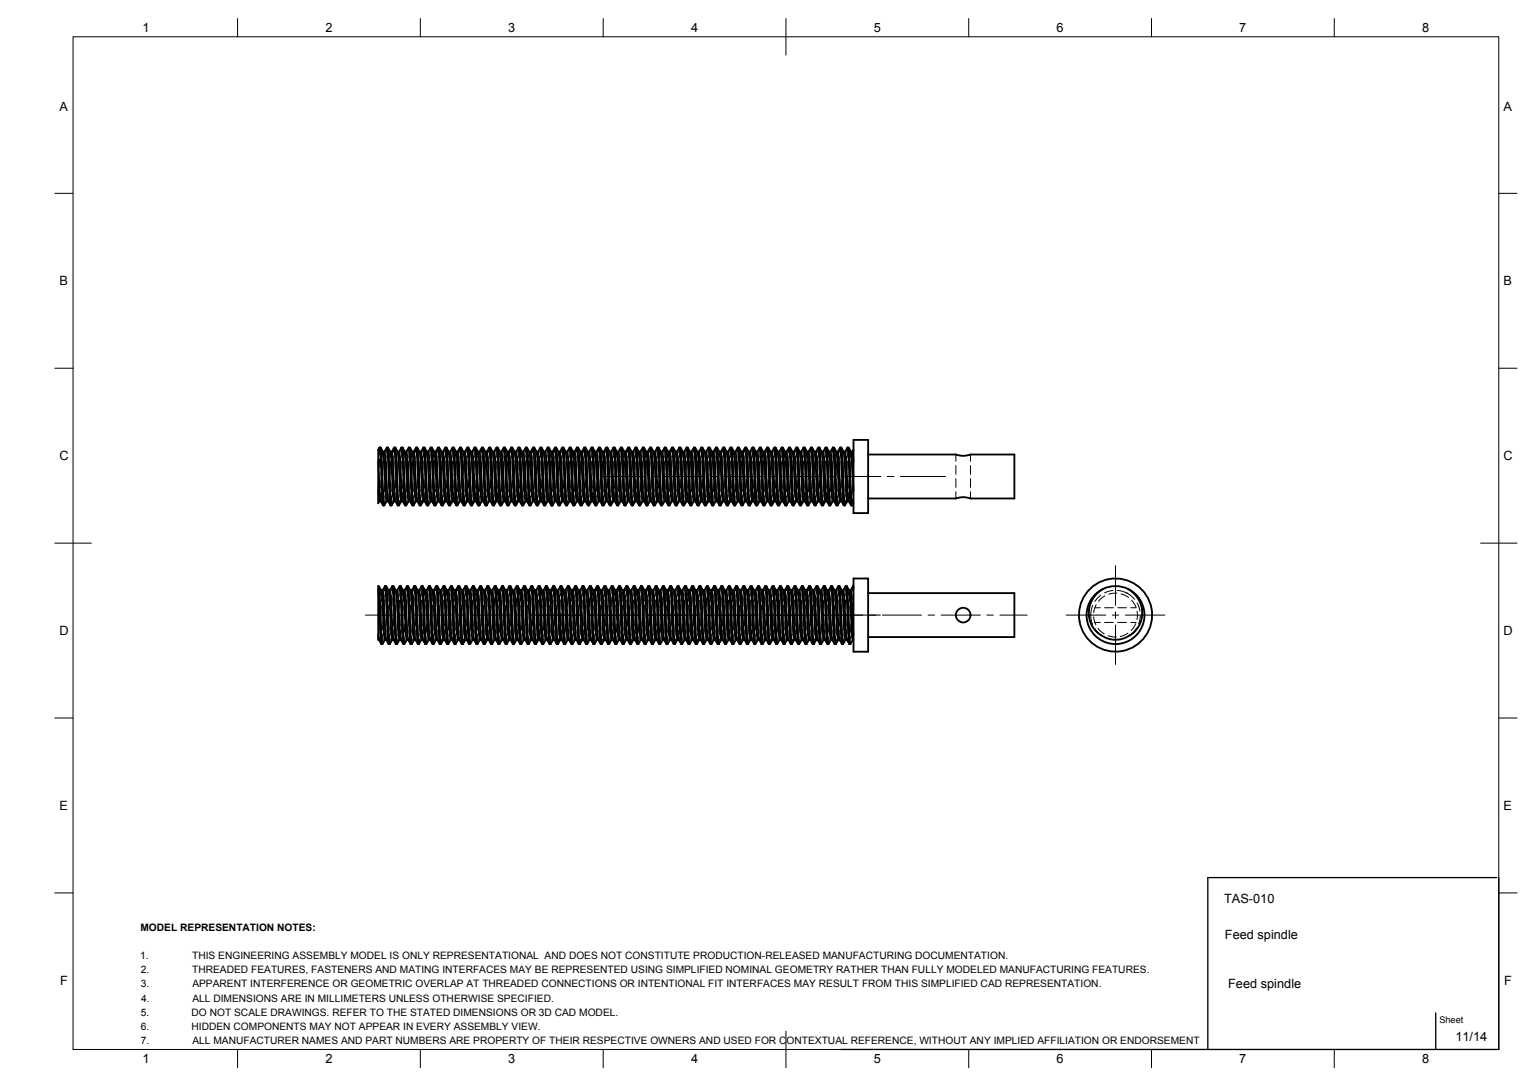
ISO-10303-21;
HEADER;
/* Generated by software containing ST-Developer
 * from STEP Tools, Inc. (www.steptools.com) 
 */

FILE_DESCRIPTION(
/* description */ (
'Independent keyed-quill tailstock, native coupled50mm slider andM16x2
 feed screw, conical dead center, bronze sleeves/thrust washers, cross
-pinned handwheel and bolted guide key. Custom center taper; no standa
rd taper compatibility, machine-bed compatibility or load rating assig
ned.'),
/* implementation_level */ '2;1');

FILE_NAME(
/* name */ 'Feed spindle.step',
/* time_stamp */ '2026-11-14T07:17:36-08:00',
/* author */ (''),
/* organization */ (''),
/* preprocessor_version */ 'ST-DEVELOPER v20.2',
/* originating_system */ 'Autodesk Translation Framework v15.17.0.0',
/* authorisation */ '');

FILE_SCHEMA (('AUTOMOTIVE_DESIGN { 1 0 10303 214 3 1 1 }'));
ENDSEC;

DATA;
#10=MECHANICAL_DESIGN_GEOMETRIC_PRESENTATION_REPRESENTATION('',(#161),#289387);
#127=SHAPE_REPRESENTATION_RELATIONSHIP('SRR','None',#289462,#144);
#144=ADVANCED_BREP_SHAPE_REPRESENTATION('',(#178),#289378);
#161=STYLED_ITEM('',(#289548),#178);
#178=MANIFOLD_SOLID_BREP('Body1',#16849);
#240=FACE_BOUND('',#1641,.T.);
#241=FACE_BOUND('',#1644,.T.);
#242=FACE_BOUND('',#1646,.T.);
#295=B_SPLINE_SURFACE_WITH_KNOTS('',3,3,((#241865,#241866,#241867,#241868,
#241869,#241870,#241871,#241872,#241873,#241874,#241875,#241876,#241877,
#241878,#241879,#241880,#241881,#241882,#241883,#241884,#241885,#241886,
#241887,#241888,#241889,#241890,#241891,#241892,#241893,#241894,#241895,
#241896,#241897,#241898,#241899,#241900,#241901,#241902,#241903,#241904,
#241905,#241906,#241907,#241908,#241909,#241910,#241911,#241912,#241913,
#241914,#241915,#241916,#241917,#241918,#241919,#241920,#241921,#241922,
#241923,#241924,#241925,#241926,#241927,#241928,#241929,#241930,#241931,
#241932,#241933,#241934,#241935,#241936,#241937,#241938,#241939,#241940,
#241941,#241942,#241943,#241944,#241945,#241946,#241947,#241948,#241949,
#241950,#241951,#241952,#241953,#241954,#241955,#241956,#241957,#241958,
#241959,#241960,#241961,#241962,#241963,#241964,#241965,#241966,#241967,
#241968,#241969,#241970,#241971,#241972,#241973,#241974,#241975,#241976,
#241977,#241978,#241979,#241980,#241981,#241982,#241983,#241984,#241985,
#241986,#241987,#241988,#241989,#241990,#241991,#241992,#241993,#241994,
#241995,#241996,#241997,#241998,#241999,#242000,#242001,#242002,#242003,
#242004,#242005,#242006,#242007,#242008,#242009,#242010,#242011,#242012,
#242013,#242014,#242015,#242016,#242017,#242018,#242019,#242020,#242021,
#242022,#242023,#242024,#242025,#242026,#242027,#242028,#242029,#242030,
#242031,#242032,#242033,#242034,#242035,#242036,#242037,#242038,#242039,
#242040,#242041,#242042,#242043,#242044,#242045,#242046,#242047,#242048,
#242049,#242050,#242051,#242052,#242053,#242054,#242055,#242056,#242057,
#242058,#242059,#242060,#242061,#242062,#242063,#242064,#242065,#242066,
#242067,#242068,#242069,#242070,#242071,#242072,#242073,#242074,#242075,
#242076,#242077,#242078,#242079,#242080,#242081,#242082,#242083,#242084,
#242085,#242086,#242087,#242088,#242089,#242090,#242091,#242092,#242093,
#242094,#242095,#242096,#242097,#242098,#242099,#242100,#242101,#242102,
#242103,#242104,#242105,#242106,#242107,#242108,#242109,#242110,#242111,
#242112,#242113,#242114,#242115,#242116,#242117,#242118,#242119,#242120,
#242121,#242122,#242123,#242124,#242125,#242126,#242127,#242128,#242129,
#242130,#242131,#242132,#242133,#242134,#242135,#242136,#242137,#242138,
#242139,#242140,#242141,#242142,#242143,#242144,#242145,#242146,#242147,
#242148,#242149,#242150,#242151,#242152,#242153,#242154,#242155,#242156,
#242157,#242158,#242159,#242160,#242161,#242162,#242163,#242164,#242165,
#242166,#242167,#242168,#242169,#242170,#242171,#242172,#242173,#242174,
#242175,#242176,#242177,#242178,#242179,#242180,#242181,#242182,#242183,
#242184,#242185,#242186,#242187,#242188,#242189,#242190,#242191,#242192,
#242193,#242194,#242195,#242196,#242197,#242198,#242199,#242200,#242201,
#242202,#242203,#242204,#242205,#242206,#242207,#242208,#242209,#242210,
#242211,#242212,#242213,#242214,#242215,#242216,#242217,#242218,#242219,
#242220,#242221,#242222,#242223,#242224,#242225,#242226,#242227,#242228,
#242229,#242230,#242231,#242232,#242233,#242234,#242235,#242236,#242237,
#242238,#242239,#242240,#242241,#242242,#242243,#242244,#242245,#242246,
#242247,#242248,#242249,#242250,#242251,#242252,#242253,#242254,#242255,
#242256,#242257,#242258,#242259,#242260,#242261,#242262,#242263,#242264,
#242265,#242266,#242267,#242268,#242269,#242270,#242271,#242272,#242273,
#242274,#242275,#242276,#242277,#242278,#242279,#242280,#242281,#242282,
#242283,#242284,#242285,#242286,#242287,#242288,#242289,#242290,#242291,
#242292,#242293,#242294,#242295,#242296,#242297,#242298,#242299,#242300,
#242301,#242302,#242303,#242304,#242305,#242306,#242307,#242308,#242309,
#242310,#242311,#242312,#242313,#242314,#242315,#242316,#242317,#242318,
#242319,#242320,#242321,#242322,#242323,#242324,#242325,#242326,#242327,
#242328,#242329,#242330,#242331,#242332,#242333,#242334,#242335,#242336,
#242337,#242338,#242339,#242340,#242341,#242342,#242343,#242344,#242345,
#242346,#242347,#242348,#242349,#242350,#242351,#242352,#242353,#242354,
#242355,#242356,#242357,#242358,#242359,#242360,#242361,#242362,#242363,
#242364,#242365,#242366,#242367,#242368,#242369,#242370,#242371,#242372,
#242373,#242374,#242375,#242376,#242377,#242378,#242379,#242380,#242381,
#242382,#242383,#242384,#242385,#242386,#242387,#242388,#242389,#242390,
#242391,#242392,#242393,#242394,#242395,#242396,#242397,#242398,#242399,
#242400,#242401,#242402,#242403,#242404,#242405,#242406,#242407,#242408,
#242409,#242410,#242411,#242412,#242413,#242414,#242415,#242416,#242417,
#242418,#242419,#242420,#242421,#242422,#242423,#242424,#242425,#242426,
#242427,#242428,#242429,#242430,#242431,#242432,#242433,#242434,#242435,
#242436,#242437,#242438,#242439,#242440,#242441,#242442,#242443,#242444,
#242445,#242446,#242447,#242448,#242449,#242450,#242451,#242452,#242453),
(#242454,#242455,#242456,#242457,#242458,#242459,#242460,#242461,#242462,
#242463,#242464,#242465,#242466,#242467,#242468,#242469,#242470,#242471,
#242472,#242473,#242474,#242475,#242476,#242477,#242478,#242479,#242480,
#242481,#242482,#242483,#242484,#242485,#242486,#242487,#242488,#242489,
#242490,#242491,#242492,#242493,#242494,#242495,#242496,#242497,#242498,
#242499,#242500,#242501,#242502,#242503,#242504,#242505,#242506,#242507,
#242508,#242509,#242510,#242511,#242512,#242513,#242514,#242515,#242516,
#242517,#242518,#242519,#242520,#242521,#242522,#242523,#242524,#242525,
#242526,#242527,#242528,#242529,#242530,#242531,#242532,#242533,#242534,
#242535,#242536,#242537,#242538,#242539,#242540,#242541,#242542,#242543,
#242544,#242545,#242546,#242547,#242548,#242549,#242550,#242551,#242552,
#242553,#242554,#242555,#242556,#242557,#242558,#242559,#242560,#242561,
#242562,#242563,#242564,#242565,#242566,#242567,#242568,#242569,#242570,
#242571,#242572,#242573,#242574,#242575,#242576,#242577,#242578,#242579,
#242580,#242581,#242582,#242583,#242584,#242585,#242586,#242587,#242588,
#242589,#242590,#242591,#242592,#242593,#242594,#242595,#242596,#242597,
#242598,#242599,#242600,#242601,#242602,#242603,#242604,#242605,#242606,
#242607,#242608,#242609,#242610,#242611,#242612,#242613,#242614,#242615,
#242616,#242617,#242618,#242619,#242620,#242621,#242622,#242623,#242624,
#242625,#242626,#242627,#242628,#242629,#242630,#242631,#242632,#242633,
#242634,#242635,#242636,#242637,#242638,#242639,#242640,#242641,#242642,
#242643,#242644,#242645,#242646,#242647,#242648,#242649,#242650,#242651,
#242652,#242653,#242654,#242655,#242656,#242657,#242658,#242659,#242660,
#242661,#242662,#242663,#242664,#242665,#242666,#242667,#242668,#242669,
#242670,#242671,#242672,#242673,#242674,#242675,#242676,#242677,#242678,
#242679,#242680,#242681,#242682,#242683,#242684,#242685,#242686,#242687,
#242688,#242689,#242690,#242691,#242692,#242693,#242694,#242695,#242696,
#242697,#242698,#242699,#242700,#242701,#242702,#242703,#242704,#242705,
#242706,#242707,#242708,#242709,#242710,#242711,#242712,#242713,#242714,
#242715,#242716,#242717,#242718,#242719,#242720,#242721,#242722,#242723,
#242724,#242725,#242726,#242727,#242728,#242729,#242730,#242731,#242732,
#242733,#242734,#242735,#242736,#242737,#242738,#242739,#242740,#242741,
#242742,#242743,#242744,#242745,#242746,#242747,#242748,#242749,#242750,
#242751,#242752,#242753,#242754,#242755,#242756,#242757,#242758,#242759,
#242760,#242761,#242762,#242763,#242764,#242765,#242766,#242767,#242768,
#242769,#242770,#242771,#242772,#242773,#242774,#242775,#242776,#242777,
#242778,#242779,#242780,#242781,#242782,#242783,#242784,#242785,#242786,
#242787,#242788,#242789,#242790,#242791,#242792,#242793,#242794,#242795,
#242796,#242797,#242798,#242799,#242800,#242801,#242802,#242803,#242804,
#242805,#242806,#242807,#242808,#242809,#242810,#242811,#242812,#242813,
#242814,#242815,#242816,#242817,#242818,#242819,#242820,#242821,#242822,
#242823,#242824,#242825,#242826,#242827,#242828,#242829,#242830,#242831,
#242832,#242833,#242834,#242835,#242836,#242837,#242838,#242839,#242840,
#242841,#242842,#242843,#242844,#242845,#242846,#242847,#242848,#242849,
#242850,#242851,#242852,#242853,#242854,#242855,#242856,#242857,#242858,
#242859,#242860,#242861,#242862,#242863,#242864,#242865,#242866,#242867,
#242868,#242869,#242870,#242871,#242872,#242873,#242874,#242875,#242876,
#242877,#242878,#242879,#242880,#242881,#242882,#242883,#242884,#242885,
#242886,#242887,#242888,#242889,#242890,#242891,#242892,#242893,#242894,
#242895,#242896,#242897,#242898,#242899,#242900,#242901,#242902,#242903,
#242904,#242905,#242906,#242907,#242908,#242909,#242910,#242911,#242912,
#242913,#242914,#242915,#242916,#242917,#242918,#242919,#242920,#242921,
#242922,#242923,#242924,#242925,#242926,#242927,#242928,#242929,#242930,
#242931,#242932,#242933,#242934,#242935,#242936,#242937,#242938,#242939,
#242940,#242941,#242942,#242943,#242944,#242945,#242946,#242947,#242948,
#242949,#242950,#242951,#242952,#242953,#242954,#242955,#242956,#242957,
#242958,#242959,#242960,#242961,#242962,#242963,#242964,#242965,#242966,
#242967,#242968,#242969,#242970,#242971,#242972,#242973,#242974,#242975,
#242976,#242977,#242978,#242979,#242980,#242981,#242982,#242983,#242984,
#242985,#242986,#242987,#242988,#242989,#242990,#242991,#242992,#242993,
#242994,#242995,#242996,#242997,#242998,#242999,#243000,#243001,#243002,
#243003,#243004,#243005,#243006,#243007,#243008,#243009,#243010,#243011,
#243012,#243013,#243014,#243015,#243016,#243017,#243018,#243019,#243020,
#243021,#243022,#243023,#243024,#243025,#243026,#243027,#243028,#243029,
#243030,#243031,#243032,#243033,#243034,#243035,#243036,#243037,#243038,
#243039,#243040,#243041,#243042),(#243043,#243044,#243045,#243046,#243047,
#243048,#243049,#243050,#243051,#243052,#243053,#243054,#243055,#243056,
#243057,#243058,#243059,#243060,#243061,#243062,#243063,#243064,#243065,
#243066,#243067,#243068,#243069,#243070,#243071,#243072,#243073,#243074,
#243075,#243076,#243077,#243078,#243079,#243080,#243081,#243082,#243083,
#243084,#243085,#243086,#243087,#243088,#243089,#243090,#243091,#243092,
#243093,#243094,#243095,#243096,#243097,#243098,#243099,#243100,#243101,
#243102,#243103,#243104,#243105,#243106,#243107,#243108,#243109,#243110,
#243111,#243112,#243113,#243114,#243115,#243116,#243117,#243118,#243119,
#243120,#243121,#243122,#243123,#243124,#243125,#243126,#243127,#243128,
#243129,#243130,#243131,#243132,#243133,#243134,#243135,#243136,#243137,
#243138,#243139,#243140,#243141,#243142,#243143,#243144,#243145,#243146,
#243147,#243148,#243149,#243150,#243151,#243152,#243153,#243154,#243155,
#243156,#243157,#243158,#243159,#243160,#243161,#243162,#243163,#243164,
#243165,#243166,#243167,#243168,#243169,#243170,#243171,#243172,#243173,
#243174,#243175,#243176,#243177,#243178,#243179,#243180,#243181,#243182,
#243183,#243184,#243185,#243186,#243187,#243188,#243189,#243190,#243191,
#243192,#243193,#243194,#243195,#243196,#243197,#243198,#243199,#243200,
#243201,#243202,#243203,#243204,#243205,#243206,#243207,#243208,#243209,
#243210,#243211,#243212,#243213,#243214,#243215,#243216,#243217,#243218,
#243219,#243220,#243221,#243222,#243223,#243224,#243225,#243226,#243227,
#243228,#243229,#243230,#243231,#243232,#243233,#243234,#243235,#243236,
#243237,#243238,#243239,#243240,#243241,#243242,#243243,#243244,#243245,
#243246,#243247,#243248,#243249,#243250,#243251,#243252,#243253,#243254,
#243255,#243256,#243257,#243258,#243259,#243260,#243261,#243262,#243263,
#243264,#243265,#243266,#243267,#243268,#243269,#243270,#243271,#243272,
#243273,#243274,#243275,#243276,#243277,#243278,#243279,#243280,#243281,
#243282,#243283,#243284,#243285,#243286,#243287,#243288,#243289,#243290,
#243291,#243292,#243293,#243294,#243295,#243296,#243297,#243298,#243299,
#243300,#243301,#243302,#243303,#243304,#243305,#243306,#243307,#243308,
#243309,#243310,#243311,#243312,#243313,#243314,#243315,#243316,#243317,
#243318,#243319,#243320,#243321,#243322,#243323,#243324,#243325,#243326,
#243327,#243328,#243329,#243330,#243331,#243332,#243333,#243334,#243335,
#243336,#243337,#243338,#243339,#243340,#243341,#243342,#243343,#243344,
#243345,#243346,#243347,#243348,#243349,#243350,#243351,#243352,#243353,
#243354,#243355,#243356,#243357,#243358,#243359,#243360,#243361,#243362,
#243363,#243364,#243365,#243366,#243367,#243368,#243369,#243370,#243371,
#243372,#243373,#243374,#243375,#243376,#243377,#243378,#243379,#243380,
#243381,#243382,#243383,#243384,#243385,#243386,#243387,#243388,#243389,
#243390,#243391,#243392,#243393,#243394,#243395,#243396,#243397,#243398,
#243399,#243400,#243401,#243402,#243403,#243404,#243405,#243406,#243407,
#243408,#243409,#243410,#243411,#243412,#243413,#243414,#243415,#243416,
#243417,#243418,#243419,#243420,#243421,#243422,#243423,#243424,#243425,
#243426,#243427,#243428,#243429,#243430,#243431,#243432,#243433,#243434,
#243435,#243436,#243437,#243438,#243439,#243440,#243441,#243442,#243443,
#243444,#243445,#243446,#243447,#243448,#243449,#243450,#243451,#243452,
#243453,#243454,#243455,#243456,#243457,#243458,#243459,#243460,#243461,
#243462,#243463,#243464,#243465,#243466,#243467,#243468,#243469,#243470,
#243471,#243472,#243473,#243474,#243475,#243476,#243477,#243478,#243479,
#243480,#243481,#243482,#243483,#243484,#243485,#243486,#243487,#243488,
#243489,#243490,#243491,#243492,#243493,#243494,#243495,#243496,#243497,
#243498,#243499,#243500,#243501,#243502,#243503,#243504,#243505,#243506,
#243507,#243508,#243509,#243510,#243511,#243512,#243513,#243514,#243515,
#243516,#243517,#243518,#243519,#243520,#243521,#243522,#243523,#243524,
#243525,#243526,#243527,#243528,#243529,#243530,#243531,#243532,#243533,
#243534,#243535,#243536,#243537,#243538,#243539,#243540,#243541,#243542,
#243543,#243544,#243545,#243546,#243547,#243548,#243549,#243550,#243551,
#243552,#243553,#243554,#243555,#243556,#243557,#243558,#243559,#243560,
#243561,#243562,#243563,#243564,#243565,#243566,#243567,#243568,#243569,
#243570,#243571,#243572,#243573,#243574,#243575,#243576,#243577,#243578,
#243579,#243580,#243581,#243582,#243583,#243584,#243585,#243586,#243587,
#243588,#243589,#243590,#243591,#243592,#243593,#243594,#243595,#243596,
#243597,#243598,#243599,#243600,#243601,#243602,#243603,#243604,#243605,
#243606,#243607,#243608,#243609,#243610,#243611,#243612,#243613,#243614,
#243615,#243616,#243617,#243618,#243619,#243620,#243621,#243622,#243623,
#243624,#243625,#243626,#243627,#243628,#243629,#243630,#243631),(#243632,
#243633,#243634,#243635,#243636,#243637,#243638,#243639,#243640,#243641,
#243642,#243643,#243644,#243645,#243646,#243647,#243648,#243649,#243650,
#243651,#243652,#243653,#243654,#243655,#243656,#243657,#243658,#243659,
#243660,#243661,#243662,#243663,#243664,#243665,#243666,#243667,#243668,
#243669,#243670,#243671,#243672,#243673,#243674,#243675,#243676,#243677,
#243678,#243679,#243680,#243681,#243682,#243683,#243684,#243685,#243686,
#243687,#243688,#243689,#243690,#243691,#243692,#243693,#243694,#243695,
#243696,#243697,#243698,#243699,#243700,#243701,#243702,#243703,#243704,
#243705,#243706,#243707,#243708,#243709,#243710,#243711,#243712,#243713,
#243714,#243715,#243716,#243717,#243718,#243719,#243720,#243721,#243722,
#243723,#243724,#243725,#243726,#243727,#243728,#243729,#243730,#243731,
#243732,#243733,#243734,#243735,#243736,#243737,#243738,#243739,#243740,
#243741,#243742,#243743,#243744,#243745,#243746,#243747,#243748,#243749,
#243750,#243751,#243752,#243753,#243754,#243755,#243756,#243757,#243758,
#243759,#243760,#243761,#243762,#243763,#243764,#243765,#243766,#243767,
#243768,#243769,#243770,#243771,#243772,#243773,#243774,#243775,#243776,
#243777,#243778,#243779,#243780,#243781,#243782,#243783,#243784,#243785,
#243786,#243787,#243788,#243789,#243790,#243791,#243792,#243793,#243794,
#243795,#243796,#243797,#243798,#243799,#243800,#243801,#243802,#243803,
#243804,#243805,#243806,#243807,#243808,#243809,#243810,#243811,#243812,
#243813,#243814,#243815,#243816,#243817,#243818,#243819,#243820,#243821,
#243822,#243823,#243824,#243825,#243826,#243827,#243828,#243829,#243830,
#243831,#243832,#243833,#243834,#243835,#243836,#243837,#243838,#243839,
#243840,#243841,#243842,#243843,#243844,#243845,#243846,#243847,#243848,
#243849,#243850,#243851,#243852,#243853,#243854,#243855,#243856,#243857,
#243858,#243859,#243860,#243861,#243862,#243863,#243864,#243865,#243866,
#243867,#243868,#243869,#243870,#243871,#243872,#243873,#243874,#243875,
#243876,#243877,#243878,#243879,#243880,#243881,#243882,#243883,#243884,
#243885,#243886,#243887,#243888,#243889,#243890,#243891,#243892,#243893,
#243894,#243895,#243896,#243897,#243898,#243899,#243900,#243901,#243902,
#243903,#243904,#243905,#243906,#243907,#243908,#243909,#243910,#243911,
#243912,#243913,#243914,#243915,#243916,#243917,#243918,#243919,#243920,
#243921,#243922,#243923,#243924,#243925,#243926,#243927,#243928,#243929,
#243930,#243931,#243932,#243933,#243934,#243935,#243936,#243937,#243938,
#243939,#243940,#243941,#243942,#243943,#243944,#243945,#243946,#243947,
#243948,#243949,#243950,#243951,#243952,#243953,#243954,#243955,#243956,
#243957,#243958,#243959,#243960,#243961,#243962,#243963,#243964,#243965,
#243966,#243967,#243968,#243969,#243970,#243971,#243972,#243973,#243974,
#243975,#243976,#243977,#243978,#243979,#243980,#243981,#243982,#243983,
#243984,#243985,#243986,#243987,#243988,#243989,#243990,#243991,#243992,
#243993,#243994,#243995,#243996,#243997,#243998,#243999,#244000,#244001,
#244002,#244003,#244004,#244005,#244006,#244007,#244008,#244009,#244010,
#244011,#244012,#244013,#244014,#244015,#244016,#244017,#244018,#244019,
#244020,#244021,#244022,#244023,#244024,#244025,#244026,#244027,#244028,
#244029,#244030,#244031,#244032,#244033,#244034,#244035,#244036,#244037,
#244038,#244039,#244040,#244041,#244042,#244043,#244044,#244045,#244046,
#244047,#244048,#244049,#244050,#244051,#244052,#244053,#244054,#244055,
#244056,#244057,#244058,#244059,#244060,#244061,#244062,#244063,#244064,
#244065,#244066,#244067,#244068,#244069,#244070,#244071,#244072,#244073,
#244074,#244075,#244076,#244077,#244078,#244079,#244080,#244081,#244082,
#244083,#244084,#244085,#244086,#244087,#244088,#244089,#244090,#244091,
#244092,#244093,#244094,#244095,#244096,#244097,#244098,#244099,#244100,
#244101,#244102,#244103,#244104,#244105,#244106,#244107,#244108,#244109,
#244110,#244111,#244112,#244113,#244114,#244115,#244116,#244117,#244118,
#244119,#244120,#244121,#244122,#244123,#244124,#244125,#244126,#244127,
#244128,#244129,#244130,#244131,#244132,#244133,#244134,#244135,#244136,
#244137,#244138,#244139,#244140,#244141,#244142,#244143,#244144,#244145,
#244146,#244147,#244148,#244149,#244150,#244151,#244152,#244153,#244154,
#244155,#244156,#244157,#244158,#244159,#244160,#244161,#244162,#244163,
#244164,#244165,#244166,#244167,#244168,#244169,#244170,#244171,#244172,
#244173,#244174,#244175,#244176,#244177,#244178,#244179,#244180,#244181,
#244182,#244183,#244184,#244185,#244186,#244187,#244188,#244189,#244190,
#244191,#244192,#244193,#244194,#244195,#244196,#244197,#244198,#244199,
#244200,#244201,#244202,#244203,#244204,#244205,#244206,#244207,#244208,
#244209,#244210,#244211,#244212,#244213,#244214,#244215,#244216,#244217,
#244218,#244219,#244220)),.UNSPECIFIED.,.F.,.F.,.F.,(4,4),(4,1,1,1,1,1,
1,1,1,1,1,1,1,1,1,1,1,1,1,1,1,1,1,1,1,1,1,1,1,1,1,1,1,1,1,1,1,1,1,1,1,1,
1,1,1,1,1,1,1,1,1,1,1,1,1,1,1,1,1,1,1,1,1,1,1,1,1,1,1,1,1,1,1,1,1,1,1,1,
1,1,1,1,1,1,1,1,1,1,1,1,1,1,1,1,1,1,1,1,1,1,1,1,1,1,1,1,1,1,1,1,1,1,1,1,
1,1,1,1,1,1,1,1,1,1,1,1,1,1,1,1,1,1,1,1,1,1,1,1,1,1,1,1,1,1,1,1,1,1,1,1,
1,1,1,1,1,1,1,1,1,1,1,1,1,1,1,1,1,1,1,1,1,1,1,1,1,1,1,1,1,1,1,1,1,1,1,1,
1,1,1,1,1,1,1,1,1,1,1,1,1,1,1,1,1,1,1,1,1,1,1,1,1,1,1,1,1,1,1,1,1,1,1,1,
1,1,1,1,1,1,1,1,1,1,1,1,1,1,1,1,1,1,1,1,1,1,1,1,1,1,1,1,1,1,1,1,1,1,1,1,
1,1,1,1,1,1,1,1,1,1,1,1,1,1,1,1,1,1,1,1,1,1,1,1,1,1,1,1,1,1,1,1,1,1,1,1,
1,1,1,1,1,1,1,1,1,1,1,1,1,1,1,1,1,1,1,1,1,1,1,1,1,1,1,1,1,1,1,1,1,1,1,1,
1,1,1,1,1,1,1,1,1,1,1,1,1,1,1,1,1,1,1,1,1,1,1,1,1,1,1,1,1,1,1,1,1,1,1,1,
1,1,1,1,1,1,1,1,1,1,1,1,1,1,1,1,1,1,1,1,1,1,1,1,1,1,1,1,1,1,1,1,1,1,1,1,
1,1,1,1,1,1,1,1,1,1,1,1,1,1,1,1,1,1,1,1,1,1,1,1,1,1,1,1,1,1,1,1,1,1,1,1,
1,1,1,1,1,1,1,1,1,1,1,1,1,1,1,1,1,1,1,1,1,1,1,1,1,1,1,1,1,1,1,1,1,1,1,1,
1,1,1,1,1,1,1,1,1,1,1,1,1,1,1,1,1,1,1,1,1,1,1,1,1,1,1,1,1,1,1,1,1,1,1,1,
1,1,1,1,1,1,1,1,1,1,1,1,1,1,1,1,1,1,1,1,1,1,1,1,1,1,1,1,1,1,1,1,1,1,1,1,
1,1,1,1,1,1,1,1,1,1,1,1,1,1,1,1,1,1,1,1,1,1,1,1,1,1,1,1,1,1,1,1,1,1,1,1,
1,1,1,1,4),(-0.000839536803422264,0.135425581403526),(8.30104296596843,
8.80049912255811,9.2998689904892,9.79923885842029,10.2986087263514,11.2973484622136,
12.2960881980758,13.2948279339379,13.794197801869,14.2935676698001,14.7929375377312,
15.2923074056623,16.2910471415245,16.7904170094556,17.2897868773867,18.2885266132489,
19.287266349111,20.2860060849732,20.7853759529043,21.2847458208354,21.7841156887665,
22.2834855566976,23.2822252925598,23.7815951604909,24.280965028422,25.2797047642841,
26.2784445001463,27.2771842360085,27.7765541039396,28.2759239718707,28.7752938398018,
29.2746637077329,30.2734034435951,30.7727733115261,31.2721431794572,32.2708829153194,
33.2696226511816,34.2683623870438,34.7677322549749,35.267102122906,35.7664719908371,
36.2658418587681,37.2645815946303,37.7639514625614,38.2633213304925,39.2620610663547,
40.2608008022169,41.2595405380791,41.7589104060102,42.2582802739413,42.7576501418723,
43.2570200098034,44.2557597456656,44.7551296135967,45.2544994815278,46.25323921739,
47.2519789532522,48.2507186891144,48.7500885570454,49.2494584249765,49.7488282929076,
50.2481981608387,51.2469378967009,51.746307764632,52.2456776325631,53.2444173684253,
54.2431571042874,55.2418968401496,55.7412667080807,56.2406365760118,56.7400064439429,
57.239376311874,58.2381160477362,58.7374859156673,59.2368557835984,60.2355955194606,
61.2343352553227,62.2330749911849,62.732444859116,63.2318147270471,63.7311845949782,
64.2305544629093,65.2292941987715,65.7286640667025,66.2280339346336,67.2267736704958,
68.225513406358,69.2242531422202,69.7236230101513,70.2229928780824,70.7223627460135,
71.2217326139446,72.2204723498067,72.7198422177378,73.2192120856689,74.2179518215311,
75.2166915573933,76.2154312932555,76.7148011611866,77.2141710291177,77.7135408970487,
78.2129107649798,79.211650500842,79.7110203687731,80.2103902367042,81.2091299725664,
82.2078697084286,83.2066094442908,83.7059793122218,84.2053491801529,84.704719048084,
85.2040889160151,86.2028286518773,86.7021985198084,87.2015683877395,88.2003081236017,
89.1990478594639,90.197787595326,90.6971574632571,91.1965273311882,91.6958971991193,
92.1952670670504,93.1940068029126,93.6933766708437,94.1927465387748,95.191486274637,
96.1902260104991,97.1889657463613,97.6883356142924,98.1877054822235,98.6870753501546,
99.1864452180857,100.185184953948,100.684554821879,101.18392468981,102.182664425672,
103.181404161534,104.180143897397,104.679513765328,105.178883633259,105.67825350119,
106.177623369121,107.176363104983,107.675732972914,108.175102840845,109.173842576708,
110.17258231257,111.171322048432,111.670691916363,112.170061784294,112.669431652225,
113.168801520156,114.167541256018,114.66691112395,115.166280991881,116.165020727743,
117.163760463605,118.162500199467,118.661870067398,119.161239935329,119.66060980326,
120.159979671192,121.158719407054,121.658089274985,122.157459142916,123.156198878778,
124.15493861464,125.153678350502,125.653048218434,126.152418086365,126.651787954296,
127.151157822227,128.149897558089,128.64926742602,129.148637293951,130.147377029813,
131.146116765676,132.144856501538,132.644226369469,133.1435962374,133.642966105331,
134.142335973262,135.141075709124,135.640445577055,136.139815444986,137.138555180849,
138.137294916711,139.136034652573,139.635404520504,140.134774388435,140.634144256366,
141.133514124297,142.13225386016,142.631623728091,143.130993596022,144.129733331884,
145.128473067746,146.127212803608,146.626582671539,147.12595253947,147.625322407402,
148.124692275333,149.123432011195,149.622801879126,150.122171747057,151.120911482919,
152.119651218781,153.118390954644,153.617760822575,154.117130690506,154.616500558437,
155.115870426368,156.11461016223,156.613980030161,157.113349898092,158.112089633955,
159.110829369817,160.109569105679,160.60893897361,161.108308841541,161.607678709472,
162.107048577403,163.105788313265,163.605158181197,164.104528049128,165.10326778499,
166.102007520852,167.100747256714,167.600117124645,168.099486992576,168.598856860507,
169.098226728439,170.096966464301,170.596336332232,171.095706200163,172.094445936025,
173.093185671887,174.091925407749,174.591295275681,175.090665143612,175.590035011543,
176.089404879474,177.088144615336,177.587514483267,178.086884351198,179.08562408706,
180.084363822923,181.083103558785,181.582473426716,182.081843294647,182.581213162578,
183.080583030509,184.079322766371,184.578692634302,185.078062502233,186.076802238096,
187.075541973958,188.07428170982,188.573651577751,189.073021445682,189.572391313613,
190.071761181544,191.070500917407,191.569870785338,192.069240653269,193.067980389131,
194.066720124993,195.065459860855,195.564829728786,196.064199596717,196.563569464649,
197.06293933258,198.061679068442,198.561048936373,199.060418804304,200.059158540166,
201.057898276028,202.056638011891,202.556007879822,203.055377747753,203.554747615684,
204.054117483615,205.052857219477,205.552227087408,206.051596955339,207.050336691201,
208.049076427064,209.047816162926,209.547186030857,210.046555898788,210.545925766719,
211.04529563465,212.044035370512,212.543405238443,213.042775106375,214.041514842237,
215.040254578099,216.038994313961,217.037734049823,218.036473785686,219.035213521548,
220.03395325741,221.032692993272,221.532062861203,222.031432729134,223.030172464996,
223.529542332928,224.028912200859,224.52828206879,225.027651936721,226.026391672583,
227.025131408445,228.023871144307,228.523241012238,229.02261088017,230.021350616032,
230.520720483963,231.020090351894,231.519460219825,232.018830087756,233.017569823618,
234.01630955948,235.015049295343,235.514419163274,236.013789031205,237.012528767067,
237.511898634998,238.011268502929,238.51063837086,239.010008238791,240.008747974654,
241.007487710516,242.006227446378,242.505597314309,243.00496718224,244.003706918102,
244.503076786033,245.002446653964,245.501816521896,246.001186389827,246.999926125689,
247.998665861551,248.997405597413,249.496775465344,249.996145333275,250.994885069138,
251.494254937069,251.993624805,252.492994672931,252.992364540862,253.991104276724,
254.989844012586,255.988583748448,256.48795361638,256.987323484311,257.986063220173,
258.485433088104,258.984802956035,259.484172823966,259.983542691897,260.982282427759,
261.981022163622,262.979761899484,263.479131767415,263.978501635346,264.977241371208,
265.476611239139,265.97598110707,266.475350975001,266.974720842932,267.973460578795,
268.972200314657,269.970940050519,270.47030991845,270.969679786381,271.968419522243,
272.467789390175,272.967159258106,273.466529126037,273.965898993968,274.96463872983,
275.963378465692,276.962118201554,277.461488069485,277.960857937417,278.959597673279,
279.45896754121,279.958337409141,280.457707277072,280.957077145003,281.955816880865,
282.954556616727,283.95329635259,284.452666220521,284.952036088452,285.950775824314,
286.450145692245,286.949515560176,287.448885428107,287.948255296038,288.946995031901,
289.945734767763,290.944474503625,291.443844371556,291.943214239487,292.941953975349,
293.44132384328,293.940693711211,294.440063579143,294.939433447074,295.938173182936,
296.936912918798,297.93565265466,298.435022522591,298.934392390522,299.933132126385,
300.432501994316,300.931871862247,301.431241730178,301.930611598109,302.929351333971,
303.928091069833,304.926830805695,305.426200673627,305.925570541558,306.92431027742,
307.423680145351,307.923050013282,308.422419881213,308.921789749144,309.920529485006,
310.919269220869,311.918008956731,312.417378824662,312.916748692593,313.915488428455,
314.414858296386,314.914228164317,315.413598032248,315.912967900179,316.911707636042,
317.910447371904,318.909187107766,319.408556975697,319.907926843628,320.90666657949,
321.406036447421,321.905406315353,322.404776183284,322.904146051215,323.902885787077,
324.901625522939,325.900365258801,326.399735126732,326.899104994664,327.897844730526,
328.397214598457,328.896584466388,329.395954334319,329.89532420225,330.894063938112,
331.892803673974,332.891543409837,333.390913277768,333.890283145699,334.889022881561,
335.388392749492,335.887762617423,336.387132485354,336.886502353285,337.885242089147,
338.88398182501,339.882721560872,340.382091428803,340.881461296734,341.880201032596,
342.379570900527,342.878940768458,343.37831063639,343.877680504321,344.876420240183,
345.875159976045,346.873899711907,347.373269579838,347.872639447769,348.871379183632,
349.370749051563,349.870118919494,350.369488787425,350.868858655356,351.867598391218,
352.86633812708,353.865077862942,354.364447730874,354.863817598805,355.862557334667,
356.361927202598,356.861297070529,357.36066693846,357.860036806391,358.858776542253,
359.857516278115,360.856256013978,361.355625881909,361.85499574984,362.853735485702,
363.353105353633,363.852475221564,364.351845089495,364.851214957426,365.849954693289,
366.848694429151,367.847434165013,368.346804032944,368.846173900875,369.844913636737,
370.344283504668,370.8436533726,371.343023240531,371.842393108462,372.841132844324,
373.839872580186,374.838612316048,375.337982183979,375.83735205191,376.836091787773,
377.335461655704,377.834831523635,378.334201391566,378.833571259497,379.832310995359,
380.831050731221,381.829790467084,382.329160335015,382.828530202946,383.827269938808,
384.326639806739,384.82600967467,385.325379542601,385.824749410532,386.823489146394,
387.822228882257,388.820968618119,389.32033848605,389.819708353981,390.818448089843,
391.317817957774,391.817187825705,392.316557693636,392.815927561568,393.81466729743,
394.813407033292,395.812146769154,396.311516637085,396.810886505016,397.809626240879,
398.30899610881,398.808365976741,399.307735844672,399.807105712603,400.805845448465,
401.804585184327,402.803324920189,403.302694788121,403.802064656052,404.800804391914,
405.300174259845,405.799544127776,406.298913995707,406.798283863638,407.7970235995,
408.795763335362,409.794503071225,410.293872939156,410.793242807087,411.791982542949,
412.29135241088,412.790722278811,413.290092146742,413.789462014673,414.788201750536,
415.786941486398,416.78568122226,417.285051090191,417.784420958122,418.283790826053,
418.783223976954),.UNSPECIFIED.);
#296=B_SPLINE_SURFACE_WITH_KNOTS('',3,3,((#244442,#244443,#244444,#244445,
#244446,#244447,#244448,#244449,#244450,#244451,#244452,#244453,#244454,
#244455,#244456,#244457,#244458,#244459,#244460,#244461,#244462,#244463,
#244464,#244465,#244466,#244467,#244468,#244469,#244470,#244471,#244472,
#244473,#244474,#244475,#244476,#244477,#244478,#244479,#244480,#244481,
#244482,#244483,#244484,#244485,#244486,#244487,#244488,#244489,#244490,
#244491,#244492,#244493,#244494,#244495,#244496,#244497,#244498,#244499,
#244500,#244501,#244502,#244503,#244504,#244505,#244506,#244507,#244508,
#244509,#244510,#244511,#244512,#244513,#244514,#244515,#244516,#244517,
#244518,#244519,#244520,#244521,#244522,#244523,#244524,#244525,#244526,
#244527,#244528,#244529,#244530,#244531,#244532,#244533,#244534,#244535,
#244536,#244537,#244538,#244539,#244540,#244541,#244542,#244543,#244544,
#244545,#244546,#244547,#244548,#244549,#244550,#244551,#244552,#244553,
#244554,#244555,#244556,#244557,#244558,#244559,#244560,#244561,#244562,
#244563,#244564,#244565,#244566,#244567,#244568,#244569,#244570,#244571,
#244572,#244573,#244574,#244575,#244576,#244577,#244578,#244579,#244580,
#244581,#244582,#244583,#244584,#244585,#244586,#244587,#244588,#244589,
#244590,#244591,#244592,#244593,#244594,#244595,#244596,#244597,#244598,
#244599,#244600,#244601,#244602,#244603,#244604,#244605,#244606,#244607,
#244608,#244609,#244610,#244611,#244612,#244613,#244614,#244615,#244616,
#244617,#244618,#244619,#244620,#244621,#244622,#244623,#244624,#244625,
#244626,#244627,#244628,#244629,#244630,#244631,#244632,#244633,#244634,
#244635,#244636,#244637,#244638,#244639,#244640,#244641,#244642,#244643,
#244644,#244645,#244646,#244647,#244648,#244649,#244650,#244651,#244652,
#244653,#244654,#244655,#244656,#244657,#244658,#244659,#244660,#244661,
#244662,#244663,#244664,#244665,#244666,#244667,#244668,#244669,#244670,
#244671,#244672,#244673,#244674,#244675,#244676,#244677,#244678,#244679,
#244680,#244681,#244682,#244683,#244684,#244685,#244686,#244687,#244688,
#244689,#244690,#244691,#244692,#244693,#244694,#244695,#244696,#244697,
#244698,#244699,#244700,#244701,#244702,#244703,#244704,#244705,#244706,
#244707,#244708,#244709,#244710,#244711,#244712,#244713,#244714,#244715,
#244716,#244717,#244718,#244719,#244720,#244721,#244722,#244723,#244724,
#244725,#244726,#244727,#244728,#244729,#244730,#244731,#244732,#244733,
#244734,#244735,#244736,#244737,#244738,#244739,#244740,#244741,#244742,
#244743,#244744,#244745,#244746,#244747,#244748,#244749,#244750,#244751,
#244752,#244753,#244754,#244755,#244756,#244757,#244758,#244759,#244760,
#244761,#244762,#244763,#244764,#244765,#244766,#244767,#244768,#244769,
#244770,#244771,#244772,#244773,#244774,#244775,#244776,#244777,#244778,
#244779,#244780,#244781,#244782,#244783,#244784,#244785,#244786,#244787,
#244788,#244789,#244790,#244791,#244792,#244793,#244794,#244795,#244796,
#244797,#244798,#244799,#244800,#244801,#244802,#244803,#244804,#244805,
#244806,#244807,#244808,#244809,#244810,#244811,#244812,#244813,#244814,
#244815,#244816,#244817,#244818,#244819,#244820,#244821,#244822,#244823,
#244824,#244825,#244826,#244827,#244828,#244829,#244830,#244831,#244832,
#244833,#244834,#244835,#244836,#244837,#244838,#244839,#244840,#244841,
#244842,#244843,#244844,#244845,#244846,#244847,#244848,#244849,#244850,
#244851,#244852,#244853,#244854,#244855,#244856,#244857,#244858,#244859,
#244860,#244861,#244862,#244863,#244864,#244865,#244866,#244867,#244868,
#244869,#244870,#244871,#244872,#244873,#244874,#244875,#244876,#244877,
#244878,#244879,#244880,#244881,#244882,#244883,#244884,#244885,#244886,
#244887,#244888,#244889,#244890,#244891,#244892,#244893,#244894,#244895,
#244896,#244897,#244898,#244899,#244900,#244901,#244902,#244903,#244904,
#244905,#244906,#244907,#244908,#244909,#244910,#244911,#244912,#244913,
#244914,#244915,#244916,#244917,#244918,#244919,#244920,#244921,#244922,
#244923,#244924,#244925,#244926,#244927,#244928,#244929,#244930,#244931,
#244932,#244933,#244934,#244935,#244936,#244937,#244938,#244939,#244940,
#244941,#244942,#244943,#244944,#244945,#244946,#244947,#244948,#244949,
#244950,#244951,#244952,#244953,#244954,#244955,#244956,#244957,#244958,
#244959,#244960,#244961,#244962,#244963,#244964,#244965,#244966,#244967,
#244968,#244969,#244970,#244971,#244972,#244973,#244974,#244975,#244976,
#244977,#244978,#244979,#244980,#244981,#244982,#244983,#244984,#244985,
#244986,#244987,#244988,#244989,#244990,#244991,#244992,#244993,#244994,
#244995,#244996,#244997,#244998,#244999,#245000,#245001,#245002,#245003,
#245004,#245005,#245006,#245007,#245008,#245009,#245010,#245011,#245012,
#245013,#245014,#245015,#245016,#245017,#245018,#245019,#245020,#245021,
#245022,#245023,#245024,#245025,#245026,#245027,#245028,#245029,#245030),
(#245031,#245032,#245033,#245034,#245035,#245036,#245037,#245038,#245039,
#245040,#245041,#245042,#245043,#245044,#245045,#245046,#245047,#245048,
#245049,#245050,#245051,#245052,#245053,#245054,#245055,#245056,#245057,
#245058,#245059,#245060,#245061,#245062,#245063,#245064,#245065,#245066,
#245067,#245068,#245069,#245070,#245071,#245072,#245073,#245074,#245075,
#245076,#245077,#245078,#245079,#245080,#245081,#245082,#245083,#245084,
#245085,#245086,#245087,#245088,#245089,#245090,#245091,#245092,#245093,
#245094,#245095,#245096,#245097,#245098,#245099,#245100,#245101,#245102,
#245103,#245104,#245105,#245106,#245107,#245108,#245109,#245110,#245111,
#245112,#245113,#245114,#245115,#245116,#245117,#245118,#245119,#245120,
#245121,#245122,#245123,#245124,#245125,#245126,#245127,#245128,#245129,
#245130,#245131,#245132,#245133,#245134,#245135,#245136,#245137,#245138,
#245139,#245140,#245141,#245142,#245143,#245144,#245145,#245146,#245147,
#245148,#245149,#245150,#245151,#245152,#245153,#245154,#245155,#245156,
#245157,#245158,#245159,#245160,#245161,#245162,#245163,#245164,#245165,
#245166,#245167,#245168,#245169,#245170,#245171,#245172,#245173,#245174,
#245175,#245176,#245177,#245178,#245179,#245180,#245181,#245182,#245183,
#245184,#245185,#245186,#245187,#245188,#245189,#245190,#245191,#245192,
#245193,#245194,#245195,#245196,#245197,#245198,#245199,#245200,#245201,
#245202,#245203,#245204,#245205,#245206,#245207,#245208,#245209,#245210,
#245211,#245212,#245213,#245214,#245215,#245216,#245217,#245218,#245219,
#245220,#245221,#245222,#245223,#245224,#245225,#245226,#245227,#245228,
#245229,#245230,#245231,#245232,#245233,#245234,#245235,#245236,#245237,
#245238,#245239,#245240,#245241,#245242,#245243,#245244,#245245,#245246,
#245247,#245248,#245249,#245250,#245251,#245252,#245253,#245254,#245255,
#245256,#245257,#245258,#245259,#245260,#245261,#245262,#245263,#245264,
#245265,#245266,#245267,#245268,#245269,#245270,#245271,#245272,#245273,
#245274,#245275,#245276,#245277,#245278,#245279,#245280,#245281,#245282,
#245283,#245284,#245285,#245286,#245287,#245288,#245289,#245290,#245291,
#245292,#245293,#245294,#245295,#245296,#245297,#245298,#245299,#245300,
#245301,#245302,#245303,#245304,#245305,#245306,#245307,#245308,#245309,
#245310,#245311,#245312,#245313,#245314,#245315,#245316,#245317,#245318,
#245319,#245320,#245321,#245322,#245323,#245324,#245325,#245326,#245327,
#245328,#245329,#245330,#245331,#245332,#245333,#245334,#245335,#245336,
#245337,#245338,#245339,#245340,#245341,#245342,#245343,#245344,#245345,
#245346,#245347,#245348,#245349,#245350,#245351,#245352,#245353,#245354,
#245355,#245356,#245357,#245358,#245359,#245360,#245361,#245362,#245363,
#245364,#245365,#245366,#245367,#245368,#245369,#245370,#245371,#245372,
#245373,#245374,#245375,#245376,#245377,#245378,#245379,#245380,#245381,
#245382,#245383,#245384,#245385,#245386,#245387,#245388,#245389,#245390,
#245391,#245392,#245393,#245394,#245395,#245396,#245397,#245398,#245399,
#245400,#245401,#245402,#245403,#245404,#245405,#245406,#245407,#245408,
#245409,#245410,#245411,#245412,#245413,#245414,#245415,#245416,#245417,
#245418,#245419,#245420,#245421,#245422,#245423,#245424,#245425,#245426,
#245427,#245428,#245429,#245430,#245431,#245432,#245433,#245434,#245435,
#245436,#245437,#245438,#245439,#245440,#245441,#245442,#245443,#245444,
#245445,#245446,#245447,#245448,#245449,#245450,#245451,#245452,#245453,
#245454,#245455,#245456,#245457,#245458,#245459,#245460,#245461,#245462,
#245463,#245464,#245465,#245466,#245467,#245468,#245469,#245470,#245471,
#245472,#245473,#245474,#245475,#245476,#245477,#245478,#245479,#245480,
#245481,#245482,#245483,#245484,#245485,#245486,#245487,#245488,#245489,
#245490,#245491,#245492,#245493,#245494,#245495,#245496,#245497,#245498,
#245499,#245500,#245501,#245502,#245503,#245504,#245505,#245506,#245507,
#245508,#245509,#245510,#245511,#245512,#245513,#245514,#245515,#245516,
#245517,#245518,#245519,#245520,#245521,#245522,#245523,#245524,#245525,
#245526,#245527,#245528,#245529,#245530,#245531,#245532,#245533,#245534,
#245535,#245536,#245537,#245538,#245539,#245540,#245541,#245542,#245543,
#245544,#245545,#245546,#245547,#245548,#245549,#245550,#245551,#245552,
#245553,#245554,#245555,#245556,#245557,#245558,#245559,#245560,#245561,
#245562,#245563,#245564,#245565,#245566,#245567,#245568,#245569,#245570,
#245571,#245572,#245573,#245574,#245575,#245576,#245577,#245578,#245579,
#245580,#245581,#245582,#245583,#245584,#245585,#245586,#245587,#245588,
#245589,#245590,#245591,#245592,#245593,#245594,#245595,#245596,#245597,
#245598,#245599,#245600,#245601,#245602,#245603,#245604,#245605,#245606,
#245607,#245608,#245609,#245610,#245611,#245612,#245613,#245614,#245615,
#245616,#245617,#245618,#245619),(#245620,#245621,#245622,#245623,#245624,
#245625,#245626,#245627,#245628,#245629,#245630,#245631,#245632,#245633,
#245634,#245635,#245636,#245637,#245638,#245639,#245640,#245641,#245642,
#245643,#245644,#245645,#245646,#245647,#245648,#245649,#245650,#245651,
#245652,#245653,#245654,#245655,#245656,#245657,#245658,#245659,#245660,
#245661,#245662,#245663,#245664,#245665,#245666,#245667,#245668,#245669,
#245670,#245671,#245672,#245673,#245674,#245675,#245676,#245677,#245678,
#245679,#245680,#245681,#245682,#245683,#245684,#245685,#245686,#245687,
#245688,#245689,#245690,#245691,#245692,#245693,#245694,#245695,#245696,
#245697,#245698,#245699,#245700,#245701,#245702,#245703,#245704,#245705,
#245706,#245707,#245708,#245709,#245710,#245711,#245712,#245713,#245714,
#245715,#245716,#245717,#245718,#245719,#245720,#245721,#245722,#245723,
#245724,#245725,#245726,#245727,#245728,#245729,#245730,#245731,#245732,
#245733,#245734,#245735,#245736,#245737,#245738,#245739,#245740,#245741,
#245742,#245743,#245744,#245745,#245746,#245747,#245748,#245749,#245750,
#245751,#245752,#245753,#245754,#245755,#245756,#245757,#245758,#245759,
#245760,#245761,#245762,#245763,#245764,#245765,#245766,#245767,#245768,
#245769,#245770,#245771,#245772,#245773,#245774,#245775,#245776,#245777,
#245778,#245779,#245780,#245781,#245782,#245783,#245784,#245785,#245786,
#245787,#245788,#245789,#245790,#245791,#245792,#245793,#245794,#245795,
#245796,#245797,#245798,#245799,#245800,#245801,#245802,#245803,#245804,
#245805,#245806,#245807,#245808,#245809,#245810,#245811,#245812,#245813,
#245814,#245815,#245816,#245817,#245818,#245819,#245820,#245821,#245822,
#245823,#245824,#245825,#245826,#245827,#245828,#245829,#245830,#245831,
#245832,#245833,#245834,#245835,#245836,#245837,#245838,#245839,#245840,
#245841,#245842,#245843,#245844,#245845,#245846,#245847,#245848,#245849,
#245850,#245851,#245852,#245853,#245854,#245855,#245856,#245857,#245858,
#245859,#245860,#245861,#245862,#245863,#245864,#245865,#245866,#245867,
#245868,#245869,#245870,#245871,#245872,#245873,#245874,#245875,#245876,
#245877,#245878,#245879,#245880,#245881,#245882,#245883,#245884,#245885,
#245886,#245887,#245888,#245889,#245890,#245891,#245892,#245893,#245894,
#245895,#245896,#245897,#245898,#245899,#245900,#245901,#245902,#245903,
#245904,#245905,#245906,#245907,#245908,#245909,#245910,#245911,#245912,
#245913,#245914,#245915,#245916,#245917,#245918,#245919,#245920,#245921,
#245922,#245923,#245924,#245925,#245926,#245927,#245928,#245929,#245930,
#245931,#245932,#245933,#245934,#245935,#245936,#245937,#245938,#245939,
#245940,#245941,#245942,#245943,#245944,#245945,#245946,#245947,#245948,
#245949,#245950,#245951,#245952,#245953,#245954,#245955,#245956,#245957,
#245958,#245959,#245960,#245961,#245962,#245963,#245964,#245965,#245966,
#245967,#245968,#245969,#245970,#245971,#245972,#245973,#245974,#245975,
#245976,#245977,#245978,#245979,#245980,#245981,#245982,#245983,#245984,
#245985,#245986,#245987,#245988,#245989,#245990,#245991,#245992,#245993,
#245994,#245995,#245996,#245997,#245998,#245999,#246000,#246001,#246002,
#246003,#246004,#246005,#246006,#246007,#246008,#246009,#246010,#246011,
#246012,#246013,#246014,#246015,#246016,#246017,#246018,#246019,#246020,
#246021,#246022,#246023,#246024,#246025,#246026,#246027,#246028,#246029,
#246030,#246031,#246032,#246033,#246034,#246035,#246036,#246037,#246038,
#246039,#246040,#246041,#246042,#246043,#246044,#246045,#246046,#246047,
#246048,#246049,#246050,#246051,#246052,#246053,#246054,#246055,#246056,
#246057,#246058,#246059,#246060,#246061,#246062,#246063,#246064,#246065,
#246066,#246067,#246068,#246069,#246070,#246071,#246072,#246073,#246074,
#246075,#246076,#246077,#246078,#246079,#246080,#246081,#246082,#246083,
#246084,#246085,#246086,#246087,#246088,#246089,#246090,#246091,#246092,
#246093,#246094,#246095,#246096,#246097,#246098,#246099,#246100,#246101,
#246102,#246103,#246104,#246105,#246106,#246107,#246108,#246109,#246110,
#246111,#246112,#246113,#246114,#246115,#246116,#246117,#246118,#246119,
#246120,#246121,#246122,#246123,#246124,#246125,#246126,#246127,#246128,
#246129,#246130,#246131,#246132,#246133,#246134,#246135,#246136,#246137,
#246138,#246139,#246140,#246141,#246142,#246143,#246144,#246145,#246146,
#246147,#246148,#246149,#246150,#246151,#246152,#246153,#246154,#246155,
#246156,#246157,#246158,#246159,#246160,#246161,#246162,#246163,#246164,
#246165,#246166,#246167,#246168,#246169,#246170,#246171,#246172,#246173,
#246174,#246175,#246176,#246177,#246178,#246179,#246180,#246181,#246182,
#246183,#246184,#246185,#246186,#246187,#246188,#246189,#246190,#246191,
#246192,#246193,#246194,#246195,#246196,#246197,#246198,#246199,#246200,
#246201,#246202,#246203,#246204,#246205,#246206,#246207,#246208),(#246209,
#246210,#246211,#246212,#246213,#246214,#246215,#246216,#246217,#246218,
#246219,#246220,#246221,#246222,#246223,#246224,#246225,#246226,#246227,
#246228,#246229,#246230,#246231,#246232,#246233,#246234,#246235,#246236,
#246237,#246238,#246239,#246240,#246241,#246242,#246243,#246244,#246245,
#246246,#246247,#246248,#246249,#246250,#246251,#246252,#246253,#246254,
#246255,#246256,#246257,#246258,#246259,#246260,#246261,#246262,#246263,
#246264,#246265,#246266,#246267,#246268,#246269,#246270,#246271,#246272,
#246273,#246274,#246275,#246276,#246277,#246278,#246279,#246280,#246281,
#246282,#246283,#246284,#246285,#246286,#246287,#246288,#246289,#246290,
#246291,#246292,#246293,#246294,#246295,#246296,#246297,#246298,#246299,
#246300,#246301,#246302,#246303,#246304,#246305,#246306,#246307,#246308,
#246309,#246310,#246311,#246312,#246313,#246314,#246315,#246316,#246317,
#246318,#246319,#246320,#246321,#246322,#246323,#246324,#246325,#246326,
#246327,#246328,#246329,#246330,#246331,#246332,#246333,#246334,#246335,
#246336,#246337,#246338,#246339,#246340,#246341,#246342,#246343,#246344,
#246345,#246346,#246347,#246348,#246349,#246350,#246351,#246352,#246353,
#246354,#246355,#246356,#246357,#246358,#246359,#246360,#246361,#246362,
#246363,#246364,#246365,#246366,#246367,#246368,#246369,#246370,#246371,
#246372,#246373,#246374,#246375,#246376,#246377,#246378,#246379,#246380,
#246381,#246382,#246383,#246384,#246385,#246386,#246387,#246388,#246389,
#246390,#246391,#246392,#246393,#246394,#246395,#246396,#246397,#246398,
#246399,#246400,#246401,#246402,#246403,#246404,#246405,#246406,#246407,
#246408,#246409,#246410,#246411,#246412,#246413,#246414,#246415,#246416,
#246417,#246418,#246419,#246420,#246421,#246422,#246423,#246424,#246425,
#246426,#246427,#246428,#246429,#246430,#246431,#246432,#246433,#246434,
#246435,#246436,#246437,#246438,#246439,#246440,#246441,#246442,#246443,
#246444,#246445,#246446,#246447,#246448,#246449,#246450,#246451,#246452,
#246453,#246454,#246455,#246456,#246457,#246458,#246459,#246460,#246461,
#246462,#246463,#246464,#246465,#246466,#246467,#246468,#246469,#246470,
#246471,#246472,#246473,#246474,#246475,#246476,#246477,#246478,#246479,
#246480,#246481,#246482,#246483,#246484,#246485,#246486,#246487,#246488,
#246489,#246490,#246491,#246492,#246493,#246494,#246495,#246496,#246497,
#246498,#246499,#246500,#246501,#246502,#246503,#246504,#246505,#246506,
#246507,#246508,#246509,#246510,#246511,#246512,#246513,#246514,#246515,
#246516,#246517,#246518,#246519,#246520,#246521,#246522,#246523,#246524,
#246525,#246526,#246527,#246528,#246529,#246530,#246531,#246532,#246533,
#246534,#246535,#246536,#246537,#246538,#246539,#246540,#246541,#246542,
#246543,#246544,#246545,#246546,#246547,#246548,#246549,#246550,#246551,
#246552,#246553,#246554,#246555,#246556,#246557,#246558,#246559,#246560,
#246561,#246562,#246563,#246564,#246565,#246566,#246567,#246568,#246569,
#246570,#246571,#246572,#246573,#246574,#246575,#246576,#246577,#246578,
#246579,#246580,#246581,#246582,#246583,#246584,#246585,#246586,#246587,
#246588,#246589,#246590,#246591,#246592,#246593,#246594,#246595,#246596,
#246597,#246598,#246599,#246600,#246601,#246602,#246603,#246604,#246605,
#246606,#246607,#246608,#246609,#246610,#246611,#246612,#246613,#246614,
#246615,#246616,#246617,#246618,#246619,#246620,#246621,#246622,#246623,
#246624,#246625,#246626,#246627,#246628,#246629,#246630,#246631,#246632,
#246633,#246634,#246635,#246636,#246637,#246638,#246639,#246640,#246641,
#246642,#246643,#246644,#246645,#246646,#246647,#246648,#246649,#246650,
#246651,#246652,#246653,#246654,#246655,#246656,#246657,#246658,#246659,
#246660,#246661,#246662,#246663,#246664,#246665,#246666,#246667,#246668,
#246669,#246670,#246671,#246672,#246673,#246674,#246675,#246676,#246677,
#246678,#246679,#246680,#246681,#246682,#246683,#246684,#246685,#246686,
#246687,#246688,#246689,#246690,#246691,#246692,#246693,#246694,#246695,
#246696,#246697,#246698,#246699,#246700,#246701,#246702,#246703,#246704,
#246705,#246706,#246707,#246708,#246709,#246710,#246711,#246712,#246713,
#246714,#246715,#246716,#246717,#246718,#246719,#246720,#246721,#246722,
#246723,#246724,#246725,#246726,#246727,#246728,#246729,#246730,#246731,
#246732,#246733,#246734,#246735,#246736,#246737,#246738,#246739,#246740,
#246741,#246742,#246743,#246744,#246745,#246746,#246747,#246748,#246749,
#246750,#246751,#246752,#246753,#246754,#246755,#246756,#246757,#246758,
#246759,#246760,#246761,#246762,#246763,#246764,#246765,#246766,#246767,
#246768,#246769,#246770,#246771,#246772,#246773,#246774,#246775,#246776,
#246777,#246778,#246779,#246780,#246781,#246782,#246783,#246784,#246785,
#246786,#246787,#246788,#246789,#246790,#246791,#246792,#246793,#246794,
#246795,#246796,#246797)),.UNSPECIFIED.,.F.,.F.,.F.,(4,4),(4,1,1,1,1,1,
1,1,1,1,1,1,1,1,1,1,1,1,1,1,1,1,1,1,1,1,1,1,1,1,1,1,1,1,1,1,1,1,1,1,1,1,
1,1,1,1,1,1,1,1,1,1,1,1,1,1,1,1,1,1,1,1,1,1,1,1,1,1,1,1,1,1,1,1,1,1,1,1,
1,1,1,1,1,1,1,1,1,1,1,1,1,1,1,1,1,1,1,1,1,1,1,1,1,1,1,1,1,1,1,1,1,1,1,1,
1,1,1,1,1,1,1,1,1,1,1,1,1,1,1,1,1,1,1,1,1,1,1,1,1,1,1,1,1,1,1,1,1,1,1,1,
1,1,1,1,1,1,1,1,1,1,1,1,1,1,1,1,1,1,1,1,1,1,1,1,1,1,1,1,1,1,1,1,1,1,1,1,
1,1,1,1,1,1,1,1,1,1,1,1,1,1,1,1,1,1,1,1,1,1,1,1,1,1,1,1,1,1,1,1,1,1,1,1,
1,1,1,1,1,1,1,1,1,1,1,1,1,1,1,1,1,1,1,1,1,1,1,1,1,1,1,1,1,1,1,1,1,1,1,1,
1,1,1,1,1,1,1,1,1,1,1,1,1,1,1,1,1,1,1,1,1,1,1,1,1,1,1,1,1,1,1,1,1,1,1,1,
1,1,1,1,1,1,1,1,1,1,1,1,1,1,1,1,1,1,1,1,1,1,1,1,1,1,1,1,1,1,1,1,1,1,1,1,
1,1,1,1,1,1,1,1,1,1,1,1,1,1,1,1,1,1,1,1,1,1,1,1,1,1,1,1,1,1,1,1,1,1,1,1,
1,1,1,1,1,1,1,1,1,1,1,1,1,1,1,1,1,1,1,1,1,1,1,1,1,1,1,1,1,1,1,1,1,1,1,1,
1,1,1,1,1,1,1,1,1,1,1,1,1,1,1,1,1,1,1,1,1,1,1,1,1,1,1,1,1,1,1,1,1,1,1,1,
1,1,1,1,1,1,1,1,1,1,1,1,1,1,1,1,1,1,1,1,1,1,1,1,1,1,1,1,1,1,1,1,1,1,1,1,
1,1,1,1,1,1,1,1,1,1,1,1,1,1,1,1,1,1,1,1,1,1,1,1,1,1,1,1,1,1,1,1,1,1,1,1,
1,1,1,1,1,1,1,1,1,1,1,1,1,1,1,1,1,1,1,1,1,1,1,1,1,1,1,1,1,1,1,1,1,1,1,1,
1,1,1,1,1,1,1,1,1,1,1,1,1,1,1,1,1,1,1,1,1,1,1,1,1,1,1,1,1,1,1,1,1,1,1,1,
1,1,1,1,4),(-0.00304463950594017,0.132890720296283),(11.6147257896704,12.1144027157503,
12.6137725836814,13.1131424516125,13.6125123195436,14.6112520554058,15.6099917912679,
16.6087315271301,17.1081013950612,17.6074712629923,18.1068411309234,18.6062109988545,
19.6049507347167,20.1043206026478,20.6036904705788,21.602430206441,22.6011699423032,
23.5999096781654,24.0992795460965,24.5986494140276,25.0980192819587,25.5973891498898,
26.5961288857519,27.095498753683,27.5948686216141,28.5936083574763,29.5923480933385,
30.5910878292007,31.0904576971318,31.5898275650629,32.0891974329939,32.588567300925,
33.5873070367872,34.0866769047183,34.5860467726494,35.5847865085116,36.5835262443738,
37.582265980236,38.081635848167,38.5810057160981,39.0803755840292,39.5797454519603,
40.5784851878225,41.0778550557536,41.5772249236847,42.5759646595469,43.5747043954091,
44.5734441312712,45.0728139992023,45.5721838671334,46.0715537350645,46.5709236029956,
47.5696633388578,48.0690332067889,48.56840307472,49.5671428105821,50.5658825464443,
51.5646222823065,52.0639921502376,52.5633620181687,53.0627318860998,53.5621017540309,
54.5608414898931,55.0602113578242,55.5595812257552,56.5583209616174,57.5570606974796,
58.5558004333418,59.0551703012729,59.554540169204,60.0539100371351,60.5532799050662,
61.5520196409283,62.0513895088594,62.5507593767905,63.5494991126527,64.5482388485149,
65.5469785843771,66.0463484523082,66.5457183202393,67.0450881881704,67.5444580561014,
68.5431977919636,69.0425676598947,69.5419375278258,70.540677263688,71.5394169995502,
72.5381567354124,73.0375266033435,73.5368964712745,74.0362663392056,74.5356362071367,
75.5343759429989,76.03374581093,76.5331156788611,77.5318554147233,78.5305951505855,
79.5293348864476,80.0287047543787,80.5280746223098,81.0274444902409,81.526814358172,
82.5255540940342,83.0249239619653,83.5242938298964,84.5230335657586,85.5217733016207,
86.5205130374829,87.019882905414,87.5192527733451,88.0186226412762,88.5179925092073,
89.5167322450695,90.0161021130006,90.5154719809317,91.5142117167938,92.512951452656,
93.5116911885182,94.0110610564493,94.5104309243804,95.0098007923115,95.5091706602426,
96.5079103961047,97.0072802640358,97.5066501319669,98.5053898678291,99.5041296036913,
100.502869339553,101.002239207485,101.501609075416,102.000978943347,102.500348811278,
103.49908854714,103.998458415071,104.497828283002,105.496568018864,106.495307754727,
107.494047490589,107.99341735852,108.492787226451,108.992157094382,109.491526962313,
110.490266698175,110.989636566106,111.489006434037,112.4877461699,113.486485905762,
114.485225641624,114.984595509555,115.483965377486,115.983335245417,116.482705113348,
117.481444849211,117.980814717142,118.480184585073,119.478924320935,120.477664056797,
121.476403792659,121.97577366059,122.475143528521,122.974513396453,123.473883264384,
124.472623000246,124.971992868177,125.471362736108,126.47010247197,127.468842207832,
128.467581943695,128.966951811626,129.466321679557,129.965691547488,130.465061415419,
131.463801151281,131.963171019212,132.462540887143,133.461280623006,134.460020358868,
135.45876009473,135.958129962661,136.457499830592,136.956869698523,137.456239566454,
138.454979302316,138.954349170247,139.453719038179,140.452458774041,141.451198509903,
142.449938245765,142.949308113696,143.448677981627,143.948047849558,144.44741771749,
145.446157453352,145.945527321283,146.444897189214,147.443636925076,148.442376660938,
149.4411163968,149.940486264732,150.439856132663,150.939226000594,151.438595868525,
152.437335604387,152.936705472318,153.436075340249,154.434815076111,155.433554811974,
156.432294547836,156.931664415767,157.431034283698,157.930404151629,158.42977401956,
159.428513755422,159.927883623353,160.427253491284,161.425993227147,162.424732963009,
163.423472698871,163.922842566802,164.422212434733,164.921582302664,165.420952170595,
166.419691906458,166.919061774389,167.41843164232,168.417171378182,169.415911114044,
170.414650849906,170.914020717837,171.413390585768,171.9127604537,172.412130321631,
173.410870057493,173.910239925424,174.409609793355,175.408349529217,176.407089265079,
177.405829000942,177.905198868873,178.404568736804,178.903938604735,179.403308472666,
180.402048208528,180.901418076459,181.40078794439,182.399527680252,183.398267416115,
184.397007151977,184.896377019908,185.395746887839,185.89511675577,186.394486623701,
187.393226359563,187.892596227494,188.391966095426,189.390705831288,190.38944556715,
191.388185303012,191.887555170943,192.386925038874,192.886294906805,193.385664774736,
194.384404510599,194.88377437853,195.383144246461,196.381883982323,197.380623718185,
198.379363454047,198.878733321978,199.37810318991,199.877473057841,200.376842925772,
201.375582661634,201.874952529565,202.374322397496,203.373062133358,204.37180186922,
205.370541605083,205.869911473014,206.369281340945,206.868651208876,207.368021076807,
208.366760812669,208.8661306806,209.365500548531,210.364240284394,211.362980020256,
212.361719756118,212.861089624049,213.36045949198,213.859829359911,214.359199227842,
215.357938963704,215.857308831636,216.356678699567,217.355418435429,218.354158171291,
219.352897907153,220.351637643015,221.350377378878,222.34911711474,223.347856850602,
224.346596586464,224.845966454395,225.345336322326,226.344076058189,226.84344592612,
227.342815794051,227.842185661982,228.341555529913,229.340295265775,230.339035001637,
231.337774737499,231.837144605431,232.336514473362,233.335254209224,233.834624077155,
234.333993945086,234.833363813017,235.332733680948,236.33147341681,237.330213152673,
238.328952888535,238.828322756466,239.327692624397,240.326432360259,240.82580222819,
241.325172096121,241.824541964052,242.323911831983,243.322651567846,244.321391303708,
245.32013103957,245.819500907501,246.318870775432,247.317610511294,247.816980379225,
248.316350247157,248.815720115088,249.315089983019,250.313829718881,251.312569454743,
252.311309190605,252.810679058536,253.310048926467,254.30878866233,254.808158530261,
255.307528398192,255.806898266123,256.306268134054,257.305007869916,258.303747605778,
259.302487341641,259.801857209572,260.301227077503,261.299966813365,261.799336681296,
262.298706549227,262.798076417158,263.297446285089,264.296186020951,265.294925756814,
266.293665492676,266.793035360607,267.292405228538,268.2911449644,268.790514832331,
269.289884700262,269.789254568193,270.288624436125,271.287364171987,272.286103907849,
273.284843643711,273.784213511642,274.283583379573,275.282323115435,275.781692983366,
276.281062851298,276.780432719229,277.27980258716,278.278542323022,279.277282058884,
280.276021794746,280.775391662677,281.274761530609,282.273501266471,282.772871134402,
283.272241002333,283.771610870264,284.270980738195,285.269720474057,286.268460209919,
287.267199945782,287.766569813713,288.265939681644,289.264679417506,289.764049285437,
290.263419153368,290.762789021299,291.26215888923,292.260898625093,293.259638360955,
294.258378096817,294.757747964748,295.257117832679,296.255857568541,296.755227436472,
297.254597304403,297.753967172335,298.253337040266,299.252076776128,300.25081651199,
301.249556247852,301.748926115783,302.248295983714,303.247035719577,303.746405587508,
304.245775455439,304.74514532337,305.244515191301,306.243254927163,307.241994663025,
308.240734398887,308.740104266819,309.23947413475,310.238213870612,310.737583738543,
311.236953606474,311.736323474405,312.235693342336,313.234433078198,314.233172814061,
315.231912549923,315.731282417854,316.230652285785,317.229392021647,317.728761889578,
318.228131757509,318.72750162544,319.226871493372,320.225611229234,321.224350965096,
322.223090700958,322.722460568889,323.22183043682,324.220570172682,324.719940040613,
325.219309908545,325.718679776476,326.218049644407,327.216789380269,328.215529116131,
329.214268851993,329.713638719924,330.213008587855,331.211748323718,331.711118191649,
332.21048805958,332.709857927511,333.209227795442,334.207967531304,335.206707267166,
336.205447003029,336.70481687096,337.204186738891,338.202926474753,338.702296342684,
339.201666210615,339.701036078546,340.200405946477,341.19914568234,342.197885418202,
343.196625154064,343.695995021995,344.195364889926,345.194104625788,345.693474493719,
346.19284436165,346.692214229582,347.191584097513,348.190323833375,349.189063569237,
350.187803305099,350.68717317303,351.186543040961,352.185282776823,352.684652644755,
353.184022512686,353.683392380617,354.182762248548,355.18150198441,356.180241720272,
357.178981456134,357.678351324065,358.177721191997,359.176460927859,359.67583079579,
360.175200663721,360.674570531652,361.173940399583,362.172680135445,363.171419871308,
364.17015960717,364.669529475101,365.168899343032,366.167639078894,366.667008946825,
367.166378814756,367.665748682687,368.165118550618,369.163858286481,370.162598022343,
371.161337758205,371.660707626136,372.160077494067,373.158817229929,373.65818709786,
374.157556965792,374.656926833723,375.156296701654,376.155036437516,377.153776173378,
378.15251590924,378.651885777171,379.151255645102,380.149995380965,380.649365248896,
381.148735116827,381.648104984758,382.147474852689,383.146214588551,384.144954324413,
385.143694060276,385.643063928207,386.142433796138,387.141173532,387.640543399931,
388.139913267862,388.639283135793,389.138653003724,390.137392739586,391.136132475449,
392.134872211311,392.634242079242,393.133611947173,394.132351683035,394.631721550966,
395.131091418897,395.630461286828,396.12983115476,397.128570890622,398.127310626484,
399.126050362346,399.625420230277,400.124790098208,401.12352983407,401.622899702002,
402.122269569933,402.621639437864,403.121009305795,404.119749041657,405.118488777519,
406.117228513381,406.616598381312,407.115968249244,408.114707985106,408.614077853037,
409.113447720968,409.612817588899,410.11218745683,411.110927192692,412.109666928554,
413.108406664417,413.607776532348,414.107146400279,415.105886136141,415.605256004072,
416.104625872003,416.603995739934,417.103365607865,418.102105343728,419.10084507959,
420.099584815452,420.598954683383,421.098324551314,421.597694419245,422.097674725987),
 .UNSPECIFIED.);
#373=PLANE('',#17657);
#374=PLANE('',#17658);
#375=PLANE('',#17665);
#376=PLANE('',#17666);
#866=FACE_OUTER_BOUND('',#1569,.T.);
#867=FACE_OUTER_BOUND('',#1570,.T.);
#868=FACE_OUTER_BOUND('',#1571,.T.);
#869=FACE_OUTER_BOUND('',#1572,.T.);
#870=FACE_OUTER_BOUND('',#1573,.T.);
#871=FACE_OUTER_BOUND('',#1574,.T.);
#872=FACE_OUTER_BOUND('',#1575,.T.);
#873=FACE_OUTER_BOUND('',#1576,.T.);
#874=FACE_OUTER_BOUND('',#1577,.T.);
#875=FACE_OUTER_BOUND('',#1578,.T.);
#876=FACE_OUTER_BOUND('',#1579,.T.);
#877=FACE_OUTER_BOUND('',#1580,.T.);
#878=FACE_OUTER_BOUND('',#1581,.T.);
#879=FACE_OUTER_BOUND('',#1582,.T.);
#880=FACE_OUTER_BOUND('',#1583,.T.);
#881=FACE_OUTER_BOUND('',#1584,.T.);
#882=FACE_OUTER_BOUND('',#1585,.T.);
#883=FACE_OUTER_BOUND('',#1586,.T.);
#884=FACE_OUTER_BOUND('',#1587,.T.);
#885=FACE_OUTER_BOUND('',#1588,.T.);
#886=FACE_OUTER_BOUND('',#1589,.T.);
#887=FACE_OUTER_BOUND('',#1590,.T.);
#888=FACE_OUTER_BOUND('',#1591,.T.);
#889=FACE_OUTER_BOUND('',#1592,.T.);
#890=FACE_OUTER_BOUND('',#1593,.T.);
#891=FACE_OUTER_BOUND('',#1594,.T.);
#892=FACE_OUTER_BOUND('',#1595,.T.);
#893=FACE_OUTER_BOUND('',#1596,.T.);
#894=FACE_OUTER_BOUND('',#1597,.T.);
#895=FACE_OUTER_BOUND('',#1598,.T.);
#896=FACE_OUTER_BOUND('',#1599,.T.);
#897=FACE_OUTER_BOUND('',#1600,.T.);
#898=FACE_OUTER_BOUND('',#1601,.T.);
#899=FACE_OUTER_BOUND('',#1602,.T.);
#900=FACE_OUTER_BOUND('',#1603,.T.);
#901=FACE_OUTER_BOUND('',#1604,.T.);
#902=FACE_OUTER_BOUND('',#1605,.T.);
#903=FACE_OUTER_BOUND('',#1606,.T.);
#904=FACE_OUTER_BOUND('',#1607,.T.);
#905=FACE_OUTER_BOUND('',#1608,.T.);
#906=FACE_OUTER_BOUND('',#1609,.T.);
#907=FACE_OUTER_BOUND('',#1610,.T.);
#908=FACE_OUTER_BOUND('',#1611,.T.);
#909=FACE_OUTER_BOUND('',#1612,.T.);
#910=FACE_OUTER_BOUND('',#1613,.T.);
#911=FACE_OUTER_BOUND('',#1614,.T.);
#912=FACE_OUTER_BOUND('',#1615,.T.);
#913=FACE_OUTER_BOUND('',#1616,.T.);
#914=FACE_OUTER_BOUND('',#1617,.T.);
#915=FACE_OUTER_BOUND('',#1618,.T.);
#916=FACE_OUTER_BOUND('',#1619,.T.);
#917=FACE_OUTER_BOUND('',#1620,.T.);
#918=FACE_OUTER_BOUND('',#1621,.T.);
#919=FACE_OUTER_BOUND('',#1622,.T.);
#920=FACE_OUTER_BOUND('',#1623,.T.);
#921=FACE_OUTER_BOUND('',#1624,.T.);
#922=FACE_OUTER_BOUND('',#1625,.T.);
#923=FACE_OUTER_BOUND('',#1626,.T.);
#924=FACE_OUTER_BOUND('',#1627,.T.);
#925=FACE_OUTER_BOUND('',#1628,.T.);
#926=FACE_OUTER_BOUND('',#1629,.T.);
#927=FACE_OUTER_BOUND('',#1630,.T.);
#928=FACE_OUTER_BOUND('',#1631,.T.);
#929=FACE_OUTER_BOUND('',#1632,.T.);
#930=FACE_OUTER_BOUND('',#1633,.T.);
#931=FACE_OUTER_BOUND('',#1634,.T.);
#932=FACE_OUTER_BOUND('',#1635,.T.);
#933=FACE_OUTER_BOUND('',#1636,.T.);
#934=FACE_OUTER_BOUND('',#1637,.T.);
#935=FACE_OUTER_BOUND('',#1638,.T.);
#936=FACE_OUTER_BOUND('',#1639,.T.);
#937=FACE_OUTER_BOUND('',#1640,.T.);
#938=FACE_OUTER_BOUND('',#1642,.T.);
#939=FACE_OUTER_BOUND('',#1643,.T.);
#940=FACE_OUTER_BOUND('',#1645,.T.);
#941=FACE_OUTER_BOUND('',#1647,.T.);
#1569=EDGE_LOOP('',(#13799,#13800,#13801,#13802));
#1570=EDGE_LOOP('',(#13803,#13804,#13805,#13806,#13807,#13808));
#1571=EDGE_LOOP('',(#13809,#13810,#13811,#13812,#13813,#13814));
#1572=EDGE_LOOP('',(#13815,#13816,#13817,#13818,#13819,#13820));
#1573=EDGE_LOOP('',(#13821,#13822,#13823,#13824,#13825,#13826));
#1574=EDGE_LOOP('',(#13827,#13828,#13829,#13830,#13831,#13832));
#1575=EDGE_LOOP('',(#13833,#13834,#13835,#13836,#13837,#13838));
#1576=EDGE_LOOP('',(#13839,#13840,#13841,#13842,#13843,#13844));
#1577=EDGE_LOOP('',(#13845,#13846,#13847,#13848,#13849,#13850));
#1578=EDGE_LOOP('',(#13851,#13852,#13853,#13854,#13855,#13856));
#1579=EDGE_LOOP('',(#13857,#13858,#13859,#13860,#13861,#13862));
#1580=EDGE_LOOP('',(#13863,#13864,#13865,#13866,#13867,#13868));
#1581=EDGE_LOOP('',(#13869,#13870,#13871,#13872,#13873,#13874));
#1582=EDGE_LOOP('',(#13875,#13876,#13877,#13878,#13879,#13880));
#1583=EDGE_LOOP('',(#13881,#13882,#13883,#13884,#13885,#13886));
#1584=EDGE_LOOP('',(#13887,#13888,#13889,#13890,#13891,#13892));
#1585=EDGE_LOOP('',(#13893,#13894,#13895,#13896,#13897,#13898));
#1586=EDGE_LOOP('',(#13899,#13900,#13901,#13902,#13903,#13904));
#1587=EDGE_LOOP('',(#13905,#13906,#13907,#13908,#13909,#13910));
#1588=EDGE_LOOP('',(#13911,#13912,#13913,#13914,#13915,#13916));
#1589=EDGE_LOOP('',(#13917,#13918,#13919,#13920,#13921,#13922));
#1590=EDGE_LOOP('',(#13923,#13924,#13925,#13926,#13927,#13928));
#1591=EDGE_LOOP('',(#13929,#13930,#13931,#13932,#13933,#13934));
#1592=EDGE_LOOP('',(#13935,#13936,#13937,#13938,#13939,#13940));
#1593=EDGE_LOOP('',(#13941,#13942,#13943,#13944,#13945,#13946));
#1594=EDGE_LOOP('',(#13947,#13948,#13949,#13950,#13951,#13952));
#1595=EDGE_LOOP('',(#13953,#13954,#13955,#13956,#13957,#13958));
#1596=EDGE_LOOP('',(#13959,#13960,#13961,#13962,#13963,#13964));
#1597=EDGE_LOOP('',(#13965,#13966,#13967,#13968,#13969,#13970));
#1598=EDGE_LOOP('',(#13971,#13972,#13973,#13974,#13975,#13976));
#1599=EDGE_LOOP('',(#13977,#13978,#13979,#13980,#13981,#13982));
#1600=EDGE_LOOP('',(#13983,#13984,#13985,#13986,#13987,#13988));
#1601=EDGE_LOOP('',(#13989,#13990,#13991,#13992,#13993,#13994));
#1602=EDGE_LOOP('',(#13995,#13996,#13997,#13998,#13999,#14000));
#1603=EDGE_LOOP('',(#14001,#14002,#14003,#14004,#14005,#14006));
#1604=EDGE_LOOP('',(#14007,#14008,#14009,#14010,#14011,#14012));
#1605=EDGE_LOOP('',(#14013,#14014,#14015,#14016,#14017,#14018));
#1606=EDGE_LOOP('',(#14019,#14020,#14021,#14022,#14023,#14024));
#1607=EDGE_LOOP('',(#14025,#14026,#14027,#14028,#14029,#14030));
#1608=EDGE_LOOP('',(#14031,#14032,#14033,#14034,#14035,#14036));
#1609=EDGE_LOOP('',(#14037,#14038,#14039,#14040,#14041,#14042));
#1610=EDGE_LOOP('',(#14043,#14044,#14045,#14046,#14047,#14048));
#1611=EDGE_LOOP('',(#14049,#14050,#14051,#14052,#14053,#14054));
#1612=EDGE_LOOP('',(#14055,#14056,#14057,#14058,#14059,#14060));
#1613=EDGE_LOOP('',(#14061,#14062,#14063,#14064,#14065,#14066));
#1614=EDGE_LOOP('',(#14067,#14068,#14069,#14070,#14071,#14072));
#1615=EDGE_LOOP('',(#14073,#14074,#14075,#14076,#14077,#14078));
#1616=EDGE_LOOP('',(#14079,#14080,#14081,#14082,#14083,#14084));
#1617=EDGE_LOOP('',(#14085,#14086,#14087,#14088,#14089,#14090));
#1618=EDGE_LOOP('',(#14091,#14092,#14093,#14094,#14095,#14096));
#1619=EDGE_LOOP('',(#14097,#14098,#14099,#14100,#14101,#14102));
#1620=EDGE_LOOP('',(#14103,#14104,#14105,#14106,#14107,#14108));
#1621=EDGE_LOOP('',(#14109,#14110,#14111,#14112,#14113,#14114));
#1622=EDGE_LOOP('',(#14115,#14116,#14117,#14118,#14119,#14120));
#1623=EDGE_LOOP('',(#14121,#14122,#14123,#14124,#14125,#14126));
#1624=EDGE_LOOP('',(#14127,#14128,#14129,#14130,#14131,#14132));
#1625=EDGE_LOOP('',(#14133,#14134,#14135,#14136,#14137,#14138));
#1626=EDGE_LOOP('',(#14139,#14140,#14141,#14142,#14143,#14144));
#1627=EDGE_LOOP('',(#14145,#14146,#14147,#14148,#14149,#14150));
#1628=EDGE_LOOP('',(#14151,#14152,#14153,#14154,#14155,#14156));
#1629=EDGE_LOOP('',(#14157,#14158,#14159,#14160,#14161,#14162));
#1630=EDGE_LOOP('',(#14163,#14164,#14165,#14166,#14167,#14168));
#1631=EDGE_LOOP('',(#14169,#14170,#14171,#14172,#14173,#14174));
#1632=EDGE_LOOP('',(#14175,#14176,#14177,#14178,#14179,#14180));
#1633=EDGE_LOOP('',(#14181,#14182,#14183,#14184,#14185,#14186));
#1634=EDGE_LOOP('',(#14187,#14188,#14189,#14190,#14191,#14192,#14193,#14194,
#14195,#14196,#14197,#14198,#14199,#14200,#14201,#14202,#14203,#14204,#14205,
#14206,#14207,#14208,#14209,#14210,#14211,#14212,#14213,#14214,#14215,#14216,
#14217,#14218,#14219,#14220,#14221,#14222,#14223,#14224,#14225,#14226,#14227,
#14228,#14229,#14230,#14231,#14232,#14233,#14234,#14235,#14236,#14237,#14238,
#14239,#14240,#14241,#14242,#14243,#14244,#14245,#14246,#14247,#14248,#14249,
#14250,#14251,#14252,#14253,#14254,#14255,#14256,#14257,#14258,#14259,#14260,
#14261,#14262,#14263,#14264,#14265,#14266,#14267,#14268,#14269,#14270,#14271,
#14272,#14273,#14274,#14275,#14276,#14277,#14278,#14279,#14280,#14281,#14282,
#14283,#14284,#14285));
#1635=EDGE_LOOP('',(#14286,#14287,#14288,#14289,#14290,#14291));
#1636=EDGE_LOOP('',(#14292,#14293,#14294,#14295,#14296,#14297,#14298,#14299));
#1637=EDGE_LOOP('',(#14300,#14301,#14302,#14303,#14304,#14305,#14306,#14307,
#14308,#14309,#14310,#14311,#14312,#14313,#14314,#14315,#14316,#14317,#14318,
#14319,#14320,#14321,#14322,#14323,#14324,#14325,#14326,#14327,#14328,#14329,
#14330,#14331,#14332,#14333,#14334,#14335,#14336,#14337,#14338,#14339,#14340,
#14341,#14342,#14343,#14344,#14345,#14346,#14347,#14348,#14349,#14350,#14351,
#14352,#14353,#14354,#14355,#14356,#14357,#14358,#14359,#14360,#14361,#14362,
#14363,#14364,#14365,#14366,#14367,#14368,#14369,#14370,#14371,#14372,#14373,
#14374,#14375,#14376,#14377,#14378,#14379,#14380,#14381,#14382,#14383,#14384,
#14385,#14386,#14387,#14388,#14389,#14390,#14391,#14392,#14393,#14394,#14395,
#14396,#14397,#14398,#14399,#14400,#14401,#14402,#14403,#14404,#14405,#14406,
#14407,#14408,#14409,#14410,#14411,#14412,#14413,#14414,#14415,#14416,#14417,
#14418,#14419,#14420,#14421,#14422,#14423,#14424,#14425,#14426,#14427,#14428,
#14429,#14430,#14431,#14432,#14433,#14434,#14435,#14436,#14437,#14438,#14439,
#14440,#14441,#14442,#14443,#14444,#14445,#14446,#14447,#14448,#14449,#14450,
#14451,#14452,#14453,#14454,#14455,#14456,#14457,#14458,#14459,#14460,#14461,
#14462,#14463,#14464,#14465,#14466,#14467,#14468,#14469,#14470,#14471,#14472,
#14473,#14474,#14475,#14476,#14477,#14478,#14479,#14480,#14481));
#1638=EDGE_LOOP('',(#14482,#14483,#14484,#14485,#14486,#14487,#14488,#14489,
#14490,#14491,#14492,#14493,#14494,#14495,#14496,#14497,#14498,#14499,#14500,
#14501,#14502,#14503,#14504,#14505,#14506,#14507,#14508,#14509,#14510,#14511,
#14512,#14513,#14514,#14515,#14516,#14517,#14518,#14519,#14520,#14521,#14522,
#14523,#14524,#14525,#14526,#14527,#14528,#14529,#14530,#14531,#14532,#14533,
#14534,#14535,#14536,#14537,#14538,#14539,#14540,#14541,#14542,#14543,#14544,
#14545,#14546,#14547,#14548,#14549,#14550,#14551,#14552,#14553,#14554,#14555,
#14556,#14557,#14558,#14559,#14560,#14561,#14562,#14563,#14564,#14565,#14566,
#14567,#14568,#14569,#14570,#14571,#14572,#14573,#14574,#14575,#14576,#14577,
#14578,#14579,#14580,#14581,#14582,#14583,#14584,#14585,#14586,#14587,#14588,
#14589,#14590,#14591,#14592,#14593,#14594,#14595,#14596,#14597,#14598,#14599,
#14600,#14601,#14602,#14603,#14604,#14605,#14606,#14607,#14608,#14609,#14610,
#14611,#14612,#14613,#14614,#14615,#14616,#14617,#14618,#14619,#14620,#14621,
#14622,#14623,#14624,#14625,#14626,#14627,#14628,#14629,#14630,#14631,#14632,
#14633,#14634,#14635,#14636,#14637,#14638,#14639,#14640,#14641,#14642,#14643,
#14644,#14645,#14646,#14647,#14648,#14649,#14650,#14651,#14652,#14653,#14654,
#14655,#14656,#14657,#14658,#14659,#14660,#14661,#14662));
#1639=EDGE_LOOP('',(#14663,#14664,#14665,#14666));
#1640=EDGE_LOOP('',(#14667));
#1641=EDGE_LOOP('',(#14668));
#1642=EDGE_LOOP('',(#14669,#14670,#14671,#14672));
#1643=EDGE_LOOP('',(#14673,#14674,#14675,#14676,#14677,#14678,#14679,#14680,
#14681));
#1644=EDGE_LOOP('',(#14682,#14683,#14684));
#1645=EDGE_LOOP('',(#14685));
#1646=EDGE_LOOP('',(#14686,#14687,#14688,#14689));
#1647=EDGE_LOOP('',(#14690));
#1917=CIRCLE('',#17586,6.767);
#1918=CIRCLE('',#17652,7.911);
#1919=CIRCLE('',#17653,7.911);
#1920=CIRCLE('',#17655,6.767);
#1921=CIRCLE('',#17659,10.);
#1922=CIRCLE('',#17660,6.);
#1923=CIRCLE('',#17662,10.);
#1924=CIRCLE('',#17664,6.);
#3267=B_SPLINE_CURVE_WITH_KNOTS('',3,(#185306,#185307,#185308,#185309,#185310,
#185311,#185312,#185313,#185314,#185315,#185316,#185317,#185318,#185319,
#185320,#185321,#185322,#185323,#185324,#185325,#185326,#185327,#185328,
#185329,#185330,#185331,#185332,#185333,#185334,#185335,#185336,#185337,
#185338,#185339,#185340,#185341,#185342,#185343,#185344,#185345,#185346,
#185347,#185348,#185349,#185350,#185351,#185352,#185353,#185354,#185355,
#185356,#185357,#185358,#185359,#185360,#185361,#185362,#185363,#185364,
#185365,#185366,#185367,#185368,#185369,#185370,#185371,#185372,#185373,
#185374,#185375,#185376,#185377,#185378,#185379,#185380,#185381,#185382,
#185383,#185384,#185385,#185386,#185387,#185388,#185389,#185390,#185391,
#185392,#185393,#185394,#185395,#185396,#185397,#185398,#185399,#185400,
#185401,#185402,#185403,#185404,#185405,#185406,#185407,#185408,#185409,
#185410,#185411,#185412,#185413,#185414,#185415,#185416,#185417,#185418,
#185419,#185420,#185421,#185422,#185423,#185424,#185425,#185426,#185427,
#185428,#185429,#185430,#185431,#185432,#185433,#185434,#185435,#185436,
#185437,#185438),.UNSPECIFIED.,.F.,.F.,(4,3,3,3,3,3,3,3,3,3,3,3,3,3,3,3,
3,3,3,3,3,3,3,3,3,3,3,3,3,3,3,3,3,3,3,3,3,3,3,3,3,3,3,3,4),(10.3763777524407,
10.4542232522646,10.53200845239,10.6097484354634,10.6874582514084,10.7651674175212,
10.8428794104451,10.9206078434063,10.9983663362618,11.0762147773958,11.1541105300842,
11.2321249227821,11.2973484622136,11.3732369885882,11.4490299366276,11.5247441915214,
11.6003965522182,11.6760037517047,11.7535143075011,11.8290965955637,11.904686794747,
11.9802999913294,12.059247043016,12.134995161763,12.2108009921308,12.2867151833181,
12.2960881980758,12.374419020755,12.4526550318628,12.5308110341746,12.6089017742511,
12.6869419524188,12.764949288339,12.842939589717,12.9209261159944,12.9989221219091,
13.076974473593,13.1550558360197,13.233223596569,13.2948279339379,13.3750325299376,
13.4551442153435,13.5352002283623,13.6151987913663,13.6615588095422),
 .UNSPECIFIED.);
#3268=B_SPLINE_CURVE_WITH_KNOTS('',3,(#185441,#185442,#185443,#185444,#185445,
#185446,#185447,#185448,#185449,#185450,#185451,#185452,#185453,#185454,
#185455,#185456,#185457,#185458,#185459,#185460,#185461,#185462,#185463,
#185464,#185465,#185466,#185467,#185468,#185469,#185470,#185471,#185472,
#185473,#185474,#185475,#185476,#185477,#185478,#185479,#185480,#185481,
#185482,#185483,#185484,#185485,#185486,#185487,#185488,#185489,#185490,
#185491,#185492,#185493,#185494,#185495,#185496,#185497,#185498,#185499,
#185500,#185501,#185502,#185503,#185504,#185505,#185506,#185507,#185508,
#185509,#185510,#185511,#185512,#185513,#185514,#185515,#185516,#185517,
#185518,#185519,#185520,#185521,#185522),.UNSPECIFIED.,.F.,.F.,(4,3,3,3,
3,3,3,3,3,3,3,3,3,3,3,3,3,3,3,3,3,3,3,3,3,3,3,4),(11.6150328478192,11.6997947966607,
11.7845824496215,11.8693850422671,11.9541730765905,12.0389208866034,12.1144027157503,
12.1914322579443,12.2684369525882,12.3454311630728,12.4224505903829,12.4994839724856,
12.5765733135033,12.6137725836814,12.7012857649444,12.7888168916037,12.8762822893983,
12.9636620303614,13.0508381795771,13.1131424516125,13.1910545333156,13.2689596642437,
13.3468712530953,13.4248300535109,13.5028157561103,13.5808723881572,13.6125123195436,
13.6615967360777),.UNSPECIFIED.);
#3269=B_SPLINE_CURVE_WITH_KNOTS('',3,(#185528,#185529,#185530,#185531,#185532,
#185533,#185534,#185535,#185536,#185537,#185538,#185539,#185540,#185541,
#185542,#185543,#185544,#185545,#185546,#185547,#185548,#185549,#185550,
#185551,#185552,#185553,#185554,#185555,#185556,#185557,#185558,#185559,
#185560,#185561,#185562,#185563,#185564,#185565,#185566,#185567,#185568,
#185569,#185570,#185571,#185572,#185573,#185574,#185575,#185576,#185577,
#185578,#185579,#185580,#185581,#185582,#185583,#185584,#185585,#185586,
#185587,#185588,#185589,#185590,#185591,#185592,#185593,#185594,#185595,
#185596,#185597,#185598,#185599,#185600,#185601,#185602,#185603,#185604,
#185605,#185606,#185607,#185608,#185609,#185610,#185611,#185612,#185613,
#185614,#185615,#185616,#185617,#185618,#185619,#185620,#185621,#185622,
#185623,#185624,#185625,#185626,#185627,#185628,#185629,#185630,#185631,
#185632,#185633,#185634,#185635,#185636,#185637,#185638,#185639,#185640,
#185641,#185642,#185643,#185644,#185645,#185646,#185647,#185648,#185649,
#185650,#185651,#185652,#185653,#185654,#185655,#185656,#185657,#185658,
#185659,#185660,#185661,#185662,#185663,#185664,#185665,#185666,#185667,
#185668,#185669,#185670,#185671,#185672,#185673,#185674,#185675,#185676,
#185677,#185678,#185679,#185680,#185681,#185682,#185683,#185684),
 .UNSPECIFIED.,.F.,.F.,(4,3,3,3,3,3,3,3,3,3,3,3,3,3,3,3,3,3,3,3,3,3,3,3,
3,3,3,3,3,3,3,3,3,3,3,3,3,3,3,3,3,3,3,3,3,3,3,3,3,3,3,3,4),(15.7079632679498,
15.7904254740354,15.8728873318234,15.9553488481645,16.0378100299085,16.1202708839052,
16.202731417004,16.2851916360542,16.3676515479046,16.4501111594039,16.5325704774007,
16.6150295087427,16.697488260278,16.7799467388542,16.8624049513188,16.944862904519,
17.0273206053015,17.1097780605135,17.1922352770009,17.2782478647903,17.3615725592112,
17.4440391647695,17.5265049261203,17.6089698706785,17.6914340258564,17.7738974190637,
17.8563600777072,17.9388220291911,18.0212833009174,18.1037439202856,18.1862039146928,
18.268663311534,18.3511221382023,18.4335804220887,18.5160381905821,18.5984954710698,
18.6826293845192,18.7650953828176,18.8475597593663,18.9300226238083,19.0124840857651,
19.094944254839,19.1774032406137,19.2598611526566,19.3454582693571,19.4279230063008,
19.5103847785989,19.5928440246899,19.6753011828687,19.7577637017675,19.8402213730509,
19.9226801639591,19.9446380862602),.UNSPECIFIED.);
#3270=B_SPLINE_CURVE_WITH_KNOTS('',3,(#185685,#185686,#185687,#185688,#185689,
#185690,#185691,#185692,#185693,#185694,#185695,#185696,#185697,#185698,
#185699,#185700,#185701,#185702,#185703,#185704,#185705,#185706,#185707,
#185708,#185709,#185710,#185711,#185712,#185713,#185714,#185715,#185716,
#185717,#185718,#185719,#185720,#185721,#185722,#185723,#185724,#185725,
#185726,#185727,#185728,#185729,#185730,#185731,#185732,#185733,#185734,
#185735,#185736,#185737,#185738,#185739,#185740,#185741,#185742,#185743,
#185744,#185745,#185746,#185747,#185748,#185749,#185750,#185751,#185752,
#185753,#185754,#185755,#185756,#185757,#185758,#185759,#185760,#185761,
#185762,#185763,#185764,#185765,#185766),.UNSPECIFIED.,.F.,.F.,(4,3,3,3,
3,3,3,3,3,3,3,3,3,3,3,3,3,3,3,3,3,3,3,3,3,3,3,4),(13.6615588095422,13.7414980263516,
13.794197801869,13.8750436869468,13.955930516902,14.0403398051265,14.1213664543982,
14.2024435631694,14.2836058572761,14.2935676698001,14.3790087171045,14.4643727588897,
14.5495839125019,14.6346852202888,14.719586329486,14.7929375377312,14.8694577764537,
14.9459724650645,15.0224962268134,15.0990757955442,15.1756865300405,15.252380955568,
15.2923074056623,15.379635702775,15.4667829706427,15.5537849884522,15.6404952190153,
15.7079632679498),.UNSPECIFIED.);
#3271=B_SPLINE_CURVE_WITH_KNOTS('',3,(#185768,#185769,#185770,#185771,#185772,
#185773,#185774,#185775,#185776,#185777,#185778,#185779,#185780,#185781,
#185782,#185783,#185784,#185785,#185786,#185787,#185788,#185789,#185790,
#185791,#185792,#185793,#185794,#185795,#185796,#185797,#185798,#185799,
#185800,#185801,#185802,#185803,#185804,#185805,#185806,#185807,#185808,
#185809,#185810,#185811,#185812,#185813,#185814,#185815,#185816,#185817,
#185818,#185819,#185820,#185821,#185822,#185823,#185824,#185825,#185826,
#185827,#185828,#185829,#185830,#185831,#185832,#185833,#185834,#185835,
#185836,#185837,#185838,#185839,#185840,#185841,#185842,#185843,#185844,
#185845,#185846,#185847,#185848,#185849),.UNSPECIFIED.,.F.,.F.,(4,3,3,3,
3,3,3,3,3,3,3,3,3,3,3,3,3,3,3,3,3,3,3,3,3,3,3,4),(13.6615967360777,13.7400356036608,
13.8184202198503,13.8967647778476,13.9750834408796,14.0546045176954,14.1329331115179,
14.2112797336207,14.2896572211474,14.370055929712,14.4485745617826,14.5299133085942,
14.6112520554058,14.6871405817804,14.7629335298198,14.8386477847136,14.9143001454103,
14.9899073448968,15.0674179006932,15.1430001887558,15.2185903879391,15.2942035845215,
15.3731506362081,15.4488987549552,15.5247045853228,15.6006187765102,15.6099917912679,
15.7079632679497),.UNSPECIFIED.);
#3272=B_SPLINE_CURVE_WITH_KNOTS('',3,(#185850,#185851,#185852,#185853,#185854,
#185855,#185856,#185857,#185858,#185859,#185860,#185861,#185862,#185863,
#185864,#185865,#185866,#185867,#185868,#185869,#185870,#185871,#185872,
#185873,#185874,#185875,#185876,#185877,#185878,#185879,#185880,#185881,
#185882,#185883,#185884,#185885,#185886,#185887,#185888,#185889,#185890,
#185891,#185892,#185893,#185894,#185895,#185896,#185897,#185898,#185899,
#185900,#185901,#185902,#185903,#185904,#185905,#185906,#185907,#185908,
#185909,#185910,#185911,#185912,#185913,#185914,#185915,#185916,#185917,
#185918,#185919,#185920,#185921,#185922,#185923,#185924,#185925,#185926,
#185927,#185928,#185929,#185930,#185931,#185932,#185933,#185934,#185935,
#185936,#185937,#185938,#185939,#185940,#185941,#185942,#185943,#185944,
#185945,#185946,#185947,#185948,#185949,#185950,#185951,#185952,#185953,
#185954,#185955,#185956,#185957,#185958,#185959,#185960,#185961,#185962,
#185963,#185964,#185965,#185966,#185967,#185968,#185969,#185970,#185971,
#185972,#185973,#185974,#185975,#185976,#185977,#185978,#185979,#185980,
#185981,#185982,#185983,#185984,#185985,#185986,#185987,#185988,#185989,
#185990,#185991,#185992,#185993,#185994,#185995,#185996,#185997,#185998,
#185999,#186000,#186001,#186002,#186003,#186004,#186005,#186006,#186007,
#186008,#186009,#186010,#186011,#186012,#186013,#186014,#186015,#186016,
#186017,#186018,#186019,#186020,#186021),.UNSPECIFIED.,.F.,.F.,(4,3,3,3,
3,3,3,3,3,3,3,3,3,3,3,3,3,3,3,3,3,3,3,3,3,3,3,3,3,3,3,3,3,3,3,3,3,3,3,3,
3,3,3,3,3,3,3,3,3,3,3,3,3,3,3,3,3,4),(15.7079632680314,15.7849793680378,
15.8619042262796,15.9387539940356,16.0155447640273,16.092293415879,16.1690200754061,
16.2457392290518,16.322465356366,16.3992465261494,16.4760567060718,16.5529541571788,
16.6087315271301,16.6889240591598,16.7690457679708,16.8491062886745,16.9291045159356,
17.0090647219482,17.0889926797773,17.1081013950612,17.1889472801389,17.2698341100947,
17.3542433983191,17.4352700475907,17.5163471563621,17.5975094504688,17.6074712629923,
17.6929123102967,17.7782763520816,17.8634875056938,17.948588813481,18.033489922678,
18.1068411309234,18.1833613696459,18.2598760582566,18.336399820006,18.4129793887368,
18.4895901232335,18.5662845487608,18.6062109988545,18.6857500135597,18.7652285718676,
18.8446589586676,18.9240534212649,19.0034241783015,19.0827960418154,19.1621705106544,
19.2415586849842,19.3209716725316,19.4004560674958,19.4799788538006,19.5595906113493,
19.6049507347167,19.6826484633713,19.760232488877,19.8377508195051,19.9152048727785,
19.9450452040236),.UNSPECIFIED.);
#3273=B_SPLINE_CURVE_WITH_KNOTS('',3,(#186027,#186028,#186029,#186030,#186031,
#186032,#186033,#186034,#186035,#186036,#186037,#186038,#186039,#186040,
#186041,#186042,#186043,#186044,#186045,#186046,#186047,#186048,#186049,
#186050,#186051,#186052,#186053,#186054,#186055,#186056,#186057,#186058,
#186059,#186060,#186061,#186062,#186063,#186064,#186065,#186066,#186067,
#186068,#186069,#186070,#186071,#186072,#186073,#186074,#186075,#186076,
#186077,#186078,#186079,#186080,#186081,#186082,#186083,#186084,#186085,
#186086,#186087,#186088,#186089,#186090,#186091,#186092,#186093,#186094,
#186095,#186096,#186097,#186098,#186099,#186100,#186101,#186102,#186103,
#186104,#186105,#186106,#186107,#186108,#186109,#186110,#186111,#186112,
#186113,#186114,#186115,#186116,#186117,#186118,#186119,#186120,#186121,
#186122,#186123,#186124,#186125,#186126,#186127,#186128,#186129,#186130,
#186131,#186132,#186133,#186134,#186135,#186136,#186137,#186138,#186139,
#186140,#186141,#186142,#186143,#186144,#186145,#186146,#186147,#186148,
#186149,#186150,#186151,#186152,#186153,#186154,#186155,#186156,#186157,
#186158,#186159,#186160,#186161,#186162,#186163,#186164,#186165,#186166,
#186167,#186168,#186169,#186170,#186171,#186172,#186173,#186174,#186175,
#186176,#186177,#186178,#186179,#186180,#186181,#186182,#186183,#186184,
#186185,#186186,#186187,#186188,#186189,#186190,#186191,#186192,#186193,
#186194,#186195),.UNSPECIFIED.,.F.,.F.,(4,3,3,3,3,3,3,3,3,3,3,3,3,3,3,3,
3,3,3,3,3,3,3,3,3,3,3,3,3,3,3,3,3,3,3,3,3,3,3,3,3,3,3,3,3,3,3,3,3,3,3,3,
3,3,3,3,4),(21.9911485751294,22.0726737883961,22.154293407887,22.2360745796861,
22.2834855566976,22.3630326170872,22.4425194078618,22.5219581940468,22.6013612031951,
22.6807406342982,22.7601213131529,22.839504673154,22.918901797279,22.99832377612,
23.0778171653712,23.1573489506337,23.236969634884,23.2822252925598,23.3598810959616,
23.4374507067199,23.5149480581544,23.5923767409349,23.6697656311381,23.7471285688627,
23.7815951604909,23.8650899412174,23.9487415907991,24.0326319574194,24.1166363736405,
24.2008273023064,24.280965028422,24.3584623761376,24.4358776955364,24.5132266162488,
24.5905247202617,24.6677875526241,24.7450435667727,24.8222987213559,24.8995670637133,
24.9768626459753,25.0542462549469,25.1316754641953,25.2092248062607,25.2797047642841,
25.3557591657399,25.4317180853077,25.5075983137797,25.5834165609126,25.6591894742179,
25.7349418055907,25.8106859395986,25.8864368811234,25.9622096389604,26.0380580195377,
26.113949162002,26.1899412660023,26.2270156338182),.UNSPECIFIED.);
#3274=B_SPLINE_CURVE_WITH_KNOTS('',3,(#186196,#186197,#186198,#186199,#186200,
#186201,#186202,#186203,#186204,#186205,#186206,#186207,#186208,#186209,
#186210,#186211,#186212,#186213,#186214,#186215,#186216,#186217,#186218,
#186219,#186220,#186221,#186222,#186223,#186224,#186225,#186226,#186227,
#186228,#186229,#186230,#186231,#186232,#186233,#186234,#186235,#186236,
#186237,#186238,#186239,#186240,#186241,#186242,#186243,#186244,#186245,
#186246,#186247,#186248,#186249,#186250,#186251,#186252,#186253,#186254,
#186255,#186256,#186257,#186258,#186259,#186260,#186261,#186262,#186263,
#186264,#186265,#186266,#186267,#186268,#186269,#186270,#186271),
 .UNSPECIFIED.,.F.,.F.,(4,3,3,3,3,3,3,3,3,3,3,3,3,3,3,3,3,3,3,3,3,3,3,3,
3,4),(19.9446380862602,20.0270996900187,20.1095606278978,20.1920209272959,
20.274480615609,20.3569397202312,20.4393982685543,20.5218562879684,20.6043138058615,
20.6909909789407,20.7734577645493,20.8559228776805,20.9383864279875,21.0208485251015,
21.1033092786334,21.1857687981754,21.2682271933024,21.3506845735733,21.4331509593925,
21.5156141610166,21.5980746169651,21.6805327656015,21.7629983696133,21.8454582481907,
21.9279223599272,21.9911485751294),.UNSPECIFIED.);
#3275=B_SPLINE_CURVE_WITH_KNOTS('',3,(#186273,#186274,#186275,#186276,#186277,
#186278,#186279,#186280,#186281,#186282,#186283,#186284,#186285,#186286,
#186287,#186288,#186289,#186290,#186291,#186292,#186293,#186294,#186295,
#186296,#186297,#186298,#186299,#186300,#186301,#186302,#186303,#186304,
#186305,#186306,#186307,#186308,#186309,#186310,#186311,#186312,#186313,
#186314,#186315,#186316,#186317,#186318,#186319,#186320,#186321,#186322,
#186323,#186324,#186325,#186326,#186327,#186328,#186329,#186330,#186331,
#186332,#186333,#186334,#186335,#186336,#186337,#186338,#186339,#186340,
#186341,#186342,#186343,#186344,#186345,#186346,#186347,#186348,#186349,
#186350,#186351),.UNSPECIFIED.,.F.,.F.,(4,3,3,3,3,3,3,3,3,3,3,3,3,3,3,3,
3,3,3,3,3,3,3,3,3,3,4),(19.9450452040236,20.0246829033357,20.1043206026478,
20.1877984857314,20.271432448796,20.3553042128251,20.4392896029479,20.5234611307425,
20.6036904705788,20.6811895841971,20.758606693462,20.8359574260042,20.9132573618335,
20.9905220440399,21.0677799289761,21.1450369669192,21.2223072034865,21.2996046890923,
21.3769902053478,21.4544213269495,21.5319725714035,21.602430206441,21.6880000236565,
21.7731542207063,21.8580499988725,21.9425343151533,21.9911485750218),
 .UNSPECIFIED.);
#3276=B_SPLINE_CURVE_WITH_KNOTS('',3,(#186352,#186353,#186354,#186355,#186356,
#186357,#186358,#186359,#186360,#186361,#186362,#186363,#186364,#186365,
#186366,#186367,#186368,#186369,#186370,#186371,#186372,#186373,#186374,
#186375,#186376,#186377,#186378,#186379,#186380,#186381,#186382,#186383,
#186384,#186385,#186386,#186387,#186388,#186389,#186390,#186391,#186392,
#186393,#186394,#186395,#186396,#186397,#186398,#186399,#186400,#186401,
#186402,#186403,#186404,#186405,#186406,#186407,#186408,#186409,#186410,
#186411,#186412,#186413,#186414,#186415,#186416,#186417,#186418,#186419,
#186420,#186421,#186422,#186423,#186424,#186425,#186426,#186427,#186428,
#186429,#186430,#186431,#186432,#186433,#186434,#186435,#186436,#186437,
#186438,#186439,#186440,#186441,#186442,#186443,#186444,#186445,#186446,
#186447,#186448,#186449,#186450,#186451,#186452,#186453,#186454,#186455,
#186456,#186457,#186458,#186459,#186460,#186461,#186462,#186463,#186464,
#186465,#186466,#186467,#186468,#186469,#186470,#186471,#186472,#186473,
#186474,#186475,#186476,#186477,#186478,#186479,#186480,#186481,#186482,
#186483,#186484,#186485,#186486,#186487,#186488,#186489,#186490,#186491,
#186492,#186493,#186494,#186495,#186496,#186497,#186498,#186499,#186500,
#186501,#186502,#186503,#186504,#186505,#186506,#186507,#186508,#186509,
#186510,#186511,#186512,#186513,#186514,#186515,#186516,#186517),
 .UNSPECIFIED.,.F.,.F.,(4,3,3,3,3,3,3,3,3,3,3,3,3,3,3,3,3,3,3,3,3,3,3,3,
3,3,3,3,3,3,3,3,3,3,3,3,3,3,3,3,3,3,3,3,3,3,3,3,3,3,3,3,3,3,3,4),(21.9911485751293,
22.0674915472375,22.1438420973543,22.2202147938274,22.2966242166123,22.3731393315767,
22.4497090626853,22.5264184263459,22.6011699423032,22.6797052338162,22.758147708736,
22.8365118763931,22.9148121906576,22.9930630597149,23.0712819476143,23.1494841985966,
23.2276828124449,23.3058907843889,23.3841537662605,23.462445209092,23.5408203684972,
23.5999096781654,23.6795524499783,23.7591249324589,23.8386380197198,23.9180942011272,
23.9975162177901,24.0769137064076,24.0992795460965,24.180509249891,24.2617877412199,
24.3460031594218,24.4274336038537,24.5130415089407,24.5986494140276,24.6838926817792,
24.7690577231954,24.8540720556098,24.9389793277104,25.0236937917839,25.0980192819587,
25.1745623672306,25.2510999951783,25.3276467728086,25.4042493995774,25.4808832323577,
25.5576007087503,25.5973891498898,25.6769295574756,25.7564129775381,25.8358505730622,
25.9152534756883,25.9946399097677,26.0740134122289,26.1534040307968,26.2275350298928),
 .UNSPECIFIED.);
#3277=B_SPLINE_CURVE_WITH_KNOTS('',3,(#186523,#186524,#186525,#186526,#186527,
#186528,#186529,#186530,#186531,#186532,#186533,#186534,#186535,#186536,
#186537,#186538,#186539,#186540,#186541,#186542,#186543,#186544,#186545,
#186546,#186547,#186548,#186549,#186550,#186551,#186552,#186553,#186554,
#186555,#186556,#186557,#186558,#186559,#186560,#186561,#186562,#186563,
#186564,#186565,#186566,#186567,#186568,#186569,#186570,#186571,#186572,
#186573,#186574,#186575,#186576,#186577,#186578,#186579,#186580,#186581,
#186582,#186583,#186584,#186585,#186586,#186587,#186588,#186589,#186590,
#186591,#186592,#186593,#186594,#186595,#186596,#186597,#186598,#186599,
#186600,#186601,#186602,#186603,#186604,#186605,#186606,#186607,#186608,
#186609,#186610,#186611,#186612,#186613,#186614,#186615,#186616,#186617,
#186618,#186619,#186620,#186621,#186622,#186623,#186624,#186625,#186626,
#186627,#186628,#186629,#186630,#186631,#186632,#186633,#186634,#186635,
#186636,#186637,#186638,#186639,#186640,#186641,#186642,#186643,#186644,
#186645,#186646,#186647,#186648,#186649,#186650,#186651,#186652,#186653,
#186654,#186655,#186656,#186657,#186658,#186659,#186660,#186661,#186662,
#186663,#186664,#186665,#186666,#186667,#186668,#186669,#186670,#186671,
#186672,#186673,#186674,#186675,#186676,#186677,#186678,#186679,#186680,
#186681,#186682,#186683,#186684,#186685,#186686,#186687,#186688,#186689,
#186690,#186691,#186692,#186693,#186694),.UNSPECIFIED.,.F.,.F.,(4,3,3,3,
3,3,3,3,3,3,3,3,3,3,3,3,3,3,3,3,3,3,3,3,3,3,3,3,3,3,3,3,3,3,3,3,3,3,3,3,
3,3,3,3,3,3,3,3,3,3,3,3,3,3,3,3,3,4),(28.274333882309,28.2759239718707,
28.3611672689883,28.4463323419476,28.5313467086318,28.6162540162447,28.7009685173684,
28.7752938398018,28.8518368432037,28.9283743879683,29.0049210811626,29.0815236218832,
29.1581573676352,29.2348747559209,29.2746637077329,29.3542108077167,29.4336976389849,
29.5131364664643,29.5925395176092,29.6719189913133,29.7512997134264,29.8306831170345,
29.9100802850296,29.9895023079184,30.0689957411893,30.1485275704695,30.2281482983423,
30.2734034435951,30.3510592018246,30.4286287675895,30.506126074255,30.5835547127227,
30.6609435588824,30.7383064530928,30.7727733115261,30.8562681185707,30.9399197955601,
31.0238101908009,31.1078146361851,31.1920055944091,31.2721431794572,31.3496405261199,
31.4270558444663,31.5044047641279,31.5817028670928,31.6589656984109,31.7362217115251,
31.8134768650799,31.8907452064159,31.9680407876647,32.0454243956414,32.1228536039036,
32.2004029450071,32.2708829153194,32.3469363365831,32.4229060797825,32.4987893170115,
32.5119151775653),.UNSPECIFIED.);
#3278=B_SPLINE_CURVE_WITH_KNOTS('',3,(#186695,#186696,#186697,#186698,#186699,
#186700,#186701,#186702,#186703,#186704,#186705,#186706,#186707,#186708,
#186709,#186710,#186711,#186712,#186713,#186714,#186715,#186716,#186717,
#186718,#186719,#186720,#186721,#186722,#186723,#186724,#186725,#186726,
#186727,#186728,#186729,#186730,#186731,#186732,#186733,#186734,#186735,
#186736,#186737,#186738,#186739,#186740,#186741,#186742,#186743,#186744,
#186745,#186746,#186747,#186748,#186749,#186750,#186751,#186752,#186753,
#186754,#186755,#186756,#186757,#186758,#186759,#186760,#186761,#186762,
#186763,#186764,#186765,#186766,#186767,#186768,#186769,#186770,#186771,
#186772,#186773,#186774,#186775,#186776),.UNSPECIFIED.,.F.,.F.,(4,3,3,3,
3,3,3,3,3,3,3,3,3,3,3,3,3,3,3,3,3,3,3,3,3,3,3,4),(26.2270156338182,26.2784445001463,
26.3569804390247,26.4354235674566,26.5137883938099,26.5920893709949,26.6703409062375,
26.7485604625677,26.8267633829094,26.9049626661928,26.9831713067947,27.0614349524559,
27.1397270569375,27.2181028689108,27.2771842360085,27.356826142552,27.4363977624051,
27.5159099914782,27.5953653252633,27.6747865014101,27.7541831630675,27.7765541039396,
27.8577521425003,27.938998564499,28.0228323939217,28.1042298637321,28.189281872961,
28.2743338821898),.UNSPECIFIED.);
#3279=B_SPLINE_CURVE_WITH_KNOTS('',3,(#186778,#186779,#186780,#186781,#186782,
#186783,#186784,#186785,#186786,#186787,#186788,#186789,#186790,#186791,
#186792,#186793,#186794,#186795,#186796,#186797,#186798,#186799,#186800,
#186801,#186802,#186803,#186804,#186805,#186806,#186807,#186808,#186809,
#186810,#186811,#186812,#186813,#186814,#186815,#186816,#186817,#186818,
#186819,#186820,#186821,#186822,#186823,#186824,#186825,#186826,#186827,
#186828,#186829,#186830,#186831,#186832,#186833,#186834,#186835,#186836,
#186837,#186838,#186839,#186840,#186841,#186842,#186843,#186844,#186845,
#186846,#186847,#186848,#186849,#186850,#186851,#186852,#186853,#186854,
#186855,#186856,#186857,#186858,#186859),.UNSPECIFIED.,.F.,.F.,(4,3,3,3,
3,3,3,3,3,3,3,3,3,3,3,3,3,3,3,3,3,3,3,3,3,3,3,4),(26.2275350298928,26.3069550152091,
26.3864462180847,26.4659751401512,26.5455941531207,26.5961288857519,26.6737846891537,
26.7513542999119,26.8288516513463,26.9062803341267,26.9836692243299,27.0610321620547,
27.095498753683,27.1789935344097,27.2626451839921,27.3465355506126,27.4305399668345,
27.5147308955004,27.5948686216141,27.6711802459415,27.7473856470892,27.8235298949968,
27.8996279536925,27.9756947522701,28.0517610378082,28.1278240927466,28.2039301637871,
28.2743338823088),.UNSPECIFIED.);
#3280=B_SPLINE_CURVE_WITH_KNOTS('',3,(#186860,#186861,#186862,#186863,#186864,
#186865,#186866,#186867,#186868,#186869,#186870,#186871,#186872,#186873,
#186874,#186875,#186876,#186877,#186878,#186879,#186880,#186881,#186882,
#186883,#186884,#186885,#186886,#186887,#186888,#186889,#186890,#186891,
#186892,#186893,#186894,#186895,#186896,#186897,#186898,#186899,#186900,
#186901,#186902,#186903,#186904,#186905,#186906,#186907,#186908,#186909,
#186910,#186911,#186912,#186913,#186914,#186915,#186916,#186917,#186918,
#186919,#186920,#186921,#186922,#186923,#186924,#186925,#186926,#186927,
#186928,#186929,#186930,#186931,#186932,#186933,#186934,#186935,#186936,
#186937,#186938,#186939,#186940,#186941,#186942,#186943,#186944,#186945,
#186946,#186947,#186948,#186949,#186950,#186951,#186952,#186953,#186954,
#186955,#186956,#186957,#186958,#186959,#186960,#186961,#186962,#186963,
#186964,#186965,#186966,#186967,#186968,#186969,#186970,#186971,#186972,
#186973,#186974,#186975,#186976,#186977,#186978,#186979,#186980,#186981,
#186982,#186983,#186984,#186985,#186986,#186987,#186988,#186989,#186990,
#186991,#186992,#186993,#186994,#186995,#186996,#186997,#186998,#186999,
#187000,#187001,#187002,#187003,#187004,#187005,#187006,#187007,#187008,
#187009,#187010,#187011,#187012,#187013,#187014,#187015,#187016,#187017,
#187018,#187019,#187020,#187021,#187022,#187023,#187024,#187025,#187026,
#187027,#187028),.UNSPECIFIED.,.F.,.F.,(4,3,3,3,3,3,3,3,3,3,3,3,3,3,3,3,
3,3,3,3,3,3,3,3,3,3,3,3,3,3,3,3,3,3,3,3,3,3,3,3,3,3,3,3,3,3,3,3,3,3,3,3,
3,3,3,3,4),(28.2743338824115,28.3702372203524,28.4672653007767,28.5654433825602,
28.5936083574763,28.669659806962,28.7456163996417,28.8214949223753,28.8973120818936,
28.9730845234877,29.050492469719,29.1262405199265,29.2019965838076,29.2777756722776,
29.3564187775428,29.4323316922924,29.5083020741959,29.584379569782,29.5923480933385,
29.6708840322169,29.7493271606488,29.8276919870021,29.9059929641869,29.9842444994295,
30.0624640557597,30.1406669761014,30.2188662593847,30.2970748999866,30.3753385456478,
30.4536306501294,30.5320064621028,30.5910878292007,30.6707297357442,30.7503013555972,
30.8298135846705,30.9092689184556,30.9886900946024,31.0680867562597,31.0904576971318,
31.1716877944818,31.2529666862774,31.3371819059738,31.4186127601752,31.504220162619,
31.5898275650629,31.6750708621805,31.7602359351399,31.8452503018241,31.9301576094371,
32.0148721105607,32.0891974329939,32.165737337151,32.2422704943354,32.3188353761641,
32.3954178255919,32.4720627947504,32.5104908631869),.UNSPECIFIED.);
#3281=B_SPLINE_CURVE_WITH_KNOTS('',3,(#187034,#187035,#187036,#187037,#187038,
#187039,#187040,#187041,#187042,#187043,#187044,#187045,#187046,#187047,
#187048,#187049,#187050,#187051,#187052,#187053,#187054,#187055,#187056,
#187057,#187058,#187059,#187060,#187061,#187062,#187063,#187064,#187065,
#187066,#187067,#187068,#187069,#187070,#187071,#187072,#187073,#187074,
#187075,#187076,#187077,#187078,#187079,#187080,#187081,#187082,#187083,
#187084,#187085,#187086,#187087,#187088,#187089,#187090,#187091,#187092,
#187093,#187094,#187095,#187096,#187097,#187098,#187099,#187100,#187101,
#187102,#187103,#187104,#187105,#187106,#187107,#187108,#187109,#187110,
#187111,#187112,#187113,#187114,#187115,#187116,#187117,#187118,#187119,
#187120,#187121,#187122,#187123,#187124,#187125,#187126,#187127,#187128,
#187129,#187130,#187131,#187132,#187133,#187134,#187135,#187136,#187137,
#187138,#187139,#187140,#187141,#187142,#187143,#187144,#187145,#187146,
#187147,#187148,#187149,#187150,#187151,#187152,#187153,#187154,#187155,
#187156,#187157,#187158,#187159,#187160,#187161,#187162,#187163,#187164,
#187165,#187166,#187167,#187168,#187169,#187170,#187171,#187172,#187173,
#187174,#187175,#187176,#187177,#187178,#187179,#187180,#187181,#187182,
#187183,#187184,#187185,#187186,#187187,#187188,#187189,#187190,#187191,
#187192,#187193,#187194,#187195,#187196,#187197,#187198,#187199),
 .UNSPECIFIED.,.F.,.F.,(4,3,3,3,3,3,3,3,3,3,3,3,3,3,3,3,3,3,3,3,3,3,3,3,
3,3,3,3,3,3,3,3,3,3,3,3,3,3,3,3,3,3,3,3,3,3,3,3,3,3,3,3,3,3,3,4),(34.5575191896334,
34.6328940346518,34.7082620826187,34.7677322549749,34.8489623516055,34.9302412426614,
35.0144564627225,35.0958873161479,35.181494719527,35.267102122906,35.3523454212009,
35.4375104953517,35.5225248632253,35.6074321720173,35.6921466742857,35.7664719908371,
35.8430149938238,35.9195525381677,35.9960992309372,36.0727017712263,36.1493355165433,
36.2260529043906,36.2658418587681,36.3453889588483,36.4248757902154,36.5043146177953,
36.583717669043,36.6630971428506,36.7424778650691,36.8218612687835,36.9012584368857,
36.980680459882,37.0601738932601,37.1397057226475,37.2193264506264,37.2645815946303,
37.3422373528249,37.4198069185552,37.4973042251867,37.5747328636208,37.6521217097477,
37.7294846039253,37.7639514625614,37.8474462696074,37.9310979465984,38.0149883418392,
38.0989927872228,38.1831837454459,38.2633213304925,38.3408158465093,38.4182316833689,
38.4955830039888,38.5728791596455,38.650142327992,38.7273960430041,38.7941774417346),
 .UNSPECIFIED.);
#3282=B_SPLINE_CURVE_WITH_KNOTS('',3,(#187200,#187201,#187202,#187203,#187204,
#187205,#187206,#187207,#187208,#187209,#187210,#187211,#187212,#187213,
#187214,#187215,#187216,#187217,#187218,#187219,#187220,#187221,#187222,
#187223,#187224,#187225,#187226,#187227,#187228,#187229,#187230,#187231,
#187232,#187233,#187234,#187235,#187236,#187237,#187238,#187239,#187240,
#187241,#187242,#187243,#187244,#187245,#187246,#187247,#187248,#187249,
#187250,#187251,#187252,#187253,#187254,#187255,#187256,#187257,#187258,
#187259,#187260,#187261,#187262,#187263,#187264,#187265,#187266,#187267,
#187268,#187269,#187270,#187271,#187272,#187273,#187274,#187275,#187276,
#187277,#187278,#187279,#187280,#187281),.UNSPECIFIED.,.F.,.F.,(4,3,3,3,
3,3,3,3,3,3,3,3,3,3,3,3,3,3,3,3,3,3,3,3,3,3,3,4),(32.5119151775653,32.5877233929837,
32.6634897706898,32.7392563807513,32.8150046791788,32.8907632674804,32.9665471583332,
33.0424205102964,33.118339341866,33.1943848037333,33.2696226511816,33.3481585912356,
33.4266017208537,33.5049665484019,33.5832675267887,33.6615190632388,33.7397386207794,
33.8179415423325,33.8961408268268,33.9743494686376,34.0526131154981,34.1309052211746,
34.2092810343257,34.2683623870438,34.3540517742216,34.4396129126855,34.5249606887323,
34.5575191894886),.UNSPECIFIED.);
#3283=B_SPLINE_CURVE_WITH_KNOTS('',3,(#187283,#187284,#187285,#187286,#187287,
#187288,#187289,#187290,#187291,#187292,#187293,#187294,#187295,#187296,
#187297,#187298,#187299,#187300,#187301,#187302,#187303,#187304,#187305,
#187306,#187307,#187308,#187309,#187310,#187311,#187312,#187313,#187314,
#187315,#187316,#187317,#187318,#187319,#187320,#187321,#187322,#187323,
#187324,#187325,#187326,#187327,#187328,#187329,#187330,#187331,#187332,
#187333,#187334,#187335,#187336,#187337,#187338,#187339,#187340,#187341,
#187342,#187343,#187344,#187345,#187346,#187347,#187348,#187349,#187350,
#187351,#187352,#187353,#187354,#187355,#187356,#187357,#187358,#187359,
#187360,#187361,#187362,#187363,#187364),.UNSPECIFIED.,.F.,.F.,(4,3,3,3,
3,3,3,3,3,3,3,3,3,3,3,3,3,3,3,3,3,3,3,3,3,3,3,4),(32.5104908631869,32.588567300925,
32.6681144009088,32.7476012321771,32.8270400596564,32.9064431108012,32.9858225845053,
33.0652033066184,33.1445867102266,33.2239838782218,33.3034059011105,33.3828993343814,
33.4624311636617,33.5420518915345,33.5873070367872,33.6649627950167,33.7425323607817,
33.8200296674471,33.8974583059148,33.9748471520747,34.0522100462851,34.0866769047183,
34.1690285568191,34.2515062577281,34.3341851486432,34.4169666610317,34.4999193372927,
34.5575191894884),.UNSPECIFIED.);
#3284=B_SPLINE_CURVE_WITH_KNOTS('',3,(#187365,#187366,#187367,#187368,#187369,
#187370,#187371,#187372,#187373,#187374,#187375,#187376,#187377,#187378,
#187379,#187380,#187381,#187382,#187383,#187384,#187385,#187386,#187387,
#187388,#187389,#187390,#187391,#187392,#187393,#187394,#187395,#187396,
#187397,#187398,#187399,#187400,#187401,#187402,#187403,#187404,#187405,
#187406,#187407,#187408,#187409,#187410,#187411,#187412,#187413,#187414,
#187415,#187416,#187417,#187418,#187419,#187420,#187421,#187422,#187423,
#187424,#187425,#187426,#187427,#187428,#187429,#187430,#187431,#187432,
#187433,#187434,#187435,#187436,#187437,#187438,#187439,#187440,#187441,
#187442,#187443,#187444,#187445,#187446,#187447,#187448,#187449,#187450,
#187451,#187452,#187453,#187454,#187455,#187456,#187457,#187458,#187459,
#187460,#187461,#187462,#187463,#187464,#187465,#187466,#187467,#187468,
#187469,#187470,#187471,#187472,#187473,#187474,#187475,#187476,#187477,
#187478,#187479,#187480,#187481,#187482,#187483,#187484,#187485,#187486,
#187487,#187488,#187489,#187490,#187491,#187492,#187493,#187494,#187495,
#187496,#187497,#187498,#187499,#187500,#187501,#187502,#187503,#187504,
#187505,#187506,#187507,#187508,#187509,#187510,#187511,#187512,#187513,
#187514,#187515,#187516,#187517,#187518,#187519,#187520,#187521,#187522,
#187523,#187524,#187525,#187526,#187527,#187528,#187529,#187530,#187531,
#187532,#187533,#187534,#187535,#187536),.UNSPECIFIED.,.F.,.F.,(4,3,3,3,
3,3,3,3,3,3,3,3,3,3,3,3,3,3,3,3,3,3,3,3,3,3,3,3,3,3,3,3,3,3,3,3,3,3,3,3,
3,3,3,3,3,3,3,3,3,3,3,3,3,3,3,3,3,4),(34.5575191895731,34.5860467726494,
34.6635441193121,34.7409594376583,34.8183083573198,34.8956064602846,34.9728692916032,
35.0501253047173,35.1273804582721,35.2046487996079,35.2819443808566,35.3593279888334,
35.4367571970956,35.5143065381991,35.5847865085116,35.6608379562356,35.7367945471342,
35.8126730680686,35.8884902257706,35.9642626655325,36.0416706128877,36.117418661229,
36.1931747232324,36.2689538098139,36.3475969184539,36.4235098313013,36.499480211296,
36.5755577049752,36.5835262443738,36.6620621844278,36.7405053140459,36.8188701415938,
36.8971711199808,36.9754226564305,37.0536422139711,37.1318451355242,37.2100444200183,
37.288253061829,37.3665167086894,37.4448088143658,37.5231846275169,37.582265980236,
37.6619078866581,37.7414795063955,37.8209917353596,37.9004470690454,37.9798682450988,
38.0592649066717,38.081635848167,38.1628659447976,38.244144835853,38.3283600559143,
38.4097909093397,38.4953983127189,38.5810057160981,38.6662559661317,38.7514079237039,
38.7947201030774),.UNSPECIFIED.);
#3285=B_SPLINE_CURVE_WITH_KNOTS('',3,(#187542,#187543,#187544,#187545,#187546,
#187547,#187548,#187549,#187550,#187551,#187552,#187553,#187554,#187555,
#187556,#187557,#187558,#187559,#187560,#187561,#187562,#187563,#187564,
#187565,#187566,#187567,#187568,#187569,#187570,#187571,#187572,#187573,
#187574,#187575,#187576,#187577,#187578,#187579,#187580,#187581,#187582,
#187583,#187584,#187585,#187586,#187587,#187588,#187589,#187590,#187591,
#187592,#187593,#187594,#187595,#187596,#187597,#187598,#187599,#187600,
#187601,#187602,#187603,#187604,#187605,#187606,#187607,#187608,#187609,
#187610,#187611,#187612,#187613,#187614,#187615,#187616,#187617,#187618,
#187619,#187620,#187621,#187622,#187623,#187624,#187625,#187626,#187627,
#187628,#187629,#187630,#187631,#187632,#187633,#187634,#187635,#187636,
#187637,#187638,#187639,#187640,#187641,#187642,#187643,#187644,#187645,
#187646,#187647,#187648,#187649,#187650,#187651,#187652,#187653,#187654,
#187655,#187656,#187657,#187658,#187659,#187660,#187661,#187662,#187663,
#187664,#187665,#187666,#187667,#187668,#187669,#187670,#187671,#187672,
#187673,#187674,#187675,#187676,#187677,#187678,#187679,#187680,#187681,
#187682,#187683,#187684,#187685,#187686,#187687,#187688,#187689,#187690,
#187691,#187692,#187693,#187694,#187695,#187696,#187697,#187698,#187699,
#187700,#187701,#187702,#187703,#187704,#187705,#187706,#187707),
 .UNSPECIFIED.,.F.,.F.,(4,3,3,3,3,3,3,3,3,3,3,3,3,3,3,3,3,3,3,3,3,3,3,3,
3,3,3,3,3,3,3,3,3,3,3,3,3,3,3,3,3,3,3,3,3,3,3,3,3,3,3,3,3,3,3,4),(40.840704496776,
40.9237050242495,41.0076639027069,41.0909770223219,41.1752587802005,41.2595405380791,
41.3391824445055,41.4187540642474,41.4982662932161,41.5777216269065,41.657142802964,
41.736539464541,41.7589104060102,41.840140502636,41.9214193936874,42.0056346137509,
42.0870654671712,42.1726728705562,42.2582802739413,42.3435235722402,42.4286886463948,
42.5137030142724,42.5986103230683,42.6833248253405,42.7576501418723,42.8341931448579,
42.910730689201,42.9872773819693,43.0638799222574,43.1405136675733,43.2172310554195,
43.2570200098034,43.3365671098839,43.4160539412511,43.4954927688313,43.5748958200785,
43.654275293886,43.7336560161045,43.8130394198191,43.892436587921,43.9718586109174,
44.0513520442956,44.1308838736832,44.2105046016622,44.2557597456656,44.3334155038604,
44.4109850695909,44.488482376222,44.5659110146563,44.643299860783,44.7206627549609,
44.7551296135967,44.8386682155131,44.9223372298337,45.0062151375915,45.0768851922591),
 .UNSPECIFIED.);
#3286=B_SPLINE_CURVE_WITH_KNOTS('',3,(#187708,#187709,#187710,#187711,#187712,
#187713,#187714,#187715,#187716,#187717,#187718,#187719,#187720,#187721,
#187722,#187723,#187724,#187725,#187726,#187727,#187728,#187729,#187730,
#187731,#187732,#187733,#187734,#187735,#187736,#187737,#187738,#187739,
#187740,#187741,#187742,#187743,#187744,#187745,#187746,#187747,#187748,
#187749,#187750,#187751,#187752,#187753,#187754,#187755,#187756,#187757,
#187758,#187759,#187760,#187761,#187762,#187763,#187764,#187765,#187766,
#187767,#187768,#187769,#187770,#187771,#187772,#187773,#187774,#187775,
#187776,#187777,#187778,#187779,#187780,#187781,#187782,#187783,#187784,
#187785,#187786,#187787,#187788,#187789),.UNSPECIFIED.,.F.,.F.,(4,3,3,3,
3,3,3,3,3,3,3,3,3,3,3,3,3,3,3,3,3,3,3,3,3,3,3,4),(38.7941774417346,38.8714431711455,
38.9487342341965,39.027065942236,39.1044888483819,39.1832749573683,39.2620610663547,
39.3381125140738,39.4140691049675,39.4899476258966,39.5657647835933,39.6415372233501,
39.7189451707085,39.7946932190448,39.8704492810428,39.9462283676192,40.0248714762686,
40.1007843891105,40.1767547690997,40.2528322627735,40.2608008022169,40.3424778464143,
40.4240390918976,40.5054902891725,40.5892938410464,40.6705052510868,40.7556048738775,
40.8407044966682),.UNSPECIFIED.);
#3287=B_SPLINE_CURVE_WITH_KNOTS('',3,(#187791,#187792,#187793,#187794,#187795,
#187796,#187797,#187798,#187799,#187800,#187801,#187802,#187803,#187804,
#187805,#187806,#187807,#187808,#187809,#187810,#187811,#187812,#187813,
#187814,#187815,#187816,#187817,#187818,#187819,#187820,#187821,#187822,
#187823,#187824,#187825,#187826,#187827,#187828,#187829,#187830,#187831,
#187832,#187833,#187834,#187835,#187836,#187837,#187838,#187839,#187840,
#187841,#187842,#187843,#187844,#187845,#187846,#187847,#187848,#187849,
#187850,#187851,#187852,#187853,#187854,#187855,#187856,#187857,#187858,
#187859,#187860,#187861,#187862,#187863,#187864,#187865,#187866,#187867,
#187868,#187869,#187870,#187871,#187872),.UNSPECIFIED.,.F.,.F.,(4,3,3,3,
3,3,3,3,3,3,3,3,3,3,3,3,3,3,3,3,3,3,3,3,3,3,3,4),(38.7947201030774,38.8796814331916,
38.9645296960449,39.0491959488369,39.0803755840292,39.1569185870159,39.2334561313597,
39.3100028241287,39.3866053644178,39.4632391097346,39.5399564975818,39.5797454519603,
39.6592925520407,39.7387793834081,39.8182182109875,39.897621262235,39.9770007360423,
40.0563814582608,40.1357648619751,40.2151620300772,40.2945840530733,40.3740774864513,
40.4536093158385,40.5332300438175,40.5784851878225,40.6649478372961,40.752826166982,
40.840704496668),.UNSPECIFIED.);
#3288=B_SPLINE_CURVE_WITH_KNOTS('',3,(#187873,#187874,#187875,#187876,#187877,
#187878,#187879,#187880,#187881,#187882,#187883,#187884,#187885,#187886,
#187887,#187888,#187889,#187890,#187891,#187892,#187893,#187894,#187895,
#187896,#187897,#187898,#187899,#187900,#187901,#187902,#187903,#187904,
#187905,#187906,#187907,#187908,#187909,#187910,#187911,#187912,#187913,
#187914,#187915,#187916,#187917,#187918,#187919,#187920,#187921,#187922,
#187923,#187924,#187925,#187926,#187927,#187928,#187929,#187930,#187931,
#187932,#187933,#187934,#187935,#187936,#187937,#187938,#187939,#187940,
#187941,#187942,#187943,#187944,#187945,#187946,#187947,#187948,#187949,
#187950,#187951,#187952,#187953,#187954,#187955,#187956,#187957,#187958,
#187959,#187960,#187961,#187962,#187963,#187964,#187965,#187966,#187967,
#187968,#187969,#187970,#187971,#187972,#187973,#187974,#187975,#187976,
#187977,#187978,#187979,#187980,#187981,#187982,#187983,#187984,#187985,
#187986,#187987,#187988,#187989,#187990,#187991,#187992,#187993,#187994,
#187995,#187996,#187997,#187998,#187999,#188000,#188001,#188002,#188003,
#188004,#188005,#188006,#188007,#188008,#188009,#188010,#188011,#188012,
#188013,#188014,#188015,#188016,#188017,#188018,#188019,#188020,#188021,
#188022,#188023,#188024,#188025,#188026,#188027,#188028,#188029),
 .UNSPECIFIED.,.F.,.F.,(4,3,3,3,3,3,3,3,3,3,3,3,3,3,3,3,3,3,3,3,3,3,3,3,
3,3,3,3,3,3,3,3,3,3,3,3,3,3,3,3,3,3,3,3,3,3,3,3,3,3,3,3,4),(40.840704496668,
40.9231667027535,41.0056285605417,41.0880900768827,41.1705512586267,41.2530121126234,
41.3354726457222,41.4179328647724,41.5003927766228,41.5828523881221,41.6653117061188,
41.7477707374609,41.8302294889962,41.9126879675725,41.9951461800371,42.0776041332372,
42.1600618340199,42.2425192892318,42.3249765057192,42.4109890935085,42.4943137879295,
42.5767803934878,42.6592461548385,42.7417110993968,42.8241752545748,42.906638647782,
42.9891013064255,43.0715632579094,43.1540245296357,43.2364851490039,43.3189451434111,
43.4014045402525,43.4838633669209,43.5663216508072,43.6487794193006,43.7312366997883,
43.8153706132377,43.8978366115361,43.9803009880848,44.0627638525268,44.1452253144836,
44.2276854835575,44.3101444693322,44.3926023813751,44.4781994980755,44.5606642350192,
44.6431260073173,44.7255852534083,44.808042411587,44.8905049304858,44.9729626017693,
45.0554213926776,45.0773793149784),.UNSPECIFIED.);
#3289=B_SPLINE_CURVE_WITH_KNOTS('',3,(#188035,#188036,#188037,#188038,#188039,
#188040,#188041,#188042,#188043,#188044,#188045,#188046,#188047,#188048,
#188049,#188050,#188051,#188052,#188053,#188054,#188055,#188056,#188057,
#188058,#188059,#188060,#188061,#188062,#188063,#188064,#188065,#188066,
#188067,#188068,#188069,#188070,#188071,#188072,#188073,#188074,#188075,
#188076,#188077,#188078,#188079,#188080,#188081,#188082,#188083,#188084,
#188085,#188086,#188087,#188088,#188089,#188090,#188091,#188092,#188093,
#188094,#188095,#188096,#188097,#188098,#188099,#188100,#188101,#188102,
#188103,#188104,#188105,#188106,#188107,#188108,#188109,#188110,#188111,
#188112,#188113,#188114,#188115,#188116,#188117,#188118,#188119,#188120,
#188121,#188122,#188123,#188124,#188125,#188126,#188127,#188128,#188129,
#188130,#188131,#188132,#188133,#188134,#188135,#188136,#188137,#188138,
#188139,#188140,#188141,#188142,#188143,#188144,#188145,#188146,#188147,
#188148,#188149,#188150,#188151,#188152,#188153,#188154,#188155,#188156,
#188157,#188158,#188159,#188160,#188161,#188162,#188163,#188164,#188165,
#188166,#188167,#188168,#188169,#188170,#188171,#188172,#188173,#188174,
#188175,#188176,#188177,#188178,#188179,#188180,#188181,#188182,#188183,
#188184,#188185,#188186,#188187,#188188,#188189,#188190,#188191,#188192,
#188193,#188194,#188195,#188196,#188197,#188198,#188199,#188200),
 .UNSPECIFIED.,.F.,.F.,(4,3,3,3,3,3,3,3,3,3,3,3,3,3,3,3,3,3,3,3,3,3,3,3,
3,3,3,3,3,3,3,3,3,3,3,3,3,3,3,3,3,3,3,3,3,3,3,3,3,3,3,3,3,3,3,4),(47.1238898038478,
47.2519789532522,47.3305148933068,47.4089580229256,47.4873228504744,47.5656238288619,
47.6438753653124,47.7220949228536,47.8002978444074,47.8784971289024,47.9567057707139,
48.0349694175751,48.1132615232523,48.191637336404,48.2507186891144,48.3303605955408,
48.4099322152827,48.4894444442513,48.5688997779416,48.6483209539991,48.7277176155761,
48.7500885570454,48.8313186536713,48.9125975447225,48.996812764786,49.0782436182063,
49.1638510215914,49.2494584249765,49.3347017232755,49.4198667974303,49.5048811653079,
49.5897884741038,49.674502976376,49.7488282929076,49.8253712958932,49.9019088402362,
49.9784555330044,50.0550580732925,50.1316918186085,50.2084092064547,50.2481981608387,
50.3277452609192,50.4072320922864,50.4866709198666,50.566073971114,50.6454534449221,
50.7248341671407,50.8042175708552,50.8836147389574,50.9630367619537,51.0425301953319,
51.1220620247194,51.2016827526985,51.2469378967009,51.3245982517907,51.3612654433028),
 .UNSPECIFIED.);
#3290=B_SPLINE_CURVE_WITH_KNOTS('',3,(#188201,#188202,#188203,#188204,#188205,
#188206,#188207,#188208,#188209,#188210,#188211,#188212,#188213,#188214,
#188215,#188216,#188217,#188218,#188219,#188220,#188221,#188222,#188223,
#188224,#188225,#188226,#188227,#188228,#188229,#188230,#188231,#188232,
#188233,#188234,#188235,#188236,#188237,#188238,#188239,#188240,#188241,
#188242,#188243,#188244,#188245,#188246,#188247,#188248,#188249,#188250,
#188251,#188252,#188253,#188254,#188255,#188256,#188257,#188258,#188259,
#188260,#188261,#188262,#188263,#188264,#188265,#188266,#188267,#188268,
#188269,#188270,#188271,#188272,#188273,#188274,#188275,#188276,#188277,
#188278,#188279,#188280,#188281,#188282,#188283,#188284,#188285),
 .UNSPECIFIED.,.F.,.F.,(4,3,3,3,3,3,3,3,3,3,3,3,3,3,3,3,3,3,3,3,3,3,3,3,
3,3,3,3,4),(45.0768851922591,45.1609818802953,45.2452240064905,45.2544994815278,
45.3319968281964,45.409412146549,45.4867610662168,45.5640591691881,45.6413220005125,
45.7185780136331,45.7958331671945,45.8731015085371,45.9503970897929,46.0277806977766,
46.1052099060459,46.1827592471565,46.25323921739,46.328304170038,46.4032756128253,
46.4781708251655,46.553006967628,46.6278037590125,46.7025804818811,46.7773525137875,
46.8521352282683,46.9269801359669,47.0018586874943,47.0768308934441,47.1238898037031),
 .UNSPECIFIED.);
#3291=B_SPLINE_CURVE_WITH_KNOTS('',3,(#188287,#188288,#188289,#188290,#188291,
#188292,#188293,#188294,#188295,#188296,#188297,#188298,#188299,#188300,
#188301,#188302,#188303,#188304,#188305,#188306,#188307,#188308,#188309,
#188310,#188311,#188312,#188313,#188314,#188315,#188316,#188317,#188318,
#188319,#188320,#188321,#188322,#188323,#188324,#188325,#188326,#188327,
#188328,#188329,#188330,#188331,#188332,#188333,#188334,#188335,#188336,
#188337,#188338,#188339,#188340,#188341,#188342,#188343,#188344,#188345,
#188346,#188347,#188348,#188349,#188350,#188351,#188352,#188353,#188354,
#188355,#188356,#188357,#188358,#188359,#188360,#188361,#188362),
 .UNSPECIFIED.,.F.,.F.,(4,3,3,3,3,3,3,3,3,3,3,3,3,3,3,3,3,3,3,3,3,3,3,3,
3,4),(45.0773793149784,45.1598409187369,45.242301856616,45.3247621560141,
45.4072218443272,45.4896809489494,45.5721394972725,45.6545975166866,45.7370550345797,
45.8237322076589,45.9061989932676,45.9886641063988,46.0711276567057,46.1535897538197,
46.2360505073517,46.3185100268937,46.4009684220207,46.4834258022916,46.5658921881108,
46.648355389735,46.7308158456834,46.8132739943198,46.8957395983315,46.9781994769089,
47.0606635886454,47.1238898038476),.UNSPECIFIED.);
#3292=B_SPLINE_CURVE_WITH_KNOTS('',3,(#188363,#188364,#188365,#188366,#188367,
#188368,#188369,#188370,#188371,#188372,#188373,#188374,#188375,#188376,
#188377,#188378,#188379,#188380,#188381,#188382,#188383,#188384,#188385,
#188386,#188387,#188388,#188389,#188390,#188391,#188392,#188393,#188394,
#188395,#188396,#188397,#188398,#188399,#188400,#188401,#188402,#188403,
#188404,#188405,#188406,#188407,#188408,#188409,#188410,#188411,#188412,
#188413,#188414,#188415,#188416,#188417,#188418,#188419,#188420,#188421,
#188422,#188423,#188424,#188425,#188426,#188427,#188428,#188429,#188430,
#188431,#188432,#188433,#188434,#188435,#188436,#188437,#188438,#188439,
#188440,#188441,#188442,#188443,#188444,#188445,#188446,#188447,#188448,
#188449,#188450,#188451,#188452,#188453,#188454,#188455,#188456,#188457,
#188458,#188459,#188460,#188461,#188462,#188463,#188464,#188465,#188466,
#188467,#188468,#188469,#188470,#188471,#188472,#188473,#188474,#188475,
#188476,#188477,#188478,#188479,#188480,#188481,#188482,#188483,#188484,
#188485,#188486,#188487,#188488,#188489,#188490,#188491,#188492,#188493,
#188494,#188495,#188496,#188497,#188498,#188499,#188500,#188501,#188502,
#188503,#188504,#188505,#188506,#188507,#188508,#188509,#188510,#188511,
#188512,#188513,#188514,#188515,#188516,#188517,#188518,#188519,#188520,
#188521,#188522,#188523,#188524,#188525,#188526,#188527,#188528,#188529,
#188530,#188531),.UNSPECIFIED.,.F.,.F.,(4,3,3,3,3,3,3,3,3,3,3,3,3,3,3,3,
3,3,3,3,3,3,3,3,3,3,3,3,3,3,3,3,3,3,3,3,3,3,3,3,3,3,3,3,3,3,3,3,3,3,3,3,
3,3,3,3,4),(47.1238898038476,47.2096860330639,47.2996803595124,47.3859918106304,
47.4724364228933,47.5590287646913,47.5696633388578,47.6473190970526,47.724888662783,
47.8023859694146,47.8798146078488,47.9572034539753,48.0345663481531,48.0690332067889,
48.1525280138346,48.2361796908249,48.3200700860656,48.4040745314492,48.4882654896721,
48.56840307472,48.6459004213886,48.7233157397411,48.8006646594089,48.8779627623801,
48.9552255937045,49.0324816068252,49.1097367603867,49.1870051017294,49.264300682985,
49.3416842909687,49.4191134992377,49.4966628403483,49.5671428105821,49.6431942583012,
49.7191508491948,49.7950293701242,49.8708465278211,49.9466189675774,50.0240269149358,
50.0997749632719,50.17553102527,50.2513101118463,50.3299532204958,50.4058661333378,
50.4818365133272,50.5579140070008,50.5658825464443,50.644430733797,50.7228840545284,
50.8025633954618,50.8808565526102,50.9591043756868,51.0373198985842,51.118069619437,
51.1962715095341,51.2782951457648,51.3603187819955),.UNSPECIFIED.);
#3293=B_SPLINE_CURVE_WITH_KNOTS('',3,(#188537,#188538,#188539,#188540,#188541,
#188542,#188543,#188544,#188545,#188546,#188547,#188548,#188549,#188550,
#188551,#188552,#188553,#188554,#188555,#188556,#188557,#188558,#188559,
#188560,#188561,#188562,#188563,#188564,#188565,#188566,#188567,#188568,
#188569,#188570,#188571,#188572,#188573,#188574,#188575,#188576,#188577,
#188578,#188579,#188580,#188581,#188582,#188583,#188584,#188585,#188586,
#188587,#188588,#188589,#188590,#188591,#188592,#188593,#188594,#188595,
#188596,#188597,#188598,#188599,#188600,#188601,#188602,#188603,#188604,
#188605,#188606,#188607,#188608,#188609,#188610,#188611,#188612,#188613,
#188614,#188615,#188616,#188617,#188618,#188619,#188620,#188621,#188622,
#188623,#188624,#188625,#188626,#188627,#188628,#188629,#188630,#188631,
#188632,#188633,#188634,#188635,#188636,#188637,#188638,#188639,#188640,
#188641,#188642,#188643,#188644,#188645,#188646,#188647,#188648,#188649,
#188650,#188651,#188652,#188653,#188654,#188655,#188656,#188657,#188658,
#188659,#188660,#188661,#188662,#188663,#188664,#188665,#188666,#188667,
#188668,#188669,#188670,#188671,#188672,#188673,#188674,#188675,#188676,
#188677,#188678,#188679,#188680,#188681,#188682,#188683,#188684,#188685,
#188686,#188687,#188688,#188689,#188690,#188691,#188692,#188693,#188694,
#188695,#188696,#188697,#188698,#188699,#188700,#188701,#188702,#188703,
#188704,#188705),.UNSPECIFIED.,.F.,.F.,(4,3,3,3,3,3,3,3,3,3,3,3,3,3,3,3,
3,3,3,3,3,3,3,3,3,3,3,3,3,3,3,3,3,3,3,3,3,3,3,3,3,3,3,3,3,3,3,3,3,3,3,3,
3,3,3,3,4),(53.407075111169,53.4818186122275,53.5564918818662,53.6311121197668,
53.7076177428319,53.7821957165587,53.856775421336,53.9313722927244,54.0093184956152,
54.0840378541353,54.1588108193862,54.2336875061842,54.2431571042874,54.3216930443421,
54.4001361739608,54.4785010015096,54.5568019798971,54.6350535163474,54.7132730738886,
54.7914759954425,54.8696752799374,54.947883921749,55.0261475686102,55.1044396742875,
55.1828154874391,55.2418968401496,55.321538746576,55.401110366318,55.4806225952867,
55.5600779289768,55.6394991050345,55.7188957666113,55.7412667080807,55.8224968047066,
55.9037756957573,55.9879909158209,56.0694217692412,56.1550291726265,56.2406365760118,
56.3258798743107,56.4110449484651,56.4960593163427,56.5809666251388,56.665681127411,
56.7400064439429,56.8165494469285,56.8930869912719,56.9696336840399,57.0462362243281,
57.1228699696442,57.1995873574904,57.239376311874,57.3189296601009,57.4001097541118,
57.4795461996596,57.5615981179021,57.6436500361446),.UNSPECIFIED.);
#3294=B_SPLINE_CURVE_WITH_KNOTS('',3,(#188706,#188707,#188708,#188709,#188710,
#188711,#188712,#188713,#188714,#188715,#188716,#188717,#188718,#188719,
#188720,#188721,#188722,#188723,#188724,#188725,#188726,#188727,#188728,
#188729,#188730,#188731,#188732,#188733,#188734,#188735,#188736,#188737,
#188738,#188739,#188740,#188741,#188742,#188743,#188744,#188745,#188746,
#188747,#188748,#188749,#188750,#188751,#188752,#188753,#188754,#188755,
#188756,#188757,#188758,#188759,#188760,#188761,#188762,#188763,#188764,
#188765,#188766,#188767,#188768,#188769,#188770,#188771,#188772,#188773,
#188774,#188775,#188776,#188777,#188778,#188779,#188780,#188781,#188782,
#188783,#188784),.UNSPECIFIED.,.F.,.F.,(4,3,3,3,3,3,3,3,3,3,3,3,3,3,3,3,
3,3,3,3,3,3,3,3,3,3,4),(51.3612654433028,51.4387991235156,51.5162537536312,
51.5936620423316,51.6710398777053,51.746307764632,51.8298025716777,51.9134542486678,
51.9973446439085,52.0813490892922,52.1655400475151,52.2456776325631,52.3231749792317,
52.4005902975842,52.477939217252,52.555237320223,52.6325001515477,52.7097561646683,
52.7870113182299,52.8642796595726,52.9415752408281,53.0189588488118,53.0963880570809,
53.1739373981914,53.2444173684253,53.3640063522608,53.4070751110274),
 .UNSPECIFIED.);
#3295=B_SPLINE_CURVE_WITH_KNOTS('',3,(#188786,#188787,#188788,#188789,#188790,
#188791,#188792,#188793,#188794,#188795,#188796,#188797,#188798,#188799,
#188800,#188801,#188802,#188803,#188804,#188805,#188806,#188807,#188808,
#188809,#188810,#188811,#188812,#188813,#188814,#188815,#188816,#188817,
#188818,#188819,#188820,#188821,#188822,#188823,#188824,#188825,#188826,
#188827,#188828,#188829,#188830,#188831,#188832,#188833,#188834,#188835,
#188836,#188837,#188838,#188839,#188840,#188841,#188842,#188843,#188844,
#188845,#188846,#188847,#188848,#188849,#188850,#188851,#188852,#188853,
#188854,#188855,#188856,#188857,#188858,#188859,#188860,#188861,#188862,
#188863,#188864,#188865,#188866,#188867),.UNSPECIFIED.,.F.,.F.,(4,3,3,3,
3,3,3,3,3,3,3,3,3,3,3,3,3,3,3,3,3,3,3,3,3,3,3,4),(51.3603187819955,51.4386160327591,
51.5169947417649,51.5646222823065,51.6442641887329,51.723835808475,51.8033480374435,
51.8828033711338,51.9622245471915,52.0416212087684,52.0639921502376,52.1452222468635,
52.2265011379145,52.310716357978,52.3921472113984,52.4777546147836,52.5633620181687,
52.6486053164676,52.7337703906224,52.8187847585,52.9036920672959,52.9884065695682,
53.0627318860998,53.1365034122465,53.2102786527495,53.2840539656421,53.3578729667789,
53.4064687028836),.UNSPECIFIED.);
#3296=B_SPLINE_CURVE_WITH_KNOTS('',3,(#188868,#188869,#188870,#188871,#188872,
#188873,#188874,#188875,#188876,#188877,#188878,#188879,#188880,#188881,
#188882,#188883,#188884,#188885,#188886,#188887,#188888,#188889,#188890,
#188891,#188892,#188893,#188894,#188895,#188896,#188897,#188898,#188899,
#188900,#188901,#188902,#188903,#188904,#188905,#188906,#188907,#188908,
#188909,#188910,#188911,#188912,#188913,#188914,#188915,#188916,#188917,
#188918,#188919,#188920,#188921,#188922,#188923,#188924,#188925,#188926,
#188927,#188928,#188929,#188930,#188931,#188932,#188933,#188934,#188935,
#188936,#188937,#188938,#188939,#188940,#188941,#188942,#188943,#188944,
#188945,#188946,#188947,#188948,#188949,#188950,#188951,#188952,#188953,
#188954,#188955,#188956,#188957,#188958,#188959,#188960,#188961,#188962,
#188963,#188964,#188965,#188966,#188967,#188968,#188969,#188970,#188971,
#188972,#188973,#188974,#188975,#188976,#188977,#188978,#188979,#188980,
#188981,#188982,#188983,#188984,#188985,#188986,#188987,#188988,#188989,
#188990,#188991,#188992,#188993,#188994,#188995,#188996,#188997,#188998,
#188999,#189000,#189001,#189002,#189003,#189004,#189005,#189006,#189007,
#189008,#189009,#189010,#189011,#189012,#189013,#189014,#189015,#189016,
#189017,#189018,#189019,#189020,#189021,#189022,#189023,#189024),
 .UNSPECIFIED.,.F.,.F.,(4,3,3,3,3,3,3,3,3,3,3,3,3,3,3,3,3,3,3,3,3,3,3,3,
3,3,3,3,3,3,3,3,3,3,3,3,3,3,3,3,3,3,3,3,3,3,3,3,3,3,3,3,4),(53.4070751110272,
53.4895373171128,53.5719991749009,53.6544606912419,53.7369218729858,53.8193827269824,
53.9018432600811,53.9843034791314,54.0667633909818,54.1492230024812,54.2316823204779,
54.3141413518198,54.3966001033552,54.4790585819315,54.5615167943962,54.6439747475963,
54.7264324483789,54.8088899035909,54.8913471200785,54.9773597078678,55.0606844022887,
55.1431510078471,55.2256167691978,55.308081713756,55.3905458689339,55.4730092621412,
55.5554719207847,55.6379338722686,55.7203951439949,55.8028557633631,55.8853157577703,
55.9677751546117,56.0502339812801,56.1326922651665,56.2151500336598,56.2976073141475,
56.3817412275969,56.4642072258953,56.546671602444,56.629134466886,56.7115959288428,
56.7940560979166,56.8765150836914,56.9589729957343,57.0445701124347,57.1270348493784,
57.2094966216766,57.2919558677675,57.3744130259463,57.4568755448451,57.5393332161285,
57.6217920070367,57.6437499293376),.UNSPECIFIED.);
#3297=B_SPLINE_CURVE_WITH_KNOTS('',3,(#189030,#189031,#189032,#189033,#189034,
#189035,#189036,#189037,#189038,#189039,#189040,#189041,#189042,#189043,
#189044,#189045,#189046,#189047,#189048,#189049,#189050,#189051,#189052,
#189053,#189054,#189055,#189056,#189057,#189058,#189059,#189060,#189061,
#189062,#189063,#189064,#189065,#189066,#189067,#189068,#189069,#189070,
#189071,#189072,#189073,#189074,#189075,#189076,#189077,#189078,#189079,
#189080,#189081,#189082,#189083,#189084,#189085,#189086,#189087,#189088,
#189089,#189090,#189091,#189092,#189093,#189094,#189095,#189096,#189097,
#189098,#189099,#189100,#189101,#189102,#189103,#189104,#189105,#189106,
#189107,#189108,#189109,#189110,#189111,#189112,#189113,#189114,#189115,
#189116,#189117,#189118,#189119,#189120,#189121,#189122,#189123,#189124,
#189125,#189126,#189127,#189128,#189129,#189130,#189131,#189132,#189133,
#189134,#189135,#189136,#189137,#189138,#189139,#189140,#189141,#189142,
#189143,#189144,#189145,#189146,#189147,#189148,#189149,#189150,#189151,
#189152,#189153,#189154,#189155,#189156,#189157,#189158,#189159,#189160,
#189161,#189162,#189163,#189164,#189165,#189166,#189167,#189168,#189169,
#189170,#189171,#189172,#189173,#189174,#189175,#189176,#189177,#189178,
#189179,#189180,#189181,#189182,#189183,#189184,#189185,#189186,#189187,
#189188,#189189,#189190,#189191,#189192,#189193,#189194,#189195,#189196,
#189197,#189198),.UNSPECIFIED.,.F.,.F.,(4,3,3,3,3,3,3,3,3,3,3,3,3,3,3,3,
3,3,3,3,3,3,3,3,3,3,3,3,3,3,3,3,3,3,3,3,3,3,3,3,3,3,3,3,3,3,3,3,3,3,3,3,
3,3,3,3,4),(59.690260418207,59.7714338090463,59.8527099136974,59.9340935351152,
60.015661963685,60.0973276863695,60.1791662424323,60.2355955194606,60.3116469671796,
60.3876035580731,60.4634820790026,60.5392992366994,60.6150716764559,60.6924796238143,
60.7682276721505,60.8439837341485,60.9197628207247,60.9984059293742,61.0743188422161,
61.1502892222055,61.2263667158793,61.2343352553227,61.3128711953773,61.391314324996,
61.4696791525447,61.5479801309325,61.6262316673828,61.704451224924,61.7826541464778,
61.8608534309728,61.9390620727846,62.0173257196457,62.0956178253228,62.1739936384745,
62.2330749911849,62.3127168976113,62.3922885173533,62.4718007463221,62.5512560800124,
62.63067725607,62.7100739176467,62.732444859116,62.8136749557419,62.8949538467934,
62.9791690668568,63.0605999202773,63.1462073236622,63.2318147270471,63.3170580253461,
63.4022230995004,63.4872374673781,63.5721447761732,63.6568592784457,63.7311845949782,
63.8077235797901,63.8842647097723,63.926723068348),.UNSPECIFIED.);
#3298=B_SPLINE_CURVE_WITH_KNOTS('',3,(#189199,#189200,#189201,#189202,#189203,
#189204,#189205,#189206,#189207,#189208,#189209,#189210,#189211,#189212,
#189213,#189214,#189215,#189216,#189217,#189218,#189219,#189220,#189221,
#189222,#189223,#189224,#189225,#189226,#189227,#189228,#189229,#189230,
#189231,#189232,#189233,#189234,#189235,#189236,#189237,#189238,#189239,
#189240,#189241,#189242,#189243,#189244,#189245,#189246,#189247,#189248,
#189249,#189250,#189251,#189252,#189253,#189254,#189255,#189256,#189257,
#189258,#189259,#189260,#189261,#189262,#189263,#189264,#189265,#189266,
#189267,#189268,#189269,#189270,#189271,#189272,#189273,#189274,#189275,
#189276,#189277,#189278,#189279,#189280),.UNSPECIFIED.,.F.,.F.,(4,3,3,3,
3,3,3,3,3,3,3,3,3,3,3,3,3,3,3,3,3,3,3,3,3,3,3,4),(57.6436500361446,57.7230305488865,
57.8024147228682,57.8818136413679,57.9612383959083,58.040734811436,58.120270524691,
58.199893569992,58.2381160477362,58.3157718059308,58.3933413716611,58.4708386782927,
58.5482673167271,58.6256561628535,58.7030190570312,58.7374859156673,58.8209807227125,
58.9046323997037,58.9885227949444,59.0725272403283,59.1567181985513,59.2368557835984,
59.3178587346514,59.3987378950705,59.4794550555494,59.5600762076632,59.6405734332376,
59.6902604181083),.UNSPECIFIED.);
#3299=B_SPLINE_CURVE_WITH_KNOTS('',3,(#189282,#189283,#189284,#189285,#189286,
#189287,#189288,#189289,#189290,#189291,#189292,#189293,#189294,#189295,
#189296,#189297,#189298,#189299,#189300,#189301,#189302,#189303,#189304,
#189305,#189306,#189307,#189308,#189309,#189310,#189311,#189312,#189313,
#189314,#189315,#189316,#189317,#189318,#189319,#189320,#189321,#189322,
#189323,#189324,#189325,#189326,#189327,#189328,#189329,#189330,#189331,
#189332,#189333,#189334,#189335,#189336,#189337,#189338,#189339,#189340,
#189341,#189342,#189343,#189344,#189345,#189346,#189347,#189348,#189349,
#189350,#189351,#189352,#189353,#189354,#189355,#189356,#189357),
 .UNSPECIFIED.,.F.,.F.,(4,3,3,3,3,3,3,3,3,3,3,3,3,3,3,3,3,3,3,3,3,3,3,3,
3,4),(57.6437499293376,57.7262115330961,57.8086724709752,57.8911327703733,
57.9735924586864,58.0560515633085,58.1385101116317,58.2209681310457,58.3034256489388,
58.3901028220181,58.4725696076267,58.5550347207579,58.6374982710648,58.7199603681788,
58.8024211217109,58.8848806412531,58.96733903638,59.0497964166511,59.1322628024703,
59.2147260040945,59.2971864600429,59.3796446086792,59.4621102126909,59.5445700912683,
59.6270342030048,59.6902604182068),.UNSPECIFIED.);
#3300=B_SPLINE_CURVE_WITH_KNOTS('',3,(#189358,#189359,#189360,#189361,#189362,
#189363,#189364,#189365,#189366,#189367,#189368,#189369,#189370,#189371,
#189372,#189373,#189374,#189375,#189376,#189377,#189378,#189379,#189380,
#189381,#189382,#189383,#189384,#189385,#189386,#189387,#189388,#189389,
#189390,#189391,#189392,#189393,#189394,#189395,#189396,#189397,#189398,
#189399,#189400,#189401,#189402,#189403,#189404,#189405,#189406,#189407,
#189408,#189409,#189410,#189411,#189412,#189413,#189414,#189415,#189416,
#189417,#189418,#189419,#189420,#189421,#189422,#189423,#189424,#189425,
#189426,#189427,#189428,#189429,#189430,#189431,#189432,#189433,#189434,
#189435,#189436,#189437,#189438,#189439,#189440,#189441,#189442,#189443,
#189444,#189445,#189446,#189447,#189448,#189449,#189450,#189451,#189452,
#189453,#189454,#189455,#189456,#189457,#189458,#189459,#189460,#189461,
#189462,#189463,#189464,#189465,#189466,#189467,#189468,#189469,#189470,
#189471,#189472,#189473,#189474,#189475,#189476,#189477,#189478,#189479,
#189480,#189481,#189482,#189483,#189484,#189485,#189486,#189487,#189488,
#189489,#189490,#189491,#189492,#189493,#189494,#189495,#189496,#189497,
#189498,#189499,#189500,#189501,#189502,#189503,#189504,#189505,#189506,
#189507,#189508,#189509,#189510,#189511,#189512,#189513,#189514,#189515,
#189516,#189517,#189518,#189519,#189520,#189521,#189522,#189523,#189524,
#189525,#189526),.UNSPECIFIED.,.F.,.F.,(4,3,3,3,3,3,3,3,3,3,3,3,3,3,3,3,
3,3,3,3,3,3,3,3,3,3,3,3,3,3,3,3,3,3,3,3,3,3,3,3,3,3,3,3,3,3,3,3,3,3,3,3,
3,3,3,3,4),(59.6906622995972,59.7735023348937,59.8562048725928,59.9388187775212,
60.0213101921048,60.0539100371351,60.1304530401207,60.2069905844637,60.2835372772316,
60.3601398175197,60.4367735628356,60.5134909506818,60.5532799050662,60.6328270051466,
60.7123138365137,60.7917526640939,60.8711557153416,60.9505351891497,61.0299159113684,
61.1092993150829,61.1886964831849,61.2681185061813,61.3476119395595,61.427143768947,
61.5067644969261,61.5520196409283,61.6296753991229,61.7072449648534,61.7847422714853,
61.8621709099195,61.9395597560468,62.0169226502247,62.0513895088594,62.1348843159051,
62.2185359928955,62.3024263881361,62.3864308335196,62.4706217917426,62.5507593767905,
62.628256723459,62.7056720418116,62.7830209614793,62.8603190644503,62.9375818957749,
63.0148379088958,63.0920930624573,63.1693614037999,63.246656985055,63.3240405930387,
63.401469801308,63.4790191424186,63.5494991126527,63.625565547796,63.7015113736145,
63.7773881367892,63.8532008171584,63.9274178287548),.UNSPECIFIED.);
#3301=B_SPLINE_CURVE_WITH_KNOTS('',3,(#189532,#189533,#189534,#189535,#189536,
#189537,#189538,#189539,#189540,#189541,#189542,#189543,#189544,#189545,
#189546,#189547,#189548,#189549,#189550,#189551,#189552,#189553,#189554,
#189555,#189556,#189557,#189558,#189559,#189560,#189561,#189562,#189563,
#189564,#189565,#189566,#189567,#189568,#189569,#189570,#189571,#189572,
#189573,#189574,#189575,#189576,#189577,#189578,#189579,#189580,#189581,
#189582,#189583,#189584,#189585,#189586,#189587,#189588,#189589,#189590,
#189591,#189592,#189593,#189594,#189595,#189596,#189597,#189598,#189599,
#189600,#189601,#189602,#189603,#189604,#189605,#189606,#189607,#189608,
#189609,#189610,#189611,#189612,#189613,#189614,#189615,#189616,#189617,
#189618,#189619,#189620,#189621,#189622,#189623,#189624,#189625,#189626,
#189627,#189628,#189629,#189630,#189631,#189632,#189633,#189634,#189635,
#189636,#189637,#189638,#189639,#189640,#189641,#189642,#189643,#189644,
#189645,#189646,#189647,#189648,#189649,#189650,#189651,#189652,#189653,
#189654,#189655,#189656,#189657,#189658,#189659,#189660,#189661,#189662,
#189663,#189664,#189665,#189666,#189667,#189668,#189669,#189670,#189671,
#189672,#189673,#189674,#189675,#189676,#189677,#189678,#189679,#189680,
#189681,#189682,#189683,#189684,#189685,#189686,#189687,#189688,#189689,
#189690,#189691,#189692,#189693,#189694,#189695,#189696,#189697,#189698,
#189699,#189700),.UNSPECIFIED.,.F.,.F.,(4,3,3,3,3,3,3,3,3,3,3,3,3,3,3,3,
3,3,3,3,3,3,3,3,3,3,3,3,3,3,3,3,3,3,3,3,3,3,3,3,3,3,3,3,3,3,3,3,3,3,3,3,
3,3,3,3,4),(65.9734457253866,66.0711042468504,66.1699732343143,66.2280339346336,
66.3055312813023,66.3829465996547,66.4602955193225,66.5375936222937,66.6148564536183,
66.692112466739,66.7693676203005,66.8466359616432,66.9239315428988,67.0013151508825,
67.0787443591515,67.1562937002621,67.2267736704958,67.3028251182149,67.3787817091085,
67.4546602300379,67.5304773877348,67.6062498274911,67.6836577748495,67.7594058231856,
67.8351618851837,67.91094097176,67.9895840804095,68.0654969932515,68.141467373241,
68.2175448669146,68.225513406358,68.3040493464127,68.3824924760314,68.4608573035802,
68.5391582819678,68.6174098184182,68.6956293759595,68.7738322975133,68.8520315820083,
68.9302402238199,69.008503870681,69.0867959763583,69.1651717895099,69.2242531422202,
69.3038950486466,69.3834666683886,69.4629788973572,69.5424342310475,69.6218554071051,
69.701252068682,69.7236230101513,69.8048514931,69.8861287412328,69.9675063542346,
70.0489314636608,70.1304618817983,70.2100096701984),.UNSPECIFIED.);
#3302=B_SPLINE_CURVE_WITH_KNOTS('',3,(#189701,#189702,#189703,#189704,#189705,
#189706,#189707,#189708,#189709,#189710,#189711,#189712,#189713,#189714,
#189715,#189716,#189717,#189718,#189719,#189720,#189721,#189722,#189723,
#189724,#189725,#189726,#189727,#189728,#189729,#189730,#189731,#189732,
#189733,#189734,#189735,#189736,#189737,#189738,#189739,#189740,#189741,
#189742,#189743,#189744,#189745,#189746,#189747,#189748,#189749,#189750,
#189751,#189752,#189753,#189754,#189755,#189756,#189757,#189758,#189759,
#189760,#189761,#189762,#189763,#189764,#189765,#189766,#189767,#189768,
#189769,#189770,#189771,#189772,#189773,#189774,#189775,#189776,#189777,
#189778,#189779,#189780,#189781,#189782,#189783,#189784,#189785),
 .UNSPECIFIED.,.F.,.F.,(4,3,3,3,3,3,3,3,3,3,3,3,3,3,3,3,3,3,3,3,3,3,3,3,
3,3,3,3,4),(63.926723068348,64.0033159369046,64.0799341730901,64.1566430225131,
64.2305544629093,64.3101015629897,64.3895883943566,64.4690272219369,64.5484302731841,
64.6278097469924,64.7071904692108,64.7865738729253,64.8659710410277,64.9453930640241,
65.0248864974022,65.1044183267901,65.1840390547689,65.2292941987715,65.3069499569662,
65.3845195226964,65.4620168293273,65.5394454677618,65.6168343138883,65.6941972080664,
65.7286640667025,65.8058153750841,65.8830026586947,65.9602676708148,65.9734457253088),
 .UNSPECIFIED.);
#3303=B_SPLINE_CURVE_WITH_KNOTS('',3,(#189787,#189788,#189789,#189790,#189791,
#189792,#189793,#189794,#189795,#189796,#189797,#189798,#189799,#189800,
#189801,#189802,#189803,#189804,#189805,#189806,#189807,#189808,#189809,
#189810,#189811,#189812,#189813,#189814,#189815,#189816,#189817,#189818,
#189819,#189820,#189821,#189822,#189823,#189824,#189825,#189826,#189827,
#189828,#189829,#189830,#189831,#189832,#189833,#189834,#189835,#189836,
#189837,#189838,#189839,#189840,#189841,#189842,#189843,#189844,#189845,
#189846,#189847,#189848,#189849,#189850,#189851,#189852,#189853,#189854,
#189855,#189856,#189857,#189858,#189859,#189860,#189861,#189862,#189863,
#189864,#189865,#189866,#189867,#189868,#189869,#189870,#189871),
 .UNSPECIFIED.,.F.,.F.,(4,3,3,3,3,3,3,3,3,3,3,3,3,3,3,3,3,3,3,3,3,3,3,3,
3,3,3,3,4),(63.9274178287548,64.0050204562248,64.0807684977985,64.1565242830619,
64.2323028227389,64.3112868291829,64.3871990601391,64.4631685755102,64.5392454837294,
64.5482388485149,64.6267747885695,64.7052179181885,64.7835827457373,64.861883724125,
64.9401352605756,65.018354818117,65.0965577396707,65.1747570241658,65.252965665978,
65.3312293128392,65.4095214185164,65.4878972316681,65.5469785843771,65.6279655672961,
65.7088722640397,65.789683790522,65.8704366165766,65.9511241904645,65.9734457252612),
 .UNSPECIFIED.);
#3304=B_SPLINE_CURVE_WITH_KNOTS('',3,(#189872,#189873,#189874,#189875,#189876,
#189877,#189878,#189879,#189880,#189881,#189882,#189883,#189884,#189885,
#189886,#189887,#189888,#189889,#189890,#189891,#189892,#189893,#189894,
#189895,#189896,#189897,#189898,#189899,#189900,#189901,#189902,#189903,
#189904,#189905,#189906,#189907,#189908,#189909,#189910,#189911,#189912,
#189913,#189914,#189915,#189916,#189917,#189918,#189919,#189920,#189921,
#189922,#189923,#189924,#189925,#189926,#189927,#189928,#189929,#189930,
#189931,#189932,#189933,#189934,#189935,#189936,#189937,#189938,#189939,
#189940,#189941,#189942,#189943,#189944,#189945,#189946,#189947,#189948,
#189949,#189950,#189951,#189952,#189953,#189954,#189955,#189956,#189957,
#189958,#189959,#189960,#189961,#189962,#189963,#189964,#189965,#189966,
#189967,#189968,#189969,#189970,#189971,#189972,#189973,#189974,#189975,
#189976,#189977,#189978,#189979,#189980,#189981,#189982,#189983,#189984,
#189985,#189986,#189987,#189988,#189989,#189990,#189991,#189992,#189993,
#189994,#189995,#189996,#189997,#189998,#189999,#190000,#190001,#190002,
#190003,#190004,#190005,#190006,#190007,#190008,#190009,#190010,#190011,
#190012,#190013,#190014,#190015,#190016,#190017,#190018,#190019,#190020,
#190021,#190022,#190023,#190024,#190025,#190026,#190027,#190028,#190029,
#190030,#190031,#190032,#190033,#190034,#190035,#190036,#190037),
 .UNSPECIFIED.,.F.,.F.,(4,3,3,3,3,3,3,3,3,3,3,3,3,3,3,3,3,3,3,3,3,3,3,3,
3,3,3,3,3,3,3,3,3,3,3,3,3,3,3,3,3,3,3,3,3,3,3,3,3,3,3,3,3,3,3,4),(65.9734457253864,
66.0463484523082,66.1275785489341,66.2088574399853,66.2930726600488,66.3745035134692,
66.4601109168542,66.5457183202393,66.6309616185382,66.7161266926928,66.8011410605704,
66.8860483693661,66.9707628716383,67.0450881881704,67.121631191156,67.1981687354991,
67.2747154282674,67.3513179685556,67.4279517138715,67.5046691017177,67.5444580561014,
67.6240051561819,67.7034919875491,67.7829308151293,67.8623338663768,67.9417133401849,
68.0210940624036,68.100477466118,68.1798746342201,68.2592966572163,68.3387900905945,
68.4183219199819,68.497942647961,68.5431977919636,68.6208535501583,68.6984231158888,
68.7759204225202,68.8533490609544,68.930737907081,69.0081008012588,69.0425676598947,
69.1260624669404,69.2097141439304,69.2936045391711,69.3776089845548,69.4617999427777,
69.5419375278258,69.6194523907518,69.696859920406,69.7742050948759,69.8515020304642,
69.9287648132369,70.0060176813371,70.083263625084,70.1605369550174,70.2098018511721),
 .UNSPECIFIED.);
#3305=B_SPLINE_CURVE_WITH_KNOTS('',3,(#190043,#190044,#190045,#190046,#190047,
#190048,#190049,#190050,#190051,#190052,#190053,#190054,#190055,#190056,
#190057,#190058,#190059,#190060,#190061,#190062,#190063,#190064,#190065,
#190066,#190067,#190068,#190069,#190070,#190071,#190072,#190073,#190074,
#190075,#190076,#190077,#190078,#190079,#190080,#190081,#190082,#190083,
#190084,#190085,#190086,#190087,#190088,#190089,#190090,#190091,#190092,
#190093,#190094,#190095,#190096,#190097,#190098,#190099,#190100,#190101,
#190102,#190103,#190104,#190105,#190106,#190107,#190108,#190109,#190110,
#190111,#190112,#190113,#190114,#190115,#190116,#190117,#190118,#190119,
#190120,#190121,#190122,#190123,#190124,#190125,#190126,#190127,#190128,
#190129,#190130,#190131,#190132,#190133,#190134,#190135,#190136,#190137,
#190138,#190139,#190140,#190141,#190142,#190143,#190144,#190145,#190146,
#190147,#190148,#190149,#190150,#190151,#190152,#190153,#190154,#190155,
#190156,#190157,#190158,#190159,#190160,#190161,#190162,#190163,#190164,
#190165,#190166,#190167,#190168,#190169,#190170,#190171,#190172,#190173,
#190174,#190175,#190176,#190177,#190178,#190179,#190180,#190181,#190182,
#190183,#190184,#190185,#190186,#190187,#190188,#190189,#190190,#190191,
#190192,#190193,#190194,#190195,#190196,#190197,#190198,#190199,#190200,
#190201,#190202,#190203,#190204,#190205,#190206,#190207,#190208,#190209,
#190210,#190211),.UNSPECIFIED.,.F.,.F.,(4,3,3,3,3,3,3,3,3,3,3,3,3,3,3,3,
3,3,3,3,3,3,3,3,3,3,3,3,3,3,3,3,3,3,3,3,3,3,3,3,3,3,3,3,3,3,3,3,3,3,3,3,
3,3,3,3,4),(72.256631032664,72.3331585331301,72.4096077409919,72.4871663601784,
72.5634973406898,72.6416697792138,72.7198422177378,72.8033370247836,72.8869887017734,
72.9708790970142,73.0548835423979,73.1390745006208,73.2192120856689,73.2967094323376,
73.3741247506899,73.4514736703576,73.5287717733287,73.6060346046528,73.6832906177735,
73.7605457713351,73.8378141126778,73.915109693933,73.9924933019167,74.0699225101859,
74.1474718512964,74.2179518215311,74.2940032692501,74.3699598601438,74.4458383810733,
74.52165553877,74.5974279785262,74.6748359258846,74.7505839742207,74.8263400362187,
74.902119122795,74.9807622314445,75.0566751442866,75.1326455242761,75.2087230179496,
75.2166915573933,75.295227497448,75.3736706270668,75.4520354546155,75.530336433003,
75.6085879694537,75.686807526995,75.7650104485489,75.8432097330439,75.9214183748554,
75.9996820217166,76.0779741273936,76.1563499405453,76.2154312932555,76.2950688021106,
76.3746420616796,76.4541474077323,76.4935350358379),.UNSPECIFIED.);
#3306=B_SPLINE_CURVE_WITH_KNOTS('',3,(#190212,#190213,#190214,#190215,#190216,
#190217,#190218,#190219,#190220,#190221,#190222,#190223,#190224,#190225,
#190226,#190227,#190228,#190229,#190230,#190231,#190232,#190233,#190234,
#190235,#190236,#190237,#190238,#190239,#190240,#190241,#190242,#190243,
#190244,#190245,#190246,#190247,#190248,#190249,#190250,#190251,#190252,
#190253,#190254,#190255,#190256,#190257,#190258,#190259,#190260,#190261,
#190262,#190263,#190264,#190265,#190266,#190267,#190268,#190269,#190270,
#190271,#190272,#190273,#190274,#190275,#190276,#190277,#190278,#190279,
#190280,#190281,#190282,#190283,#190284,#190285,#190286,#190287,#190288,
#190289,#190290,#190291,#190292,#190293,#190294,#190295,#190296),
 .UNSPECIFIED.,.F.,.F.,(4,3,3,3,3,3,3,3,3,3,3,3,3,3,3,3,3,3,3,3,3,3,3,3,
3,3,3,3,4),(70.2100096701984,70.2229928780824,70.3082361763814,70.3934012505361,
70.4784156184137,70.5633229272095,70.6480374294818,70.7223627460135,70.7989057489991,
70.8754432933422,70.9519899861104,71.0285925263986,71.1052262717146,71.1819436595607,
71.2217326139446,71.3012797140251,71.3807665453923,71.4602053729725,71.53960842422,
71.6189878980283,71.6983686202469,71.7777520239615,71.8571491920635,71.9365712150598,
72.0160646484379,72.0955964778254,72.1752172058044,72.2204723498067,72.2566310325662),
 .UNSPECIFIED.);
#3307=B_SPLINE_CURVE_WITH_KNOTS('',3,(#190298,#190299,#190300,#190301,#190302,
#190303,#190304,#190305,#190306,#190307,#190308,#190309,#190310,#190311,
#190312,#190313,#190314,#190315,#190316,#190317,#190318,#190319,#190320,
#190321,#190322,#190323,#190324,#190325,#190326,#190327,#190328,#190329,
#190330,#190331,#190332,#190333,#190334,#190335,#190336,#190337,#190338,
#190339,#190340,#190341,#190342,#190343,#190344,#190345,#190346,#190347,
#190348,#190349,#190350,#190351,#190352,#190353,#190354,#190355,#190356,
#190357,#190358,#190359,#190360,#190361,#190362,#190363,#190364,#190365,
#190366,#190367,#190368,#190369,#190370,#190371,#190372,#190373,#190374,
#190375,#190376,#190377,#190378,#190379,#190380,#190381,#190382),
 .UNSPECIFIED.,.F.,.F.,(4,3,3,3,3,3,3,3,3,3,3,3,3,3,3,3,3,3,3,3,3,3,3,3,
3,3,3,3,4),(70.2098018511721,70.2871221325254,70.3645333234971,70.4419981804235,
70.5195694389141,70.540677263688,70.6167287114071,70.6926853023007,70.7685638232301,
70.844380980927,70.9201534206834,70.9975613680417,71.0733094163779,71.1490654783759,
71.2248445649522,71.3034876736017,71.3794005864437,71.4553709664332,71.5314484601067,
71.5394169995502,71.6181874416752,71.6979928905366,71.7765557243939,71.8550549720682,
71.9335033793759,72.0142852926734,72.0926727142568,72.1746518734114,72.256631032566),
 .UNSPECIFIED.);
#3308=B_SPLINE_CURVE_WITH_KNOTS('',3,(#190383,#190384,#190385,#190386,#190387,
#190388,#190389,#190390,#190391,#190392,#190393,#190394,#190395,#190396,
#190397,#190398,#190399,#190400,#190401,#190402,#190403,#190404,#190405,
#190406,#190407,#190408,#190409,#190410,#190411,#190412,#190413,#190414,
#190415,#190416,#190417,#190418,#190419,#190420,#190421,#190422,#190423,
#190424,#190425,#190426,#190427,#190428,#190429,#190430,#190431,#190432,
#190433,#190434,#190435,#190436,#190437,#190438,#190439,#190440,#190441,
#190442,#190443,#190444,#190445,#190446,#190447,#190448,#190449,#190450,
#190451,#190452,#190453,#190454,#190455,#190456,#190457,#190458,#190459,
#190460,#190461,#190462,#190463,#190464,#190465,#190466,#190467,#190468,
#190469,#190470,#190471,#190472,#190473,#190474,#190475,#190476,#190477,
#190478,#190479,#190480,#190481,#190482,#190483,#190484,#190485,#190486,
#190487,#190488,#190489,#190490,#190491,#190492,#190493,#190494,#190495,
#190496,#190497,#190498,#190499,#190500,#190501,#190502,#190503,#190504,
#190505,#190506,#190507,#190508,#190509,#190510,#190511,#190512,#190513,
#190514,#190515,#190516,#190517,#190518,#190519,#190520,#190521,#190522,
#190523,#190524,#190525,#190526,#190527,#190528,#190529,#190530,#190531,
#190532,#190533,#190534,#190535,#190536,#190537,#190538,#190539,#190540,
#190541,#190542,#190543,#190544,#190545,#190546,#190547,#190548),
 .UNSPECIFIED.,.F.,.F.,(4,3,3,3,3,3,3,3,3,3,3,3,3,3,3,3,3,3,3,3,3,3,3,3,
3,3,3,3,3,3,3,3,3,3,3,3,3,3,3,3,3,3,3,3,3,3,3,3,3,3,3,3,3,3,3,4),(72.2566310326855,
72.3483969715894,72.4432768535009,72.5381567354124,72.6177986418387,72.6973702615807,
72.7768824905492,72.8563378242394,72.9357590002969,73.0151556618737,73.0375266033435,
73.1187566999694,73.2000355910207,73.2842508110841,73.3656816645046,73.4512890678896,
73.5368964712745,73.6221397695734,73.7073048437281,73.7923192116057,73.8772265204015,
73.9619410226737,74.0362663392056,74.1128093421912,74.1893468865343,74.2658935793025,
74.3424961195907,74.4191298649066,74.4958472527529,74.5356362071367,74.6151833072172,
74.6946701385845,74.7741089661647,74.8535120174121,74.9328914912201,75.0122722134388,
75.0916556171533,75.1710527852555,75.2504748082516,75.3299682416298,75.4095000710173,
75.4891207989964,75.5343759429989,75.6120317011936,75.6896012669241,75.7670985735555,
75.8445272119897,75.9219160581163,75.9992789522941,76.03374581093,76.1172286053278,
76.2008689671098,76.2847376552225,76.3687219964419,76.4528751460584,76.4932994035531),
 .UNSPECIFIED.);
#3309=B_SPLINE_CURVE_WITH_KNOTS('',3,(#190554,#190555,#190556,#190557,#190558,
#190559,#190560,#190561,#190562,#190563,#190564,#190565,#190566,#190567,
#190568,#190569,#190570,#190571,#190572,#190573,#190574,#190575,#190576,
#190577,#190578,#190579,#190580,#190581,#190582,#190583,#190584,#190585,
#190586,#190587,#190588,#190589,#190590,#190591,#190592,#190593,#190594,
#190595,#190596,#190597,#190598,#190599,#190600,#190601,#190602,#190603,
#190604,#190605,#190606,#190607,#190608,#190609,#190610,#190611,#190612,
#190613,#190614,#190615,#190616,#190617,#190618,#190619,#190620,#190621,
#190622,#190623,#190624,#190625,#190626,#190627,#190628,#190629,#190630,
#190631,#190632,#190633,#190634,#190635,#190636,#190637,#190638,#190639,
#190640,#190641,#190642,#190643,#190644,#190645,#190646,#190647,#190648,
#190649,#190650,#190651,#190652,#190653,#190654,#190655,#190656,#190657,
#190658,#190659,#190660,#190661,#190662,#190663,#190664,#190665,#190666,
#190667,#190668,#190669,#190670,#190671,#190672,#190673,#190674,#190675,
#190676,#190677,#190678,#190679,#190680,#190681,#190682,#190683,#190684,
#190685,#190686,#190687,#190688,#190689,#190690,#190691,#190692,#190693,
#190694,#190695,#190696,#190697,#190698,#190699,#190700,#190701,#190702,
#190703,#190704,#190705,#190706,#190707,#190708,#190709,#190710),
 .UNSPECIFIED.,.F.,.F.,(4,3,3,3,3,3,3,3,3,3,3,3,3,3,3,3,3,3,3,3,3,3,3,3,
3,3,3,3,3,3,3,3,3,3,3,3,3,3,3,3,3,3,3,3,3,3,3,3,3,3,3,3,4),(78.5398163397457,
78.6222785458313,78.7047404036194,78.7872019199604,78.8696631017043,78.952123955701,
79.0345844887998,79.11704470785,79.1995046197004,79.2819642311997,79.3644235491964,
79.4468825805385,79.529341332074,79.6117998106502,79.694258023115,79.7767159763152,
79.8591736770979,79.9416311323097,80.0240883487972,80.1101009365866,80.1934256310075,
80.2758922365658,80.3583579979165,80.4408229424747,80.5232870976527,80.60575049086,
80.6882131495035,80.7706751009875,80.8531363727139,80.9355969920821,81.0180569864893,
81.1005163833306,81.1829752099989,81.2654334938853,81.3478912623787,81.4303485428664,
81.5144824563158,81.5969484546142,81.6794128311629,81.7618756956048,81.8443371575617,
81.9267973266356,82.0092563124103,82.0917142244532,82.1773113411536,82.2597760780973,
82.3422378503955,82.4246970964865,82.5071542546652,82.589616773564,82.6720744448474,
82.7545332357556,82.7764911580561),.UNSPECIFIED.);
#3310=B_SPLINE_CURVE_WITH_KNOTS('',3,(#190711,#190712,#190713,#190714,#190715,
#190716,#190717,#190718,#190719,#190720,#190721,#190722,#190723,#190724,
#190725,#190726,#190727,#190728,#190729,#190730,#190731,#190732,#190733,
#190734,#190735,#190736,#190737,#190738,#190739,#190740,#190741,#190742,
#190743,#190744,#190745,#190746,#190747,#190748,#190749,#190750,#190751,
#190752,#190753,#190754,#190755,#190756,#190757,#190758,#190759,#190760,
#190761,#190762,#190763,#190764,#190765,#190766,#190767,#190768,#190769,
#190770,#190771,#190772,#190773,#190774,#190775,#190776,#190777,#190778,
#190779,#190780,#190781,#190782,#190783,#190784,#190785,#190786,#190787,
#190788,#190789),.UNSPECIFIED.,.F.,.F.,(4,3,3,3,3,3,3,3,3,3,3,3,3,3,3,3,
3,3,3,3,3,3,3,3,3,3,4),(76.4935350358379,76.5729722034727,76.6523811635924,
76.7148011611866,76.7960312578123,76.8773101488636,76.9615253689272,77.0429562223475,
77.1285636257326,77.2141710291177,77.2994143274164,77.3845794015709,77.4695937694484,
77.5545010782443,77.6392155805164,77.7135408970487,77.7900839000344,77.8666214443776,
77.9431681371463,78.0197706774343,78.09640442275,78.1731218105964,78.2129107649798,
78.3067930419023,78.4004431333198,78.4934298877469,78.5398163397457),
 .UNSPECIFIED.);
#3311=B_SPLINE_CURVE_WITH_KNOTS('',3,(#190791,#190792,#190793,#190794,#190795,
#190796,#190797,#190798,#190799,#190800,#190801,#190802,#190803,#190804,
#190805,#190806,#190807,#190808,#190809,#190810,#190811,#190812,#190813,
#190814,#190815,#190816,#190817,#190818,#190819,#190820,#190821,#190822,
#190823,#190824,#190825,#190826,#190827,#190828,#190829,#190830,#190831,
#190832,#190833,#190834,#190835,#190836,#190837,#190838,#190839,#190840,
#190841,#190842,#190843,#190844,#190845,#190846,#190847,#190848,#190849,
#190850,#190851,#190852,#190853,#190854,#190855,#190856,#190857,#190858,
#190859,#190860,#190861,#190862,#190863,#190864,#190865,#190866,#190867,
#190868,#190869,#190870,#190871,#190872,#190873,#190874,#190875,#190876,
#190877,#190878),.UNSPECIFIED.,.F.,.F.,(4,3,3,3,3,3,3,3,3,3,3,3,3,3,3,3,
3,3,3,3,3,3,3,3,3,3,3,3,3,4),(76.4932994035531,76.5331156788611,76.6106130255297,
76.6880283438822,76.76537726355,76.8426753665212,76.9199381978456,76.9971942109663,
77.0744493645278,77.1517177058706,77.2290132871261,77.3063968951098,77.3838261033788,
77.4613754444894,77.5318554147233,77.6079068624424,77.683863453336,77.7597419742654,
77.8355591319623,77.9113315717187,77.9887395190771,78.0644875674132,78.1402436294113,
78.2160227159876,78.2946658246371,78.370578737479,78.4465491174684,78.5226266111422,
78.5305951505855,78.5398163397456),.UNSPECIFIED.);
#3312=B_SPLINE_CURVE_WITH_KNOTS('',3,(#190879,#190880,#190881,#190882,#190883,
#190884,#190885,#190886,#190887,#190888,#190889,#190890,#190891,#190892,
#190893,#190894,#190895,#190896,#190897,#190898,#190899,#190900,#190901,
#190902,#190903,#190904,#190905,#190906,#190907,#190908,#190909,#190910,
#190911,#190912,#190913,#190914,#190915,#190916,#190917,#190918,#190919,
#190920,#190921,#190922,#190923,#190924,#190925,#190926,#190927,#190928,
#190929,#190930,#190931,#190932,#190933,#190934,#190935,#190936,#190937,
#190938,#190939,#190940,#190941,#190942,#190943,#190944,#190945,#190946,
#190947,#190948,#190949,#190950,#190951,#190952,#190953,#190954,#190955,
#190956,#190957,#190958,#190959,#190960,#190961,#190962,#190963,#190964,
#190965,#190966,#190967,#190968,#190969,#190970,#190971,#190972,#190973,
#190974,#190975,#190976,#190977,#190978,#190979,#190980,#190981,#190982,
#190983,#190984,#190985,#190986,#190987,#190988,#190989,#190990,#190991,
#190992,#190993,#190994,#190995,#190996,#190997,#190998,#190999,#191000,
#191001,#191002,#191003,#191004,#191005,#191006,#191007,#191008,#191009,
#191010,#191011,#191012,#191013,#191014,#191015,#191016,#191017,#191018,
#191019,#191020,#191021,#191022,#191023,#191024,#191025,#191026,#191027,
#191028,#191029,#191030,#191031,#191032,#191033,#191034,#191035,#191036,
#191037,#191038,#191039,#191040,#191041,#191042,#191043,#191044,#191045,
#191046,#191047),.UNSPECIFIED.,.F.,.F.,(4,3,3,3,3,3,3,3,3,3,3,3,3,3,3,3,
3,3,3,3,3,3,3,3,3,3,3,3,3,3,3,3,3,3,3,3,3,3,3,3,3,3,3,3,3,3,3,3,3,3,3,3,
3,3,3,3,4),(78.539816339824,78.6181976215257,78.6964854105407,78.7746944375514,
78.8528393777969,78.9309348609844,79.0089986587314,79.087046253989,79.1650908450107,
79.2431456257895,79.3212559760837,79.3993959103608,79.4776186213982,79.5293348864476,
79.608976792874,79.688548412616,79.7680606415843,79.8475159752746,79.9269371513323,
80.0063338129092,80.0287047543787,80.1099348510046,80.1912137420557,80.2754289621192,
80.3568598155396,80.4424672189247,80.5280746223098,80.6133179206088,80.6984829947637,
80.7834973626413,80.8684046714371,80.9531191737094,81.0274444902409,81.1039874932265,
81.1805250375696,81.2570717303378,81.3336742706259,81.4103080159419,81.4870254037881,
81.526814358172,81.6063614582525,81.6858482896197,81.7652871172,81.8446901684473,
81.9240696422554,82.0034503644741,82.0828337681886,82.1622309362907,82.2416529592869,
82.3211463926651,82.4006782220526,82.4802989500318,82.5255540940342,82.6032094524399,
82.680786144195,82.7582804784433,82.7771312059986),.UNSPECIFIED.);
#3313=B_SPLINE_CURVE_WITH_KNOTS('',3,(#191053,#191054,#191055,#191056,#191057,
#191058,#191059,#191060,#191061,#191062,#191063,#191064,#191065,#191066,
#191067,#191068,#191069,#191070,#191071,#191072,#191073,#191074,#191075,
#191076,#191077,#191078,#191079,#191080,#191081,#191082,#191083,#191084,
#191085,#191086,#191087,#191088,#191089,#191090,#191091,#191092,#191093,
#191094,#191095,#191096,#191097,#191098,#191099,#191100,#191101,#191102,
#191103,#191104,#191105,#191106,#191107,#191108,#191109,#191110,#191111,
#191112,#191113,#191114,#191115,#191116,#191117,#191118,#191119,#191120,
#191121,#191122,#191123,#191124,#191125,#191126,#191127,#191128,#191129,
#191130,#191131,#191132,#191133,#191134,#191135,#191136,#191137,#191138,
#191139,#191140,#191141,#191142,#191143,#191144,#191145,#191146,#191147,
#191148,#191149,#191150,#191151,#191152,#191153,#191154,#191155,#191156,
#191157,#191158,#191159,#191160,#191161,#191162,#191163,#191164,#191165,
#191166,#191167,#191168,#191169,#191170,#191171,#191172,#191173,#191174,
#191175,#191176,#191177,#191178,#191179,#191180,#191181,#191182,#191183,
#191184,#191185,#191186,#191187,#191188,#191189,#191190,#191191,#191192,
#191193,#191194,#191195,#191196,#191197,#191198,#191199,#191200,#191201,
#191202,#191203,#191204,#191205,#191206,#191207,#191208,#191209,#191210,
#191211,#191212,#191213,#191214,#191215,#191216,#191217,#191218,#191219,
#191220,#191221),.UNSPECIFIED.,.F.,.F.,(4,3,3,3,3,3,3,3,3,3,3,3,3,3,3,3,
3,3,3,3,3,3,3,3,3,3,3,3,3,3,3,3,3,3,3,3,3,3,3,3,3,3,3,3,3,3,3,3,3,3,3,3,
3,3,3,3,4),(84.8230016469253,84.9016360502303,84.9803592002422,85.0591284898765,
85.1380107058712,85.2040889160151,85.2836360160956,85.3631228474628,85.4425616750429,
85.5219647262902,85.601344200098,85.6807249223166,85.7601083260311,85.8395054941333,
85.9189275171295,85.9984209505077,86.0779527798951,86.1575735078742,86.2028286518773,
86.280484410072,86.3580539758025,86.4355512824339,86.5129799208681,86.5903687669946,
86.6677316611725,86.7021985198084,86.7856933268541,86.8693450038441,86.9532353990847,
87.0372398444685,87.1214308026914,87.2015683877395,87.2790657344081,87.3564810527606,
87.4338299724283,87.5111280753995,87.5883909067241,87.6656469198448,87.7429020734063,
87.820170414749,87.8974659960045,87.9748496039882,88.0522788122573,88.1298281533679,
88.2003081236017,88.2763679139956,88.3523311401638,88.4282145998417,88.5070125135111,
88.5827841972536,88.658531741077,88.73427015711,88.8100144490699,88.8858076076066,
88.9616299313289,89.0375258059729,89.058597909197),.UNSPECIFIED.);
#3314=B_SPLINE_CURVE_WITH_KNOTS('',3,(#191222,#191223,#191224,#191225,#191226,
#191227,#191228,#191229,#191230,#191231,#191232,#191233,#191234,#191235,
#191236,#191237,#191238,#191239,#191240,#191241,#191242,#191243,#191244,
#191245,#191246,#191247,#191248,#191249,#191250,#191251,#191252,#191253,
#191254,#191255,#191256,#191257,#191258,#191259,#191260,#191261,#191262,
#191263,#191264,#191265,#191266,#191267,#191268,#191269,#191270,#191271,
#191272,#191273,#191274,#191275,#191276,#191277,#191278,#191279,#191280,
#191281,#191282,#191283,#191284,#191285,#191286,#191287,#191288,#191289,
#191290,#191291,#191292,#191293,#191294,#191295,#191296,#191297),
 .UNSPECIFIED.,.F.,.F.,(4,3,3,3,3,3,3,3,3,3,3,3,3,3,3,3,3,3,3,3,3,3,3,3,
3,4),(82.7764911580561,82.8589527618145,82.9414136996937,83.0238739990917,
83.1063336874048,83.188792792027,83.2712513403501,83.3537093597642,83.4361668776573,
83.5228440507365,83.6053108363451,83.6877759494763,83.7702394997832,83.8527015968972,
83.9351623504291,84.0176218699713,84.1000802650985,84.1825376453695,84.2650040311887,
84.3474672328128,84.4299276887613,84.5123858373977,84.5948514414094,84.6773113199869,
84.7597754317234,84.8230016469253),.UNSPECIFIED.);
#3315=B_SPLINE_CURVE_WITH_KNOTS('',3,(#191299,#191300,#191301,#191302,#191303,
#191304,#191305,#191306,#191307,#191308,#191309,#191310,#191311,#191312,
#191313,#191314,#191315,#191316,#191317,#191318,#191319,#191320,#191321,
#191322,#191323,#191324,#191325,#191326,#191327,#191328,#191329,#191330,
#191331,#191332,#191333,#191334,#191335,#191336,#191337,#191338,#191339,
#191340,#191341,#191342,#191343,#191344,#191345,#191346,#191347,#191348,
#191349,#191350,#191351,#191352,#191353,#191354,#191355,#191356,#191357,
#191358,#191359,#191360,#191361,#191362,#191363,#191364,#191365,#191366,
#191367,#191368,#191369,#191370,#191371,#191372,#191373,#191374,#191375,
#191376,#191377,#191378,#191379,#191380),.UNSPECIFIED.,.F.,.F.,(4,3,3,3,
3,3,3,3,3,3,3,3,3,3,3,3,3,3,3,3,3,3,3,3,3,3,3,4),(82.7771312059986,82.8545490138819,
82.9319300501453,83.0092874835167,83.0249239619653,83.1084187690111,83.1920704460012,
83.2759608412419,83.3599652866256,83.4441562448485,83.5242938298964,83.601791176565,
83.6792064949175,83.7565554145853,83.8338535175563,83.9111163488808,83.9883723620015,
84.0656275155629,84.1428958569057,84.2201914381612,84.2975750461449,84.375004254414,
84.4525535955245,84.5230335657586,84.6158752198683,84.7080796541723,84.7992061973053,
84.8230016467793),.UNSPECIFIED.);
#3316=B_SPLINE_CURVE_WITH_KNOTS('',3,(#191381,#191382,#191383,#191384,#191385,
#191386,#191387,#191388,#191389,#191390,#191391,#191392,#191393,#191394,
#191395,#191396,#191397,#191398,#191399,#191400,#191401,#191402,#191403,
#191404,#191405,#191406,#191407,#191408,#191409,#191410,#191411,#191412,
#191413,#191414,#191415,#191416,#191417,#191418,#191419,#191420,#191421,
#191422,#191423,#191424,#191425,#191426,#191427,#191428,#191429,#191430,
#191431,#191432,#191433,#191434,#191435,#191436,#191437,#191438,#191439,
#191440,#191441,#191442,#191443,#191444,#191445,#191446,#191447,#191448,
#191449,#191450,#191451,#191452,#191453,#191454,#191455,#191456,#191457,
#191458,#191459,#191460,#191461,#191462,#191463,#191464,#191465,#191466,
#191467,#191468,#191469,#191470,#191471,#191472,#191473,#191474,#191475,
#191476,#191477,#191478,#191479,#191480,#191481,#191482,#191483,#191484,
#191485,#191486,#191487,#191488,#191489,#191490,#191491,#191492,#191493,
#191494,#191495,#191496,#191497,#191498,#191499,#191500,#191501,#191502,
#191503,#191504,#191505,#191506,#191507,#191508,#191509,#191510,#191511,
#191512,#191513,#191514,#191515,#191516,#191517,#191518,#191519,#191520,
#191521,#191522,#191523,#191524,#191525,#191526,#191527,#191528,#191529,
#191530,#191531,#191532,#191533,#191534,#191535,#191536,#191537,#191538,
#191539,#191540,#191541,#191542,#191543,#191544,#191545,#191546,#191547,
#191548,#191549),.UNSPECIFIED.,.F.,.F.,(4,3,3,3,3,3,3,3,3,3,3,3,3,3,3,3,
3,3,3,3,3,3,3,3,3,3,3,3,3,3,3,3,3,3,3,3,3,3,3,3,3,3,3,3,3,3,3,3,3,3,3,3,
3,3,3,3,4),(84.8230016469252,84.8981957460114,84.9761429404625,85.0513035388916,
85.126469067077,85.2016547669266,85.2768759001131,85.3521896409006,85.4275584136209,
85.5030372070134,85.5217733016207,85.6003092416753,85.6787523712939,85.7571171988428,
85.83541817723,85.9136697136805,85.9918892712217,86.0700921927756,86.1482914772705,
86.2265001190823,86.3047637659434,86.3830558716207,86.4614316847723,86.5205130374829,
86.6001549439093,86.6797265636513,86.7592387926201,86.8386941263103,86.9181153023685,
86.997511963945,87.019882905414,87.1011130020399,87.1823918930907,87.2666071131543,
87.3480379665746,87.4336453699599,87.5192527733451,87.6044960716438,87.689661145799,
87.7746755136765,87.8595828224724,87.9442973247445,88.0186226412762,88.0951656442619,
88.1717031886047,88.2482498813727,88.3248524216608,88.4014861669768,88.4782035548231,
88.5179925092073,88.59753722332,88.677023957123,88.756463877152,88.8358679414933,
88.9152488021237,88.9946280383445,89.0594462566544),.UNSPECIFIED.);
#3317=B_SPLINE_CURVE_WITH_KNOTS('',3,(#191555,#191556,#191557,#191558,#191559,
#191560,#191561,#191562,#191563,#191564,#191565,#191566,#191567,#191568,
#191569,#191570,#191571,#191572,#191573,#191574,#191575,#191576,#191577,
#191578,#191579,#191580,#191581,#191582,#191583,#191584,#191585,#191586,
#191587,#191588,#191589,#191590,#191591,#191592,#191593,#191594,#191595,
#191596,#191597,#191598,#191599,#191600,#191601,#191602,#191603,#191604,
#191605,#191606,#191607,#191608,#191609,#191610,#191611,#191612,#191613,
#191614,#191615,#191616,#191617,#191618,#191619,#191620,#191621,#191622,
#191623,#191624,#191625,#191626,#191627,#191628,#191629,#191630,#191631,
#191632,#191633,#191634,#191635,#191636,#191637,#191638,#191639,#191640,
#191641,#191642,#191643,#191644,#191645,#191646,#191647,#191648,#191649,
#191650,#191651,#191652,#191653,#191654,#191655,#191656,#191657,#191658,
#191659,#191660,#191661,#191662,#191663,#191664,#191665,#191666,#191667,
#191668,#191669,#191670,#191671,#191672,#191673,#191674,#191675,#191676,
#191677,#191678,#191679,#191680,#191681,#191682,#191683,#191684,#191685,
#191686,#191687,#191688,#191689,#191690,#191691,#191692,#191693,#191694,
#191695,#191696,#191697,#191698,#191699,#191700,#191701,#191702,#191703,
#191704,#191705,#191706,#191707,#191708,#191709,#191710,#191711,#191712,
#191713,#191714,#191715,#191716,#191717,#191718,#191719,#191720),
 .UNSPECIFIED.,.F.,.F.,(4,3,3,3,3,3,3,3,3,3,3,3,3,3,3,3,3,3,3,3,3,3,3,3,
3,3,3,3,3,3,3,3,3,3,3,3,3,3,3,3,3,3,3,3,3,3,3,3,3,3,3,3,3,3,3,4),(91.1061869541049,
91.1965273311882,91.2817706294871,91.3669357036419,91.4519500715196,91.5368573803156,
91.6215718825877,91.6958971991193,91.7724402021049,91.8489777464479,91.9255244392161,
92.0021269795043,92.0787607248203,92.1554781126665,92.1952670670504,92.2748141671309,
92.3543009984982,92.4337398260784,92.5131428773258,92.5925223511339,92.6719030733525,
92.751286477067,92.8306836451692,92.9101056681653,92.9895991015435,93.0691309309309,
93.14875165891,93.1940068029126,93.2716625611073,93.3492321268378,93.4267294334692,
93.5041580719034,93.58154691803,93.6589098122078,93.6933766708437,93.7768714778894,
93.8605231548795,93.9444135501201,94.0284179955038,94.1126089537267,94.1927465387748,
94.2702438854434,94.3476592037959,94.4250081234637,94.5023062264348,94.5795690577594,
94.65682507088,94.7340802244415,94.8113485657843,94.8886441470398,94.9660277550235,
95.0434569632925,95.1210063044031,95.191486274637,95.2676491241019,95.3438119735668),
 .UNSPECIFIED.);
#3318=B_SPLINE_CURVE_WITH_KNOTS('',3,(#191721,#191722,#191723,#191724,#191725,
#191726,#191727,#191728,#191729,#191730,#191731,#191732,#191733,#191734,
#191735,#191736,#191737,#191738,#191739,#191740,#191741,#191742,#191743,
#191744,#191745,#191746,#191747,#191748,#191749,#191750,#191751,#191752,
#191753,#191754,#191755,#191756,#191757,#191758,#191759,#191760,#191761,
#191762,#191763,#191764,#191765,#191766,#191767,#191768,#191769,#191770,
#191771,#191772,#191773,#191774,#191775,#191776,#191777,#191778,#191779,
#191780,#191781,#191782,#191783,#191784,#191785,#191786,#191787,#191788,
#191789,#191790,#191791,#191792,#191793,#191794,#191795,#191796,#191797,
#191798,#191799,#191800,#191801,#191802),.UNSPECIFIED.,.F.,.F.,(4,3,3,3,
3,3,3,3,3,3,3,3,3,3,3,3,3,3,3,3,3,3,3,3,3,3,3,4),(89.058597909197,89.1346476530498,
89.1990478594639,89.2775837995186,89.3560269291372,89.4343917566861,89.5126927350737,
89.590944271524,89.6691638290653,89.7473667506191,89.8255660351141,89.9037746769256,
89.9820383237868,90.0603304294641,90.1387062426157,90.197787595326,90.2774295017524,
90.3570011214944,90.4365133504632,90.5159686841535,90.5953898602109,90.6747865217878,
90.6971574632571,90.7769810610411,90.8592825342846,90.9392150863258,91.0227010201705,
91.1061869540151),.UNSPECIFIED.);
#3319=B_SPLINE_CURVE_WITH_KNOTS('',3,(#191804,#191805,#191806,#191807,#191808,
#191809,#191810,#191811,#191812,#191813,#191814,#191815,#191816,#191817,
#191818,#191819,#191820,#191821,#191822,#191823,#191824,#191825,#191826,
#191827,#191828,#191829,#191830,#191831,#191832,#191833,#191834,#191835,
#191836,#191837,#191838,#191839,#191840,#191841,#191842,#191843,#191844,
#191845,#191846,#191847,#191848,#191849,#191850,#191851,#191852,#191853,
#191854,#191855,#191856,#191857,#191858,#191859,#191860,#191861,#191862,
#191863,#191864,#191865,#191866,#191867,#191868,#191869,#191870,#191871,
#191872,#191873,#191874,#191875,#191876,#191877,#191878,#191879,#191880,
#191881,#191882,#191883,#191884,#191885),.UNSPECIFIED.,.F.,.F.,(4,3,3,3,
3,3,3,3,3,3,3,3,3,3,3,3,3,3,3,3,3,3,3,3,3,3,3,4),(89.0594462566544,89.1388400688914,
89.2182567002861,89.2977441991114,89.3772682231841,89.4568844740184,89.5167322450695,
89.5943880032642,89.6719575689949,89.7494548756267,89.8268835140609,89.9042723601875,
89.9816352543653,90.0161021130006,90.0995969200461,90.1832485970364,90.2671389922769,
90.35114343766,90.4353343958829,90.5154719809317,90.5929183426514,90.6702799673374,
90.7475710092086,90.8248055785584,90.9019963422042,90.9791610576861,91.0563236669859,
91.1061869541047),.UNSPECIFIED.);
#3320=B_SPLINE_CURVE_WITH_KNOTS('',3,(#191886,#191887,#191888,#191889,#191890,
#191891,#191892,#191893,#191894,#191895,#191896,#191897,#191898,#191899,
#191900,#191901,#191902,#191903,#191904,#191905,#191906,#191907,#191908,
#191909,#191910,#191911,#191912,#191913,#191914,#191915,#191916,#191917,
#191918,#191919,#191920,#191921,#191922,#191923,#191924,#191925,#191926,
#191927,#191928,#191929,#191930,#191931,#191932,#191933,#191934,#191935,
#191936,#191937,#191938,#191939,#191940,#191941,#191942,#191943,#191944,
#191945,#191946,#191947,#191948,#191949,#191950,#191951,#191952,#191953,
#191954,#191955,#191956,#191957,#191958,#191959,#191960,#191961,#191962,
#191963,#191964,#191965,#191966,#191967,#191968,#191969,#191970,#191971,
#191972,#191973,#191974,#191975,#191976,#191977,#191978,#191979,#191980,
#191981,#191982,#191983,#191984,#191985,#191986,#191987,#191988,#191989,
#191990,#191991,#191992,#191993,#191994,#191995,#191996,#191997,#191998,
#191999,#192000,#192001,#192002,#192003,#192004,#192005,#192006,#192007,
#192008,#192009,#192010,#192011,#192012,#192013,#192014,#192015,#192016,
#192017,#192018,#192019,#192020,#192021,#192022,#192023,#192024,#192025,
#192026,#192027,#192028,#192029,#192030,#192031,#192032,#192033,#192034,
#192035,#192036,#192037,#192038,#192039,#192040,#192041,#192042,#192043,
#192044,#192045,#192046,#192047,#192048,#192049,#192050,#192051,#192052,
#192053,#192054),.UNSPECIFIED.,.F.,.F.,(4,3,3,3,3,3,3,3,3,3,3,3,3,3,3,3,
3,3,3,3,3,3,3,3,3,3,3,3,3,3,3,3,3,3,3,3,3,3,3,3,3,3,3,3,3,3,3,3,3,3,3,3,
3,3,3,3,4),(91.1061869542419,91.1938025881983,91.2820948836687,91.3707154500607,
91.4597496548414,91.5142117167938,91.5902631645129,91.6662197554065,91.7420982763358,
91.8179154340327,91.893687873789,91.9710958211474,92.0468438694835,92.1225999314816,
92.1983790180579,92.2770221267074,92.3529350395494,92.4289054195389,92.5049829132124,
92.512951452656,92.5914873927107,92.6699305223293,92.7482953498781,92.8265963282656,
92.904847864716,92.9830674222573,93.0612703438111,93.139469628306,93.2176782701176,
93.2959419169788,93.3742340226561,93.4526098358077,93.5116911885182,93.5913330949446,
93.6709047146866,93.7504169436552,93.8298722773454,93.9092934534031,93.98869011498,
94.0110610564493,94.0922911530752,94.1735700441262,94.2577852641898,94.3392161176101,
94.4248235209953,94.5104309243804,94.5956742226793,94.6808392968341,94.7658536647118,
94.8507609735076,94.9354754757799,95.0098007923115,95.0863384425137,95.1628822781568,
95.2394299895684,95.3160157765372,95.3423550910411),.UNSPECIFIED.);
#3321=B_SPLINE_CURVE_WITH_KNOTS('',3,(#192060,#192061,#192062,#192063,#192064,
#192065,#192066,#192067,#192068,#192069,#192070,#192071,#192072,#192073,
#192074,#192075,#192076,#192077,#192078,#192079,#192080,#192081,#192082,
#192083,#192084,#192085,#192086,#192087,#192088,#192089,#192090,#192091,
#192092,#192093,#192094,#192095,#192096,#192097,#192098,#192099,#192100,
#192101,#192102,#192103,#192104,#192105,#192106,#192107,#192108,#192109,
#192110,#192111,#192112,#192113,#192114,#192115,#192116,#192117,#192118,
#192119,#192120,#192121,#192122,#192123,#192124,#192125,#192126,#192127,
#192128,#192129,#192130,#192131,#192132,#192133,#192134,#192135,#192136,
#192137,#192138,#192139,#192140,#192141,#192142,#192143,#192144,#192145,
#192146,#192147,#192148,#192149,#192150,#192151,#192152,#192153,#192154,
#192155,#192156,#192157,#192158,#192159,#192160,#192161,#192162,#192163,
#192164,#192165,#192166,#192167,#192168,#192169,#192170,#192171,#192172,
#192173,#192174,#192175,#192176,#192177,#192178,#192179,#192180,#192181,
#192182,#192183,#192184,#192185,#192186,#192187,#192188,#192189,#192190,
#192191,#192192,#192193,#192194,#192195,#192196,#192197,#192198,#192199,
#192200,#192201,#192202,#192203,#192204,#192205,#192206,#192207,#192208,
#192209,#192210,#192211,#192212,#192213,#192214,#192215,#192216,#192217,
#192218,#192219,#192220,#192221,#192222,#192223,#192224,#192225),
 .UNSPECIFIED.,.F.,.F.,(4,3,3,3,3,3,3,3,3,3,3,3,3,3,3,3,3,3,3,3,3,3,3,3,
3,3,3,3,3,3,3,3,3,3,3,3,3,3,3,3,3,3,3,3,3,3,3,3,3,3,3,3,3,3,3,4),(97.3893722613826,
97.4652312909182,97.5410553653612,97.6168713919726,97.6883356142924,97.7695657109184,
97.8508446019692,97.9350598220328,98.0164906754531,98.1020980788383,98.1877054822235,
98.2729487805224,98.3581138546769,98.4431282225546,98.5280355313507,98.612750033623,
98.6870753501546,98.7636183531402,98.8401558974831,98.916702590252,98.9933051305401,
99.069938875856,99.1466562637022,99.1864452180857,99.2659923181663,99.3454791495333,
99.4249179771133,99.5043210283606,99.5837005021682,99.6630812243868,99.7424646281013,
99.8218617962035,99.9012838191999,99.9807772525781,100.060309081966,100.139929809945,
100.185184953948,100.262840712143,100.340410277873,100.417907584505,100.495336222939,
100.572725069066,100.650087963244,100.684554821879,100.768049628925,100.851701305914,
100.935591701155,101.019596146539,101.103787104761,101.18392468981,101.261427571921,
101.338850375907,101.416193775241,101.49349100672,101.570755819008,101.626277039953),
 .UNSPECIFIED.);
#3322=B_SPLINE_CURVE_WITH_KNOTS('',3,(#192226,#192227,#192228,#192229,#192230,
#192231,#192232,#192233,#192234,#192235,#192236,#192237,#192238,#192239,
#192240,#192241,#192242,#192243,#192244,#192245,#192246,#192247,#192248,
#192249,#192250,#192251,#192252,#192253,#192254,#192255,#192256,#192257,
#192258,#192259,#192260,#192261,#192262,#192263,#192264,#192265,#192266,
#192267,#192268,#192269,#192270,#192271,#192272,#192273,#192274,#192275,
#192276,#192277,#192278,#192279,#192280,#192281,#192282,#192283,#192284,
#192285,#192286,#192287,#192288,#192289,#192290,#192291,#192292,#192293,
#192294,#192295,#192296,#192297,#192298,#192299,#192300,#192301,#192302,
#192303,#192304,#192305,#192306,#192307),.UNSPECIFIED.,.F.,.F.,(4,3,3,3,
3,3,3,3,3,3,3,3,3,3,3,3,3,3,3,3,3,3,3,3,3,3,3,4),(95.3438119735668,95.4196902029664,
95.4955071389005,95.5712794264404,95.6486477494477,95.7243957997551,95.8001519186736,
95.8759311171591,95.9545048404941,96.0304178924257,96.1103219514624,96.1902260104991,
96.2687619505538,96.3472050801724,96.4255699077212,96.5038708861088,96.5821224225593,
96.6603419801005,96.7385449016544,96.8167441861493,96.8949528279609,96.973216474822,
97.0515085804993,97.129884393651,97.1889657463613,97.280334839224,97.371304386611,
97.3893722612845),.UNSPECIFIED.);
#3323=B_SPLINE_CURVE_WITH_KNOTS('',3,(#192309,#192310,#192311,#192312,#192313,
#192314,#192315,#192316,#192317,#192318,#192319,#192320,#192321,#192322,
#192323,#192324,#192325,#192326,#192327,#192328,#192329,#192330,#192331,
#192332,#192333,#192334,#192335,#192336,#192337,#192338,#192339,#192340,
#192341,#192342,#192343,#192344,#192345,#192346,#192347,#192348,#192349,
#192350,#192351,#192352,#192353,#192354,#192355,#192356,#192357,#192358,
#192359,#192360,#192361,#192362,#192363,#192364,#192365,#192366,#192367,
#192368,#192369,#192370,#192371,#192372,#192373,#192374,#192375,#192376,
#192377,#192378,#192379,#192380,#192381,#192382,#192383,#192384,#192385,
#192386,#192387,#192388,#192389,#192390,#192391,#192392,#192393),
 .UNSPECIFIED.,.F.,.F.,(4,3,3,3,3,3,3,3,3,3,3,3,3,3,3,3,3,3,3,3,3,3,3,3,
3,3,3,3,4),(95.3423550910411,95.419002585791,95.4957287477094,95.5091706602426,
95.5887177603231,95.6682045916903,95.7476434192705,95.8270464705179,95.9064259443261,
95.9858066665447,96.0651900702593,96.1445872383614,96.2240092613575,96.3035026947357,
96.3830345241231,96.4626552521022,96.5079103961047,96.5855661542994,96.6631357200298,
96.7406330266612,96.8180616650954,96.895450511222,96.9728134053998,97.0072802640358,
97.0868812783776,97.1666126545292,97.2464127750382,97.3263553451898,97.3893722611653),
 .UNSPECIFIED.);
#3324=B_SPLINE_CURVE_WITH_KNOTS('',3,(#192394,#192395,#192396,#192397,#192398,
#192399,#192400,#192401,#192402,#192403,#192404,#192405,#192406,#192407,
#192408,#192409,#192410,#192411,#192412,#192413,#192414,#192415,#192416,
#192417,#192418,#192419,#192420,#192421,#192422,#192423,#192424,#192425,
#192426,#192427,#192428,#192429,#192430,#192431,#192432,#192433,#192434,
#192435,#192436,#192437,#192438,#192439,#192440,#192441,#192442,#192443,
#192444,#192445,#192446,#192447,#192448,#192449,#192450,#192451,#192452,
#192453,#192454,#192455,#192456,#192457,#192458,#192459,#192460,#192461,
#192462,#192463,#192464,#192465,#192466,#192467,#192468,#192469,#192470,
#192471,#192472,#192473,#192474,#192475,#192476,#192477,#192478,#192479,
#192480,#192481,#192482,#192483,#192484,#192485,#192486,#192487,#192488,
#192489,#192490,#192491,#192492,#192493,#192494,#192495,#192496,#192497,
#192498,#192499,#192500,#192501,#192502,#192503,#192504,#192505,#192506,
#192507,#192508,#192509,#192510,#192511,#192512,#192513,#192514,#192515,
#192516,#192517,#192518,#192519,#192520,#192521,#192522,#192523,#192524,
#192525,#192526,#192527,#192528,#192529,#192530,#192531,#192532,#192533,
#192534,#192535,#192536,#192537,#192538,#192539,#192540,#192541,#192542,
#192543,#192544,#192545,#192546,#192547,#192548,#192549,#192550,#192551,
#192552,#192553,#192554,#192555,#192556,#192557,#192558,#192559,#192560,
#192561,#192562),.UNSPECIFIED.,.F.,.F.,(4,3,3,3,3,3,3,3,3,3,3,3,3,3,3,3,
3,3,3,3,3,3,3,3,3,3,3,3,3,3,3,3,3,3,3,3,3,3,3,3,3,3,3,3,3,3,3,3,3,3,3,3,
3,3,3,3,4),(97.3893722612844,97.5066501319669,97.5841474786355,97.661562796988,
97.738911716656,97.8162098196274,97.8934726509519,97.9707286640726,98.0479838176341,
98.1252521589769,98.2025477402324,98.2799313482162,98.3573605564852,98.4349098975958,
98.5053898678291,98.5814413155481,98.6573979064417,98.733276427371,98.8090935850679,
98.8848660248241,98.9622739721825,99.0380220205186,99.1137780825166,99.1895571690929,
99.2682002777425,99.3441131905844,99.4200835705738,99.4961610642474,99.5041296036913,
99.582665543746,99.6611086733647,99.7394735009136,99.8177744793012,99.8960260157516,
99.9742455732929,100.052448494847,100.130647779342,100.208856421153,100.287120068014,
100.365412173692,100.443787986843,100.502869339553,100.582511245979,100.662082865721,
100.74159509469,100.82105042838,100.900471604438,100.979868266015,101.002239207485,
101.083469304111,101.164748195163,101.248963415226,101.330394268647,101.416001672031,
101.501609075416,101.586852402349,101.626377961936),.UNSPECIFIED.);
#3325=B_SPLINE_CURVE_WITH_KNOTS('',3,(#192568,#192569,#192570,#192571,#192572,
#192573,#192574,#192575,#192576,#192577,#192578,#192579,#192580,#192581,
#192582,#192583,#192584,#192585,#192586,#192587,#192588,#192589,#192590,
#192591,#192592,#192593,#192594,#192595,#192596,#192597,#192598,#192599,
#192600,#192601,#192602,#192603,#192604,#192605,#192606,#192607,#192608,
#192609,#192610,#192611,#192612,#192613,#192614,#192615,#192616,#192617,
#192618,#192619,#192620,#192621,#192622,#192623,#192624,#192625,#192626,
#192627,#192628,#192629,#192630,#192631,#192632,#192633,#192634,#192635,
#192636,#192637,#192638,#192639,#192640,#192641,#192642,#192643,#192644,
#192645,#192646,#192647,#192648,#192649,#192650,#192651,#192652,#192653,
#192654,#192655,#192656,#192657,#192658,#192659,#192660,#192661,#192662,
#192663,#192664,#192665,#192666,#192667,#192668,#192669,#192670,#192671,
#192672,#192673,#192674,#192675,#192676,#192677,#192678,#192679,#192680,
#192681,#192682,#192683,#192684,#192685,#192686,#192687,#192688,#192689,
#192690,#192691,#192692,#192693,#192694,#192695,#192696,#192697,#192698,
#192699,#192700,#192701,#192702,#192703,#192704,#192705,#192706,#192707,
#192708,#192709,#192710,#192711,#192712,#192713,#192714,#192715,#192716,
#192717,#192718,#192719,#192720,#192721,#192722,#192723,#192724),
 .UNSPECIFIED.,.F.,.F.,(4,3,3,3,3,3,3,3,3,3,3,3,3,3,3,3,3,3,3,3,3,3,3,3,
3,3,3,3,3,3,3,3,3,3,3,3,3,3,3,3,3,3,3,3,3,3,3,3,3,3,3,3,4),(103.672557568464,
103.75501977455,103.837481632338,103.919943148679,104.002404330423,104.084865184419,
104.167325717518,104.249785936568,104.332245848419,104.414705459918,104.497164777915,
104.579623809257,104.662082560792,104.744541039368,104.826999251833,104.909457205033,
104.991914905816,105.074372361028,105.156829577515,105.242842165305,105.326166859726,
105.408633465284,105.491099226635,105.573564171193,105.656028326371,105.738491719578,
105.820954378222,105.903416329706,105.985877601432,106.0683382208,106.150798215207,
106.233257612049,106.315716438717,106.398174722603,106.480632491097,106.563089771585,
106.647223685034,106.729689683332,106.812154059881,106.894616924323,106.97707838628,
107.059538555354,107.141997541128,107.224455453171,107.310052569872,107.392517306815,
107.474979079114,107.557438325205,107.639895483383,107.722358002282,107.804815673566,
107.887274464474,107.909232386775),.UNSPECIFIED.);
#3326=B_SPLINE_CURVE_WITH_KNOTS('',3,(#192725,#192726,#192727,#192728,#192729,
#192730,#192731,#192732,#192733,#192734,#192735,#192736,#192737,#192738,
#192739,#192740,#192741,#192742,#192743,#192744,#192745,#192746,#192747,
#192748,#192749,#192750,#192751,#192752,#192753,#192754,#192755,#192756,
#192757,#192758,#192759,#192760,#192761,#192762,#192763,#192764,#192765,
#192766,#192767,#192768,#192769,#192770,#192771,#192772,#192773,#192774,
#192775,#192776,#192777,#192778,#192779,#192780,#192781,#192782,#192783,
#192784,#192785,#192786,#192787,#192788,#192789,#192790,#192791,#192792,
#192793,#192794,#192795,#192796,#192797,#192798,#192799,#192800,#192801,
#192802,#192803,#192804,#192805,#192806,#192807,#192808,#192809),
 .UNSPECIFIED.,.F.,.F.,(4,3,3,3,3,3,3,3,3,3,3,3,3,3,3,3,3,3,3,3,3,3,3,3,
3,3,3,3,4),(101.626277039953,101.703531015496,101.780794228109,101.858080727786,
101.939226652258,102.016644139276,102.094116948687,102.171693488692,102.182664425672,
102.258715873391,102.334672464285,102.410550985214,102.486368142911,102.562140582667,
102.639548530025,102.715296578361,102.79105264036,102.866831726936,102.945474835586,
103.021387748428,103.097358128417,103.173435622091,103.181404161534,103.266548277653,
103.351528959913,103.436236242929,103.520771012648,103.605017726543,103.672557568464),
 .UNSPECIFIED.);
#3327=B_SPLINE_CURVE_WITH_KNOTS('',3,(#192811,#192812,#192813,#192814,#192815,
#192816,#192817,#192818,#192819,#192820,#192821,#192822,#192823,#192824,
#192825,#192826,#192827,#192828,#192829,#192830,#192831,#192832,#192833,
#192834,#192835,#192836,#192837,#192838,#192839,#192840,#192841,#192842,
#192843,#192844,#192845,#192846,#192847,#192848,#192849,#192850,#192851,
#192852,#192853,#192854,#192855,#192856,#192857,#192858,#192859,#192860,
#192861,#192862,#192863,#192864,#192865,#192866,#192867,#192868,#192869,
#192870,#192871,#192872,#192873,#192874,#192875,#192876,#192877,#192878,
#192879,#192880,#192881,#192882,#192883,#192884,#192885,#192886,#192887,
#192888,#192889,#192890,#192891,#192892),.UNSPECIFIED.,.F.,.F.,(4,3,3,3,
3,3,3,3,3,3,3,3,3,3,3,3,3,3,3,3,3,3,3,3,3,3,3,4),(101.626377961936,101.71150068053,
101.796466817973,101.881320416128,101.965990945276,102.000978943347,102.077521946333,
102.154059490676,102.230606183444,102.307208723732,102.383842469048,102.460559856894,
102.500348811278,102.579895911359,102.659382742726,102.738821570306,102.818224621553,
102.897604095361,102.97698481758,103.056368221294,103.135765389396,103.215187412392,
103.29468084577,103.374212675158,103.453833403137,103.49908854714,103.592986426315,
103.672557568464),.UNSPECIFIED.);
#3328=B_SPLINE_CURVE_WITH_KNOTS('',3,(#192893,#192894,#192895,#192896,#192897,
#192898,#192899,#192900,#192901,#192902,#192903,#192904,#192905,#192906,
#192907,#192908,#192909,#192910,#192911,#192912,#192913,#192914,#192915,
#192916,#192917,#192918,#192919,#192920,#192921,#192922,#192923,#192924,
#192925,#192926,#192927,#192928,#192929,#192930,#192931,#192932,#192933,
#192934,#192935,#192936,#192937,#192938,#192939,#192940,#192941,#192942,
#192943,#192944,#192945,#192946,#192947,#192948,#192949,#192950,#192951,
#192952,#192953,#192954,#192955,#192956,#192957,#192958,#192959,#192960,
#192961,#192962,#192963,#192964,#192965,#192966,#192967,#192968,#192969,
#192970,#192971,#192972,#192973,#192974,#192975,#192976,#192977,#192978,
#192979,#192980,#192981,#192982,#192983,#192984,#192985,#192986,#192987,
#192988,#192989,#192990,#192991,#192992,#192993,#192994,#192995,#192996,
#192997,#192998,#192999,#193000,#193001,#193002,#193003,#193004,#193005,
#193006,#193007,#193008,#193009,#193010,#193011,#193012,#193013,#193014,
#193015,#193016,#193017,#193018,#193019,#193020,#193021,#193022,#193023,
#193024,#193025,#193026,#193027,#193028,#193029,#193030,#193031,#193032,
#193033,#193034,#193035,#193036,#193037,#193038,#193039,#193040,#193041,
#193042,#193043,#193044,#193045,#193046,#193047,#193048,#193049,#193050,
#193051,#193052,#193053,#193054,#193055,#193056,#193057,#193058,#193059,
#193060,#193061,#193062,#193063,#193064),.UNSPECIFIED.,.F.,.F.,(4,3,3,3,
3,3,3,3,3,3,3,3,3,3,3,3,3,3,3,3,3,3,3,3,3,3,3,3,3,3,3,3,3,3,3,3,3,3,3,3,
3,3,3,3,3,3,3,3,3,3,3,3,3,3,3,3,3,4),(103.67255756858,103.746175586763,
103.819744102075,103.893283544664,103.966817544084,103.998458415071,104.081953222117,
104.165604899106,104.249495294347,104.33349973973,104.417690697953,104.497828283002,
104.575325629671,104.652740948023,104.730089867691,104.807387970662,104.884650801987,
104.961906815107,105.039161968669,105.116430310012,105.193725891267,105.271109499251,
105.34853870752,105.426088048631,105.496568018864,105.572619466583,105.648576057477,
105.724454578406,105.800271736103,105.876044175859,105.953452123218,106.029200171554,
106.104956233552,106.180735320128,106.259378428778,106.33529134162,106.41126172161,
106.487339215283,106.495307754727,106.573843694782,106.652286824401,106.73065165195,
106.808952630337,106.887204166788,106.96542372433,107.043626645884,107.121825930379,
107.20003457219,107.278298219051,107.356590324728,107.43496613788,107.494047490589,
107.573696677105,107.653274666236,107.732778556315,107.812238285843,107.891659120703,
107.909226129751),.UNSPECIFIED.);
#3329=B_SPLINE_CURVE_WITH_KNOTS('',3,(#193070,#193071,#193072,#193073,#193074,
#193075,#193076,#193077,#193078,#193079,#193080,#193081,#193082,#193083,
#193084,#193085,#193086,#193087,#193088,#193089,#193090,#193091,#193092,
#193093,#193094,#193095,#193096,#193097,#193098,#193099,#193100,#193101,
#193102,#193103,#193104,#193105,#193106,#193107,#193108,#193109,#193110,
#193111,#193112,#193113,#193114,#193115,#193116,#193117,#193118,#193119,
#193120,#193121,#193122,#193123,#193124,#193125,#193126,#193127,#193128,
#193129,#193130,#193131,#193132,#193133,#193134,#193135,#193136,#193137,
#193138,#193139,#193140,#193141,#193142,#193143,#193144,#193145,#193146,
#193147,#193148,#193149,#193150,#193151,#193152,#193153,#193154,#193155,
#193156,#193157,#193158,#193159,#193160,#193161,#193162,#193163,#193164,
#193165,#193166,#193167,#193168,#193169,#193170,#193171,#193172,#193173,
#193174,#193175,#193176,#193177,#193178,#193179,#193180,#193181,#193182,
#193183,#193184,#193185,#193186,#193187,#193188,#193189,#193190,#193191,
#193192,#193193,#193194,#193195,#193196,#193197,#193198,#193199,#193200,
#193201,#193202,#193203,#193204,#193205,#193206,#193207,#193208,#193209,
#193210,#193211,#193212,#193213,#193214,#193215,#193216,#193217,#193218,
#193219,#193220,#193221,#193222,#193223,#193224,#193225,#193226,#193227,
#193228,#193229,#193230,#193231,#193232,#193233,#193234,#193235,#193236,
#193237,#193238),.UNSPECIFIED.,.F.,.F.,(4,3,3,3,3,3,3,3,3,3,3,3,3,3,3,3,
3,3,3,3,3,3,3,3,3,3,3,3,3,3,3,3,3,3,3,3,3,3,3,3,3,3,3,3,3,3,3,3,3,3,3,3,
3,3,3,3,4),(109.955742875644,110.055365128407,110.157813204224,110.17258231257,
110.251118252625,110.329561382243,110.407926209792,110.48622718818,110.56447872463,
110.642698282171,110.720901203725,110.79910048822,110.877309130032,110.955572776893,
111.03386488257,111.112240695722,111.171322048432,111.250963954858,111.3305355746,
111.410047803569,111.489503137259,111.568924313317,111.648320974894,111.670691916363,
111.751922012989,111.83320090404,111.917416124103,111.998846977524,112.084454380909,
112.170061784294,112.255305082593,112.340470156748,112.425484524625,112.510391833421,
112.595106335693,112.669431652225,112.745974655211,112.822512199553,112.899058892321,
112.975661432609,113.052295177925,113.129012565771,113.168801520156,113.248348620237,
113.327835451604,113.407274279184,113.486677330432,113.56605680424,113.645437526458,
113.724820930173,113.804218098275,113.883640121271,113.96313355465,114.042665384037,
114.122286112016,114.167541256018,114.192890879176),.UNSPECIFIED.);
#3330=B_SPLINE_CURVE_WITH_KNOTS('',3,(#193239,#193240,#193241,#193242,#193243,
#193244,#193245,#193246,#193247,#193248,#193249,#193250,#193251,#193252,
#193253,#193254,#193255,#193256,#193257,#193258,#193259,#193260,#193261,
#193262,#193263,#193264,#193265,#193266,#193267,#193268,#193269,#193270,
#193271,#193272,#193273,#193274,#193275,#193276,#193277,#193278,#193279,
#193280,#193281,#193282,#193283,#193284,#193285,#193286,#193287,#193288,
#193289,#193290,#193291,#193292,#193293,#193294,#193295,#193296,#193297,
#193298,#193299,#193300,#193301,#193302,#193303,#193304,#193305,#193306,
#193307,#193308,#193309,#193310,#193311,#193312,#193313,#193314),
 .UNSPECIFIED.,.F.,.F.,(4,3,3,3,3,3,3,3,3,3,3,3,3,3,3,3,3,3,3,3,3,3,3,3,
3,4),(107.909232386775,107.991693990533,108.074154928412,108.15661522781,
108.239074916123,108.321534020746,108.403992569069,108.486450588483,108.568908106376,
108.655585279455,108.738052065064,108.820517178195,108.902980728502,108.985442825616,
109.067903579148,109.15036309869,109.232821493817,109.315278874088,109.397745259907,
109.480208461531,109.56266891748,109.645127066116,109.727592670128,109.810052548705,
109.892516660442,109.955742875644),.UNSPECIFIED.);
#3331=B_SPLINE_CURVE_WITH_KNOTS('',3,(#193316,#193317,#193318,#193319,#193320,
#193321,#193322,#193323,#193324,#193325,#193326,#193327,#193328,#193329,
#193330,#193331,#193332,#193333,#193334,#193335,#193336,#193337,#193338,
#193339,#193340,#193341,#193342,#193343,#193344,#193345,#193346,#193347,
#193348,#193349,#193350,#193351,#193352,#193353,#193354,#193355,#193356,
#193357,#193358,#193359,#193360,#193361,#193362,#193363,#193364,#193365,
#193366,#193367,#193368,#193369,#193370,#193371,#193372,#193373,#193374,
#193375,#193376,#193377,#193378,#193379,#193380,#193381,#193382,#193383,
#193384,#193385,#193386,#193387,#193388,#193389,#193390,#193391,#193392,
#193393,#193394,#193395,#193396,#193397),.UNSPECIFIED.,.F.,.F.,(4,3,3,3,
3,3,3,3,3,3,3,3,3,3,3,3,3,3,3,3,3,3,3,3,3,3,3,4),(107.909226129751,107.988618440932,
107.99341735852,108.074647455146,108.155926346196,108.24014156626,108.32157241968,
108.407179823066,108.492787226451,108.57803052475,108.663195598904,108.748209966782,
108.833117275578,108.91783177785,108.992157094382,109.068700097368,109.145237641711,
109.221784334479,109.298386874767,109.375020620084,109.45173800793,109.491526962313,
109.576384599114,109.661154257058,109.745770463507,109.830278775386,109.9146126653,
109.955655827855),.UNSPECIFIED.);
#3332=B_SPLINE_CURVE_WITH_KNOTS('',3,(#193398,#193399,#193400,#193401,#193402,
#193403,#193404,#193405,#193406,#193407,#193408,#193409,#193410,#193411,
#193412,#193413,#193414,#193415,#193416,#193417,#193418,#193419,#193420,
#193421,#193422,#193423,#193424,#193425,#193426,#193427,#193428,#193429,
#193430,#193431,#193432,#193433,#193434,#193435,#193436,#193437,#193438,
#193439,#193440,#193441,#193442,#193443,#193444,#193445,#193446,#193447,
#193448,#193449,#193450,#193451,#193452,#193453,#193454,#193455,#193456,
#193457,#193458,#193459,#193460,#193461,#193462,#193463,#193464,#193465,
#193466,#193467,#193468,#193469,#193470,#193471,#193472,#193473,#193474,
#193475,#193476,#193477,#193478,#193479,#193480,#193481,#193482,#193483,
#193484,#193485,#193486,#193487,#193488,#193489,#193490,#193491,#193492,
#193493,#193494,#193495,#193496,#193497,#193498,#193499,#193500,#193501,
#193502,#193503,#193504,#193505,#193506,#193507,#193508,#193509,#193510,
#193511,#193512,#193513,#193514,#193515,#193516,#193517,#193518,#193519,
#193520,#193521,#193522,#193523,#193524,#193525,#193526,#193527,#193528,
#193529,#193530,#193531,#193532,#193533,#193534,#193535,#193536,#193537,
#193538,#193539,#193540,#193541,#193542,#193543,#193544,#193545,#193546,
#193547,#193548,#193549,#193550,#193551,#193552,#193553,#193554),
 .UNSPECIFIED.,.F.,.F.,(4,3,3,3,3,3,3,3,3,3,3,3,3,3,3,3,3,3,3,3,3,3,3,3,
3,3,3,3,3,3,3,3,3,3,3,3,3,3,3,3,3,3,3,3,3,3,3,3,3,3,3,3,4),(109.95577038367,
110.038232589638,110.120694447311,110.203155963539,110.285617145173,110.368077999061,
110.450538532054,110.532998751001,110.61545866275,110.69791827415,110.78037759205,
110.862836623298,110.945295374741,111.027753853227,111.110212065604,111.192670018719,
111.275127719419,111.35758517455,111.440042390959,111.526054119178,111.609377980889,
111.691844586179,111.77431034727,111.856775291577,111.939239446512,112.021702839485,
112.104165497903,112.18662744917,112.269088720687,112.351549339856,112.434009334072,
112.51646873073,112.598927557224,112.681385840945,112.763843609281,112.846300889621,
112.930433189891,113.012899187698,113.095363563787,113.177826427801,113.260287889363,
113.342748058073,113.425207043517,113.507664955261,113.593259047597,113.675723783724,
113.758185555317,113.840644800816,113.923101958515,114.005564475944,114.088022146208,
114.170480934839,114.192417693954),.UNSPECIFIED.);
#3333=B_SPLINE_CURVE_WITH_KNOTS('',3,(#193560,#193561,#193562,#193563,#193564,
#193565,#193566,#193567,#193568,#193569,#193570,#193571,#193572,#193573,
#193574,#193575,#193576,#193577,#193578,#193579,#193580,#193581,#193582,
#193583,#193584,#193585,#193586,#193587,#193588,#193589,#193590,#193591,
#193592,#193593,#193594,#193595,#193596,#193597,#193598,#193599,#193600,
#193601,#193602,#193603,#193604,#193605,#193606,#193607,#193608,#193609,
#193610,#193611,#193612,#193613,#193614,#193615,#193616,#193617,#193618,
#193619,#193620,#193621,#193622,#193623,#193624,#193625,#193626,#193627,
#193628,#193629,#193630,#193631,#193632,#193633,#193634,#193635,#193636,
#193637,#193638,#193639,#193640,#193641,#193642,#193643,#193644,#193645,
#193646,#193647,#193648,#193649,#193650,#193651,#193652,#193653,#193654,
#193655,#193656,#193657,#193658,#193659,#193660,#193661,#193662,#193663,
#193664,#193665,#193666,#193667,#193668,#193669,#193670,#193671,#193672,
#193673,#193674,#193675,#193676,#193677,#193678,#193679,#193680,#193681,
#193682,#193683,#193684,#193685,#193686,#193687,#193688,#193689,#193690,
#193691,#193692,#193693,#193694,#193695,#193696,#193697,#193698,#193699,
#193700,#193701,#193702,#193703,#193704,#193705,#193706,#193707,#193708,
#193709,#193710,#193711,#193712,#193713,#193714,#193715,#193716,#193717,
#193718,#193719,#193720,#193721,#193722,#193723,#193724,#193725,#193726,
#193727,#193728),.UNSPECIFIED.,.F.,.F.,(4,3,3,3,3,3,3,3,3,3,3,3,3,3,3,3,
3,3,3,3,3,3,3,3,3,3,3,3,3,3,3,3,3,3,3,3,3,3,3,3,3,3,3,3,3,3,3,3,3,3,3,3,
3,3,3,3,4),(116.238928182907,116.314137825691,116.389260630726,116.464313746745,
116.539314224263,116.617370004181,116.692328870866,116.767289769362,116.842268021846,
116.917278970001,116.992379284292,117.067532383174,117.142793754632,117.163760463605,
117.24229640366,117.320739533279,117.399104360828,117.477405339215,117.555656875666,
117.633876433207,117.712079354761,117.790278639256,117.868487281067,117.946750927929,
118.025043033606,118.103418846758,118.162500199467,118.242142105893,118.321713725635,
118.401225954604,118.480681288294,118.560102464352,118.639499125928,118.661870067398,
118.743100164024,118.824379055075,118.908594275139,118.990025128559,119.075632531944,
119.161239935329,119.246483233628,119.331648307784,119.416662675662,119.501569984457,
119.58628448673,119.66060980326,119.737152806246,119.813690350589,119.890237043357,
119.966839583645,120.043473328961,120.120190716807,120.159979671192,120.239520074869,
120.319006382661,120.398442502006,120.475571182131),.UNSPECIFIED.);
#3334=B_SPLINE_CURVE_WITH_KNOTS('',3,(#193729,#193730,#193731,#193732,#193733,
#193734,#193735,#193736,#193737,#193738,#193739,#193740,#193741,#193742,
#193743,#193744,#193745,#193746,#193747,#193748,#193749,#193750,#193751,
#193752,#193753,#193754,#193755,#193756,#193757,#193758,#193759,#193760,
#193761,#193762,#193763,#193764,#193765,#193766,#193767,#193768,#193769,
#193770,#193771,#193772,#193773,#193774,#193775,#193776,#193777,#193778,
#193779,#193780,#193781,#193782,#193783,#193784,#193785,#193786,#193787,
#193788,#193789,#193790,#193791,#193792,#193793,#193794,#193795,#193796,
#193797,#193798,#193799,#193800,#193801,#193802,#193803,#193804,#193805,
#193806,#193807),.UNSPECIFIED.,.F.,.F.,(4,3,3,3,3,3,3,3,3,3,3,3,3,3,3,3,
3,3,3,3,3,3,3,3,3,3,4),(114.192890879176,114.270516977951,114.3480614362,
114.427773858137,114.505186939995,114.586049031973,114.66691112395,114.750405930996,
114.834057607986,114.917948003227,115.001952448611,115.086143406834,115.166280991881,
115.24377833855,115.321193656902,115.39854257657,115.475840679541,115.553103510865,
115.630359523986,115.707614677547,115.78488301889,115.862178600146,115.939562208129,
116.016991416398,116.094540757509,116.165020727743,116.238928182823),
 .UNSPECIFIED.);
#3335=B_SPLINE_CURVE_WITH_KNOTS('',3,(#193809,#193810,#193811,#193812,#193813,
#193814,#193815,#193816,#193817,#193818,#193819,#193820,#193821,#193822,
#193823,#193824,#193825,#193826,#193827,#193828,#193829,#193830,#193831,
#193832,#193833,#193834,#193835,#193836,#193837,#193838,#193839,#193840,
#193841,#193842,#193843,#193844,#193845,#193846,#193847,#193848,#193849,
#193850,#193851,#193852,#193853,#193854,#193855,#193856,#193857,#193858,
#193859,#193860,#193861,#193862,#193863,#193864,#193865,#193866,#193867,
#193868,#193869,#193870,#193871,#193872,#193873,#193874,#193875,#193876,
#193877,#193878,#193879,#193880,#193881,#193882,#193883,#193884),
 .UNSPECIFIED.,.F.,.F.,(4,3,3,3,3,3,3,3,3,3,3,3,3,3,3,3,3,3,3,3,3,3,3,3,
3,4),(114.192417693954,114.274879297712,114.357340235592,114.43980053499,
114.522260223303,114.604719327925,114.687177876248,114.769635895662,114.852093413555,
114.938770586626,115.021237372234,115.103702485365,115.186166035672,115.268628132786,
115.351088886318,115.43354840586,115.516006800987,115.598464181258,115.680930567077,
115.763393768702,115.84585422465,115.928312373286,116.010777977298,116.093237855875,
116.175701967612,116.238928182684),.UNSPECIFIED.);
#3336=B_SPLINE_CURVE_WITH_KNOTS('',3,(#193885,#193886,#193887,#193888,#193889,
#193890,#193891,#193892,#193893,#193894,#193895,#193896,#193897,#193898,
#193899,#193900,#193901,#193902,#193903,#193904,#193905,#193906,#193907,
#193908,#193909,#193910,#193911,#193912,#193913,#193914,#193915,#193916,
#193917,#193918,#193919,#193920,#193921,#193922,#193923,#193924,#193925,
#193926,#193927,#193928,#193929,#193930,#193931,#193932,#193933,#193934,
#193935,#193936,#193937,#193938,#193939,#193940,#193941,#193942,#193943,
#193944,#193945,#193946,#193947,#193948,#193949,#193950,#193951,#193952,
#193953,#193954,#193955,#193956,#193957,#193958,#193959,#193960,#193961,
#193962,#193963,#193964,#193965,#193966,#193967,#193968,#193969,#193970,
#193971,#193972,#193973,#193974,#193975,#193976,#193977,#193978,#193979,
#193980,#193981,#193982,#193983,#193984,#193985,#193986,#193987,#193988,
#193989,#193990,#193991,#193992,#193993,#193994,#193995,#193996,#193997,
#193998,#193999,#194000,#194001,#194002,#194003,#194004,#194005,#194006,
#194007,#194008,#194009,#194010,#194011,#194012,#194013,#194014,#194015,
#194016,#194017,#194018,#194019,#194020,#194021,#194022,#194023,#194024,
#194025,#194026,#194027,#194028,#194029,#194030,#194031,#194032,#194033,
#194034,#194035,#194036,#194037,#194038,#194039,#194040,#194041),
 .UNSPECIFIED.,.F.,.F.,(4,3,3,3,3,3,3,3,3,3,3,3,3,3,3,3,3,3,3,3,3,3,3,3,
3,3,3,3,3,3,3,3,3,3,3,3,3,3,3,3,3,3,3,3,3,3,3,3,3,3,3,3,4),(116.238928182823,
116.321390388909,116.403852246697,116.486313763038,116.568774944782,116.651235798778,
116.733696331877,116.816156550927,116.898616462778,116.981076074277,117.063535392274,
117.145994423616,117.228453175152,117.310911653728,117.393369866193,117.475827819393,
117.558285520175,117.640742975387,117.723200191875,117.809212779664,117.892537474085,
117.975004079643,118.057469840994,118.139934785552,118.22239894073,118.304862333937,
118.387324992581,118.469786944065,118.552248215791,118.634708835159,118.717168829567,
118.799628226408,118.882087053076,118.964545336963,119.047003105456,119.129460385944,
119.213594299393,119.296060297691,119.37852467424,119.460987538682,119.543449000639,
119.625909169713,119.708368155488,119.790826067531,119.876423184231,119.958887921175,
120.041349693473,120.123808939564,120.206266097742,120.288728616641,120.371186287925,
120.453645078833,120.475603001134),.UNSPECIFIED.);
#3337=B_SPLINE_CURVE_WITH_KNOTS('',3,(#194047,#194048,#194049,#194050,#194051,
#194052,#194053,#194054,#194055,#194056,#194057,#194058,#194059,#194060,
#194061,#194062,#194063,#194064,#194065,#194066,#194067,#194068,#194069,
#194070,#194071,#194072,#194073,#194074,#194075,#194076,#194077,#194078,
#194079,#194080,#194081,#194082,#194083,#194084,#194085,#194086,#194087,
#194088,#194089,#194090,#194091,#194092,#194093,#194094,#194095,#194096,
#194097,#194098,#194099,#194100,#194101,#194102,#194103,#194104,#194105,
#194106,#194107,#194108,#194109,#194110,#194111,#194112,#194113,#194114,
#194115,#194116,#194117,#194118,#194119,#194120,#194121,#194122,#194123,
#194124,#194125,#194126,#194127,#194128,#194129,#194130,#194131,#194132,
#194133,#194134,#194135,#194136,#194137,#194138,#194139,#194140,#194141,
#194142,#194143,#194144,#194145,#194146,#194147,#194148,#194149,#194150,
#194151,#194152,#194153,#194154,#194155,#194156,#194157,#194158,#194159,
#194160,#194161,#194162,#194163,#194164,#194165,#194166,#194167,#194168,
#194169,#194170,#194171,#194172,#194173,#194174,#194175,#194176,#194177,
#194178,#194179,#194180,#194181,#194182,#194183,#194184,#194185,#194186,
#194187,#194188,#194189,#194190,#194191,#194192,#194193,#194194,#194195,
#194196,#194197,#194198,#194199,#194200,#194201,#194202,#194203,#194204,
#194205,#194206,#194207,#194208,#194209,#194210,#194211,#194212,#194213,
#194214,#194215),.UNSPECIFIED.,.F.,.F.,(4,3,3,3,3,3,3,3,3,3,3,3,3,3,3,3,
3,3,3,3,3,3,3,3,3,3,3,3,3,3,3,3,3,3,3,3,3,3,3,3,3,3,3,3,3,3,3,3,3,3,3,3,
3,3,3,3,4),(122.522113490003,122.6013741636,122.680240720641,122.75914499531,
122.838098684334,122.917623732945,122.996756414602,123.07647764669,123.156198878778,
123.232250326497,123.308206917391,123.38408543832,123.459902596017,123.535675035773,
123.613082983131,123.688831031467,123.764587093465,123.840366180041,123.919009288691,
123.994922201533,124.070892581522,124.146970075196,124.15493861464,124.233474554695,
124.311917684314,124.390282511863,124.46858349025,124.5468350267,124.625054584241,
124.703257505795,124.78145679029,124.859665432102,124.937929078963,125.01622118464,
125.094596997792,125.153678350502,125.233320256929,125.312891876671,125.392404105639,
125.47185943933,125.551280615387,125.630677276964,125.653048218434,125.73427831506,
125.815557206111,125.899772426174,125.981203279595,126.06681068298,126.152418086365,
126.237661384664,126.322826458819,126.407840826696,126.492748135492,126.577462637764,
126.651787954296,126.728328092807,126.758858075524),.UNSPECIFIED.);
#3338=B_SPLINE_CURVE_WITH_KNOTS('',3,(#194216,#194217,#194218,#194219,#194220,
#194221,#194222,#194223,#194224,#194225,#194226,#194227,#194228,#194229,
#194230,#194231,#194232,#194233,#194234,#194235,#194236,#194237,#194238,
#194239,#194240,#194241,#194242,#194243,#194244,#194245,#194246,#194247,
#194248,#194249,#194250,#194251,#194252,#194253,#194254,#194255,#194256,
#194257,#194258,#194259,#194260,#194261,#194262,#194263,#194264,#194265,
#194266,#194267,#194268,#194269,#194270,#194271,#194272,#194273,#194274,
#194275,#194276,#194277,#194278,#194279,#194280,#194281,#194282,#194283,
#194284,#194285,#194286,#194287,#194288,#194289,#194290,#194291,#194292,
#194293,#194294,#194295,#194296,#194297),.UNSPECIFIED.,.F.,.F.,(4,3,3,3,
3,3,3,3,3,3,3,3,3,3,3,3,3,3,3,3,3,3,3,3,3,3,3,4),(120.475571182131,120.55495116409,
120.634331973151,120.713715144904,120.793111762126,120.872532915006,120.952025395174,
121.031555977971,121.111175974327,121.158719407054,121.236375165248,121.313944730979,
121.39144203761,121.468870676044,121.54625952217,121.623622416347,121.658089274985,
121.741584082031,121.825235759021,121.909126154262,121.993130599645,122.077321557868,
122.157459142916,122.242489520718,122.327223768168,122.411766191998,122.496020247112,
122.522113489888),.UNSPECIFIED.);
#3339=B_SPLINE_CURVE_WITH_KNOTS('',3,(#194299,#194300,#194301,#194302,#194303,
#194304,#194305,#194306,#194307,#194308,#194309,#194310,#194311,#194312,
#194313,#194314,#194315,#194316,#194317,#194318,#194319,#194320,#194321,
#194322,#194323,#194324,#194325,#194326,#194327,#194328,#194329,#194330,
#194331,#194332,#194333,#194334,#194335,#194336,#194337,#194338,#194339,
#194340,#194341,#194342,#194343,#194344,#194345,#194346,#194347,#194348,
#194349,#194350,#194351,#194352,#194353,#194354,#194355,#194356,#194357,
#194358,#194359,#194360,#194361,#194362,#194363,#194364,#194365,#194366,
#194367,#194368,#194369,#194370,#194371,#194372,#194373,#194374),
 .UNSPECIFIED.,.F.,.F.,(4,3,3,3,3,3,3,3,3,3,3,3,3,3,3,3,3,3,3,3,3,3,3,3,
3,4),(120.475603001134,120.558064604892,120.640525542771,120.722985842169,
120.805445530482,120.887904635105,120.970363183428,121.052821202842,121.135278720735,
121.221955893814,121.304422679423,121.386887792554,121.469351342861,121.551813439975,
121.634274193507,121.716733713049,121.799192108176,121.881649488447,121.964115874266,
122.04657907589,122.129039531839,122.211497680475,122.293963284487,122.376423163064,
122.458887274801,122.522113490003),.UNSPECIFIED.);
#3340=B_SPLINE_CURVE_WITH_KNOTS('',3,(#194375,#194376,#194377,#194378,#194379,
#194380,#194381,#194382,#194383,#194384,#194385,#194386,#194387,#194388,
#194389,#194390,#194391,#194392,#194393,#194394,#194395,#194396,#194397,
#194398,#194399,#194400,#194401,#194402,#194403,#194404,#194405,#194406,
#194407,#194408,#194409,#194410,#194411,#194412,#194413,#194414,#194415,
#194416,#194417,#194418,#194419,#194420,#194421,#194422,#194423,#194424,
#194425,#194426,#194427,#194428,#194429,#194430,#194431,#194432,#194433,
#194434,#194435,#194436,#194437,#194438,#194439,#194440,#194441,#194442,
#194443,#194444,#194445,#194446,#194447,#194448,#194449,#194450,#194451,
#194452,#194453,#194454,#194455,#194456,#194457,#194458,#194459,#194460,
#194461,#194462,#194463,#194464,#194465,#194466,#194467,#194468,#194469,
#194470,#194471,#194472,#194473,#194474,#194475,#194476,#194477,#194478,
#194479,#194480,#194481,#194482,#194483,#194484,#194485,#194486,#194487,
#194488,#194489,#194490,#194491,#194492,#194493,#194494,#194495,#194496,
#194497,#194498,#194499,#194500,#194501,#194502,#194503,#194504,#194505,
#194506,#194507,#194508,#194509,#194510,#194511,#194512,#194513,#194514,
#194515,#194516,#194517,#194518,#194519,#194520,#194521,#194522,#194523,
#194524,#194525,#194526,#194527,#194528,#194529,#194530,#194531,#194532,
#194533,#194534,#194535,#194536,#194537,#194538,#194539,#194540,#194541,
#194542,#194543),.UNSPECIFIED.,.F.,.F.,(4,3,3,3,3,3,3,3,3,3,3,3,3,3,3,3,
3,3,3,3,3,3,3,3,3,3,3,3,3,3,3,3,3,3,3,3,3,3,3,3,3,3,3,3,3,3,3,3,3,3,3,3,
3,3,3,3,4),(122.522220451277,122.606401533941,122.690490111526,122.774431321878,
122.858272049895,122.941960963335,122.974513396453,123.051056399439,123.127593943782,
123.204140636549,123.280743176838,123.357376922153,123.434094309999,123.473883264384,
123.553430364464,123.632917195832,123.712356023412,123.791759074659,123.871138548467,
123.950519270686,124.0299026744,124.109299842502,124.188721865498,124.268215298876,
124.347747128264,124.427367856243,124.472623000246,124.550278758441,124.627848324171,
124.705345630803,124.782774269237,124.860163115363,124.937526009541,124.971992868177,
125.055487675223,125.139139352212,125.223029747452,125.307034192836,125.391225151059,
125.471362736108,125.548860082777,125.626275401129,125.703624320797,125.780922423768,
125.858185255093,125.935441268213,126.012696421775,126.089964763117,126.167260344372,
126.244643952356,126.322073160625,126.399622501736,126.47010247197,126.546145536087,
126.622105287442,126.697977128334,126.759584805783),.UNSPECIFIED.);
#3341=B_SPLINE_CURVE_WITH_KNOTS('',3,(#194549,#194550,#194551,#194552,#194553,
#194554,#194555,#194556,#194557,#194558,#194559,#194560,#194561,#194562,
#194563,#194564,#194565,#194566,#194567,#194568,#194569,#194570,#194571,
#194572,#194573,#194574,#194575,#194576,#194577,#194578,#194579,#194580,
#194581,#194582,#194583,#194584,#194585,#194586,#194587,#194588,#194589,
#194590,#194591,#194592,#194593,#194594,#194595,#194596,#194597,#194598,
#194599,#194600,#194601,#194602,#194603,#194604,#194605,#194606,#194607,
#194608,#194609,#194610,#194611,#194612,#194613,#194614,#194615,#194616,
#194617,#194618,#194619,#194620,#194621,#194622,#194623,#194624,#194625,
#194626,#194627,#194628,#194629,#194630,#194631,#194632,#194633,#194634,
#194635,#194636,#194637,#194638,#194639,#194640,#194641,#194642,#194643,
#194644,#194645,#194646,#194647,#194648,#194649,#194650,#194651,#194652,
#194653,#194654,#194655,#194656,#194657,#194658,#194659,#194660,#194661,
#194662,#194663,#194664,#194665,#194666,#194667,#194668,#194669,#194670,
#194671,#194672,#194673,#194674,#194675,#194676,#194677,#194678,#194679,
#194680,#194681,#194682,#194683,#194684,#194685,#194686,#194687,#194688,
#194689,#194690,#194691,#194692,#194693,#194694,#194695,#194696,#194697,
#194698,#194699,#194700,#194701,#194702,#194703,#194704,#194705,#194706,
#194707,#194708,#194709,#194710,#194711,#194712,#194713,#194714,#194715,
#194716,#194717),.UNSPECIFIED.,.F.,.F.,(4,3,3,3,3,3,3,3,3,3,3,3,3,3,3,3,
3,3,3,3,3,3,3,3,3,3,3,3,3,3,3,3,3,3,3,3,3,3,3,3,3,3,3,3,3,3,3,3,3,3,3,3,
3,3,3,3,4),(128.805298797316,128.895499662665,128.986091025251,129.077130579346,
129.148637293951,129.22613464062,129.303549958972,129.38089887864,129.458196981611,
129.535459812936,129.612715826056,129.689970979618,129.767239320961,129.844534902216,
129.9219185102,129.999347718469,130.07689705958,130.147377029813,130.223428477532,
130.299385068426,130.375263589355,130.451080747052,130.526853186808,130.604261134167,
130.680009182503,130.755765244501,130.831544331078,130.910187439727,130.986100352569,
131.062070732559,131.138148226232,131.146116765676,131.224652705731,131.303095835349,
131.381460662898,131.459761641286,131.538013177737,131.616232735278,131.694435656832,
131.772634941327,131.850843583138,131.92910723,132.007399335677,132.085775148829,
132.144856501538,132.224498407964,132.304070027706,132.383582256675,132.463037590365,
132.542458766422,132.621855427999,132.644226369469,132.725444205775,132.806752399596,
132.888103408676,132.969548948727,133.041617861985),.UNSPECIFIED.);
#3342=B_SPLINE_CURVE_WITH_KNOTS('',3,(#194718,#194719,#194720,#194721,#194722,
#194723,#194724,#194725,#194726,#194727,#194728,#194729,#194730,#194731,
#194732,#194733,#194734,#194735,#194736,#194737,#194738,#194739,#194740,
#194741,#194742,#194743,#194744,#194745,#194746,#194747,#194748,#194749,
#194750,#194751,#194752,#194753,#194754,#194755,#194756,#194757,#194758,
#194759,#194760,#194761,#194762,#194763,#194764,#194765,#194766,#194767,
#194768,#194769,#194770,#194771,#194772,#194773,#194774,#194775,#194776,
#194777,#194778,#194779,#194780,#194781,#194782,#194783,#194784,#194785,
#194786,#194787,#194788,#194789,#194790,#194791,#194792,#194793,#194794,
#194795,#194796,#194797,#194798,#194799),.UNSPECIFIED.,.F.,.F.,(4,3,3,3,
3,3,3,3,3,3,3,3,3,3,3,3,3,3,3,3,3,3,3,3,3,3,3,4),(126.758858075524,126.835397517614,
126.914337593767,126.990951939283,127.071054880755,127.151157822227,127.230704922307,
127.310191753675,127.389630581255,127.469033632501,127.54841310631,127.627793828529,
127.707177232243,127.786574400345,127.865996423342,127.94548985672,128.025021686108,
128.104642414087,128.149897558089,128.227553316283,128.305122882014,128.382620188644,
128.460048827078,128.537437673205,128.614800567382,128.64926742602,128.727283111602,
128.805298797183),.UNSPECIFIED.);
#3343=B_SPLINE_CURVE_WITH_KNOTS('',3,(#194801,#194802,#194803,#194804,#194805,
#194806,#194807,#194808,#194809,#194810,#194811,#194812,#194813,#194814,
#194815,#194816,#194817,#194818,#194819,#194820,#194821,#194822,#194823,
#194824,#194825,#194826,#194827,#194828,#194829,#194830,#194831,#194832,
#194833,#194834,#194835,#194836,#194837,#194838,#194839,#194840,#194841,
#194842,#194843,#194844,#194845,#194846,#194847,#194848,#194849,#194850,
#194851,#194852,#194853,#194854,#194855,#194856,#194857,#194858,#194859,
#194860,#194861,#194862,#194863,#194864,#194865,#194866,#194867,#194868,
#194869,#194870,#194871,#194872,#194873,#194874,#194875,#194876,#194877,
#194878,#194879,#194880,#194881,#194882),.UNSPECIFIED.,.F.,.F.,(4,3,3,3,
3,3,3,3,3,3,3,3,3,3,3,3,3,3,3,3,3,3,3,3,3,3,3,4),(126.759584805783,126.835364369514,
126.914549099304,126.990297266019,127.066050982518,127.141825258102,127.217635116655,
127.293538098483,127.369495818183,127.445564880084,127.468842207832,127.547378147886,
127.625821277505,127.704186105054,127.782487083442,127.860738619892,127.938958177434,
128.017161098987,128.095360383483,128.173569025294,128.251832672155,128.330124777833,
128.408500590984,128.467581943695,128.552011157067,128.635508513281,128.720403655231,
128.805298797182),.UNSPECIFIED.);
#3344=B_SPLINE_CURVE_WITH_KNOTS('',3,(#194883,#194884,#194885,#194886,#194887,
#194888,#194889,#194890,#194891,#194892,#194893,#194894,#194895,#194896,
#194897,#194898,#194899,#194900,#194901,#194902,#194903,#194904,#194905,
#194906,#194907,#194908,#194909,#194910,#194911,#194912,#194913,#194914,
#194915,#194916,#194917,#194918,#194919,#194920,#194921,#194922,#194923,
#194924,#194925,#194926,#194927,#194928,#194929,#194930,#194931,#194932,
#194933,#194934,#194935,#194936,#194937,#194938,#194939,#194940,#194941,
#194942,#194943,#194944,#194945,#194946,#194947,#194948,#194949,#194950,
#194951,#194952,#194953,#194954,#194955,#194956,#194957,#194958,#194959,
#194960,#194961,#194962,#194963,#194964,#194965,#194966,#194967,#194968,
#194969,#194970,#194971,#194972,#194973,#194974,#194975,#194976,#194977,
#194978,#194979,#194980,#194981,#194982,#194983,#194984,#194985,#194986,
#194987,#194988,#194989,#194990,#194991,#194992,#194993,#194994,#194995,
#194996,#194997,#194998,#194999,#195000,#195001,#195002,#195003,#195004,
#195005,#195006,#195007,#195008,#195009,#195010,#195011,#195012,#195013,
#195014,#195015,#195016,#195017,#195018,#195019,#195020,#195021,#195022,
#195023,#195024,#195025,#195026,#195027,#195028,#195029,#195030,#195031,
#195032,#195033,#195034,#195035,#195036,#195037,#195038,#195039,#195040,
#195041,#195042,#195043,#195044,#195045,#195046,#195047,#195048,#195049,
#195050,#195051),.UNSPECIFIED.,.F.,.F.,(4,3,3,3,3,3,3,3,3,3,3,3,3,3,3,3,
3,3,3,3,3,3,3,3,3,3,3,3,3,3,3,3,3,3,3,3,3,3,3,3,3,3,3,3,3,3,3,3,3,3,3,3,
3,3,3,3,4),(128.805298797286,128.880674391654,128.95604640739,128.966951811626,
129.048181908252,129.129460799303,129.213676019366,129.295106872787,129.380714276172,
129.466321679557,129.551564977856,129.63673005201,129.721744419888,129.806651728683,
129.891366230955,129.965691547488,130.042234550474,130.118772094817,130.195318787584,
130.271921327873,130.348555073189,130.425272461035,130.465061415419,130.544608515499,
130.624095346867,130.703534174447,130.782937225694,130.862316699502,130.941697421721,
131.021080825435,131.100477993537,131.179900016534,131.259393449912,131.338925279299,
131.418546007278,131.463801151281,131.541456909475,131.619026475206,131.696523781837,
131.773952420271,131.851341266397,131.928704160575,131.963171019212,132.046665826258,
132.130317503248,132.214207898489,132.298212343873,132.382403302096,132.462540887143,
132.540031362984,132.617443924814,132.694792732576,132.772091906516,132.849356943872,
132.926601905208,133.003851393021,133.041832180143),.UNSPECIFIED.);
#3345=B_SPLINE_CURVE_WITH_KNOTS('',3,(#195057,#195058,#195059,#195060,#195061,
#195062,#195063,#195064,#195065,#195066,#195067,#195068,#195069,#195070,
#195071,#195072,#195073,#195074,#195075,#195076,#195077,#195078,#195079,
#195080,#195081,#195082,#195083,#195084,#195085,#195086,#195087,#195088,
#195089,#195090,#195091,#195092,#195093,#195094,#195095,#195096,#195097,
#195098,#195099,#195100,#195101,#195102,#195103,#195104,#195105,#195106,
#195107,#195108,#195109,#195110,#195111,#195112,#195113,#195114,#195115,
#195116,#195117,#195118,#195119,#195120,#195121,#195122,#195123,#195124,
#195125,#195126,#195127,#195128,#195129,#195130,#195131,#195132,#195133,
#195134,#195135,#195136,#195137,#195138,#195139,#195140,#195141,#195142,
#195143,#195144,#195145,#195146,#195147,#195148,#195149,#195150,#195151,
#195152,#195153,#195154,#195155,#195156,#195157,#195158,#195159,#195160,
#195161,#195162,#195163,#195164,#195165,#195166,#195167,#195168,#195169,
#195170,#195171,#195172,#195173,#195174,#195175,#195176,#195177,#195178,
#195179,#195180,#195181,#195182,#195183,#195184,#195185,#195186,#195187,
#195188,#195189,#195190,#195191,#195192,#195193,#195194,#195195,#195196,
#195197,#195198,#195199,#195200,#195201,#195202,#195203,#195204,#195205,
#195206,#195207,#195208,#195209,#195210,#195211,#195212,#195213,#195214,
#195215,#195216,#195217,#195218,#195219,#195220,#195221,#195222,#195223,
#195224,#195225,#195226,#195227,#195228),.UNSPECIFIED.,.F.,.F.,(4,3,3,3,
3,3,3,3,3,3,3,3,3,3,3,3,3,3,3,3,3,3,3,3,3,3,3,3,3,3,3,3,3,3,3,3,3,3,3,3,
3,3,3,3,3,3,3,3,3,3,3,3,3,3,3,3,3,4),(135.088484104362,135.141075709124,
135.218731467319,135.296301033049,135.37379833968,135.451226978114,135.528615824241,
135.605978718418,135.640445577055,135.723940384101,135.807592061091,135.891482456332,
135.975486901716,136.059677859939,136.139815444986,136.217312791655,136.294728110007,
136.372077029675,136.449375132646,136.526637963971,136.603893977092,136.681149130653,
136.758417471996,136.835713053252,136.913096661236,136.990525869505,137.068075210615,
137.138555180849,137.214606628568,137.290563219462,137.366441740391,137.442258898088,
137.518031337845,137.595439285203,137.67118733354,137.746943395538,137.822722482114,
137.901365590763,137.977278503605,138.053248883594,138.129326377268,138.137294916711,
138.215830856766,138.294273986384,138.372638813933,138.450939792321,138.529191328772,
138.607410886313,138.685613807867,138.763813092361,138.842021734173,138.920285381034,
138.998577486712,139.076953299863,139.136034652573,139.215687266484,139.295257544978,
139.325441263557),.UNSPECIFIED.);
#3346=B_SPLINE_CURVE_WITH_KNOTS('',3,(#195229,#195230,#195231,#195232,#195233,
#195234,#195235,#195236,#195237,#195238,#195239,#195240,#195241,#195242,
#195243,#195244,#195245,#195246,#195247,#195248,#195249,#195250,#195251,
#195252,#195253,#195254,#195255,#195256,#195257,#195258,#195259,#195260,
#195261,#195262,#195263,#195264,#195265,#195266,#195267,#195268,#195269,
#195270,#195271,#195272,#195273,#195274,#195275,#195276,#195277,#195278,
#195279,#195280,#195281,#195282,#195283,#195284,#195285,#195286,#195287,
#195288,#195289,#195290,#195291,#195292,#195293,#195294,#195295,#195296,
#195297,#195298,#195299,#195300,#195301,#195302,#195303,#195304,#195305,
#195306,#195307,#195308,#195309,#195310),.UNSPECIFIED.,.F.,.F.,(4,3,3,3,
3,3,3,3,3,3,3,3,3,3,3,3,3,3,3,3,3,3,3,3,3,3,3,4),(133.041617861985,133.123183016486,
133.1435962374,133.228839535699,133.314004609853,133.399018977731,133.483926286527,
133.568640788799,133.642966105331,133.719509108317,133.79604665266,133.872593345428,
133.949195885716,134.025829631032,134.102547018878,134.142335973262,134.221219674072,
134.300040126623,134.378810938376,134.457545679513,134.536412982609,134.615128988621,
134.693851432986,134.772592595606,134.851565472774,134.930412978058,135.009448541169,
135.088484104279),.UNSPECIFIED.);
#3347=B_SPLINE_CURVE_WITH_KNOTS('',3,(#195312,#195313,#195314,#195315,#195316,
#195317,#195318,#195319,#195320,#195321,#195322,#195323,#195324,#195325,
#195326,#195327,#195328,#195329,#195330,#195331,#195332,#195333,#195334,
#195335,#195336,#195337,#195338,#195339,#195340,#195341,#195342,#195343,
#195344,#195345,#195346,#195347,#195348,#195349,#195350,#195351,#195352,
#195353,#195354,#195355,#195356,#195357,#195358,#195359,#195360,#195361,
#195362,#195363,#195364,#195365,#195366,#195367,#195368,#195369,#195370,
#195371,#195372,#195373,#195374,#195375,#195376,#195377,#195378,#195379,
#195380,#195381,#195382,#195383,#195384,#195385,#195386,#195387,#195388,
#195389,#195390,#195391,#195392,#195393,#195394,#195395,#195396),
 .UNSPECIFIED.,.F.,.F.,(4,3,3,3,3,3,3,3,3,3,3,3,3,3,3,3,3,3,3,3,3,3,3,3,
3,3,3,3,4),(133.041832180143,133.119112147236,133.196426261864,133.27383067654,
133.351286907555,133.42885258256,133.461280623006,133.537332070725,133.613288661619,
133.689167182548,133.764984340245,133.840756780002,133.91816472736,133.993912775696,
134.069668837694,134.14544792427,134.22409103292,134.300003945762,134.375974325751,
134.452051819425,134.460020358868,134.54038040468,134.620637838083,134.700802381432,
134.780883694742,134.860868989518,134.940796938601,135.020664980668,135.088484104362),
 .UNSPECIFIED.);
#3348=B_SPLINE_CURVE_WITH_KNOTS('',3,(#195397,#195398,#195399,#195400,#195401,
#195402,#195403,#195404,#195405,#195406,#195407,#195408,#195409,#195410,
#195411,#195412,#195413,#195414,#195415,#195416,#195417,#195418,#195419,
#195420,#195421,#195422,#195423,#195424,#195425,#195426,#195427,#195428,
#195429,#195430,#195431,#195432,#195433,#195434,#195435,#195436,#195437,
#195438,#195439,#195440,#195441,#195442,#195443,#195444,#195445,#195446,
#195447,#195448,#195449,#195450,#195451,#195452,#195453,#195454,#195455,
#195456,#195457,#195458,#195459,#195460,#195461,#195462,#195463,#195464,
#195465,#195466,#195467,#195468,#195469,#195470,#195471,#195472,#195473,
#195474,#195475,#195476,#195477,#195478,#195479,#195480,#195481,#195482,
#195483,#195484,#195485,#195486,#195487,#195488,#195489,#195490,#195491,
#195492,#195493,#195494,#195495,#195496,#195497,#195498,#195499,#195500,
#195501,#195502,#195503,#195504,#195505,#195506,#195507,#195508,#195509,
#195510,#195511,#195512,#195513,#195514,#195515,#195516,#195517,#195518,
#195519,#195520,#195521,#195522,#195523,#195524,#195525,#195526,#195527,
#195528,#195529,#195530,#195531,#195532,#195533,#195534,#195535,#195536,
#195537,#195538,#195539,#195540,#195541,#195542,#195543,#195544,#195545,
#195546,#195547,#195548,#195549,#195550,#195551,#195552,#195553,#195554,
#195555,#195556,#195557,#195558,#195559,#195560,#195561,#195562,#195563,
#195564,#195565),.UNSPECIFIED.,.F.,.F.,(4,3,3,3,3,3,3,3,3,3,3,3,3,3,3,3,
3,3,3,3,3,3,3,3,3,3,3,3,3,3,3,3,3,3,3,3,3,3,3,3,3,3,3,3,3,3,3,3,3,3,3,3,
3,3,3,3,4),(135.088484104466,135.173794025916,135.259420181161,135.345202545235,
135.431180372423,135.45876009473,135.538402001156,135.617973620898,135.697485849867,
135.776941183557,135.856362359615,135.935759021192,135.958129962661,136.039360059287,
136.120638950338,136.204854170401,136.286285023822,136.371892427207,136.457499830592,
136.542743128891,136.627908203046,136.712922570923,136.797829879719,136.882544381991,
136.956869698523,137.033412701509,137.109950245852,137.18649693862,137.263099478908,
137.339733224224,137.41645061207,137.456239566454,137.535786666534,137.615273497902,
137.694712325482,137.774115376729,137.853494850537,137.932875572756,138.01225897647,
138.091656144572,138.171078167568,138.250571600946,138.330103430334,138.409724158313,
138.454979302316,138.532635060511,138.610204626241,138.687701932873,138.765130571307,
138.842519417434,138.919882311612,138.954349170247,139.037805216196,139.121502012315,
139.205322739821,139.289322335834,139.324800290729),.UNSPECIFIED.);
#3349=B_SPLINE_CURVE_WITH_KNOTS('',3,(#195571,#195572,#195573,#195574,#195575,
#195576,#195577,#195578,#195579,#195580,#195581,#195582,#195583,#195584,
#195585,#195586,#195587,#195588,#195589,#195590,#195591,#195592,#195593,
#195594,#195595,#195596,#195597,#195598,#195599,#195600,#195601,#195602,
#195603,#195604,#195605,#195606,#195607,#195608,#195609,#195610,#195611,
#195612,#195613,#195614,#195615,#195616,#195617,#195618,#195619,#195620,
#195621,#195622,#195623,#195624,#195625,#195626,#195627,#195628,#195629,
#195630,#195631,#195632,#195633,#195634,#195635,#195636,#195637,#195638,
#195639,#195640,#195641,#195642,#195643,#195644,#195645,#195646,#195647,
#195648,#195649,#195650,#195651,#195652,#195653,#195654,#195655,#195656,
#195657,#195658,#195659,#195660,#195661,#195662,#195663,#195664,#195665,
#195666,#195667,#195668,#195669,#195670,#195671,#195672,#195673,#195674,
#195675,#195676,#195677,#195678,#195679,#195680,#195681,#195682,#195683,
#195684,#195685,#195686,#195687,#195688,#195689,#195690,#195691,#195692,
#195693,#195694,#195695,#195696,#195697,#195698,#195699,#195700,#195701,
#195702,#195703,#195704,#195705,#195706,#195707,#195708,#195709,#195710,
#195711,#195712,#195713,#195714,#195715,#195716,#195717,#195718,#195719,
#195720,#195721,#195722,#195723,#195724,#195725,#195726,#195727),
 .UNSPECIFIED.,.F.,.F.,(4,3,3,3,3,3,3,3,3,3,3,3,3,3,3,3,3,3,3,3,3,3,3,3,
3,3,3,3,3,3,3,3,3,3,3,3,3,3,3,3,3,3,3,3,3,3,3,3,3,3,3,3,4),(141.371669411542,
141.454131617628,141.536593475416,141.619054991757,141.701516173501,141.783977027497,
141.866437560596,141.948897779646,142.031357691497,142.113817302996,142.196276620993,
142.278735652335,142.36119440387,142.443652882447,142.526111094911,142.608569048111,
142.691026748894,142.773484204106,142.855941420593,142.941954008383,143.025278702804,
143.107745308362,143.190211069713,143.272676014271,143.355140169449,143.437603562656,
143.5200662213,143.602528172784,143.68498944451,143.767450063878,143.849910058285,
143.932369455127,144.014828281795,144.097286565681,144.179744334175,144.262201614663,
144.346335528112,144.42880152641,144.511265902959,144.593728767401,144.676190229358,
144.758650398432,144.841109384206,144.923567296249,145.00916441295,145.091629149893,
145.174090922191,145.256550168282,145.339007326461,145.42146984536,145.503927516643,
145.586386307552,145.608344229852),.UNSPECIFIED.);
#3350=B_SPLINE_CURVE_WITH_KNOTS('',3,(#195728,#195729,#195730,#195731,#195732,
#195733,#195734,#195735,#195736,#195737,#195738,#195739,#195740,#195741,
#195742,#195743,#195744,#195745,#195746,#195747,#195748,#195749,#195750,
#195751,#195752,#195753,#195754,#195755,#195756,#195757,#195758,#195759,
#195760,#195761,#195762,#195763,#195764,#195765,#195766,#195767,#195768,
#195769,#195770,#195771,#195772,#195773,#195774,#195775,#195776,#195777,
#195778,#195779,#195780,#195781,#195782,#195783,#195784,#195785,#195786,
#195787,#195788,#195789,#195790,#195791,#195792,#195793,#195794,#195795,
#195796,#195797,#195798,#195799,#195800,#195801,#195802,#195803,#195804,
#195805,#195806),.UNSPECIFIED.,.F.,.F.,(4,3,3,3,3,3,3,3,3,3,3,3,3,3,3,3,
3,3,3,3,3,3,3,3,3,3,4),(139.325441263557,139.404922780061,139.484363981108,
139.563776237547,139.635404520504,139.71663461713,139.797913508182,139.882128728245,
139.963559581665,140.04916698505,140.134774388435,140.220017686734,140.305182760888,
140.390197128765,140.475104437561,140.559818939832,140.634144256366,140.710687259352,
140.787224803695,140.863771496464,140.940374036752,141.017007782067,141.093725169914,
141.133514124297,141.240036454045,141.344973964139,141.371669411542),
 .UNSPECIFIED.);
#3351=B_SPLINE_CURVE_WITH_KNOTS('',3,(#195808,#195809,#195810,#195811,#195812,
#195813,#195814,#195815,#195816,#195817,#195818,#195819,#195820,#195821,
#195822,#195823,#195824,#195825,#195826,#195827,#195828,#195829,#195830,
#195831,#195832,#195833,#195834,#195835,#195836,#195837,#195838,#195839,
#195840,#195841,#195842,#195843,#195844,#195845,#195846,#195847,#195848,
#195849,#195850,#195851,#195852,#195853,#195854,#195855,#195856,#195857,
#195858,#195859,#195860,#195861,#195862,#195863,#195864,#195865,#195866,
#195867,#195868,#195869,#195870,#195871,#195872,#195873,#195874,#195875,
#195876,#195877,#195878,#195879,#195880,#195881,#195882,#195883,#195884,
#195885,#195886,#195887,#195888,#195889,#195890,#195891,#195892),
 .UNSPECIFIED.,.F.,.F.,(4,3,3,3,3,3,3,3,3,3,3,3,3,3,3,3,3,3,3,3,3,3,3,3,
3,3,3,3,4),(139.324800290729,139.409016625214,139.453719038179,139.531216384848,
139.6086317032,139.685980622868,139.763278725839,139.840541557164,139.917797570284,
139.995052723846,140.072321065189,140.149616646444,140.227000254428,140.304429462697,
140.381978803807,140.452458774041,140.527741820882,140.60293120538,140.678044107417,
140.753097598991,140.83041907555,140.905413675403,140.980403801278,141.055404759923,
141.130431870016,141.205537522519,141.280690322145,141.355940608412,141.371669411466),
 .UNSPECIFIED.);
#3352=B_SPLINE_CURVE_WITH_KNOTS('',3,(#195893,#195894,#195895,#195896,#195897,
#195898,#195899,#195900,#195901,#195902,#195903,#195904,#195905,#195906,
#195907,#195908,#195909,#195910,#195911,#195912,#195913,#195914,#195915,
#195916,#195917,#195918,#195919,#195920,#195921,#195922,#195923,#195924,
#195925,#195926,#195927,#195928,#195929,#195930,#195931,#195932,#195933,
#195934,#195935,#195936,#195937,#195938,#195939,#195940,#195941,#195942,
#195943,#195944,#195945,#195946,#195947,#195948,#195949,#195950,#195951,
#195952,#195953,#195954,#195955,#195956,#195957,#195958,#195959,#195960,
#195961,#195962,#195963,#195964,#195965,#195966,#195967,#195968,#195969,
#195970,#195971,#195972,#195973,#195974,#195975,#195976,#195977,#195978,
#195979,#195980,#195981,#195982,#195983,#195984,#195985,#195986,#195987,
#195988,#195989,#195990,#195991,#195992,#195993,#195994,#195995,#195996,
#195997,#195998,#195999,#196000,#196001,#196002,#196003,#196004,#196005,
#196006,#196007,#196008,#196009,#196010,#196011,#196012,#196013,#196014,
#196015,#196016,#196017,#196018,#196019,#196020,#196021,#196022,#196023,
#196024,#196025,#196026,#196027,#196028,#196029,#196030,#196031,#196032,
#196033,#196034,#196035,#196036,#196037,#196038,#196039,#196040,#196041,
#196042,#196043,#196044,#196045,#196046,#196047,#196048,#196049,#196050,
#196051,#196052,#196053,#196054,#196055,#196056,#196057,#196058),
 .UNSPECIFIED.,.F.,.F.,(4,3,3,3,3,3,3,3,3,3,3,3,3,3,3,3,3,3,3,3,3,3,3,3,
3,3,3,3,3,3,3,3,3,3,3,3,3,3,3,3,3,3,3,3,3,3,3,3,3,3,3,3,3,3,3,4),(141.371669411541,
141.451198509903,141.529734449958,141.608177579576,141.686542407125,141.764843385513,
141.843094921964,141.921314479505,141.999517401059,142.077716685554,142.155925327365,
142.234188974226,142.312481079904,142.390856893055,142.449938245765,142.529580152191,
142.609151771933,142.688664000902,142.768119334592,142.84754051065,142.926937172227,
142.949308113696,143.030538210322,143.111817101372,143.196032321436,143.277463174856,
143.363070578242,143.448677981627,143.533921279926,143.619086354082,143.70410072196,
143.789008030756,143.873722533028,143.948047849558,144.024590852544,144.101128396887,
144.177675089655,144.254277629943,144.330911375259,144.407628763105,144.44741771749,
144.526964817571,144.606451648938,144.685890476518,144.765293527766,144.844673001574,
144.924053723792,145.003437127507,145.082834295609,145.162256318606,145.241749751984,
145.321281581371,145.40090230935,145.446157453352,145.5276156997,145.609073946049),
 .UNSPECIFIED.);
#3353=B_SPLINE_CURVE_WITH_KNOTS('',3,(#196064,#196065,#196066,#196067,#196068,
#196069,#196070,#196071,#196072,#196073,#196074,#196075,#196076,#196077,
#196078,#196079,#196080,#196081,#196082,#196083,#196084,#196085,#196086,
#196087,#196088,#196089,#196090,#196091,#196092,#196093,#196094,#196095,
#196096,#196097,#196098,#196099,#196100,#196101,#196102,#196103,#196104,
#196105,#196106,#196107,#196108,#196109,#196110,#196111,#196112,#196113,
#196114,#196115,#196116,#196117,#196118,#196119,#196120,#196121,#196122,
#196123,#196124,#196125,#196126,#196127,#196128,#196129,#196130,#196131,
#196132,#196133,#196134,#196135,#196136,#196137,#196138,#196139,#196140,
#196141,#196142,#196143,#196144,#196145,#196146,#196147,#196148,#196149,
#196150,#196151,#196152,#196153,#196154,#196155,#196156,#196157,#196158,
#196159,#196160,#196161,#196162,#196163,#196164,#196165,#196166,#196167,
#196168,#196169,#196170,#196171,#196172,#196173,#196174,#196175,#196176,
#196177,#196178,#196179,#196180,#196181,#196182,#196183,#196184,#196185,
#196186,#196187,#196188,#196189,#196190,#196191,#196192,#196193,#196194,
#196195,#196196,#196197,#196198,#196199,#196200,#196201,#196202,#196203,
#196204,#196205,#196206,#196207,#196208,#196209,#196210,#196211,#196212,
#196213,#196214,#196215,#196216,#196217,#196218,#196219,#196220,#196221,
#196222,#196223,#196224,#196225,#196226,#196227,#196228,#196229),
 .UNSPECIFIED.,.F.,.F.,(4,3,3,3,3,3,3,3,3,3,3,3,3,3,3,3,3,3,3,3,3,3,3,3,
3,3,3,3,3,3,3,3,3,3,3,3,3,3,3,3,3,3,3,3,3,3,3,3,3,3,3,3,3,3,3,4),(147.655171343303,
147.73209130362,147.809015725201,147.887934862734,147.964942280489,148.044817277911,
148.124692275333,148.204239375413,148.283726206781,148.363165034361,148.442568085608,
148.521947559416,148.601328281635,148.68071168535,148.760108853452,148.839530876448,
148.919024309826,148.998556139214,149.078176867193,149.123432011195,149.20108776939,
149.27865733512,149.356154641751,149.433583280185,149.510972126311,149.588335020489,
149.622801879126,149.706296686172,149.789948363162,149.873838758403,149.957843203787,
150.042034162009,150.122171747057,150.199669093726,150.277084412078,150.354433331746,
150.431731434717,150.508994266042,150.586250279162,150.663505432724,150.740773774066,
150.818069355322,150.895452963306,150.972882171574,151.050431512685,151.120911482919,
151.196977001861,151.272944877175,151.350133540636,151.425945761604,151.501716956229,
151.577462159768,151.655710166041,151.73146722759,151.810960706224,151.890454184858),
 .UNSPECIFIED.);
#3354=B_SPLINE_CURVE_WITH_KNOTS('',3,(#196230,#196231,#196232,#196233,#196234,
#196235,#196236,#196237,#196238,#196239,#196240,#196241,#196242,#196243,
#196244,#196245,#196246,#196247,#196248,#196249,#196250,#196251,#196252,
#196253,#196254,#196255,#196256,#196257,#196258,#196259,#196260,#196261,
#196262,#196263,#196264,#196265,#196266,#196267,#196268,#196269,#196270,
#196271,#196272,#196273,#196274,#196275,#196276,#196277,#196278,#196279,
#196280,#196281,#196282,#196283,#196284,#196285,#196286,#196287,#196288,
#196289,#196290,#196291,#196292,#196293,#196294,#196295,#196296,#196297,
#196298,#196299,#196300,#196301,#196302,#196303,#196304,#196305),
 .UNSPECIFIED.,.F.,.F.,(4,3,3,3,3,3,3,3,3,3,3,3,3,3,3,3,3,3,3,3,3,3,3,3,
3,4),(145.608344229852,145.69080583361,145.77326677149,145.855727070888,
145.938186759201,146.020645863823,146.103104412146,146.18556243156,146.268019949453,
146.354697122532,146.437163908141,146.519629021272,146.602092571579,146.684554668693,
146.767015422225,146.849474941767,146.931933336894,147.014390717165,147.096857102985,
147.179320304609,147.261780760557,147.344238909193,147.426704513205,147.509164391782,
147.591628503519,147.654854718721),.UNSPECIFIED.);
#3355=B_SPLINE_CURVE_WITH_KNOTS('',3,(#196307,#196308,#196309,#196310,#196311,
#196312,#196313,#196314,#196315,#196316,#196317,#196318,#196319,#196320,
#196321,#196322,#196323,#196324,#196325,#196326,#196327,#196328,#196329,
#196330,#196331,#196332,#196333,#196334,#196335,#196336,#196337,#196338,
#196339,#196340,#196341,#196342,#196343,#196344,#196345,#196346,#196347,
#196348,#196349,#196350,#196351,#196352,#196353,#196354,#196355,#196356,
#196357,#196358,#196359,#196360,#196361,#196362,#196363,#196364,#196365,
#196366,#196367,#196368,#196369,#196370,#196371,#196372,#196373,#196374,
#196375,#196376,#196377,#196378,#196379,#196380,#196381,#196382,#196383,
#196384,#196385),.UNSPECIFIED.,.F.,.F.,(4,3,3,3,3,3,3,3,3,3,3,3,3,3,3,3,
3,3,3,3,3,3,3,3,3,3,4),(145.609073946049,145.68656484209,145.763988977529,
145.841374551929,145.918735111077,145.945527321283,146.029022128329,146.112673805319,
146.19656420056,146.280568645943,146.364759604166,146.444897189214,146.522394535883,
146.599809854235,146.677158773903,146.754456876874,146.831719708198,146.908975721319,
146.986230874881,147.063499216223,147.140794797479,147.218178405462,147.295607613731,
147.373156954842,147.443636925076,147.549245821898,147.654854718721),
 .UNSPECIFIED.);
#3356=B_SPLINE_CURVE_WITH_KNOTS('',3,(#196386,#196387,#196388,#196389,#196390,
#196391,#196392,#196393,#196394,#196395,#196396,#196397,#196398,#196399,
#196400,#196401,#196402,#196403,#196404,#196405,#196406,#196407,#196408,
#196409,#196410,#196411,#196412,#196413,#196414,#196415,#196416,#196417,
#196418,#196419,#196420,#196421,#196422,#196423,#196424,#196425,#196426,
#196427,#196428,#196429,#196430,#196431,#196432,#196433,#196434,#196435,
#196436,#196437,#196438,#196439,#196440,#196441,#196442,#196443,#196444,
#196445,#196446,#196447,#196448,#196449,#196450,#196451,#196452,#196453,
#196454,#196455,#196456,#196457,#196458,#196459,#196460,#196461,#196462,
#196463,#196464,#196465,#196466,#196467,#196468,#196469,#196470,#196471,
#196472,#196473,#196474,#196475,#196476,#196477,#196478,#196479,#196480,
#196481,#196482,#196483,#196484,#196485,#196486,#196487,#196488,#196489,
#196490,#196491,#196492,#196493,#196494,#196495,#196496,#196497,#196498,
#196499,#196500,#196501,#196502,#196503,#196504,#196505,#196506,#196507,
#196508,#196509,#196510,#196511,#196512,#196513,#196514,#196515,#196516,
#196517,#196518,#196519,#196520,#196521,#196522,#196523,#196524,#196525,
#196526,#196527,#196528,#196529,#196530,#196531,#196532,#196533,#196534,
#196535,#196536,#196537,#196538,#196539,#196540,#196541,#196542,#196543,
#196544,#196545,#196546,#196547,#196548,#196549,#196550,#196551,#196552,
#196553,#196554),.UNSPECIFIED.,.F.,.F.,(4,3,3,3,3,3,3,3,3,3,3,3,3,3,3,3,
3,3,3,3,3,3,3,3,3,3,3,3,3,3,3,3,3,3,3,3,3,3,3,3,3,3,3,3,3,3,3,3,3,3,3,3,
3,3,3,3,4),(147.654854718845,147.729591060665,147.804268784978,147.878905015242,
147.953528146011,148.028147561493,148.102778681513,148.177436942878,148.252181161896,
148.326973368477,148.401877963143,148.442376660938,148.520912600993,148.599355730611,
148.67772055816,148.756021536547,148.834273072998,148.912492630539,148.990695552093,
149.068894836588,149.147103478399,149.225367125261,149.303659230938,149.38203504409,
149.4411163968,149.520758303226,149.600329922968,149.679842151936,149.759297485627,
149.838718661684,149.918115323261,149.940486264732,150.021716361358,150.102995252409,
150.187210472473,150.268641325893,150.354248729278,150.439856132663,150.525099430962,
150.610264505116,150.695278872994,150.78018618179,150.864900684061,150.939226000594,
151.01576900358,151.092306547923,151.168853240691,151.245455780979,151.322089526295,
151.398806914141,151.438595868525,151.518145880864,151.597636918564,151.677073113388,
151.756475815793,151.835859086637,151.891383072134),.UNSPECIFIED.);
#3357=B_SPLINE_CURVE_WITH_KNOTS('',3,(#196560,#196561,#196562,#196563,#196564,
#196565,#196566,#196567,#196568,#196569,#196570,#196571,#196572,#196573,
#196574,#196575,#196576,#196577,#196578,#196579,#196580,#196581,#196582,
#196583,#196584,#196585,#196586,#196587,#196588,#196589,#196590,#196591,
#196592,#196593,#196594,#196595,#196596,#196597,#196598,#196599,#196600,
#196601,#196602,#196603,#196604,#196605,#196606,#196607,#196608,#196609,
#196610,#196611,#196612,#196613,#196614,#196615,#196616,#196617,#196618,
#196619,#196620,#196621,#196622,#196623,#196624,#196625,#196626,#196627,
#196628,#196629,#196630,#196631,#196632,#196633,#196634,#196635,#196636,
#196637,#196638,#196639,#196640,#196641,#196642,#196643,#196644,#196645,
#196646,#196647,#196648,#196649,#196650,#196651,#196652,#196653,#196654,
#196655,#196656,#196657,#196658,#196659,#196660,#196661,#196662,#196663,
#196664,#196665,#196666,#196667,#196668,#196669,#196670,#196671,#196672,
#196673,#196674,#196675,#196676,#196677,#196678,#196679,#196680,#196681,
#196682,#196683,#196684,#196685,#196686,#196687,#196688,#196689,#196690,
#196691,#196692,#196693,#196694,#196695,#196696,#196697,#196698,#196699,
#196700,#196701,#196702,#196703,#196704,#196705,#196706,#196707,#196708,
#196709,#196710,#196711,#196712,#196713,#196714,#196715,#196716,#196717,
#196718,#196719,#196720,#196721,#196722,#196723,#196724,#196725),
 .UNSPECIFIED.,.F.,.F.,(4,3,3,3,3,3,3,3,3,3,3,3,3,3,3,3,3,3,3,3,3,3,3,3,
3,3,3,3,3,3,3,3,3,3,3,3,3,3,3,3,3,3,3,3,3,3,3,3,3,3,3,3,3,3,3,4),(153.938040025994,
154.027615078815,154.117130690506,154.202373988805,154.28753906296,154.372553430837,
154.457460739633,154.542175241905,154.616500558437,154.693043561423,154.769581105765,
154.846127798534,154.922730338822,154.999364084138,155.076081471984,155.115870426368,
155.195417526448,155.274904357816,155.354343185396,155.433746236643,155.513125710451,
155.59250643267,155.671889836384,155.751287004487,155.830709027483,155.910202460861,
155.989734290248,156.069355018227,156.11461016223,156.192265920425,156.269835486155,
156.347332792786,156.42476143122,156.502150277347,156.579513171524,156.613980030161,
156.697474837207,156.781126514197,156.865016909438,156.949021354822,157.033212313045,
157.113349898092,157.190847244761,157.268262563113,157.345611482781,157.422909585752,
157.500172417077,157.577428430198,157.654683583759,157.731951925102,157.809247506357,
157.886631114341,157.96406032261,158.041609663721,158.112089633955,158.17544691121),
 .UNSPECIFIED.);
#3358=B_SPLINE_CURVE_WITH_KNOTS('',3,(#196726,#196727,#196728,#196729,#196730,
#196731,#196732,#196733,#196734,#196735,#196736,#196737,#196738,#196739,
#196740,#196741,#196742,#196743,#196744,#196745,#196746,#196747,#196748,
#196749,#196750,#196751,#196752,#196753,#196754,#196755,#196756,#196757,
#196758,#196759,#196760,#196761,#196762,#196763,#196764,#196765,#196766,
#196767,#196768,#196769,#196770,#196771,#196772,#196773,#196774,#196775,
#196776,#196777,#196778,#196779,#196780,#196781,#196782,#196783,#196784,
#196785,#196786,#196787,#196788,#196789,#196790,#196791,#196792,#196793,
#196794,#196795,#196796,#196797,#196798,#196799,#196800,#196801,#196802,
#196803,#196804,#196805,#196806,#196807),.UNSPECIFIED.,.F.,.F.,(4,3,3,3,
3,3,3,3,3,3,3,3,3,3,3,3,3,3,3,3,3,3,3,3,3,3,3,4),(151.890454184858,151.966371647742,
152.043011433262,152.119651218781,152.198187158836,152.276630288454,152.354995116003,
152.433296094391,152.511547630842,152.589767188383,152.667970109937,152.746169394432,
152.824378036243,152.902641683104,152.980933788782,153.059309601933,153.118390954644,
153.198032861071,153.277604480813,153.357116709783,153.436572043473,153.515993219531,
153.595389881108,153.617760822575,153.697830623407,153.777060453003,153.857550239452,
153.938040025901),.UNSPECIFIED.);
#3359=B_SPLINE_CURVE_WITH_KNOTS('',3,(#196809,#196810,#196811,#196812,#196813,
#196814,#196815,#196816,#196817,#196818,#196819,#196820,#196821,#196822,
#196823,#196824,#196825,#196826,#196827,#196828,#196829,#196830,#196831,
#196832,#196833,#196834,#196835,#196836,#196837,#196838,#196839,#196840,
#196841,#196842,#196843,#196844,#196845,#196846,#196847,#196848,#196849,
#196850,#196851,#196852,#196853,#196854,#196855,#196856,#196857,#196858,
#196859,#196860,#196861,#196862,#196863,#196864,#196865,#196866,#196867,
#196868,#196869,#196870,#196871,#196872,#196873,#196874,#196875,#196876,
#196877,#196878,#196879,#196880,#196881,#196882,#196883,#196884,#196885,
#196886,#196887,#196888,#196889,#196890),.UNSPECIFIED.,.F.,.F.,(4,3,3,3,
3,3,3,3,3,3,3,3,3,3,3,3,3,3,3,3,3,3,3,3,3,3,3,4),(151.891383072134,151.97076450571,
152.05015637347,152.129569762885,152.209053657481,152.288572885094,152.368186515532,
152.437335604387,152.514991362581,152.592560928312,152.670058234943,152.747486873377,
152.824875719503,152.902238613681,152.936705472318,153.020200279363,153.103851956354,
153.187742351595,153.271746796978,153.355937755201,153.436075340249,153.515525194001,
153.594871057291,153.674124288318,153.753272553693,153.832358942751,153.911381727581,
153.938040025901),.UNSPECIFIED.);
#3360=B_SPLINE_CURVE_WITH_KNOTS('',3,(#196891,#196892,#196893,#196894,#196895,
#196896,#196897,#196898,#196899,#196900,#196901,#196902,#196903,#196904,
#196905,#196906,#196907,#196908,#196909,#196910,#196911,#196912,#196913,
#196914,#196915,#196916,#196917,#196918,#196919,#196920,#196921,#196922,
#196923,#196924,#196925,#196926,#196927,#196928,#196929,#196930,#196931,
#196932,#196933,#196934,#196935,#196936,#196937,#196938,#196939,#196940,
#196941,#196942,#196943,#196944,#196945,#196946,#196947,#196948,#196949,
#196950,#196951,#196952,#196953,#196954,#196955,#196956,#196957,#196958,
#196959,#196960,#196961,#196962,#196963,#196964,#196965,#196966,#196967,
#196968,#196969,#196970,#196971,#196972,#196973,#196974,#196975,#196976,
#196977,#196978,#196979,#196980,#196981,#196982,#196983,#196984,#196985,
#196986,#196987,#196988,#196989,#196990,#196991,#196992,#196993,#196994,
#196995,#196996,#196997,#196998,#196999,#197000,#197001,#197002,#197003,
#197004,#197005,#197006,#197007,#197008,#197009,#197010,#197011,#197012,
#197013,#197014,#197015,#197016,#197017,#197018,#197019,#197020,#197021,
#197022,#197023,#197024,#197025,#197026,#197027,#197028,#197029,#197030,
#197031,#197032,#197033,#197034,#197035,#197036,#197037,#197038,#197039,
#197040,#197041,#197042,#197043,#197044,#197045,#197046,#197047,#197048,
#197049,#197050,#197051,#197052,#197053,#197054,#197055,#197056,#197057,
#197058,#197059),.UNSPECIFIED.,.F.,.F.,(4,3,3,3,3,3,3,3,3,3,3,3,3,3,3,3,
3,3,3,3,3,3,3,3,3,3,3,3,3,3,3,3,3,3,3,3,3,3,3,3,3,3,3,3,3,3,3,3,3,3,3,3,
3,3,3,3,4),(153.938040026018,154.021006808716,154.104150032445,154.187570243097,
154.271128008187,154.354917908727,154.434815076111,154.51086652383,154.586823114724,
154.662701635653,154.73851879335,154.814291233106,154.891699180465,154.967447228801,
155.043203290799,155.118982377375,155.197625486025,155.273538398867,155.349508778856,
155.42558627253,155.433554811974,155.512090752029,155.590533881648,155.668898709196,
155.747199687584,155.825451224035,155.903670781576,155.98187370313,156.060072987625,
156.138281629436,156.216545276298,156.294837381975,156.373213195127,156.432294547836,
156.511936454262,156.591508074004,156.671020302973,156.750475636663,156.82989681272,
156.909293474297,156.931664415767,157.012894512393,157.094173403444,157.178388623507,
157.259819476928,157.345426880313,157.431034283698,157.516277581997,157.601442656152,
157.686457024029,157.771364332825,157.856078835097,157.930404151629,158.006946635292,
158.083479310245,158.16002739832,158.174370687208),.UNSPECIFIED.);
#3361=B_SPLINE_CURVE_WITH_KNOTS('',3,(#197065,#197066,#197067,#197068,#197069,
#197070,#197071,#197072,#197073,#197074,#197075,#197076,#197077,#197078,
#197079,#197080,#197081,#197082,#197083,#197084,#197085,#197086,#197087,
#197088,#197089,#197090,#197091,#197092,#197093,#197094,#197095,#197096,
#197097,#197098,#197099,#197100,#197101,#197102,#197103,#197104,#197105,
#197106,#197107,#197108,#197109,#197110,#197111,#197112,#197113,#197114,
#197115,#197116,#197117,#197118,#197119,#197120,#197121,#197122,#197123,
#197124,#197125,#197126,#197127,#197128,#197129,#197130,#197131,#197132,
#197133,#197134,#197135,#197136,#197137,#197138,#197139,#197140,#197141,
#197142,#197143,#197144,#197145,#197146,#197147,#197148,#197149,#197150,
#197151,#197152,#197153,#197154,#197155,#197156,#197157,#197158,#197159,
#197160,#197161,#197162,#197163,#197164,#197165,#197166,#197167,#197168,
#197169,#197170,#197171,#197172,#197173,#197174,#197175,#197176,#197177,
#197178,#197179,#197180,#197181,#197182,#197183,#197184,#197185,#197186,
#197187,#197188,#197189,#197190,#197191,#197192,#197193,#197194,#197195,
#197196,#197197,#197198,#197199,#197200,#197201,#197202,#197203,#197204,
#197205,#197206,#197207,#197208,#197209,#197210,#197211,#197212,#197213,
#197214,#197215,#197216,#197217,#197218,#197219,#197220,#197221,#197222,
#197223,#197224,#197225,#197226,#197227,#197228,#197229,#197230),
 .UNSPECIFIED.,.F.,.F.,(4,3,3,3,3,3,3,3,3,3,3,3,3,3,3,3,3,3,3,3,3,3,3,3,
3,3,3,3,3,3,3,3,3,3,3,3,3,3,3,3,3,3,3,3,3,3,3,3,3,3,3,3,3,3,3,4),(160.221225333176,
160.298250388259,160.375922534597,160.452848578413,160.530893776012,160.60893897361,
160.690169070236,160.771447961287,160.85566318135,160.937094034771,161.022701438156,
161.108308841541,161.19355213984,161.278717213994,161.363731581872,161.448638890667,
161.533353392939,161.607678709472,161.684221712458,161.7607592568,161.837305949568,
161.913908489857,161.990542235172,162.067259623018,162.107048577403,162.186595677484,
162.266082508851,162.345521336431,162.424924387679,162.504303861487,162.583684583706,
162.66306798742,162.742465155522,162.821887178519,162.901380611897,162.980912441285,
163.060533169264,163.105788313265,163.18344407146,163.26101363719,163.338510943822,
163.415939582256,163.493328428382,163.57069132256,163.605158181197,163.688652988243,
163.772304665233,163.856195060474,163.940199505858,164.024390464081,164.104528049128,
164.182040570407,164.259450079704,164.33680020683,164.414096438049,164.458358196858),
 .UNSPECIFIED.);
#3362=B_SPLINE_CURVE_WITH_KNOTS('',3,(#197231,#197232,#197233,#197234,#197235,
#197236,#197237,#197238,#197239,#197240,#197241,#197242,#197243,#197244,
#197245,#197246,#197247,#197248,#197249,#197250,#197251,#197252,#197253,
#197254,#197255,#197256,#197257,#197258,#197259,#197260,#197261,#197262,
#197263,#197264,#197265,#197266,#197267,#197268,#197269,#197270,#197271,
#197272,#197273,#197274,#197275,#197276,#197277,#197278,#197279,#197280,
#197281,#197282,#197283,#197284,#197285,#197286,#197287,#197288,#197289,
#197290,#197291,#197292,#197293,#197294,#197295,#197296,#197297,#197298,
#197299,#197300,#197301,#197302,#197303,#197304,#197305,#197306,#197307,
#197308,#197309,#197310,#197311,#197312,#197313,#197314,#197315),
 .UNSPECIFIED.,.F.,.F.,(4,3,3,3,3,3,3,3,3,3,3,3,3,3,3,3,3,3,3,3,3,3,3,3,
3,3,3,3,4),(158.17544691121,158.251418173854,158.3273085691,158.403134815705,
158.478913568005,158.557903043232,158.633651177154,158.709405131614,158.785179916075,
158.860990554791,158.936894403711,159.012853234892,159.088923024484,159.110829369817,
159.189365309872,159.26780843949,159.346173267039,159.424474245426,159.502725781877,
159.580945339418,159.659148260972,159.737347545467,159.815556187278,159.893819834139,
159.972111939817,160.050487752968,160.109569105679,160.211051659851,160.22122533308),
 .UNSPECIFIED.);
#3363=B_SPLINE_CURVE_WITH_KNOTS('',3,(#197317,#197318,#197319,#197320,#197321,
#197322,#197323,#197324,#197325,#197326,#197327,#197328,#197329,#197330,
#197331,#197332,#197333,#197334,#197335,#197336,#197337,#197338,#197339,
#197340,#197341,#197342,#197343,#197344,#197345,#197346,#197347,#197348,
#197349,#197350,#197351,#197352,#197353,#197354,#197355,#197356,#197357,
#197358,#197359,#197360,#197361,#197362,#197363,#197364,#197365,#197366,
#197367,#197368,#197369,#197370,#197371,#197372,#197373,#197374,#197375,
#197376,#197377,#197378,#197379,#197380,#197381,#197382,#197383,#197384,
#197385,#197386,#197387,#197388,#197389,#197390,#197391,#197392,#197393,
#197394,#197395,#197396,#197397,#197398,#197399,#197400,#197401),
 .UNSPECIFIED.,.F.,.F.,(4,3,3,3,3,3,3,3,3,3,3,3,3,3,3,3,3,3,3,3,3,3,3,3,
3,3,3,3,4),(158.174370687208,158.250978071601,158.327619117061,158.404341050154,
158.42977401956,158.50932111964,158.588807951008,158.668246778588,158.747649829835,
158.827029303643,158.906410025862,158.985793429576,159.065190597678,159.144612620674,
159.224106054052,159.30363788344,159.383258611419,159.428513755422,159.506169513617,
159.583739079347,159.661236385978,159.738665024412,159.816053870539,159.893416764717,
159.927883623353,160.005717791887,160.083593193719,160.161573552186,160.221225332989),
 .UNSPECIFIED.);
#3364=B_SPLINE_CURVE_WITH_KNOTS('',3,(#197402,#197403,#197404,#197405,#197406,
#197407,#197408,#197409,#197410,#197411,#197412,#197413,#197414,#197415,
#197416,#197417,#197418,#197419,#197420,#197421,#197422,#197423,#197424,
#197425,#197426,#197427,#197428,#197429,#197430,#197431,#197432,#197433,
#197434,#197435,#197436,#197437,#197438,#197439,#197440,#197441,#197442,
#197443,#197444,#197445,#197446,#197447,#197448,#197449,#197450,#197451,
#197452,#197453,#197454,#197455,#197456,#197457,#197458,#197459,#197460,
#197461,#197462,#197463,#197464,#197465,#197466,#197467,#197468,#197469,
#197470,#197471,#197472,#197473,#197474,#197475,#197476,#197477,#197478,
#197479,#197480,#197481,#197482,#197483,#197484,#197485,#197486,#197487,
#197488,#197489,#197490,#197491,#197492,#197493,#197494,#197495,#197496,
#197497,#197498,#197499,#197500,#197501,#197502,#197503,#197504,#197505,
#197506,#197507,#197508,#197509,#197510,#197511,#197512,#197513,#197514,
#197515,#197516,#197517,#197518,#197519,#197520,#197521,#197522,#197523,
#197524,#197525,#197526,#197527,#197528,#197529,#197530,#197531,#197532,
#197533,#197534,#197535,#197536,#197537,#197538,#197539,#197540,#197541,
#197542,#197543,#197544,#197545,#197546,#197547,#197548,#197549,#197550,
#197551,#197552,#197553,#197554,#197555,#197556,#197557,#197558,#197559,
#197560,#197561,#197562,#197563,#197564,#197565,#197566,#197567,#197568,
#197569,#197570),.UNSPECIFIED.,.F.,.F.,(4,3,3,3,3,3,3,3,3,3,3,3,3,3,3,3,
3,3,3,3,3,3,3,3,3,3,3,3,3,3,3,3,3,3,3,3,3,3,3,3,3,3,3,3,3,3,3,3,3,3,3,3,
3,3,3,3,4),(160.22122533308,160.326650068649,160.427253491284,160.504750837953,
160.582166156305,160.659515075973,160.736813178944,160.814076010268,160.891332023389,
160.968587176951,161.045855518293,161.123151099549,161.200534707533,161.277963915802,
161.355513256912,161.425993227147,161.502044674866,161.57800126576,161.653879786689,
161.729696944386,161.805469384142,161.882877331501,161.958625379837,162.034381441835,
162.110160528411,162.188803637061,162.264716549903,162.340686929892,162.416764423566,
162.424732963009,162.503268903064,162.581712032682,162.660076860231,162.738377838619,
162.816629375069,162.89484893261,162.973051854164,163.051251138659,163.12945978047,
163.207723427332,163.286015533009,163.36439134616,163.423472698871,163.503114605297,
163.582686225039,163.662198454008,163.741653787698,163.821074963756,163.900471625333,
163.922842566802,164.004072663428,164.085351554479,164.169566774542,164.250997627963,
164.336605031348,164.422212434733,164.457960367931),.UNSPECIFIED.);
#3365=B_SPLINE_CURVE_WITH_KNOTS('',3,(#197576,#197577,#197578,#197579,#197580,
#197581,#197582,#197583,#197584,#197585,#197586,#197587,#197588,#197589,
#197590,#197591,#197592,#197593,#197594,#197595,#197596,#197597,#197598,
#197599,#197600,#197601,#197602,#197603,#197604,#197605,#197606,#197607,
#197608,#197609,#197610,#197611,#197612,#197613,#197614,#197615,#197616,
#197617,#197618,#197619,#197620,#197621,#197622,#197623,#197624,#197625,
#197626,#197627,#197628,#197629,#197630,#197631,#197632,#197633,#197634,
#197635,#197636,#197637,#197638,#197639,#197640,#197641,#197642,#197643,
#197644,#197645,#197646,#197647,#197648,#197649,#197650,#197651,#197652,
#197653,#197654,#197655,#197656,#197657,#197658,#197659,#197660,#197661,
#197662,#197663,#197664,#197665,#197666,#197667,#197668,#197669,#197670,
#197671,#197672,#197673,#197674,#197675,#197676,#197677,#197678,#197679,
#197680,#197681,#197682,#197683,#197684,#197685,#197686,#197687,#197688,
#197689,#197690,#197691,#197692,#197693,#197694,#197695,#197696,#197697,
#197698,#197699,#197700,#197701,#197702,#197703,#197704,#197705,#197706,
#197707,#197708,#197709,#197710,#197711,#197712,#197713,#197714,#197715,
#197716,#197717,#197718,#197719,#197720,#197721,#197722,#197723,#197724,
#197725,#197726,#197727,#197728,#197729,#197730,#197731,#197732),
 .UNSPECIFIED.,.F.,.F.,(4,3,3,3,3,3,3,3,3,3,3,3,3,3,3,3,3,3,3,3,3,3,3,3,
3,3,3,3,3,3,3,3,3,3,3,3,3,3,3,3,3,3,3,3,3,3,3,3,3,3,3,3,4),(166.50441064026,
166.586872846346,166.669334704134,166.751796220475,166.834257402219,166.916718256215,
166.999178789314,167.081639008364,167.164098920215,167.246558531714,167.329017849711,
167.411476881053,167.493935632588,167.576394111165,167.658852323629,167.74131027683,
167.823767977612,167.906225432824,167.988682649311,168.074695237101,168.158019931522,
168.24048653708,168.322952298431,168.405417242989,168.487881398167,168.570344791374,
168.652807450018,168.735269401502,168.817730673228,168.900191292596,168.982651287003,
169.065110683845,169.147569510513,169.2300277944,169.312485562893,169.394942843381,
169.47907675683,169.561542755128,169.644007131677,169.726469996119,169.808931458076,
169.89139162715,169.973850612924,170.056308524967,170.141905641668,170.224370378611,
170.30683215091,170.389291397001,170.471748555179,170.554211074078,170.636668745362,
170.71912753627,170.74108545857),.UNSPECIFIED.);
#3366=B_SPLINE_CURVE_WITH_KNOTS('',3,(#197733,#197734,#197735,#197736,#197737,
#197738,#197739,#197740,#197741,#197742,#197743,#197744,#197745,#197746,
#197747,#197748,#197749,#197750,#197751,#197752,#197753,#197754,#197755,
#197756,#197757,#197758,#197759,#197760,#197761,#197762,#197763,#197764,
#197765,#197766,#197767,#197768,#197769,#197770,#197771,#197772,#197773,
#197774,#197775,#197776,#197777,#197778,#197779,#197780,#197781,#197782,
#197783,#197784,#197785,#197786,#197787,#197788,#197789,#197790,#197791,
#197792,#197793,#197794,#197795,#197796,#197797,#197798,#197799,#197800,
#197801,#197802,#197803,#197804,#197805,#197806,#197807,#197808,#197809,
#197810,#197811,#197812,#197813,#197814,#197815,#197816,#197817),
 .UNSPECIFIED.,.F.,.F.,(4,3,3,3,3,3,3,3,3,3,3,3,3,3,3,3,3,3,3,3,3,3,3,3,
3,3,3,3,4),(164.458358196858,164.538971895374,164.616225717916,164.69348733951,
164.770770809529,164.84809018696,164.925500388357,165.002963990101,165.080534426416,
165.10326778499,165.179319232709,165.255275823603,165.331154344532,165.406971502229,
165.482743941986,165.560151889344,165.63589993768,165.711655999678,165.787435086255,
165.866078194904,165.941991107746,166.017961487735,166.094038981409,166.102007520852,
166.192747188222,166.283004388607,166.372894866779,166.462116729469,166.50441064026),
 .UNSPECIFIED.);
#3367=B_SPLINE_CURVE_WITH_KNOTS('',3,(#197819,#197820,#197821,#197822,#197823,
#197824,#197825,#197826,#197827,#197828,#197829,#197830,#197831,#197832,
#197833,#197834,#197835,#197836,#197837,#197838,#197839,#197840,#197841,
#197842,#197843,#197844,#197845,#197846,#197847,#197848,#197849,#197850,
#197851,#197852,#197853,#197854,#197855,#197856,#197857,#197858,#197859,
#197860,#197861,#197862,#197863,#197864,#197865,#197866,#197867,#197868,
#197869,#197870,#197871,#197872,#197873,#197874,#197875,#197876,#197877,
#197878,#197879,#197880,#197881,#197882,#197883,#197884,#197885,#197886,
#197887,#197888,#197889,#197890,#197891,#197892,#197893,#197894,#197895,
#197896,#197897,#197898,#197899,#197900),.UNSPECIFIED.,.F.,.F.,(4,3,3,3,
3,3,3,3,3,3,3,3,3,3,3,3,3,3,3,3,3,3,3,3,3,3,3,4),(164.457960367931,164.543173052602,
164.628300019108,164.713270916212,164.798129799875,164.882804581115,164.921582302664,
164.99812530565,165.074662849993,165.151209542761,165.227812083049,165.304445828365,
165.381163216212,165.420952170595,165.500499270676,165.579986102043,165.659424929623,
165.73882798087,165.818207454679,165.897588176897,165.976971580612,166.056368748714,
166.13579077171,166.215284205088,166.294816034476,166.374436762455,166.419691906458,
166.50441064026),.UNSPECIFIED.);
#3368=B_SPLINE_CURVE_WITH_KNOTS('',3,(#197901,#197902,#197903,#197904,#197905,
#197906,#197907,#197908,#197909,#197910,#197911,#197912,#197913,#197914,
#197915,#197916,#197917,#197918,#197919,#197920,#197921,#197922,#197923,
#197924,#197925,#197926,#197927,#197928,#197929,#197930,#197931,#197932,
#197933,#197934,#197935,#197936,#197937,#197938,#197939,#197940,#197941,
#197942,#197943,#197944,#197945,#197946,#197947,#197948,#197949,#197950,
#197951,#197952,#197953,#197954,#197955,#197956,#197957,#197958,#197959,
#197960,#197961,#197962,#197963,#197964,#197965,#197966,#197967,#197968,
#197969,#197970,#197971,#197972,#197973,#197974,#197975,#197976,#197977,
#197978,#197979,#197980,#197981,#197982,#197983,#197984,#197985,#197986,
#197987,#197988,#197989,#197990,#197991,#197992,#197993,#197994,#197995,
#197996,#197997,#197998,#197999,#198000,#198001,#198002,#198003,#198004,
#198005,#198006,#198007,#198008,#198009,#198010,#198011,#198012,#198013,
#198014,#198015,#198016,#198017,#198018,#198019,#198020,#198021,#198022,
#198023,#198024,#198025,#198026,#198027,#198028,#198029,#198030,#198031,
#198032,#198033,#198034,#198035,#198036,#198037,#198038,#198039,#198040,
#198041,#198042,#198043,#198044,#198045,#198046,#198047,#198048,#198049,
#198050,#198051,#198052,#198053,#198054,#198055,#198056,#198057,#198058,
#198059,#198060,#198061,#198062,#198063,#198064,#198065,#198066,#198067,
#198068,#198069),.UNSPECIFIED.,.F.,.F.,(4,3,3,3,3,3,3,3,3,3,3,3,3,3,3,3,
3,3,3,3,3,3,3,3,3,3,3,3,3,3,3,3,3,3,3,3,3,3,3,3,3,3,3,3,3,3,3,3,3,3,3,3,
3,3,3,3,4),(166.504410640392,166.579684414951,166.654890959035,166.730040860453,
166.805157710638,166.880263168721,166.919061774389,167.002556581435,167.086208258425,
167.170098653666,167.25410309905,167.338294057273,167.41843164232,167.495928988989,
167.573344307341,167.650693227009,167.727991329979,167.805254161304,167.882510174425,
167.959765327986,168.037033669329,168.114329250584,168.191712858568,168.269142066837,
168.346691407948,168.417171378182,168.493222825901,168.569179416795,168.645057937724,
168.720875095421,168.796647535178,168.874055482536,168.949803530872,169.02555959287,
169.101338679446,169.179981788096,169.255894700938,169.331865080927,169.4079425746,
169.415911114044,169.494447054099,169.572890183717,169.651255011266,169.729555989654,
169.807807526105,169.886027083646,169.9642300052,170.042429289695,170.120637931507,
170.198901578368,170.277193684045,170.355569497197,170.414650849906,170.496300351367,
170.575865621596,170.658557238673,170.74124885575),.UNSPECIFIED.);
#3369=B_SPLINE_CURVE_WITH_KNOTS('',3,(#198075,#198076,#198077,#198078,#198079,
#198080,#198081,#198082,#198083,#198084,#198085,#198086,#198087,#198088,
#198089,#198090,#198091,#198092,#198093,#198094,#198095,#198096,#198097,
#198098,#198099,#198100,#198101,#198102,#198103,#198104,#198105,#198106,
#198107,#198108,#198109,#198110,#198111,#198112,#198113,#198114,#198115,
#198116,#198117,#198118,#198119,#198120,#198121,#198122,#198123,#198124,
#198125,#198126,#198127,#198128,#198129,#198130,#198131,#198132,#198133,
#198134,#198135,#198136,#198137,#198138,#198139,#198140,#198141,#198142,
#198143,#198144,#198145,#198146,#198147,#198148,#198149,#198150,#198151,
#198152,#198153,#198154,#198155,#198156,#198157,#198158,#198159,#198160,
#198161,#198162,#198163,#198164,#198165,#198166,#198167,#198168,#198169,
#198170,#198171,#198172,#198173,#198174,#198175,#198176,#198177,#198178,
#198179,#198180,#198181,#198182,#198183,#198184,#198185,#198186,#198187,
#198188,#198189,#198190,#198191,#198192,#198193,#198194,#198195,#198196,
#198197,#198198,#198199,#198200,#198201,#198202,#198203,#198204,#198205,
#198206,#198207,#198208,#198209,#198210,#198211,#198212,#198213,#198214,
#198215,#198216,#198217,#198218,#198219,#198220,#198221,#198222,#198223,
#198224,#198225,#198226,#198227,#198228,#198229,#198230,#198231,#198232,
#198233,#198234,#198235,#198236,#198237,#198238,#198239,#198240),
 .UNSPECIFIED.,.F.,.F.,(4,3,3,3,3,3,3,3,3,3,3,3,3,3,3,3,3,3,3,3,3,3,3,3,
3,3,3,3,3,3,3,3,3,3,3,3,3,3,3,3,3,3,3,3,3,3,3,3,3,3,3,3,3,3,3,4),(172.787595947439,
172.876862502991,172.966706250952,173.057285678573,173.093185671887,173.171721611942,
173.25016474156,173.328529569109,173.406830547497,173.485082083947,173.563301641489,
173.641504563043,173.719703847538,173.79791248935,173.876176136211,173.954468241888,
174.03284405504,174.091925407749,174.171567314175,174.251138933917,174.330651162886,
174.410106496576,174.489527672634,174.568924334211,174.591295275681,174.672525372307,
174.753804263359,174.838019483422,174.919450336843,175.005057740227,175.090665143612,
175.175908441911,175.261073516065,175.346087883942,175.430995192738,175.51570969501,
175.590035011543,175.666578014529,175.743115558872,175.81966225164,175.896264791928,
175.972898537244,176.04961592509,176.089404879474,176.168953942453,176.248442212459,
176.327881956182,176.407285402419,176.486671556819,176.566048604272,176.645427626364,
176.724819704607,176.804267800039,176.883744007039,176.96329955227,177.02436573765),
 .UNSPECIFIED.);
#3370=B_SPLINE_CURVE_WITH_KNOTS('',3,(#198241,#198242,#198243,#198244,#198245,
#198246,#198247,#198248,#198249,#198250,#198251,#198252,#198253,#198254,
#198255,#198256,#198257,#198258,#198259,#198260,#198261,#198262,#198263,
#198264,#198265,#198266,#198267,#198268,#198269,#198270,#198271,#198272,
#198273,#198274,#198275,#198276,#198277,#198278,#198279,#198280,#198281,
#198282,#198283,#198284,#198285,#198286,#198287,#198288,#198289,#198290,
#198291,#198292,#198293,#198294,#198295,#198296,#198297,#198298,#198299,
#198300,#198301,#198302,#198303,#198304,#198305,#198306,#198307,#198308,
#198309,#198310,#198311,#198312,#198313,#198314,#198315,#198316),
 .UNSPECIFIED.,.F.,.F.,(4,3,3,3,3,3,3,3,3,3,3,3,3,3,3,3,3,3,3,3,3,3,3,3,
3,4),(170.74108545857,170.823547062329,170.906008000208,170.988468299606,
171.070927987919,171.153387092541,171.235845640864,171.318303660278,171.400761178171,
171.48743835125,171.569905136859,171.65237024999,171.734833800297,171.817295897411,
171.899756650943,171.982216170485,172.064674565612,172.147131945883,172.229598331702,
172.312061533327,172.394521989275,172.476980137911,172.559445741923,172.6419056205,
172.724369732237,172.787595947439),.UNSPECIFIED.);
#3371=B_SPLINE_CURVE_WITH_KNOTS('',3,(#198318,#198319,#198320,#198321,#198322,
#198323,#198324,#198325,#198326,#198327,#198328,#198329,#198330,#198331,
#198332,#198333,#198334,#198335,#198336,#198337,#198338,#198339,#198340,
#198341,#198342,#198343,#198344,#198345,#198346,#198347,#198348,#198349,
#198350,#198351,#198352,#198353,#198354,#198355,#198356,#198357,#198358,
#198359,#198360,#198361,#198362,#198363,#198364,#198365,#198366,#198367,
#198368,#198369,#198370,#198371,#198372,#198373,#198374,#198375,#198376,
#198377,#198378,#198379,#198380,#198381,#198382,#198383,#198384,#198385,
#198386,#198387,#198388,#198389,#198390,#198391,#198392,#198393,#198394,
#198395,#198396,#198397,#198398,#198399),.UNSPECIFIED.,.F.,.F.,(4,3,3,3,
3,3,3,3,3,3,3,3,3,3,3,3,3,3,3,3,3,3,3,3,3,3,3,4),(170.74124885575,170.820666993372,
170.900061492849,170.914020717837,170.995250814463,171.076529705514,171.160744925578,
171.242175778998,171.327783182383,171.413390585768,171.498633884067,171.583798958223,
171.668813326101,171.753720634897,171.83843513717,171.9127604537,171.989303456686,
172.065841001029,172.142387693797,172.218990234086,172.295623979402,172.372341367248,
172.412130321631,172.505996728083,172.595652790931,172.685089950228,172.774119132675,
172.787595947439),.UNSPECIFIED.);
#3372=B_SPLINE_CURVE_WITH_KNOTS('',3,(#198400,#198401,#198402,#198403,#198404,
#198405,#198406,#198407,#198408,#198409,#198410,#198411,#198412,#198413,
#198414,#198415,#198416,#198417,#198418,#198419,#198420,#198421,#198422,
#198423,#198424,#198425,#198426,#198427,#198428,#198429,#198430,#198431,
#198432,#198433,#198434,#198435,#198436,#198437,#198438,#198439,#198440,
#198441,#198442,#198443,#198444,#198445,#198446,#198447,#198448,#198449,
#198450,#198451,#198452,#198453,#198454,#198455,#198456,#198457,#198458,
#198459,#198460,#198461,#198462,#198463,#198464,#198465,#198466,#198467,
#198468,#198469,#198470,#198471,#198472,#198473,#198474,#198475,#198476,
#198477,#198478,#198479,#198480,#198481,#198482,#198483,#198484,#198485,
#198486,#198487,#198488,#198489,#198490,#198491,#198492,#198493,#198494,
#198495,#198496,#198497,#198498,#198499,#198500,#198501,#198502,#198503,
#198504,#198505,#198506,#198507,#198508,#198509,#198510,#198511,#198512,
#198513,#198514,#198515,#198516,#198517,#198518,#198519,#198520,#198521,
#198522,#198523,#198524,#198525,#198526,#198527,#198528,#198529,#198530,
#198531,#198532,#198533,#198534,#198535,#198536,#198537,#198538,#198539,
#198540,#198541,#198542,#198543,#198544,#198545,#198546,#198547,#198548,
#198549,#198550,#198551,#198552,#198553,#198554,#198555,#198556),
 .UNSPECIFIED.,.F.,.F.,(4,3,3,3,3,3,3,3,3,3,3,3,3,3,3,3,3,3,3,3,3,3,3,3,
3,3,3,3,3,3,3,3,3,3,3,3,3,3,3,3,3,3,3,3,3,3,3,3,3,3,3,3,4),(172.787595947439,
172.870058153525,172.952520011313,173.034981527654,173.117442709398,173.199903563394,
173.282364096493,173.364824315543,173.447284227394,173.529743838893,173.61220315689,
173.694662188232,173.777120939767,173.859579418344,173.942037630808,174.024495584008,
174.106953284791,174.189410740003,174.271867956491,174.35788054428,174.441205238701,
174.523671844259,174.60613760561,174.688602550168,174.771066705346,174.853530098553,
174.935992757197,175.018454708681,175.100915980407,175.183376599775,175.265836594182,
175.348295991024,175.430754817692,175.513213101579,175.595670870072,175.67812815056,
175.762262064009,175.844728062307,175.927192438856,176.009655303298,176.092116765255,
176.174576934329,176.257035920104,176.339493832146,176.425090948847,176.507555685791,
176.590017458089,176.67247670418,176.754933862358,176.837396381257,176.919854052541,
177.002312843449,177.02427076575),.UNSPECIFIED.);
#3373=B_SPLINE_CURVE_WITH_KNOTS('',3,(#198562,#198563,#198564,#198565,#198566,
#198567,#198568,#198569,#198570,#198571,#198572,#198573,#198574,#198575,
#198576,#198577,#198578,#198579,#198580,#198581,#198582,#198583,#198584,
#198585,#198586,#198587,#198588,#198589,#198590,#198591,#198592,#198593,
#198594,#198595,#198596,#198597,#198598,#198599,#198600,#198601,#198602,
#198603,#198604,#198605,#198606,#198607,#198608,#198609,#198610,#198611,
#198612,#198613,#198614,#198615,#198616,#198617,#198618,#198619,#198620,
#198621,#198622,#198623,#198624,#198625,#198626,#198627,#198628,#198629,
#198630,#198631,#198632,#198633,#198634,#198635,#198636,#198637,#198638,
#198639,#198640,#198641,#198642,#198643,#198644,#198645,#198646,#198647,
#198648,#198649,#198650,#198651,#198652,#198653,#198654,#198655,#198656,
#198657,#198658,#198659,#198660,#198661,#198662,#198663,#198664,#198665,
#198666,#198667,#198668,#198669,#198670,#198671,#198672,#198673,#198674,
#198675,#198676,#198677,#198678,#198679,#198680,#198681,#198682,#198683,
#198684,#198685,#198686,#198687,#198688,#198689,#198690,#198691,#198692,
#198693,#198694,#198695,#198696,#198697,#198698,#198699,#198700,#198701,
#198702,#198703,#198704,#198705,#198706,#198707,#198708,#198709,#198710,
#198711,#198712,#198713,#198714,#198715,#198716,#198717,#198718,#198719,
#198720,#198721,#198722,#198723,#198724,#198725,#198726,#198727,#198728,
#198729,#198730,#198731,#198732,#198733),.UNSPECIFIED.,.F.,.F.,(4,3,3,3,
3,3,3,3,3,3,3,3,3,3,3,3,3,3,3,3,3,3,3,3,3,3,3,3,3,3,3,3,3,3,3,3,3,3,3,3,
3,3,3,3,3,3,3,3,3,3,3,3,3,3,3,3,3,4),(179.070781254619,179.08562408706,
179.161675534779,179.237632125673,179.313510646602,179.389327804299,179.465100244055,
179.542508191414,179.61825623975,179.694012301748,179.769791388324,179.848434496974,
179.924347409816,180.000317789805,180.076395283479,180.084363822923,180.162899762978,
180.241342892596,180.319707720146,180.398008698533,180.476260234983,180.554479792525,
180.632682714078,180.710881998573,180.789090640385,180.867354287246,180.945646392924,
181.024022206075,181.083103558785,181.162745465211,181.242317084953,181.321829313921,
181.401284647611,181.480705823669,181.560102485245,181.582473426716,181.663703523342,
181.744982414393,181.829197634456,181.910628487877,181.996235891262,182.081843294647,
182.167086592946,182.252251667101,182.337266034979,182.422173343774,182.506887846047,
182.581213162578,182.657756165564,182.734293709907,182.810840402675,182.887442942963,
182.964076688279,183.040794076125,183.080583030509,183.160132981289,183.239615331457,
183.307446438644),.UNSPECIFIED.);
#3374=B_SPLINE_CURVE_WITH_KNOTS('',3,(#198734,#198735,#198736,#198737,#198738,
#198739,#198740,#198741,#198742,#198743,#198744,#198745,#198746,#198747,
#198748,#198749,#198750,#198751,#198752,#198753,#198754,#198755,#198756,
#198757,#198758,#198759,#198760,#198761,#198762,#198763,#198764,#198765,
#198766,#198767,#198768,#198769,#198770,#198771,#198772,#198773,#198774,
#198775,#198776,#198777,#198778,#198779,#198780,#198781,#198782,#198783,
#198784,#198785,#198786,#198787,#198788,#198789,#198790,#198791,#198792,
#198793,#198794,#198795,#198796,#198797,#198798,#198799,#198800,#198801,
#198802,#198803,#198804,#198805,#198806,#198807,#198808,#198809,#198810,
#198811,#198812,#198813,#198814,#198815),.UNSPECIFIED.,.F.,.F.,(4,3,3,3,
3,3,3,3,3,3,3,3,3,3,3,3,3,3,3,3,3,3,3,3,3,3,3,4),(177.02436573765,177.088144615336,
177.165800373531,177.243369939261,177.320867245892,177.398295884327,177.475684730453,
177.553047624631,177.587514483267,177.671009290313,177.754660967303,177.838551362544,
177.922555807927,178.00674676615,178.086884351198,178.164139151355,178.241311843178,
178.318418290553,178.395474308542,178.472495674665,178.549511188248,178.626526849768,
178.703556916167,178.780615650056,178.857762652621,178.934956926078,179.012268091969,
179.070781254542),.UNSPECIFIED.);
#3375=B_SPLINE_CURVE_WITH_KNOTS('',3,(#198817,#198818,#198819,#198820,#198821,
#198822,#198823,#198824,#198825,#198826,#198827,#198828,#198829,#198830,
#198831,#198832,#198833,#198834,#198835,#198836,#198837,#198838,#198839,
#198840,#198841,#198842,#198843,#198844,#198845,#198846,#198847,#198848,
#198849,#198850,#198851,#198852,#198853,#198854,#198855,#198856,#198857,
#198858,#198859,#198860,#198861,#198862,#198863,#198864,#198865,#198866,
#198867,#198868,#198869,#198870,#198871,#198872,#198873,#198874,#198875,
#198876,#198877,#198878,#198879,#198880,#198881,#198882,#198883,#198884,
#198885,#198886,#198887,#198888,#198889,#198890,#198891,#198892),
 .UNSPECIFIED.,.F.,.F.,(4,3,3,3,3,3,3,3,3,3,3,3,3,3,3,3,3,3,3,3,3,3,3,3,
3,4),(177.02427076575,177.106732369508,177.189193307387,177.271653606785,
177.354113295099,177.436572399721,177.519030948044,177.601488967458,177.683946485351,
177.77062365843,177.853090444039,177.93555555717,178.018019107477,178.100481204591,
178.182941958123,178.265401477665,178.347859872792,178.430317253063,178.512783638882,
178.595246840506,178.677707296455,178.760165445091,178.842631049103,178.92509092768,
179.007555039417,179.070781254619),.UNSPECIFIED.);
#3376=B_SPLINE_CURVE_WITH_KNOTS('',3,(#198893,#198894,#198895,#198896,#198897,
#198898,#198899,#198900,#198901,#198902,#198903,#198904,#198905,#198906,
#198907,#198908,#198909,#198910,#198911,#198912,#198913,#198914,#198915,
#198916,#198917,#198918,#198919,#198920,#198921,#198922,#198923,#198924,
#198925,#198926,#198927,#198928,#198929,#198930,#198931,#198932,#198933,
#198934,#198935,#198936,#198937,#198938,#198939,#198940,#198941,#198942,
#198943,#198944,#198945,#198946,#198947,#198948,#198949,#198950,#198951,
#198952,#198953,#198954,#198955,#198956,#198957,#198958,#198959,#198960,
#198961,#198962,#198963,#198964,#198965,#198966,#198967,#198968,#198969,
#198970,#198971,#198972,#198973,#198974,#198975,#198976,#198977,#198978,
#198979,#198980,#198981,#198982,#198983,#198984,#198985,#198986,#198987,
#198988,#198989,#198990,#198991,#198992,#198993,#198994,#198995,#198996,
#198997,#198998,#198999,#199000,#199001,#199002,#199003,#199004,#199005,
#199006,#199007,#199008,#199009,#199010,#199011,#199012,#199013,#199014,
#199015,#199016,#199017,#199018,#199019,#199020,#199021,#199022,#199023,
#199024,#199025,#199026,#199027,#199028,#199029,#199030,#199031,#199032,
#199033,#199034,#199035,#199036,#199037,#199038,#199039,#199040,#199041,
#199042,#199043,#199044,#199045,#199046,#199047,#199048,#199049,#199050,
#199051,#199052,#199053,#199054,#199055,#199056,#199057,#199058,#199059,
#199060,#199061),.UNSPECIFIED.,.F.,.F.,(4,3,3,3,3,3,3,3,3,3,3,3,3,3,3,3,
3,3,3,3,3,3,3,3,3,3,3,3,3,3,3,3,3,3,3,3,3,3,3,3,3,3,3,3,3,3,3,3,3,3,3,3,
3,3,3,3,4),(179.070781254619,179.153913059131,179.234053402285,179.314265484234,
179.394594630683,179.403308472666,179.482855572747,179.562342404114,179.641781231694,
179.721184282941,179.800563756749,179.879944478968,179.959327882683,180.038725050785,
180.118147073781,180.197640507159,180.277172336546,180.356793064525,180.402048208528,
180.479703966723,180.557273532453,180.634770839085,180.712199477519,180.789588323645,
180.866951217823,180.901418076459,180.984912883505,181.068564560495,181.152454955735,
181.236459401119,181.320650359341,181.40078794439,181.478285291059,181.555700609411,
181.633049529079,181.71034763205,181.787610463375,181.864866476496,181.942121630057,
182.0193899714,182.096685552655,182.174069160639,182.251498368908,182.329047710019,
182.399527680252,182.475584479301,182.551545305904,182.627426953978,182.703246135693,
182.779020318668,182.854770603365,182.930512001994,183.006259518897,183.082065779061,
183.15790101961,183.233833983586,183.306487245332),.UNSPECIFIED.);
#3377=B_SPLINE_CURVE_WITH_KNOTS('',3,(#199067,#199068,#199069,#199070,#199071,
#199072,#199073,#199074,#199075,#199076,#199077,#199078,#199079,#199080,
#199081,#199082,#199083,#199084,#199085,#199086,#199087,#199088,#199089,
#199090,#199091,#199092,#199093,#199094,#199095,#199096,#199097,#199098,
#199099,#199100,#199101,#199102,#199103,#199104,#199105,#199106,#199107,
#199108,#199109,#199110,#199111,#199112,#199113,#199114,#199115,#199116,
#199117,#199118,#199119,#199120,#199121,#199122,#199123,#199124,#199125,
#199126,#199127,#199128,#199129,#199130,#199131,#199132,#199133,#199134,
#199135,#199136,#199137,#199138,#199139,#199140,#199141,#199142,#199143,
#199144,#199145,#199146,#199147,#199148,#199149,#199150,#199151,#199152,
#199153,#199154,#199155,#199156,#199157,#199158,#199159,#199160,#199161,
#199162,#199163,#199164,#199165,#199166,#199167,#199168,#199169,#199170,
#199171,#199172,#199173,#199174,#199175,#199176,#199177,#199178,#199179,
#199180,#199181,#199182,#199183,#199184,#199185,#199186,#199187,#199188,
#199189,#199190,#199191,#199192,#199193,#199194,#199195,#199196,#199197,
#199198,#199199,#199200,#199201,#199202,#199203,#199204,#199205,#199206,
#199207,#199208,#199209,#199210,#199211,#199212,#199213,#199214,#199215,
#199216,#199217,#199218,#199219,#199220,#199221,#199222,#199223,#199224,
#199225,#199226,#199227,#199228,#199229,#199230,#199231,#199232,#199233,
#199234,#199235,#199236,#199237,#199238),.UNSPECIFIED.,.F.,.F.,(4,3,3,3,
3,3,3,3,3,3,3,3,3,3,3,3,3,3,3,3,3,3,3,3,3,3,3,3,3,3,3,3,3,3,3,3,3,3,3,3,
3,3,3,3,3,3,3,3,3,3,3,3,3,3,3,3,3,4),(185.353966561799,185.431397596384,
185.512073176598,185.589494048608,185.66692687484,185.744385501764,185.821883787648,
185.899477736777,185.977127970281,186.054888344769,186.076802238096,186.152853685815,
186.228810276709,186.304688797638,186.380505955335,186.456278395092,186.53368634245,
186.609434390786,186.685190452784,186.76096953936,186.83961264801,186.915525560852,
186.991495940841,187.067573434515,187.075541973958,187.154077914013,187.232521043631,
187.31088587118,187.389186849568,187.467438386018,187.545657943559,187.623860865113,
187.702060149608,187.78026879142,187.858532438281,187.936824543958,188.015200357109,
188.07428170982,188.153923616247,188.233495235989,188.313007464958,188.392462798648,
188.471883974706,188.551280636283,188.573651577751,188.654881674376,188.736160565427,
188.82037578549,188.90180663891,188.987414042296,189.073021445682,189.158264743983,
189.24342981814,189.32844418602,189.413351494817,189.498065997092,189.572391313613,
189.59099683695),.UNSPECIFIED.);
#3378=B_SPLINE_CURVE_WITH_KNOTS('',3,(#199239,#199240,#199241,#199242,#199243,
#199244,#199245,#199246,#199247,#199248,#199249,#199250,#199251,#199252,
#199253,#199254,#199255,#199256,#199257,#199258,#199259,#199260,#199261,
#199262,#199263,#199264,#199265,#199266,#199267,#199268,#199269,#199270,
#199271,#199272,#199273,#199274,#199275,#199276,#199277,#199278,#199279,
#199280,#199281,#199282,#199283,#199284,#199285,#199286,#199287,#199288,
#199289,#199290,#199291,#199292,#199293,#199294,#199295,#199296,#199297,
#199298,#199299,#199300,#199301,#199302,#199303,#199304,#199305,#199306,
#199307,#199308,#199309,#199310,#199311,#199312,#199313,#199314,#199315,
#199316,#199317),.UNSPECIFIED.,.F.,.F.,(4,3,3,3,3,3,3,3,3,3,3,3,3,3,3,3,
3,3,3,3,3,3,3,3,3,3,4),(183.307446438644,183.386853957618,183.466236117432,
183.54561737589,183.624999696255,183.7043941609,183.783811858775,183.863300537031,
183.942826121031,184.022443246328,184.079322766371,184.156978524565,184.234548090295,
184.312045396926,184.38947403536,184.466862881487,184.544225775665,184.578692634302,
184.662187441348,184.745839118338,184.829729513579,184.913733958962,184.997924917185,
185.078062502233,185.169457246868,185.261711904271,185.353966561674),
 .UNSPECIFIED.);
#3379=B_SPLINE_CURVE_WITH_KNOTS('',3,(#199319,#199320,#199321,#199322,#199323,
#199324,#199325,#199326,#199327,#199328,#199329,#199330,#199331,#199332,
#199333,#199334,#199335,#199336,#199337,#199338,#199339,#199340,#199341,
#199342,#199343,#199344,#199345,#199346,#199347,#199348,#199349,#199350,
#199351,#199352,#199353,#199354,#199355,#199356,#199357,#199358,#199359,
#199360,#199361,#199362,#199363,#199364,#199365,#199366,#199367,#199368,
#199369,#199370,#199371,#199372,#199373,#199374,#199375,#199376,#199377,
#199378,#199379,#199380,#199381,#199382,#199383,#199384,#199385,#199386,
#199387,#199388,#199389,#199390,#199391,#199392,#199393,#199394,#199395,
#199396,#199397,#199398,#199399,#199400,#199401,#199402,#199403),
 .UNSPECIFIED.,.F.,.F.,(4,3,3,3,3,3,3,3,3,3,3,3,3,3,3,3,3,3,3,3,3,3,3,3,
3,3,3,3,4),(183.306487245332,183.382560392752,183.398267416115,183.47680335617,
183.555246485789,183.633611313337,183.711912291725,183.790163828176,183.868383385717,
183.946586307271,184.024785591766,184.102994233577,184.181257880439,184.259549986116,
184.337925799268,184.397007151977,184.476649058403,184.556220678145,184.635732907114,
184.715188240804,184.794609416862,184.874006078439,184.896377019908,184.976854947956,
185.057372730165,185.13797882469,185.218630132761,185.299378318199,185.353966561691),
 .UNSPECIFIED.);
#3380=B_SPLINE_CURVE_WITH_KNOTS('',3,(#199404,#199405,#199406,#199407,#199408,
#199409,#199410,#199411,#199412,#199413,#199414,#199415,#199416,#199417,
#199418,#199419,#199420,#199421,#199422,#199423,#199424,#199425,#199426,
#199427,#199428,#199429,#199430,#199431,#199432,#199433,#199434,#199435,
#199436,#199437,#199438,#199439,#199440,#199441,#199442,#199443,#199444,
#199445,#199446,#199447,#199448,#199449,#199450,#199451,#199452,#199453,
#199454,#199455,#199456,#199457,#199458,#199459,#199460,#199461,#199462,
#199463,#199464,#199465,#199466,#199467,#199468,#199469,#199470,#199471,
#199472,#199473,#199474,#199475,#199476,#199477,#199478,#199479,#199480,
#199481,#199482,#199483,#199484,#199485,#199486,#199487,#199488,#199489,
#199490,#199491,#199492,#199493,#199494,#199495,#199496,#199497,#199498,
#199499,#199500,#199501,#199502,#199503,#199504,#199505,#199506,#199507,
#199508,#199509,#199510,#199511,#199512,#199513,#199514,#199515,#199516,
#199517,#199518,#199519,#199520,#199521,#199522,#199523,#199524,#199525,
#199526,#199527,#199528,#199529,#199530,#199531,#199532,#199533,#199534,
#199535,#199536,#199537,#199538,#199539,#199540,#199541,#199542,#199543,
#199544,#199545,#199546,#199547,#199548,#199549,#199550,#199551,#199552,
#199553,#199554,#199555,#199556,#199557,#199558,#199559,#199560,#199561,
#199562,#199563,#199564,#199565,#199566,#199567,#199568,#199569,#199570,
#199571,#199572),.UNSPECIFIED.,.F.,.F.,(4,3,3,3,3,3,3,3,3,3,3,3,3,3,3,3,
3,3,3,3,3,3,3,3,3,3,3,3,3,3,3,3,3,3,3,3,3,3,3,3,3,3,3,3,3,3,3,3,3,3,3,3,
3,3,3,3,4),(185.353966561798,185.395746887839,185.480990186138,185.566155260292,
185.65116962817,185.736076936966,185.820791439238,185.89511675577,185.971659758756,
186.048197303098,186.124743995867,186.201346536155,186.277980281471,186.354697669317,
186.394486623701,186.474033723781,186.553520555149,186.632959382729,186.712362433976,
186.791741907784,186.871122630003,186.950506033717,187.029903201819,187.109325224816,
187.188818658194,187.268350487581,187.34797121556,187.393226359563,187.470882117758,
187.548451683488,187.62594899012,187.703377628554,187.780766474681,187.858129368859,
187.892596227494,187.97609103454,188.05974271153,188.143633106771,188.227637552155,
188.311828510378,188.391966095426,188.469463442095,188.546878760447,188.624227680115,
188.701525783086,188.778788614411,188.856044627531,188.933299781093,189.010568122436,
189.087863703691,189.165247311675,189.242676519944,189.320225861055,189.390705831288,
189.466769112667,189.542722467021,189.591595664567),.UNSPECIFIED.);
#3381=B_SPLINE_CURVE_WITH_KNOTS('',3,(#199578,#199579,#199580,#199581,#199582,
#199583,#199584,#199585,#199586,#199587,#199588,#199589,#199590,#199591,
#199592,#199593,#199594,#199595,#199596,#199597,#199598,#199599,#199600,
#199601,#199602,#199603,#199604,#199605,#199606,#199607,#199608,#199609,
#199610,#199611,#199612,#199613,#199614,#199615,#199616,#199617,#199618,
#199619,#199620,#199621,#199622,#199623,#199624,#199625,#199626,#199627,
#199628,#199629,#199630,#199631,#199632,#199633,#199634,#199635,#199636,
#199637,#199638,#199639,#199640,#199641,#199642,#199643,#199644,#199645,
#199646,#199647,#199648,#199649,#199650,#199651,#199652,#199653,#199654,
#199655,#199656,#199657,#199658,#199659,#199660,#199661,#199662,#199663,
#199664,#199665,#199666,#199667,#199668,#199669,#199670,#199671,#199672,
#199673,#199674,#199675,#199676,#199677,#199678,#199679,#199680,#199681,
#199682,#199683,#199684,#199685,#199686,#199687,#199688,#199689,#199690,
#199691,#199692,#199693,#199694,#199695,#199696,#199697,#199698,#199699,
#199700,#199701,#199702,#199703,#199704,#199705,#199706,#199707,#199708,
#199709,#199710,#199711,#199712,#199713,#199714,#199715,#199716,#199717,
#199718,#199719,#199720,#199721,#199722,#199723,#199724,#199725,#199726,
#199727,#199728,#199729,#199730,#199731,#199732,#199733,#199734,#199735,
#199736,#199737,#199738,#199739,#199740,#199741,#199742,#199743,#199744,
#199745,#199746),.UNSPECIFIED.,.F.,.F.,(4,3,3,3,3,3,3,3,3,3,3,3,3,3,3,3,
3,3,3,3,3,3,3,3,3,3,3,3,3,3,3,3,3,3,3,3,3,3,3,3,3,3,3,3,3,3,3,3,3,3,3,3,
3,3,3,3,4),(191.637151869054,191.722777560031,191.809393333341,191.89558240367,
191.982411528469,192.069240653269,192.146737999944,192.224153318303,192.301502237977,
192.378800340955,192.456063172286,192.533319185413,192.610574338981,192.687842680331,
192.765138261593,192.842521869583,192.919951077859,192.997500418976,193.067980389131,
193.144031836845,193.219988427734,193.295866948658,193.37168410635,193.447456546102,
193.524864493463,193.600612541795,193.676368603788,193.752147690359,193.830790799018,
193.906703711855,193.98267409184,194.058751585509,194.066720124993,194.14525606503,
194.22369919463,194.302064022161,194.38036500053,194.458616536963,194.536836094486,
194.615039016022,194.693238300499,194.771446942293,194.849710589137,194.928002694797,
195.006378507932,195.065459860855,195.145101767453,195.224673387365,195.304185616502,
195.383640950358,195.463062126579,195.542458788317,195.564829728786,195.646075149419,
195.727358735464,195.808726488626,195.873338800186),.UNSPECIFIED.);
#3382=B_SPLINE_CURVE_WITH_KNOTS('',3,(#199747,#199748,#199749,#199750,#199751,
#199752,#199753,#199754,#199755,#199756,#199757,#199758,#199759,#199760,
#199761,#199762,#199763,#199764,#199765,#199766,#199767,#199768,#199769,
#199770,#199771,#199772,#199773,#199774,#199775,#199776,#199777,#199778,
#199779,#199780,#199781,#199782,#199783,#199784,#199785,#199786,#199787,
#199788,#199789,#199790,#199791,#199792,#199793,#199794,#199795,#199796,
#199797,#199798,#199799,#199800,#199801,#199802,#199803,#199804,#199805,
#199806,#199807,#199808,#199809,#199810,#199811,#199812,#199813,#199814,
#199815,#199816,#199817,#199818,#199819,#199820,#199821,#199822,#199823,
#199824,#199825,#199826,#199827,#199828,#199829,#199830,#199831),
 .UNSPECIFIED.,.F.,.F.,(4,3,3,3,3,3,3,3,3,3,3,3,3,3,3,3,3,3,3,3,3,3,3,3,
3,3,3,3,4),(189.59099683695,189.667537169314,189.744075593563,189.820626716693,
189.897235631924,189.973878939468,190.050602334764,190.071761181544,190.151308281625,
190.230795112993,190.310233940575,190.389636991823,190.46901646563,190.54839718785,
190.627780591565,190.707177759668,190.786599782666,190.866093216045,190.945625045432,
191.025245773412,191.070500917407,191.148156675604,191.225726241338,191.303223547972,
191.380652186409,191.458041032538,191.535403926719,191.569870785338,191.637151868978),
 .UNSPECIFIED.);
#3383=B_SPLINE_CURVE_WITH_KNOTS('',3,(#199833,#199834,#199835,#199836,#199837,
#199838,#199839,#199840,#199841,#199842,#199843,#199844,#199845,#199846,
#199847,#199848,#199849,#199850,#199851,#199852,#199853,#199854,#199855,
#199856,#199857,#199858,#199859,#199860,#199861,#199862,#199863,#199864,
#199865,#199866,#199867,#199868,#199869,#199870,#199871,#199872,#199873,
#199874,#199875,#199876,#199877,#199878,#199879,#199880,#199881,#199882,
#199883,#199884,#199885,#199886,#199887,#199888,#199889,#199890,#199891,
#199892,#199893,#199894,#199895,#199896,#199897,#199898,#199899,#199900,
#199901,#199902,#199903,#199904,#199905,#199906,#199907,#199908,#199909,
#199910,#199911,#199912,#199913,#199914),.UNSPECIFIED.,.F.,.F.,(4,3,3,3,
3,3,3,3,3,3,3,3,3,3,3,3,3,3,3,3,3,3,3,3,3,3,3,4),(189.591595664567,189.667432750365,
189.743219200234,189.818971628897,189.894720555063,189.970471825777,190.04624044869,
190.122041443609,190.197934494988,190.273879391914,190.349940250266,190.38944556715,
190.467981507205,190.546424636823,190.624789464372,190.70309044276,190.78134197921,
190.859561536751,190.937764458305,191.0159637428,191.094172384611,191.172436031473,
191.25072813715,191.329103950301,191.388185303012,191.476084222021,191.563689717781,
191.637151868978),.UNSPECIFIED.);
#3384=B_SPLINE_CURVE_WITH_KNOTS('',3,(#199915,#199916,#199917,#199918,#199919,
#199920,#199921,#199922,#199923,#199924,#199925,#199926,#199927,#199928,
#199929,#199930,#199931,#199932,#199933,#199934,#199935,#199936,#199937,
#199938,#199939,#199940,#199941,#199942,#199943,#199944,#199945,#199946,
#199947,#199948,#199949,#199950,#199951,#199952,#199953,#199954,#199955,
#199956,#199957,#199958,#199959,#199960,#199961,#199962,#199963,#199964,
#199965,#199966,#199967,#199968,#199969,#199970,#199971,#199972,#199973,
#199974,#199975,#199976,#199977,#199978,#199979,#199980,#199981,#199982,
#199983,#199984,#199985,#199986,#199987,#199988,#199989,#199990,#199991,
#199992,#199993,#199994,#199995,#199996,#199997,#199998,#199999,#200000,
#200001,#200002,#200003,#200004,#200005,#200006,#200007,#200008,#200009,
#200010,#200011,#200012,#200013,#200014,#200015,#200016,#200017,#200018,
#200019,#200020,#200021,#200022,#200023,#200024,#200025,#200026,#200027,
#200028,#200029,#200030,#200031,#200032,#200033,#200034,#200035,#200036,
#200037,#200038,#200039,#200040,#200041,#200042,#200043,#200044,#200045,
#200046,#200047,#200048,#200049,#200050,#200051,#200052,#200053,#200054,
#200055,#200056,#200057,#200058,#200059,#200060,#200061,#200062,#200063,
#200064,#200065,#200066,#200067,#200068,#200069,#200070,#200071,#200072,
#200073,#200074,#200075,#200076,#200077,#200078,#200079,#200080,#200081,
#200082,#200083),.UNSPECIFIED.,.F.,.F.,(4,3,3,3,3,3,3,3,3,3,3,3,3,3,3,3,
3,3,3,3,3,3,3,3,3,3,3,3,3,3,3,3,3,3,3,3,3,3,3,3,3,3,3,3,3,3,3,3,3,3,3,3,
3,3,3,3,4),(191.63715186911,191.712667239094,191.788156227102,191.863640540428,
191.887555170943,191.968785267568,192.050064158618,192.134279378682,192.215710232102,
192.301317635488,192.386925038874,192.472168337175,192.557333411333,192.642347779213,
192.727255088011,192.811969590285,192.886294906805,192.962837909789,193.03937545413,
193.115922146896,193.192524687182,193.269158432496,193.34587582034,193.385664774736,
193.465211874817,193.544698706185,193.624137533766,193.703540585014,193.782920058823,
193.862300781042,193.941684184758,194.021081352861,194.100503375858,194.179996809237,
194.259528638625,194.339149366605,194.384404510599,194.462060268796,194.539629834529,
194.617127141162,194.694555779599,194.771944625727,194.849307519907,194.88377437853,
194.967269185567,195.050920862549,195.134811257781,195.218815703156,195.303006661369,
195.383144246461,195.46064239363,195.538061228243,195.615414915786,195.692710924807,
195.769973698718,195.847219668722,195.873920875799),.UNSPECIFIED.);
#3385=B_SPLINE_CURVE_WITH_KNOTS('',3,(#200089,#200090,#200091,#200092,#200093,
#200094,#200095,#200096,#200097,#200098,#200099,#200100,#200101,#200102,
#200103,#200104,#200105,#200106,#200107,#200108,#200109,#200110,#200111,
#200112,#200113,#200114,#200115,#200116,#200117,#200118,#200119,#200120,
#200121,#200122,#200123,#200124,#200125,#200126,#200127,#200128,#200129,
#200130,#200131,#200132,#200133,#200134,#200135,#200136,#200137,#200138,
#200139,#200140,#200141,#200142,#200143,#200144,#200145,#200146,#200147,
#200148,#200149,#200150,#200151,#200152,#200153,#200154,#200155,#200156,
#200157,#200158,#200159,#200160,#200161,#200162,#200163,#200164,#200165,
#200166,#200167,#200168,#200169,#200170,#200171,#200172,#200173,#200174,
#200175,#200176,#200177,#200178,#200179,#200180,#200181,#200182,#200183,
#200184,#200185,#200186,#200187,#200188,#200189,#200190,#200191,#200192,
#200193,#200194,#200195,#200196,#200197,#200198,#200199,#200200,#200201,
#200202,#200203,#200204,#200205,#200206,#200207,#200208,#200209,#200210,
#200211,#200212,#200213,#200214,#200215,#200216,#200217,#200218,#200219,
#200220,#200221,#200222,#200223,#200224,#200225,#200226,#200227,#200228,
#200229,#200230,#200231,#200232,#200233,#200234,#200235,#200236,#200237,
#200238,#200239,#200240,#200241,#200242,#200243,#200244,#200245),
 .UNSPECIFIED.,.F.,.F.,(4,3,3,3,3,3,3,3,3,3,3,3,3,3,3,3,3,3,3,3,3,3,3,3,
3,3,3,3,3,3,3,3,3,3,3,3,3,3,3,3,3,3,3,3,3,3,3,3,3,3,3,3,4),(197.920337176158,
198.002799382244,198.085261240032,198.167722756373,198.250183938117,198.332644792113,
198.415105325212,198.497565544262,198.580025456113,198.662485067612,198.744944385609,
198.827403416951,198.909862168486,198.992320647062,199.074778859527,199.157236812727,
199.239694513509,199.322151968721,199.404609185209,199.490621772998,199.573946467419,
199.656413072977,199.738878834328,199.821343778886,199.903807934064,199.986271327272,
200.068733985915,200.151195937399,200.233657209125,200.316117828494,200.398577822901,
200.481037219742,200.56349604641,200.645954330297,200.72841209879,200.810869379278,
200.895003292727,200.977469291026,201.059933667574,201.142396532016,201.224857993973,
201.307318163047,201.389777148822,201.472235060865,201.557832177565,201.640296914509,
201.722758686807,201.805217932898,201.887675091076,201.970137609975,202.052595281259,
202.135054072167,202.157011994468),.UNSPECIFIED.);
#3386=B_SPLINE_CURVE_WITH_KNOTS('',3,(#200246,#200247,#200248,#200249,#200250,
#200251,#200252,#200253,#200254,#200255,#200256,#200257,#200258,#200259,
#200260,#200261,#200262,#200263,#200264,#200265,#200266,#200267,#200268,
#200269,#200270,#200271,#200272,#200273,#200274,#200275,#200276,#200277,
#200278,#200279,#200280,#200281,#200282,#200283,#200284,#200285,#200286,
#200287,#200288,#200289,#200290,#200291,#200292,#200293,#200294,#200295,
#200296,#200297,#200298,#200299,#200300,#200301,#200302,#200303,#200304,
#200305,#200306,#200307,#200308,#200309,#200310,#200311,#200312,#200313,
#200314,#200315,#200316,#200317,#200318,#200319,#200320,#200321,#200322,
#200323,#200324,#200325,#200326,#200327),.UNSPECIFIED.,.F.,.F.,(4,3,3,3,
3,3,3,3,3,3,3,3,3,3,3,3,3,3,3,3,3,3,3,3,3,3,3,4),(195.873338800186,195.954809490736,
196.0363716785,196.064199596717,196.149442895975,196.234607971085,196.319622339893,
196.404529649599,196.489244152733,196.563569464649,196.640112467048,196.716650010802,
196.79319670298,196.869799242676,196.946432987399,197.023150374653,197.06293933258,
197.141254613705,197.219504647999,197.297703969043,197.375870244731,197.454019045512,
197.532163481228,197.610316656745,197.688526923362,197.766765200274,197.845093906415,
197.920020567871),.UNSPECIFIED.);
#3387=B_SPLINE_CURVE_WITH_KNOTS('',3,(#200329,#200330,#200331,#200332,#200333,
#200334,#200335,#200336,#200337,#200338,#200339,#200340,#200341,#200342,
#200343,#200344,#200345,#200346,#200347,#200348,#200349,#200350,#200351,
#200352,#200353,#200354,#200355,#200356,#200357,#200358,#200359,#200360,
#200361,#200362,#200363,#200364,#200365,#200366,#200367,#200368,#200369,
#200370,#200371,#200372,#200373,#200374,#200375,#200376,#200377,#200378,
#200379,#200380,#200381,#200382,#200383,#200384,#200385,#200386,#200387,
#200388,#200389,#200390,#200391,#200392,#200393,#200394,#200395,#200396,
#200397,#200398,#200399,#200400,#200401,#200402,#200403,#200404,#200405,
#200406,#200407,#200408,#200409,#200410,#200411,#200412,#200413),
 .UNSPECIFIED.,.F.,.F.,(4,3,3,3,3,3,3,3,3,3,3,3,3,3,3,3,3,3,3,3,3,3,3,3,
3,3,3,3,4),(195.873920875799,195.951178998411,196.028455164163,196.105763428659,
196.183161355019,196.260609253835,196.338169692647,196.381883982323,196.457935430037,
196.533892020926,196.60977054185,196.685587699543,196.761360139294,196.838768086655,
196.914516134987,196.99027219698,197.066051283551,197.14469439221,197.220607305047,
197.296577685031,197.3726551787,197.380623718185,197.463675812328,197.54659562608,
197.629382895476,197.71197907297,197.794456993383,197.876765736192,197.920337176158),
 .UNSPECIFIED.);
#3388=B_SPLINE_CURVE_WITH_KNOTS('',3,(#200414,#200415,#200416,#200417,#200418,
#200419,#200420,#200421,#200422,#200423,#200424,#200425,#200426,#200427,
#200428,#200429,#200430,#200431,#200432,#200433,#200434,#200435,#200436,
#200437,#200438,#200439,#200440,#200441,#200442,#200443,#200444,#200445,
#200446,#200447,#200448,#200449,#200450,#200451,#200452,#200453,#200454,
#200455,#200456,#200457,#200458,#200459,#200460,#200461,#200462,#200463,
#200464,#200465,#200466,#200467,#200468,#200469,#200470,#200471,#200472,
#200473,#200474,#200475,#200476,#200477,#200478,#200479,#200480,#200481,
#200482,#200483,#200484,#200485,#200486,#200487,#200488,#200489,#200490,
#200491,#200492,#200493,#200494,#200495,#200496,#200497,#200498,#200499,
#200500,#200501,#200502,#200503,#200504,#200505,#200506,#200507,#200508,
#200509,#200510,#200511,#200512,#200513,#200514,#200515,#200516,#200517,
#200518,#200519,#200520,#200521,#200522,#200523,#200524,#200525,#200526,
#200527,#200528,#200529,#200530,#200531,#200532,#200533,#200534,#200535,
#200536,#200537,#200538,#200539,#200540,#200541,#200542,#200543,#200544,
#200545,#200546,#200547,#200548,#200549,#200550,#200551,#200552,#200553,
#200554,#200555,#200556,#200557,#200558,#200559,#200560,#200561,#200562,
#200563,#200564,#200565,#200566,#200567,#200568,#200569,#200570,#200571,
#200572,#200573,#200574,#200575,#200576,#200577,#200578,#200579,#200580,
#200581,#200582),.UNSPECIFIED.,.F.,.F.,(4,3,3,3,3,3,3,3,3,3,3,3,3,3,3,3,
3,3,3,3,3,3,3,3,3,3,3,3,3,3,3,3,3,3,3,3,3,3,3,3,3,3,3,3,3,3,3,3,3,3,3,3,
3,3,3,3,4),(197.920337176249,198.001811496667,198.083366322772,198.16506079004,
198.246827236305,198.328722029106,198.379363454047,198.459005360645,198.538576980557,
198.618089209695,198.697544543551,198.776965719773,198.856362381511,198.878733321978,
198.959963418148,199.041242308738,199.125457529031,199.206888381984,199.292495785947,
199.37810318991,199.463346489168,199.548511564278,199.633525933087,199.718433242792,
199.803147745927,199.877473057841,199.95401606024,200.030553603994,200.107100296171,
200.183702835867,200.26033658059,200.337053967844,200.376842925772,200.456390025619,
200.535876856751,200.615315684094,200.694718735104,200.774098208674,200.853478930655,
200.932862334133,201.012259502,201.091681524763,201.171174957912,201.250706787073,
201.330327514831,201.375582661634,201.453238422483,201.530807990849,201.608305300095,
201.685733941103,201.763122789781,201.840485686468,201.874952529565,201.958466595275,
202.042112648761,202.125946971428,202.156438065284),.UNSPECIFIED.);
#3389=B_SPLINE_CURVE_WITH_KNOTS('',3,(#200588,#200589,#200590,#200591,#200592,
#200593,#200594,#200595,#200596,#200597,#200598,#200599,#200600,#200601,
#200602,#200603,#200604,#200605,#200606,#200607,#200608,#200609,#200610,
#200611,#200612,#200613,#200614,#200615,#200616,#200617,#200618,#200619,
#200620,#200621,#200622,#200623,#200624,#200625,#200626,#200627,#200628,
#200629,#200630,#200631,#200632,#200633,#200634,#200635,#200636,#200637,
#200638,#200639,#200640,#200641,#200642,#200643,#200644,#200645,#200646,
#200647,#200648,#200649,#200650,#200651,#200652,#200653,#200654,#200655,
#200656,#200657,#200658,#200659,#200660,#200661,#200662,#200663,#200664,
#200665,#200666,#200667,#200668,#200669,#200670,#200671,#200672,#200673,
#200674,#200675,#200676,#200677,#200678,#200679,#200680,#200681,#200682,
#200683,#200684,#200685,#200686,#200687,#200688,#200689,#200690,#200691,
#200692,#200693,#200694,#200695,#200696,#200697,#200698,#200699,#200700,
#200701,#200702,#200703,#200704,#200705,#200706,#200707,#200708,#200709,
#200710,#200711,#200712,#200713,#200714,#200715,#200716,#200717,#200718,
#200719,#200720,#200721,#200722,#200723,#200724,#200725,#200726,#200727,
#200728,#200729,#200730,#200731,#200732,#200733,#200734,#200735,#200736,
#200737,#200738,#200739,#200740,#200741,#200742,#200743,#200744,#200745,
#200746,#200747,#200748,#200749,#200750,#200751,#200752,#200753,#200754,
#200755,#200756),.UNSPECIFIED.,.F.,.F.,(4,3,3,3,3,3,3,3,3,3,3,3,3,3,3,3,
3,3,3,3,3,3,3,3,3,3,3,3,3,3,3,3,3,3,3,3,3,3,3,3,3,3,3,3,3,3,3,3,3,3,3,3,
3,3,3,3,4),(204.203659867042,204.282057378475,204.36039811403,204.438696428595,
204.516973582366,204.595240588629,204.673510413808,204.751796023574,204.830147683781,
204.908533223077,204.987014140183,205.052857219477,205.130514306352,205.208085189046,
205.285583799584,205.36301371886,205.440403832364,205.517767970131,205.552227087408,
205.635719308127,205.71936831139,205.803255943232,205.887257587671,205.971445730659,
206.051596955339,206.129094684765,206.206510387096,206.283859691591,206.361158179864,
206.438421396594,206.515677793993,206.592933331113,206.670202054961,206.747498017334,
206.82488200221,206.902311585639,206.97986129538,207.050336691201,207.126389643378,
207.202347740836,207.27822776957,207.354046435493,207.429820383108,207.507227388603,
207.582976938562,207.658734499003,207.734515080148,207.813155416877,207.889069804123,
207.965041652723,208.041120598871,208.049076427064,208.127620794225,208.206046135226,
208.284403138728,208.362691339206,208.440597004682),.UNSPECIFIED.);
#3390=B_SPLINE_CURVE_WITH_KNOTS('',3,(#200757,#200758,#200759,#200760,#200761,
#200762,#200763,#200764,#200765,#200766,#200767,#200768,#200769,#200770,
#200771,#200772,#200773,#200774,#200775,#200776,#200777,#200778,#200779,
#200780,#200781,#200782,#200783,#200784,#200785,#200786,#200787,#200788,
#200789,#200790,#200791,#200792,#200793,#200794,#200795,#200796,#200797,
#200798,#200799,#200800,#200801,#200802,#200803,#200804,#200805,#200806,
#200807,#200808,#200809,#200810,#200811,#200812,#200813,#200814,#200815,
#200816,#200817,#200818,#200819,#200820,#200821,#200822,#200823,#200824,
#200825,#200826,#200827,#200828,#200829,#200830,#200831,#200832),
 .UNSPECIFIED.,.F.,.F.,(4,3,3,3,3,3,3,3,3,3,3,3,3,3,3,3,3,3,3,3,3,3,3,3,
3,4),(202.157011994468,202.239473598227,202.321934536106,202.404394835504,
202.486854523817,202.569313628439,202.651772176762,202.734230196176,202.816687714069,
202.903364887149,202.985831672757,203.068296785888,203.150760336195,203.233222433309,
203.315683186841,203.398142706383,203.48060110151,203.563058481781,203.645524867601,
203.727988069225,203.810448525173,203.89290667381,203.975372277821,204.057832156399,
204.140296268135,204.203522483337),.UNSPECIFIED.);
#3391=B_SPLINE_CURVE_WITH_KNOTS('',3,(#200834,#200835,#200836,#200837,#200838,
#200839,#200840,#200841,#200842,#200843,#200844,#200845,#200846,#200847,
#200848,#200849,#200850,#200851,#200852,#200853,#200854,#200855,#200856,
#200857,#200858,#200859,#200860,#200861,#200862,#200863,#200864,#200865,
#200866,#200867,#200868,#200869,#200870,#200871,#200872,#200873,#200874,
#200875,#200876,#200877,#200878,#200879,#200880,#200881,#200882,#200883,
#200884,#200885,#200886,#200887,#200888,#200889,#200890,#200891,#200892,
#200893,#200894,#200895,#200896,#200897,#200898,#200899,#200900,#200901,
#200902,#200903,#200904,#200905,#200906,#200907,#200908,#200909,#200910,
#200911,#200912,#200913,#200914,#200915),.UNSPECIFIED.,.F.,.F.,(4,3,3,3,
3,3,3,3,3,3,3,3,3,3,3,3,3,3,3,3,3,3,3,3,3,3,3,4),(202.156438065284,202.240482660956,
202.324695436608,202.374322397496,202.451819746577,202.529235067353,202.606583989454,
202.683882094865,202.761144928634,202.838400944198,202.915656100203,202.992924443985,
203.070220027675,203.147603638072,203.225032848747,203.302582192226,203.373062133358,
203.448085410478,203.523014838254,203.597867719145,203.673574564657,203.748326540048,
203.823058147509,203.897784777458,203.974219203903,204.049010926107,204.126266704672,
204.203522483237),.UNSPECIFIED.);
#3392=B_SPLINE_CURVE_WITH_KNOTS('',3,(#200916,#200917,#200918,#200919,#200920,
#200921,#200922,#200923,#200924,#200925,#200926,#200927,#200928,#200929,
#200930,#200931,#200932,#200933,#200934,#200935,#200936,#200937,#200938,
#200939,#200940,#200941,#200942,#200943,#200944,#200945,#200946,#200947,
#200948,#200949,#200950,#200951,#200952,#200953,#200954,#200955,#200956,
#200957,#200958,#200959,#200960,#200961,#200962,#200963,#200964,#200965,
#200966,#200967,#200968,#200969,#200970,#200971,#200972,#200973,#200974,
#200975,#200976,#200977,#200978,#200979,#200980,#200981,#200982,#200983,
#200984,#200985,#200986,#200987,#200988,#200989,#200990,#200991,#200992,
#200993,#200994,#200995,#200996,#200997,#200998,#200999,#201000,#201001,
#201002,#201003,#201004,#201005,#201006,#201007,#201008,#201009,#201010,
#201011,#201012,#201013,#201014,#201015,#201016,#201017,#201018,#201019,
#201020,#201021,#201022,#201023,#201024,#201025,#201026,#201027,#201028,
#201029,#201030,#201031,#201032,#201033,#201034,#201035,#201036,#201037,
#201038,#201039,#201040,#201041,#201042,#201043,#201044,#201045,#201046,
#201047,#201048,#201049,#201050,#201051,#201052,#201053,#201054,#201055,
#201056,#201057,#201058,#201059,#201060,#201061,#201062,#201063,#201064,
#201065,#201066,#201067,#201068,#201069,#201070,#201071,#201072,#201073,
#201074,#201075,#201076,#201077,#201078,#201079,#201080,#201081),
 .UNSPECIFIED.,.F.,.F.,(4,3,3,3,3,3,3,3,3,3,3,3,3,3,3,3,3,3,3,3,3,3,3,3,
3,3,3,3,3,3,3,3,3,3,3,3,3,3,3,3,3,3,3,3,3,3,3,3,3,3,3,3,3,3,3,4),(204.203522483337,
204.315702114456,204.37180186922,204.450337797205,204.528780914758,204.607145730263,
204.685446696645,204.763698221147,204.841917766874,204.920120676704,204.998319949582,
205.076528579899,205.154792215521,205.233084310092,205.311460112448,205.370541605083,
205.450183583791,205.529755275205,205.609267575084,205.688722978227,205.768144222806,
205.847540951289,205.869911473014,205.951141426241,206.032420172309,206.116635464468,
206.198066171773,206.283673756359,206.369281340945,206.454524813157,206.539690059704,
206.624704594246,206.709612065255,206.794326720147,206.868651208876,206.945194212473,
207.021731757981,207.098278452464,207.174880995286,207.251514743603,207.328232135144,
207.368021076807,207.447567895918,207.527054444051,207.606492986769,207.685895752165,
207.765274939768,207.844655376906,207.924038496621,208.003435382372,208.08285712523,
208.162350283778,208.241881841262,208.321502304389,208.366760812669,208.440825084745),
 .UNSPECIFIED.);
#3393=B_SPLINE_CURVE_WITH_KNOTS('',3,(#201087,#201088,#201089,#201090,#201091,
#201092,#201093,#201094,#201095,#201096,#201097,#201098,#201099,#201100,
#201101,#201102,#201103,#201104,#201105,#201106,#201107,#201108,#201109,
#201110,#201111,#201112,#201113,#201114,#201115,#201116,#201117,#201118,
#201119,#201120,#201121,#201122,#201123,#201124,#201125,#201126,#201127,
#201128,#201129,#201130,#201131,#201132,#201133,#201134,#201135,#201136,
#201137,#201138,#201139,#201140,#201141,#201142,#201143,#201144,#201145,
#201146,#201147,#201148,#201149,#201150,#201151,#201152,#201153,#201154,
#201155,#201156,#201157,#201158,#201159,#201160,#201161,#201162,#201163,
#201164,#201165,#201166,#201167,#201168,#201169,#201170,#201171,#201172,
#201173,#201174,#201175,#201176,#201177,#201178,#201179,#201180,#201181,
#201182,#201183,#201184,#201185,#201186,#201187,#201188,#201189,#201190,
#201191,#201192,#201193,#201194,#201195,#201196,#201197,#201198,#201199,
#201200,#201201,#201202,#201203,#201204,#201205,#201206,#201207,#201208,
#201209,#201210,#201211,#201212,#201213,#201214,#201215,#201216,#201217,
#201218,#201219,#201220,#201221,#201222,#201223,#201224,#201225,#201226,
#201227,#201228,#201229,#201230,#201231,#201232,#201233,#201234,#201235,
#201236,#201237,#201238,#201239,#201240,#201241,#201242,#201243),
 .UNSPECIFIED.,.F.,.F.,(4,3,3,3,3,3,3,3,3,3,3,3,3,3,3,3,3,3,3,3,3,3,3,3,
3,3,3,3,3,3,3,3,3,3,3,3,3,3,3,3,3,3,3,3,3,3,3,3,3,3,3,3,4),(210.486707790517,
210.569169996603,210.651631854391,210.734093370732,210.816554552476,210.899015406472,
210.981475939571,211.063936158621,211.146396070472,211.228855681971,211.311314999968,
211.39377403131,211.476232782845,211.558691261421,211.641149473886,211.723607427086,
211.806065127869,211.888522583081,211.970979799568,212.056992387357,212.140317081778,
212.222783687337,212.305249448687,212.387714393245,212.470178548423,212.552641941631,
212.635104600274,212.717566551758,212.800027823484,212.882488442853,212.96494843726,
213.047407834101,213.12986666077,213.212324944656,213.294782713149,213.377239993637,
213.461373907087,213.543839905385,213.626304281934,213.708767146376,213.791228608333,
213.873688777406,213.956147763181,214.038605675224,214.124202791924,214.206667528868,
214.289129301166,214.371588547257,214.454045705436,214.536508224335,214.618965895618,
214.701424686527,214.723382608827),.UNSPECIFIED.);
#3394=B_SPLINE_CURVE_WITH_KNOTS('',3,(#201244,#201245,#201246,#201247,#201248,
#201249,#201250,#201251,#201252,#201253,#201254,#201255,#201256,#201257,
#201258,#201259,#201260,#201261,#201262,#201263,#201264,#201265,#201266,
#201267,#201268,#201269,#201270,#201271,#201272,#201273,#201274,#201275,
#201276,#201277,#201278,#201279,#201280,#201281,#201282,#201283,#201284,
#201285,#201286,#201287,#201288,#201289,#201290,#201291,#201292,#201293,
#201294,#201295,#201296,#201297,#201298,#201299,#201300,#201301,#201302,
#201303,#201304,#201305,#201306,#201307,#201308,#201309,#201310,#201311,
#201312,#201313,#201314,#201315,#201316,#201317,#201318,#201319,#201320,
#201321,#201322,#201323,#201324,#201325),.UNSPECIFIED.,.F.,.F.,(4,3,3,3,
3,3,3,3,3,3,3,3,3,3,3,3,3,3,3,3,3,3,3,3,3,3,3,4),(208.440597004682,208.518812276007,
208.597010896499,208.675205870884,208.753410199333,208.831669612429,208.909957488982,
208.988329272838,209.047816162926,209.12747366929,209.207060694072,209.286588100935,
209.366058206105,209.44549389951,209.524904654142,209.547186030857,209.628406451149,
209.709675712718,209.793895759235,209.875317275478,209.960936587133,210.046555898788,
210.132401266205,210.220977897283,210.306584737466,210.392072940271,210.477374349878,
210.486707790517),.UNSPECIFIED.);
#3395=B_SPLINE_CURVE_WITH_KNOTS('',3,(#201327,#201328,#201329,#201330,#201331,
#201332,#201333,#201334,#201335,#201336,#201337,#201338,#201339,#201340,
#201341,#201342,#201343,#201344,#201345,#201346,#201347,#201348,#201349,
#201350,#201351,#201352,#201353,#201354,#201355,#201356,#201357,#201358,
#201359,#201360,#201361,#201362,#201363,#201364,#201365,#201366,#201367,
#201368,#201369,#201370,#201371,#201372,#201373,#201374,#201375,#201376,
#201377,#201378,#201379,#201380,#201381,#201382,#201383,#201384,#201385,
#201386,#201387,#201388,#201389,#201390,#201391,#201392,#201393,#201394,
#201395,#201396,#201397,#201398,#201399,#201400,#201401,#201402,#201403,
#201404,#201405),.UNSPECIFIED.,.F.,.F.,(4,3,3,3,3,3,3,3,3,3,3,3,3,3,3,3,
3,3,3,3,3,3,3,3,3,3,4),(208.440825084745,208.518399650002,208.59590129923,
208.673333362129,208.750725044706,208.828090323961,208.8661306806,208.94962290132,
209.033271904583,209.117159536426,209.201161180865,209.285349323853,209.365500548531,
209.442998277957,209.520413980288,209.597763284783,209.675061773056,209.752324989785,
209.829581387185,209.906836924305,209.984105648153,210.061401610526,210.138785595401,
210.21621517883,210.293764888572,210.364240284394,210.486707790517),
 .UNSPECIFIED.);
#3396=B_SPLINE_CURVE_WITH_KNOTS('',3,(#201406,#201407,#201408,#201409,#201410,
#201411,#201412,#201413,#201414,#201415,#201416,#201417,#201418,#201419,
#201420,#201421,#201422,#201423,#201424,#201425,#201426,#201427,#201428,
#201429,#201430,#201431,#201432,#201433,#201434,#201435,#201436,#201437,
#201438,#201439,#201440,#201441,#201442,#201443,#201444,#201445,#201446,
#201447,#201448,#201449,#201450,#201451,#201452,#201453,#201454,#201455,
#201456,#201457,#201458,#201459,#201460,#201461,#201462,#201463,#201464,
#201465,#201466,#201467,#201468,#201469,#201470,#201471,#201472,#201473,
#201474,#201475,#201476,#201477,#201478,#201479,#201480,#201481,#201482,
#201483,#201484,#201485,#201486,#201487,#201488,#201489,#201490,#201491,
#201492,#201493,#201494,#201495,#201496,#201497,#201498,#201499,#201500,
#201501,#201502,#201503,#201504,#201505,#201506,#201507,#201508,#201509,
#201510,#201511,#201512,#201513,#201514,#201515,#201516,#201517,#201518,
#201519,#201520,#201521,#201522,#201523,#201524,#201525,#201526,#201527,
#201528,#201529,#201530,#201531,#201532,#201533,#201534,#201535,#201536,
#201537,#201538,#201539,#201540,#201541,#201542,#201543,#201544,#201545,
#201546,#201547,#201548,#201549,#201550,#201551,#201552,#201553,#201554,
#201555,#201556,#201557,#201558,#201559,#201560,#201561,#201562,#201563,
#201564,#201565,#201566,#201567,#201568,#201569,#201570,#201571,#201572,
#201573,#201574),.UNSPECIFIED.,.F.,.F.,(4,3,3,3,3,3,3,3,3,3,3,3,3,3,3,3,
3,3,3,3,3,3,3,3,3,3,3,3,3,3,3,3,3,3,3,3,3,3,3,3,3,3,3,3,3,3,3,3,3,3,3,3,
3,3,3,3,4),(210.486707790606,210.561591694908,210.636397075426,210.711141145154,
210.785841020379,210.86052438242,210.935201569189,211.009887983622,211.084599042084,
211.159395255186,211.234237161341,211.30919544728,211.362980020256,211.44151141379,
211.519950009753,211.598310322816,211.676606812219,211.754853891543,211.833069058421,
211.911267633218,211.989462620625,212.067667020809,212.145926536013,212.224214567682,
212.30258643611,212.361719756118,212.441377262482,212.520964287265,212.600491694128,
212.679961799299,212.759397492703,212.838808247335,212.861089624049,212.942310044341,
213.023579305909,213.107799352426,213.189220868669,213.274840180325,213.36045949198,
213.445640227046,213.530742457118,213.615694795245,213.70054100553,213.785196810594,
213.859829359911,213.936480639936,214.01312726593,214.089783766943,214.166496860638,
214.243241660399,214.320070344098,214.359199227842,214.438616377869,214.517958670035,
214.59725648799,214.67651754967,214.723306029336),.UNSPECIFIED.);
#3397=B_SPLINE_CURVE_WITH_KNOTS('',3,(#201580,#201581,#201582,#201583,#201584,
#201585,#201586,#201587,#201588,#201589,#201590,#201591,#201592,#201593,
#201594,#201595,#201596,#201597,#201598,#201599,#201600,#201601,#201602,
#201603,#201604,#201605,#201606,#201607,#201608,#201609,#201610,#201611,
#201612,#201613,#201614,#201615,#201616,#201617,#201618,#201619,#201620,
#201621,#201622,#201623,#201624,#201625,#201626,#201627,#201628,#201629,
#201630,#201631,#201632,#201633,#201634,#201635,#201636,#201637,#201638,
#201639,#201640,#201641,#201642,#201643,#201644,#201645,#201646,#201647,
#201648,#201649,#201650,#201651,#201652,#201653,#201654,#201655,#201656,
#201657,#201658,#201659,#201660,#201661,#201662,#201663,#201664,#201665,
#201666,#201667,#201668,#201669,#201670,#201671,#201672,#201673,#201674,
#201675,#201676,#201677,#201678,#201679,#201680,#201681,#201682,#201683,
#201684,#201685,#201686,#201687,#201688,#201689,#201690,#201691,#201692,
#201693,#201694,#201695,#201696,#201697,#201698,#201699,#201700,#201701,
#201702,#201703,#201704,#201705,#201706,#201707,#201708,#201709,#201710,
#201711,#201712,#201713,#201714,#201715,#201716,#201717,#201718,#201719,
#201720,#201721,#201722,#201723,#201724,#201725,#201726,#201727,#201728,
#201729,#201730,#201731,#201732,#201733,#201734,#201735,#201736),
 .UNSPECIFIED.,.F.,.F.,(4,3,3,3,3,3,3,3,3,3,3,3,3,3,3,3,3,3,3,3,3,3,3,3,
3,3,3,3,3,3,3,3,3,3,3,3,3,3,3,3,3,3,3,3,3,3,3,3,3,3,3,3,4),(216.769893097833,
216.852355303918,216.934817161707,217.017278678048,217.099739859792,217.182200713788,
217.264661246887,217.347121465937,217.429581377788,217.512040989287,217.594500307284,
217.676959338626,217.759418090161,217.841876568737,217.924334781202,218.006792734402,
218.089250435185,218.171707890397,218.254165106884,218.34017769467,218.423502389086,
218.505968994645,218.588434755995,218.670899700554,218.753363855732,218.835827248939,
218.918289907582,219.000751859066,219.083213130793,219.165673750161,219.248133744568,
219.330593141409,219.413051968078,219.495510251964,219.577968020457,219.660425300945,
219.744559214386,219.827025212685,219.909489589234,219.991952453676,220.074413915632,
220.156874084706,220.239333070481,220.321790982524,220.407388099209,220.489852836153,
220.572314608451,220.654773854542,220.737231012721,220.81969353162,220.902151202903,
220.984609993811,221.006567916007),.UNSPECIFIED.);
#3398=B_SPLINE_CURVE_WITH_KNOTS('',3,(#201737,#201738,#201739,#201740,#201741,
#201742,#201743,#201744,#201745,#201746,#201747,#201748,#201749,#201750,
#201751,#201752,#201753,#201754,#201755,#201756,#201757,#201758,#201759,
#201760,#201761,#201762,#201763,#201764,#201765,#201766,#201767,#201768,
#201769,#201770,#201771,#201772,#201773,#201774,#201775,#201776,#201777,
#201778,#201779,#201780,#201781,#201782,#201783,#201784,#201785,#201786,
#201787,#201788,#201789,#201790,#201791,#201792,#201793,#201794,#201795,
#201796,#201797,#201798,#201799,#201800,#201801,#201802,#201803,#201804,
#201805,#201806,#201807,#201808,#201809,#201810,#201811,#201812),
 .UNSPECIFIED.,.F.,.F.,(4,3,3,3,3,3,3,3,3,3,3,3,3,3,3,3,3,3,3,3,3,3,3,3,
3,4),(214.723382608827,214.805844212586,214.888305150465,214.970765449863,
215.053225138176,215.135684242798,215.218142791121,215.300600810535,215.383058328428,
215.469735501508,215.552202287116,215.634667400247,215.717130950554,215.799593047668,
215.8820538012,215.964513320742,216.04697171587,216.12942909614,216.21189548196,
216.294358683584,216.376819139532,216.459277288168,216.54174289218,216.624202770757,
216.706666882494,216.769893097696),.UNSPECIFIED.);
#3399=B_SPLINE_CURVE_WITH_KNOTS('',3,(#201814,#201815,#201816,#201817,#201818,
#201819,#201820,#201821,#201822,#201823,#201824,#201825,#201826,#201827,
#201828,#201829,#201830,#201831,#201832,#201833,#201834,#201835,#201836,
#201837,#201838,#201839,#201840,#201841,#201842,#201843,#201844,#201845,
#201846,#201847,#201848,#201849,#201850,#201851,#201852,#201853,#201854,
#201855,#201856,#201857,#201858,#201859,#201860,#201861,#201862,#201863,
#201864,#201865,#201866,#201867,#201868,#201869,#201870,#201871,#201872,
#201873,#201874,#201875,#201876,#201877,#201878,#201879,#201880,#201881,
#201882,#201883,#201884,#201885,#201886,#201887,#201888,#201889,#201890,
#201891,#201892),.UNSPECIFIED.,.F.,.F.,(4,3,3,3,3,3,3,3,3,3,3,3,3,3,3,3,
3,3,3,3,3,3,3,3,3,3,4),(214.723306029336,214.802635146132,214.881875088531,
214.961124965084,215.040396134553,215.119781841841,215.199161307098,215.278640892757,
215.357938963704,215.435976917764,215.513924367901,215.591794836693,215.669588534833,
215.747337684786,215.825052758298,215.857308831636,215.940275422997,216.023384773408,
216.10671977981,216.190163817788,216.273795292611,216.356678699567,216.439821239611,
216.522721408167,216.605477260346,216.688004917172,216.769893097696),
 .UNSPECIFIED.);
#3400=B_SPLINE_CURVE_WITH_KNOTS('',3,(#201893,#201894,#201895,#201896,#201897,
#201898,#201899,#201900,#201901,#201902,#201903,#201904,#201905,#201906,
#201907,#201908,#201909,#201910,#201911,#201912,#201913,#201914,#201915,
#201916,#201917,#201918,#201919,#201920,#201921,#201922,#201923,#201924,
#201925,#201926,#201927,#201928,#201929,#201930,#201931,#201932,#201933,
#201934,#201935,#201936,#201937,#201938,#201939,#201940,#201941,#201942,
#201943,#201944,#201945,#201946,#201947,#201948,#201949,#201950,#201951,
#201952,#201953,#201954,#201955,#201956,#201957,#201958,#201959,#201960,
#201961,#201962,#201963,#201964,#201965,#201966,#201967,#201968,#201969,
#201970,#201971,#201972,#201973,#201974,#201975,#201976,#201977,#201978,
#201979,#201980,#201981,#201982,#201983,#201984,#201985,#201986,#201987,
#201988,#201989,#201990,#201991,#201992,#201993,#201994,#201995,#201996,
#201997,#201998,#201999,#202000,#202001,#202002,#202003,#202004,#202005,
#202006,#202007,#202008,#202009,#202010,#202011,#202012,#202013,#202014,
#202015,#202016,#202017,#202018,#202019,#202020,#202021,#202022,#202023,
#202024,#202025,#202026,#202027,#202028,#202029,#202030,#202031,#202032,
#202033,#202034,#202035,#202036,#202037,#202038,#202039,#202040,#202041,
#202042,#202043,#202044,#202045,#202046,#202047,#202048,#202049),
 .UNSPECIFIED.,.F.,.F.,(4,3,3,3,3,3,3,3,3,3,3,3,3,3,3,3,3,3,3,3,3,3,3,3,
3,3,3,3,3,3,3,3,3,3,3,3,3,3,3,3,3,3,3,3,3,3,3,3,3,3,3,3,4),(216.769893097696,
216.852355303782,216.93481716157,217.017278677911,217.099739859655,217.182200713651,
217.26466124675,217.3471214658,217.429581377651,217.51204098915,217.594500307147,
217.676959338489,217.759418090024,217.8418765686,217.924334781065,218.006792734265,
218.089250435048,218.171707890259,218.254165106747,218.340177694536,218.423502388957,
218.505968994516,218.588434755866,218.670899700425,218.753363855603,218.83582724881,
218.918289907453,219.000751858937,219.083213130664,219.165673750032,219.248133744439,
219.330593141281,219.413051967949,219.495510251835,219.577968020329,219.660425300816,
219.744559214266,219.827025212564,219.909489589113,219.991952453555,220.074413915512,
220.156874084585,220.23933307036,220.321790982403,220.407388099104,220.489852836047,
220.572314608345,220.654773854437,220.737231012615,220.819693531514,220.902151202797,
220.984609993706,221.006567916007),.UNSPECIFIED.);
#3401=B_SPLINE_CURVE_WITH_KNOTS('',3,(#202055,#202056,#202057,#202058,#202059,
#202060,#202061,#202062,#202063,#202064,#202065,#202066,#202067,#202068,
#202069,#202070,#202071,#202072,#202073,#202074,#202075,#202076,#202077,
#202078,#202079,#202080,#202081,#202082,#202083,#202084,#202085,#202086,
#202087,#202088,#202089,#202090,#202091,#202092,#202093,#202094,#202095,
#202096,#202097,#202098,#202099,#202100,#202101,#202102,#202103,#202104,
#202105,#202106,#202107,#202108,#202109,#202110,#202111,#202112,#202113,
#202114,#202115,#202116,#202117,#202118,#202119,#202120,#202121,#202122,
#202123,#202124,#202125,#202126,#202127,#202128,#202129,#202130,#202131,
#202132,#202133,#202134,#202135,#202136,#202137,#202138,#202139,#202140,
#202141,#202142,#202143,#202144,#202145,#202146,#202147,#202148,#202149,
#202150,#202151,#202152,#202153,#202154,#202155,#202156,#202157,#202158,
#202159,#202160,#202161,#202162,#202163,#202164,#202165,#202166,#202167,
#202168,#202169,#202170,#202171,#202172,#202173,#202174,#202175,#202176,
#202177,#202178,#202179,#202180,#202181,#202182,#202183,#202184,#202185,
#202186,#202187,#202188,#202189,#202190,#202191,#202192,#202193,#202194,
#202195,#202196,#202197,#202198,#202199,#202200,#202201,#202202,#202203,
#202204,#202205,#202206,#202207,#202208,#202209,#202210,#202211),
 .UNSPECIFIED.,.F.,.F.,(4,3,3,3,3,3,3,3,3,3,3,3,3,3,3,3,3,3,3,3,3,3,3,3,
3,3,3,3,3,3,3,3,3,3,3,3,3,3,3,3,3,3,3,3,3,3,3,3,3,3,3,3,4),(223.053078404876,
223.135540610962,223.21800246875,223.300463985091,223.382925166835,223.465386020831,
223.54784655393,223.63030677298,223.712766684831,223.79522629633,223.877685614327,
223.960144645669,224.042603397204,224.125061875781,224.207520088245,224.289978041446,
224.372435742228,224.45489319744,224.537350413927,224.623363001717,224.706687696138,
224.789154301696,224.871620063047,224.954085007605,225.036549162783,225.11901255599,
225.201475214634,225.283937166118,225.366398437844,225.448859057212,225.531319051619,
225.613778448461,225.696237275129,225.778695559015,225.861153327509,225.943610607997,
226.027744521446,226.110210519744,226.192674896293,226.275137760735,226.357599222692,
226.440059391766,226.52251837754,226.604976289583,226.690573406284,226.773038143227,
226.855499915526,226.937959161617,227.020416319795,227.102878838694,227.185336509978,
227.267795300886,227.289753223187),.UNSPECIFIED.);
#3402=B_SPLINE_CURVE_WITH_KNOTS('',3,(#202212,#202213,#202214,#202215,#202216,
#202217,#202218,#202219,#202220,#202221,#202222,#202223,#202224,#202225,
#202226,#202227,#202228,#202229,#202230,#202231,#202232,#202233,#202234,
#202235,#202236,#202237,#202238,#202239,#202240,#202241,#202242,#202243,
#202244,#202245,#202246,#202247,#202248,#202249,#202250,#202251,#202252,
#202253,#202254,#202255,#202256,#202257,#202258,#202259,#202260,#202261,
#202262,#202263,#202264,#202265,#202266,#202267,#202268,#202269,#202270,
#202271,#202272,#202273,#202274,#202275,#202276,#202277,#202278,#202279,
#202280,#202281,#202282,#202283,#202284,#202285,#202286,#202287),
 .UNSPECIFIED.,.F.,.F.,(4,3,3,3,3,3,3,3,3,3,3,3,3,3,3,3,3,3,3,3,3,3,3,3,
3,4),(221.006567916007,221.089029519765,221.171490457645,221.253950757043,
221.336410445356,221.418869549978,221.501328098301,221.583786117715,221.666243635608,
221.752920808681,221.83538759429,221.917852707421,222.000316257728,222.082778354842,
222.165239108374,222.247698627916,222.330157023043,222.412614403314,222.495080789133,
222.577543990757,222.660004446706,222.742462595342,222.824928199354,222.907388077931,
222.989852189668,223.053078404776),.UNSPECIFIED.);
#3403=B_SPLINE_CURVE_WITH_KNOTS('',3,(#202289,#202290,#202291,#202292,#202293,
#202294,#202295,#202296,#202297,#202298,#202299,#202300,#202301,#202302,
#202303,#202304,#202305,#202306,#202307,#202308,#202309,#202310,#202311,
#202312,#202313,#202314,#202315,#202316,#202317,#202318,#202319,#202320,
#202321,#202322,#202323,#202324,#202325,#202326,#202327,#202328,#202329,
#202330,#202331,#202332,#202333,#202334,#202335,#202336,#202337,#202338,
#202339,#202340,#202341,#202342,#202343,#202344,#202345,#202346,#202347,
#202348,#202349,#202350,#202351,#202352,#202353,#202354,#202355,#202356,
#202357,#202358,#202359,#202360,#202361,#202362,#202363,#202364),
 .UNSPECIFIED.,.F.,.F.,(4,3,3,3,3,3,3,3,3,3,3,3,3,3,3,3,3,3,3,3,3,3,3,3,
3,4),(221.006567916007,221.089029519765,221.171490457645,221.253950757043,
221.336410445356,221.418869549978,221.501328098301,221.583786117715,221.666243635608,
221.752920808687,221.835387594296,221.917852707427,222.000316257734,222.082778354848,
222.16523910838,222.247698627922,222.330157023049,222.41261440332,222.49508078914,
222.577543990764,222.660004446712,222.742462595349,222.82492819936,222.907388077938,
222.989852189674,223.053078404876),.UNSPECIFIED.);
#3404=B_SPLINE_CURVE_WITH_KNOTS('',3,(#202365,#202366,#202367,#202368,#202369,
#202370,#202371,#202372,#202373,#202374,#202375,#202376,#202377,#202378,
#202379,#202380,#202381,#202382,#202383,#202384,#202385,#202386,#202387,
#202388,#202389,#202390,#202391,#202392,#202393,#202394,#202395,#202396,
#202397,#202398,#202399,#202400,#202401,#202402,#202403,#202404,#202405,
#202406,#202407,#202408,#202409,#202410,#202411,#202412,#202413,#202414,
#202415,#202416,#202417,#202418,#202419,#202420,#202421,#202422,#202423,
#202424,#202425,#202426,#202427,#202428,#202429,#202430,#202431,#202432,
#202433,#202434,#202435,#202436,#202437,#202438,#202439,#202440,#202441,
#202442,#202443,#202444,#202445,#202446,#202447,#202448,#202449,#202450,
#202451,#202452,#202453,#202454,#202455,#202456,#202457,#202458,#202459,
#202460,#202461,#202462,#202463,#202464,#202465,#202466,#202467,#202468,
#202469,#202470,#202471,#202472,#202473,#202474,#202475,#202476,#202477,
#202478,#202479,#202480,#202481,#202482,#202483,#202484,#202485,#202486,
#202487,#202488,#202489,#202490,#202491,#202492,#202493,#202494,#202495,
#202496,#202497,#202498,#202499,#202500,#202501,#202502,#202503,#202504,
#202505,#202506,#202507,#202508,#202509,#202510,#202511,#202512,#202513,
#202514,#202515,#202516,#202517,#202518,#202519,#202520,#202521,#202522,
#202523,#202524,#202525,#202526,#202527,#202528,#202529,#202530,#202531,
#202532,#202533),.UNSPECIFIED.,.F.,.F.,(4,3,3,3,3,3,3,3,3,3,3,3,3,3,3,3,
3,3,3,3,3,3,3,3,3,3,3,3,3,3,3,3,3,3,3,3,3,3,3,3,3,3,3,3,3,3,3,3,3,3,3,3,
3,3,3,3,4),(223.053078404876,223.146044225602,223.239870824975,223.334650264296,
223.347856850602,223.425228790324,223.50250728684,223.57970819008,223.656847293021,
223.733940343337,223.811010726514,223.88807060416,223.965134183421,224.042215670963,
224.11937156828,224.196565293471,224.27386814163,224.346596586464,224.430258111719,
224.513792070736,224.597126498715,224.680337882208,224.763350731037,224.845966454395,
224.923687048301,225.001432708213,225.079216808168,225.157095805485,225.235029123069,
225.313073998632,225.345336322326,225.424826154287,225.504240563609,225.583592175005,
225.662893565209,225.742157272041,225.821401806291,225.900636566179,225.97987290514,
226.059122176085,226.138425714033,226.217757875254,226.297165193625,226.344076058189,
226.420902169192,226.497660888859,226.574366832784,226.651035335283,226.727681881201,
226.804331550368,226.84344592612,226.928048974059,227.012797780636,227.097735349666,
227.182762072976,227.267898039824,227.289635416186),.UNSPECIFIED.);
#3405=B_SPLINE_CURVE_WITH_KNOTS('',3,(#202539,#202540,#202541,#202542,#202543,
#202544,#202545,#202546,#202547,#202548,#202549,#202550,#202551,#202552,
#202553,#202554,#202555,#202556,#202557,#202558,#202559,#202560,#202561,
#202562,#202563,#202564,#202565,#202566,#202567,#202568,#202569,#202570,
#202571,#202572,#202573,#202574,#202575,#202576,#202577,#202578,#202579,
#202580,#202581,#202582,#202583,#202584,#202585,#202586,#202587,#202588,
#202589,#202590,#202591,#202592,#202593,#202594,#202595,#202596,#202597,
#202598,#202599,#202600,#202601,#202602,#202603,#202604,#202605,#202606,
#202607,#202608,#202609,#202610,#202611,#202612,#202613,#202614,#202615,
#202616,#202617,#202618,#202619,#202620,#202621,#202622,#202623,#202624,
#202625,#202626,#202627,#202628,#202629,#202630,#202631,#202632,#202633,
#202634,#202635,#202636,#202637,#202638,#202639,#202640,#202641,#202642,
#202643,#202644,#202645,#202646,#202647,#202648,#202649,#202650,#202651,
#202652,#202653,#202654,#202655,#202656,#202657,#202658,#202659,#202660,
#202661,#202662,#202663,#202664,#202665,#202666,#202667,#202668,#202669,
#202670,#202671,#202672,#202673,#202674,#202675,#202676,#202677,#202678,
#202679,#202680,#202681,#202682,#202683,#202684,#202685,#202686,#202687,
#202688,#202689,#202690,#202691,#202692,#202693,#202694,#202695),
 .UNSPECIFIED.,.F.,.F.,(4,3,3,3,3,3,3,3,3,3,3,3,3,3,3,3,3,3,3,3,3,3,3,3,
3,3,3,3,3,3,3,3,3,3,3,3,3,3,3,3,3,3,3,3,3,3,3,3,3,3,3,3,4),(229.336263712056,
229.418725918142,229.50118777593,229.583649292271,229.666110474015,229.748571328011,
229.83103186111,229.91349208016,229.995951992011,230.07841160351,230.160870921507,
230.243329952849,230.325788704384,230.40824718296,230.490705395425,230.573163348626,
230.655621049408,230.73807850462,230.820535721107,230.906548308897,230.989873003318,
231.072339608876,231.154805370227,231.237270314785,231.319734469963,231.40219786317,
231.484660521814,231.567122473298,231.649583745024,231.732044364392,231.814504358799,
231.896963755641,231.979422582309,232.061880866195,232.144338634689,232.226795915176,
232.310929828626,232.393395826924,232.475860203473,232.558323067915,232.640784529872,
232.723244698946,232.80570368472,232.888161596763,232.973758713464,233.056223450407,
233.138685222705,233.221144468796,233.303601626975,233.386064145874,233.468521817157,
233.550980608065,233.572938530366),.UNSPECIFIED.);
#3406=B_SPLINE_CURVE_WITH_KNOTS('',3,(#202696,#202697,#202698,#202699,#202700,
#202701,#202702,#202703,#202704,#202705,#202706,#202707,#202708,#202709,
#202710,#202711,#202712,#202713,#202714,#202715,#202716,#202717,#202718,
#202719,#202720,#202721,#202722,#202723,#202724,#202725,#202726,#202727,
#202728,#202729,#202730,#202731,#202732,#202733,#202734,#202735,#202736,
#202737,#202738,#202739,#202740,#202741,#202742,#202743,#202744,#202745,
#202746,#202747,#202748,#202749,#202750,#202751,#202752,#202753,#202754,
#202755,#202756,#202757,#202758,#202759,#202760,#202761,#202762,#202763,
#202764,#202765,#202766,#202767,#202768,#202769,#202770,#202771),
 .UNSPECIFIED.,.F.,.F.,(4,3,3,3,3,3,3,3,3,3,3,3,3,3,3,3,3,3,3,3,3,3,3,3,
3,4),(227.289753223187,227.372214826945,227.454675764825,227.537136064223,
227.619595752536,227.702054857158,227.784513405481,227.866971424895,227.949428942788,
228.036106115859,228.118572901467,228.201038014598,228.283501564905,228.365963662019,
228.448424415551,228.530883935093,228.61334233022,228.695799710491,228.778266096311,
228.860729297935,228.943189753883,229.025647902519,229.108113506531,229.190573385109,
229.273037496845,229.336263711915),.UNSPECIFIED.);
#3407=B_SPLINE_CURVE_WITH_KNOTS('',3,(#202773,#202774,#202775,#202776,#202777,
#202778,#202779,#202780,#202781,#202782,#202783,#202784,#202785,#202786,
#202787,#202788,#202789,#202790,#202791,#202792,#202793,#202794,#202795,
#202796,#202797,#202798,#202799,#202800,#202801,#202802,#202803,#202804,
#202805,#202806,#202807,#202808,#202809,#202810,#202811,#202812,#202813,
#202814,#202815,#202816,#202817,#202818,#202819,#202820,#202821,#202822,
#202823,#202824,#202825,#202826,#202827,#202828,#202829,#202830,#202831,
#202832,#202833,#202834,#202835,#202836,#202837,#202838,#202839,#202840,
#202841,#202842,#202843,#202844,#202845,#202846,#202847,#202848,#202849,
#202850,#202851,#202852,#202853,#202854),.UNSPECIFIED.,.F.,.F.,(4,3,3,3,
3,3,3,3,3,3,3,3,3,3,3,3,3,3,3,3,3,3,3,3,3,3,3,4),(227.289635416186,227.342815794051,
227.424363071555,227.505834823778,227.589922533329,227.671238744506,227.756712203244,
227.842185661982,227.92160317053,228.001039463831,228.0805052851,228.160044679029,
228.239626033312,228.319291542762,228.341555529913,228.419862015423,228.498101914488,
228.576289748601,228.654440001667,228.732567129521,228.810702261164,228.888845478722,
228.967009877278,229.045208561738,229.123500253565,229.201842044087,229.280300540696,
229.336263712055),.UNSPECIFIED.);
#3408=B_SPLINE_CURVE_WITH_KNOTS('',3,(#202855,#202856,#202857,#202858,#202859,
#202860,#202861,#202862,#202863,#202864,#202865,#202866,#202867,#202868,
#202869,#202870,#202871,#202872,#202873,#202874,#202875,#202876,#202877,
#202878,#202879,#202880,#202881,#202882,#202883,#202884,#202885,#202886,
#202887,#202888,#202889,#202890,#202891,#202892,#202893,#202894,#202895,
#202896,#202897,#202898,#202899,#202900,#202901,#202902,#202903,#202904,
#202905,#202906,#202907,#202908,#202909,#202910,#202911,#202912,#202913,
#202914,#202915,#202916,#202917,#202918,#202919,#202920,#202921,#202922,
#202923,#202924,#202925,#202926,#202927,#202928,#202929,#202930,#202931,
#202932,#202933,#202934,#202935,#202936,#202937,#202938,#202939,#202940,
#202941,#202942,#202943,#202944,#202945,#202946,#202947,#202948,#202949,
#202950,#202951,#202952,#202953,#202954,#202955,#202956,#202957,#202958,
#202959,#202960,#202961,#202962,#202963,#202964,#202965,#202966,#202967,
#202968,#202969,#202970,#202971,#202972,#202973,#202974,#202975,#202976,
#202977,#202978,#202979,#202980,#202981,#202982,#202983,#202984,#202985,
#202986,#202987,#202988,#202989,#202990,#202991,#202992,#202993,#202994,
#202995,#202996,#202997,#202998,#202999,#203000,#203001,#203002,#203003,
#203004,#203005,#203006,#203007,#203008,#203009,#203010,#203011,#203012,
#203013,#203014,#203015,#203016,#203017,#203018,#203019,#203020,#203021,
#203022,#203023,#203024,#203025,#203026,#203027,#203028,#203029),
 .UNSPECIFIED.,.F.,.F.,(4,3,3,3,3,3,3,3,3,3,3,3,3,3,3,3,3,3,3,3,3,3,3,3,
3,3,3,3,3,3,3,3,3,3,3,3,3,3,3,3,3,3,3,3,3,3,3,3,3,3,3,3,3,3,3,3,3,3,4),
(229.336263712185,229.340295265775,229.416353221658,229.492315499975,229.568198891192,
229.644020104713,229.719795787656,229.797200689403,229.872949950271,229.948706465713,
230.024485245331,230.103122684408,230.179033385957,230.255000894413,230.331074602357,
230.339035001637,230.416594219665,230.494061133937,230.571451411116,230.648780662822,
230.726064456727,230.803325886015,230.880576971315,230.957831759866,231.035104298339,
231.112450023129,231.189833183896,231.267323063712,231.337774737499,231.421991210269,
231.506081087413,231.589964966738,231.673719256124,231.757258365679,231.837144605431,
231.914513048451,231.991899904669,232.069318971392,232.14682519985,232.224381119235,
232.302043799002,232.336514473362,232.416134948255,232.4956825069,232.575169462654,
232.654608082181,232.73401059438,232.813395523447,232.892771468578,232.972149511684,
233.051540734651,233.130985683765,233.210458979456,233.290005809806,233.335254209224,
233.411970858466,233.492647251187,233.569241113093,233.573323643909),
 .UNSPECIFIED.);
#3409=B_SPLINE_CURVE_WITH_KNOTS('',3,(#203035,#203036,#203037,#203038,#203039,
#203040,#203041,#203042,#203043,#203044,#203045,#203046,#203047,#203048,
#203049,#203050,#203051,#203052,#203053,#203054,#203055,#203056,#203057,
#203058,#203059,#203060,#203061,#203062,#203063,#203064,#203065,#203066,
#203067,#203068,#203069,#203070,#203071,#203072,#203073,#203074,#203075,
#203076,#203077,#203078,#203079,#203080,#203081,#203082,#203083,#203084,
#203085,#203086,#203087,#203088,#203089,#203090,#203091,#203092,#203093,
#203094,#203095,#203096,#203097,#203098,#203099,#203100,#203101,#203102,
#203103,#203104,#203105,#203106,#203107,#203108,#203109,#203110,#203111,
#203112,#203113,#203114,#203115,#203116,#203117,#203118,#203119,#203120,
#203121,#203122,#203123,#203124,#203125,#203126,#203127,#203128,#203129,
#203130,#203131,#203132,#203133,#203134,#203135,#203136,#203137,#203138,
#203139,#203140,#203141,#203142,#203143,#203144,#203145,#203146,#203147,
#203148,#203149,#203150,#203151,#203152,#203153,#203154,#203155,#203156,
#203157,#203158,#203159,#203160,#203161,#203162,#203163,#203164,#203165,
#203166,#203167,#203168,#203169,#203170,#203171,#203172,#203173,#203174,
#203175,#203176,#203177,#203178,#203179,#203180,#203181,#203182,#203183,
#203184,#203185,#203186,#203187,#203188,#203189,#203190,#203191,#203192,
#203193,#203194,#203195,#203196,#203197,#203198,#203199,#203200),
 .UNSPECIFIED.,.F.,.F.,(4,3,3,3,3,3,3,3,3,3,3,3,3,3,3,3,3,3,3,3,3,3,3,3,
3,3,3,3,3,3,3,3,3,3,3,3,3,3,3,3,3,3,3,3,3,3,3,3,3,3,3,3,3,3,3,4),(235.619449019235,
235.699335060132,235.779370913976,235.859484258981,235.939758663195,236.013789031205,
236.093409769729,236.172957597161,236.252444826208,236.33188372289,236.411286515463,
236.490671728125,236.57004795844,236.649426287752,236.728817797384,236.808263031978,
236.887736612522,236.967283724338,237.012528767067,237.089243773325,237.165891685097,
237.242487196245,237.319046093354,237.395583476844,237.47212499671,237.511898634998,
237.596574974064,237.681397459474,237.766419831286,237.851528714047,237.936758254381,
238.011268502929,238.092824765124,238.174305704323,238.258388870958,238.339714623005,
238.425176496933,238.51063837086,238.590041711906,238.669463483232,238.74891446104,
238.82843862743,238.908004538146,238.987654386521,239.010008238791,239.088392843705,
239.166709649306,239.244973074348,239.323198686606,239.401404021146,239.479602079275,
239.55780585563,239.636059705318,239.714338858029,239.792698452621,239.855869977774),
 .UNSPECIFIED.);
#3410=B_SPLINE_CURVE_WITH_KNOTS('',3,(#203201,#203202,#203203,#203204,#203205,
#203206,#203207,#203208,#203209,#203210,#203211,#203212,#203213,#203214,
#203215,#203216,#203217,#203218,#203219,#203220,#203221,#203222,#203223,
#203224,#203225,#203226,#203227,#203228,#203229,#203230,#203231,#203232,
#203233,#203234,#203235,#203236,#203237,#203238,#203239,#203240,#203241,
#203242,#203243,#203244,#203245,#203246,#203247,#203248,#203249,#203250,
#203251,#203252,#203253,#203254,#203255,#203256,#203257,#203258,#203259,
#203260,#203261,#203262,#203263,#203264,#203265,#203266,#203267,#203268,
#203269,#203270,#203271,#203272,#203273,#203274,#203275,#203276),
 .UNSPECIFIED.,.F.,.F.,(4,3,3,3,3,3,3,3,3,3,3,3,3,3,3,3,3,3,3,3,3,3,3,3,
3,4),(233.572938530366,233.655400134125,233.737861072004,233.820321371402,
233.902781059715,233.985240164337,234.06769871266,234.150156732074,234.232614249967,
234.319291423047,234.401758208655,234.484223321786,234.566686872093,234.649148969207,
234.731609722739,234.814069242281,234.896527637408,234.978985017679,235.061451403499,
235.143914605123,235.226375061071,235.308833209708,235.391298813719,235.473758692297,
235.556222804033,235.619449019235),.UNSPECIFIED.);
#3411=B_SPLINE_CURVE_WITH_KNOTS('',3,(#203278,#203279,#203280,#203281,#203282,
#203283,#203284,#203285,#203286,#203287,#203288,#203289,#203290,#203291,
#203292,#203293,#203294,#203295,#203296,#203297,#203298,#203299,#203300,
#203301,#203302,#203303,#203304,#203305,#203306,#203307,#203308,#203309,
#203310,#203311,#203312,#203313,#203314,#203315,#203316,#203317,#203318,
#203319,#203320,#203321,#203322,#203323,#203324,#203325,#203326,#203327,
#203328,#203329,#203330,#203331,#203332,#203333,#203334,#203335,#203336,
#203337,#203338,#203339,#203340,#203341,#203342,#203343,#203344,#203345,
#203346,#203347,#203348,#203349,#203350,#203351,#203352,#203353,#203354,
#203355,#203356,#203357,#203358,#203359),.UNSPECIFIED.,.F.,.F.,(4,3,3,3,
3,3,3,3,3,3,3,3,3,3,3,3,3,3,3,3,3,3,3,3,3,3,3,4),(233.573323643909,233.649879644271,
233.726415517639,233.802955814209,233.834624077155,233.919300567095,234.004123210958,
234.08914574956,234.174254802649,234.259484515824,234.333993945086,234.415550063061,
234.497030857161,234.581114096125,234.662439703222,234.74790175812,234.833363813017,
234.912767221105,234.992189060828,235.071640108233,235.15116434557,235.230730327984,
235.310380248706,235.332733680948,235.424797298135,235.516554834754,235.607711152124,
235.619449019114),.UNSPECIFIED.);
#3412=B_SPLINE_CURVE_WITH_KNOTS('',3,(#203360,#203361,#203362,#203363,#203364,
#203365,#203366,#203367,#203368,#203369,#203370,#203371,#203372,#203373,
#203374,#203375,#203376,#203377,#203378,#203379,#203380,#203381,#203382,
#203383,#203384,#203385,#203386,#203387,#203388,#203389,#203390,#203391,
#203392,#203393,#203394,#203395,#203396,#203397,#203398,#203399,#203400,
#203401,#203402,#203403,#203404,#203405,#203406,#203407,#203408,#203409,
#203410,#203411,#203412,#203413,#203414,#203415,#203416,#203417,#203418,
#203419,#203420,#203421,#203422,#203423,#203424,#203425,#203426,#203427,
#203428,#203429,#203430,#203431,#203432,#203433,#203434,#203435,#203436,
#203437,#203438,#203439,#203440,#203441,#203442,#203443,#203444,#203445,
#203446,#203447,#203448,#203449,#203450,#203451,#203452,#203453,#203454,
#203455,#203456,#203457,#203458,#203459,#203460,#203461,#203462,#203463,
#203464,#203465,#203466,#203467,#203468,#203469,#203470,#203471,#203472,
#203473,#203474,#203475,#203476,#203477,#203478,#203479,#203480,#203481,
#203482,#203483,#203484,#203485,#203486,#203487,#203488,#203489,#203490,
#203491,#203492,#203493,#203494,#203495,#203496,#203497,#203498,#203499,
#203500,#203501,#203502,#203503,#203504,#203505,#203506,#203507,#203508,
#203509,#203510,#203511,#203512,#203513,#203514,#203515,#203516,#203517,
#203518,#203519,#203520,#203521,#203522,#203523,#203524,#203525,#203526,
#203527,#203528),.UNSPECIFIED.,.F.,.F.,(4,3,3,3,3,3,3,3,3,3,3,3,3,3,3,3,
3,3,3,3,3,3,3,3,3,3,3,3,3,3,3,3,3,3,3,3,3,3,3,3,3,3,3,3,3,3,3,3,3,3,3,3,
3,3,3,3,4),(235.619449019235,235.697894778131,235.777092107966,235.855561918656,
235.934054701829,236.012583029286,236.092305626167,236.170984086526,236.251228751668,
236.33147341681,236.407529924543,236.483490743517,236.559372665115,236.635192399599,
236.710966594905,236.788372414626,236.864120171709,236.9398751782,237.01565244439,
237.09429262146,237.170201808871,237.24616780175,237.322240000284,237.330213152673,
237.407772006574,237.485238552846,237.562628458535,237.639957335639,237.717240752206,
237.794501801216,237.871752504505,237.949006909641,238.026279063626,238.10362440421,
238.18100718038,238.258496678449,238.328952888535,238.41317216454,238.497264836661,
238.581151455782,238.664908438605,238.748450134982,238.828322756466,238.905689954775,
238.983075546777,239.060493331147,239.13799825538,239.215552857275,239.29321420689,
239.327692624397,239.407311064205,239.486859579851,239.566349380978,239.645784629109,
239.725186637447,239.804569105013,239.856287383305),.UNSPECIFIED.);
#3413=B_SPLINE_CURVE_WITH_KNOTS('',3,(#203534,#203535,#203536,#203537,#203538,
#203539,#203540,#203541,#203542,#203543,#203544,#203545,#203546,#203547,
#203548,#203549,#203550,#203551,#203552,#203553,#203554,#203555,#203556,
#203557,#203558,#203559,#203560,#203561,#203562,#203563,#203564,#203565,
#203566,#203567,#203568,#203569,#203570,#203571,#203572,#203573,#203574,
#203575,#203576,#203577,#203578,#203579,#203580,#203581,#203582,#203583,
#203584,#203585,#203586,#203587,#203588,#203589,#203590,#203591,#203592,
#203593,#203594,#203595,#203596,#203597,#203598,#203599,#203600,#203601,
#203602,#203603,#203604,#203605,#203606,#203607,#203608,#203609,#203610,
#203611,#203612,#203613,#203614,#203615,#203616,#203617,#203618,#203619,
#203620,#203621,#203622,#203623,#203624,#203625,#203626,#203627,#203628,
#203629,#203630,#203631,#203632,#203633,#203634,#203635,#203636,#203637,
#203638,#203639,#203640,#203641,#203642,#203643,#203644,#203645,#203646,
#203647,#203648,#203649,#203650,#203651,#203652,#203653,#203654,#203655,
#203656,#203657,#203658,#203659,#203660,#203661,#203662,#203663,#203664,
#203665,#203666,#203667,#203668,#203669,#203670,#203671,#203672,#203673,
#203674,#203675,#203676,#203677,#203678,#203679,#203680,#203681,#203682,
#203683,#203684,#203685,#203686,#203687,#203688,#203689,#203690,#203691,
#203692,#203693,#203694,#203695,#203696,#203697,#203698,#203699),
 .UNSPECIFIED.,.F.,.F.,(4,3,3,3,3,3,3,3,3,3,3,3,3,3,3,3,3,3,3,3,3,3,3,3,
3,3,3,3,3,3,3,3,3,3,3,3,3,3,3,3,3,3,3,3,3,3,3,3,3,3,3,3,3,3,3,4),(241.902634326415,
242.006227446378,242.090446729262,242.174539408226,242.258426034031,242.342183023408,
242.425724726058,242.505597314309,242.582964510105,242.660350099558,242.737767881348,
242.815272802963,242.892827402217,242.970488749172,243.00496718224,243.084587920985,
243.164135748642,243.243622977918,243.323061874832,243.402464667639,243.481849880538,
243.561226111091,243.640604440643,243.719995950514,243.799441185346,243.878914766127,
243.958461878178,244.003706918102,244.080421924948,244.15706983731,244.233665349047,
244.310224246743,244.38676163082,244.46330315127,244.503076786033,244.587753124243,
244.67257560876,244.757597979638,244.84270686145,244.927936400827,245.002446653964,
245.084002916623,245.165483856288,245.24956702269,245.330892775201,245.416354648549,
245.501816521896,245.581219862781,245.660641633943,245.740092611585,245.819616777805,
245.899182688351,245.978832536554,246.001186389827,246.079561984822,246.139559773273),
 .UNSPECIFIED.);
#3414=B_SPLINE_CURVE_WITH_KNOTS('',3,(#203700,#203701,#203702,#203703,#203704,
#203705,#203706,#203707,#203708,#203709,#203710,#203711,#203712,#203713,
#203714,#203715,#203716,#203717,#203718,#203719,#203720,#203721,#203722,
#203723,#203724,#203725,#203726,#203727,#203728,#203729,#203730,#203731,
#203732,#203733,#203734,#203735,#203736,#203737,#203738,#203739,#203740,
#203741,#203742,#203743,#203744,#203745,#203746,#203747,#203748,#203749,
#203750,#203751,#203752,#203753,#203754,#203755,#203756,#203757,#203758,
#203759,#203760,#203761,#203762,#203763,#203764,#203765,#203766,#203767,
#203768,#203769,#203770,#203771,#203772,#203773,#203774,#203775,#203776,
#203777,#203778,#203779,#203780,#203781,#203782,#203783,#203784),
 .UNSPECIFIED.,.F.,.F.,(4,3,3,3,3,3,3,3,3,3,3,3,3,3,3,3,3,3,3,3,3,3,3,3,
3,3,3,3,4),(239.855869977774,239.934394266809,240.008747974654,240.084804481403,
240.160765299393,240.236647220008,240.31246695351,240.388241147837,240.465646968172,
240.541394724282,240.617149729805,240.692926995031,240.771567173902,240.847476360366,
240.923442352304,240.999514549909,241.007487710516,241.084375069617,241.161170469761,
241.23789018103,241.314550412522,241.391167984801,241.467763329302,241.5443510339,
241.620945679481,241.697594875386,241.774273250137,241.851037515127,241.902634326295),
 .UNSPECIFIED.);
#3415=B_SPLINE_CURVE_WITH_KNOTS('',3,(#203786,#203787,#203788,#203789,#203790,
#203791,#203792,#203793,#203794,#203795,#203796,#203797,#203798,#203799,
#203800,#203801,#203802,#203803,#203804,#203805,#203806,#203807,#203808,
#203809,#203810,#203811,#203812,#203813,#203814,#203815,#203816,#203817,
#203818,#203819,#203820,#203821,#203822,#203823,#203824,#203825,#203826,
#203827,#203828,#203829,#203830,#203831,#203832,#203833,#203834,#203835,
#203836,#203837,#203838,#203839,#203840,#203841,#203842,#203843,#203844,
#203845,#203846,#203847,#203848,#203849,#203850,#203851,#203852,#203853,
#203854,#203855,#203856,#203857,#203858,#203859,#203860,#203861,#203862,
#203863,#203864),.UNSPECIFIED.,.F.,.F.,(4,3,3,3,3,3,3,3,3,3,3,3,3,3,3,3,
3,3,3,3,3,3,3,3,3,3,4),(239.856287383305,239.935663723181,240.015049380833,
240.094487130204,240.173949680295,240.25349100907,240.326432360259,240.403147366517,
240.479795278289,240.556390789437,240.632949686546,240.709487070035,240.786028589902,
240.82580222819,240.910478567256,240.995301052666,241.080323424478,241.165432307238,
241.250661847573,241.325172096121,241.406728358316,241.488209297516,241.57229246415,
241.653618216198,241.739080090125,241.824541964052,241.902634326414),
 .UNSPECIFIED.);
#3416=B_SPLINE_CURVE_WITH_KNOTS('',3,(#203865,#203866,#203867,#203868,#203869,
#203870,#203871,#203872,#203873,#203874,#203875,#203876,#203877,#203878,
#203879,#203880,#203881,#203882,#203883,#203884,#203885,#203886,#203887,
#203888,#203889,#203890,#203891,#203892,#203893,#203894,#203895,#203896,
#203897,#203898,#203899,#203900,#203901,#203902,#203903,#203904,#203905,
#203906,#203907,#203908,#203909,#203910,#203911,#203912,#203913,#203914,
#203915,#203916,#203917,#203918,#203919,#203920,#203921,#203922,#203923,
#203924,#203925,#203926,#203927,#203928,#203929,#203930,#203931,#203932,
#203933,#203934,#203935,#203936,#203937,#203938,#203939,#203940,#203941,
#203942,#203943,#203944,#203945,#203946,#203947,#203948,#203949,#203950,
#203951,#203952,#203953,#203954,#203955,#203956,#203957,#203958,#203959,
#203960,#203961,#203962,#203963,#203964,#203965,#203966,#203967,#203968,
#203969,#203970,#203971,#203972,#203973,#203974,#203975,#203976,#203977,
#203978,#203979,#203980,#203981,#203982,#203983,#203984,#203985,#203986,
#203987,#203988,#203989,#203990,#203991,#203992,#203993,#203994,#203995,
#203996,#203997,#203998,#203999,#204000,#204001,#204002,#204003,#204004,
#204005,#204006,#204007,#204008,#204009,#204010,#204011,#204012,#204013,
#204014,#204015,#204016,#204017,#204018,#204019,#204020,#204021,#204022,
#204023,#204024,#204025,#204026,#204027,#204028,#204029,#204030,#204031,
#204032,#204033),.UNSPECIFIED.,.F.,.F.,(4,3,3,3,3,3,3,3,3,3,3,3,3,3,3,3,
3,3,3,3,3,3,3,3,3,3,3,3,3,3,3,3,3,3,3,3,3,3,3,3,3,3,3,3,3,3,3,3,3,3,3,3,
3,3,3,3,4),(241.902634326536,241.983440650617,242.064301316456,242.145262351786,
242.226279264729,242.307391413021,242.323911831983,242.402290852836,242.480603604135,
242.558864500272,242.637087918053,242.715288206196,242.793496395342,242.871712448815,
242.949949366026,243.028220156162,243.106583735617,243.184996865057,243.263527247552,
243.322651567846,243.398708074595,243.474668892585,243.5505508132,243.626370546702,
243.702144741029,243.779550561364,243.855298317474,243.931053322997,244.006830588223,
244.085470767094,244.161379953558,244.237345945495,244.313418143101,244.321391303708,
244.39895015526,244.476416699161,244.55380660246,244.63113547716,244.708418891309,
244.785679937888,244.862930638738,244.94018504143,245.017457192969,245.094802531113,
245.172185304844,245.249674800498,245.32013103957,245.404350322454,245.488443001418,
245.572329627223,245.656086616601,245.739628319251,245.819500907501,245.899271539307,
245.976664252389,246.057623843556,246.138583434724),.UNSPECIFIED.);
#3417=B_SPLINE_CURVE_WITH_KNOTS('',3,(#204039,#204040,#204041,#204042,#204043,
#204044,#204045,#204046,#204047,#204048,#204049,#204050,#204051,#204052,
#204053,#204054,#204055,#204056,#204057,#204058,#204059,#204060,#204061,
#204062,#204063,#204064,#204065,#204066,#204067,#204068,#204069,#204070,
#204071,#204072,#204073,#204074,#204075,#204076,#204077,#204078,#204079,
#204080,#204081,#204082,#204083,#204084,#204085,#204086,#204087,#204088,
#204089,#204090,#204091,#204092,#204093,#204094,#204095,#204096,#204097,
#204098,#204099,#204100,#204101,#204102,#204103,#204104,#204105,#204106,
#204107,#204108,#204109,#204110,#204111,#204112,#204113,#204114,#204115,
#204116,#204117,#204118,#204119,#204120,#204121,#204122,#204123,#204124,
#204125,#204126,#204127,#204128,#204129,#204130,#204131,#204132,#204133,
#204134,#204135,#204136,#204137,#204138,#204139,#204140,#204141,#204142,
#204143,#204144,#204145,#204146,#204147,#204148,#204149,#204150,#204151,
#204152,#204153,#204154,#204155,#204156,#204157,#204158,#204159,#204160,
#204161,#204162,#204163,#204164,#204165,#204166,#204167,#204168,#204169,
#204170,#204171,#204172,#204173,#204174,#204175,#204176,#204177,#204178,
#204179,#204180,#204181,#204182,#204183,#204184,#204185,#204186,#204187,
#204188,#204189,#204190,#204191,#204192,#204193,#204194,#204195,#204196,
#204197,#204198,#204199,#204200,#204201,#204202,#204203,#204204,#204205,
#204206,#204207),.UNSPECIFIED.,.F.,.F.,(4,3,3,3,3,3,3,3,3,3,3,3,3,3,3,3,
3,3,3,3,3,3,3,3,3,3,3,3,3,3,3,3,3,3,3,3,3,3,3,3,3,3,3,3,3,3,3,3,3,3,3,3,
3,3,3,3,4),(248.185819633708,248.261585952686,248.337281052035,248.412921758733,
248.488529494103,248.564121002797,248.639711417477,248.715315869224,248.790988245108,
248.866696742503,248.942505670427,248.997405597413,249.081624880306,249.165717559279,
249.249604185092,249.333361174478,249.416902877136,249.496775465344,249.574142661138,
249.651528250589,249.728946032378,249.806450953991,249.884005553243,249.961666900196,
249.996145333275,250.075766072019,250.155313899675,250.234801128951,250.314240025864,
250.39364281867,250.473028031569,250.552404262121,250.631782591672,250.711174101543,
250.790619336374,250.870092917155,250.949640029205,250.994885069138,251.071600075987,
251.148247988351,251.224843500091,251.301402397789,251.377939781868,251.454481302321,
251.494254937069,251.578931275277,251.66375375979,251.748776130666,251.833885012474,
251.919114551848,251.993624805,252.075187818711,252.15667533995,252.238070811612,
252.319408121063,252.400678092138,252.422853579701),.UNSPECIFIED.);
#3418=B_SPLINE_CURVE_WITH_KNOTS('',3,(#204208,#204209,#204210,#204211,#204212,
#204213,#204214,#204215,#204216,#204217,#204218,#204219,#204220,#204221,
#204222,#204223,#204224,#204225,#204226,#204227,#204228,#204229,#204230,
#204231,#204232,#204233,#204234,#204235,#204236,#204237,#204238,#204239,
#204240,#204241,#204242,#204243,#204244,#204245,#204246,#204247,#204248,
#204249,#204250,#204251,#204252,#204253,#204254,#204255,#204256,#204257,
#204258,#204259,#204260,#204261,#204262,#204263,#204264,#204265,#204266,
#204267,#204268,#204269,#204270,#204271,#204272,#204273,#204274,#204275,
#204276,#204277,#204278,#204279,#204280,#204281,#204282,#204283,#204284,
#204285,#204286,#204287,#204288,#204289),.UNSPECIFIED.,.F.,.F.,(4,3,3,3,
3,3,3,3,3,3,3,3,3,3,3,3,3,3,3,3,3,3,3,3,3,3,3,4),(246.139559773273,246.217831512834,
246.296062413031,246.374266828305,246.452475053539,246.53068810268,246.608918973935,
246.687180673534,246.76553436775,246.843934857852,246.922457968968,246.999926125689,
247.075982632443,247.151943450437,247.227825371056,247.303645104563,247.379419298894,
247.456825119226,247.532572875341,247.608327880869,247.6841051461,247.762745324963,
247.838654511431,247.914620503374,247.990692700984,247.998665861551,248.133851106609,
248.185819633594),.UNSPECIFIED.);
#3419=B_SPLINE_CURVE_WITH_KNOTS('',3,(#204291,#204292,#204293,#204294,#204295,
#204296,#204297,#204298,#204299,#204300,#204301,#204302,#204303,#204304,
#204305,#204306,#204307,#204308,#204309,#204310,#204311,#204312,#204313,
#204314,#204315,#204316,#204317,#204318,#204319,#204320,#204321,#204322,
#204323,#204324,#204325,#204326,#204327,#204328,#204329,#204330,#204331,
#204332,#204333,#204334,#204335,#204336,#204337,#204338,#204339,#204340,
#204341,#204342,#204343,#204344,#204345,#204346,#204347,#204348,#204349,
#204350,#204351,#204352,#204353,#204354,#204355,#204356,#204357,#204358,
#204359,#204360,#204361,#204362,#204363,#204364,#204365,#204366,#204367,
#204368,#204369,#204370,#204371,#204372,#204373,#204374,#204375),
 .UNSPECIFIED.,.F.,.F.,(4,3,3,3,3,3,3,3,3,3,3,3,3,3,3,3,3,3,3,3,3,3,3,3,
3,3,3,3,4),(246.138583434724,246.216144908096,246.293810662186,246.318870775432,
246.398491514177,246.478039341834,246.55752657111,246.636965468024,246.716368260831,
246.79575347373,246.875129704283,246.954508033835,247.033899543706,247.113344778538,
247.192818359319,247.27236547137,247.317610511294,247.394325518141,247.470973430503,
247.547568942239,247.624127839936,247.700665224013,247.777206744463,247.816980379225,
247.899501894936,247.982178186873,248.064933619021,248.147813992888,248.185432795619),
 .UNSPECIFIED.);
#3420=B_SPLINE_CURVE_WITH_KNOTS('',3,(#204376,#204377,#204378,#204379,#204380,
#204381,#204382,#204383,#204384,#204385,#204386,#204387,#204388,#204389,
#204390,#204391,#204392,#204393,#204394,#204395,#204396,#204397,#204398,
#204399,#204400,#204401,#204402,#204403,#204404,#204405,#204406,#204407,
#204408,#204409,#204410,#204411,#204412,#204413,#204414,#204415,#204416,
#204417,#204418,#204419,#204420,#204421,#204422,#204423,#204424,#204425,
#204426,#204427,#204428,#204429,#204430,#204431,#204432,#204433,#204434,
#204435,#204436,#204437,#204438,#204439,#204440,#204441,#204442,#204443,
#204444,#204445,#204446,#204447,#204448,#204449,#204450,#204451,#204452,
#204453,#204454,#204455,#204456,#204457,#204458,#204459,#204460,#204461,
#204462,#204463,#204464,#204465,#204466,#204467,#204468,#204469,#204470,
#204471,#204472,#204473,#204474,#204475,#204476,#204477,#204478,#204479,
#204480,#204481,#204482,#204483,#204484,#204485,#204486,#204487,#204488,
#204489,#204490,#204491,#204492,#204493,#204494,#204495,#204496,#204497,
#204498,#204499,#204500,#204501,#204502,#204503,#204504,#204505,#204506,
#204507,#204508,#204509,#204510,#204511,#204512,#204513,#204514,#204515,
#204516,#204517,#204518,#204519,#204520,#204521,#204522,#204523,#204524,
#204525,#204526,#204527,#204528,#204529,#204530,#204531,#204532),
 .UNSPECIFIED.,.F.,.F.,(4,3,3,3,3,3,3,3,3,3,3,3,3,3,3,3,3,3,3,3,3,3,3,3,
3,3,3,3,3,3,3,3,3,3,3,3,3,3,3,3,3,3,3,3,3,3,3,3,3,3,3,3,4),(248.185819633594,
248.26828183968,248.350743697468,248.433205213809,248.515666395553,248.598127249549,
248.680587782648,248.763048001698,248.845507913549,248.927967525048,249.010426843045,
249.092885874387,249.175344625922,249.257803104499,249.340261316964,249.422719270164,
249.505176970946,249.587634426158,249.670091642646,249.756104230435,249.839428924856,
249.921895530414,250.004361291765,250.086826236323,250.169290391501,250.251753784709,
250.334216443352,250.416678394836,250.499139666562,250.581600285931,250.664060280338,
250.746519677179,250.828978503847,250.911436787734,250.993894556227,251.076351836715,
251.160485750164,251.242951748463,251.325416125011,251.407878989453,251.49034045141,
251.572800620484,251.655259606259,251.737717518302,251.823314635002,251.905779371946,
251.988241144244,252.070700390335,252.153157548514,252.235620067412,252.318077738696,
252.400536529604,252.422494451905),.UNSPECIFIED.);
#3421=B_SPLINE_CURVE_WITH_KNOTS('',3,(#204538,#204539,#204540,#204541,#204542,
#204543,#204544,#204545,#204546,#204547,#204548,#204549,#204550,#204551,
#204552,#204553,#204554,#204555,#204556,#204557,#204558,#204559,#204560,
#204561,#204562,#204563,#204564,#204565,#204566,#204567,#204568,#204569,
#204570,#204571,#204572,#204573,#204574,#204575,#204576,#204577,#204578,
#204579,#204580,#204581,#204582,#204583,#204584,#204585,#204586,#204587,
#204588,#204589,#204590,#204591,#204592,#204593,#204594,#204595,#204596,
#204597,#204598,#204599,#204600,#204601,#204602,#204603,#204604,#204605,
#204606,#204607,#204608,#204609,#204610,#204611,#204612,#204613,#204614,
#204615,#204616,#204617,#204618,#204619,#204620,#204621,#204622,#204623,
#204624,#204625,#204626,#204627,#204628,#204629,#204630,#204631,#204632,
#204633,#204634,#204635,#204636,#204637,#204638,#204639,#204640,#204641,
#204642,#204643,#204644,#204645,#204646,#204647,#204648,#204649,#204650,
#204651,#204652,#204653,#204654,#204655,#204656,#204657,#204658,#204659,
#204660,#204661,#204662,#204663,#204664,#204665,#204666,#204667,#204668,
#204669,#204670,#204671,#204672,#204673,#204674,#204675,#204676,#204677,
#204678,#204679,#204680,#204681,#204682,#204683,#204684,#204685,#204686,
#204687,#204688,#204689,#204690,#204691,#204692,#204693,#204694),
 .UNSPECIFIED.,.F.,.F.,(4,3,3,3,3,3,3,3,3,3,3,3,3,3,3,3,3,3,3,3,3,3,3,3,
3,3,3,3,3,3,3,3,3,3,3,3,3,3,3,3,3,3,3,3,3,3,3,3,3,3,3,3,4),(254.469004940774,
254.55146714686,254.633929004648,254.716390520989,254.798851702733,254.881312556729,
254.963773089828,255.046233308878,255.128693220729,255.211152832228,255.293612150225,
255.376071181567,255.458529933102,255.540988411679,255.623446624143,255.705904577343,
255.788362278126,255.870819733338,255.953276949825,256.039289537614,256.122614232035,
256.205080837594,256.287546598944,256.370011543503,256.452475698681,256.534939091888,
256.617401750531,256.699863702015,256.782324973742,256.86478559311,256.947245587517,
257.029704984358,257.112163811027,257.194622094913,257.277079863406,257.359537143894,
257.443671057344,257.526137055642,257.608601432191,257.691064296633,257.773525758589,
257.855985927663,257.938444913438,258.020902825481,258.106499942181,258.188964679125,
258.271426451423,258.353885697514,258.436342855693,258.518805374592,258.601263045875,
258.683721836783,258.705679759084),.UNSPECIFIED.);
#3422=B_SPLINE_CURVE_WITH_KNOTS('',3,(#204695,#204696,#204697,#204698,#204699,
#204700,#204701,#204702,#204703,#204704,#204705,#204706,#204707,#204708,
#204709,#204710,#204711,#204712,#204713,#204714,#204715,#204716,#204717,
#204718,#204719,#204720,#204721,#204722,#204723,#204724,#204725,#204726,
#204727,#204728,#204729,#204730,#204731,#204732,#204733,#204734,#204735,
#204736,#204737,#204738,#204739,#204740,#204741,#204742,#204743,#204744,
#204745,#204746,#204747,#204748,#204749,#204750,#204751,#204752,#204753,
#204754,#204755,#204756,#204757,#204758,#204759,#204760,#204761,#204762,
#204763,#204764,#204765,#204766,#204767,#204768,#204769,#204770,#204771,
#204772,#204773,#204774,#204775,#204776),.UNSPECIFIED.,.F.,.F.,(4,3,3,3,
3,3,3,3,3,3,3,3,3,3,3,3,3,3,3,3,3,3,3,3,3,3,3,4),(252.422853579701,252.492994672931,
252.572398013815,252.651819784978,252.731270762618,252.810794928837,252.890360839383,
252.970010687586,252.992364540862,253.070743561732,253.149056313048,253.227317209201,
253.305540627,253.38374091516,253.461949104325,253.540165157816,253.618402075045,
253.696672865199,253.775036444672,253.853449574132,253.931979956645,253.991104276724,
254.07139109245,254.151529610741,254.231469705656,254.311296548631,254.390970577163,
254.469004940774),.UNSPECIFIED.);
#3423=B_SPLINE_CURVE_WITH_KNOTS('',3,(#204778,#204779,#204780,#204781,#204782,
#204783,#204784,#204785,#204786,#204787,#204788,#204789,#204790,#204791,
#204792,#204793,#204794,#204795,#204796,#204797,#204798,#204799,#204800,
#204801,#204802,#204803,#204804,#204805,#204806,#204807,#204808,#204809,
#204810,#204811,#204812,#204813,#204814,#204815,#204816,#204817,#204818,
#204819,#204820,#204821,#204822,#204823,#204824,#204825,#204826,#204827,
#204828,#204829,#204830,#204831,#204832,#204833,#204834,#204835,#204836,
#204837,#204838,#204839,#204840,#204841,#204842,#204843,#204844,#204845,
#204846,#204847,#204848,#204849,#204850,#204851,#204852,#204853),
 .UNSPECIFIED.,.F.,.F.,(4,3,3,3,3,3,3,3,3,3,3,3,3,3,3,3,3,3,3,3,3,3,3,3,
3,4),(252.422494451905,252.504956055664,252.587416993543,252.669877292941,
252.752336981254,252.834796085876,252.917254634199,252.999712653613,253.082170171506,
253.168847344586,253.251314130194,253.333779243325,253.416242793632,253.498704890746,
253.581165644278,253.66362516382,253.746083558948,253.828540939219,253.911007325038,
253.993470526662,254.075930982611,254.158389131247,254.240854735259,254.323314613836,
254.405778725573,254.469004940774),.UNSPECIFIED.);
#3424=B_SPLINE_CURVE_WITH_KNOTS('',3,(#204854,#204855,#204856,#204857,#204858,
#204859,#204860,#204861,#204862,#204863,#204864,#204865,#204866,#204867,
#204868,#204869,#204870,#204871,#204872,#204873,#204874,#204875,#204876,
#204877,#204878,#204879,#204880,#204881,#204882,#204883,#204884,#204885,
#204886,#204887,#204888,#204889,#204890,#204891,#204892,#204893,#204894,
#204895,#204896,#204897,#204898,#204899,#204900,#204901,#204902,#204903,
#204904,#204905,#204906,#204907,#204908,#204909,#204910,#204911,#204912,
#204913,#204914,#204915,#204916,#204917,#204918,#204919,#204920,#204921,
#204922,#204923,#204924,#204925,#204926,#204927,#204928,#204929,#204930,
#204931,#204932,#204933,#204934,#204935,#204936,#204937,#204938,#204939,
#204940,#204941,#204942,#204943,#204944,#204945,#204946,#204947,#204948,
#204949,#204950,#204951,#204952,#204953,#204954,#204955,#204956,#204957,
#204958,#204959,#204960,#204961,#204962,#204963,#204964,#204965,#204966,
#204967,#204968,#204969,#204970,#204971,#204972,#204973,#204974,#204975,
#204976,#204977,#204978,#204979,#204980,#204981,#204982,#204983,#204984,
#204985,#204986,#204987,#204988,#204989,#204990,#204991,#204992,#204993,
#204994,#204995,#204996,#204997,#204998,#204999,#205000,#205001,#205002,
#205003,#205004,#205005,#205006,#205007,#205008,#205009,#205010,#205011,
#205012,#205013,#205014,#205015,#205016,#205017,#205018,#205019,#205020,
#205021,#205022,#205023,#205024,#205025),.UNSPECIFIED.,.F.,.F.,(4,3,3,3,
3,3,3,3,3,3,3,3,3,3,3,3,3,3,3,3,3,3,3,3,3,3,3,3,3,3,3,3,3,3,3,3,3,3,3,3,
3,3,3,3,3,3,3,3,3,3,3,3,3,3,3,3,3,4),(254.46960918162,254.543372393565,
254.617102384427,254.690811973322,254.764532044339,254.808158530261,254.892834868469,
254.977657352983,255.062679723859,255.147788605667,255.233018145042,255.307528398192,
255.389084660852,255.470565600517,255.554648766919,255.635974519431,255.721436392777,
255.806898266123,255.886301607007,255.96572337817,256.045174355811,256.124698522031,
256.204264432576,256.283914280779,256.306268134054,256.384647154924,256.46295990624,
256.541220802393,256.619444220193,256.697644508353,256.775852697518,256.854068751008,
256.932305668238,257.010576458391,257.088940037864,257.167353167323,257.245883549836,
257.305007869916,257.38106437667,257.457025194664,257.532907115283,257.60872684879,
257.684501043121,257.761906863454,257.837654619569,257.913409625097,257.989186890327,
258.06782706919,258.143736255659,258.219702247601,258.295774445211,258.303747605778,
258.381317928865,258.46245396008,258.539836629605,258.617165310272,258.694446707613,
258.705862053727),.UNSPECIFIED.);
#3425=B_SPLINE_CURVE_WITH_KNOTS('',3,(#205031,#205032,#205033,#205034,#205035,
#205036,#205037,#205038,#205039,#205040,#205041,#205042,#205043,#205044,
#205045,#205046,#205047,#205048,#205049,#205050,#205051,#205052,#205053,
#205054,#205055,#205056,#205057,#205058,#205059,#205060,#205061,#205062,
#205063,#205064,#205065,#205066,#205067,#205068,#205069,#205070,#205071,
#205072,#205073,#205074,#205075,#205076,#205077,#205078,#205079,#205080,
#205081,#205082,#205083,#205084,#205085,#205086,#205087,#205088,#205089,
#205090,#205091,#205092,#205093,#205094,#205095,#205096,#205097,#205098,
#205099,#205100,#205101,#205102,#205103,#205104,#205105,#205106,#205107,
#205108,#205109,#205110,#205111,#205112,#205113,#205114,#205115,#205116,
#205117,#205118,#205119,#205120,#205121,#205122,#205123,#205124,#205125,
#205126,#205127,#205128,#205129,#205130,#205131,#205132,#205133,#205134,
#205135,#205136,#205137,#205138,#205139,#205140,#205141,#205142,#205143,
#205144,#205145,#205146,#205147,#205148,#205149,#205150,#205151,#205152,
#205153,#205154,#205155,#205156,#205157,#205158,#205159,#205160,#205161,
#205162,#205163,#205164,#205165,#205166,#205167,#205168,#205169,#205170,
#205171,#205172,#205173,#205174,#205175,#205176,#205177,#205178,#205179,
#205180,#205181,#205182,#205183,#205184,#205185,#205186,#205187,#205188,
#205189,#205190,#205191,#205192,#205193,#205194,#205195,#205196,#205197,
#205198,#205199),.UNSPECIFIED.,.F.,.F.,(4,3,3,3,3,3,3,3,3,3,3,3,3,3,3,3,
3,3,3,3,3,3,3,3,3,3,3,3,3,3,3,3,3,3,3,3,3,3,3,3,3,3,3,3,3,3,3,3,3,3,3,3,
3,3,3,3,4),(260.752190247953,260.870697092815,260.982282427759,261.058338934513,
261.134299752507,261.210181673126,261.286001406633,261.361775600964,261.439181421297,
261.514929177412,261.59068418294,261.66646144817,261.745101627033,261.821010813502,
261.896976805445,261.973049003055,261.981022163622,262.058581015167,262.136047559062,
262.213437462355,262.290766337048,262.368049751191,262.445310797763,262.522561498607,
262.599815901293,262.677088052825,262.754433390962,262.831816164687,262.909305660335,
262.979761899484,263.063981182377,263.14807386135,263.231960487163,263.31571747655,
263.399259179208,263.479131767415,263.556498963208,263.633884552659,263.711302334447,
263.78880725606,263.866361855312,263.944023202264,263.978501635346,264.05812237409,
264.137670201746,264.217157431022,264.296596327935,264.375999120742,264.45538433364,
264.534760564193,264.614138893743,264.693530403614,264.772975638445,264.852449219226,
264.931996331276,264.977241371208,264.989258096655),.UNSPECIFIED.);
#3426=B_SPLINE_CURVE_WITH_KNOTS('',3,(#205200,#205201,#205202,#205203,#205204,
#205205,#205206,#205207,#205208,#205209,#205210,#205211,#205212,#205213,
#205214,#205215,#205216,#205217,#205218,#205219,#205220,#205221,#205222,
#205223,#205224,#205225,#205226,#205227,#205228,#205229,#205230,#205231,
#205232,#205233,#205234,#205235,#205236,#205237,#205238,#205239,#205240,
#205241,#205242,#205243,#205244,#205245,#205246,#205247,#205248,#205249,
#205250,#205251,#205252,#205253,#205254,#205255,#205256,#205257,#205258,
#205259,#205260,#205261,#205262,#205263,#205264,#205265,#205266,#205267,
#205268,#205269,#205270,#205271,#205272,#205273,#205274,#205275),
 .UNSPECIFIED.,.F.,.F.,(4,3,3,3,3,3,3,3,3,3,3,3,3,3,3,3,3,3,3,3,3,3,3,3,
3,4),(258.705679759084,258.788141362843,258.870602300722,258.95306260012,
259.035522288433,259.117981393055,259.200439941378,259.282897960792,259.365355478686,
259.452032651765,259.534499437373,259.616964550504,259.699428100811,259.781890197925,
259.864350951457,259.946810471,260.029268866127,260.111726246397,260.194192632217,
260.276655833841,260.359116289789,260.441574438425,260.524040042437,260.606499921014,
260.688964032751,260.752190247953),.UNSPECIFIED.);
#3427=B_SPLINE_CURVE_WITH_KNOTS('',3,(#205277,#205278,#205279,#205280,#205281,
#205282,#205283,#205284,#205285,#205286,#205287,#205288,#205289,#205290,
#205291,#205292,#205293,#205294,#205295,#205296,#205297,#205298,#205299,
#205300,#205301,#205302,#205303,#205304,#205305,#205306,#205307,#205308,
#205309,#205310,#205311,#205312,#205313,#205314,#205315,#205316,#205317,
#205318,#205319,#205320,#205321,#205322,#205323,#205324,#205325,#205326,
#205327,#205328,#205329,#205330,#205331,#205332,#205333,#205334,#205335,
#205336,#205337,#205338,#205339,#205340,#205341,#205342,#205343,#205344,
#205345,#205346,#205347,#205348,#205349,#205350,#205351,#205352,#205353,
#205354,#205355,#205356,#205357,#205358),.UNSPECIFIED.,.F.,.F.,(4,3,3,3,
3,3,3,3,3,3,3,3,3,3,3,3,3,3,3,3,3,3,3,3,3,3,3,4),(258.705862053727,258.783119976353,
258.860370296477,258.937627060954,259.014904317578,259.09225596849,259.169647521608,
259.247141993696,259.302487341641,259.386706624534,259.470799303508,259.554685929322,
259.638442918708,259.721984621366,259.801857209572,259.879224405365,259.956609994816,
260.034027776602,260.111532698215,260.189087297467,260.266748644419,260.301227077503,
260.387540615977,260.473730924891,260.55969365616,260.645493440371,260.731032807719,
260.752190247953),.UNSPECIFIED.);
#3428=B_SPLINE_CURVE_WITH_KNOTS('',3,(#205359,#205360,#205361,#205362,#205363,
#205364,#205365,#205366,#205367,#205368,#205369,#205370,#205371,#205372,
#205373,#205374,#205375,#205376,#205377,#205378,#205379,#205380,#205381,
#205382,#205383,#205384,#205385,#205386,#205387,#205388,#205389,#205390,
#205391,#205392,#205393,#205394,#205395,#205396,#205397,#205398,#205399,
#205400,#205401,#205402,#205403,#205404,#205405,#205406,#205407,#205408,
#205409,#205410,#205411,#205412,#205413,#205414,#205415,#205416,#205417,
#205418,#205419,#205420,#205421,#205422,#205423,#205424,#205425,#205426,
#205427,#205428,#205429,#205430,#205431,#205432,#205433,#205434,#205435,
#205436,#205437,#205438,#205439,#205440,#205441,#205442,#205443,#205444,
#205445,#205446,#205447,#205448,#205449,#205450,#205451,#205452,#205453,
#205454,#205455,#205456,#205457,#205458,#205459,#205460,#205461,#205462,
#205463,#205464,#205465,#205466,#205467,#205468,#205469,#205470,#205471,
#205472,#205473,#205474,#205475,#205476,#205477,#205478,#205479,#205480,
#205481,#205482,#205483,#205484,#205485,#205486,#205487,#205488,#205489,
#205490,#205491,#205492,#205493,#205494,#205495,#205496,#205497,#205498,
#205499,#205500,#205501,#205502,#205503,#205504,#205505,#205506,#205507,
#205508,#205509,#205510,#205511,#205512,#205513,#205514,#205515),
 .UNSPECIFIED.,.F.,.F.,(4,3,3,3,3,3,3,3,3,3,3,3,3,3,3,3,3,3,3,3,3,3,3,3,
3,3,3,3,3,3,3,3,3,3,3,3,3,3,3,3,3,3,3,3,3,3,3,3,3,3,3,3,4),(260.752190247953,
260.834652454039,260.917114311827,260.999575828168,261.082037009912,261.164497863908,
261.246958397007,261.329418616057,261.411878527908,261.494338139407,261.576797457404,
261.659256488746,261.741715240281,261.824173718857,261.906631931322,261.989089884522,
262.071547585305,262.154005040516,262.236462257004,262.322474844793,262.405799539214,
262.488266144772,262.570731906123,262.653196850681,262.735661005859,262.818124399067,
262.90058705771,262.983049009194,263.06551028092,263.147970900289,263.230430894696,
263.312890291537,263.395349118206,263.477807402092,263.560265170585,263.642722451073,
263.726856364523,263.809322362821,263.89178673937,263.974249603812,264.056711065768,
264.139171234842,264.221630220617,264.30408813266,264.38968524936,264.472149986304,
264.554611758602,264.637071004693,264.719528162872,264.801990681771,264.884448353054,
264.966907143962,264.988865066264),.UNSPECIFIED.);
#3429=B_SPLINE_CURVE_WITH_KNOTS('',3,(#205521,#205522,#205523,#205524,#205525,
#205526,#205527,#205528,#205529,#205530,#205531,#205532,#205533,#205534,
#205535,#205536,#205537,#205538,#205539,#205540,#205541,#205542,#205543,
#205544,#205545,#205546,#205547,#205548,#205549,#205550,#205551,#205552,
#205553,#205554,#205555,#205556,#205557,#205558,#205559,#205560,#205561,
#205562,#205563,#205564,#205565,#205566,#205567,#205568,#205569,#205570,
#205571,#205572,#205573,#205574,#205575,#205576,#205577,#205578,#205579,
#205580,#205581,#205582,#205583,#205584,#205585,#205586,#205587,#205588,
#205589,#205590,#205591,#205592,#205593,#205594,#205595,#205596,#205597,
#205598,#205599,#205600,#205601,#205602,#205603,#205604,#205605,#205606,
#205607,#205608,#205609,#205610,#205611,#205612,#205613,#205614,#205615,
#205616,#205617,#205618,#205619,#205620,#205621,#205622,#205623,#205624,
#205625,#205626,#205627,#205628,#205629,#205630,#205631,#205632,#205633,
#205634,#205635,#205636,#205637,#205638,#205639,#205640,#205641,#205642,
#205643,#205644,#205645,#205646,#205647,#205648,#205649,#205650,#205651,
#205652,#205653,#205654,#205655,#205656,#205657,#205658,#205659,#205660,
#205661,#205662,#205663,#205664,#205665,#205666,#205667,#205668,#205669,
#205670,#205671,#205672,#205673,#205674,#205675,#205676,#205677,#205678,
#205679,#205680,#205681,#205682,#205683,#205684,#205685,#205686,#205687,
#205688,#205689),.UNSPECIFIED.,.F.,.F.,(4,3,3,3,3,3,3,3,3,3,3,3,3,3,3,3,
3,3,3,3,3,3,3,3,3,3,3,3,3,3,3,3,3,3,3,3,3,3,3,3,3,3,3,3,3,3,3,3,3,3,3,3,
3,3,3,3,4),(267.035375555214,267.113226162742,267.191012379613,267.268749321261,
267.346452067757,267.424828131637,267.502524314221,267.580233460035,267.657969206467,
267.736842049549,267.814710913995,267.894085746395,267.973460578795,268.049517085549,
268.125477903543,268.201359824162,268.277179557669,268.352953752,268.430359572332,
268.506107328447,268.581862333975,268.657639599206,268.736279778069,268.812188964538,
268.88815495648,268.96422715409,268.972200314657,269.049759166202,269.127225710097,
269.20461561339,269.281944488083,269.359227902226,269.436488948798,269.513739649642,
269.590994052327,269.668266203859,269.745611541997,269.822994315722,269.900483811369,
269.970940050519,270.055159333412,270.139252012385,270.223138638198,270.306895627585,
270.390437330243,270.47030991845,270.547677114243,270.625062703694,270.702480485482,
270.779985407095,270.857540006347,270.935201353299,270.969679786381,271.049292724175,
271.128841433105,271.208322864593,271.272348741102),.UNSPECIFIED.);
#3430=B_SPLINE_CURVE_WITH_KNOTS('',3,(#205690,#205691,#205692,#205693,#205694,
#205695,#205696,#205697,#205698,#205699,#205700,#205701,#205702,#205703,
#205704,#205705,#205706,#205707,#205708,#205709,#205710,#205711,#205712,
#205713,#205714,#205715,#205716,#205717,#205718,#205719,#205720,#205721,
#205722,#205723,#205724,#205725,#205726,#205727,#205728,#205729,#205730,
#205731,#205732,#205733,#205734,#205735,#205736,#205737,#205738,#205739,
#205740,#205741,#205742,#205743,#205744,#205745,#205746,#205747,#205748,
#205749,#205750,#205751,#205752,#205753,#205754,#205755,#205756,#205757,
#205758,#205759,#205760,#205761,#205762,#205763,#205764,#205765,#205766,
#205767,#205768,#205769,#205770,#205771),.UNSPECIFIED.,.F.,.F.,(4,3,3,3,
3,3,3,3,3,3,3,3,3,3,3,3,3,3,3,3,3,3,3,3,3,3,3,4),(264.989258096655,265.06596162616,
265.142600364666,265.21918899973,265.295743664136,265.372278865214,265.448818639486,
265.476611239139,265.561287577347,265.646110061861,265.731132432737,265.816241314545,
265.90147085392,265.97598110707,266.057537369729,266.139018309395,266.223101475797,
266.304427228308,266.389889101655,266.475350975001,266.554754315885,266.634176087048,
266.713627064688,266.793151230908,266.872717141453,266.952366989656,266.974720842932,
267.035375555133),.UNSPECIFIED.);
#3431=B_SPLINE_CURVE_WITH_KNOTS('',3,(#205773,#205774,#205775,#205776,#205777,
#205778,#205779,#205780,#205781,#205782,#205783,#205784,#205785,#205786,
#205787,#205788,#205789,#205790,#205791,#205792,#205793,#205794,#205795,
#205796,#205797,#205798,#205799,#205800,#205801,#205802,#205803,#205804,
#205805,#205806,#205807,#205808,#205809,#205810,#205811,#205812,#205813,
#205814,#205815,#205816,#205817,#205818,#205819,#205820,#205821,#205822,
#205823,#205824,#205825,#205826,#205827,#205828,#205829,#205830,#205831,
#205832,#205833,#205834,#205835,#205836,#205837,#205838,#205839,#205840,
#205841,#205842,#205843,#205844,#205845,#205846,#205847,#205848),
 .UNSPECIFIED.,.F.,.F.,(4,3,3,3,3,3,3,3,3,3,3,3,3,3,3,3,3,3,3,3,3,3,3,3,
3,4),(264.988865066264,265.071326670023,265.153787607902,265.2362479073,
265.318707595613,265.401166700235,265.483625248558,265.566083267972,265.648540785865,
265.735217958945,265.817684744553,265.900149857685,265.982613407991,266.065075505105,
266.147536258637,266.22999577818,266.312454173307,266.394911553578,266.477377939397,
266.559841141021,266.642301596969,266.724759745606,266.807225349617,266.889685228195,
266.972149339931,267.035375555133),.UNSPECIFIED.);
#3432=B_SPLINE_CURVE_WITH_KNOTS('',3,(#205849,#205850,#205851,#205852,#205853,
#205854,#205855,#205856,#205857,#205858,#205859,#205860,#205861,#205862,
#205863,#205864,#205865,#205866,#205867,#205868,#205869,#205870,#205871,
#205872,#205873,#205874,#205875,#205876,#205877,#205878,#205879,#205880,
#205881,#205882,#205883,#205884,#205885,#205886,#205887,#205888,#205889,
#205890,#205891,#205892,#205893,#205894,#205895,#205896,#205897,#205898,
#205899,#205900,#205901,#205902,#205903,#205904,#205905,#205906,#205907,
#205908,#205909,#205910,#205911,#205912,#205913,#205914,#205915,#205916,
#205917,#205918,#205919,#205920,#205921,#205922,#205923,#205924,#205925,
#205926,#205927,#205928,#205929,#205930,#205931,#205932,#205933,#205934,
#205935,#205936,#205937,#205938,#205939,#205940,#205941,#205942,#205943,
#205944,#205945,#205946,#205947,#205948,#205949,#205950,#205951,#205952,
#205953,#205954,#205955,#205956,#205957,#205958,#205959,#205960,#205961,
#205962,#205963,#205964,#205965,#205966,#205967,#205968,#205969,#205970,
#205971,#205972,#205973,#205974,#205975,#205976,#205977,#205978,#205979,
#205980,#205981,#205982,#205983,#205984,#205985,#205986,#205987,#205988,
#205989,#205990,#205991,#205992,#205993,#205994,#205995,#205996,#205997,
#205998,#205999,#206000,#206001,#206002,#206003,#206004,#206005,#206006,
#206007,#206008,#206009,#206010,#206011,#206012,#206013,#206014),
 .UNSPECIFIED.,.F.,.F.,(4,3,3,3,3,3,3,3,3,3,3,3,3,3,3,3,3,3,3,3,3,3,3,3,
3,3,3,3,3,3,3,3,3,3,3,3,3,3,3,3,3,3,3,3,3,3,3,3,3,3,3,3,3,3,3,4),(267.035375555133,
267.121673149256,267.208406509972,267.292405228538,267.372025967282,267.451573794938,
267.531061024214,267.610499921127,267.689902713933,267.769287926832,267.848664157384,
267.928042486935,268.007433996806,268.086879231637,268.166352812418,268.245899924467,
268.2911449644,268.367859971249,268.444507883613,268.521103395352,268.597662293051,
268.67419967713,268.750741197582,268.790514832331,268.875191170539,268.960013655052,
269.045036025928,269.130144907736,269.21537444711,269.289884700262,269.371440962922,
269.452921902588,269.537005068989,269.618330821502,269.703792694847,269.789254568193,
269.868657909077,269.94807968024,270.027530657881,270.107054824101,270.186620734646,
270.266270582849,270.288624436125,270.36700396344,270.445317071958,270.523578176484,
270.601801654128,270.6800018538,270.758208900558,270.836423602087,270.914658957359,
270.992927974971,271.071286312509,271.149694125371,271.228211424852,271.272446552927),
 .UNSPECIFIED.);
#3433=B_SPLINE_CURVE_WITH_KNOTS('',3,(#206020,#206021,#206022,#206023,#206024,
#206025,#206026,#206027,#206028,#206029,#206030,#206031,#206032,#206033,
#206034,#206035,#206036,#206037,#206038,#206039,#206040,#206041,#206042,
#206043,#206044,#206045,#206046,#206047,#206048,#206049,#206050,#206051,
#206052,#206053,#206054,#206055,#206056,#206057,#206058,#206059,#206060,
#206061,#206062,#206063,#206064,#206065,#206066,#206067,#206068,#206069,
#206070,#206071,#206072,#206073,#206074,#206075,#206076,#206077,#206078,
#206079,#206080,#206081,#206082,#206083,#206084,#206085,#206086,#206087,
#206088,#206089,#206090,#206091,#206092,#206093,#206094,#206095,#206096,
#206097,#206098,#206099,#206100,#206101,#206102,#206103,#206104,#206105,
#206106,#206107,#206108,#206109,#206110,#206111,#206112,#206113,#206114,
#206115,#206116,#206117,#206118,#206119,#206120,#206121,#206122,#206123,
#206124,#206125,#206126,#206127,#206128,#206129,#206130,#206131,#206132,
#206133,#206134,#206135,#206136,#206137,#206138,#206139,#206140,#206141,
#206142,#206143,#206144,#206145,#206146,#206147,#206148,#206149,#206150,
#206151,#206152,#206153,#206154,#206155,#206156,#206157,#206158,#206159,
#206160,#206161,#206162,#206163,#206164,#206165,#206166,#206167,#206168,
#206169,#206170,#206171,#206172,#206173,#206174,#206175,#206176),
 .UNSPECIFIED.,.F.,.F.,(4,3,3,3,3,3,3,3,3,3,3,3,3,3,3,3,3,3,3,3,3,3,3,3,
3,3,3,3,3,3,3,3,3,3,3,3,3,3,3,3,3,3,3,3,3,3,3,3,3,3,3,3,4),(273.318560862312,
273.401023068398,273.483484926186,273.565946442527,273.648407624271,273.730868478267,
273.813329011366,273.895789230416,273.978249142267,274.060708753766,274.143168071763,
274.225627103105,274.30808585464,274.390544333217,274.473002545681,274.555460498881,
274.637918199664,274.720375654876,274.802832871364,274.888845459153,274.972170153574,
275.054636759132,275.137102520483,275.219567465041,275.302031620219,275.384495013426,
275.46695767207,275.549419623554,275.63188089528,275.714341514648,275.796801509056,
275.879260905897,275.961719732565,276.044178016452,276.126635784945,276.209093065433,
276.293226978882,276.375692977181,276.458157353729,276.540620218171,276.623081680128,
276.705541849202,276.788000834977,276.87045874702,276.95605586372,277.038520600664,
277.120982372962,277.203441619053,277.285898777232,277.36836129613,277.450818967414,
277.533277758322,277.555235680623),.UNSPECIFIED.);
#3434=B_SPLINE_CURVE_WITH_KNOTS('',3,(#206177,#206178,#206179,#206180,#206181,
#206182,#206183,#206184,#206185,#206186,#206187,#206188,#206189,#206190,
#206191,#206192,#206193,#206194,#206195,#206196,#206197,#206198,#206199,
#206200,#206201,#206202,#206203,#206204,#206205,#206206,#206207,#206208,
#206209,#206210,#206211,#206212,#206213,#206214,#206215,#206216,#206217,
#206218,#206219,#206220,#206221,#206222,#206223,#206224,#206225,#206226,
#206227,#206228,#206229,#206230,#206231,#206232,#206233,#206234,#206235,
#206236,#206237,#206238,#206239,#206240,#206241,#206242,#206243,#206244,
#206245,#206246,#206247,#206248,#206249,#206250,#206251,#206252,#206253,
#206254,#206255,#206256,#206257,#206258),.UNSPECIFIED.,.F.,.F.,(4,3,3,3,
3,3,3,3,3,3,3,3,3,3,3,3,3,3,3,3,3,3,3,3,3,3,3,4),(271.272348741102,271.351757590811,
271.431145833752,271.51052294159,271.589899996501,271.669288079255,271.748728990676,
271.828196272274,271.907739962812,271.968419522243,272.045134529092,272.121782441457,
272.198377953196,272.274936850894,272.351474234974,272.428015755426,272.467789390175,
272.552465728384,272.637288212897,272.722310583774,272.807419465583,272.892649004958,
272.967159258106,273.055009659157,273.138354386056,273.221613149921,273.304753508643,
273.318560862312),.UNSPECIFIED.);
#3435=B_SPLINE_CURVE_WITH_KNOTS('',3,(#206260,#206261,#206262,#206263,#206264,
#206265,#206266,#206267,#206268,#206269,#206270,#206271,#206272,#206273,
#206274,#206275,#206276,#206277,#206278,#206279,#206280,#206281,#206282,
#206283,#206284,#206285,#206286,#206287,#206288,#206289,#206290,#206291,
#206292,#206293,#206294,#206295,#206296,#206297,#206298,#206299,#206300,
#206301,#206302,#206303,#206304,#206305,#206306,#206307,#206308,#206309,
#206310,#206311,#206312,#206313,#206314,#206315,#206316,#206317,#206318,
#206319,#206320,#206321,#206322,#206323,#206324,#206325,#206326,#206327,
#206328,#206329,#206330,#206331,#206332,#206333,#206334,#206335,#206336,
#206337,#206338,#206339,#206340,#206341,#206342,#206343,#206344,#206345,
#206346,#206347),.UNSPECIFIED.,.F.,.F.,(4,3,3,3,3,3,3,3,3,3,3,3,3,3,3,3,
3,3,3,3,3,3,3,3,3,3,3,3,3,4),(271.272446552927,271.287364171987,271.363420678741,
271.439381496735,271.515263417354,271.591083150861,271.666857345192,271.744263165524,
271.82001092164,271.895765927168,271.971543192398,272.050183371261,272.12609255773,
272.202058549672,272.278130747282,272.286103907849,272.363662759394,272.441129303289,
272.518519206582,272.595848081275,272.673131495418,272.75039254199,272.827643242834,
272.904897645519,272.982169797051,273.059515135189,273.136897908914,273.214387404561,
273.284843643711,273.318560862174),.UNSPECIFIED.);
#3436=B_SPLINE_CURVE_WITH_KNOTS('',3,(#206348,#206349,#206350,#206351,#206352,
#206353,#206354,#206355,#206356,#206357,#206358,#206359,#206360,#206361,
#206362,#206363,#206364,#206365,#206366,#206367,#206368,#206369,#206370,
#206371,#206372,#206373,#206374,#206375,#206376,#206377,#206378,#206379,
#206380,#206381,#206382,#206383,#206384,#206385,#206386,#206387,#206388,
#206389,#206390,#206391,#206392,#206393,#206394,#206395,#206396,#206397,
#206398,#206399,#206400,#206401,#206402,#206403,#206404,#206405,#206406,
#206407,#206408,#206409,#206410,#206411,#206412,#206413,#206414,#206415,
#206416,#206417,#206418,#206419,#206420,#206421,#206422,#206423,#206424,
#206425,#206426,#206427,#206428,#206429,#206430,#206431,#206432,#206433,
#206434,#206435,#206436,#206437,#206438,#206439,#206440,#206441,#206442,
#206443,#206444,#206445,#206446,#206447,#206448,#206449,#206450,#206451,
#206452,#206453,#206454,#206455,#206456,#206457,#206458,#206459,#206460,
#206461,#206462,#206463,#206464,#206465,#206466,#206467,#206468,#206469,
#206470,#206471,#206472,#206473,#206474,#206475,#206476,#206477,#206478,
#206479,#206480,#206481,#206482,#206483,#206484,#206485,#206486,#206487,
#206488,#206489,#206490,#206491,#206492,#206493,#206494,#206495,#206496,
#206497,#206498,#206499,#206500,#206501,#206502,#206503,#206504,#206505,
#206506,#206507,#206508,#206509,#206510,#206511,#206512,#206513,#206514,
#206515,#206516),.UNSPECIFIED.,.F.,.F.,(4,3,3,3,3,3,3,3,3,3,3,3,3,3,3,3,
3,3,3,3,3,3,3,3,3,3,3,3,3,3,3,3,3,3,3,3,3,3,3,3,3,3,3,3,3,3,3,3,3,3,3,3,
3,3,3,3,4),(273.318560862312,273.401319579048,273.483951878501,273.566402426066,
273.648741291947,273.730919046419,273.784213511642,273.861580707435,273.938966296886,
274.016384078674,274.093889000286,274.171443599539,274.249104946491,274.283583379573,
274.363204118317,274.442751945973,274.522239175248,274.601678072162,274.681080864968,
274.760466077867,274.839842308419,274.919220637969,274.99861214784,275.078057382671,
275.157530963452,275.237078075502,275.282323115435,275.359038122284,275.435686034648,
275.512281546387,275.588840444086,275.665377828165,275.741919348617,275.781692983366,
275.866369321574,275.951191806088,276.036214176964,276.121323058773,276.206552598148,
276.281062851298,276.362619113958,276.444100053624,276.528183220025,276.609508972537,
276.694970845883,276.780432719229,276.859836060113,276.939257831275,277.018708808916,
277.098232975136,277.177798885681,277.257448733884,277.27980258716,277.358178317146,
277.436494507362,277.514754126766,277.555413490998),.UNSPECIFIED.);
#3437=B_SPLINE_CURVE_WITH_KNOTS('',3,(#206522,#206523,#206524,#206525,#206526,
#206527,#206528,#206529,#206530,#206531,#206532,#206533,#206534,#206535,
#206536,#206537,#206538,#206539,#206540,#206541,#206542,#206543,#206544,
#206545,#206546,#206547,#206548,#206549,#206550,#206551,#206552,#206553,
#206554,#206555,#206556,#206557,#206558,#206559,#206560,#206561,#206562,
#206563,#206564,#206565,#206566,#206567,#206568,#206569,#206570,#206571,
#206572,#206573,#206574,#206575,#206576,#206577,#206578,#206579,#206580,
#206581,#206582,#206583,#206584,#206585,#206586,#206587,#206588,#206589,
#206590,#206591,#206592,#206593,#206594,#206595,#206596,#206597,#206598,
#206599,#206600,#206601,#206602,#206603,#206604,#206605,#206606,#206607,
#206608,#206609,#206610,#206611,#206612,#206613,#206614,#206615,#206616,
#206617,#206618,#206619,#206620,#206621,#206622,#206623,#206624,#206625,
#206626,#206627,#206628,#206629,#206630,#206631,#206632,#206633,#206634,
#206635,#206636,#206637,#206638,#206639,#206640,#206641,#206642,#206643,
#206644,#206645,#206646,#206647,#206648,#206649,#206650,#206651,#206652,
#206653,#206654,#206655,#206656,#206657,#206658,#206659,#206660,#206661,
#206662,#206663,#206664,#206665,#206666,#206667,#206668,#206669,#206670,
#206671,#206672,#206673,#206674,#206675,#206676,#206677,#206678,#206679,
#206680,#206681,#206682,#206683,#206684,#206685,#206686,#206687,#206688,
#206689,#206690),.UNSPECIFIED.,.F.,.F.,(4,3,3,3,3,3,3,3,3,3,3,3,3,3,3,3,
3,3,3,3,3,3,3,3,3,3,3,3,3,3,3,3,3,3,3,3,3,3,3,3,3,3,3,3,3,3,3,3,3,3,3,3,
3,3,3,3,4),(279.601746169492,279.690893979404,279.778229212141,279.868283310641,
279.958337409141,280.039893671801,280.121374611467,280.205457777868,280.28678353038,
280.372245403726,280.457707277072,280.537110617956,280.616532389119,280.69598336676,
280.77550753298,280.855073443525,280.934723291728,280.957077145003,281.035456165873,
281.113768917189,281.192029813342,281.270253231142,281.348453519301,281.426661708466,
281.504877761956,281.583114679186,281.66138546934,281.739749048813,281.818162178272,
281.896692560785,281.955816880865,282.031873387619,282.107834205613,282.183716126232,
282.259535859739,282.33531005407,282.412715874402,282.488463630518,282.564218636046,
282.639995901276,282.718636080139,282.794545266608,282.87051125855,282.94658345616,
282.954556616727,283.032122093181,283.109593983157,283.186987958972,283.268342910669,
283.345623807737,283.422879230533,283.500123234353,283.577369865329,283.654659144348,
283.731973167213,283.80935508972,283.837827572545),.UNSPECIFIED.);
#3438=B_SPLINE_CURVE_WITH_KNOTS('',3,(#206691,#206692,#206693,#206694,#206695,
#206696,#206697,#206698,#206699,#206700,#206701,#206702,#206703,#206704,
#206705,#206706,#206707,#206708,#206709,#206710,#206711,#206712,#206713,
#206714,#206715,#206716,#206717,#206718,#206719,#206720,#206721,#206722,
#206723,#206724,#206725,#206726,#206727,#206728,#206729,#206730,#206731,
#206732,#206733,#206734,#206735,#206736,#206737,#206738,#206739,#206740,
#206741,#206742,#206743,#206744,#206745,#206746,#206747,#206748,#206749,
#206750,#206751,#206752,#206753,#206754,#206755,#206756,#206757,#206758,
#206759,#206760,#206761,#206762,#206763,#206764,#206765,#206766),
 .UNSPECIFIED.,.F.,.F.,(4,3,3,3,3,3,3,3,3,3,3,3,3,3,3,3,3,3,3,3,3,3,3,3,
3,4),(277.555235680623,277.637697284382,277.720158222261,277.802618521659,
277.885078209972,277.967537314594,278.049995862917,278.132453882331,278.214911400224,
278.301588573303,278.384055358912,278.466520472043,278.54898402235,278.631446119464,
278.713906872996,278.796366392538,278.878824787665,278.961282167936,279.043748553756,
279.12621175538,279.208672211328,279.291130359965,279.373595963976,279.456055842554,
279.53851995429,279.601746169492),.UNSPECIFIED.);
#3439=B_SPLINE_CURVE_WITH_KNOTS('',3,(#206768,#206769,#206770,#206771,#206772,
#206773,#206774,#206775,#206776,#206777,#206778,#206779,#206780,#206781,
#206782,#206783,#206784,#206785,#206786,#206787,#206788,#206789,#206790,
#206791,#206792,#206793,#206794,#206795,#206796,#206797,#206798,#206799,
#206800,#206801,#206802,#206803,#206804,#206805,#206806,#206807,#206808,
#206809,#206810,#206811,#206812,#206813,#206814,#206815,#206816,#206817,
#206818,#206819,#206820,#206821,#206822,#206823,#206824,#206825,#206826,
#206827,#206828,#206829,#206830,#206831,#206832,#206833,#206834,#206835,
#206836,#206837,#206838,#206839,#206840,#206841,#206842,#206843,#206844,
#206845,#206846,#206847,#206848,#206849,#206850,#206851,#206852),
 .UNSPECIFIED.,.F.,.F.,(4,3,3,3,3,3,3,3,3,3,3,3,3,3,3,3,3,3,3,3,3,3,3,3,
3,3,3,3,4),(277.555413490998,277.633623098407,277.714238001484,277.792448912532,
277.870674844257,277.948928800526,278.03133218115,278.109724211507,278.18817289723,
278.266725737398,278.278542323022,278.354598829776,278.43055964777,278.506441568389,
278.582261301896,278.658035496228,278.73544131656,278.811189072675,278.886944078203,
278.962721343433,279.041361522296,279.117270708765,279.193236700707,279.269308898317,
279.277282058884,279.374587676882,279.471153022842,279.566208583516,279.601746169384),
 .UNSPECIFIED.);
#3440=B_SPLINE_CURVE_WITH_KNOTS('',3,(#206853,#206854,#206855,#206856,#206857,
#206858,#206859,#206860,#206861,#206862,#206863,#206864,#206865,#206866,
#206867,#206868,#206869,#206870,#206871,#206872,#206873,#206874,#206875,
#206876,#206877,#206878,#206879,#206880,#206881,#206882,#206883,#206884,
#206885,#206886,#206887,#206888,#206889,#206890,#206891,#206892,#206893,
#206894,#206895,#206896,#206897,#206898,#206899,#206900,#206901,#206902,
#206903,#206904,#206905,#206906,#206907,#206908,#206909,#206910,#206911,
#206912,#206913,#206914,#206915,#206916,#206917,#206918,#206919,#206920,
#206921,#206922,#206923,#206924,#206925,#206926,#206927,#206928,#206929,
#206930,#206931,#206932,#206933,#206934,#206935,#206936,#206937,#206938,
#206939,#206940,#206941,#206942,#206943,#206944,#206945,#206946,#206947,
#206948,#206949,#206950,#206951,#206952,#206953,#206954,#206955,#206956,
#206957,#206958,#206959,#206960,#206961,#206962,#206963,#206964,#206965,
#206966,#206967,#206968,#206969,#206970,#206971,#206972,#206973,#206974,
#206975,#206976,#206977,#206978,#206979,#206980,#206981,#206982,#206983,
#206984,#206985,#206986,#206987,#206988,#206989,#206990,#206991,#206992,
#206993,#206994,#206995,#206996,#206997,#206998,#206999,#207000,#207001,
#207002,#207003,#207004,#207005,#207006,#207007,#207008,#207009,#207010,
#207011,#207012,#207013,#207014,#207015,#207016,#207017,#207018),
 .UNSPECIFIED.,.F.,.F.,(4,3,3,3,3,3,3,3,3,3,3,3,3,3,3,3,3,3,3,3,3,3,3,3,
3,3,3,3,3,3,3,3,3,3,3,3,3,3,3,3,3,3,3,3,3,3,3,3,3,3,3,3,3,3,3,4),(279.601746169492,
279.677896898556,279.754018294861,279.830125479646,279.906233317609,279.982356672213,
280.058551322595,280.13478287845,280.211120338645,280.276021794746,280.360241077639,
280.444333756613,280.528220382426,280.611977371813,280.695519074471,280.775391662677,
280.85275885847,280.930144447921,281.00756222971,281.085067151323,281.162621750575,
281.240283097528,281.274761530609,281.354382269353,281.43393009701,281.513417326285,
281.592856223199,281.672259016005,281.751644228904,281.831020459456,281.910398789006,
281.989790298877,282.069235533708,282.148709114489,282.228256226539,282.273501266471,
282.350216273319,282.426864185683,282.503459697422,282.58001859512,282.656555979199,
282.733097499651,282.772871134402,282.85754747261,282.942369957124,283.027392328,
283.112501209809,283.197730749184,283.272241002333,283.353797264993,283.435278204658,
283.51936137106,283.600687123572,283.686148996918,283.771610870264,283.838466116601),
 .UNSPECIFIED.);
#3441=B_SPLINE_CURVE_WITH_KNOTS('',3,(#207024,#207025,#207026,#207027,#207028,
#207029,#207030,#207031,#207032,#207033,#207034,#207035,#207036,#207037,
#207038,#207039,#207040,#207041,#207042,#207043,#207044,#207045,#207046,
#207047,#207048,#207049,#207050,#207051,#207052,#207053,#207054,#207055,
#207056,#207057,#207058,#207059,#207060,#207061,#207062,#207063,#207064,
#207065,#207066,#207067,#207068,#207069,#207070,#207071,#207072,#207073,
#207074,#207075,#207076,#207077,#207078,#207079,#207080,#207081,#207082,
#207083,#207084,#207085,#207086,#207087,#207088,#207089,#207090,#207091,
#207092,#207093,#207094,#207095,#207096,#207097,#207098,#207099,#207100,
#207101,#207102,#207103,#207104,#207105,#207106,#207107,#207108,#207109,
#207110,#207111,#207112,#207113,#207114,#207115,#207116,#207117,#207118,
#207119,#207120,#207121,#207122,#207123,#207124,#207125,#207126,#207127,
#207128,#207129,#207130,#207131,#207132,#207133,#207134,#207135,#207136,
#207137,#207138,#207139,#207140,#207141,#207142,#207143,#207144,#207145,
#207146,#207147,#207148,#207149,#207150,#207151,#207152,#207153,#207154,
#207155,#207156,#207157,#207158,#207159,#207160,#207161,#207162,#207163,
#207164,#207165,#207166,#207167,#207168,#207169,#207170,#207171,#207172,
#207173,#207174,#207175,#207176,#207177,#207178,#207179,#207180),
 .UNSPECIFIED.,.F.,.F.,(4,3,3,3,3,3,3,3,3,3,3,3,3,3,3,3,3,3,3,3,3,3,3,3,
3,3,3,3,3,3,3,3,3,3,3,3,3,3,3,3,3,3,3,3,3,3,3,3,3,3,3,3,4),(285.884931476672,
285.967393682758,286.049855540546,286.132317056887,286.214778238631,286.297239092627,
286.379699625726,286.462159844776,286.544619756627,286.627079368126,286.709538686123,
286.791997717465,286.874456469,286.956914947577,287.039373160041,287.121831113241,
287.204288814024,287.286746269236,287.369203485723,287.455216073513,287.538540767934,
287.621007373492,287.703473134843,287.785938079401,287.868402234579,287.950865627786,
288.033328286429,288.115790237913,288.19825150964,288.280712129008,288.363172123415,
288.445631520256,288.528090346925,288.610548630811,288.693006399305,288.775463679792,
288.859597593242,288.94206359154,289.024527968089,289.106990832531,289.189452294488,
289.271912463561,289.354371449336,289.436829361379,289.52242647808,289.604891215023,
289.687352987321,289.769812233412,289.852269391591,289.93473191049,290.017189581773,
290.099648372681,290.121606294983),.UNSPECIFIED.);
#3442=B_SPLINE_CURVE_WITH_KNOTS('',3,(#207181,#207182,#207183,#207184,#207185,
#207186,#207187,#207188,#207189,#207190,#207191,#207192,#207193,#207194,
#207195,#207196,#207197,#207198,#207199,#207200,#207201,#207202,#207203,
#207204,#207205,#207206,#207207,#207208,#207209,#207210,#207211,#207212,
#207213,#207214,#207215,#207216,#207217,#207218,#207219,#207220,#207221,
#207222,#207223,#207224,#207225,#207226,#207227,#207228,#207229,#207230,
#207231,#207232,#207233,#207234,#207235,#207236,#207237,#207238,#207239,
#207240,#207241,#207242,#207243,#207244,#207245,#207246,#207247,#207248,
#207249,#207250,#207251,#207252,#207253,#207254,#207255,#207256,#207257,
#207258,#207259,#207260,#207261,#207262),.UNSPECIFIED.,.F.,.F.,(4,3,3,3,
3,3,3,3,3,3,3,3,3,3,3,3,3,3,3,3,3,3,3,3,3,3,3,4),(283.837827572545,283.91532849993,
283.95329635259,284.037515635483,284.121608314457,284.20549494027,284.289251929657,
284.372793632315,284.452666220521,284.530033416314,284.607419005765,284.684836787553,
284.762341709166,284.839896308418,284.91755765537,284.952036088452,285.030919142487,
285.109727320616,285.188474397012,285.267174100836,285.345843525019,285.42449680193,
285.50314632775,285.581804494266,285.660516220107,285.739254640006,285.818075735445,
285.884931476672),.UNSPECIFIED.);
#3443=B_SPLINE_CURVE_WITH_KNOTS('',3,(#207264,#207265,#207266,#207267,#207268,
#207269,#207270,#207271,#207272,#207273,#207274,#207275,#207276,#207277,
#207278,#207279,#207280,#207281,#207282,#207283,#207284,#207285,#207286,
#207287,#207288,#207289,#207290,#207291,#207292,#207293,#207294,#207295,
#207296,#207297,#207298,#207299,#207300,#207301,#207302,#207303,#207304,
#207305,#207306,#207307,#207308,#207309,#207310,#207311,#207312,#207313,
#207314,#207315,#207316,#207317,#207318,#207319,#207320,#207321,#207322,
#207323,#207324,#207325,#207326,#207327,#207328,#207329,#207330,#207331,
#207332,#207333,#207334,#207335,#207336,#207337,#207338,#207339,#207340,
#207341,#207342,#207343,#207344,#207345),.UNSPECIFIED.,.F.,.F.,(4,3,3,3,
3,3,3,3,3,3,3,3,3,3,3,3,3,3,3,3,3,3,3,3,3,3,3,4),(283.838466116601,283.917884258935,
283.997329903907,284.076848386575,284.156407041973,284.236052385932,284.270980738195,
284.349359759065,284.427672510381,284.505933406534,284.584156824334,284.662357112494,
284.740565301659,284.818781355149,284.897018272379,284.975289062533,285.053652642006,
285.132065771465,285.210596153978,285.269720474057,285.346621849384,285.423135263213,
285.49956483542,285.575925339308,285.653176873649,285.729441285927,285.807186381299,
285.884931476671),.UNSPECIFIED.);
#3444=B_SPLINE_CURVE_WITH_KNOTS('',3,(#207346,#207347,#207348,#207349,#207350,
#207351,#207352,#207353,#207354,#207355,#207356,#207357,#207358,#207359,
#207360,#207361,#207362,#207363,#207364,#207365,#207366,#207367,#207368,
#207369,#207370,#207371,#207372,#207373,#207374,#207375,#207376,#207377,
#207378,#207379,#207380,#207381,#207382,#207383,#207384,#207385,#207386,
#207387,#207388,#207389,#207390,#207391,#207392,#207393,#207394,#207395,
#207396,#207397,#207398,#207399,#207400,#207401,#207402,#207403,#207404,
#207405,#207406,#207407,#207408,#207409,#207410,#207411,#207412,#207413,
#207414,#207415,#207416,#207417,#207418,#207419,#207420,#207421,#207422,
#207423,#207424,#207425,#207426,#207427,#207428,#207429,#207430,#207431,
#207432,#207433,#207434,#207435,#207436,#207437,#207438,#207439,#207440,
#207441,#207442,#207443,#207444,#207445,#207446,#207447,#207448,#207449,
#207450,#207451,#207452,#207453,#207454,#207455,#207456,#207457,#207458,
#207459,#207460,#207461,#207462,#207463,#207464,#207465,#207466,#207467,
#207468,#207469,#207470,#207471,#207472,#207473,#207474,#207475,#207476,
#207477,#207478,#207479,#207480,#207481,#207482,#207483,#207484,#207485,
#207486,#207487,#207488,#207489,#207490,#207491,#207492,#207493,#207494,
#207495,#207496,#207497,#207498,#207499,#207500,#207501,#207502,#207503,
#207504,#207505,#207506,#207507,#207508,#207509,#207510,#207511,#207512,
#207513,#207514),.UNSPECIFIED.,.F.,.F.,(4,3,3,3,3,3,3,3,3,3,3,3,3,3,3,3,
3,3,3,3,3,3,3,3,3,3,3,3,3,3,3,3,3,3,3,3,3,3,3,3,3,3,3,3,3,3,3,3,3,3,3,3,
3,3,3,3,4),(285.884931476781,285.969634154445,286.054843488019,286.140319279605,
286.226170945113,286.268460209919,286.346019061464,286.423485605359,286.500875508652,
286.578204383345,286.655487797488,286.73274884406,286.809999544904,286.88725394759,
286.964526099121,287.041871437259,287.119254210984,287.196743706632,287.267199945782,
287.351419228675,287.435511907649,287.519398533462,287.603155522849,287.686697225507,
287.766569813713,287.843937009506,287.921322598957,287.998740380744,288.076245302357,
288.153799901609,288.231461248562,288.265939681644,288.345560420388,288.425108248044,
288.50459547732,288.584034374233,288.66343716704,288.742822379939,288.822198610491,
288.901576940041,288.980968449912,289.060413684743,289.139887265524,289.219434377574,
289.264679417506,289.341394424355,289.418042336719,289.494637848458,289.571196746156,
289.647734130235,289.724275650687,289.764049285437,289.848685666388,289.933540329203,
290.018502099263,290.103596709339,290.121230634672),.UNSPECIFIED.);
#3445=B_SPLINE_CURVE_WITH_KNOTS('',3,(#207520,#207521,#207522,#207523,#207524,
#207525,#207526,#207527,#207528,#207529,#207530,#207531,#207532,#207533,
#207534,#207535,#207536,#207537,#207538,#207539,#207540,#207541,#207542,
#207543,#207544,#207545,#207546,#207547,#207548,#207549,#207550,#207551,
#207552,#207553,#207554,#207555,#207556,#207557,#207558,#207559,#207560,
#207561,#207562,#207563,#207564,#207565,#207566,#207567,#207568,#207569,
#207570,#207571,#207572,#207573,#207574,#207575,#207576,#207577,#207578,
#207579,#207580,#207581,#207582,#207583,#207584,#207585,#207586,#207587,
#207588,#207589,#207590,#207591,#207592,#207593,#207594,#207595,#207596,
#207597,#207598,#207599,#207600,#207601,#207602,#207603,#207604,#207605,
#207606,#207607,#207608,#207609,#207610,#207611,#207612,#207613,#207614,
#207615,#207616,#207617,#207618,#207619,#207620,#207621,#207622,#207623,
#207624,#207625,#207626,#207627,#207628,#207629,#207630,#207631,#207632,
#207633,#207634,#207635,#207636,#207637,#207638,#207639,#207640,#207641,
#207642,#207643,#207644,#207645,#207646,#207647,#207648,#207649,#207650,
#207651,#207652,#207653,#207654,#207655,#207656,#207657,#207658,#207659,
#207660,#207661,#207662,#207663,#207664,#207665,#207666,#207667,#207668,
#207669,#207670,#207671,#207672,#207673,#207674,#207675,#207676),
 .UNSPECIFIED.,.F.,.F.,(4,3,3,3,3,3,3,3,3,3,3,3,3,3,3,3,3,3,3,3,3,3,3,3,
3,3,3,3,3,3,3,3,3,3,3,3,3,3,3,3,3,3,3,3,3,3,3,3,3,3,3,3,4),(292.168116783851,
292.250578989937,292.333040847725,292.415502364066,292.49796354581,292.580424399806,
292.662884932905,292.745345151956,292.827805063806,292.910264675305,292.992723993302,
293.075183024644,293.157641776179,293.240100254756,293.32255846722,293.405016420421,
293.487474121203,293.569931576415,293.652388792902,293.738401380692,293.821726075113,
293.904192680671,293.986658442022,294.06912338658,294.151587541758,294.234050934965,
294.316513593609,294.398975545093,294.481436816819,294.563897436187,294.646357430594,
294.728816827435,294.811275654104,294.89373393799,294.976191706484,295.058648986971,
295.142782900421,295.225248898719,295.307713275268,295.39017613971,295.472637601667,
295.555097770741,295.637556756515,295.720014668558,295.805611785259,295.888076522202,
295.970538294501,296.052997540592,296.13545469877,296.217917217669,296.300374888952,
296.382833679861,296.404791602162),.UNSPECIFIED.);
#3446=B_SPLINE_CURVE_WITH_KNOTS('',3,(#207677,#207678,#207679,#207680,#207681,
#207682,#207683,#207684,#207685,#207686,#207687,#207688,#207689,#207690,
#207691,#207692,#207693,#207694,#207695,#207696,#207697,#207698,#207699,
#207700,#207701,#207702,#207703,#207704,#207705,#207706,#207707,#207708,
#207709,#207710,#207711,#207712,#207713,#207714,#207715,#207716,#207717,
#207718,#207719,#207720,#207721,#207722,#207723,#207724,#207725,#207726,
#207727,#207728,#207729,#207730,#207731,#207732,#207733,#207734,#207735,
#207736,#207737,#207738,#207739,#207740,#207741,#207742,#207743,#207744,
#207745,#207746,#207747,#207748,#207749,#207750,#207751,#207752),
 .UNSPECIFIED.,.F.,.F.,(4,3,3,3,3,3,3,3,3,3,3,3,3,3,3,3,3,3,3,3,3,3,3,3,
3,4),(290.121606294983,290.204067898741,290.28652883662,290.368989136018,
290.451448824331,290.533907928953,290.616366477277,290.698824496691,290.781282014584,
290.867959187655,290.950425973264,291.032891086395,291.115354636702,291.197816733816,
291.280277487348,291.36273700689,291.445195402017,291.527652782288,291.610119168107,
291.692582369731,291.77504282568,291.857500974316,291.939966578328,292.022426456905,
292.104890568642,292.168116783727),.UNSPECIFIED.);
#3447=B_SPLINE_CURVE_WITH_KNOTS('',3,(#207754,#207755,#207756,#207757,#207758,
#207759,#207760,#207761,#207762,#207763,#207764,#207765,#207766,#207767,
#207768,#207769,#207770,#207771,#207772,#207773,#207774,#207775,#207776,
#207777,#207778,#207779,#207780,#207781,#207782,#207783,#207784,#207785,
#207786,#207787,#207788,#207789,#207790,#207791,#207792,#207793,#207794,
#207795,#207796,#207797,#207798,#207799,#207800,#207801,#207802,#207803,
#207804,#207805,#207806,#207807,#207808,#207809,#207810,#207811,#207812,
#207813,#207814,#207815,#207816,#207817,#207818,#207819,#207820,#207821,
#207822,#207823,#207824,#207825,#207826,#207827,#207828,#207829,#207830,
#207831,#207832,#207833,#207834,#207835),.UNSPECIFIED.,.F.,.F.,(4,3,3,3,
3,3,3,3,3,3,3,3,3,3,3,3,3,3,3,3,3,3,3,3,3,3,3,4),(290.121230634672,290.206467138343,
290.263419153368,290.344975416028,290.426456355693,290.510539522095,290.591865274607,
290.677327147953,290.762789021299,290.842192362183,290.921614133346,291.001065110987,
291.080589277207,291.160155187752,291.239805035956,291.26215888923,291.339336164723,
291.416444333208,291.493499236476,291.570516676688,291.647524024901,291.724528938895,
291.801545691994,291.878588561729,291.955715695224,292.032887936344,292.110173370506,
292.168116783776),.UNSPECIFIED.);
#3448=B_SPLINE_CURVE_WITH_KNOTS('',3,(#207836,#207837,#207838,#207839,#207840,
#207841,#207842,#207843,#207844,#207845,#207846,#207847,#207848,#207849,
#207850,#207851,#207852,#207853,#207854,#207855,#207856,#207857,#207858,
#207859,#207860,#207861,#207862,#207863,#207864,#207865,#207866,#207867,
#207868,#207869,#207870,#207871,#207872,#207873,#207874,#207875,#207876,
#207877,#207878,#207879,#207880,#207881,#207882,#207883,#207884,#207885,
#207886,#207887,#207888,#207889,#207890,#207891,#207892,#207893,#207894,
#207895,#207896,#207897,#207898,#207899,#207900,#207901,#207902,#207903,
#207904,#207905,#207906,#207907,#207908,#207909,#207910,#207911,#207912,
#207913,#207914,#207915,#207916,#207917,#207918,#207919,#207920,#207921,
#207922,#207923,#207924,#207925,#207926,#207927,#207928,#207929,#207930,
#207931,#207932,#207933,#207934,#207935,#207936,#207937,#207938,#207939,
#207940,#207941,#207942,#207943,#207944,#207945,#207946,#207947,#207948,
#207949,#207950,#207951,#207952,#207953,#207954,#207955,#207956,#207957,
#207958,#207959,#207960,#207961,#207962,#207963,#207964,#207965,#207966,
#207967,#207968,#207969,#207970,#207971,#207972,#207973,#207974,#207975,
#207976,#207977,#207978,#207979,#207980,#207981,#207982,#207983,#207984,
#207985,#207986,#207987,#207988,#207989,#207990,#207991,#207992,#207993,
#207994,#207995,#207996,#207997,#207998,#207999,#208000,#208001,#208002,
#208003,#208004),.UNSPECIFIED.,.F.,.F.,(4,3,3,3,3,3,3,3,3,3,3,3,3,3,3,3,
3,3,3,3,3,3,3,3,3,3,3,3,3,3,3,3,3,3,3,3,3,3,3,3,3,3,3,3,3,3,3,3,3,3,3,3,
3,3,3,3,4),(292.168116783851,292.260898625093,292.336955131847,292.412915949841,
292.48879787046,292.564617603967,292.640391798298,292.71779761863,292.793545374746,
292.869300380274,292.945077645504,293.023717824367,293.099627010836,293.175593002778,
293.251665200388,293.259638360955,293.3371972125,293.414663756395,293.492053659688,
293.569382534381,293.646665948524,293.723926995096,293.80117769594,293.878432098625,
293.955704250157,294.033049588295,294.110432362019,294.187921857667,294.258378096817,
294.34259737971,294.426690058683,294.510576684497,294.594333673883,294.677875376541,
294.757747964748,294.835115160541,294.912500749992,294.98991853178,295.067423453393,
295.144978052645,295.222639399597,295.257117832679,295.336738571423,295.416286399079,
295.495773628355,295.575212525268,295.654615318075,295.734000530974,295.813376761526,
295.892755091076,295.972146600947,296.051591835778,296.131065416559,296.210612528609,
296.255857568541,296.332566656646,296.405314229998),.UNSPECIFIED.);
#3449=B_SPLINE_CURVE_WITH_KNOTS('',3,(#208010,#208011,#208012,#208013,#208014,
#208015,#208016,#208017,#208018,#208019,#208020,#208021,#208022,#208023,
#208024,#208025,#208026,#208027,#208028,#208029,#208030,#208031,#208032,
#208033,#208034,#208035,#208036,#208037,#208038,#208039,#208040,#208041,
#208042,#208043,#208044,#208045,#208046,#208047,#208048,#208049,#208050,
#208051,#208052,#208053,#208054,#208055,#208056,#208057,#208058,#208059,
#208060,#208061,#208062,#208063,#208064,#208065,#208066,#208067,#208068,
#208069,#208070,#208071,#208072,#208073,#208074,#208075,#208076,#208077,
#208078,#208079,#208080,#208081,#208082,#208083,#208084,#208085,#208086,
#208087,#208088,#208089,#208090,#208091,#208092,#208093,#208094,#208095,
#208096,#208097,#208098,#208099,#208100,#208101,#208102,#208103,#208104,
#208105,#208106,#208107,#208108,#208109,#208110,#208111,#208112,#208113,
#208114,#208115,#208116,#208117,#208118,#208119,#208120,#208121,#208122,
#208123,#208124,#208125,#208126,#208127,#208128,#208129,#208130,#208131,
#208132,#208133,#208134,#208135,#208136,#208137,#208138,#208139,#208140,
#208141,#208142,#208143,#208144,#208145,#208146,#208147,#208148,#208149,
#208150,#208151,#208152,#208153,#208154,#208155,#208156,#208157,#208158,
#208159,#208160,#208161,#208162,#208163,#208164,#208165,#208166,#208167,
#208168,#208169,#208170,#208171,#208172,#208173,#208174,#208175,#208176,
#208177,#208178),.UNSPECIFIED.,.F.,.F.,(4,3,3,3,3,3,3,3,3,3,3,3,3,3,3,3,
3,3,3,3,3,3,3,3,3,3,3,3,3,3,3,3,3,3,3,3,3,3,3,3,3,3,3,3,3,3,3,3,3,3,3,3,
3,3,3,3,4),(298.451450161677,298.529117122841,298.606810096865,298.684542527595,
298.76236807435,298.840249052095,298.918235314131,298.934392390522,299.014013129267,
299.093560956922,299.173048186198,299.252487083111,299.331889875918,299.411275088816,
299.490651319369,299.570029648919,299.64942115879,299.728866393621,299.808339974402,
299.887887086451,299.933132126385,300.009847133234,300.086495045598,300.163090557338,
300.239649455036,300.316186839115,300.392728359568,300.432501994316,300.517178332524,
300.602000817038,300.687023187913,300.772132069722,300.857361609096,300.931871862247,
301.013428124907,301.094909064573,301.178992230974,301.260317983486,301.345779856832,
301.431241730178,301.510645071062,301.590066842225,301.669517819866,301.749041986087,
301.828607896631,301.908257744834,301.930611598109,302.008999852534,302.087319417554,
302.165577787803,302.243801614261,302.322003913219,302.400197685959,302.47841807422,
302.556651617678,302.634942192783,302.687552226885),.UNSPECIFIED.);
#3450=B_SPLINE_CURVE_WITH_KNOTS('',3,(#208179,#208180,#208181,#208182,#208183,
#208184,#208185,#208186,#208187,#208188,#208189,#208190,#208191,#208192,
#208193,#208194,#208195,#208196,#208197,#208198,#208199,#208200,#208201,
#208202,#208203,#208204,#208205,#208206,#208207,#208208,#208209,#208210,
#208211,#208212,#208213,#208214,#208215,#208216,#208217,#208218,#208219,
#208220,#208221,#208222,#208223,#208224,#208225,#208226,#208227,#208228,
#208229,#208230,#208231,#208232,#208233,#208234,#208235,#208236,#208237,
#208238,#208239,#208240,#208241,#208242,#208243,#208244,#208245,#208246,
#208247,#208248,#208249,#208250,#208251,#208252,#208253,#208254),
 .UNSPECIFIED.,.F.,.F.,(4,3,3,3,3,3,3,3,3,3,3,3,3,3,3,3,3,3,3,3,3,3,3,3,
3,4),(296.404791602162,296.487253205921,296.5697141438,296.652174443198,
296.734634131511,296.817093236133,296.899551784456,296.98200980387,297.064467321763,
297.151144494843,297.233611280451,297.316076393582,297.398539943889,297.481002041003,
297.563462794535,297.645922314077,297.728380709205,297.810838089475,297.893304475295,
297.975767676919,298.058228132867,298.140686281504,298.223151885515,298.305611764093,
298.388075875829,298.451302091031),.UNSPECIFIED.);
#3451=B_SPLINE_CURVE_WITH_KNOTS('',3,(#208256,#208257,#208258,#208259,#208260,
#208261,#208262,#208263,#208264,#208265,#208266,#208267,#208268,#208269,
#208270,#208271,#208272,#208273,#208274,#208275,#208276,#208277,#208278,
#208279,#208280,#208281,#208282,#208283,#208284,#208285,#208286,#208287,
#208288,#208289,#208290,#208291,#208292,#208293,#208294,#208295,#208296,
#208297,#208298,#208299,#208300,#208301,#208302,#208303,#208304,#208305,
#208306,#208307,#208308,#208309,#208310,#208311,#208312,#208313,#208314,
#208315,#208316,#208317,#208318,#208319,#208320,#208321,#208322,#208323,
#208324,#208325,#208326,#208327,#208328,#208329,#208330,#208331,#208332,
#208333,#208334),.UNSPECIFIED.,.F.,.F.,(4,3,3,3,3,3,3,3,3,3,3,3,3,3,3,3,
3,3,3,3,3,3,3,3,3,3,4),(296.405314229998,296.481912058359,296.558472403764,
296.635010567897,296.711552741933,296.755227436472,296.83990377468,296.924726259194,
297.009748630071,297.094857511879,297.180087051255,297.254597304403,297.336153567063,
297.417634506729,297.50171767313,297.583043425642,297.668505298989,297.753967172335,
297.83337051322,297.912792284383,297.992243262024,298.071767428245,298.15133333879,
298.230983186994,298.253337040266,298.356769259851,298.451302090931),
 .UNSPECIFIED.);
#3452=B_SPLINE_CURVE_WITH_KNOTS('',3,(#208335,#208336,#208337,#208338,#208339,
#208340,#208341,#208342,#208343,#208344,#208345,#208346,#208347,#208348,
#208349,#208350,#208351,#208352,#208353,#208354,#208355,#208356,#208357,
#208358,#208359,#208360,#208361,#208362,#208363,#208364,#208365,#208366,
#208367,#208368,#208369,#208370,#208371,#208372,#208373,#208374,#208375,
#208376,#208377,#208378,#208379,#208380,#208381,#208382,#208383,#208384,
#208385,#208386,#208387,#208388,#208389,#208390,#208391,#208392,#208393,
#208394,#208395,#208396,#208397,#208398,#208399,#208400,#208401,#208402,
#208403,#208404,#208405,#208406,#208407,#208408,#208409,#208410,#208411,
#208412,#208413,#208414,#208415,#208416,#208417,#208418,#208419,#208420,
#208421,#208422,#208423,#208424,#208425,#208426,#208427,#208428,#208429,
#208430,#208431,#208432,#208433,#208434,#208435,#208436,#208437,#208438,
#208439,#208440,#208441,#208442,#208443,#208444,#208445,#208446,#208447,
#208448,#208449,#208450,#208451,#208452,#208453,#208454,#208455,#208456,
#208457,#208458,#208459,#208460,#208461,#208462,#208463,#208464,#208465,
#208466,#208467,#208468,#208469,#208470,#208471,#208472,#208473,#208474,
#208475,#208476,#208477,#208478,#208479,#208480,#208481,#208482,#208483,
#208484,#208485,#208486,#208487,#208488,#208489,#208490,#208491,#208492,
#208493,#208494,#208495,#208496,#208497,#208498,#208499,#208500,#208501,
#208502,#208503,#208504,#208505,#208506),.UNSPECIFIED.,.F.,.F.,(4,3,3,3,
3,3,3,3,3,3,3,3,3,3,3,3,3,3,3,3,3,3,3,3,3,3,3,3,3,3,3,3,3,3,3,3,3,3,3,3,
3,3,3,3,3,3,3,3,3,3,3,3,3,3,3,3,3,4),(298.451302091031,298.529010392149,
298.606680654895,298.687355170049,298.765010704575,298.842676268073,298.920365536129,
298.998092194966,299.075910410184,299.153782671309,299.231760731932,299.252076776128,
299.328133282882,299.404094100876,299.479976021495,299.555795755002,299.631569949333,
299.708975769665,299.784723525781,299.860478531309,299.936255796539,300.014895975402,
300.09080516187,300.166771153813,300.242843351423,300.25081651199,300.328375363535,
300.40584190743,300.483231810723,300.560560685416,300.637844099558,300.71510514613,
300.792355846974,300.86961024966,300.946882401192,301.024227739329,301.101610513054,
301.179100008702,301.249556247852,301.333775530745,301.417868209718,301.501754835531,
301.585511824918,301.669053527576,301.748926115783,301.826293311576,301.903678901027,
301.981096682815,302.058601604427,302.13615620368,302.213817550632,302.248295983714,
302.327921744234,302.407476581218,302.486958355055,302.56639657612,302.645798576232,
302.688221398627),.UNSPECIFIED.);
#3453=B_SPLINE_CURVE_WITH_KNOTS('',3,(#208512,#208513,#208514,#208515,#208516,
#208517,#208518,#208519,#208520,#208521,#208522,#208523,#208524,#208525,
#208526,#208527,#208528,#208529,#208530,#208531,#208532,#208533,#208534,
#208535,#208536,#208537,#208538,#208539,#208540,#208541,#208542,#208543,
#208544,#208545,#208546,#208547,#208548,#208549,#208550,#208551,#208552,
#208553,#208554,#208555,#208556,#208557,#208558,#208559,#208560,#208561,
#208562,#208563,#208564,#208565,#208566,#208567,#208568,#208569,#208570,
#208571,#208572,#208573,#208574,#208575,#208576,#208577,#208578,#208579,
#208580,#208581,#208582,#208583,#208584,#208585,#208586,#208587,#208588,
#208589,#208590,#208591,#208592,#208593,#208594,#208595,#208596,#208597,
#208598,#208599,#208600,#208601,#208602,#208603,#208604,#208605,#208606,
#208607,#208608,#208609,#208610,#208611,#208612,#208613,#208614,#208615,
#208616,#208617,#208618,#208619,#208620,#208621,#208622,#208623,#208624,
#208625,#208626,#208627,#208628,#208629,#208630,#208631,#208632,#208633,
#208634,#208635,#208636,#208637,#208638,#208639,#208640,#208641,#208642,
#208643,#208644,#208645,#208646,#208647,#208648,#208649,#208650,#208651,
#208652,#208653,#208654,#208655,#208656,#208657,#208658,#208659,#208660,
#208661,#208662,#208663,#208664,#208665,#208666,#208667,#208668,#208669,
#208670,#208671,#208672,#208673,#208674,#208675,#208676,#208677),
 .UNSPECIFIED.,.F.,.F.,(4,3,3,3,3,3,3,3,3,3,3,3,3,3,3,3,3,3,3,3,3,3,3,3,
3,3,3,3,3,3,3,3,3,3,3,3,3,3,3,3,3,3,3,3,3,3,3,3,3,3,3,3,3,3,3,4),(304.734487398304,
304.836061119486,304.926830805695,305.011050088588,305.095142767561,305.179029393374,
305.262786382761,305.346328085419,305.426200673627,305.50356786942,305.580953458871,
305.658371240659,305.735876162272,305.813430761524,305.891092108477,305.925570541558,
306.005191280302,306.084739107958,306.164226337234,306.243665234147,306.323068026953,
306.402453239852,306.481829470404,306.561207799955,306.640599309826,306.720044544657,
306.799518125437,306.879065237487,306.92431027742,307.001025284269,307.077673196633,
307.154268708372,307.23082760607,307.307364990149,307.383906510601,307.423680145351,
307.508356483559,307.593178968073,307.678201338949,307.763310220757,307.848539760132,
307.923050013282,308.004606275942,308.086087215608,308.170170382009,308.251496134521,
308.336958007867,308.422419881213,308.501823222097,308.581244993259,308.6606959709,
308.74022013712,308.819786047665,308.899435895868,308.921789749144,308.971301374524),
 .UNSPECIFIED.);
#3454=B_SPLINE_CURVE_WITH_KNOTS('',3,(#208678,#208679,#208680,#208681,#208682,
#208683,#208684,#208685,#208686,#208687,#208688,#208689,#208690,#208691,
#208692,#208693,#208694,#208695,#208696,#208697,#208698,#208699,#208700,
#208701,#208702,#208703,#208704,#208705,#208706,#208707,#208708,#208709,
#208710,#208711,#208712,#208713,#208714,#208715,#208716,#208717,#208718,
#208719,#208720,#208721,#208722,#208723,#208724,#208725,#208726,#208727,
#208728,#208729,#208730,#208731,#208732,#208733,#208734,#208735,#208736,
#208737,#208738,#208739,#208740,#208741,#208742,#208743,#208744,#208745,
#208746,#208747,#208748,#208749,#208750,#208751,#208752,#208753,#208754,
#208755,#208756,#208757,#208758,#208759,#208760,#208761,#208762),
 .UNSPECIFIED.,.F.,.F.,(4,3,3,3,3,3,3,3,3,3,3,3,3,3,3,3,3,3,3,3,3,3,3,3,
3,3,3,3,4),(302.687552226885,302.76594779,302.847649561986,302.929351333971,
303.005407840725,303.081368658719,303.157250579338,303.233070312845,303.308844507176,
303.386250327508,303.461998083623,303.537753089152,303.613530354382,303.692170533245,
303.768079719713,303.844045711655,303.920117909266,303.928091069833,304.005110795359,
304.082036975103,304.158885782019,304.235664478819,304.312404053226,304.389119020399,
304.465823878307,304.542555067192,304.61930074801,304.696103995048,304.73448739821),
 .UNSPECIFIED.);
#3455=B_SPLINE_CURVE_WITH_KNOTS('',3,(#208764,#208765,#208766,#208767,#208768,
#208769,#208770,#208771,#208772,#208773,#208774,#208775,#208776,#208777,
#208778,#208779,#208780,#208781,#208782,#208783,#208784,#208785,#208786,
#208787,#208788,#208789,#208790,#208791,#208792,#208793,#208794,#208795,
#208796,#208797,#208798,#208799,#208800,#208801,#208802,#208803,#208804,
#208805,#208806,#208807,#208808,#208809,#208810,#208811,#208812,#208813,
#208814,#208815,#208816,#208817,#208818,#208819,#208820,#208821,#208822,
#208823,#208824,#208825,#208826,#208827,#208828,#208829,#208830,#208831,
#208832,#208833,#208834,#208835,#208836,#208837,#208838,#208839,#208840,
#208841,#208842),.UNSPECIFIED.,.F.,.F.,(4,3,3,3,3,3,3,3,3,3,3,3,3,3,3,3,
3,3,3,3,3,3,3,3,3,3,4),(302.688221398627,302.76760043219,302.846976406087,
302.926360400764,303.006529230468,303.085988619068,303.166512169322,303.247035719577,
303.323750726426,303.40039863879,303.476994150529,303.553553048227,303.630090432306,
303.706631952759,303.746405587508,303.831081925716,303.91590441023,304.000926781105,
304.086035662914,304.171265202288,304.245775455439,304.327392409246,304.408933645812,
304.490379591283,304.571766001586,304.653126699898,304.73448739821),
 .UNSPECIFIED.);
#3456=B_SPLINE_CURVE_WITH_KNOTS('',3,(#208843,#208844,#208845,#208846,#208847,
#208848,#208849,#208850,#208851,#208852,#208853,#208854,#208855,#208856,
#208857,#208858,#208859,#208860,#208861,#208862,#208863,#208864,#208865,
#208866,#208867,#208868,#208869,#208870,#208871,#208872,#208873,#208874,
#208875,#208876,#208877,#208878,#208879,#208880,#208881,#208882,#208883,
#208884,#208885,#208886,#208887,#208888,#208889,#208890,#208891,#208892,
#208893,#208894,#208895,#208896,#208897,#208898,#208899,#208900,#208901,
#208902,#208903,#208904,#208905,#208906,#208907,#208908,#208909,#208910,
#208911,#208912,#208913,#208914,#208915,#208916,#208917,#208918,#208919,
#208920,#208921,#208922,#208923,#208924,#208925,#208926,#208927,#208928,
#208929,#208930,#208931,#208932,#208933,#208934,#208935,#208936,#208937,
#208938,#208939,#208940,#208941,#208942,#208943,#208944,#208945,#208946,
#208947,#208948,#208949,#208950,#208951,#208952,#208953,#208954,#208955,
#208956,#208957,#208958,#208959,#208960,#208961,#208962,#208963,#208964,
#208965,#208966,#208967,#208968,#208969,#208970,#208971,#208972,#208973,
#208974,#208975,#208976,#208977,#208978,#208979,#208980,#208981,#208982,
#208983,#208984,#208985,#208986,#208987,#208988,#208989,#208990,#208991,
#208992,#208993,#208994,#208995,#208996,#208997,#208998,#208999),
 .UNSPECIFIED.,.F.,.F.,(4,3,3,3,3,3,3,3,3,3,3,3,3,3,3,3,3,3,3,3,3,3,3,3,
3,3,3,3,3,3,3,3,3,3,3,3,3,3,3,3,3,3,3,3,3,3,3,3,3,3,3,3,4),(304.73448739821,
304.816949604296,304.899411462084,304.981872978425,305.064334160169,305.146795014165,
305.229255547264,305.311715766314,305.394175678165,305.476635289664,305.559094607661,
305.641553639003,305.724012390538,305.806470869114,305.888929081579,305.971387034779,
306.053844735562,306.136302190773,306.218759407261,306.30477199505,306.388096689471,
306.47056329503,306.55302905638,306.635494000938,306.717958156116,306.800421549324,
306.882884207967,306.965346159451,307.047807431178,307.130268050546,307.212728044953,
307.295187441794,307.377646268463,307.460104552349,307.542562320842,307.62501960133,
307.70915351478,307.791619513078,307.874083889627,307.956546754069,308.039008216026,
308.121468385099,308.203927370874,308.286385282917,308.371982399617,308.454447136561,
308.536908908859,308.61936815495,308.701825313129,308.784287832028,308.866745503311,
308.94920429422,308.971162216521),.UNSPECIFIED.);
#3457=B_SPLINE_CURVE_WITH_KNOTS('',3,(#209005,#209006,#209007,#209008,#209009,
#209010,#209011,#209012,#209013,#209014,#209015,#209016,#209017,#209018,
#209019,#209020,#209021,#209022,#209023,#209024,#209025,#209026,#209027,
#209028,#209029,#209030,#209031,#209032,#209033,#209034,#209035,#209036,
#209037,#209038,#209039,#209040,#209041,#209042,#209043,#209044,#209045,
#209046,#209047,#209048,#209049,#209050,#209051,#209052,#209053,#209054,
#209055,#209056,#209057,#209058,#209059,#209060,#209061,#209062,#209063,
#209064,#209065,#209066,#209067,#209068,#209069,#209070,#209071,#209072,
#209073,#209074,#209075,#209076,#209077,#209078,#209079,#209080,#209081,
#209082,#209083,#209084,#209085,#209086,#209087,#209088,#209089,#209090,
#209091,#209092,#209093,#209094,#209095,#209096,#209097,#209098,#209099,
#209100,#209101,#209102,#209103,#209104,#209105,#209106,#209107,#209108,
#209109,#209110,#209111,#209112,#209113,#209114,#209115,#209116,#209117,
#209118,#209119,#209120,#209121,#209122,#209123,#209124,#209125,#209126,
#209127,#209128,#209129,#209130,#209131,#209132,#209133,#209134,#209135,
#209136,#209137,#209138,#209139,#209140,#209141,#209142,#209143,#209144,
#209145,#209146,#209147,#209148,#209149,#209150,#209151,#209152,#209153,
#209154,#209155,#209156,#209157,#209158,#209159,#209160,#209161,#209162,
#209163,#209164,#209165,#209166,#209167,#209168,#209169,#209170,#209171,
#209172,#209173),.UNSPECIFIED.,.F.,.F.,(4,3,3,3,3,3,3,3,3,3,3,3,3,3,3,3,
3,3,3,3,3,3,3,3,3,3,3,3,3,3,3,3,3,3,3,3,3,3,3,3,3,3,3,3,3,3,3,3,3,3,3,3,
3,3,3,3,4),(311.01767270548,311.093953767193,311.170148397586,311.246273239023,
311.322344867964,311.398384892228,311.474409360757,311.550433196865,311.626471321894,
311.702578658091,311.778721948788,311.854968836195,311.918008956731,312.002228239624,
312.086320918597,312.170207544411,312.253964533797,312.337506236455,312.417378824662,
312.494746020455,312.572131609906,312.649549391694,312.727054313307,312.804608912559,
312.882270259511,312.916748692593,312.996369431337,313.075917258994,313.155404488269,
313.234843385183,313.314246177989,313.393631390888,313.47300762144,313.55238595099,
313.631777460861,313.711222695692,313.790696276473,313.870243388523,313.915488428455,
313.992203435304,314.068851347668,314.145446859406,314.222005757105,314.298543141184,
314.375084661636,314.414858296386,314.499534634594,314.584357119108,314.669379489983,
314.754488371792,314.839717911167,314.914228164317,314.999378556216,315.080847967622,
315.162254743281,315.243589025594,315.254829731915),.UNSPECIFIED.);
#3458=B_SPLINE_CURVE_WITH_KNOTS('',3,(#209174,#209175,#209176,#209177,#209178,
#209179,#209180,#209181,#209182,#209183,#209184,#209185,#209186,#209187,
#209188,#209189,#209190,#209191,#209192,#209193,#209194,#209195,#209196,
#209197,#209198,#209199,#209200,#209201,#209202,#209203,#209204,#209205,
#209206,#209207,#209208,#209209,#209210,#209211,#209212,#209213,#209214,
#209215,#209216,#209217,#209218,#209219,#209220,#209221,#209222,#209223,
#209224,#209225,#209226,#209227,#209228,#209229,#209230,#209231,#209232,
#209233,#209234,#209235,#209236,#209237,#209238,#209239,#209240,#209241,
#209242,#209243,#209244,#209245,#209246,#209247,#209248,#209249,#209250,
#209251,#209252,#209253,#209254,#209255),.UNSPECIFIED.,.F.,.F.,(4,3,3,3,
3,3,3,3,3,3,3,3,3,3,3,3,3,3,3,3,3,3,3,3,3,3,3,4),(308.971301374524,309.049636861122,
309.127915186984,309.206150741656,309.284357883102,309.36387933334,309.44209114063,
309.520319240875,309.598576638973,309.679064850481,309.757460633806,309.838995059406,
309.920529485006,309.99658599176,310.072546809754,310.148428730373,310.22424846388,
310.300022658211,310.377428478544,310.453176234659,310.528931240187,310.604708505418,
310.68334868428,310.759257870749,310.835223862692,310.911296060302,310.919269220869,
311.01767270539),.UNSPECIFIED.);
#3459=B_SPLINE_CURVE_WITH_KNOTS('',3,(#209257,#209258,#209259,#209260,#209261,
#209262,#209263,#209264,#209265,#209266,#209267,#209268,#209269,#209270,
#209271,#209272,#209273,#209274,#209275,#209276,#209277,#209278,#209279,
#209280,#209281,#209282,#209283,#209284,#209285,#209286,#209287,#209288,
#209289,#209290,#209291,#209292,#209293,#209294,#209295,#209296,#209297,
#209298,#209299,#209300,#209301,#209302,#209303,#209304,#209305,#209306,
#209307,#209308,#209309,#209310,#209311,#209312,#209313,#209314,#209315,
#209316,#209317,#209318,#209319,#209320,#209321,#209322,#209323,#209324,
#209325,#209326,#209327,#209328,#209329,#209330,#209331,#209332),
 .UNSPECIFIED.,.F.,.F.,(4,3,3,3,3,3,3,3,3,3,3,3,3,3,3,3,3,3,3,3,3,3,3,3,
3,4),(308.971162216521,309.05362382028,309.136084758159,309.218545057557,
309.30100474587,309.383463850492,309.465922398815,309.548380418229,309.630837936122,
309.717515109202,309.79998189481,309.882447007941,309.964910558248,310.047372655362,
310.129833408894,310.212292928437,310.294751323564,310.377208703835,310.459675089654,
310.542138291278,310.624598747227,310.707056895863,310.789522499874,310.871982378452,
310.954446490188,311.01767270539),.UNSPECIFIED.);
#3460=B_SPLINE_CURVE_WITH_KNOTS('',3,(#209333,#209334,#209335,#209336,#209337,
#209338,#209339,#209340,#209341,#209342,#209343,#209344,#209345,#209346,
#209347,#209348,#209349,#209350,#209351,#209352,#209353,#209354,#209355,
#209356,#209357,#209358,#209359,#209360,#209361,#209362,#209363,#209364,
#209365,#209366,#209367,#209368,#209369,#209370,#209371,#209372,#209373,
#209374,#209375,#209376,#209377,#209378,#209379,#209380,#209381,#209382,
#209383,#209384,#209385,#209386,#209387,#209388,#209389,#209390,#209391,
#209392,#209393,#209394,#209395,#209396,#209397,#209398,#209399,#209400,
#209401,#209402,#209403,#209404,#209405,#209406,#209407,#209408,#209409,
#209410,#209411,#209412,#209413,#209414,#209415,#209416,#209417,#209418,
#209419,#209420,#209421,#209422,#209423,#209424,#209425,#209426,#209427,
#209428,#209429,#209430,#209431,#209432,#209433,#209434,#209435,#209436,
#209437,#209438,#209439,#209440,#209441,#209442,#209443,#209444,#209445,
#209446,#209447,#209448,#209449,#209450,#209451,#209452,#209453,#209454,
#209455,#209456,#209457,#209458,#209459,#209460,#209461,#209462,#209463,
#209464,#209465,#209466,#209467,#209468,#209469,#209470,#209471,#209472,
#209473,#209474,#209475,#209476,#209477,#209478,#209479,#209480,#209481,
#209482,#209483,#209484,#209485,#209486,#209487,#209488,#209489),
 .UNSPECIFIED.,.F.,.F.,(4,3,3,3,3,3,3,3,3,3,3,3,3,3,3,3,3,3,3,3,3,3,3,3,
3,3,3,3,3,3,3,3,3,3,3,3,3,3,3,3,3,3,3,3,3,3,3,3,3,3,3,3,4),(311.017672705512,
311.100134911598,311.182596769386,311.265058285727,311.347519467471,311.429980321467,
311.512440854566,311.594901073616,311.677360985467,311.759820596966,311.842279914962,
311.924738946305,312.00719769784,312.089656176416,312.172114388881,312.254572342081,
312.337030042864,312.419487498075,312.501944714563,312.587957302349,312.671281996766,
312.753748602324,312.836214363675,312.918679308233,313.001143463411,313.083606856618,
313.166069515262,313.248531466746,313.330992738472,313.41345335784,313.495913352248,
313.578372749089,313.660831575757,313.743289859644,313.825747628137,313.908204908625,
313.992338822067,314.074804820365,314.157269196914,314.239732061356,314.322193523313,
314.404653692387,314.487112678161,314.569570590204,314.655167706891,314.737632443835,
314.820094216133,314.902553462224,314.985010620403,315.067473139302,315.149930810585,
315.232389601493,315.254347523701),.UNSPECIFIED.);
#3461=B_SPLINE_CURVE_WITH_KNOTS('',3,(#209495,#209496,#209497,#209498,#209499,
#209500,#209501,#209502,#209503,#209504,#209505,#209506,#209507,#209508,
#209509,#209510,#209511,#209512,#209513,#209514,#209515,#209516,#209517,
#209518,#209519,#209520,#209521,#209522,#209523,#209524,#209525,#209526,
#209527,#209528,#209529,#209530,#209531,#209532,#209533,#209534,#209535,
#209536,#209537,#209538,#209539,#209540,#209541,#209542,#209543,#209544,
#209545,#209546,#209547,#209548,#209549,#209550,#209551,#209552,#209553,
#209554,#209555,#209556,#209557,#209558,#209559,#209560,#209561,#209562,
#209563,#209564,#209565,#209566,#209567,#209568,#209569,#209570,#209571,
#209572,#209573,#209574,#209575,#209576,#209577,#209578,#209579,#209580,
#209581,#209582,#209583,#209584,#209585,#209586,#209587,#209588,#209589,
#209590,#209591,#209592,#209593,#209594,#209595,#209596,#209597,#209598,
#209599,#209600,#209601,#209602,#209603,#209604,#209605,#209606,#209607,
#209608,#209609,#209610,#209611,#209612,#209613,#209614,#209615,#209616,
#209617,#209618,#209619,#209620,#209621,#209622,#209623,#209624,#209625,
#209626,#209627,#209628,#209629,#209630,#209631,#209632,#209633,#209634,
#209635,#209636,#209637,#209638,#209639,#209640,#209641,#209642,#209643,
#209644,#209645,#209646,#209647,#209648,#209649,#209650,#209651),
 .UNSPECIFIED.,.F.,.F.,(4,3,3,3,3,3,3,3,3,3,3,3,3,3,3,3,3,3,3,3,3,3,3,3,
3,3,3,3,3,3,3,3,3,3,3,3,3,3,3,3,3,3,3,3,3,3,3,3,3,3,3,3,4),(317.300858012569,
317.383320218654,317.465782076443,317.548243592784,317.630704774528,317.713165628524,
317.795626161623,317.878086380673,317.960546292524,318.043005904023,318.12546522202,
318.207924253362,318.290383004897,318.372841483474,318.455299695938,318.537757649138,
318.620215349921,318.702672805133,318.785130021621,318.87114260941,318.954467303831,
319.036933909389,319.11939967074,319.201864615298,319.284328770476,319.366792163684,
319.449254822327,319.531716773811,319.614178045537,319.696638664905,319.779098659313,
319.861558056154,319.944016882822,320.026475166709,320.108932935202,320.19139021569,
320.275524129139,320.357990127438,320.440454503986,320.522917368428,320.605378830385,
320.687838999459,320.770297985234,320.852755897277,320.938353013977,321.020817750921,
321.103279523219,321.18573876931,321.268195927489,321.350658446387,321.433116117671,
321.515574908579,321.53753283088),.UNSPECIFIED.);
#3462=B_SPLINE_CURVE_WITH_KNOTS('',3,(#209652,#209653,#209654,#209655,#209656,
#209657,#209658,#209659,#209660,#209661,#209662,#209663,#209664,#209665,
#209666,#209667,#209668,#209669,#209670,#209671,#209672,#209673,#209674,
#209675,#209676,#209677,#209678,#209679,#209680,#209681,#209682,#209683,
#209684,#209685,#209686,#209687,#209688,#209689,#209690,#209691,#209692,
#209693,#209694,#209695,#209696,#209697,#209698,#209699,#209700,#209701,
#209702,#209703,#209704,#209705,#209706,#209707,#209708,#209709,#209710,
#209711,#209712,#209713,#209714,#209715,#209716,#209717,#209718,#209719,
#209720,#209721,#209722,#209723,#209724,#209725,#209726,#209727,#209728,
#209729,#209730,#209731,#209732,#209733),.UNSPECIFIED.,.F.,.F.,(4,3,3,3,
3,3,3,3,3,3,3,3,3,3,3,3,3,3,3,3,3,3,3,3,3,3,3,4),(315.254829731915,315.336077616719,
315.413598032248,315.493001373132,315.572423144295,315.651874121936,315.731398288156,
315.810964198701,315.890614046905,315.912967900179,315.991346921049,316.069659672365,
316.147920568519,316.226143986317,316.304344274478,316.382552463643,316.460768517133,
316.539005434362,316.617276224517,316.69563980399,316.774052933449,316.852583315962,
316.911707636042,316.996155050202,317.080227623508,317.164072839184,317.247562802763,
317.300858012569),.UNSPECIFIED.);
#3463=B_SPLINE_CURVE_WITH_KNOTS('',3,(#209735,#209736,#209737,#209738,#209739,
#209740,#209741,#209742,#209743,#209744,#209745,#209746,#209747,#209748,
#209749,#209750,#209751,#209752,#209753,#209754,#209755,#209756,#209757,
#209758,#209759,#209760,#209761,#209762,#209763,#209764,#209765,#209766,
#209767,#209768,#209769,#209770,#209771,#209772,#209773,#209774,#209775,
#209776,#209777,#209778,#209779,#209780,#209781,#209782,#209783,#209784,
#209785,#209786,#209787,#209788,#209789,#209790,#209791,#209792,#209793,
#209794,#209795,#209796,#209797,#209798,#209799,#209800,#209801,#209802,
#209803,#209804,#209805,#209806,#209807,#209808,#209809,#209810),
 .UNSPECIFIED.,.F.,.F.,(4,3,3,3,3,3,3,3,3,3,3,3,3,3,3,3,3,3,3,3,3,3,3,3,
3,4),(315.254347523701,315.33680912722,315.419270064869,315.501730364046,
315.584190052149,315.66664915657,315.749107704702,315.831565723934,315.914023241655,
316.000698597585,316.083165382623,316.165630495219,316.248094045028,316.33055614168,
316.413016894785,316.495476413938,316.577934808711,316.660392188665,316.742858573359,
316.825321774004,316.907782229117,316.990240377063,317.072705978894,317.155165855869,
317.237629963513,317.300828936529),.UNSPECIFIED.);
#3464=B_SPLINE_CURVE_WITH_KNOTS('',3,(#209811,#209812,#209813,#209814,#209815,
#209816,#209817,#209818,#209819,#209820,#209821,#209822,#209823,#209824,
#209825,#209826,#209827,#209828,#209829,#209830,#209831,#209832,#209833,
#209834,#209835,#209836,#209837,#209838,#209839,#209840,#209841,#209842,
#209843,#209844,#209845,#209846,#209847,#209848,#209849,#209850,#209851,
#209852,#209853,#209854,#209855,#209856,#209857,#209858,#209859,#209860,
#209861,#209862,#209863,#209864,#209865,#209866,#209867,#209868,#209869,
#209870,#209871,#209872,#209873,#209874,#209875,#209876,#209877,#209878,
#209879,#209880,#209881,#209882,#209883,#209884,#209885,#209886,#209887,
#209888,#209889,#209890,#209891,#209892,#209893,#209894,#209895,#209896,
#209897,#209898,#209899,#209900,#209901,#209902,#209903,#209904,#209905,
#209906,#209907,#209908,#209909,#209910,#209911,#209912,#209913,#209914,
#209915,#209916,#209917,#209918,#209919,#209920,#209921,#209922,#209923,
#209924,#209925,#209926,#209927,#209928,#209929,#209930,#209931,#209932,
#209933,#209934,#209935,#209936,#209937,#209938,#209939,#209940,#209941,
#209942,#209943,#209944,#209945,#209946,#209947,#209948,#209949,#209950,
#209951,#209952,#209953,#209954,#209955,#209956,#209957,#209958,#209959,
#209960,#209961,#209962,#209963,#209964,#209965,#209966,#209967,#209968,
#209969,#209970,#209971,#209972,#209973,#209974,#209975,#209976,#209977,
#209978,#209979),.UNSPECIFIED.,.F.,.F.,(4,3,3,3,3,3,3,3,3,3,3,3,3,3,3,3,
3,3,3,3,3,3,3,3,3,3,3,3,3,3,3,3,3,3,3,3,3,3,3,3,3,3,3,3,3,3,3,3,3,3,3,3,
3,3,3,3,4),(317.301372217802,317.376455735683,317.451484791519,317.526477606148,
317.601448232661,317.676427587139,317.728761889578,317.813438227786,317.898260712299,
317.983283083175,318.068391964983,318.153621504358,318.228131757509,318.309688020169,
318.391168959835,318.475252126236,318.556577878748,318.642039752094,318.72750162544,
318.806904966324,318.886326737487,318.965777715128,319.045301881349,319.124867791894,
319.204517640097,319.226871493372,319.305250514242,319.383563265558,319.461824161712,
319.54004757951,319.618247867671,319.696456056835,319.774672110326,319.852909027555,
319.931179817709,320.009543397182,320.087956526641,320.166486909154,320.225611229234,
320.301667735988,320.377628553982,320.453510474601,320.529330208108,320.60510440244,
320.682510222772,320.758257978887,320.834012984415,320.909790249645,320.988430428508,
321.064339614977,321.140305606919,321.216377804529,321.224350965096,321.302732003581,
321.380196773245,321.459035946141,321.537875119036),.UNSPECIFIED.);
#3465=B_SPLINE_CURVE_WITH_KNOTS('',3,(#209985,#209986,#209987,#209988,#209989,
#209990,#209991,#209992,#209993,#209994,#209995,#209996,#209997,#209998,
#209999,#210000,#210001,#210002,#210003,#210004,#210005,#210006,#210007,
#210008,#210009,#210010,#210011,#210012,#210013,#210014,#210015,#210016,
#210017,#210018,#210019,#210020,#210021,#210022,#210023,#210024,#210025,
#210026,#210027,#210028,#210029,#210030,#210031,#210032,#210033,#210034,
#210035,#210036,#210037,#210038,#210039,#210040,#210041,#210042,#210043,
#210044,#210045,#210046,#210047,#210048,#210049,#210050,#210051,#210052,
#210053,#210054,#210055,#210056,#210057,#210058,#210059,#210060,#210061,
#210062,#210063,#210064,#210065,#210066,#210067,#210068,#210069,#210070,
#210071,#210072,#210073,#210074,#210075,#210076,#210077,#210078,#210079,
#210080,#210081,#210082,#210083,#210084,#210085,#210086,#210087,#210088,
#210089,#210090,#210091,#210092,#210093,#210094,#210095,#210096,#210097,
#210098,#210099,#210100,#210101,#210102,#210103,#210104,#210105,#210106,
#210107,#210108,#210109,#210110,#210111,#210112,#210113,#210114,#210115,
#210116,#210117,#210118,#210119,#210120,#210121,#210122,#210123,#210124,
#210125,#210126,#210127,#210128,#210129,#210130,#210131,#210132,#210133,
#210134,#210135,#210136,#210137,#210138,#210139,#210140,#210141,#210142,
#210143,#210144,#210145,#210146,#210147,#210148,#210149,#210150,#210151,
#210152,#210153),.UNSPECIFIED.,.F.,.F.,(4,3,3,3,3,3,3,3,3,3,3,3,3,3,3,3,
3,3,3,3,3,3,3,3,3,3,3,3,3,3,3,3,3,3,3,3,3,3,3,3,3,3,3,3,3,3,3,3,3,3,3,3,
3,3,3,3,4),(323.584043319749,323.68144335902,323.780080950349,323.879872029107,
323.902885787077,323.978942293831,324.054903111825,324.130785032444,324.206604765951,
324.282378960282,324.359784780614,324.43553253673,324.511287542258,324.587064807488,
324.665704986351,324.74161417282,324.817580164762,324.893652362372,324.901625522939,
324.979184374484,325.056650918379,325.134040821672,325.211369696365,325.288653110508,
325.365914157079,325.443164857923,325.520419260609,325.597691412141,325.675036750278,
325.752419524003,325.829909019651,325.900365258801,325.984584541694,326.068677220668,
326.152563846481,326.236320835868,326.319862538526,326.399735126732,326.477102322525,
326.554487911977,326.631905693764,326.709410615377,326.78696521463,326.864626561582,
326.899104994664,326.978728931666,327.058279322512,327.137768482614,327.217208680182,
327.296612065701,327.375994527022,327.455367152634,327.534741023188,327.614150901509,
327.693578847173,327.773065486166,327.820873168898),.UNSPECIFIED.);
#3466=B_SPLINE_CURVE_WITH_KNOTS('',3,(#210154,#210155,#210156,#210157,#210158,
#210159,#210160,#210161,#210162,#210163,#210164,#210165,#210166,#210167,
#210168,#210169,#210170,#210171,#210172,#210173,#210174,#210175,#210176,
#210177,#210178,#210179,#210180,#210181,#210182,#210183,#210184,#210185,
#210186,#210187,#210188,#210189,#210190,#210191,#210192,#210193,#210194,
#210195,#210196,#210197,#210198,#210199,#210200,#210201,#210202,#210203,
#210204,#210205,#210206,#210207,#210208,#210209,#210210,#210211,#210212,
#210213,#210214,#210215,#210216,#210217,#210218,#210219,#210220,#210221,
#210222,#210223,#210224,#210225,#210226,#210227,#210228,#210229),
 .UNSPECIFIED.,.F.,.F.,(4,3,3,3,3,3,3,3,3,3,3,3,3,3,3,3,3,3,3,3,3,3,3,3,
3,4),(321.53753283088,321.619994434639,321.702455372518,321.784915671916,
321.867375360229,321.949834464851,322.032293013174,322.114751032588,322.197208550481,
322.283885723561,322.366352509169,322.448817622301,322.531281172607,322.613743269721,
322.696204023253,322.778663542796,322.861121937922,322.943579318193,323.026045704013,
323.108508905637,323.190969361585,323.273427510222,323.355893114233,323.438352992811,
323.520817104547,323.584043319749),.UNSPECIFIED.);
#3467=B_SPLINE_CURVE_WITH_KNOTS('',3,(#210231,#210232,#210233,#210234,#210235,
#210236,#210237,#210238,#210239,#210240,#210241,#210242,#210243,#210244,
#210245,#210246,#210247,#210248,#210249,#210250,#210251,#210252,#210253,
#210254,#210255,#210256,#210257,#210258,#210259,#210260,#210261,#210262,
#210263,#210264,#210265,#210266,#210267,#210268,#210269,#210270,#210271,
#210272,#210273,#210274,#210275,#210276,#210277,#210278,#210279,#210280,
#210281,#210282,#210283,#210284,#210285,#210286,#210287,#210288,#210289,
#210290,#210291,#210292,#210293,#210294,#210295,#210296,#210297,#210298,
#210299,#210300,#210301,#210302,#210303,#210304,#210305,#210306,#210307,
#210308,#210309),.UNSPECIFIED.,.F.,.F.,(4,3,3,3,3,3,3,3,3,3,3,3,3,3,3,3,
3,3,3,3,3,3,3,3,3,3,4),(321.537875119036,321.615156708834,321.692416922816,
321.76966747806,321.846922421929,321.924195801598,322.001542675429,322.078927602483,
322.156418288634,322.223090700958,322.307309983851,322.391402662824,322.475289288637,
322.559046278023,322.642587980681,322.722460568889,322.799827764682,322.877213354133,
322.95463113592,323.032136057532,323.109690656785,323.187352003737,323.22183043682,
323.31390668278,323.405745640809,323.496945780501,323.584043319749),
 .UNSPECIFIED.);
#3468=B_SPLINE_CURVE_WITH_KNOTS('',3,(#210310,#210311,#210312,#210313,#210314,
#210315,#210316,#210317,#210318,#210319,#210320,#210321,#210322,#210323,
#210324,#210325,#210326,#210327,#210328,#210329,#210330,#210331,#210332,
#210333,#210334,#210335,#210336,#210337,#210338,#210339,#210340,#210341,
#210342,#210343,#210344,#210345,#210346,#210347,#210348,#210349,#210350,
#210351,#210352,#210353,#210354,#210355,#210356,#210357,#210358,#210359,
#210360,#210361,#210362,#210363,#210364,#210365,#210366,#210367,#210368,
#210369,#210370,#210371,#210372,#210373,#210374,#210375,#210376,#210377,
#210378,#210379,#210380,#210381,#210382,#210383,#210384,#210385,#210386,
#210387,#210388,#210389,#210390,#210391,#210392,#210393,#210394,#210395,
#210396,#210397,#210398,#210399,#210400,#210401,#210402,#210403,#210404,
#210405,#210406,#210407,#210408,#210409,#210410,#210411,#210412,#210413,
#210414,#210415,#210416,#210417,#210418,#210419,#210420,#210421,#210422,
#210423,#210424,#210425,#210426,#210427,#210428,#210429,#210430,#210431,
#210432,#210433,#210434,#210435,#210436,#210437,#210438,#210439,#210440,
#210441,#210442,#210443,#210444,#210445,#210446,#210447,#210448,#210449,
#210450,#210451,#210452,#210453,#210454,#210455,#210456,#210457,#210458,
#210459,#210460,#210461,#210462,#210463,#210464,#210465,#210466),
 .UNSPECIFIED.,.F.,.F.,(4,3,3,3,3,3,3,3,3,3,3,3,3,3,3,3,3,3,3,3,3,3,3,3,
3,3,3,3,3,3,3,3,3,3,3,3,3,3,3,3,3,3,3,3,3,3,3,3,3,3,3,3,4),(323.584043319749,
323.666505525835,323.748967383623,323.831428899964,323.913890081708,323.996350935704,
324.078811468803,324.161271687853,324.243731599704,324.326191211203,324.4086505292,
324.491109560542,324.573568312077,324.656026790653,324.738485003118,324.820942956318,
324.903400657101,324.985858112313,325.0683153288,325.154327916589,325.23765261101,
325.320119216569,325.402584977919,325.485049922478,325.567514077656,325.649977470863,
325.732440129506,325.81490208099,325.897363352717,325.979823972085,326.062283966492,
326.144743363333,326.227202190002,326.309660473888,326.392118242381,326.474575522869,
326.558709436318,326.641175434617,326.723639811166,326.806102675608,326.888564137564,
326.971024306638,327.053483292413,327.135941204456,327.221538321156,327.3040030581,
327.386464830398,327.468924076489,327.551381234668,327.633843753567,327.71630142485,
327.798760215758,327.82071813806),.UNSPECIFIED.);
#3469=B_SPLINE_CURVE_WITH_KNOTS('',3,(#210472,#210473,#210474,#210475,#210476,
#210477,#210478,#210479,#210480,#210481,#210482,#210483,#210484,#210485,
#210486,#210487,#210488,#210489,#210490,#210491,#210492,#210493,#210494,
#210495,#210496,#210497,#210498,#210499,#210500,#210501,#210502,#210503,
#210504,#210505,#210506,#210507,#210508,#210509,#210510,#210511,#210512,
#210513,#210514,#210515,#210516,#210517,#210518,#210519,#210520,#210521,
#210522,#210523,#210524,#210525,#210526,#210527,#210528,#210529,#210530,
#210531,#210532,#210533,#210534,#210535,#210536,#210537,#210538,#210539,
#210540,#210541,#210542,#210543,#210544,#210545,#210546,#210547,#210548,
#210549,#210550,#210551,#210552,#210553,#210554,#210555,#210556,#210557,
#210558,#210559,#210560,#210561,#210562,#210563,#210564,#210565,#210566,
#210567,#210568,#210569,#210570,#210571,#210572,#210573,#210574,#210575,
#210576,#210577,#210578,#210579,#210580,#210581,#210582,#210583,#210584,
#210585,#210586,#210587,#210588,#210589,#210590,#210591,#210592,#210593,
#210594,#210595,#210596,#210597,#210598,#210599,#210600,#210601,#210602,
#210603,#210604,#210605,#210606,#210607,#210608,#210609,#210610,#210611,
#210612,#210613,#210614,#210615,#210616,#210617,#210618,#210619,#210620,
#210621,#210622,#210623,#210624,#210625,#210626,#210627,#210628,#210629,
#210630,#210631,#210632,#210633,#210634,#210635,#210636,#210637,#210638,
#210639,#210640,#210641,#210642,#210643),.UNSPECIFIED.,.F.,.F.,(4,3,3,3,
3,3,3,3,3,3,3,3,3,3,3,3,3,3,3,3,3,3,3,3,3,3,3,3,3,3,3,3,3,3,3,3,3,3,3,3,
3,3,3,3,3,3,3,3,3,3,3,3,3,3,3,3,3,4),(329.867228627072,329.89532420225,
329.97370322312,330.052015974436,330.130276870589,330.208500288388,330.286700576548,
330.364908765713,330.443124819203,330.521361736433,330.599632526587,330.67799610606,
330.756409235519,330.834939618032,330.894063938112,330.970120444866,331.04608126286,
331.121963183479,331.197782916987,331.273557111318,331.35096293165,331.426710687765,
331.502465693293,331.578242958524,331.656883137386,331.732792323855,331.808758315797,
331.884830513407,331.892803673974,331.970362525519,332.047829069414,332.125218972707,
332.2025478474,332.279831261543,332.357092308115,332.434343008959,332.511597411645,
332.588869563177,332.666214901314,332.743597675039,332.821087170687,332.891543409837,
332.97576269273,333.059855371704,333.143741997517,333.227498986904,333.311040689562,
333.390913277768,333.468280473561,333.545666063012,333.6230838448,333.700588766412,
333.778143365665,333.855804712617,333.890283145699,333.969909993848,334.049453245317,
334.104148056147),.UNSPECIFIED.);
#3470=B_SPLINE_CURVE_WITH_KNOTS('',3,(#210644,#210645,#210646,#210647,#210648,
#210649,#210650,#210651,#210652,#210653,#210654,#210655,#210656,#210657,
#210658,#210659,#210660,#210661,#210662,#210663,#210664,#210665,#210666,
#210667,#210668,#210669,#210670,#210671,#210672,#210673,#210674,#210675,
#210676,#210677,#210678,#210679,#210680,#210681,#210682,#210683,#210684,
#210685,#210686,#210687,#210688,#210689,#210690,#210691,#210692,#210693,
#210694,#210695,#210696,#210697,#210698,#210699,#210700,#210701,#210702,
#210703,#210704,#210705,#210706,#210707,#210708,#210709,#210710,#210711,
#210712,#210713,#210714,#210715,#210716,#210717,#210718,#210719,#210720,
#210721,#210722),.UNSPECIFIED.,.F.,.F.,(4,3,3,3,3,3,3,3,3,3,3,3,3,3,3,3,
3,3,3,3,3,3,3,3,3,3,4),(327.820873168898,327.897844730526,327.974559737375,
328.051207649739,328.127803161478,328.204362059176,328.280899443255,328.357440963707,
328.397214598457,328.481890936665,328.566713421179,328.651735792055,328.736844673863,
328.822074213238,328.896584466388,328.978140729048,329.059621668714,329.143704835115,
329.225030587627,329.310492460973,329.395954334319,329.474589036795,329.553236576592,
329.631945717837,329.710684832125,329.789516502116,329.867228626929),
 .UNSPECIFIED.);
#3471=B_SPLINE_CURVE_WITH_KNOTS('',3,(#210724,#210725,#210726,#210727,#210728,
#210729,#210730,#210731,#210732,#210733,#210734,#210735,#210736,#210737,
#210738,#210739,#210740,#210741,#210742,#210743,#210744,#210745,#210746,
#210747,#210748,#210749,#210750,#210751,#210752,#210753,#210754,#210755,
#210756,#210757,#210758,#210759,#210760,#210761,#210762,#210763,#210764,
#210765,#210766,#210767,#210768,#210769,#210770,#210771,#210772,#210773,
#210774,#210775,#210776,#210777,#210778,#210779,#210780,#210781,#210782,
#210783,#210784,#210785,#210786,#210787,#210788,#210789,#210790,#210791,
#210792,#210793,#210794,#210795,#210796,#210797,#210798,#210799),
 .UNSPECIFIED.,.F.,.F.,(4,3,3,3,3,3,3,3,3,3,3,3,3,3,3,3,3,3,3,3,3,3,3,3,
3,4),(327.82071813806,327.903179741818,327.985640679697,328.068100979095,
328.150560667408,328.233019772031,328.315478320354,328.397936339768,328.480393857661,
328.56707103074,328.649537816349,328.73200292948,328.814466479787,328.896928576901,
328.979389330433,329.061848849975,329.144307245102,329.226764625373,329.309231011192,
329.391694212816,329.474154668765,329.556612817401,329.639078421413,329.72153829999,
329.804002411727,329.867228626928),.UNSPECIFIED.);
#3472=B_SPLINE_CURVE_WITH_KNOTS('',3,(#210800,#210801,#210802,#210803,#210804,
#210805,#210806,#210807,#210808,#210809),.UNSPECIFIED.,.F.,.F.,(4,1,1,1,
1,1,1,4),(329.867228626928,330.213008587855,331.211748323718,331.711118191649,
332.21048805958,332.709857927511,333.209227795442,334.10365230637),
 .UNSPECIFIED.);
#3473=B_SPLINE_CURVE_WITH_KNOTS('',3,(#210815,#210816,#210817,#210818,#210819,
#210820,#210821,#210822,#210823,#210824,#210825,#210826,#210827,#210828,
#210829,#210830,#210831,#210832,#210833,#210834,#210835,#210836,#210837,
#210838,#210839,#210840,#210841,#210842,#210843,#210844,#210845,#210846,
#210847,#210848,#210849,#210850,#210851,#210852,#210853,#210854,#210855,
#210856,#210857,#210858,#210859,#210860,#210861,#210862,#210863,#210864,
#210865,#210866,#210867,#210868,#210869,#210870,#210871,#210872,#210873,
#210874,#210875,#210876,#210877,#210878,#210879,#210880,#210881,#210882,
#210883,#210884,#210885,#210886,#210887,#210888,#210889,#210890,#210891,
#210892,#210893,#210894,#210895,#210896,#210897,#210898,#210899,#210900,
#210901,#210902,#210903,#210904,#210905,#210906,#210907,#210908,#210909,
#210910,#210911,#210912,#210913,#210914,#210915,#210916,#210917,#210918,
#210919,#210920,#210921,#210922,#210923,#210924,#210925,#210926,#210927,
#210928,#210929,#210930,#210931,#210932,#210933,#210934,#210935,#210936,
#210937,#210938,#210939,#210940,#210941,#210942,#210943,#210944,#210945,
#210946,#210947,#210948,#210949,#210950,#210951,#210952,#210953,#210954,
#210955,#210956,#210957,#210958,#210959,#210960,#210961,#210962,#210963,
#210964,#210965,#210966,#210967,#210968,#210969,#210970,#210971),
 .UNSPECIFIED.,.F.,.F.,(4,3,3,3,3,3,3,3,3,3,3,3,3,3,3,3,3,3,3,3,3,3,3,3,
3,3,3,3,3,3,3,3,3,3,3,3,3,3,3,3,3,3,3,3,3,3,3,3,3,3,3,3,4),(336.150413934108,
336.232876140193,336.315337997982,336.397799514323,336.480260696067,336.562721550063,
336.645182083162,336.727642302212,336.810102214063,336.892561825562,336.975021143559,
337.057480174901,337.139938926436,337.222397405013,337.304855617477,337.387313570677,
337.46977127146,337.552228726672,337.634685943159,337.720698530948,337.804023225369,
337.886489830928,337.968955592278,338.051420536837,338.133884692015,338.216348085222,
338.298810743865,338.381272695349,338.463733967076,338.546194586444,338.628654580851,
338.711113977693,338.793572804361,338.876031088247,338.958488856741,339.040946137228,
339.125080050678,339.207546048976,339.290010425525,339.372473289967,339.454934751924,
339.537394920998,339.619853906772,339.702311818815,339.787908935516,339.870373672459,
339.952835444758,340.035294690849,340.117751849027,340.200214367926,340.28267203921,
340.365130830118,340.387088752419),.UNSPECIFIED.);
#3474=B_SPLINE_CURVE_WITH_KNOTS('',3,(#210972,#210973,#210974,#210975,#210976,
#210977,#210978,#210979,#210980,#210981,#210982,#210983,#210984,#210985,
#210986,#210987,#210988,#210989,#210990,#210991,#210992,#210993,#210994,
#210995,#210996,#210997,#210998,#210999,#211000,#211001,#211002,#211003,
#211004,#211005,#211006,#211007,#211008,#211009,#211010,#211011,#211012,
#211013,#211014,#211015,#211016,#211017,#211018,#211019,#211020,#211021,
#211022,#211023,#211024,#211025,#211026,#211027,#211028,#211029,#211030,
#211031,#211032,#211033,#211034,#211035,#211036,#211037,#211038,#211039,
#211040,#211041,#211042,#211043,#211044,#211045,#211046,#211047,#211048,
#211049,#211050),.UNSPECIFIED.,.F.,.F.,(4,3,3,3,3,3,3,3,3,3,3,3,3,3,3,3,
3,3,3,3,3,3,3,3,3,3,4),(334.104148056147,334.183600716777,334.263013462116,
334.342403745438,334.421781588549,334.501158074259,334.580544283132,334.659982760416,
334.739446410458,334.818988270721,334.889022881561,334.96573788841,335.042385800774,
335.118981312513,335.195540210211,335.272077594291,335.348619114743,335.388392749492,
335.4730690877,335.557891572214,335.64291394309,335.728022824899,335.813252364273,
335.887762617423,335.973697967041,336.062055950575,336.150413934108),
 .UNSPECIFIED.);
#3475=B_SPLINE_CURVE_WITH_KNOTS('',3,(#211052,#211053,#211054,#211055,#211056,
#211057),.UNSPECIFIED.,.F.,.F.,(4,1,1,4),(334.10365230637,334.207967531304,
335.206707267166,336.150408590058),.UNSPECIFIED.);
#3476=B_SPLINE_CURVE_WITH_KNOTS('',3,(#211058,#211059,#211060,#211061,#211062,
#211063,#211064,#211065,#211066,#211067,#211068,#211069,#211070,#211071,
#211072,#211073,#211074,#211075,#211076,#211077,#211078,#211079,#211080,
#211081,#211082,#211083,#211084,#211085,#211086,#211087,#211088,#211089,
#211090,#211091,#211092,#211093,#211094,#211095,#211096,#211097,#211098,
#211099,#211100,#211101,#211102,#211103,#211104,#211105,#211106,#211107,
#211108,#211109,#211110,#211111,#211112,#211113,#211114,#211115,#211116,
#211117,#211118,#211119,#211120,#211121,#211122,#211123,#211124,#211125,
#211126,#211127,#211128,#211129,#211130,#211131,#211132,#211133,#211134,
#211135,#211136,#211137,#211138,#211139,#211140,#211141,#211142,#211143,
#211144,#211145,#211146,#211147,#211148,#211149,#211150,#211151,#211152,
#211153,#211154,#211155,#211156,#211157,#211158,#211159,#211160,#211161,
#211162,#211163,#211164,#211165,#211166,#211167,#211168,#211169,#211170,
#211171,#211172,#211173,#211174,#211175,#211176,#211177,#211178,#211179,
#211180,#211181,#211182,#211183,#211184,#211185,#211186,#211187,#211188,
#211189,#211190,#211191,#211192,#211193,#211194,#211195,#211196,#211197,
#211198,#211199,#211200,#211201,#211202,#211203,#211204,#211205,#211206,
#211207,#211208,#211209,#211210,#211211,#211212,#211213,#211214,#211215,
#211216,#211217,#211218,#211219,#211220,#211221,#211222,#211223,#211224,
#211225,#211226),.UNSPECIFIED.,.F.,.F.,(4,3,3,3,3,3,3,3,3,3,3,3,3,3,3,3,
3,3,3,3,3,3,3,3,3,3,3,3,3,3,3,3,3,3,3,3,3,3,3,3,3,3,3,3,3,3,3,3,3,3,3,3,
3,3,3,3,4),(336.150413934108,336.205447003029,336.289666285922,336.373758964895,
336.457645590708,336.541402580095,336.624944282753,336.70481687096,336.782184066753,
336.859569656204,336.936987437992,337.014492359605,337.092046958857,337.169708305809,
337.204186738891,337.283807477635,337.363355305291,337.442842534567,337.52228143148,
337.601684224287,337.681069437185,337.760445667738,337.839823997288,337.919215507159,
337.99866074199,338.078134322771,338.157681434821,338.202926474753,338.279641481602,
338.356289393966,338.432884905705,338.509443803403,338.585981187482,338.662522707934,
338.702296342684,338.786972680892,338.871795165406,338.956817536282,339.04192641809,
339.127155957465,339.201666210615,339.283222473274,339.36470341294,339.448786579342,
339.530112331853,339.6155742052,339.701036078546,339.780439419431,339.859861190593,
339.939312168234,340.018836334454,340.098402245,340.178052093203,340.200405946477,
340.278794595193,340.357108620971,340.387341982143),.UNSPECIFIED.);
#3477=B_SPLINE_CURVE_WITH_KNOTS('',3,(#211232,#211233,#211234,#211235,#211236,
#211237,#211238,#211239,#211240,#211241,#211242,#211243,#211244,#211245,
#211246,#211247,#211248,#211249,#211250,#211251,#211252,#211253,#211254,
#211255,#211256,#211257,#211258,#211259,#211260,#211261,#211262,#211263,
#211264,#211265,#211266,#211267,#211268,#211269,#211270,#211271,#211272,
#211273,#211274,#211275,#211276,#211277,#211278,#211279,#211280,#211281,
#211282,#211283,#211284,#211285,#211286,#211287,#211288,#211289,#211290,
#211291,#211292,#211293,#211294,#211295,#211296,#211297,#211298,#211299,
#211300,#211301,#211302,#211303,#211304,#211305,#211306,#211307,#211308,
#211309,#211310,#211311,#211312,#211313,#211314,#211315,#211316,#211317,
#211318,#211319,#211320,#211321,#211322,#211323,#211324,#211325,#211326,
#211327,#211328,#211329,#211330,#211331,#211332,#211333,#211334,#211335,
#211336,#211337,#211338,#211339,#211340,#211341,#211342,#211343,#211344,
#211345,#211346,#211347,#211348,#211349,#211350,#211351,#211352,#211353,
#211354,#211355,#211356,#211357,#211358,#211359,#211360,#211361,#211362,
#211363,#211364,#211365,#211366,#211367,#211368,#211369,#211370,#211371,
#211372,#211373,#211374,#211375,#211376,#211377,#211378,#211379,#211380,
#211381,#211382,#211383,#211384,#211385,#211386,#211387,#211388,#211389,
#211390,#211391,#211392,#211393,#211394,#211395,#211396,#211397,#211398,
#211399,#211400,#211401,#211402,#211403),.UNSPECIFIED.,.F.,.F.,(4,3,3,3,
3,3,3,3,3,3,3,3,3,3,3,3,3,3,3,3,3,3,3,3,3,3,3,3,3,3,3,3,3,3,3,3,3,3,3,3,
3,3,3,3,3,3,3,3,3,3,3,3,3,3,3,3,3,4),(342.433599241288,342.518884947016,
342.604327876792,342.689963352961,342.775685721844,342.86150384477,342.878940768458,
342.960497031118,343.041977970784,343.126061137185,343.207386889697,343.292848763043,
343.37831063639,343.457713977275,343.537135748437,343.616586726078,343.696110892299,
343.775676802844,343.855326651047,343.877680504321,343.956059525191,344.034372276507,
344.11263317266,344.19085659046,344.26905687862,344.347265067784,344.425481121274,
344.503718038504,344.581988828658,344.660352408131,344.73876553759,344.817295920103,
344.876420240183,344.952476746937,345.028437564931,345.10431948555,345.180139219057,
345.255913413388,345.33331923372,345.409066989835,345.484821995364,345.560599260594,
345.639239439457,345.715148625926,345.791114617868,345.867186815478,345.875159976045,
345.952730916243,346.030207285946,346.110132834588,346.187454824317,346.264735602648,
346.341989243777,346.419229803829,346.49648848957,346.573758516221,346.65107369651,
346.669611675086),.UNSPECIFIED.);
#3478=B_SPLINE_CURVE_WITH_KNOTS('',3,(#211404,#211405,#211406,#211407,#211408,
#211409,#211410,#211411,#211412,#211413,#211414,#211415,#211416,#211417,
#211418,#211419,#211420,#211421,#211422,#211423,#211424,#211425,#211426,
#211427,#211428,#211429,#211430,#211431,#211432,#211433,#211434,#211435,
#211436,#211437,#211438,#211439,#211440,#211441,#211442,#211443,#211444,
#211445,#211446,#211447,#211448,#211449,#211450,#211451,#211452,#211453,
#211454,#211455,#211456,#211457,#211458,#211459,#211460,#211461,#211462,
#211463,#211464,#211465,#211466,#211467,#211468,#211469,#211470,#211471,
#211472,#211473,#211474,#211475,#211476,#211477,#211478,#211479),
 .UNSPECIFIED.,.F.,.F.,(4,3,3,3,3,3,3,3,3,3,3,3,3,3,3,3,3,3,3,3,3,3,3,3,
3,4),(340.387088752419,340.469550356178,340.552011294057,340.634471593455,
340.716931281768,340.79939038639,340.881848934713,340.964306954127,341.04676447202,
341.1334416451,341.215908430708,341.298373543839,341.380837094146,341.46329919126,
341.545759944792,341.628219464335,341.710677859461,341.793135239732,341.875601625552,
341.958064827176,342.040525283124,342.122983431761,342.205449035772,342.28790891435,
342.370373026086,342.433599241288),.UNSPECIFIED.);
#3479=B_SPLINE_CURVE_WITH_KNOTS('',3,(#211481,#211482,#211483,#211484,#211485,
#211486,#211487,#211488,#211489,#211490,#211491,#211492,#211493,#211494,
#211495,#211496,#211497,#211498,#211499,#211500,#211501,#211502,#211503,
#211504,#211505,#211506,#211507,#211508,#211509,#211510,#211511,#211512,
#211513,#211514,#211515,#211516,#211517,#211518,#211519,#211520,#211521,
#211522,#211523,#211524,#211525,#211526,#211527,#211528,#211529,#211530,
#211531,#211532,#211533,#211534,#211535,#211536,#211537,#211538,#211539,
#211540,#211541,#211542,#211543,#211544,#211545,#211546,#211547,#211548,
#211549,#211550,#211551,#211552,#211553,#211554,#211555,#211556,#211557,
#211558,#211559,#211560,#211561,#211562,#211563,#211564,#211565),
 .UNSPECIFIED.,.F.,.F.,(4,3,3,3,3,3,3,3,3,3,3,3,3,3,3,3,3,3,3,3,3,3,3,3,
3,3,3,3,4),(340.387341982143,340.465586694626,340.543799475709,340.625717751538,
340.703927756916,340.782151266517,340.860401283073,340.938690822348,341.017074441985,
341.095512723419,341.17405872535,341.19914568234,341.275202189094,341.351163007088,
341.427044927707,341.502864661214,341.578638855545,341.656044675877,341.731792431993,
341.807547437521,341.883324702751,341.961964881614,342.037874068083,342.113840060025,
342.189912257635,342.197885418202,342.315742329745,342.42587465463,342.433599241287),
 .UNSPECIFIED.);
#3480=B_SPLINE_CURVE_WITH_KNOTS('',3,(#211566,#211567,#211568,#211569,#211570,
#211571,#211572,#211573,#211574,#211575,#211576,#211577,#211578,#211579,
#211580,#211581,#211582,#211583,#211584,#211585,#211586,#211587,#211588,
#211589,#211590,#211591,#211592,#211593,#211594,#211595,#211596,#211597,
#211598,#211599,#211600,#211601,#211602,#211603,#211604,#211605,#211606,
#211607,#211608,#211609,#211610,#211611,#211612,#211613,#211614,#211615,
#211616,#211617,#211618,#211619,#211620,#211621,#211622,#211623,#211624,
#211625,#211626,#211627,#211628,#211629,#211630,#211631,#211632,#211633,
#211634,#211635,#211636,#211637,#211638,#211639,#211640,#211641,#211642,
#211643,#211644,#211645,#211646,#211647,#211648,#211649,#211650,#211651,
#211652,#211653,#211654,#211655,#211656,#211657,#211658,#211659,#211660,
#211661,#211662,#211663,#211664,#211665,#211666,#211667,#211668,#211669,
#211670,#211671,#211672,#211673,#211674,#211675,#211676,#211677,#211678,
#211679,#211680,#211681,#211682,#211683,#211684,#211685,#211686,#211687,
#211688,#211689,#211690,#211691,#211692,#211693,#211694,#211695,#211696,
#211697,#211698,#211699,#211700,#211701,#211702,#211703,#211704,#211705,
#211706,#211707,#211708,#211709,#211710,#211711,#211712,#211713,#211714,
#211715,#211716,#211717,#211718,#211719,#211720,#211721,#211722,#211723,
#211724,#211725,#211726,#211727,#211728,#211729,#211730,#211731),
 .UNSPECIFIED.,.F.,.F.,(4,3,3,3,3,3,3,3,3,3,3,3,3,3,3,3,3,3,3,3,3,3,3,3,
3,3,3,3,3,3,3,3,3,3,3,3,3,3,3,3,3,3,3,3,3,3,3,3,3,3,3,3,3,3,3,4),(342.433599241378,
342.509334181514,342.585008870166,342.661460905653,342.737073109975,342.812679087942,
342.888293962241,342.965376760197,343.041089123994,343.118857139029,343.196625154064,
343.280844436957,343.364937115931,343.448823741744,343.532580731131,343.616122433789,
343.695995021995,343.773362217788,343.850747807239,343.928165589027,344.005670510639,
344.083225109892,344.160886456844,344.195364889926,344.27498562867,344.354533456326,
344.434020685602,344.513459582515,344.592862375321,344.67224758822,344.751623818773,
344.831002148323,344.910393658194,344.989838893025,345.069312473806,345.148859585856,
345.194104625788,345.270819632637,345.347467545,345.424063056739,345.500621954437,
345.577159338516,345.653700858968,345.693474493719,345.778150831927,345.862973316441,
345.947995687317,346.033104569126,346.118334108501,346.19284436165,346.274402663091,
346.355885589217,346.437274666338,346.518605081455,346.599864769658,346.670532447169),
 .UNSPECIFIED.);
#3481=B_SPLINE_CURVE_WITH_KNOTS('',3,(#211737,#211738,#211739,#211740,#211741,
#211742,#211743,#211744,#211745,#211746,#211747,#211748,#211749,#211750,
#211751,#211752,#211753,#211754,#211755,#211756,#211757,#211758,#211759,
#211760,#211761,#211762,#211763,#211764,#211765,#211766,#211767,#211768,
#211769,#211770,#211771,#211772,#211773,#211774,#211775,#211776,#211777,
#211778,#211779,#211780,#211781,#211782,#211783,#211784,#211785,#211786,
#211787,#211788,#211789,#211790,#211791,#211792,#211793,#211794,#211795,
#211796,#211797,#211798,#211799,#211800,#211801,#211802,#211803,#211804,
#211805,#211806,#211807,#211808,#211809,#211810,#211811,#211812,#211813,
#211814,#211815,#211816,#211817,#211818,#211819,#211820,#211821,#211822,
#211823,#211824,#211825,#211826,#211827,#211828,#211829,#211830,#211831,
#211832,#211833,#211834,#211835,#211836,#211837,#211838,#211839,#211840,
#211841,#211842,#211843,#211844,#211845,#211846,#211847,#211848,#211849,
#211850,#211851,#211852,#211853,#211854,#211855,#211856,#211857,#211858,
#211859,#211860,#211861,#211862,#211863,#211864,#211865,#211866,#211867,
#211868,#211869,#211870,#211871,#211872,#211873,#211874,#211875,#211876,
#211877,#211878,#211879,#211880,#211881,#211882,#211883,#211884,#211885,
#211886,#211887,#211888,#211889,#211890,#211891,#211892,#211893),
 .UNSPECIFIED.,.F.,.F.,(4,3,3,3,3,3,3,3,3,3,3,3,3,3,3,3,3,3,3,3,3,3,3,3,
3,3,3,3,3,3,3,3,3,3,3,3,3,3,3,3,3,3,3,3,3,3,3,3,3,3,3,3,4),(348.716784548467,
348.799246754552,348.881708612341,348.964170128682,349.046631310426,349.129092164422,
349.211552697521,349.294012916571,349.376472828422,349.458932439921,349.541391757918,
349.62385078926,349.706309540795,349.788768019372,349.871226231836,349.953684185037,
350.036141885819,350.118599341031,350.201056557519,350.287069145308,350.370393839729,
350.452860445287,350.535326206638,350.617791151196,350.700255306374,350.782718699581,
350.865181358225,350.947643309709,351.030104581435,351.112565200803,351.195025195211,
351.277484592052,351.35994341872,351.442401702607,351.5248594711,351.607316751588,
351.691450665037,351.773916663336,351.856381039885,351.938843904326,352.021305366283,
352.103765535357,352.186224521132,352.268682433175,352.354279549875,352.436744286819,
352.519206059117,352.601665305208,352.684122463387,352.766584982286,352.849042653569,
352.931501444477,352.953459366778),.UNSPECIFIED.);
#3482=B_SPLINE_CURVE_WITH_KNOTS('',3,(#211894,#211895,#211896,#211897,#211898,
#211899,#211900,#211901,#211902,#211903,#211904,#211905,#211906,#211907,
#211908,#211909,#211910,#211911,#211912,#211913,#211914,#211915,#211916,
#211917,#211918,#211919,#211920,#211921,#211922,#211923,#211924,#211925,
#211926,#211927,#211928,#211929,#211930,#211931,#211932,#211933,#211934,
#211935,#211936,#211937,#211938,#211939,#211940,#211941,#211942,#211943,
#211944,#211945,#211946,#211947,#211948,#211949,#211950,#211951,#211952,
#211953,#211954,#211955,#211956,#211957,#211958,#211959,#211960,#211961,
#211962,#211963,#211964,#211965,#211966,#211967,#211968,#211969,#211970,
#211971,#211972,#211973,#211974,#211975),.UNSPECIFIED.,.F.,.F.,(4,3,3,3,
3,3,3,3,3,3,3,3,3,3,3,3,3,3,3,3,3,3,3,3,3,3,3,4),(346.669611675086,346.747006816302,
346.824503410128,346.873899711907,346.9581189948,347.042211673773,347.126098299586,
347.209855288973,347.293396991631,347.373269579838,347.450636775631,347.528022365082,
347.60544014687,347.682945068483,347.760499667735,347.838161014688,347.872639447769,
347.951128287047,348.029541293079,348.107892883974,348.186194357667,348.264468019272,
348.342726853174,348.420983832666,348.499278733754,348.577592411052,348.655974971976,
348.716634548041),.UNSPECIFIED.);
#3483=B_SPLINE_CURVE_WITH_KNOTS('',3,(#211977,#211978,#211979,#211980,#211981,
#211982,#211983,#211984,#211985,#211986,#211987,#211988,#211989,#211990,
#211991,#211992,#211993,#211994,#211995,#211996,#211997,#211998,#211999,
#212000,#212001,#212002,#212003,#212004,#212005,#212006,#212007,#212008,
#212009,#212010,#212011,#212012,#212013,#212014,#212015,#212016,#212017,
#212018,#212019,#212020,#212021,#212022,#212023,#212024,#212025,#212026,
#212027,#212028,#212029,#212030,#212031,#212032,#212033,#212034,#212035,
#212036,#212037,#212038,#212039,#212040,#212041,#212042,#212043,#212044,
#212045,#212046,#212047,#212048,#212049,#212050,#212051,#212052,#212053,
#212054,#212055,#212056,#212057,#212058,#212059,#212060,#212061),
 .UNSPECIFIED.,.F.,.F.,(4,3,3,3,3,3,3,3,3,3,3,3,3,3,3,3,3,3,3,3,3,3,3,3,
3,3,3,3,4),(346.670532447169,346.692214229582,346.771617570467,346.851039341629,
346.930490319271,347.010014485491,347.089580396036,347.169230244239,347.191584097513,
347.269963118383,347.348275869698,347.426536765852,347.504760183652,347.582960471812,
347.661168660977,347.739384714467,347.817621631696,347.89589242185,347.974256001323,
348.052669130781,348.131199513294,348.190323833375,348.269008312196,348.347569787422,
348.426020943107,348.504342215918,348.582588647594,348.660753693213,348.716784548467),
 .UNSPECIFIED.);
#3484=B_SPLINE_CURVE_WITH_KNOTS('',3,(#212062,#212063,#212064,#212065,#212066,
#212067,#212068,#212069,#212070,#212071,#212072,#212073,#212074,#212075,
#212076,#212077,#212078,#212079,#212080,#212081,#212082,#212083,#212084,
#212085,#212086,#212087,#212088,#212089,#212090,#212091,#212092,#212093,
#212094,#212095,#212096,#212097,#212098,#212099,#212100,#212101,#212102,
#212103,#212104,#212105,#212106,#212107,#212108,#212109,#212110,#212111,
#212112,#212113,#212114,#212115,#212116,#212117,#212118,#212119,#212120,
#212121,#212122,#212123,#212124,#212125,#212126,#212127,#212128,#212129,
#212130,#212131,#212132,#212133,#212134,#212135,#212136,#212137,#212138,
#212139,#212140,#212141,#212142,#212143,#212144,#212145,#212146,#212147,
#212148,#212149,#212150,#212151,#212152,#212153,#212154,#212155,#212156,
#212157,#212158,#212159,#212160,#212161,#212162,#212163,#212164,#212165,
#212166,#212167,#212168,#212169,#212170,#212171,#212172,#212173,#212174,
#212175,#212176,#212177,#212178,#212179,#212180,#212181,#212182,#212183,
#212184,#212185,#212186,#212187,#212188,#212189,#212190,#212191,#212192,
#212193,#212194,#212195,#212196,#212197,#212198,#212199,#212200,#212201,
#212202,#212203,#212204,#212205,#212206,#212207,#212208,#212209,#212210,
#212211,#212212,#212213,#212214,#212215,#212216,#212217,#212218,#212219,
#212220,#212221,#212222,#212223,#212224,#212225,#212226,#212227,#212228,
#212229,#212230),.UNSPECIFIED.,.F.,.F.,(4,3,3,3,3,3,3,3,3,3,3,3,3,3,3,3,
3,3,3,3,3,3,3,3,3,3,3,3,3,3,3,3,3,3,3,3,3,3,3,3,3,3,3,3,3,3,3,3,3,3,3,3,
3,3,3,3,4),(348.716784548553,348.797305153374,348.877955810068,348.95883364991,
349.039831377576,349.121049133391,349.189063569237,349.266622420782,349.344088964677,
349.42147886797,349.498807742663,349.576091156806,349.653352203378,349.730602904222,
349.807857306907,349.885129458439,349.962474796577,350.039857570302,350.117347065949,
350.187803305099,350.272022587992,350.356115266965,350.440001892778,350.523758882165,
350.607300584823,350.68717317303,350.764540368823,350.841925958274,350.919343740062,
350.996848661674,351.074403260927,351.152064607879,351.186543040961,351.266163779705,
351.345711607362,351.425198836637,351.504637733551,351.584040526357,351.663425739256,
351.742801969808,351.822180299359,351.90157180923,351.981017044061,352.060490624842,
352.140037736892,352.185282776823,352.261997783672,352.338645696036,352.415241207775,
352.491800105473,352.568337489552,352.644879010005,352.684652644755,352.769339370933,
352.854150045697,352.939116054778,352.952905577053),.UNSPECIFIED.);
#3485=B_SPLINE_CURVE_WITH_KNOTS('',3,(#212236,#212237,#212238,#212239,#212240,
#212241,#212242,#212243,#212244,#212245,#212246,#212247,#212248,#212249,
#212250,#212251,#212252,#212253,#212254,#212255,#212256,#212257,#212258,
#212259,#212260,#212261,#212262,#212263,#212264,#212265,#212266,#212267,
#212268,#212269,#212270,#212271,#212272,#212273,#212274,#212275,#212276,
#212277,#212278,#212279,#212280,#212281,#212282,#212283,#212284,#212285,
#212286,#212287,#212288,#212289,#212290,#212291,#212292,#212293,#212294,
#212295,#212296,#212297,#212298,#212299,#212300,#212301,#212302,#212303,
#212304,#212305,#212306,#212307,#212308,#212309,#212310,#212311,#212312,
#212313,#212314,#212315,#212316,#212317,#212318,#212319,#212320,#212321,
#212322,#212323,#212324,#212325,#212326,#212327,#212328,#212329,#212330,
#212331,#212332,#212333,#212334,#212335,#212336,#212337,#212338,#212339,
#212340,#212341,#212342,#212343,#212344,#212345,#212346,#212347,#212348,
#212349,#212350,#212351,#212352,#212353,#212354,#212355,#212356,#212357,
#212358,#212359,#212360,#212361,#212362,#212363,#212364,#212365,#212366,
#212367,#212368,#212369,#212370,#212371,#212372,#212373,#212374,#212375,
#212376,#212377,#212378,#212379,#212380,#212381,#212382,#212383,#212384,
#212385,#212386,#212387,#212388,#212389,#212390,#212391,#212392,#212393,
#212394,#212395,#212396,#212397,#212398,#212399,#212400,#212401),
 .UNSPECIFIED.,.F.,.F.,(4,3,3,3,3,3,3,3,3,3,3,3,3,3,3,3,3,3,3,3,3,3,3,3,
3,3,3,3,3,3,3,3,3,3,3,3,3,3,3,3,3,3,3,3,3,3,3,3,3,3,3,3,3,3,3,4),(355.000265717516,
355.07862633194,355.156915835323,355.235148756737,355.313574828978,355.391742837346,
355.469901025712,355.54806247983,355.626686193539,355.704920289582,355.783738812124,
355.862557334667,355.939272341516,356.01592025388,356.092515765619,356.169074663317,
356.245612047396,356.322153567848,356.361927202598,356.446603540806,356.53142602532,
356.616448396195,356.701557278004,356.786786817379,356.861297070529,356.942853333189,
357.024334272855,357.108417439256,357.189743191768,357.275205065114,357.36066693846,
357.440070279344,357.519492050507,357.598943028148,357.678467194368,357.758033104913,
357.837682953116,357.860036806391,357.938415827261,358.016728578577,358.09498947473,
358.17321289253,358.25141318069,358.329621369855,358.407837423345,358.486074340575,
358.564345130729,358.642708710202,358.721121839661,358.799652222174,358.858776542253,
358.934848133081,359.01079790405,359.086677955374,359.162492894976,359.237285162207),
 .UNSPECIFIED.);
#3486=B_SPLINE_CURVE_WITH_KNOTS('',3,(#212402,#212403,#212404,#212405,#212406,
#212407,#212408,#212409,#212410,#212411,#212412,#212413,#212414,#212415,
#212416,#212417,#212418,#212419,#212420,#212421,#212422,#212423,#212424,
#212425,#212426,#212427,#212428,#212429,#212430,#212431,#212432,#212433,
#212434,#212435,#212436,#212437,#212438,#212439,#212440,#212441,#212442,
#212443,#212444,#212445,#212446,#212447,#212448,#212449,#212450,#212451,
#212452,#212453,#212454,#212455,#212456,#212457,#212458,#212459,#212460,
#212461,#212462,#212463,#212464,#212465,#212466,#212467,#212468,#212469,
#212470,#212471,#212472,#212473,#212474,#212475,#212476,#212477),
 .UNSPECIFIED.,.F.,.F.,(4,3,3,3,3,3,3,3,3,3,3,3,3,3,3,3,3,3,3,3,3,3,3,3,
3,4),(352.953459366778,353.035920970537,353.118381908416,353.200842207814,
353.283301896127,353.365761000749,353.448219549072,353.530677568487,353.61313508638,
353.699812259459,353.782279045067,353.864744158199,353.947207708506,354.02966980562,
354.112130559152,354.194590078694,354.277048473821,354.359505854092,354.441972239911,
354.524435441535,354.606895897483,354.68935404612,354.771819650131,354.854279528709,
354.936743640445,354.999969855647),.UNSPECIFIED.);
#3487=B_SPLINE_CURVE_WITH_KNOTS('',3,(#212479,#212480,#212481,#212482,#212483,
#212484,#212485,#212486,#212487,#212488,#212489,#212490,#212491,#212492,
#212493,#212494,#212495,#212496,#212497,#212498,#212499,#212500,#212501,
#212502,#212503,#212504,#212505,#212506,#212507,#212508,#212509,#212510,
#212511,#212512,#212513,#212514,#212515,#212516,#212517,#212518,#212519,
#212520,#212521,#212522,#212523,#212524,#212525,#212526,#212527,#212528,
#212529,#212530,#212531,#212532,#212533,#212534,#212535,#212536,#212537,
#212538,#212539,#212540,#212541,#212542,#212543,#212544,#212545,#212546,
#212547,#212548,#212549,#212550,#212551,#212552,#212553,#212554,#212555,
#212556,#212557,#212558,#212559,#212560),.UNSPECIFIED.,.F.,.F.,(4,3,3,3,
3,3,3,3,3,3,3,3,3,3,3,3,3,3,3,3,3,3,3,3,3,3,3,4),(352.952905577053,353.038027293992,
353.12326229478,353.184022512686,353.265578775345,353.347059715011,353.431142881412,
353.512468633924,353.59793050727,353.683392380617,353.762795721502,353.842217492664,
353.921668470305,354.001192636525,354.08075854707,354.160408395273,354.182762248548,
354.259467848333,354.33610345867,354.412685321611,354.489233298249,354.565764476793,
354.642293487223,354.718834955904,354.795439462035,354.872077965804,354.94880981331,
354.999969855546),.UNSPECIFIED.);
#3488=B_SPLINE_CURVE_WITH_KNOTS('',3,(#212561,#212562,#212563,#212564,#212565,
#212566,#212567,#212568,#212569,#212570,#212571,#212572,#212573,#212574,
#212575,#212576,#212577,#212578,#212579,#212580,#212581,#212582,#212583,
#212584,#212585,#212586,#212587,#212588,#212589,#212590,#212591,#212592,
#212593,#212594,#212595,#212596,#212597,#212598,#212599,#212600,#212601,
#212602,#212603,#212604,#212605,#212606,#212607,#212608,#212609,#212610,
#212611,#212612,#212613,#212614,#212615,#212616,#212617,#212618,#212619,
#212620,#212621,#212622,#212623,#212624,#212625,#212626,#212627,#212628,
#212629,#212630,#212631,#212632,#212633,#212634,#212635,#212636,#212637,
#212638,#212639,#212640,#212641,#212642,#212643,#212644,#212645,#212646,
#212647,#212648,#212649,#212650,#212651,#212652,#212653,#212654,#212655,
#212656,#212657,#212658,#212659,#212660,#212661,#212662,#212663,#212664,
#212665,#212666,#212667,#212668,#212669,#212670,#212671,#212672,#212673,
#212674,#212675,#212676,#212677,#212678,#212679,#212680,#212681,#212682,
#212683,#212684,#212685,#212686,#212687,#212688,#212689,#212690,#212691,
#212692,#212693,#212694,#212695,#212696,#212697,#212698,#212699,#212700,
#212701,#212702,#212703,#212704,#212705,#212706,#212707,#212708,#212709,
#212710,#212711,#212712,#212713,#212714,#212715,#212716,#212717,#212718,
#212719,#212720,#212721,#212722,#212723,#212724,#212725,#212726,#212727,
#212728,#212729),.UNSPECIFIED.,.F.,.F.,(4,3,3,3,3,3,3,3,3,3,3,3,3,3,3,3,
3,3,3,3,3,3,3,3,3,3,3,3,3,3,3,3,3,3,3,3,3,3,3,3,3,3,3,3,3,3,3,3,3,3,3,3,
3,3,3,3,4),(354.999969855647,355.145499078777,355.18150198441,355.257558491164,
355.333519309158,355.409401229777,355.485220963284,355.560995157615,355.638400977947,
355.714148734062,355.78990373959,355.865681004821,355.944321183684,356.020230370152,
356.096196362095,356.172268559705,356.180241720272,356.257800571817,356.335267115712,
356.412657019005,356.489985893698,356.567269307841,356.644530354413,356.721781055257,
356.799035457942,356.876307609474,356.953652947612,357.031035721336,357.108525216984,
357.178981456134,357.263200739027,357.347293418001,357.431180043814,357.514937033201,
357.598478735859,357.678351324065,357.755718519858,357.833104109309,357.910521891097,
357.98802681271,358.065581411963,358.143242758915,358.177721191997,358.257341930741,
358.336889758398,358.416376987673,358.495815884586,358.575218677393,358.654603890292,
358.733980120844,358.813358450395,358.892749960266,358.972195195097,359.051668775877,
359.131215887927,359.176460927859,359.237141913219),.UNSPECIFIED.);
#3489=B_SPLINE_CURVE_WITH_KNOTS('',3,(#212735,#212736,#212737,#212738,#212739,
#212740,#212741,#212742,#212743,#212744,#212745,#212746,#212747,#212748,
#212749,#212750,#212751,#212752,#212753,#212754,#212755,#212756,#212757,
#212758,#212759,#212760,#212761,#212762,#212763,#212764,#212765,#212766,
#212767,#212768,#212769,#212770,#212771,#212772,#212773,#212774,#212775,
#212776,#212777,#212778,#212779,#212780,#212781,#212782,#212783,#212784,
#212785,#212786,#212787,#212788,#212789,#212790,#212791,#212792,#212793,
#212794,#212795,#212796,#212797,#212798,#212799,#212800,#212801,#212802,
#212803,#212804,#212805,#212806,#212807,#212808,#212809,#212810,#212811,
#212812,#212813,#212814,#212815,#212816,#212817,#212818,#212819,#212820,
#212821,#212822,#212823,#212824,#212825,#212826,#212827,#212828,#212829,
#212830,#212831,#212832,#212833,#212834,#212835,#212836,#212837,#212838,
#212839,#212840,#212841,#212842,#212843,#212844,#212845,#212846,#212847,
#212848,#212849,#212850,#212851,#212852,#212853,#212854,#212855,#212856,
#212857,#212858,#212859,#212860,#212861,#212862,#212863,#212864,#212865,
#212866,#212867,#212868,#212869,#212870,#212871,#212872,#212873,#212874,
#212875,#212876,#212877,#212878,#212879,#212880,#212881,#212882,#212883,
#212884,#212885,#212886,#212887,#212888,#212889,#212890,#212891,#212892,
#212893,#212894,#212895,#212896,#212897,#212898,#212899,#212900,#212901,
#212902,#212903),.UNSPECIFIED.,.F.,.F.,(4,3,3,3,3,3,3,3,3,3,3,3,3,3,3,3,
3,3,3,3,3,3,3,3,3,3,3,3,3,3,3,3,3,3,3,3,3,3,3,3,3,3,3,3,3,3,3,3,3,3,3,3,
3,3,3,3,4),(361.283155162826,361.355625881909,361.432993077702,361.510378667153,
361.58779644894,361.665301370553,361.742855969805,361.820517316757,361.85499574984,
361.934616488584,362.01416431624,362.093651545516,362.173090442429,362.252493235236,
362.331878448134,362.411254678687,362.490633008237,362.570024518108,362.649469752939,
362.72894333372,362.808490445769,362.853735485702,362.930450492551,363.007098404915,
363.083693916654,363.160252814353,363.236790198432,363.313331718884,363.353105353633,
363.437781691841,363.522604176355,363.607626547231,363.692735429039,363.777964968414,
363.852475221564,363.934031484224,364.015512423889,364.099595590291,364.180921342802,
364.266383216149,364.351845089495,364.43124843038,364.510670201542,364.590121179183,
364.669645345403,364.749211255948,364.828861104151,364.851214957426,364.929607149855,
365.007915006163,365.086174026984,365.164397253256,365.242597702528,365.320801928763,
365.39900717539,365.477247391082,365.519381429312),.UNSPECIFIED.);
#3490=B_SPLINE_CURVE_WITH_KNOTS('',3,(#212904,#212905,#212906,#212907,#212908,
#212909,#212910,#212911,#212912,#212913,#212914,#212915,#212916,#212917,
#212918,#212919,#212920,#212921,#212922,#212923,#212924,#212925,#212926,
#212927,#212928,#212929,#212930,#212931,#212932,#212933,#212934,#212935,
#212936,#212937,#212938,#212939,#212940,#212941,#212942,#212943,#212944,
#212945,#212946,#212947,#212948,#212949,#212950,#212951,#212952,#212953,
#212954,#212955,#212956,#212957,#212958,#212959,#212960,#212961,#212962,
#212963,#212964,#212965,#212966,#212967,#212968,#212969,#212970,#212971,
#212972,#212973,#212974,#212975,#212976,#212977,#212978,#212979,#212980,
#212981,#212982,#212983,#212984,#212985),.UNSPECIFIED.,.F.,.F.,(4,3,3,3,
3,3,3,3,3,3,3,3,3,3,3,3,3,3,3,3,3,3,3,3,3,3,3,4),(359.237285162207,359.314814051696,
359.390561811662,359.466316650378,359.54209357802,359.620949253044,359.696858013785,
359.772823464503,359.848895295443,359.857516278115,359.93507512966,360.012541673555,
360.089931576848,360.167260451541,360.244543865684,360.321804912256,360.399055613099,
360.476310015785,360.553582167317,360.630927505455,360.708310279179,360.785799774827,
360.856256013978,360.942974708954,361.029430442254,361.115706269608,361.201641256815,
361.283155162746),.UNSPECIFIED.);
#3491=B_SPLINE_CURVE_WITH_KNOTS('',3,(#212987,#212988,#212989,#212990,#212991,
#212992,#212993,#212994,#212995,#212996,#212997,#212998,#212999,#213000,
#213001,#213002,#213003,#213004,#213005,#213006,#213007,#213008,#213009,
#213010,#213011,#213012,#213013,#213014,#213015,#213016,#213017,#213018,
#213019,#213020,#213021,#213022,#213023,#213024,#213025,#213026,#213027,
#213028,#213029,#213030,#213031,#213032,#213033,#213034,#213035,#213036,
#213037,#213038,#213039,#213040,#213041,#213042,#213043,#213044,#213045,
#213046,#213047,#213048,#213049,#213050,#213051,#213052,#213053,#213054,
#213055,#213056,#213057,#213058,#213059,#213060,#213061,#213062,#213063,
#213064,#213065),.UNSPECIFIED.,.F.,.F.,(4,3,3,3,3,3,3,3,3,3,3,3,3,3,3,3,
3,3,3,3,3,3,3,3,3,3,4),(359.237141913219,359.313802637782,359.390407892746,
359.466972944385,359.543513743999,359.620058210566,359.67583079579,359.760507133998,
359.845329618512,359.930351989387,360.015460871196,360.100690410571,360.175200663721,
360.256756926381,360.338237866047,360.422321032448,360.50364678496,360.589108658306,
360.674570531652,360.753973872537,360.833395643699,360.91284662134,360.99237078756,
361.071936698105,361.151586546308,361.173940399583,361.283155162826),
 .UNSPECIFIED.);
#3492=B_SPLINE_CURVE_WITH_KNOTS('',3,(#213066,#213067,#213068,#213069,#213070,
#213071,#213072,#213073,#213074,#213075,#213076,#213077,#213078,#213079,
#213080,#213081,#213082,#213083,#213084,#213085,#213086,#213087,#213088,
#213089,#213090,#213091,#213092,#213093,#213094,#213095,#213096,#213097,
#213098,#213099,#213100,#213101,#213102,#213103,#213104,#213105,#213106,
#213107,#213108,#213109,#213110,#213111,#213112,#213113,#213114,#213115,
#213116,#213117,#213118,#213119,#213120,#213121,#213122,#213123,#213124,
#213125,#213126,#213127,#213128,#213129,#213130,#213131,#213132,#213133,
#213134,#213135,#213136,#213137,#213138,#213139,#213140,#213141,#213142,
#213143,#213144,#213145,#213146,#213147,#213148,#213149,#213150,#213151,
#213152,#213153,#213154,#213155,#213156,#213157,#213158,#213159,#213160,
#213161,#213162,#213163,#213164,#213165,#213166,#213167,#213168,#213169,
#213170,#213171,#213172,#213173,#213174,#213175,#213176,#213177,#213178,
#213179,#213180,#213181,#213182,#213183,#213184,#213185,#213186,#213187,
#213188,#213189,#213190,#213191,#213192,#213193,#213194,#213195,#213196,
#213197,#213198,#213199,#213200,#213201,#213202,#213203,#213204,#213205,
#213206,#213207,#213208,#213209,#213210,#213211,#213212,#213213,#213214,
#213215,#213216,#213217,#213218,#213219,#213220,#213221,#213222,#213223,
#213224,#213225,#213226,#213227,#213228,#213229,#213230,#213231,#213232,
#213233,#213234,#213235,#213236,#213237),.UNSPECIFIED.,.F.,.F.,(4,3,3,3,
3,3,3,3,3,3,3,3,3,3,3,3,3,3,3,3,3,3,3,3,3,3,3,3,3,3,3,3,3,3,3,3,3,3,3,3,
3,3,3,3,3,3,3,3,3,3,3,3,3,3,3,3,3,4),(361.283155162933,361.360786413993,
361.438359570209,361.515889959261,361.593392877591,361.670898290541,361.748409428821,
361.825940131368,361.903504245392,361.981157765079,362.058862079906,362.136675654933,
362.172680135445,362.248736642199,362.324697460193,362.400579380812,362.476399114319,
362.552173308651,362.629579128983,362.705326885098,362.781081890626,362.856859155857,
362.93549933472,363.011408521188,363.087374513131,363.163446710741,363.171419871308,
363.248978722853,363.326445266748,363.403835170041,363.481164044734,363.558447458877,
363.635708505449,363.712959206293,363.790213608979,363.86748576051,363.944831098648,
364.022213872373,364.099703368021,364.17015960717,364.254378890063,364.338471569036,
364.422358194849,364.506115184235,364.589656886893,364.669529475101,364.746896670894,
364.824282260345,364.901700042133,364.979204963746,365.056759562998,365.134420909951,
365.168899343032,365.248533459538,365.328076371135,365.407565382026,365.487002394566,
365.5201243322),.UNSPECIFIED.);
#3493=B_SPLINE_CURVE_WITH_KNOTS('',3,(#213243,#213244,#213245,#213246,#213247,
#213248,#213249,#213250,#213251,#213252,#213253,#213254,#213255,#213256,
#213257,#213258,#213259,#213260,#213261,#213262,#213263,#213264,#213265,
#213266,#213267,#213268,#213269,#213270,#213271,#213272,#213273,#213274,
#213275,#213276,#213277,#213278,#213279,#213280,#213281,#213282,#213283,
#213284,#213285,#213286,#213287,#213288,#213289,#213290,#213291,#213292,
#213293,#213294,#213295,#213296,#213297,#213298,#213299,#213300,#213301,
#213302,#213303,#213304,#213305,#213306,#213307,#213308,#213309,#213310,
#213311,#213312,#213313,#213314,#213315,#213316,#213317,#213318,#213319,
#213320,#213321,#213322,#213323,#213324,#213325,#213326,#213327,#213328,
#213329,#213330,#213331,#213332,#213333,#213334,#213335,#213336,#213337,
#213338,#213339,#213340,#213341,#213342,#213343,#213344,#213345,#213346,
#213347,#213348,#213349,#213350,#213351,#213352,#213353,#213354,#213355,
#213356,#213357,#213358,#213359,#213360,#213361,#213362,#213363,#213364,
#213365,#213366,#213367,#213368,#213369,#213370,#213371,#213372,#213373,
#213374,#213375,#213376,#213377,#213378,#213379,#213380,#213381,#213382,
#213383,#213384,#213385,#213386,#213387,#213388,#213389,#213390,#213391,
#213392,#213393,#213394,#213395,#213396,#213397,#213398,#213399,#213400,
#213401,#213402,#213403,#213404,#213405,#213406,#213407,#213408),
 .UNSPECIFIED.,.F.,.F.,(4,3,3,3,3,3,3,3,3,3,3,3,3,3,3,3,3,3,3,3,3,3,3,3,
3,3,3,3,3,3,3,3,3,3,3,3,3,3,3,3,3,3,3,3,3,3,3,3,3,3,3,3,3,3,3,4),(367.566340470133,
367.65634728685,367.746832996282,367.837849218279,367.847434165013,367.931653447906,
368.015746126879,368.099632752693,368.183389742079,368.266931444738,368.346804032944,
368.424171228737,368.501556818188,368.578974599976,368.656479521589,368.734034120841,
368.811695467793,368.846173900875,368.925794639619,369.005342467275,369.084829696551,
369.164268593464,369.24367138627,369.323056599169,369.402432829721,369.481811159272,
369.561202669143,369.640647903974,369.720121484754,369.799668596804,369.844913636737,
369.921628643586,369.99827655595,370.074872067689,370.151430965388,370.227968349467,
370.304509869919,370.344283504668,370.428959842876,370.51378232739,370.598804698266,
370.683913580075,370.76914311945,370.8436533726,370.92520963526,371.006690574926,
371.090773741327,371.172099493839,371.257561367185,371.343023240531,371.422423589424,
371.501841947507,371.581323390372,371.660836601941,371.740434855231,371.802906295849),
 .UNSPECIFIED.);
#3494=B_SPLINE_CURVE_WITH_KNOTS('',3,(#213409,#213410,#213411,#213412,#213413,
#213414,#213415,#213416,#213417,#213418,#213419,#213420,#213421,#213422,
#213423,#213424,#213425,#213426,#213427,#213428,#213429,#213430,#213431,
#213432,#213433,#213434,#213435,#213436,#213437,#213438,#213439,#213440,
#213441,#213442,#213443,#213444,#213445,#213446,#213447,#213448,#213449,
#213450,#213451,#213452,#213453,#213454,#213455,#213456,#213457,#213458,
#213459,#213460,#213461,#213462,#213463,#213464,#213465,#213466,#213467,
#213468,#213469,#213470,#213471,#213472,#213473,#213474,#213475,#213476,
#213477,#213478,#213479,#213480,#213481,#213482,#213483,#213484,#213485,
#213486,#213487,#213488,#213489,#213490,#213491,#213492,#213493,#213494,
#213495,#213496),.UNSPECIFIED.,.F.,.F.,(4,3,3,3,3,3,3,3,3,3,3,3,3,3,3,3,
3,3,3,3,3,3,3,3,3,3,3,3,3,4),(365.519381429312,365.597675845742,365.676064617682,
365.754509281994,365.833059455537,365.849954693289,365.926011200043,366.001972018037,
366.077853938656,366.153673672164,366.229447866494,366.306853686826,366.382601442942,
366.45835644847,366.5341337137,366.612773892563,366.688683079032,366.764649070974,
366.840721268584,366.848694429151,366.926527682873,367.006504281264,367.084132405596,
367.161700039667,367.239221020856,367.316709157361,367.394185738152,367.471656271798,
367.549146528326,367.566340470006),.UNSPECIFIED.);
#3495=B_SPLINE_CURVE_WITH_KNOTS('',3,(#213498,#213499,#213500,#213501,#213502,
#213503,#213504,#213505,#213506,#213507,#213508,#213509,#213510,#213511,
#213512,#213513,#213514,#213515,#213516,#213517,#213518,#213519,#213520,
#213521,#213522,#213523,#213524,#213525,#213526,#213527,#213528,#213529,
#213530,#213531,#213532,#213533,#213534,#213535,#213536,#213537,#213538,
#213539,#213540,#213541,#213542,#213543,#213544,#213545,#213546,#213547,
#213548,#213549,#213550,#213551,#213552,#213553,#213554,#213555,#213556,
#213557,#213558,#213559,#213560,#213561,#213562,#213563,#213564,#213565,
#213566,#213567,#213568,#213569,#213570,#213571,#213572,#213573,#213574,
#213575,#213576),.UNSPECIFIED.,.F.,.F.,(4,3,3,3,3,3,3,3,3,3,3,3,3,3,3,3,
3,3,3,3,3,3,3,3,3,3,4),(365.5201243322,365.601063675537,365.680443602888,
365.759819387226,365.839202109013,365.921311351483,366.000768657719,366.084203868307,
366.167639078894,366.244354085743,366.321001998106,366.397597509846,366.474156407544,
366.550693791622,366.627235312075,366.667008946825,366.751685285033,366.836507769547,
366.921530140422,367.006639022231,367.091868561606,367.166378814756,367.24895402029,
367.331412181403,367.413795867861,367.49607454044,367.566340470006),
 .UNSPECIFIED.);
#3496=B_SPLINE_CURVE_WITH_KNOTS('',3,(#213577,#213578,#213579,#213580,#213581,
#213582,#213583,#213584,#213585,#213586,#213587,#213588,#213589,#213590,
#213591,#213592,#213593,#213594,#213595,#213596,#213597,#213598,#213599,
#213600,#213601,#213602,#213603,#213604,#213605,#213606,#213607,#213608,
#213609,#213610,#213611,#213612,#213613,#213614,#213615,#213616,#213617,
#213618,#213619,#213620,#213621,#213622,#213623,#213624,#213625,#213626,
#213627,#213628,#213629,#213630,#213631,#213632,#213633,#213634,#213635,
#213636,#213637,#213638,#213639,#213640,#213641,#213642,#213643,#213644,
#213645,#213646,#213647,#213648,#213649,#213650,#213651,#213652,#213653,
#213654,#213655,#213656,#213657,#213658,#213659,#213660,#213661,#213662,
#213663,#213664,#213665,#213666,#213667,#213668,#213669,#213670,#213671,
#213672,#213673,#213674,#213675,#213676,#213677,#213678,#213679,#213680,
#213681,#213682,#213683,#213684,#213685,#213686,#213687,#213688,#213689,
#213690,#213691,#213692,#213693,#213694,#213695,#213696,#213697,#213698,
#213699,#213700,#213701,#213702,#213703,#213704,#213705,#213706,#213707,
#213708,#213709,#213710,#213711,#213712,#213713,#213714,#213715,#213716,
#213717,#213718,#213719,#213720,#213721,#213722,#213723,#213724,#213725,
#213726,#213727,#213728,#213729,#213730,#213731,#213732,#213733),
 .UNSPECIFIED.,.F.,.F.,(4,3,3,3,3,3,3,3,3,3,3,3,3,3,3,3,3,3,3,3,3,3,3,3,
3,3,3,3,3,3,3,3,3,3,3,3,3,3,3,3,3,3,3,3,3,3,3,3,3,3,3,3,4),(367.566340470006,
367.648802676092,367.73126453388,367.813726050221,367.896187231965,367.978648085961,
368.06110861906,368.14356883811,368.226028749961,368.30848836146,368.390947679457,
368.473406710799,368.555865462334,368.638323940911,368.720782153375,368.803240106575,
368.885697807358,368.96815526257,369.050612479058,369.136625066847,369.219949761268,
369.302416366826,369.384882128177,369.467347072735,369.549811227913,369.63227462112,
369.714737279764,369.797199231248,369.879660502974,369.962121122342,370.044581116749,
370.127040513591,370.209499340259,370.291957624145,370.374415392639,370.456872673126,
370.541006586576,370.623472584874,370.705936961423,370.788399825865,370.870861287822,
370.953321456895,371.03578044267,371.118238354713,371.203835471413,371.286300208357,
371.368761980655,371.451221226746,371.533678384925,371.616140903824,371.698598575107,
371.781057366015,371.803015288317),.UNSPECIFIED.);
#3497=B_SPLINE_CURVE_WITH_KNOTS('',3,(#213739,#213740,#213741,#213742,#213743,
#213744,#213745,#213746,#213747,#213748,#213749,#213750,#213751,#213752,
#213753,#213754,#213755,#213756,#213757,#213758,#213759,#213760,#213761,
#213762,#213763,#213764,#213765,#213766,#213767,#213768,#213769,#213770,
#213771,#213772,#213773,#213774,#213775,#213776,#213777,#213778,#213779,
#213780,#213781,#213782,#213783,#213784,#213785,#213786,#213787,#213788,
#213789,#213790,#213791,#213792,#213793,#213794,#213795,#213796,#213797,
#213798,#213799,#213800,#213801,#213802,#213803,#213804,#213805,#213806,
#213807,#213808,#213809,#213810,#213811,#213812,#213813,#213814,#213815,
#213816,#213817,#213818,#213819,#213820,#213821,#213822,#213823,#213824,
#213825,#213826,#213827,#213828,#213829,#213830,#213831,#213832,#213833,
#213834,#213835,#213836,#213837,#213838,#213839,#213840,#213841,#213842,
#213843,#213844,#213845,#213846,#213847,#213848,#213849,#213850,#213851,
#213852,#213853,#213854,#213855,#213856,#213857,#213858,#213859,#213860,
#213861,#213862,#213863,#213864,#213865,#213866,#213867,#213868,#213869,
#213870,#213871,#213872,#213873,#213874,#213875,#213876,#213877,#213878,
#213879,#213880,#213881,#213882,#213883,#213884,#213885,#213886,#213887,
#213888,#213889,#213890,#213891,#213892,#213893,#213894,#213895,#213896,
#213897,#213898,#213899,#213900,#213901,#213902,#213903,#213904),
 .UNSPECIFIED.,.F.,.F.,(4,3,3,3,3,3,3,3,3,3,3,3,3,3,3,3,3,3,3,3,3,3,3,3,
3,3,3,3,3,3,3,3,3,3,3,3,3,3,3,3,3,3,3,3,3,3,3,3,3,3,3,3,3,3,3,4),(373.849525777278,
373.926925065778,374.004231815205,374.081461850757,374.158630941525,374.235754812016,
374.312856778804,374.389948914552,374.467045407264,374.544160444793,374.621348780657,
374.698575531326,374.775907024984,374.838612316048,374.922831598941,375.006924277914,
375.090810903727,375.174567893114,375.258109595772,375.337982183979,375.415349379772,
375.492734969224,375.570152751011,375.647657672624,375.725212271877,375.802873618829,
375.83735205191,375.916972790654,375.996520618311,376.076007847586,376.155446744499,
376.234849537306,376.314234750205,376.393610980757,376.472989310308,376.552380820179,
376.63182605501,376.71129963579,376.79084674784,376.836091787773,376.912806794622,
376.989454706986,377.066050218725,377.142609116424,377.219146500503,377.295688020955,
377.335461655704,377.420137993912,377.504960478426,377.589982849301,377.67509173111,
377.760321270484,377.834831523635,377.916387377341,378.001553171997,378.086718966652),
 .UNSPECIFIED.);
#3498=B_SPLINE_CURVE_WITH_KNOTS('',3,(#213905,#213906,#213907,#213908,#213909,
#213910,#213911,#213912,#213913,#213914,#213915,#213916,#213917,#213918,
#213919,#213920,#213921,#213922,#213923,#213924,#213925,#213926,#213927,
#213928,#213929,#213930,#213931,#213932,#213933,#213934,#213935,#213936,
#213937,#213938,#213939,#213940,#213941,#213942,#213943,#213944,#213945,
#213946,#213947,#213948,#213949,#213950,#213951,#213952,#213953,#213954,
#213955,#213956,#213957,#213958,#213959,#213960,#213961,#213962,#213963,
#213964,#213965,#213966,#213967,#213968,#213969,#213970,#213971,#213972,
#213973,#213974,#213975,#213976,#213977,#213978,#213979,#213980,#213981,
#213982,#213983,#213984,#213985,#213986,#213987,#213988,#213989,#213990,
#213991,#213992),.UNSPECIFIED.,.F.,.F.,(4,3,3,3,3,3,3,3,3,3,3,3,3,3,3,3,
3,3,3,3,3,3,3,3,3,3,3,3,3,4),(371.802906295849,371.842393108462,371.920772129332,
371.999084880648,372.077345776802,372.155569194601,372.233769482761,372.311977671926,
372.390193725416,372.468430642645,372.546701432799,372.625065012272,372.703478141731,
372.782008524244,372.841132844324,372.917189351078,372.993150169072,373.069032089691,
373.144851823198,373.220626017529,373.298031837862,373.373779593977,373.449534599505,
373.525311864735,373.603952043598,373.679861230067,373.75582722201,373.83189941962,
373.839872580186,373.849525777185),.UNSPECIFIED.);
#3499=B_SPLINE_CURVE_WITH_KNOTS('',3,(#213994,#213995,#213996,#213997,#213998,
#213999,#214000,#214001,#214002,#214003,#214004,#214005,#214006,#214007,
#214008,#214009,#214010,#214011,#214012,#214013,#214014,#214015,#214016,
#214017,#214018,#214019,#214020,#214021,#214022,#214023,#214024,#214025,
#214026,#214027,#214028,#214029,#214030,#214031,#214032,#214033,#214034,
#214035,#214036,#214037,#214038,#214039,#214040,#214041,#214042,#214043,
#214044,#214045,#214046,#214047,#214048,#214049,#214050,#214051,#214052,
#214053,#214054,#214055,#214056,#214057,#214058,#214059,#214060,#214061,
#214062,#214063,#214064,#214065,#214066,#214067,#214068,#214069),
 .UNSPECIFIED.,.F.,.F.,(4,3,3,3,3,3,3,3,3,3,3,3,3,3,3,3,3,3,3,3,3,3,3,3,
3,4),(371.803015288317,371.885476892075,371.967937829954,372.050398129352,
372.132857817666,372.215316922288,372.297775470611,372.380233490025,372.462691007918,
372.549368180997,372.631834966606,372.714300079737,372.796763630044,372.879225727158,
372.96168648069,373.044146000232,373.126604395359,373.20906177563,373.291528161449,
373.373991363073,373.456451819022,373.538909967658,373.62137557167,373.703835450247,
373.786299561984,373.849525777185),.UNSPECIFIED.);
#3500=B_SPLINE_CURVE_WITH_KNOTS('',3,(#214070,#214071,#214072,#214073,#214074,
#214075,#214076,#214077,#214078,#214079,#214080,#214081,#214082,#214083,
#214084,#214085,#214086,#214087,#214088,#214089,#214090,#214091,#214092,
#214093,#214094,#214095,#214096,#214097,#214098,#214099,#214100,#214101,
#214102,#214103,#214104,#214105,#214106,#214107,#214108,#214109,#214110,
#214111,#214112,#214113,#214114,#214115,#214116,#214117,#214118,#214119,
#214120,#214121,#214122,#214123,#214124,#214125,#214126,#214127,#214128,
#214129,#214130,#214131,#214132,#214133,#214134,#214135,#214136,#214137,
#214138,#214139,#214140,#214141,#214142,#214143,#214144,#214145,#214146,
#214147,#214148,#214149,#214150,#214151,#214152,#214153,#214154,#214155,
#214156,#214157,#214158,#214159,#214160,#214161,#214162,#214163,#214164,
#214165,#214166,#214167,#214168,#214169,#214170,#214171,#214172,#214173,
#214174,#214175,#214176,#214177,#214178,#214179,#214180,#214181,#214182,
#214183,#214184,#214185,#214186,#214187,#214188,#214189,#214190,#214191,
#214192,#214193,#214194,#214195,#214196,#214197,#214198,#214199,#214200,
#214201,#214202,#214203,#214204,#214205,#214206,#214207,#214208,#214209,
#214210,#214211,#214212,#214213,#214214,#214215,#214216,#214217,#214218,
#214219,#214220,#214221,#214222,#214223,#214224,#214225,#214226),
 .UNSPECIFIED.,.F.,.F.,(4,3,3,3,3,3,3,3,3,3,3,3,3,3,3,3,3,3,3,3,3,3,3,3,
3,3,3,3,3,3,3,3,3,3,3,3,3,3,3,3,3,3,3,3,3,3,3,3,3,3,3,3,4),(373.849525777328,
373.931987983413,374.014449841201,374.096911357542,374.179372539286,374.261833393283,
374.344293926382,374.426754145432,374.509214057282,374.591673668782,374.674132986778,
374.756592018121,374.839050769656,374.921509248232,375.003967460697,375.086425413897,
375.16888311468,375.251340569892,375.333797786379,375.419810374164,375.50313506858,
375.585601674139,375.66806743549,375.750532380048,375.832996535226,375.915459928433,
375.997922587077,376.080384538561,376.162845810287,376.245306429655,376.327766424062,
376.410225820904,376.492684647572,376.575142931458,376.657600699952,376.740057980439,
376.82419189388,376.906657892179,376.989122268728,377.07158513317,377.154046595126,
377.2365067642,377.318965749975,377.401423662018,377.487020778703,377.569485515646,
377.651947287944,377.734406534036,377.816863692214,377.899326211113,377.981783882397,
378.064242673305,378.086200595497),.UNSPECIFIED.);
#3501=B_SPLINE_CURVE_WITH_KNOTS('',3,(#214232,#214233,#214234,#214235,#214236,
#214237,#214238,#214239,#214240,#214241,#214242,#214243,#214244,#214245,
#214246,#214247,#214248,#214249,#214250,#214251,#214252,#214253,#214254,
#214255,#214256,#214257,#214258,#214259,#214260,#214261,#214262,#214263,
#214264,#214265,#214266,#214267,#214268,#214269,#214270,#214271,#214272,
#214273,#214274,#214275,#214276,#214277,#214278,#214279,#214280,#214281,
#214282,#214283,#214284,#214285,#214286,#214287,#214288,#214289,#214290,
#214291,#214292,#214293,#214294,#214295,#214296,#214297,#214298,#214299,
#214300,#214301,#214302,#214303,#214304,#214305,#214306,#214307,#214308,
#214309,#214310,#214311,#214312,#214313,#214314,#214315,#214316,#214317,
#214318,#214319,#214320,#214321,#214322,#214323,#214324,#214325,#214326,
#214327,#214328,#214329,#214330,#214331,#214332,#214333,#214334,#214335,
#214336,#214337,#214338,#214339,#214340,#214341,#214342,#214343,#214344,
#214345,#214346,#214347,#214348,#214349,#214350,#214351,#214352,#214353,
#214354,#214355,#214356,#214357,#214358,#214359,#214360,#214361,#214362,
#214363,#214364,#214365,#214366,#214367,#214368,#214369,#214370,#214371,
#214372,#214373,#214374,#214375,#214376,#214377,#214378,#214379,#214380,
#214381,#214382,#214383,#214384,#214385,#214386,#214387,#214388),
 .UNSPECIFIED.,.F.,.F.,(4,3,3,3,3,3,3,3,3,3,3,3,3,3,3,3,3,3,3,3,3,3,3,3,
3,3,3,3,3,3,3,3,3,3,3,3,3,3,3,3,3,3,3,3,3,3,3,3,3,3,3,3,4),(380.132711084365,
380.215173290451,380.297635148239,380.38009666458,380.462557846323,380.54501870032,
380.627479233419,380.709939452469,380.79239936432,380.874858975819,380.957318293816,
381.039777325158,381.122236076693,381.204694555269,381.287152767734,381.369610720934,
381.452068421717,381.534525876928,381.616983093416,381.702995681205,381.786320375626,
381.868786981185,381.951252742535,382.033717687094,382.116181842272,382.198645235479,
382.281107894122,382.363569845606,382.446031117333,382.528491736701,382.610951731108,
382.693411127949,382.775869954618,382.858328238504,382.940786006997,383.023243287485,
383.107377200935,383.189843199233,383.272307575782,383.354770440224,383.437231902181,
383.519692071254,383.602151057029,383.684608969072,383.770206085773,383.852670822716,
383.935132595015,384.017591841106,384.100048999284,384.182511518183,384.264969189467,
384.347427980375,384.369385902676),.UNSPECIFIED.);
#3502=B_SPLINE_CURVE_WITH_KNOTS('',3,(#214389,#214390,#214391,#214392,#214393,
#214394,#214395,#214396,#214397,#214398,#214399,#214400,#214401,#214402,
#214403,#214404,#214405,#214406,#214407,#214408,#214409,#214410,#214411,
#214412,#214413,#214414,#214415,#214416,#214417,#214418,#214419,#214420,
#214421,#214422,#214423,#214424,#214425,#214426,#214427,#214428,#214429,
#214430,#214431,#214432,#214433,#214434,#214435,#214436,#214437,#214438,
#214439,#214440,#214441,#214442,#214443,#214444,#214445,#214446,#214447,
#214448,#214449,#214450,#214451,#214452,#214453,#214454,#214455,#214456,
#214457,#214458,#214459,#214460,#214461,#214462,#214463,#214464,#214465,
#214466,#214467,#214468,#214469,#214470),.UNSPECIFIED.,.F.,.F.,(4,3,3,3,
3,3,3,3,3,3,3,3,3,3,3,3,3,3,3,3,3,3,3,3,3,3,3,4),(378.086718966652,378.168041453345,
378.251121422455,378.334201391566,378.41360473245,378.493026503613,378.572477481254,
378.652001647474,378.731567558019,378.811217406222,378.833571259497,378.911950280367,
378.990263031683,379.068523927837,379.146747345636,379.224947633796,379.303155822961,
379.381371876451,379.45960879368,379.537879583834,379.616243163307,379.694656292766,
379.773186675279,379.832310995359,379.92329934872,380.013756059912,380.103324611181,
380.132711084365),.UNSPECIFIED.);
#3503=B_SPLINE_CURVE_WITH_KNOTS('',3,(#214472,#214473,#214474,#214475,#214476,
#214477,#214478,#214479,#214480,#214481,#214482,#214483,#214484,#214485,
#214486,#214487,#214488,#214489,#214490,#214491,#214492,#214493,#214494,
#214495,#214496,#214497,#214498,#214499,#214500,#214501,#214502,#214503,
#214504,#214505,#214506,#214507,#214508,#214509,#214510,#214511,#214512,
#214513,#214514,#214515,#214516,#214517,#214518,#214519,#214520,#214521,
#214522,#214523,#214524,#214525,#214526,#214527,#214528,#214529,#214530,
#214531,#214532,#214533,#214534,#214535,#214536,#214537,#214538,#214539,
#214540,#214541,#214542,#214543,#214544,#214545,#214546,#214547),
 .UNSPECIFIED.,.F.,.F.,(4,3,3,3,3,3,3,3,3,3,3,3,3,3,3,3,3,3,3,3,3,3,3,3,
3,4),(378.086200595497,378.168662199255,378.251123137134,378.333583436532,
378.416043124845,378.498502229467,378.580960777791,378.663418797205,378.745876315098,
378.832553488169,378.915020273777,378.997485386909,379.079948937216,379.16241103433,
379.244871787861,379.327331307404,379.409789702531,379.492247082802,379.574713468621,
379.657176670245,379.739637126194,379.82209527483,379.904560878842,379.987020757419,
380.069484869156,380.132711084236),.UNSPECIFIED.);
#3504=B_SPLINE_CURVE_WITH_KNOTS('',3,(#214548,#214549,#214550,#214551,#214552,
#214553,#214554,#214555,#214556,#214557,#214558,#214559,#214560,#214561,
#214562,#214563,#214564,#214565,#214566,#214567,#214568,#214569,#214570,
#214571,#214572,#214573,#214574,#214575,#214576,#214577,#214578,#214579,
#214580,#214581,#214582,#214583,#214584,#214585,#214586,#214587,#214588,
#214589,#214590,#214591,#214592,#214593,#214594,#214595,#214596,#214597,
#214598,#214599,#214600,#214601,#214602,#214603,#214604,#214605,#214606,
#214607,#214608,#214609,#214610,#214611,#214612,#214613,#214614,#214615,
#214616,#214617,#214618,#214619,#214620,#214621,#214622,#214623,#214624,
#214625,#214626,#214627,#214628,#214629,#214630,#214631,#214632,#214633,
#214634,#214635,#214636,#214637,#214638,#214639,#214640,#214641,#214642,
#214643,#214644,#214645,#214646,#214647,#214648,#214649,#214650,#214651,
#214652,#214653,#214654,#214655,#214656,#214657,#214658,#214659,#214660,
#214661,#214662,#214663,#214664,#214665,#214666,#214667,#214668,#214669,
#214670,#214671,#214672,#214673,#214674,#214675,#214676,#214677,#214678,
#214679,#214680,#214681,#214682,#214683,#214684,#214685,#214686,#214687,
#214688,#214689,#214690,#214691,#214692,#214693,#214694,#214695,#214696,
#214697,#214698,#214699,#214700,#214701,#214702,#214703,#214704),
 .UNSPECIFIED.,.F.,.F.,(4,3,3,3,3,3,3,3,3,3,3,3,3,3,3,3,3,3,3,3,3,3,3,3,
3,3,3,3,3,3,3,3,3,3,3,3,3,3,3,3,3,3,3,3,3,3,3,3,3,3,3,3,4),(380.132711084365,
380.215173290451,380.297635148239,380.38009666458,380.462557846324,380.54501870032,
380.627479233419,380.709939452469,380.79239936432,380.874858975819,380.957318293816,
381.039777325158,381.122236076693,381.204694555269,381.287152767734,381.369610720934,
381.452068421717,381.534525876929,381.616983093416,381.702995681206,381.786320375626,
381.868786981185,381.951252742535,382.033717687094,382.116181842272,382.198645235479,
382.281107894122,382.363569845606,382.446031117333,382.528491736701,382.610951731108,
382.69341112795,382.775869954618,382.858328238504,382.940786006997,383.023243287485,
383.107377200935,383.189843199233,383.272307575782,383.354770440224,383.43723190218,
383.519692071254,383.602151057029,383.684608969072,383.770206085772,383.852670822716,
383.935132595014,384.017591841105,384.100048999284,384.182511518183,384.264969189466,
384.347427980374,384.369385902676),.UNSPECIFIED.);
#3505=B_SPLINE_CURVE_WITH_KNOTS('',3,(#214710,#214711,#214712,#214713,#214714,
#214715,#214716,#214717,#214718,#214719,#214720,#214721,#214722,#214723,
#214724,#214725,#214726,#214727,#214728,#214729,#214730,#214731,#214732,
#214733,#214734,#214735,#214736,#214737,#214738,#214739,#214740,#214741,
#214742,#214743,#214744,#214745,#214746,#214747,#214748,#214749,#214750,
#214751,#214752,#214753,#214754,#214755,#214756,#214757,#214758,#214759,
#214760,#214761,#214762,#214763,#214764,#214765,#214766,#214767,#214768,
#214769,#214770,#214771,#214772,#214773,#214774,#214775,#214776,#214777,
#214778,#214779,#214780,#214781,#214782,#214783,#214784,#214785,#214786,
#214787,#214788,#214789,#214790,#214791,#214792,#214793,#214794,#214795,
#214796,#214797,#214798,#214799,#214800,#214801,#214802,#214803,#214804,
#214805,#214806,#214807,#214808,#214809,#214810,#214811,#214812,#214813,
#214814,#214815,#214816,#214817,#214818,#214819,#214820,#214821,#214822,
#214823,#214824,#214825,#214826,#214827,#214828,#214829,#214830,#214831,
#214832,#214833,#214834,#214835,#214836,#214837,#214838,#214839,#214840,
#214841,#214842,#214843,#214844,#214845,#214846,#214847,#214848,#214849,
#214850,#214851,#214852,#214853,#214854,#214855,#214856,#214857,#214858,
#214859,#214860,#214861,#214862,#214863,#214864,#214865,#214866,#214867,
#214868,#214869,#214870,#214871,#214872,#214873,#214874,#214875,#214876,
#214877,#214878),.UNSPECIFIED.,.F.,.F.,(4,3,3,3,3,3,3,3,3,3,3,3,3,3,3,3,
3,3,3,3,3,3,3,3,3,3,3,3,3,3,3,3,3,3,3,3,3,3,3,3,3,3,3,3,3,3,3,3,3,3,3,3,
3,3,3,3,4),(386.415896391545,386.504650454752,386.594152180165,386.684007274919,
386.77427201933,386.823489146394,386.899545653148,386.975506471142,387.051388391762,
387.127208125269,387.202982319599,387.280388139932,387.356135896047,387.431890901575,
387.507668166805,387.586308345668,387.662217532137,387.738183524079,387.814255721689,
387.822228882257,387.899787733802,387.977254277697,388.05464418099,388.131973055683,
388.209256469826,388.286517516398,388.363768217242,388.441022619928,388.51829477146,
388.595640109597,388.673022883322,388.75051237897,388.820968618119,388.905187901012,
388.989280579985,389.073167205799,389.156924195185,389.240465897844,389.32033848605,
389.397705681843,389.475091271294,389.552509053082,389.630013974694,389.707568573947,
389.785229920899,389.819708353981,389.899336225541,389.978889817429,390.058381448263,
390.137816628524,390.217218793118,390.29659904664,390.375968477917,390.455354592249,
390.534748496362,390.614182588444,390.652606861601),.UNSPECIFIED.);
#3506=B_SPLINE_CURVE_WITH_KNOTS('',3,(#214879,#214880,#214881,#214882,#214883,
#214884,#214885,#214886,#214887,#214888,#214889,#214890,#214891,#214892,
#214893,#214894,#214895,#214896,#214897,#214898,#214899,#214900,#214901,
#214902,#214903,#214904,#214905,#214906,#214907,#214908,#214909,#214910,
#214911,#214912,#214913,#214914,#214915,#214916,#214917,#214918,#214919,
#214920,#214921,#214922,#214923,#214924,#214925,#214926,#214927,#214928,
#214929,#214930,#214931,#214932,#214933,#214934,#214935,#214936,#214937,
#214938,#214939,#214940,#214941,#214942,#214943,#214944,#214945,#214946,
#214947,#214948,#214949,#214950,#214951,#214952,#214953,#214954),
 .UNSPECIFIED.,.F.,.F.,(4,3,3,3,3,3,3,3,3,3,3,3,3,3,3,3,3,3,3,3,3,3,3,3,
3,4),(384.369385902676,384.451847506435,384.534308444314,384.616768743712,
384.699228432025,384.781687536647,384.86414608497,384.946604104384,385.029061622277,
385.115738795357,385.198205580965,385.280670694097,385.363134244403,385.445596341517,
385.528057095049,385.610516614592,385.692975009719,385.77543238999,385.857898775809,
385.940361977433,386.022822433381,386.105280582018,386.18774618603,386.270206064607,
386.352670176344,386.415896391545),.UNSPECIFIED.);
#3507=B_SPLINE_CURVE_WITH_KNOTS('',3,(#214956,#214957,#214958,#214959,#214960,
#214961,#214962,#214963,#214964,#214965,#214966,#214967,#214968,#214969,
#214970,#214971,#214972,#214973,#214974,#214975,#214976,#214977,#214978,
#214979,#214980,#214981,#214982,#214983,#214984,#214985,#214986,#214987,
#214988,#214989,#214990,#214991,#214992,#214993,#214994,#214995,#214996,
#214997,#214998,#214999,#215000,#215001,#215002,#215003,#215004,#215005,
#215006,#215007,#215008,#215009,#215010,#215011,#215012,#215013,#215014,
#215015,#215016,#215017,#215018,#215019,#215020,#215021,#215022,#215023,
#215024,#215025,#215026,#215027,#215028,#215029,#215030,#215031),
 .UNSPECIFIED.,.F.,.F.,(4,3,3,3,3,3,3,3,3,3,3,3,3,3,3,3,3,3,3,3,3,3,3,3,
3,4),(384.369385902676,384.451847506434,384.534308444313,384.616768743711,
384.699228432025,384.781687536647,384.86414608497,384.946604104384,385.029061622277,
385.11573879535,385.198205580958,385.28067069409,385.363134244396,385.44559634151,
385.528057095042,385.610516614585,385.692975009712,385.775432389983,385.857898775802,
385.940361977426,386.022822433374,386.10528058201,386.187746186022,386.2702060646,
386.352670176336,386.415896391442),.UNSPECIFIED.);
#3508=B_SPLINE_CURVE_WITH_KNOTS('',3,(#215032,#215033,#215034,#215035,#215036,
#215037,#215038,#215039,#215040,#215041,#215042,#215043,#215044,#215045,
#215046,#215047,#215048,#215049,#215050,#215051,#215052,#215053,#215054,
#215055,#215056,#215057,#215058,#215059,#215060,#215061,#215062,#215063,
#215064,#215065,#215066,#215067,#215068,#215069,#215070,#215071,#215072,
#215073,#215074,#215075,#215076,#215077,#215078,#215079,#215080,#215081,
#215082,#215083,#215084,#215085,#215086,#215087,#215088,#215089,#215090,
#215091,#215092,#215093,#215094,#215095,#215096,#215097,#215098,#215099,
#215100,#215101,#215102,#215103,#215104,#215105,#215106,#215107,#215108,
#215109,#215110,#215111,#215112,#215113,#215114,#215115,#215116,#215117,
#215118,#215119,#215120,#215121,#215122,#215123,#215124,#215125,#215126,
#215127,#215128,#215129,#215130,#215131,#215132,#215133,#215134,#215135,
#215136,#215137,#215138,#215139,#215140,#215141,#215142,#215143,#215144,
#215145,#215146,#215147,#215148,#215149,#215150,#215151,#215152,#215153,
#215154,#215155,#215156,#215157,#215158,#215159,#215160,#215161,#215162,
#215163,#215164,#215165,#215166,#215167,#215168,#215169,#215170,#215171,
#215172,#215173,#215174,#215175,#215176,#215177,#215178,#215179,#215180,
#215181,#215182,#215183,#215184,#215185,#215186,#215187,#215188),
 .UNSPECIFIED.,.F.,.F.,(4,3,3,3,3,3,3,3,3,3,3,3,3,3,3,3,3,3,3,3,3,3,3,3,
3,3,3,3,3,3,3,3,3,3,3,3,3,3,3,3,3,3,3,3,3,3,3,3,3,3,3,3,4),(386.415896391544,
386.498358597629,386.580820455418,386.663281971759,386.745743153503,386.828204007499,
386.910664540598,386.993124759648,387.075584671499,387.158044282998,387.240503600995,
387.322962632337,387.405421383872,387.487879862449,387.570338074913,387.652796028114,
387.735253728896,387.817711184108,387.900168400596,387.986180988385,388.069505682806,
388.151972288365,388.234438049715,388.316902994273,388.399367149451,388.481830542659,
388.564293201302,388.646755152786,388.729216424513,388.811677043881,388.894137038288,
388.976596435129,389.059055261798,389.141513545684,389.223971314178,389.306428594666,
389.390562508115,389.473028506413,389.555492882962,389.637955747404,389.720417209361,
389.802877378435,389.885336364209,389.967794276252,390.053391392953,390.135856129896,
390.218317902195,390.300777148286,390.383234306464,390.465696825363,390.548154496647,
390.630613287555,390.652571209856),.UNSPECIFIED.);
#3509=B_SPLINE_CURVE_WITH_KNOTS('',3,(#215194,#215195,#215196,#215197,#215198,
#215199,#215200,#215201,#215202,#215203,#215204,#215205,#215206,#215207,
#215208,#215209,#215210,#215211,#215212,#215213,#215214,#215215,#215216,
#215217,#215218,#215219,#215220,#215221,#215222,#215223,#215224,#215225,
#215226,#215227,#215228,#215229,#215230,#215231,#215232,#215233,#215234,
#215235,#215236,#215237,#215238,#215239,#215240,#215241,#215242,#215243,
#215244,#215245,#215246,#215247,#215248,#215249,#215250,#215251,#215252,
#215253,#215254,#215255,#215256,#215257,#215258,#215259,#215260,#215261,
#215262,#215263,#215264,#215265,#215266,#215267,#215268,#215269,#215270,
#215271,#215272,#215273,#215274,#215275,#215276,#215277,#215278,#215279,
#215280,#215281,#215282,#215283,#215284,#215285,#215286,#215287,#215288,
#215289,#215290,#215291,#215292,#215293,#215294,#215295,#215296,#215297,
#215298,#215299,#215300,#215301,#215302,#215303,#215304,#215305,#215306,
#215307,#215308,#215309,#215310,#215311,#215312,#215313,#215314,#215315,
#215316,#215317,#215318,#215319,#215320,#215321,#215322,#215323,#215324,
#215325,#215326,#215327,#215328,#215329,#215330,#215331,#215332,#215333,
#215334,#215335,#215336,#215337,#215338,#215339,#215340,#215341,#215342,
#215343,#215344,#215345,#215346,#215347,#215348,#215349,#215350,#215351,
#215352,#215353,#215354,#215355,#215356,#215357,#215358,#215359,#215360,
#215361,#215362,#215363,#215364,#215365),.UNSPECIFIED.,.F.,.F.,(4,3,3,3,
3,3,3,3,3,3,3,3,3,3,3,3,3,3,3,3,3,3,3,3,3,3,3,3,3,3,3,3,3,3,3,3,3,3,3,3,
3,3,3,3,3,3,3,3,3,3,3,3,3,3,3,3,3,4),(392.699081698724,392.79972704102,
392.815927561568,392.894306582437,392.972619333752,393.050880229906,393.129103647704,
393.207303935863,393.285512125028,393.363728178517,393.441965095746,393.5202358859,
393.598599465372,393.67701259483,393.755542977343,393.81466729743,393.890723804189,
393.966684622188,394.042566542813,394.118386276325,394.194160470661,394.27156629099,
394.34731404711,394.423069052643,394.498846317879,394.577486496732,394.653395683206,
394.729361675153,394.805433872768,394.813407033292,394.89096588483,394.968432428718,
395.045822332004,395.12315120669,395.200434620826,395.277695667392,395.354946368229,
395.432200770908,395.509472922434,395.586818260565,395.664201034284,395.741690529925,
395.812146769154,395.896366052048,395.980458731022,396.064345356835,396.148102346221,
396.231644048878,396.311516637085,396.388883832911,396.466269422395,396.543687204217,
396.621192125864,396.698746725151,396.776408072139,396.810886505016,396.890507206535,
396.935844184755),.UNSPECIFIED.);
#3510=B_SPLINE_CURVE_WITH_KNOTS('',3,(#215366,#215367,#215368,#215369,#215370,
#215371,#215372,#215373,#215374,#215375,#215376,#215377,#215378,#215379,
#215380,#215381,#215382,#215383,#215384,#215385,#215386,#215387,#215388,
#215389,#215390,#215391,#215392,#215393,#215394,#215395,#215396,#215397,
#215398,#215399,#215400,#215401,#215402,#215403,#215404,#215405,#215406,
#215407,#215408,#215409,#215410,#215411,#215412,#215413,#215414,#215415,
#215416,#215417,#215418,#215419,#215420,#215421,#215422,#215423,#215424,
#215425,#215426,#215427,#215428,#215429,#215430,#215431,#215432,#215433,
#215434,#215435,#215436,#215437,#215438,#215439,#215440,#215441,#215442,
#215443,#215444),.UNSPECIFIED.,.F.,.F.,(4,3,3,3,3,3,3,3,3,3,3,3,3,3,3,3,
3,3,3,3,3,3,3,3,3,3,4),(390.652606861601,390.735527475722,390.818448089843,
390.895163096693,390.971811009058,391.048406520798,391.124965418497,391.201502802577,
391.278044323031,391.317817957774,391.402494295978,391.487316780488,391.572339151359,
391.657448033164,391.742677572534,391.817187825705,391.89874408837,391.980225028041,
392.06430819444,392.145633946956,392.231095820296,392.316557693636,392.393372171278,
392.470216316175,392.547073509146,392.624000772024,392.699081698624),
 .UNSPECIFIED.);
#3511=B_SPLINE_CURVE_WITH_KNOTS('',3,(#215446,#215447,#215448,#215449,#215450,
#215451,#215452,#215453,#215454,#215455,#215456,#215457,#215458,#215459,
#215460,#215461,#215462,#215463,#215464,#215465,#215466,#215467,#215468,
#215469,#215470,#215471,#215472,#215473,#215474,#215475,#215476,#215477,
#215478,#215479,#215480,#215481,#215482,#215483,#215484,#215485,#215486,
#215487,#215488,#215489,#215490,#215491,#215492,#215493,#215494,#215495,
#215496,#215497,#215498,#215499,#215500,#215501,#215502,#215503,#215504,
#215505,#215506,#215507,#215508,#215509,#215510,#215511,#215512,#215513,
#215514,#215515,#215516,#215517,#215518,#215519,#215520,#215521),
 .UNSPECIFIED.,.F.,.F.,(4,3,3,3,3,3,3,3,3,3,3,3,3,3,3,3,3,3,3,3,3,3,3,3,
3,4),(390.652571209856,390.735032813614,390.817493751493,390.899954050891,
390.982413739205,391.064872843827,391.14733139215,391.229789411564,391.312246929457,
391.398924102536,391.481390888145,391.563856001276,391.646319551583,391.728781648697,
391.811242402229,391.893701921771,391.976160316898,392.058617697169,392.141084082989,
392.223547284613,392.306007740561,392.388465889198,392.470931493209,392.553391371787,
392.635855483523,392.699081698724),.UNSPECIFIED.);
#3512=B_SPLINE_CURVE_WITH_KNOTS('',3,(#215522,#215523,#215524,#215525,#215526,
#215527,#215528,#215529,#215530,#215531,#215532,#215533,#215534,#215535,
#215536,#215537,#215538,#215539,#215540,#215541,#215542,#215543,#215544,
#215545,#215546,#215547,#215548,#215549,#215550,#215551,#215552,#215553,
#215554,#215555,#215556,#215557,#215558,#215559,#215560,#215561,#215562,
#215563,#215564,#215565,#215566,#215567,#215568,#215569,#215570,#215571,
#215572,#215573,#215574,#215575,#215576,#215577,#215578,#215579,#215580,
#215581,#215582,#215583,#215584,#215585,#215586,#215587,#215588,#215589,
#215590,#215591,#215592,#215593,#215594,#215595,#215596,#215597,#215598,
#215599,#215600,#215601,#215602,#215603,#215604,#215605,#215606,#215607,
#215608,#215609,#215610,#215611,#215612,#215613,#215614,#215615,#215616,
#215617,#215618,#215619,#215620,#215621,#215622,#215623,#215624,#215625,
#215626,#215627,#215628,#215629,#215630,#215631,#215632,#215633,#215634,
#215635,#215636,#215637,#215638,#215639,#215640,#215641,#215642,#215643,
#215644,#215645,#215646,#215647,#215648,#215649,#215650,#215651,#215652,
#215653,#215654,#215655,#215656,#215657,#215658,#215659,#215660,#215661,
#215662,#215663,#215664,#215665,#215666,#215667,#215668,#215669,#215670,
#215671,#215672,#215673,#215674,#215675,#215676,#215677,#215678,#215679,
#215680,#215681,#215682,#215683,#215684,#215685,#215686,#215687,#215688,
#215689,#215690),.UNSPECIFIED.,.F.,.F.,(4,3,3,3,3,3,3,3,3,3,3,3,3,3,3,3,
3,3,3,3,3,3,3,3,3,3,3,3,3,3,3,3,3,3,3,3,3,3,3,3,3,3,3,3,3,3,3,3,3,3,3,3,
3,3,3,3,4),(392.699081698724,392.777830761647,392.85663332107,392.935550977874,
393.014532882935,393.093641726665,393.133611947173,393.213232685917,393.292780513573,
393.372267742848,393.451706639762,393.531109432568,393.610494645467,393.689870876019,
393.769249205569,393.84864071544,393.928085950271,394.007559531051,394.087106643101,
394.132351683035,394.209066689885,394.28571460225,394.36231011399,394.438869011689,
394.515406395769,394.591947916223,394.631721550966,394.71639788917,394.801220373679,
394.886242744551,394.971351626355,395.056581165726,395.131091418897,395.212647681562,
395.294128621233,395.378211787632,395.459537540149,395.544999413488,395.630461286828,
395.709864627708,395.789286398866,395.868737376503,395.948261542719,396.02782745326,
396.107477301459,396.12983115476,396.208217376618,396.286535395908,396.36764403172,
396.445867701643,396.524071001022,396.602266930714,396.680468484783,396.75871325386,
396.836983558174,396.915317696091,396.935404482405),.UNSPECIFIED.);
#3513=B_SPLINE_CURVE_WITH_KNOTS('',3,(#215696,#215697,#215698,#215699,#215700,
#215701,#215702,#215703,#215704,#215705,#215706,#215707,#215708,#215709,
#215710,#215711,#215712,#215713,#215714,#215715,#215716,#215717,#215718,
#215719,#215720,#215721,#215722,#215723,#215724,#215725,#215726,#215727,
#215728,#215729,#215730,#215731,#215732,#215733,#215734,#215735,#215736,
#215737,#215738,#215739,#215740,#215741,#215742,#215743,#215744,#215745,
#215746,#215747,#215748,#215749,#215750,#215751,#215752,#215753,#215754,
#215755,#215756,#215757,#215758,#215759,#215760,#215761,#215762,#215763,
#215764,#215765,#215766,#215767,#215768,#215769,#215770,#215771,#215772,
#215773,#215774,#215775,#215776,#215777,#215778,#215779,#215780,#215781,
#215782,#215783,#215784,#215785,#215786,#215787,#215788,#215789,#215790,
#215791,#215792,#215793,#215794,#215795,#215796,#215797,#215798,#215799,
#215800,#215801,#215802,#215803,#215804,#215805,#215806,#215807,#215808,
#215809,#215810,#215811,#215812,#215813,#215814,#215815,#215816,#215817,
#215818,#215819,#215820,#215821,#215822,#215823,#215824,#215825,#215826,
#215827,#215828,#215829,#215830,#215831,#215832,#215833,#215834,#215835,
#215836,#215837,#215838,#215839,#215840,#215841,#215842,#215843,#215844,
#215845,#215846,#215847,#215848,#215849,#215850,#215851,#215852,#215853,
#215854,#215855,#215856,#215857,#215858,#215859,#215860,#215861,#215862,
#215863,#215864),.UNSPECIFIED.,.F.,.F.,(4,3,3,3,3,3,3,3,3,3,3,3,3,3,3,3,
3,3,3,3,3,3,3,3,3,3,3,3,3,3,3,3,3,3,3,3,3,3,3,3,3,3,3,3,3,3,3,3,3,3,3,3,
3,3,3,3,4),(398.982267005904,399.063634215596,399.142909954305,399.225322899488,
399.307735844672,399.387139185638,399.466560956889,399.546011934626,399.625536100951,
399.705102011607,399.784751859929,399.807105712603,399.885484732299,399.963797482429,
400.042058377388,400.120281793984,400.198482080935,400.276690268887,400.354906321163,
400.433143237177,400.511414026118,400.589777604387,400.668190732646,400.746721113976,
400.805845448465,400.881901957122,400.957862777017,401.033744699532,401.10956443493,
401.185338631146,401.262744450294,401.338492208272,401.414247215654,401.490024482729,
401.568664658129,401.644573846404,401.720539840141,401.79661203952,401.804585184327,
401.882144036821,401.959610581679,402.037000485951,402.114329361636,402.191612776783,
402.268873824374,402.346124526246,402.423378929968,402.500651082543,402.577996421729,
402.655379196506,402.732868693204,402.803324920189,402.88755931429,402.971602904374,
403.05552503406,403.139244949316,403.219444425455),.UNSPECIFIED.);
#3514=B_SPLINE_CURVE_WITH_KNOTS('',3,(#215865,#215866,#215867,#215868,#215869,
#215870,#215871,#215872,#215873,#215874,#215875,#215876,#215877,#215878,
#215879,#215880,#215881,#215882,#215883,#215884,#215885,#215886,#215887,
#215888,#215889,#215890,#215891,#215892,#215893,#215894,#215895,#215896,
#215897,#215898,#215899,#215900,#215901,#215902,#215903,#215904,#215905,
#215906,#215907,#215908,#215909,#215910,#215911,#215912,#215913,#215914,
#215915,#215916,#215917,#215918,#215919,#215920,#215921,#215922,#215923,
#215924,#215925,#215926,#215927,#215928,#215929,#215930,#215931,#215932,
#215933,#215934,#215935,#215936,#215937,#215938,#215939,#215940,#215941,
#215942,#215943),.UNSPECIFIED.,.F.,.F.,(4,3,3,3,3,3,3,3,3,3,3,3,3,3,3,3,
3,3,3,3,3,3,3,3,3,3,4),(396.935844184755,397.015355975617,397.094814162802,
397.174230989716,397.253655396111,397.333034128618,397.412410198368,397.491794685822,
397.571252574586,397.650712739704,397.730252956172,397.809626240879,397.886341248167,
397.962989160966,398.039584673138,398.116143571262,398.192680955763,398.269222476631,
398.30899610881,398.39367244587,398.478494929206,398.563517298882,398.648626179487,
398.733855717675,398.808365976741,398.898235537162,398.982267005821),
 .UNSPECIFIED.);
#3515=B_SPLINE_CURVE_WITH_KNOTS('',3,(#215945,#215946,#215947,#215948,#215949,
#215950,#215951,#215952,#215953,#215954,#215955,#215956,#215957,#215958,
#215959,#215960,#215961,#215962,#215963,#215964,#215965,#215966,#215967,
#215968,#215969,#215970,#215971,#215972,#215973,#215974,#215975,#215976,
#215977,#215978,#215979,#215980,#215981,#215982,#215983,#215984,#215985,
#215986,#215987,#215988,#215989,#215990,#215991,#215992,#215993,#215994,
#215995,#215996,#215997,#215998,#215999,#216000,#216001,#216002,#216003,
#216004,#216005,#216006,#216007,#216008,#216009,#216010,#216011,#216012,
#216013,#216014,#216015,#216016,#216017,#216018,#216019,#216020,#216021,
#216022,#216023,#216024,#216025,#216026,#216027,#216028,#216029),
 .UNSPECIFIED.,.F.,.F.,(4,3,3,3,3,3,3,3,3,3,3,3,3,3,3,3,3,3,3,3,3,3,3,3,
3,3,3,3,4),(396.935404482405,397.013834312093,397.092374912414,397.128570890622,
397.204627397381,397.28058821538,397.356470136005,397.432289869517,397.508064063853,
397.585469884182,397.661217640302,397.736972645836,397.812749911071,397.891390089924,
397.967299276398,398.043265268346,398.11933746596,398.127310626484,398.204177103907,
398.280951228283,398.3576492898,398.435726504298,398.512319806502,398.588890633907,
398.66545359003,398.74465694397,398.821274599742,398.901770802766,398.982267005789),
 .UNSPECIFIED.);
#3516=B_SPLINE_CURVE_WITH_KNOTS('',3,(#216030,#216031,#216032,#216033,#216034,
#216035,#216036,#216037,#216038,#216039,#216040,#216041,#216042,#216043,
#216044,#216045,#216046,#216047,#216048,#216049,#216050,#216051,#216052,
#216053,#216054,#216055,#216056,#216057,#216058,#216059,#216060,#216061,
#216062,#216063,#216064,#216065,#216066,#216067,#216068,#216069,#216070,
#216071,#216072,#216073,#216074,#216075,#216076,#216077,#216078,#216079,
#216080,#216081,#216082,#216083,#216084,#216085,#216086,#216087,#216088,
#216089,#216090,#216091,#216092,#216093,#216094,#216095,#216096,#216097,
#216098,#216099,#216100,#216101,#216102,#216103,#216104,#216105,#216106,
#216107,#216108,#216109,#216110,#216111,#216112,#216113,#216114,#216115,
#216116,#216117,#216118,#216119,#216120,#216121,#216122,#216123,#216124,
#216125,#216126,#216127,#216128,#216129,#216130,#216131,#216132,#216133,
#216134,#216135,#216136,#216137,#216138,#216139,#216140,#216141,#216142,
#216143,#216144,#216145,#216146,#216147,#216148,#216149,#216150,#216151,
#216152,#216153,#216154,#216155,#216156,#216157,#216158,#216159,#216160,
#216161,#216162,#216163,#216164,#216165,#216166,#216167,#216168,#216169,
#216170,#216171,#216172,#216173,#216174,#216175,#216176,#216177,#216178,
#216179,#216180,#216181,#216182,#216183,#216184,#216185,#216186,#216187,
#216188,#216189,#216190,#216191,#216192,#216193,#216194,#216195,#216196,
#216197,#216198),.UNSPECIFIED.,.F.,.F.,(4,3,3,3,3,3,3,3,3,3,3,3,3,3,3,3,
3,3,3,3,3,3,3,3,3,3,3,3,3,3,3,3,3,3,3,3,3,3,3,3,3,3,3,3,3,3,3,3,3,3,3,3,
3,3,3,3,4),(398.982267005904,399.095287094402,399.126050362346,399.21026964524,
399.294362324215,399.378248950028,399.462005939414,399.545547642071,399.625420230277,
399.702787426103,399.780173015587,399.857590797408,399.935095719056,400.012650318343,
400.09031166533,400.124790098208,400.204410836847,400.283958664396,400.363445893565,
400.442884790371,400.522287583071,400.601672795864,400.681049026311,400.760427355757,
400.839818865524,400.919264100254,400.998737680935,401.078284792888,401.12352983407,
401.200244841358,401.276892754157,401.353488266328,401.430047164452,401.506584548954,
401.583126069822,401.622899702002,401.707576039062,401.792398522399,401.877420892076,
401.962529772682,402.04775931087,402.122269569933,402.203825833388,402.285306773841,
402.369389939847,402.450715693115,402.536177565489,402.621639437864,402.70104277883,
402.780464550081,402.859915527818,402.939439694143,403.0190056048,403.098655453121,
403.121009305795,403.199396366739,403.219160745219),.UNSPECIFIED.);
#3517=B_SPLINE_CURVE_WITH_KNOTS('',3,(#216204,#216205,#216206,#216207,#216208,
#216209,#216210,#216211,#216212,#216213,#216214,#216215,#216216,#216217,
#216218,#216219,#216220,#216221,#216222,#216223,#216224,#216225,#216226,
#216227,#216228,#216229,#216230,#216231,#216232,#216233,#216234,#216235,
#216236,#216237,#216238,#216239,#216240,#216241,#216242,#216243,#216244,
#216245,#216246,#216247,#216248,#216249,#216250,#216251,#216252,#216253,
#216254,#216255,#216256,#216257,#216258,#216259,#216260,#216261,#216262,
#216263,#216264,#216265,#216266,#216267,#216268,#216269,#216270,#216271,
#216272,#216273,#216274,#216275,#216276,#216277,#216278,#216279,#216280,
#216281,#216282,#216283,#216284,#216285,#216286,#216287,#216288,#216289,
#216290,#216291,#216292,#216293,#216294,#216295,#216296,#216297,#216298,
#216299,#216300,#216301,#216302,#216303,#216304,#216305,#216306,#216307,
#216308,#216309,#216310,#216311,#216312,#216313,#216314,#216315,#216316,
#216317,#216318,#216319,#216320,#216321,#216322,#216323,#216324,#216325,
#216326,#216327,#216328,#216329,#216330,#216331,#216332,#216333,#216334,
#216335,#216336,#216337,#216338,#216339,#216340,#216341,#216342,#216343,
#216344,#216345,#216346,#216347,#216348,#216349,#216350,#216351,#216352,
#216353,#216354,#216355,#216356,#216357,#216358,#216359,#216360),
 .UNSPECIFIED.,.F.,.F.,(4,3,3,3,3,3,3,3,3,3,3,3,3,3,3,3,3,3,3,3,3,3,3,3,
3,3,3,3,3,3,3,3,3,3,3,3,3,3,3,3,3,3,3,3,3,3,3,3,3,3,3,3,4),(405.265452313083,
405.347914519169,405.430376376957,405.512837893298,405.595299075042,405.677759929038,
405.760220462137,405.842680681187,405.925140593038,406.007600204537,406.090059522534,
406.172518553876,406.254977305411,406.337435783987,406.419893996452,406.502351949652,
406.584809650435,406.667267105646,406.749724322134,406.835736909923,406.919061604344,
407.001528209903,407.083993971253,407.166458915812,407.24892307099,407.331386464197,
407.41384912284,407.496311074324,407.578772346051,407.661232965419,407.743692959826,
407.826152356668,407.908611183336,407.991069467222,408.073527235716,408.155984516203,
408.240118429653,408.322584427951,408.4050488045,408.487511668942,408.569973130899,
408.652433299973,408.734892285747,408.81735019779,408.902947314491,408.985412051434,
409.067873823733,409.150333069824,409.232790228002,409.315252746901,409.397710418185,
409.480169209093,409.502127131395),.UNSPECIFIED.);
#3518=B_SPLINE_CURVE_WITH_KNOTS('',3,(#216361,#216362,#216363,#216364,#216365,
#216366,#216367,#216368,#216369,#216370,#216371,#216372,#216373,#216374,
#216375,#216376,#216377,#216378,#216379,#216380,#216381,#216382,#216383,
#216384,#216385,#216386,#216387,#216388,#216389,#216390,#216391,#216392,
#216393,#216394,#216395,#216396,#216397,#216398,#216399,#216400,#216401,
#216402,#216403,#216404,#216405,#216406,#216407,#216408,#216409,#216410,
#216411,#216412,#216413,#216414,#216415,#216416,#216417,#216418,#216419,
#216420,#216421,#216422,#216423,#216424,#216425,#216426,#216427,#216428,
#216429,#216430,#216431,#216432,#216433,#216434,#216435,#216436,#216437,
#216438,#216439,#216440,#216441,#216442),.UNSPECIFIED.,.F.,.F.,(4,3,3,3,
3,3,3,3,3,3,3,3,3,3,3,3,3,3,3,3,3,3,3,3,3,3,3,4),(403.219444425455,403.302694788121,
403.380062027565,403.457447661111,403.534865487393,403.612370453918,403.689925098347,
403.767586490629,403.802064656052,403.881685351219,403.96123313507,404.040720320409,
404.120159173352,404.199561922249,404.278947091578,404.358323278832,404.437701565444,
404.517093032819,404.596538226116,404.676011765899,404.755558838146,404.800804391914,
404.877998399174,404.955121803432,405.03262963019,405.109651357303,405.187402233883,
405.265153110462),.UNSPECIFIED.);
#3519=B_SPLINE_CURVE_WITH_KNOTS('',3,(#216444,#216445,#216446,#216447,#216448,
#216449,#216450,#216451,#216452,#216453,#216454,#216455,#216456,#216457,
#216458,#216459,#216460,#216461,#216462,#216463,#216464,#216465,#216466,
#216467,#216468,#216469,#216470,#216471,#216472,#216473,#216474,#216475,
#216476,#216477,#216478,#216479,#216480,#216481,#216482,#216483,#216484,
#216485,#216486,#216487,#216488,#216489,#216490,#216491,#216492,#216493,
#216494,#216495,#216496,#216497,#216498,#216499,#216500,#216501,#216502,
#216503,#216504,#216505,#216506,#216507,#216508,#216509,#216510,#216511,
#216512,#216513,#216514,#216515,#216516,#216517,#216518,#216519,#216520,
#216521,#216522,#216523,#216524,#216525),.UNSPECIFIED.,.F.,.F.,(4,3,3,3,
3,3,3,3,3,3,3,3,3,3,3,3,3,3,3,3,3,3,3,3,3,3,3,4),(403.219160745219,403.297459048369,
403.375709128334,403.453925353941,403.532122068307,403.610331014814,403.688551105634,
403.766795341942,403.845076736576,403.923451700316,404.00187918644,404.080418314602,
404.119749041657,404.195805550314,404.271766370209,404.347648292724,404.423468028122,
404.499242224338,404.576648043486,404.652395801464,404.728150808847,404.803928075921,
404.882568251321,404.958477439596,405.034443433334,405.110515632713,405.118488777519,
405.265452313083),.UNSPECIFIED.);
#3520=B_SPLINE_CURVE_WITH_KNOTS('',3,(#216526,#216527,#216528,#216529,#216530,
#216531,#216532,#216533,#216534,#216535,#216536,#216537,#216538,#216539,
#216540,#216541,#216542,#216543,#216544,#216545,#216546,#216547,#216548,
#216549,#216550,#216551,#216552,#216553,#216554,#216555,#216556,#216557,
#216558,#216559,#216560,#216561,#216562,#216563,#216564,#216565,#216566,
#216567,#216568,#216569,#216570,#216571,#216572,#216573,#216574,#216575,
#216576,#216577,#216578,#216579,#216580,#216581,#216582,#216583,#216584,
#216585,#216586,#216587,#216588,#216589,#216590,#216591,#216592,#216593,
#216594,#216595,#216596,#216597,#216598,#216599,#216600,#216601,#216602,
#216603,#216604,#216605,#216606,#216607,#216608,#216609,#216610,#216611,
#216612,#216613,#216614,#216615,#216616,#216617,#216618,#216619,#216620,
#216621,#216622,#216623,#216624,#216625,#216626,#216627,#216628,#216629,
#216630,#216631,#216632,#216633,#216634,#216635,#216636,#216637,#216638,
#216639,#216640,#216641,#216642,#216643,#216644,#216645,#216646,#216647,
#216648,#216649,#216650,#216651,#216652,#216653,#216654,#216655,#216656,
#216657,#216658,#216659,#216660,#216661,#216662,#216663,#216664,#216665,
#216666,#216667,#216668,#216669,#216670,#216671,#216672,#216673,#216674,
#216675,#216676,#216677,#216678,#216679,#216680,#216681,#216682,#216683,
#216684,#216685,#216686,#216687,#216688,#216689,#216690,#216691,#216692,
#216693,#216694),.UNSPECIFIED.,.F.,.F.,(4,3,3,3,3,3,3,3,3,3,3,3,3,3,3,3,
3,3,3,3,3,3,3,3,3,3,3,3,3,3,3,3,3,3,3,3,3,3,3,3,3,3,3,3,3,3,3,3,3,3,3,3,
3,3,3,3,4),(405.265452313166,405.341378517376,405.417225780084,405.493010896021,
405.571038098191,405.646755981067,405.722466089584,405.798183499663,405.873923291857,
405.949735362879,406.02559095927,406.101538247612,406.117228513381,406.201447766723,
406.285540416405,406.369427013778,406.45318397536,406.536725651581,406.616598381312,
406.693965620755,406.771351254302,406.848769080582,406.926274047107,407.003828691536,
407.081490083817,407.115968249244,407.195588944411,407.275136728262,407.354623913601,
407.434062766544,407.513465515443,407.592850684772,407.672226872027,407.751605158638,
407.830996626014,407.910441819311,407.989915359094,408.069462431341,408.114707985106,
408.191423080311,408.268071080107,408.344666678293,408.421225660755,408.497763128661,
408.574304731257,408.614077853037,408.69875415266,408.783576599501,408.868598934868,
408.953707782589,409.038937290848,409.113447720968,409.19501438971,409.276478797015,
409.357879826288,409.439202918048,409.502552124195),.UNSPECIFIED.);
#3521=B_SPLINE_CURVE_WITH_KNOTS('',3,(#216700,#216701,#216702,#216703,#216704,
#216705,#216706,#216707,#216708,#216709,#216710,#216711,#216712,#216713,
#216714,#216715,#216716,#216717,#216718,#216719,#216720,#216721,#216722,
#216723,#216724,#216725,#216726,#216727,#216728,#216729,#216730,#216731,
#216732,#216733,#216734,#216735,#216736,#216737,#216738,#216739,#216740,
#216741,#216742,#216743,#216744,#216745,#216746,#216747,#216748,#216749,
#216750,#216751,#216752,#216753,#216754,#216755,#216756,#216757,#216758,
#216759,#216760,#216761,#216762,#216763,#216764,#216765,#216766,#216767,
#216768,#216769,#216770,#216771,#216772,#216773,#216774,#216775,#216776,
#216777,#216778,#216779,#216780,#216781,#216782,#216783,#216784,#216785,
#216786,#216787,#216788,#216789,#216790,#216791,#216792,#216793,#216794,
#216795,#216796,#216797,#216798,#216799,#216800,#216801,#216802,#216803,
#216804,#216805,#216806,#216807,#216808,#216809,#216810,#216811,#216812,
#216813,#216814,#216815,#216816,#216817,#216818,#216819,#216820,#216821,
#216822,#216823,#216824,#216825,#216826,#216827,#216828,#216829,#216830,
#216831,#216832,#216833,#216834,#216835,#216836,#216837,#216838,#216839,
#216840,#216841,#216842,#216843,#216844,#216845,#216846,#216847,#216848,
#216849,#216850,#216851,#216852,#216853,#216854,#216855,#216856),
 .UNSPECIFIED.,.F.,.F.,(4,3,3,3,3,3,3,3,3,3,3,3,3,3,3,3,3,3,3,3,3,3,3,3,
3,3,3,3,3,3,3,3,3,3,3,3,3,3,3,3,3,3,3,3,3,3,3,3,3,3,3,3,4),(411.548637620348,
411.631099826433,411.713561684221,411.796023200562,411.878484382306,411.960945236303,
412.043405769402,412.125865988452,412.208325900302,412.290785511802,412.373244829798,
412.45570386114,412.538162612676,412.620621091252,412.703079303717,412.785537256917,
412.8679949577,412.950452412912,413.032909629399,413.118922217186,413.202246911604,
413.284713517163,413.367179278513,413.449644223071,413.532108378249,413.614571771457,
413.6970344301,413.779496381584,413.86195765331,413.944418272679,414.026878267086,
414.109337663927,414.191796490595,414.274254774482,414.356712542975,414.439169823463,
414.523303736907,414.605769735206,414.688234111755,414.770696976197,414.853158438153,
414.935618607227,415.018077593002,415.100535505045,415.186132621736,415.26859735868,
415.351059130978,415.433518377069,415.515975535248,415.598438054146,415.68089572543,
415.763354516338,415.785312438575),.UNSPECIFIED.);
#3522=B_SPLINE_CURVE_WITH_KNOTS('',3,(#216857,#216858,#216859,#216860,#216861,
#216862,#216863,#216864,#216865,#216866,#216867,#216868,#216869,#216870,
#216871,#216872,#216873,#216874,#216875,#216876,#216877,#216878,#216879,
#216880,#216881,#216882,#216883,#216884,#216885,#216886,#216887,#216888,
#216889,#216890,#216891,#216892,#216893,#216894,#216895,#216896,#216897,
#216898,#216899,#216900,#216901,#216902,#216903,#216904,#216905,#216906,
#216907,#216908,#216909,#216910,#216911,#216912,#216913,#216914,#216915,
#216916,#216917,#216918,#216919,#216920,#216921,#216922,#216923,#216924,
#216925,#216926,#216927,#216928,#216929,#216930,#216931,#216932),
 .UNSPECIFIED.,.F.,.F.,(4,3,3,3,3,3,3,3,3,3,3,3,3,3,3,3,3,3,3,3,3,3,3,3,
3,4),(409.502127131395,409.584588735153,409.667049673032,409.74950997243,
409.831969660743,409.914428765366,409.996887313689,410.079345333103,410.161802850996,
410.248480024075,410.330946809684,410.413411922815,410.495875473122,410.578337570236,
410.660798323768,410.74325784331,410.825716238437,410.908173618708,410.990640004527,
411.073103206151,411.1555636621,411.238021810736,411.320487414748,411.402947293325,
411.485411405062,411.548637620263),.UNSPECIFIED.);
#3523=B_SPLINE_CURVE_WITH_KNOTS('',3,(#216934,#216935,#216936,#216937,#216938,
#216939,#216940,#216941,#216942,#216943,#216944,#216945,#216946,#216947,
#216948,#216949,#216950,#216951,#216952,#216953,#216954,#216955,#216956,
#216957,#216958,#216959,#216960,#216961,#216962,#216963,#216964,#216965,
#216966,#216967,#216968,#216969,#216970,#216971,#216972,#216973,#216974,
#216975,#216976,#216977,#216978,#216979,#216980,#216981,#216982,#216983,
#216984,#216985,#216986,#216987,#216988,#216989,#216990,#216991,#216992,
#216993,#216994,#216995,#216996,#216997,#216998,#216999,#217000,#217001,
#217002,#217003,#217004,#217005,#217006,#217007,#217008,#217009,#217010,
#217011,#217012,#217013,#217014,#217015,#217016,#217017,#217018),
 .UNSPECIFIED.,.F.,.F.,(4,3,3,3,3,3,3,3,3,3,3,3,3,3,3,3,3,3,3,3,3,3,3,3,
3,3,3,3,4),(409.502552124195,409.583774702256,409.612817588899,409.692221759622,
409.771644372142,409.851096200842,409.930621227469,410.010188003439,410.089838719134,
410.11218745683,410.190565826128,410.268877919999,410.347138153801,410.425360905306,
410.50356052419,410.581768042459,410.659983424392,410.738219670257,410.81648979009,
410.894852704906,410.973265172075,411.051794902507,411.110927192692,411.192868380011,
411.274627957284,411.356135717751,411.4374923654,411.518643713388,411.548637620263),
 .UNSPECIFIED.);
#3524=B_SPLINE_CURVE_WITH_KNOTS('',3,(#217019,#217020,#217021,#217022,#217023,
#217024,#217025,#217026,#217027,#217028,#217029,#217030,#217031,#217032,
#217033,#217034,#217035,#217036,#217037,#217038,#217039,#217040,#217041,
#217042,#217043,#217044,#217045,#217046,#217047,#217048,#217049,#217050,
#217051,#217052,#217053,#217054,#217055,#217056,#217057,#217058,#217059,
#217060,#217061,#217062,#217063,#217064,#217065,#217066,#217067,#217068,
#217069,#217070,#217071,#217072,#217073,#217074,#217075,#217076,#217077,
#217078,#217079,#217080,#217081,#217082,#217083,#217084,#217085,#217086,
#217087,#217088,#217089,#217090,#217091,#217092,#217093,#217094,#217095,
#217096,#217097,#217098,#217099,#217100,#217101,#217102,#217103,#217104,
#217105,#217106,#217107,#217108,#217109,#217110,#217111,#217112,#217113,
#217114,#217115,#217116,#217117,#217118,#217119,#217120,#217121,#217122,
#217123,#217124,#217125,#217126,#217127,#217128,#217129,#217130,#217131,
#217132,#217133,#217134,#217135,#217136,#217137,#217138,#217139,#217140,
#217141,#217142,#217143,#217144,#217145,#217146,#217147,#217148,#217149,
#217150,#217151,#217152,#217153,#217154,#217155,#217156,#217157,#217158,
#217159,#217160,#217161,#217162,#217163,#217164,#217165,#217166,#217167,
#217168,#217169,#217170,#217171,#217172,#217173,#217174,#217175),
 .UNSPECIFIED.,.F.,.F.,(4,3,3,3,3,3,3,3,3,3,3,3,3,3,3,3,3,3,3,3,3,3,3,3,
3,3,3,3,3,3,3,3,3,3,3,3,3,3,3,3,3,3,3,3,3,3,3,3,3,3,3,3,4),(411.548637620263,
411.631099826349,411.713561684137,411.796023200478,411.878484382222,411.960945236218,
412.043405769317,412.125865988367,412.208325900218,412.290785511717,412.373244829714,
412.455703861056,412.538162612591,412.620621091167,412.703079303632,412.785537256832,
412.867994957615,412.950452412826,413.032909629314,413.118922217103,413.202246911524,
413.284713517082,413.367179278433,413.449644222991,413.532108378169,413.614571771376,
413.69703443002,413.779496381504,413.86195765323,413.944418272598,414.026878267006,
414.109337663847,414.191796490515,414.274254774401,414.356712542895,414.439169823382,
414.523303736832,414.60576973513,414.688234111679,414.770696976121,414.853158438078,
414.935618607152,415.018077592926,415.100535504969,415.18613262167,415.268597358613,
415.351059130912,415.433518377003,415.515975535181,415.59843805408,415.680895725363,
415.763354516271,415.785312438574),.UNSPECIFIED.);
#3525=B_SPLINE_CURVE_WITH_KNOTS('',3,(#217179,#217180,#217181,#217182,#217183,
#217184,#217185,#217186),.UNSPECIFIED.,.F.,.F.,(4,2,2,4),(-4.09265929953245,
-3.25801350823579,-2.42309659634093,-2.07498647268395),.UNSPECIFIED.);
#3526=B_SPLINE_CURVE_WITH_KNOTS('',3,(#217190,#217191,#217192,#217193,#217194,
#217195,#217196,#217197,#217198,#217199,#217200,#217201,#217202,#217203,
#217204,#217205,#217206,#217207,#217208,#217209,#217210,#217211,#217212,
#217213,#217214,#217215,#217216,#217217,#217218,#217219,#217220,#217221,
#217222,#217223,#217224,#217225,#217226,#217227,#217228,#217229,#217230,
#217231,#217232,#217233,#217234,#217235,#217236,#217237,#217238,#217239,
#217240,#217241,#217242,#217243,#217244,#217245,#217246,#217247,#217248,
#217249,#217250,#217251,#217252,#217253,#217254,#217255,#217256,#217257,
#217258,#217259,#217260,#217261,#217262,#217263,#217264,#217265,#217266,
#217267,#217268,#217269,#217270,#217271,#217272,#217273,#217274,#217275,
#217276,#217277,#217278,#217279,#217280,#217281,#217282,#217283,#217284,
#217285,#217286,#217287,#217288,#217289,#217290,#217291,#217292,#217293,
#217294,#217295,#217296,#217297,#217298,#217299,#217300,#217301,#217302,
#217303,#217304,#217305,#217306,#217307,#217308,#217309,#217310,#217311,
#217312,#217313,#217314,#217315,#217316,#217317,#217318,#217319,#217320,
#217321,#217322,#217323,#217324,#217325,#217326,#217327,#217328,#217329,
#217330,#217331,#217332,#217333,#217334,#217335,#217336,#217337,#217338,
#217339,#217340,#217341,#217342,#217343,#217344,#217345,#217346,#217347,
#217348,#217349,#217350,#217351,#217352,#217353,#217354,#217355,#217356,
#217357,#217358,#217359,#217360,#217361,#217362,#217363,#217364,#217365,
#217366,#217367,#217368,#217369,#217370,#217371,#217372,#217373,#217374,
#217375,#217376,#217377,#217378,#217379,#217380,#217381,#217382,#217383,
#217384,#217385,#217386,#217387,#217388,#217389,#217390,#217391,#217392,
#217393,#217394,#217395,#217396,#217397,#217398,#217399,#217400,#217401,
#217402,#217403,#217404,#217405,#217406,#217407,#217408,#217409,#217410,
#217411,#217412,#217413,#217414,#217415,#217416,#217417,#217418,#217419,
#217420,#217421,#217422,#217423,#217424,#217425,#217426,#217427,#217428,
#217429,#217430,#217431,#217432,#217433,#217434,#217435,#217436,#217437,
#217438,#217439,#217440,#217441,#217442,#217443,#217444,#217445,#217446,
#217447,#217448,#217449,#217450,#217451,#217452,#217453,#217454,#217455,
#217456,#217457,#217458,#217459,#217460,#217461,#217462,#217463,#217464,
#217465,#217466,#217467,#217468,#217469,#217470,#217471,#217472,#217473,
#217474,#217475,#217476,#217477,#217478,#217479,#217480,#217481,#217482,
#217483,#217484,#217485,#217486,#217487,#217488,#217489,#217490,#217491,
#217492,#217493,#217494,#217495,#217496,#217497,#217498,#217499,#217500,
#217501,#217502,#217503,#217504,#217505,#217506,#217507,#217508,#217509,
#217510,#217511,#217512,#217513,#217514,#217515,#217516,#217517,#217518,
#217519,#217520,#217521,#217522,#217523,#217524,#217525,#217526,#217527,
#217528,#217529),.UNSPECIFIED.,.F.,.F.,(4,2,2,2,2,2,2,2,2,2,2,2,2,2,2,2,
2,2,2,2,2,2,2,2,2,2,2,2,2,2,2,2,2,2,2,2,2,2,2,2,2,2,2,2,2,2,2,2,2,2,2,2,
2,2,2,2,2,2,2,2,2,2,2,2,2,2,2,2,2,2,2,2,2,2,2,2,2,2,2,2,2,2,2,2,2,2,2,2,
2,2,2,2,2,2,2,2,2,2,2,2,2,2,2,2,2,2,2,2,2,2,2,2,2,2,2,2,2,2,2,2,2,2,2,2,
2,2,2,2,2,2,2,2,2,2,2,2,2,2,2,2,2,2,2,2,2,2,2,2,2,2,2,2,2,2,2,2,2,2,2,2,
2,2,2,2,2,2,2,2,2,4),(6.83182211809342E-5,0.00813194064434937,0.0198778020713646,
0.0650590852607454,0.10988907756809,0.147886015884265,0.161149076596335,
0.173369264417413,0.185313943124287,0.204539234926209,0.259607450626017,
0.34172790800698,0.375399223369378,0.376207524066527,0.376606503276033,
0.376798210729843,0.377691036208974,0.378363680416897,0.378860988397354,
0.379223179482051,0.379483920481797,0.379669996768885,0.37980193825668,
0.379895059126323,0.380302261087459,0.380662631698573,0.380980207630575,
0.381258937597082,0.387313997030125,0.392872299510832,0.399118600020562,
0.410621479147785,0.456960892354912,0.509380295962348,0.530567103295414,
0.542989346639929,0.552108935940903,0.56064813004894,0.569007847514817,
0.582398708581225,0.616963229120582,0.717998183839658,0.751536051927716,
0.770791678898915,0.77668925813288,0.780442588016263,0.783973071226936,
0.788616501153669,0.797174617955982,0.891962341029584,1.0218154441692,1.08265661945942,
1.09647157413381,1.10339455105421,1.1099420946198,1.11703205849066,1.12950987540703,
1.16821773172323,1.24014884072464,1.39726406724103,1.50889892192508,1.54509922288968,
1.54986837336914,1.55228702605543,1.55401808601761,1.55584309579,1.55890948915915,
1.56695922950712,1.68786179283197,1.8155517854012,1.90447107743777,1.9384382540311,
1.94370745644524,1.94643333169015,1.94863870114513,1.95083409042105,1.95479288025936,
1.96693738249264,2.14384450909385,2.2647004462708,2.35787451621018,2.36261987767432,
2.36442883202812,2.36567080008746,2.36688389733508,2.36834078830516,2.37195209780184,
2.40893574495947,2.50760030700269,2.61791378444164,2.68714104507969,2.73436756649004,
2.75904775885284,2.76347290999952,2.7658333594947,2.76759118112479,2.76951035739376,
2.77290287454548,2.78284204267499,2.93428352038161,3.15314642015992,3.16594785894354,
3.16831220917512,3.16979829194121,3.1709589357742,3.17224105427437,3.1743351734981,
3.18159703193165,3.22777277277377,3.27518482878292,3.40016820841547,3.57482013283156,
3.58631013108575,3.59004180820283,3.59237471060776,3.59448423928055,3.59714354444902,
3.60248222439886,3.641600060276,3.72672183690177,3.78819849223625,3.9732529671625,
3.98588269042508,3.98971065649067,3.9919993061417,3.99383274252603,3.99629987998103,
4.00094223777758,4.02756199341562,4.08886049692501,4.28939453883896,4.32185947805448,
4.33115974765688,4.33561232274636,4.33637642441593,4.4227666423236,4.4317996201652,
4.43967724692138,4.4452577148184,4.45111407188919,4.45878527367052,4.47531496023699,
4.57237173510791,4.7365848690502,4.74832440510131,4.75236543754039,4.75525761318156,
4.75800511292837,4.7618537875373,4.76964941969628,4.84909791600552,5.02473203876403,
5.05494477875511,5.06639780060826,5.07329823327692,5.08067591766276,5.09059779513613,
5.11342016595376,5.32851101505927,5.45982460552235,5.46964741486818,5.50510763749313,
5.51009630533926,5.51244372636196,5.51427262820719,5.51625843231705,5.51942774689967,
5.52977694117077,5.58817805985445,5.86891849949769),.UNSPECIFIED.);
#3527=B_SPLINE_CURVE_WITH_KNOTS('',3,(#217531,#217532,#217533,#217534,#217535,
#217536,#217537,#217538,#217539,#217540,#217541,#217542,#217543,#217544,
#217545,#217546,#217547,#217548),.UNSPECIFIED.,.F.,.F.,(4,2,2,2,2,2,2,2,
4),(7.4068340133238,8.24175092521866,9.07666783711352,9.91158474900838,
10.7465016609032,11.5814185727981,12.416335484693,13.2512523965878,13.6900193205034),
 .UNSPECIFIED.);
#3528=B_SPLINE_CURVE_WITH_KNOTS('',3,(#217550,#217551,#217552,#217553,#217554,
#217555,#217556,#217557,#217558,#217559,#217560,#217561),.UNSPECIFIED.,
 .F.,.F.,(4,1,1,1,1,1,1,1,1,4),(13.6900193205034,13.9823563020706,14.9810960379328,
15.4804659058639,15.9798357737949,16.9785755096571,17.9773152455193,18.9760549813814,
19.4754248493125,19.9732045334931),.UNSPECIFIED.);
#3529=B_SPLINE_CURVE_WITH_KNOTS('',3,(#217563,#217564,#217565,#217566,#217567,
#217568,#217569,#217570,#217571,#217572,#217573,#217574,#217575,#217576,
#217577,#217578,#217579,#217580,#217581,#217582,#217583,#217584,#217585,
#217586,#217587,#217588,#217589,#217590,#217591,#217592,#217593,#217594,
#217595,#217596,#217597,#217598,#217599,#217600,#217601,#217602,#217603,
#217604,#217605,#217606,#217607,#217608,#217609,#217610,#217611,#217612,
#217613,#217614,#217615,#217616,#217617,#217618,#217619,#217620,#217621,
#217622,#217623,#217624,#217625,#217626,#217627,#217628,#217629,#217630,
#217631,#217632,#217633,#217634,#217635,#217636,#217637,#217638,#217639,
#217640,#217641,#217642,#217643,#217644,#217645,#217646,#217647,#217648,
#217649,#217650,#217651,#217652,#217653,#217654,#217655,#217656,#217657,
#217658,#217659,#217660,#217661,#217662,#217663,#217664,#217665,#217666,
#217667,#217668,#217669,#217670,#217671,#217672,#217673,#217674,#217675,
#217676,#217677,#217678,#217679,#217680,#217681,#217682,#217683,#217684,
#217685,#217686,#217687,#217688,#217689,#217690,#217691,#217692,#217693,
#217694,#217695,#217696,#217697,#217698,#217699,#217700,#217701,#217702,
#217703,#217704,#217705,#217706,#217707,#217708,#217709,#217710,#217711,
#217712,#217713,#217714,#217715,#217716,#217717,#217718,#217719,#217720,
#217721,#217722,#217723,#217724,#217725,#217726,#217727,#217728,#217729,
#217730,#217731,#217732,#217733,#217734,#217735,#217736,#217737,#217738,
#217739,#217740,#217741,#217742,#217743,#217744,#217745,#217746,#217747,
#217748,#217749,#217750,#217751,#217752,#217753,#217754,#217755,#217756,
#217757,#217758,#217759,#217760,#217761,#217762,#217763,#217764,#217765,
#217766,#217767,#217768,#217769,#217770,#217771,#217772,#217773,#217774,
#217775,#217776,#217777,#217778,#217779,#217780,#217781,#217782,#217783,
#217784,#217785,#217786,#217787,#217788,#217789,#217790,#217791,#217792,
#217793,#217794,#217795,#217796,#217797,#217798,#217799,#217800,#217801,
#217802,#217803,#217804,#217805,#217806,#217807,#217808,#217809,#217810,
#217811,#217812,#217813,#217814,#217815,#217816,#217817,#217818,#217819,
#217820,#217821,#217822,#217823,#217824,#217825,#217826,#217827,#217828,
#217829,#217830,#217831,#217832,#217833,#217834,#217835,#217836,#217837,
#217838,#217839,#217840,#217841,#217842,#217843,#217844,#217845,#217846,
#217847,#217848,#217849,#217850,#217851,#217852,#217853,#217854,#217855,
#217856,#217857,#217858,#217859,#217860,#217861,#217862,#217863,#217864,
#217865,#217866,#217867,#217868,#217869,#217870,#217871,#217872,#217873,
#217874,#217875,#217876,#217877,#217878,#217879,#217880,#217881,#217882,
#217883,#217884,#217885,#217886,#217887,#217888,#217889,#217890,#217891,
#217892,#217893,#217894,#217895,#217896,#217897,#217898,#217899,#217900,
#217901,#217902,#217903,#217904,#217905,#217906,#217907,#217908,#217909,
#217910,#217911,#217912,#217913,#217914,#217915,#217916,#217917,#217918,
#217919,#217920,#217921,#217922,#217923,#217924,#217925,#217926,#217927,
#217928,#217929,#217930,#217931,#217932,#217933,#217934,#217935,#217936,
#217937,#217938,#217939,#217940,#217941,#217942,#217943,#217944,#217945,
#217946,#217947,#217948,#217949,#217950,#217951,#217952,#217953,#217954,
#217955,#217956,#217957,#217958,#217959,#217960,#217961,#217962,#217963,
#217964,#217965,#217966,#217967,#217968,#217969,#217970,#217971,#217972,
#217973,#217974,#217975,#217976,#217977,#217978,#217979,#217980,#217981,
#217982,#217983,#217984,#217985,#217986,#217987,#217988,#217989,#217990,
#217991,#217992,#217993,#217994,#217995,#217996,#217997,#217998,#217999,
#218000,#218001,#218002,#218003,#218004,#218005,#218006,#218007,#218008,
#218009,#218010,#218011,#218012,#218013,#218014,#218015,#218016,#218017,
#218018,#218019,#218020,#218021,#218022,#218023,#218024,#218025,#218026,
#218027,#218028,#218029,#218030,#218031,#218032,#218033,#218034,#218035,
#218036,#218037,#218038,#218039,#218040,#218041,#218042,#218043,#218044,
#218045,#218046,#218047,#218048,#218049,#218050,#218051,#218052,#218053,
#218054,#218055,#218056,#218057,#218058,#218059,#218060,#218061,#218062,
#218063,#218064,#218065,#218066,#218067,#218068,#218069,#218070,#218071,
#218072,#218073,#218074,#218075,#218076,#218077,#218078,#218079,#218080,
#218081,#218082,#218083,#218084,#218085,#218086,#218087,#218088,#218089,
#218090,#218091,#218092,#218093,#218094,#218095,#218096,#218097,#218098,
#218099,#218100,#218101,#218102,#218103,#218104,#218105,#218106,#218107,
#218108,#218109,#218110,#218111,#218112,#218113,#218114,#218115,#218116,
#218117,#218118,#218119,#218120),.UNSPECIFIED.,.F.,.F.,(4,2,2,2,2,2,2,2,
2,2,2,2,2,2,2,2,2,2,2,2,2,2,2,2,2,2,2,2,2,2,2,2,2,2,2,2,2,2,2,2,2,2,2,2,
2,2,2,2,2,2,2,2,2,2,2,2,2,2,2,2,2,2,2,2,2,2,2,2,2,2,2,2,2,2,2,2,2,2,2,2,
2,2,2,2,2,2,2,2,2,2,2,2,2,2,2,2,2,2,2,2,2,2,2,2,2,2,2,2,2,2,2,2,2,2,2,2,
2,2,2,2,2,2,2,2,2,2,2,2,2,2,2,2,2,2,2,2,2,2,2,2,2,2,2,2,2,2,2,2,2,2,2,2,
2,2,2,2,2,2,2,2,2,2,2,2,2,2,2,2,2,2,2,2,2,2,2,2,2,2,2,2,2,2,2,2,2,2,2,2,
2,2,2,2,2,2,2,2,2,2,2,2,2,2,2,2,2,2,2,2,2,2,2,2,2,2,2,2,2,2,2,2,2,2,2,2,
2,2,2,2,2,2,2,2,2,2,2,2,2,2,2,2,2,2,2,2,2,2,2,2,2,2,2,2,2,2,2,2,2,2,2,2,
2,2,2,2,2,2,2,2,2,2,2,2,2,2,2,2,2,2,4),(0.00169250605834049,0.00408492138346118,
0.00757146341587593,0.0104864642879784,0.0134044379630337,0.0183187848536681,
0.0314251930669086,0.170038641662356,0.288246616778126,0.303248212676448,
0.312682850283399,0.319857774097023,0.327213302003405,0.334137907385634,
0.343805750427874,0.369913030709805,0.562493239480834,0.640272395212907,
0.674141160188036,0.732738320347233,0.751326615247076,0.758775020538961,
0.762603997553388,0.765004968465602,0.767247262050247,0.768895084349338,
0.77067322912686,0.773229532147553,0.780358226058807,0.865845819473271,
0.896627539123426,0.978030374063007,1.00338420047898,1.01849216416434,1.0626314665659,
1.13137426030897,1.17561627716773,1.18130973484367,1.18415594285482,1.1861996184324,
1.18835985464576,1.19200138044488,1.20163274021882,1.34763609525156,1.4273558872268,
1.48825106811496,1.54725716368977,1.56915114537342,1.58430708370833,1.59053896738361,
1.59378562833104,1.5958241951731,1.59773785231902,1.59913069596616,1.6006205429543,
1.60274150729589,1.60852089541209,1.70882652927395,1.84704032343686,1.89224868409987,
1.94901072472249,1.95825172610291,1.96209714212466,1.96600399601449,1.96959157879376,
1.97443528270748,1.98644363037358,2.10215848865768,2.27256193946883,2.33179304626633,
2.33819999325205,2.34160411413638,2.34379967855223,2.34551519579621,2.34711574192009,
2.34879671462028,2.351138022787,2.35722339457166,2.4346307920901,2.59667988280613,
2.65653767337051,2.70613894044412,2.73315286120499,2.73789419156163,2.74041154798166,
2.74228120926014,2.74461205927209,2.74850354985693,2.76127656976108,2.94347847968625,
3.06926256755972,3.12101512251245,3.14792657802399,3.16128693409591,3.16378260552575,
3.16512570652083,3.16622886772128,3.16735729484487,3.16947526759535,3.17676381392457,
3.28659948840381,3.44275564633209,3.55810092319401,3.56439981975234,3.5671565354901,
3.56918369910067,3.57105386631777,3.57358831673009,3.5798093370713,3.6434540856021,
3.708218896661,3.85523515638434,3.93931329880087,3.95883825116561,3.96161595928014,
3.96306038870735,3.96412093688517,3.96526408580681,3.96724603487886,3.97280923666566,
4.06468950815282,4.27806378875624,4.34417272045854,4.37505049827141,4.38012302218407,
4.38277775757291,4.38494101065096,4.38710742101876,4.3910498836419,4.40340717404014,
4.59468766717309,4.70527731609155,4.76821509348387,4.77573909733512,4.78156659470898,
4.78426380338545,4.78630902555112,4.78824231565617,4.79093666606993,4.79643627835568,
4.8563966320353,4.97943746243127,5.20349855664505,5.22591289852476,5.23408251376757,
5.23986005413012,5.24591639475465,5.25384118221521,5.27089992227968,5.41277846909467,
5.46850400980107,5.53603061013568,5.54345542429789,5.5471741372855,5.55021127681729,
5.55371510377716,5.55981632388456,5.58614692827814,5.70555379263311,5.80627537059302,
5.84329942029978,5.85570857535668,5.86278843508173,5.86934832450355,5.87832378549833,
5.89600420093851,5.99798307266371,6.13762691073564,6.25372136397141,6.25537273886839,
6.26069619722776,6.26911253365382,6.29910436423473,6.30382632800519,6.30618796733963,
6.30802320036033,6.31004176844181,6.31332062783319,6.3245485906103,6.39171605715386,
6.47045998545857,6.6485050995784,6.71307142051247,6.71933933256134,6.72237710036844,
6.72453900608407,6.72676399898738,6.72964425496292,6.7328019897907,6.73797991129445,
6.74830442920889,6.85302303013423,6.97746713791533,7.12353440073216,7.13308325901777,
7.13597938253975,7.13753729060472,7.13891874512614,7.14070981831484,7.1438741669414,
7.15791391799086,7.36512096624578,7.48566039335019,7.49679831909093,7.5019343165621,
7.50579404884994,7.50986757345893,7.51604961002203,7.53341279020593,7.71048193025695,
7.82771867433625,7.8742635524245,7.88163892036583,7.88417885528428,7.88591447386092,
7.88750001477075,7.88962301904988,7.89358556669983,7.91531693470139,7.95696201534709,
7.99687150909349,8.02403016709019,8.04779918487014,8.17876796890253,8.26919365609497,
8.27617767497506,8.27890618167616,8.28087904052705,8.28293749679372,8.2856483366552,
8.28863594887332,8.29359339851161,8.30360728892195,8.32931143734312,8.42580297939014,
8.65738212694162,8.66455037223573,8.66687914679954,8.69954650177493,8.70269062899539,
8.70420579870868,8.7052803061511,8.7062928117296,8.70769776547701,8.7105468061881,
8.73489968386801,8.81210712490254,8.87419522441539,8.96201943344826,9.01642874047259,
9.09713008757062,9.10374547253827,9.1065790505427,9.10859790483142,9.11046947939199,
9.11329741265741,9.12000181378065,9.23548856557561,9.48720757802478,9.49930824374196,
9.50164941912221,9.50314039560235,9.50431750755878,9.50563092405126,9.50780632775749,
9.51565405453653,9.56766377902952,9.609289670219,9.88657725912831,9.89905812311192,
9.91660666896944,9.9206670629974,9.9233367074833,9.92537035669844,9.92740178011608,
9.92978761312891,9.93321467079975,9.942862547507,9.95915312357805),
 .UNSPECIFIED.);
#3530=B_SPLINE_CURVE_WITH_KNOTS('',3,(#218122,#218123,#218124,#218125,#218126,
#218127,#218128,#218129,#218130,#218131,#218132,#218133,#218134,#218135,
#218136,#218137,#218138,#218139,#218140,#218141,#218142,#218143,#218144,
#218145,#218146,#218147,#218148,#218149,#218150,#218151,#218152,#218153,
#218154,#218155,#218156,#218157,#218158,#218159,#218160,#218161,#218162,
#218163,#218164,#218165,#218166,#218167,#218168,#218169,#218170,#218171,
#218172,#218173,#218174,#218175,#218176,#218177,#218178,#218179,#218180,
#218181,#218182,#218183,#218184,#218185,#218186,#218187,#218188,#218189,
#218190,#218191,#218192,#218193,#218194,#218195,#218196,#218197,#218198,
#218199,#218200,#218201,#218202,#218203,#218204,#218205,#218206,#218207,
#218208,#218209,#218210,#218211,#218212,#218213,#218214,#218215,#218216,
#218217,#218218,#218219,#218220,#218221,#218222,#218223,#218224,#218225,
#218226,#218227,#218228,#218229,#218230,#218231,#218232,#218233,#218234,
#218235,#218236,#218237,#218238,#218239,#218240,#218241,#218242,#218243,
#218244,#218245,#218246,#218247,#218248,#218249,#218250,#218251,#218252,
#218253,#218254,#218255,#218256,#218257,#218258,#218259,#218260,#218261,
#218262,#218263,#218264,#218265,#218266,#218267,#218268,#218269,#218270,
#218271,#218272,#218273,#218274,#218275,#218276,#218277,#218278,#218279,
#218280,#218281,#218282,#218283,#218284,#218285,#218286,#218287,#218288,
#218289,#218290,#218291,#218292,#218293,#218294,#218295,#218296,#218297,
#218298,#218299,#218300,#218301,#218302,#218303,#218304,#218305,#218306,
#218307,#218308,#218309,#218310,#218311,#218312,#218313,#218314,#218315,
#218316,#218317,#218318,#218319,#218320,#218321,#218322,#218323,#218324,
#218325,#218326,#218327,#218328,#218329,#218330,#218331,#218332,#218333,
#218334,#218335,#218336,#218337,#218338,#218339,#218340,#218341,#218342,
#218343,#218344,#218345,#218346,#218347,#218348,#218349,#218350,#218351,
#218352,#218353,#218354,#218355,#218356,#218357,#218358,#218359,#218360,
#218361,#218362,#218363,#218364,#218365,#218366,#218367,#218368,#218369,
#218370,#218371,#218372,#218373,#218374,#218375,#218376,#218377,#218378,
#218379,#218380,#218381,#218382,#218383,#218384,#218385,#218386,#218387,
#218388,#218389,#218390,#218391,#218392,#218393,#218394,#218395,#218396,
#218397,#218398,#218399,#218400,#218401,#218402,#218403,#218404,#218405,
#218406,#218407,#218408,#218409,#218410,#218411,#218412,#218413,#218414,
#218415,#218416,#218417,#218418,#218419,#218420,#218421,#218422,#218423,
#218424,#218425,#218426,#218427,#218428,#218429,#218430,#218431,#218432,
#218433,#218434,#218435,#218436,#218437,#218438,#218439,#218440,#218441,
#218442,#218443,#218444,#218445,#218446,#218447,#218448,#218449,#218450,
#218451,#218452,#218453,#218454,#218455,#218456,#218457,#218458,#218459,
#218460,#218461,#218462,#218463,#218464,#218465,#218466,#218467,#218468,
#218469,#218470,#218471,#218472,#218473,#218474,#218475,#218476,#218477,
#218478,#218479,#218480,#218481,#218482,#218483,#218484,#218485,#218486,
#218487,#218488,#218489,#218490,#218491,#218492,#218493,#218494,#218495,
#218496,#218497,#218498,#218499,#218500,#218501,#218502,#218503,#218504,
#218505,#218506,#218507,#218508,#218509,#218510,#218511,#218512,#218513,
#218514,#218515,#218516,#218517,#218518,#218519,#218520,#218521,#218522,
#218523,#218524,#218525,#218526,#218527,#218528,#218529,#218530,#218531,
#218532,#218533,#218534,#218535,#218536,#218537,#218538,#218539,#218540,
#218541,#218542,#218543,#218544,#218545,#218546,#218547,#218548,#218549,
#218550,#218551,#218552,#218553,#218554,#218555,#218556,#218557,#218558,
#218559,#218560,#218561,#218562,#218563,#218564,#218565,#218566,#218567,
#218568,#218569,#218570,#218571,#218572,#218573,#218574,#218575,#218576,
#218577,#218578,#218579,#218580,#218581,#218582,#218583,#218584,#218585,
#218586,#218587,#218588,#218589,#218590,#218591,#218592,#218593,#218594,
#218595,#218596,#218597,#218598,#218599,#218600,#218601,#218602,#218603,
#218604,#218605,#218606,#218607,#218608,#218609,#218610,#218611,#218612,
#218613,#218614,#218615,#218616,#218617,#218618,#218619,#218620,#218621,
#218622,#218623,#218624,#218625,#218626,#218627,#218628,#218629,#218630,
#218631,#218632,#218633,#218634,#218635,#218636,#218637,#218638,#218639,
#218640,#218641,#218642,#218643,#218644,#218645,#218646,#218647,#218648,
#218649,#218650,#218651,#218652,#218653,#218654,#218655,#218656,#218657,
#218658,#218659,#218660,#218661),.UNSPECIFIED.,.F.,.F.,(4,2,2,2,2,2,2,2,
2,2,2,2,2,2,2,2,2,2,2,2,2,2,2,2,2,2,2,2,2,2,2,2,2,2,2,2,2,2,2,2,2,2,2,2,
2,2,2,2,2,2,2,2,2,2,2,2,2,2,2,2,2,2,2,2,2,2,2,2,2,2,2,2,2,2,2,2,2,2,2,2,
2,2,2,2,2,2,2,2,2,2,2,2,2,2,2,2,2,2,2,2,2,2,2,2,2,2,2,2,2,2,2,2,2,2,2,2,
2,2,2,2,2,2,2,2,2,2,2,2,2,2,2,2,2,2,2,2,2,2,2,2,2,2,2,2,2,2,2,2,2,2,2,2,
2,2,2,2,2,2,2,2,2,2,2,2,2,2,2,2,2,2,2,2,2,2,2,2,2,2,2,2,2,2,2,2,2,2,2,2,
2,2,2,2,2,2,2,2,2,2,2,2,2,2,2,2,2,2,2,2,2,2,2,2,2,2,2,2,2,2,2,2,2,2,2,2,
2,2,2,2,2,2,2,2,2,2,2,2,2,2,2,2,2,2,2,2,2,2,2,2,2,2,2,2,2,2,2,2,2,2,2,2,
2,2,2,2,2,2,2,2,2,4),(0.00342832916621827,0.283631051066085,0.360738473639449,
0.366797125569613,0.369537630895681,0.371589629870451,0.373510316724189,
0.376157013520932,0.381465250250319,0.432135927861035,0.473970987694638,
0.490486145040209,0.584839881414579,0.691087837363955,0.801282838340406,
0.815459201201547,0.822813041199435,0.828809321060278,0.835736835233664,
0.84735815397142,0.892187224478493,1.04746644909393,1.09924798175357,1.12420104845123,
1.12976531983696,1.13313236569669,1.1361899876218,1.14012329694035,1.14645018770221,
1.1816016496431,1.31811911670678,1.4118220678103,1.43413700425487,1.4439979941693,
1.4513614006176,1.45827482030023,1.46789692429219,1.49358380062198,1.65834149976674,
1.77082316864897,1.87340462439512,1.88203448487255,1.88825472558852,1.89086137921176,
1.89273639802437,1.89443731040081,1.89669984513036,1.90216842222589,1.97189398654687,
2.17230806268736,2.28620335969344,2.29696219672158,2.30229945725151,2.30552354574051,
2.30844927291627,2.31068166452595,2.31282721003923,2.31580423992278,2.32347794845796,
2.42800880184614,2.51245035823726,2.64226377992633,2.70849358663467,2.71831979341818,
2.72112254116228,2.72283294847891,2.72437793238283,2.7263517871531,2.73025071001662,
2.7534621401755,2.89089511894278,2.99469886179372,3.04677265934644,3.0769198821813,
3.08436300465291,3.08871596073143,3.09214832312508,3.09658795674793,3.10446383611405,
3.13394951671107,3.2380065296938,3.39171787465741,3.44146890328936,3.4641601490627,
3.4681679228941,3.47030058874123,3.4718864342716,3.47386674964624,3.47718018814749,
3.4881085630761,3.64600810064209,3.69452879427424,3.79563316629203,3.84355904471498,
3.85905433570377,3.86304739246538,3.86540110551595,3.86747546329156,3.87005689151794,
3.8740255176707,3.89179165012771,4.17260635888201,4.23218988615659,4.27991414095278,
4.28723786676528,4.28929305289678,4.29053916104202,4.29165932937067,4.29308462615784,
4.29537028085317,4.30735870013929,4.50781327429289,4.67175734946823,4.68740606904522,
4.69130256378998,4.69357417159628,4.69556088189839,4.69801344246082,4.70174769521128,
4.7179349414876,4.98462416316624,4.98640371520551,4.98797115128335,4.98927285779437,
4.99025736250648,4.99091502581435,4.99130249642403,4.99150992298686,4.99161467056005,
4.99166594882272,5.00290355910937,5.08189136805791,5.08666560298956,5.08832601182001,
5.08947459829621,5.09053399564449,5.09196758474482,5.09469026088453,5.11072116907735,
5.14183346642671,5.19886310977924,5.36794208954646,5.40082839601826,5.42890278799879,
5.49828699802399,5.50506274644153,5.50782447757898,5.50986291418035,5.5120730653388,
5.51507970493303,5.52195515677048,5.61413902983783,5.84797672258699,5.90221721621993,
5.90802918384602,5.91069515282231,5.91274371284757,5.91493965746252,5.91838501415116,
5.92916171878568,5.9966346150914,6.13243771161565,6.33082436739837,6.35273173101311,
6.36083386186514,6.3665956032699,6.37266410510324,6.38065277495144,6.39803990893885,
6.41081100567521,6.43331815879127,6.51728848904986,6.65578103514687,6.66806336491171,
6.67216064998922,6.67507810398222,6.67784133499532,6.6816988442517,6.68946370183121,
6.76387410146639,6.91303364304987,6.92260088605829,6.96836281161855,6.98178444596241,
6.98987768752092,6.996443709225,7.00544207032008,7.0232210543294,7.124062306916,
7.26183738034302,7.37628984888066,7.41969381060556,7.42938938532284,7.43249542089468,
7.43427866588673,7.43605644464604,7.43831188856129,7.4426932598588,7.44820461570782,
7.48862257626653,7.54733320482364,7.73424366049973,7.77865576003307,7.84073978613646,
7.84763438440298,7.85040589420224,7.85270962487712,7.85506494955559,7.85849038164818,
7.86745379035613,7.98415770133822,8.03869460398933,8.21843992788006,8.25844297081749,
8.26237820602357,8.26436871234709,8.26582412541662,8.26730005760225,8.26931006642183,
8.27355776354944,8.27917321500773,8.29251559902873,8.33646720731166,8.43294670762758,
8.47179719311355,8.61321292700364,8.62475967353734,8.62942923604514,8.63333113315084,
8.63734518131892,8.64323975335657,8.65873142482336,8.72792152962356,8.76295041431008,
8.78815340392706,8.95887154948812,9.00540038507769,9.01014231011597,9.01247728302127,
9.01415734390665,9.01584514546417,9.01810087529382,9.02271114402907,9.02863198887763,
9.04189400673035,9.07602654671143,9.12113227238289,9.33054316393754,9.39829674171379,
9.40480874191826,9.40745729289208,9.40941006394441,9.41152525907372,9.41439910568962,
9.4209547454346,9.53727160818928,9.62474678035204,9.66328134892579,9.68298682188908,
9.70441564373435,9.80395315570567,9.82822705663885,9.83139999642303,9.83288808372516,
9.83402107797487,9.83522519082486,9.83644837802485,9.8382170637605,9.84130640182385,
9.96378201833553),.UNSPECIFIED.);
#3531=B_SPLINE_CURVE_WITH_KNOTS('',3,(#218663,#218664,#218665,#218666,#218667,
#218668,#218669,#218670,#218671,#218672,#218673,#218674,#218675,#218676,
#218677,#218678,#218679,#218680,#218681,#218682,#218683,#218684,#218685,
#218686,#218687,#218688,#218689,#218690,#218691,#218692,#218693,#218694,
#218695,#218696,#218697,#218698,#218699,#218700,#218701,#218702,#218703,
#218704,#218705,#218706,#218707,#218708,#218709,#218710,#218711,#218712,
#218713,#218714,#218715,#218716,#218717,#218718,#218719,#218720,#218721,
#218722,#218723,#218724,#218725,#218726,#218727,#218728,#218729,#218730,
#218731,#218732,#218733,#218734,#218735,#218736,#218737,#218738,#218739,
#218740,#218741,#218742,#218743,#218744,#218745,#218746,#218747,#218748,
#218749,#218750,#218751,#218752,#218753,#218754,#218755,#218756,#218757,
#218758,#218759,#218760,#218761,#218762,#218763,#218764,#218765,#218766,
#218767,#218768,#218769,#218770,#218771,#218772,#218773,#218774,#218775,
#218776,#218777,#218778,#218779,#218780,#218781,#218782,#218783,#218784,
#218785,#218786,#218787,#218788,#218789,#218790,#218791,#218792,#218793,
#218794,#218795,#218796,#218797,#218798,#218799,#218800,#218801,#218802,
#218803,#218804,#218805,#218806,#218807,#218808,#218809,#218810,#218811,
#218812,#218813,#218814,#218815,#218816,#218817,#218818,#218819,#218820,
#218821,#218822,#218823,#218824,#218825,#218826,#218827,#218828,#218829,
#218830,#218831,#218832,#218833,#218834,#218835,#218836,#218837,#218838,
#218839,#218840,#218841,#218842,#218843,#218844,#218845,#218846,#218847,
#218848,#218849,#218850,#218851,#218852,#218853,#218854,#218855,#218856,
#218857,#218858,#218859,#218860,#218861,#218862,#218863,#218864,#218865,
#218866,#218867,#218868,#218869,#218870,#218871,#218872,#218873,#218874,
#218875,#218876,#218877,#218878,#218879,#218880,#218881,#218882,#218883,
#218884,#218885,#218886,#218887,#218888,#218889,#218890,#218891,#218892,
#218893,#218894,#218895,#218896,#218897,#218898,#218899,#218900,#218901,
#218902,#218903,#218904,#218905,#218906,#218907,#218908,#218909,#218910,
#218911,#218912,#218913,#218914,#218915,#218916,#218917,#218918,#218919,
#218920,#218921,#218922,#218923,#218924,#218925,#218926,#218927,#218928,
#218929,#218930,#218931,#218932,#218933,#218934,#218935,#218936,#218937,
#218938,#218939,#218940,#218941,#218942,#218943,#218944,#218945,#218946,
#218947,#218948,#218949,#218950,#218951,#218952,#218953,#218954,#218955,
#218956,#218957,#218958,#218959,#218960,#218961,#218962,#218963,#218964,
#218965,#218966,#218967,#218968,#218969,#218970,#218971,#218972,#218973,
#218974,#218975,#218976,#218977,#218978,#218979,#218980,#218981,#218982,
#218983,#218984,#218985,#218986,#218987,#218988,#218989,#218990,#218991,
#218992,#218993,#218994,#218995,#218996,#218997,#218998,#218999,#219000,
#219001,#219002,#219003,#219004,#219005,#219006,#219007,#219008,#219009,
#219010,#219011,#219012,#219013,#219014,#219015,#219016,#219017,#219018,
#219019,#219020,#219021,#219022,#219023,#219024,#219025,#219026,#219027,
#219028,#219029,#219030,#219031,#219032,#219033,#219034,#219035,#219036,
#219037,#219038,#219039,#219040,#219041,#219042,#219043,#219044,#219045,
#219046,#219047,#219048,#219049,#219050,#219051,#219052,#219053,#219054,
#219055,#219056,#219057,#219058,#219059,#219060,#219061,#219062,#219063,
#219064,#219065,#219066,#219067,#219068,#219069,#219070,#219071,#219072,
#219073,#219074,#219075,#219076,#219077,#219078,#219079,#219080,#219081,
#219082,#219083,#219084,#219085,#219086,#219087,#219088,#219089,#219090,
#219091,#219092,#219093,#219094,#219095,#219096,#219097,#219098,#219099,
#219100,#219101,#219102,#219103,#219104,#219105,#219106,#219107,#219108,
#219109,#219110,#219111,#219112,#219113,#219114,#219115,#219116,#219117,
#219118,#219119,#219120,#219121,#219122,#219123,#219124,#219125,#219126,
#219127,#219128,#219129,#219130,#219131,#219132,#219133,#219134,#219135,
#219136,#219137,#219138,#219139,#219140,#219141,#219142,#219143,#219144,
#219145,#219146,#219147,#219148,#219149,#219150,#219151,#219152,#219153,
#219154,#219155,#219156,#219157,#219158,#219159,#219160,#219161,#219162,
#219163,#219164,#219165,#219166,#219167,#219168,#219169,#219170,#219171,
#219172,#219173,#219174,#219175,#219176,#219177,#219178,#219179,#219180,
#219181,#219182,#219183,#219184,#219185,#219186,#219187,#219188,#219189,
#219190,#219191,#219192),.UNSPECIFIED.,.F.,.F.,(4,2,2,2,2,2,2,2,2,2,2,2,
2,2,2,2,2,2,2,2,2,2,2,2,2,2,2,2,2,2,2,2,2,2,2,2,2,2,2,2,2,2,2,2,2,2,2,2,
2,2,2,2,2,2,2,2,2,2,2,2,2,2,2,2,2,2,2,2,2,2,2,2,2,2,2,2,2,2,2,2,2,2,2,2,
2,2,2,2,2,2,2,2,2,2,2,2,2,2,2,2,2,2,2,2,2,2,2,2,2,2,2,2,2,2,2,2,2,2,2,2,
2,2,2,2,2,2,2,2,2,2,2,2,2,2,2,2,2,2,2,2,2,2,2,2,2,2,2,2,2,2,2,2,2,2,2,2,
2,2,2,2,2,2,2,2,2,2,2,2,2,2,2,2,2,2,2,2,2,2,2,2,2,2,2,2,2,2,2,2,2,2,2,2,
2,2,2,2,2,2,2,2,2,2,2,2,2,2,2,2,2,2,2,2,2,2,2,2,2,2,2,2,2,2,2,2,2,2,2,2,
2,2,2,2,2,2,2,2,2,2,2,2,2,2,2,2,2,2,2,2,2,2,2,2,2,2,2,2,2,2,2,2,2,2,2,2,
4),(0.00135678833193775,0.0849112974682599,0.250362026703773,0.267416405184458,
0.271424401168757,0.273720086164047,0.275503948011275,0.277837536064323,
0.281905370935197,0.297768962655745,0.548144917578907,0.590757060622519,
0.658429813576954,0.665967591826151,0.66752938957349,0.668705623442331,
0.669901750382023,0.671006917428027,0.67250706999984,0.675442522770863,
0.698087591735058,0.775060481717971,0.819621842294523,0.856102387606388,
0.930047452729326,1.07845551366674,1.08501040120155,1.08795794536467,1.09015716006998,
1.09220892133065,1.09502499788795,1.10211996924262,1.18681820743318,1.35770560184273,
1.42578010787449,1.45604870462433,1.47364666932529,1.481262367681,1.48531240554683,
1.48878495046406,1.4909669948675,1.49300388787056,1.49564254820917,1.50116619853498,
1.54010957802893,1.73066308911003,1.86619755748685,1.92232050471461,1.93615723713239,
1.94344110930975,1.9488519562787,1.95562686122702,1.96707702717865,2.00755677830743,
2.12701218859459,2.2390115302356,2.24811954978529,2.25211398087694,2.25501391663153,
2.25818456154083,2.26303368368701,2.27634795535934,2.38380555866663,2.50302811984098,
2.53258948623283,2.55468037168967,2.56450204876064,2.57185935669029,2.57878402114594,
2.58844931832276,2.61452482236272,2.80178771241284,2.89190820002709,3.00075531870213,
3.00583445434993,3.00985558001541,3.01203502086102,3.01385721669238,3.01596298371126,
3.01953765921016,3.0324932441244,3.29615033944627,3.41815386923108,3.42570700543658,
3.42890210481325,3.4312106978574,3.43331237939667,3.43611876500823,3.44295023998168,
3.50608673802949,3.73789791419254,3.78531174673087,3.81929929419335,3.83825218452709,
3.84167395243639,3.84352105606655,3.84490650921318,3.84642901445017,3.84914653949791,
3.8573006734907,3.86514335002146,3.87223044585572,3.95851715611277,4.05917177086544,
4.19075736560386,4.20265954231791,4.20791191821989,4.2118008342834,4.21541290355264,
4.22035282655244,4.23261840055454,4.39093366564085,4.51525006242259,4.56320312513134,
4.58530239462114,4.5892810631282,4.59140749903535,4.59314690995691,4.59518631559077,
4.59867162217512,4.61152270672273,4.85716944564892,4.91272030567231,4.97082441324231,
4.98142451881819,4.98490309334031,4.98691779298153,4.98879252427598,4.99135479671747,
4.99630940899933,5.02823687628295,5.09990645506393,5.31358328234852,5.35016422589624,
5.36360158692659,5.37206007109417,5.40565409288447,5.40912680533124,5.41053384363057,
5.41158004344229,5.41272172306244,5.41429355756304,5.4180601653288,5.49590390544152,
5.67890047502349,5.74268343905978,5.80407864277238,5.81024455641712,5.81276924339384,
5.81463686185594,5.81666576885071,5.81943288069444,5.82579053885241,5.93389233704926,
6.11491083760101,6.20126556599649,6.20651059715833,6.2084256932473,6.2095552797128,
6.2106196138646,6.21209493525669,6.21501928685218,6.23635714518638,6.31773781865796,
6.45834865378636,6.61360636289424,6.6236797545484,6.6273079130548,6.62941124156517,
6.63136978096582,6.63404872322197,6.63923623375321,6.67294704222562,6.7502242588908,
6.9476979251212,7.02137505619447,7.02682530116526,7.02951134725714,7.03144230396704,
7.0332830136525,7.03586981784371,7.04067747924981,7.04703829465804,7.10063066007351,
7.20815699909149,7.34182013975535,7.35142628432431,7.3747712178758,7.38048596022667,
7.46305795471251,7.47524427712935,7.48289869735073,7.48892093247349,7.49453120091331,
7.50442000585867,7.53384700936255,7.57982322846128,7.68079260201834,7.71168068145007,
7.78163222917901,7.78909067834207,7.79281531994721,7.79578107269749,7.79910884046136,
7.80269930766009,7.80810667311621,7.81803337042311,7.8413464288574,7.94950972258716,
8.08127755737829,8.09624288142532,8.10556879378987,8.11285833400293,8.11969721084495,
8.13168331848794,8.17057963374346,8.23775088025926,8.36692615312483,8.49716252185221,
8.50371452653134,8.50750235320915,8.54433828515561,8.54889750221964,8.55122753263064,
8.55294558950003,8.55480699207006,8.55663437350001,8.56101574365353,8.59065994101801,
8.61522211780292,8.71309035524783,8.94841616827017,8.96320862286803,8.9675392510887,
8.97009273776712,8.97211862896137,8.9748178210844,8.97981096434038,9.00617830229802,
9.05766916499873,9.16378168996786,9.2067956661907,9.25444323354422,9.37134331817222,
9.37916210360649,9.38183564811077,9.38334845915371,9.38473458039316,9.38659682619818,
9.38857936531182,9.39170553119581,9.42561522673847,9.49852059576848,9.53022821423388,
9.56274593904948,9.73050279021206,9.74106333724318,9.74619334311474,9.74985475586656,
9.75371383150755,9.75749518935319,9.76243558929581,9.77025600448147,9.77104986109147,
9.96040829415487),.UNSPECIFIED.);
#3532=B_SPLINE_CURVE_WITH_KNOTS('',3,(#219194,#219195,#219196,#219197,#219198,
#219199,#219200,#219201,#219202,#219203,#219204,#219205,#219206,#219207,
#219208,#219209,#219210,#219211,#219212,#219213,#219214,#219215,#219216,
#219217,#219218,#219219,#219220,#219221,#219222,#219223,#219224,#219225,
#219226,#219227,#219228,#219229,#219230,#219231,#219232,#219233,#219234,
#219235,#219236,#219237,#219238,#219239,#219240,#219241,#219242,#219243,
#219244,#219245,#219246,#219247,#219248,#219249,#219250,#219251,#219252,
#219253,#219254,#219255,#219256,#219257,#219258,#219259,#219260,#219261,
#219262,#219263,#219264,#219265,#219266,#219267,#219268,#219269,#219270,
#219271,#219272,#219273,#219274,#219275,#219276,#219277,#219278,#219279,
#219280,#219281,#219282,#219283,#219284,#219285,#219286,#219287,#219288,
#219289,#219290,#219291,#219292,#219293,#219294,#219295,#219296,#219297,
#219298,#219299,#219300,#219301,#219302,#219303,#219304,#219305,#219306,
#219307,#219308,#219309,#219310,#219311,#219312,#219313,#219314,#219315,
#219316,#219317,#219318,#219319,#219320,#219321,#219322,#219323,#219324,
#219325,#219326,#219327,#219328,#219329,#219330,#219331,#219332,#219333,
#219334,#219335,#219336,#219337,#219338,#219339,#219340,#219341,#219342,
#219343,#219344,#219345,#219346,#219347,#219348,#219349,#219350,#219351,
#219352,#219353,#219354,#219355,#219356,#219357,#219358,#219359,#219360,
#219361,#219362,#219363,#219364,#219365,#219366,#219367,#219368,#219369,
#219370,#219371,#219372,#219373,#219374,#219375,#219376,#219377,#219378,
#219379,#219380,#219381,#219382,#219383,#219384,#219385,#219386,#219387,
#219388,#219389,#219390,#219391,#219392,#219393,#219394,#219395,#219396,
#219397,#219398,#219399,#219400,#219401,#219402,#219403,#219404,#219405,
#219406,#219407,#219408,#219409,#219410,#219411,#219412,#219413,#219414,
#219415,#219416,#219417,#219418,#219419,#219420,#219421,#219422,#219423,
#219424,#219425,#219426,#219427,#219428,#219429,#219430,#219431,#219432,
#219433,#219434,#219435,#219436,#219437,#219438,#219439,#219440,#219441,
#219442,#219443,#219444,#219445,#219446,#219447,#219448,#219449,#219450,
#219451,#219452),.UNSPECIFIED.,.F.,.F.,(4,3,3,3,3,3,3,3,3,3,3,3,3,3,3,3,
3,3,3,3,3,3,3,3,3,3,3,3,3,3,3,3,3,3,3,3,3,3,3,3,3,3,3,3,3,3,3,3,3,3,3,3,
3,3,3,3,3,3,3,3,3,3,3,3,3,3,3,3,3,3,3,3,3,3,3,3,3,3,3,3,3,3,3,3,3,3,4),
(57.6723164707605,57.7662350129566,57.8613028416319,57.9269046800067,58.0014341497759,
58.0758874780915,58.1502785677462,58.2246212803993,58.2989294454143,58.3732168683317,
58.447512414101,58.5218169201686,58.5961428835196,58.6705028101348,58.7449484930452,
58.8194433462206,58.8940402919011,58.9256444158688,58.9987833595532,59.0718342768603,
59.1448121008823,59.2177316953978,59.290607870374,59.3634553959561,59.4363028931159,
59.5091540416538,59.5820221907546,59.6549207008071,59.72790614237,59.8009389551458,
59.8740833792634,59.924384151731,59.9999124403979,60.0753546357312,60.1507236434258,
60.2260323213889,60.3012934877895,60.3790222877649,60.4542324850901,60.5294367097886,
60.6046465200537,60.6798734750397,60.7551563646492,60.8304724115199,60.9058593207772,
60.9231238875932,60.9997157879941,61.0762424899349,61.1527136858269,61.2291305460875,
61.3055145849215,61.3818747483341,61.4224937555243,61.5006130240034,61.5787773274772,
61.6569914044661,61.7352965271544,61.8136499537537,61.8920890435195,61.9218636234553,
62.003842402042,62.0857491512826,62.1696202363085,62.251285648823,62.3362595701047,
62.4212334913864,62.4948451654926,62.5684515323452,62.6420655842472,62.7157318767762,
62.7894254047999,62.8632008778658,62.9206033593175,62.9971040841234,63.0735488513046,
63.1499485708849,63.2263141204909,63.302656352682,63.3797421954942,63.4560840088709,
63.5324360965132,63.6088083206211,63.6864420142607,63.7629136912539,63.8411283932168,
63.9193430951797,63.9555017779401),.UNSPECIFIED.);
#3533=B_SPLINE_CURVE_WITH_KNOTS('',3,(#219454,#219455,#219456,#219457,#219458,
#219459,#219460,#219461,#219462,#219463,#219464,#219465,#219466),
 .UNSPECIFIED.,.F.,.F.,(4,1,1,1,1,1,1,1,1,1,4),(63.955503203756,64.4187129631108,
64.9180828310419,65.9168225669041,66.9155623027663,67.9143020386285,68.4136719065595,
68.9130417744906,69.4124116424217,69.9117815103529,70.2386870851197),
 .UNSPECIFIED.);
#3534=B_SPLINE_CURVE_WITH_KNOTS('',3,(#219468,#219469,#219470,#219471,#219472,
#219473,#219474,#219475,#219476,#219477,#219478,#219479,#219480,#219481,
#219482,#219483,#219484,#219485),.UNSPECIFIED.,.F.,.F.,(4,2,2,2,2,2,2,2,
4),(70.2386870851197,71.0736039970146,71.9085209089094,72.7434378208043,
73.5783547326992,74.413271644594,75.2481885564889,76.0831054683838,76.5218723922993),
 .UNSPECIFIED.);
#3535=B_SPLINE_CURVE_WITH_KNOTS('',3,(#219487,#219488,#219489,#219490,#219491,
#219492,#219493,#219494,#219495,#219496,#219497,#219498,#219499,#219500,
#219501,#219502,#219503,#219504,#219505,#219506,#219507,#219508,#219509,
#219510,#219511,#219512,#219513,#219514,#219515,#219516,#219517,#219518,
#219519,#219520,#219521,#219522,#219523,#219524,#219525,#219526,#219527,
#219528,#219529,#219530,#219531,#219532,#219533,#219534,#219535,#219536,
#219537,#219538,#219539,#219540,#219541,#219542,#219543,#219544,#219545,
#219546,#219547,#219548,#219549,#219550,#219551,#219552,#219553,#219554,
#219555,#219556,#219557,#219558,#219559,#219560,#219561,#219562,#219563,
#219564,#219565,#219566,#219567,#219568,#219569,#219570,#219571,#219572,
#219573,#219574,#219575,#219576,#219577,#219578,#219579,#219580,#219581,
#219582,#219583,#219584,#219585,#219586,#219587,#219588,#219589,#219590,
#219591,#219592,#219593,#219594,#219595,#219596,#219597,#219598,#219599,
#219600,#219601,#219602,#219603,#219604,#219605,#219606,#219607,#219608,
#219609,#219610,#219611,#219612,#219613,#219614,#219615,#219616,#219617,
#219618,#219619,#219620,#219621,#219622,#219623,#219624,#219625,#219626,
#219627,#219628,#219629,#219630,#219631,#219632,#219633,#219634,#219635,
#219636,#219637,#219638,#219639,#219640,#219641,#219642,#219643,#219644,
#219645,#219646,#219647,#219648,#219649,#219650,#219651,#219652,#219653,
#219654,#219655,#219656,#219657,#219658,#219659,#219660,#219661,#219662,
#219663,#219664,#219665,#219666,#219667,#219668,#219669,#219670,#219671,
#219672,#219673,#219674,#219675,#219676,#219677,#219678,#219679,#219680,
#219681,#219682,#219683,#219684,#219685,#219686,#219687,#219688,#219689,
#219690,#219691,#219692,#219693,#219694,#219695,#219696,#219697,#219698,
#219699,#219700,#219701,#219702,#219703,#219704,#219705,#219706,#219707,
#219708,#219709,#219710,#219711,#219712,#219713,#219714,#219715,#219716,
#219717,#219718,#219719,#219720,#219721,#219722,#219723,#219724,#219725,
#219726,#219727,#219728,#219729,#219730,#219731,#219732,#219733,#219734,
#219735,#219736,#219737,#219738,#219739,#219740,#219741,#219742,#219743,
#219744,#219745,#219746,#219747,#219748),.UNSPECIFIED.,.F.,.F.,(4,3,3,3,
3,3,3,3,3,3,3,3,3,3,3,3,3,3,3,3,3,3,3,3,3,3,3,3,3,3,3,3,3,3,3,3,3,3,3,3,
3,3,3,3,3,3,3,3,3,3,3,3,3,3,3,3,3,3,3,3,3,3,3,3,3,3,3,3,3,3,3,3,3,3,3,3,
3,3,3,3,3,3,3,3,3,3,3,4),(76.5218723922993,76.5974953734188,76.6738614454111,
76.749610786608,76.826285223998,76.9029596613881,76.979460386194,77.0559051533751,
77.1323048729554,77.2086704225614,77.2850126547524,77.3620984975647,77.4384403109414,
77.5147923985836,77.5911646226914,77.6687983163311,77.7452699933244,77.8234846952873,
77.9016993972503,77.9763812119391,78.0509830640905,78.1255173476643,78.1999859051987,
78.2744161207925,78.3488210325928,78.4010692651814,78.4813665136047,78.5618089865093,
78.6464665231601,78.7272466695768,78.8081281805109,78.8891449809138,78.9004391331125,
78.9749686028818,79.0494219311975,79.1238130208523,79.1981557335055,79.2724638985205,
79.346751321438,79.4210468672074,79.4953513732751,79.5696773366261,79.6440372632414,
79.7184829461518,79.7929777993273,79.8675747450079,79.8991788689747,79.9723178126591,
80.0453687299662,80.1183465539882,80.1912661485037,80.2641423234798,80.3369898490617,
80.4098373462215,80.4826884947594,80.5555566438602,80.6284551539126,80.7014405954755,
80.7744734082513,80.8476178323689,80.8979186048369,80.9734468935038,81.048889088837,
81.1242580965317,81.1995667744947,81.2748279408952,81.3525567408707,81.4277669381958,
81.5029711628943,81.5781809731595,81.6534079281456,81.728690817755,81.8040068646258,
81.8793937738832,81.896658340699,81.9732502410998,82.0497769430406,82.1262481389325,
82.2026649991931,82.2790490380269,82.3554092014394,82.3960282086301,82.4727948422462,
82.5495919908356,82.62645942842,82.7033661826157,82.7803503634339,82.8050576994789),
 .UNSPECIFIED.);
#3536=B_SPLINE_CURVE_WITH_KNOTS('',3,(#219750,#219751,#219752,#219753,#219754,
#219755,#219756,#219757,#219758,#219759,#219760,#219761,#219762),
 .UNSPECIFIED.,.F.,.F.,(4,1,1,1,1,1,1,1,1,1,4),(82.8050576994789,82.8953980765612,
83.3947679444923,83.8941378124234,84.8928775482856,85.3922474162167,85.8916172841478,
86.8903570200099,87.8890967558721,88.8878364917343,89.0882430066585),
 .UNSPECIFIED.);
#3537=B_SPLINE_CURVE_WITH_KNOTS('',3,(#219764,#219765,#219766,#219767,#219768,
#219769,#219770,#219771,#219772,#219773,#219774,#219775,#219776,#219777,
#219778,#219779,#219780,#219781,#219782,#219783,#219784,#219785,#219786,
#219787,#219788,#219789,#219790,#219791,#219792,#219793,#219794,#219795,
#219796,#219797,#219798,#219799,#219800,#219801,#219802,#219803,#219804,
#219805,#219806,#219807,#219808,#219809,#219810,#219811,#219812,#219813,
#219814,#219815,#219816,#219817,#219818,#219819,#219820,#219821,#219822,
#219823,#219824,#219825,#219826,#219827,#219828,#219829,#219830,#219831,
#219832,#219833,#219834,#219835,#219836,#219837,#219838,#219839,#219840,
#219841,#219842,#219843,#219844,#219845,#219846,#219847,#219848,#219849,
#219850,#219851,#219852,#219853,#219854,#219855,#219856,#219857,#219858,
#219859,#219860,#219861,#219862,#219863,#219864,#219865,#219866,#219867,
#219868,#219869,#219870,#219871,#219872,#219873,#219874,#219875,#219876,
#219877,#219878,#219879,#219880,#219881,#219882,#219883,#219884,#219885,
#219886,#219887,#219888,#219889,#219890,#219891,#219892,#219893,#219894,
#219895,#219896,#219897,#219898,#219899,#219900,#219901,#219902,#219903,
#219904,#219905,#219906,#219907,#219908,#219909,#219910,#219911,#219912,
#219913,#219914,#219915,#219916,#219917,#219918,#219919,#219920,#219921,
#219922,#219923,#219924,#219925,#219926,#219927,#219928,#219929,#219930,
#219931,#219932,#219933,#219934,#219935,#219936,#219937,#219938,#219939,
#219940,#219941,#219942,#219943,#219944,#219945,#219946,#219947,#219948,
#219949,#219950,#219951,#219952,#219953,#219954,#219955,#219956,#219957,
#219958,#219959,#219960,#219961,#219962,#219963,#219964,#219965,#219966,
#219967,#219968,#219969,#219970,#219971,#219972,#219973,#219974,#219975,
#219976,#219977,#219978,#219979,#219980,#219981,#219982,#219983,#219984,
#219985,#219986,#219987,#219988,#219989,#219990,#219991,#219992,#219993,
#219994,#219995,#219996,#219997,#219998,#219999,#220000,#220001,#220002,
#220003,#220004,#220005,#220006,#220007,#220008,#220009,#220010,#220011,
#220012,#220013,#220014,#220015,#220016,#220017,#220018,#220019),
 .UNSPECIFIED.,.F.,.F.,(4,3,3,3,3,3,3,3,3,3,3,3,3,3,3,3,3,3,3,3,3,3,3,3,
3,3,3,3,3,3,3,3,3,3,3,3,3,3,3,3,3,3,3,3,3,3,3,3,3,3,3,3,3,3,3,3,3,3,3,3,
3,3,3,3,3,3,3,3,3,3,3,3,3,3,3,3,3,3,3,3,3,3,3,3,3,4),(89.0882430066585,
89.1629838449102,89.2359045239601,89.3115554418127,89.3872063596654,89.4653256281447,
89.5434899316183,89.6217040086076,89.7000091312961,89.7783625578954,89.8568016476615,
89.8865762275965,89.9685550061832,90.0504617554236,90.1343328404496,90.2159982529641,
90.3009721742459,90.3859460955276,90.4595577696338,90.5331641364866,90.6067781883886,
90.6804444809175,90.7541380089414,90.8279134820071,90.8853159634587,90.9618166882646,
91.0382614554458,91.1146611750261,91.1910267246322,91.2673689568237,91.3444547996359,
91.4207966130128,91.4971487006549,91.5735209247626,91.6511546184022,91.7276262953954,
91.8058409973582,91.8840556993209,91.9587375140096,92.0333393661611,92.1078736497346,
92.1823422072689,92.2567724228627,92.3311773346629,92.3834255672519,92.463722815675,
92.5441652885799,92.6288228252307,92.7096029716479,92.7904844825828,92.8715012829858,
92.8827954351831,92.9573249049524,93.0317782332682,93.106169322923,93.1805120355759,
93.2548202005907,93.3291076235081,93.4034031692775,93.4777076753451,93.552033638696,
93.6263935653112,93.7008392482215,93.7753341013972,93.8499310470776,93.8815351710452,
93.9546741147296,94.0277250320366,94.1007028560584,94.173622450574,94.2464986255501,
94.3193461511323,94.3921936482919,94.4650447968299,94.5379129459309,94.6108114559836,
94.6837968975463,94.7568297103218,94.8299741344395,94.8802749069074,94.9621583016442,
95.0438908023668,95.1257751802347,95.2070912819773,95.2892597979077,95.3714283138381),
 .UNSPECIFIED.);
#3538=B_SPLINE_CURVE_WITH_KNOTS('',3,(#220021,#220022,#220023,#220024,#220025,
#220026,#220027,#220028,#220029,#220030,#220031,#220032,#220033,#220034,
#220035,#220036,#220037,#220038,#220039,#220040,#220041,#220042,#220043,
#220044,#220045,#220046,#220047,#220048,#220049,#220050,#220051,#220052,
#220053,#220054,#220055,#220056,#220057,#220058,#220059,#220060,#220061,
#220062,#220063,#220064,#220065,#220066,#220067,#220068,#220069,#220070,
#220071,#220072,#220073,#220074,#220075,#220076,#220077,#220078,#220079,
#220080,#220081,#220082,#220083,#220084,#220085,#220086,#220087,#220088,
#220089,#220090,#220091,#220092,#220093,#220094,#220095,#220096,#220097,
#220098,#220099,#220100,#220101,#220102,#220103,#220104,#220105,#220106,
#220107,#220108,#220109,#220110,#220111,#220112,#220113,#220114,#220115,
#220116,#220117,#220118,#220119,#220120,#220121,#220122,#220123,#220124,
#220125,#220126,#220127,#220128,#220129,#220130,#220131,#220132,#220133,
#220134,#220135,#220136,#220137,#220138,#220139,#220140,#220141,#220142,
#220143,#220144,#220145,#220146,#220147,#220148,#220149,#220150,#220151,
#220152,#220153,#220154,#220155,#220156,#220157,#220158,#220159,#220160,
#220161,#220162,#220163,#220164,#220165,#220166,#220167,#220168,#220169,
#220170,#220171,#220172,#220173,#220174,#220175,#220176,#220177,#220178,
#220179,#220180,#220181,#220182,#220183,#220184,#220185,#220186,#220187,
#220188,#220189,#220190,#220191,#220192,#220193,#220194,#220195,#220196,
#220197,#220198,#220199,#220200,#220201,#220202,#220203,#220204,#220205,
#220206,#220207,#220208,#220209,#220210,#220211,#220212,#220213,#220214,
#220215,#220216,#220217,#220218,#220219,#220220,#220221,#220222,#220223,
#220224,#220225,#220226,#220227,#220228,#220229,#220230,#220231,#220232,
#220233,#220234,#220235,#220236,#220237,#220238,#220239,#220240,#220241,
#220242,#220243,#220244,#220245,#220246,#220247,#220248,#220249,#220250,
#220251,#220252,#220253,#220254,#220255,#220256,#220257,#220258,#220259,
#220260,#220261,#220262,#220263,#220264,#220265,#220266,#220267,#220268,
#220269,#220270,#220271,#220272,#220273,#220274,#220275,#220276,#220277,
#220278,#220279,#220280,#220281,#220282,#220283,#220284,#220285,#220286,
#220287,#220288,#220289,#220290,#220291,#220292,#220293,#220294,#220295,
#220296,#220297,#220298,#220299,#220300,#220301,#220302,#220303,#220304,
#220305,#220306,#220307,#220308,#220309,#220310,#220311,#220312,#220313,
#220314,#220315,#220316,#220317,#220318,#220319,#220320,#220321,#220322,
#220323,#220324,#220325,#220326,#220327,#220328,#220329,#220330,#220331,
#220332,#220333,#220334,#220335,#220336,#220337,#220338,#220339,#220340,
#220341,#220342,#220343,#220344,#220345,#220346,#220347,#220348,#220349,
#220350,#220351,#220352,#220353,#220354,#220355,#220356,#220357,#220358,
#220359,#220360,#220361,#220362,#220363,#220364,#220365,#220366,#220367,
#220368,#220369,#220370,#220371,#220372,#220373,#220374,#220375,#220376,
#220377,#220378,#220379,#220380,#220381,#220382,#220383,#220384,#220385,
#220386,#220387,#220388,#220389,#220390,#220391,#220392,#220393,#220394,
#220395,#220396,#220397,#220398,#220399,#220400,#220401,#220402,#220403,
#220404,#220405,#220406,#220407,#220408,#220409,#220410,#220411,#220412,
#220413,#220414,#220415,#220416,#220417,#220418,#220419,#220420,#220421,
#220422,#220423,#220424,#220425,#220426,#220427,#220428,#220429,#220430,
#220431,#220432,#220433,#220434,#220435,#220436,#220437,#220438,#220439,
#220440,#220441,#220442,#220443,#220444,#220445,#220446,#220447,#220448,
#220449,#220450,#220451,#220452,#220453,#220454,#220455,#220456,#220457,
#220458,#220459,#220460,#220461,#220462,#220463,#220464,#220465,#220466,
#220467,#220468,#220469,#220470,#220471,#220472,#220473,#220474,#220475,
#220476,#220477,#220478,#220479,#220480,#220481,#220482,#220483,#220484,
#220485,#220486,#220487,#220488,#220489,#220490,#220491,#220492,#220493,
#220494,#220495,#220496,#220497,#220498,#220499,#220500,#220501,#220502,
#220503,#220504,#220505,#220506,#220507,#220508,#220509,#220510,#220511,
#220512,#220513,#220514,#220515,#220516,#220517,#220518,#220519,#220520,
#220521,#220522,#220523,#220524,#220525,#220526,#220527,#220528,#220529,
#220530,#220531,#220532,#220533,#220534,#220535,#220536,#220537,#220538,
#220539,#220540,#220541,#220542,#220543,#220544,#220545,#220546,#220547,
#220548,#220549,#220550,#220551,#220552,#220553,#220554,#220555,#220556,
#220557,#220558),.UNSPECIFIED.,.F.,.F.,(4,2,2,2,2,2,2,2,2,2,2,2,2,2,2,2,
2,2,2,2,2,2,2,2,2,2,2,2,2,2,2,2,2,2,2,2,2,2,2,2,2,2,2,2,2,2,2,2,2,2,2,2,
2,2,2,2,2,2,2,2,2,2,2,2,2,2,2,2,2,2,2,2,2,2,2,2,2,2,2,2,2,2,2,2,2,2,2,2,
2,2,2,2,2,2,2,2,2,2,2,2,2,2,2,2,2,2,2,2,2,2,2,2,2,2,2,2,2,2,2,2,2,2,2,2,
2,2,2,2,2,2,2,2,2,2,2,2,2,2,2,2,2,2,2,2,2,2,2,2,2,2,2,2,2,2,2,2,2,2,2,2,
2,2,2,2,2,2,2,2,2,2,2,2,2,2,2,2,2,2,2,2,2,2,2,2,2,2,2,2,2,2,2,2,2,2,2,2,
2,2,2,2,2,2,2,2,2,2,2,2,2,2,2,2,2,2,2,2,2,2,2,2,2,2,2,2,2,2,2,2,2,2,2,2,
2,2,2,2,2,2,2,2,2,2,2,2,2,2,2,2,2,2,2,2,2,2,2,2,2,2,2,2,2,2,2,2,2,2,2,2,
4),(0.00144023023890332,0.0188352441522348,0.0286240747235862,0.0320264665064641,
0.034401950934542,0.0364310360599029,0.0384721181132475,0.0411577116316496,
0.0452708277222326,0.0634610453250711,0.0760085167908262,0.352519182779323,
0.373658015965884,0.423576959264981,0.433506795172639,0.436846024628858,
0.439017742336696,0.441074958351601,0.443798416142434,0.449926042113504,
0.510964764186585,0.655162687143893,0.858795601058024,0.880268179166108,
0.888940947904201,0.895122893279219,0.900711915761007,0.908143516087384,
0.913790892828657,0.948548411783089,1.16549407514662,1.19259001574114,1.19828764660113,
1.20168164513884,1.20473368822417,1.20861837620083,1.21478406144893,1.24704524323629,
1.32729344738685,1.43982947292849,1.49458470983966,1.50821191257729,1.51634732222258,
1.52363249898271,1.53291882318514,1.55220293962084,1.57982827843173,1.64256155500931,
1.8211317721868,1.90989618222559,1.95287835821233,1.95765014281574,1.95998924026183,
1.96165093475284,1.96339150443963,1.96580849772034,1.97069945568749,2.03322229580789,
2.26757814736068,2.35742605323967,2.36690386149683,2.3717662308098,2.37479174050958,
2.37757361565507,2.37978623446255,2.38198524778634,2.38515830116659,2.39407408555732,
2.53621071498992,2.69152738339444,2.70956712254707,2.77734345088054,2.78728155706024,
2.79009575634249,2.79180883892596,2.79335344003183,2.79532295066489,2.79920105508675,
2.82200422641208,2.83021153916663,2.83806875528213,2.84860838412361,2.85163575133896,
2.88918425693327,2.9818226688322,3.13783646361113,3.15037392426803,3.15573872948844,
3.15964768256213,3.16323419892985,3.16807853487824,3.17979513073606,3.28524022044815,
3.40284750589108,3.52028170954202,3.53422586185235,3.53768064061847,3.53969265320981,
3.54145127212847,3.54362109605788,3.54691995754242,3.5611722394563,3.80260460346203,
3.91301657289305,3.92846852468512,3.93245753268311,3.93481022159704,3.93688451468692,
3.93946695952734,3.94343919726604,3.96125229793376,4.26476507035458,4.3530851174613,
4.35756796736892,4.35927277032363,4.36044189402177,4.3615827862087,4.36295557908335,
4.36630940139405,4.39757533309571,4.4075722626596,4.45999316779878,4.62981835601763,
4.68654418773814,4.73232327747958,4.7558611664724,4.76028759756685,4.76267562172917,
4.76446576367316,4.76671909321462,4.77053308599018,4.78348822409693,4.98221680467369,
5.14432299168534,5.15459965785234,5.15681531121783,5.15826746538052,5.15944108709222,
5.16077990766441,5.16306828961999,5.1721426027617,5.24031539593307,5.35941274712733,
5.46605877873562,5.46928864799795,5.49685230089605,5.5673330761146,5.57413581157382,
5.57690228970075,5.57894195542656,5.58115124680858,5.58415281721192,5.59099981010166,
5.6961298515114,5.77014561470142,5.83936481622827,5.85790850607198,5.96769864668797,
5.97560875774998,5.97844386007364,5.98041572498261,5.98224295359785,5.98472936221921,
5.98950033826606,6.01952346240784,6.09156508481059,6.25393037786808,6.27481435911482,
6.40537180532509,6.42338818380982,6.4313936839041,6.43748431914233,6.44398016216563,
6.45415631574082,6.4867195625245,6.53874938699504,6.68394184829103,6.73185830236833,
6.73873685294598,6.74241527817458,6.74545121175061,6.74898962280641,6.75524529526294,
6.78378187726126,6.91678785863251,6.99764802407582,7.00417155628134,7.03913997633799,
7.05125760652064,7.05828206084589,7.06486048783464,7.07397123416969,7.09233334477615,
7.20291984640308,7.36292443563327,7.49156309097314,7.49824352238908,7.50095236925486,
7.50282960572948,7.50466862267205,7.50726360245302,7.51341161203112,7.59934647328734,
7.8972450792491,7.91328942986097,7.91770518649558,7.92030410315222,7.92255161646135,
7.92529407213015,7.93048681649165,7.96081504083705,8.01427203493585,8.06724767933589,
8.10991975273886,8.12423205614896,8.13660174287348,8.1475548872055,8.15785302321648,
8.16755211428555,8.17674004568409,8.32040272382137,8.3293531831775,8.33212045499302,
8.33381487393204,8.3353239644011,8.3372332553652,8.3409476579724,8.36570580076754,
8.42761507744329,8.57824115777725,8.68204003919545,8.69203550369335,8.69702611196787,
8.70065145344625,8.70453164618465,8.70972874845631,8.72125556241187,8.90719934899358,
9.0077235406749,9.07290673418962,9.07846548217621,9.08089527502724,9.08267459918955,
9.0843234831423,9.08685937845684,9.09298559287519,9.18523492126532,9.41381663160004,
9.46700189852647,9.47323485054633,9.47576803623214,9.47788458640844,9.48005975562622,
9.4832436704937,9.4916907266521,9.6062770726423,9.83863674155126,9.84567994066315,
9.86899345205559,9.89643833095047,9.89943482306625,9.90091372081988,9.90197866263517,
9.9030504309227,9.90414428284082,9.90556436281459,9.90780983704934,9.90931945351448,
9.96250952171965),.UNSPECIFIED.);
#3539=B_SPLINE_CURVE_WITH_KNOTS('',3,(#220560,#220561,#220562,#220563,#220564,
#220565,#220566,#220567,#220568,#220569,#220570,#220571,#220572),
 .UNSPECIFIED.,.F.,.F.,(4,1,1,1,1,1,1,1,1,1,4),(107.938353794554,108.862631208978,
109.86137094484,110.360740812771,110.860110680702,111.359480548633,111.858850416565,
112.857590152427,113.356960020358,113.856329888289,114.220975245612),
 .UNSPECIFIED.);
#3540=B_SPLINE_CURVE_WITH_KNOTS('',3,(#220574,#220575,#220576,#220577,#220578,
#220579,#220580,#220581,#220582,#220583,#220584,#220585,#220586,#220587,
#220588,#220589,#220590,#220591,#220592,#220593,#220594,#220595,#220596,
#220597,#220598,#220599,#220600,#220601,#220602,#220603,#220604,#220605,
#220606,#220607,#220608,#220609,#220610,#220611,#220612,#220613,#220614,
#220615,#220616,#220617,#220618,#220619,#220620,#220621,#220622,#220623,
#220624,#220625,#220626,#220627,#220628,#220629,#220630,#220631,#220632,
#220633,#220634,#220635,#220636,#220637,#220638,#220639,#220640,#220641,
#220642,#220643,#220644,#220645,#220646,#220647,#220648,#220649,#220650,
#220651,#220652,#220653,#220654,#220655,#220656,#220657,#220658,#220659,
#220660,#220661,#220662,#220663,#220664,#220665,#220666,#220667,#220668,
#220669,#220670,#220671,#220672,#220673,#220674,#220675,#220676,#220677,
#220678,#220679,#220680,#220681,#220682,#220683,#220684,#220685,#220686,
#220687,#220688,#220689,#220690,#220691,#220692,#220693,#220694,#220695,
#220696,#220697,#220698,#220699,#220700,#220701,#220702,#220703,#220704,
#220705,#220706,#220707,#220708,#220709,#220710,#220711,#220712,#220713,
#220714,#220715,#220716,#220717,#220718,#220719,#220720,#220721,#220722,
#220723,#220724,#220725,#220726,#220727,#220728,#220729,#220730,#220731,
#220732,#220733,#220734,#220735,#220736,#220737,#220738,#220739,#220740,
#220741,#220742,#220743,#220744,#220745,#220746,#220747,#220748,#220749,
#220750,#220751,#220752,#220753,#220754,#220755,#220756,#220757,#220758,
#220759,#220760,#220761,#220762,#220763,#220764,#220765,#220766,#220767,
#220768,#220769,#220770,#220771,#220772,#220773,#220774,#220775,#220776,
#220777,#220778,#220779,#220780,#220781,#220782,#220783,#220784,#220785,
#220786,#220787,#220788,#220789,#220790,#220791,#220792,#220793,#220794,
#220795,#220796,#220797,#220798,#220799,#220800,#220801,#220802,#220803,
#220804,#220805,#220806,#220807,#220808,#220809,#220810,#220811,#220812,
#220813,#220814,#220815,#220816,#220817,#220818,#220819,#220820,#220821,
#220822,#220823,#220824,#220825,#220826,#220827,#220828,#220829,#220830,
#220831,#220832,#220833,#220834,#220835),.UNSPECIFIED.,.F.,.F.,(4,3,3,3,
3,3,3,3,3,3,3,3,3,3,3,3,3,3,3,3,3,3,3,3,3,3,3,3,3,3,3,3,3,3,3,3,3,3,3,3,
3,3,3,3,3,3,3,3,3,3,3,3,3,3,3,3,3,3,3,3,3,3,3,3,3,3,3,3,3,3,3,3,3,3,3,3,
3,3,3,3,3,3,3,3,3,3,3,4),(114.220984235377,114.300244908974,114.376091153155,
114.451972074714,114.527898076741,114.603879587423,114.679971804733,114.756128068702,
114.832399526875,114.855069624151,114.928208567835,115.001259485142,115.074237309164,
115.14715690368,115.220033078656,115.292880604238,115.365728101397,115.438579249935,
115.511447399036,115.584345909089,115.657331350652,115.730364163428,115.803508587545,
115.853809360013,115.92933764868,116.004779844013,116.080148851707,116.15545752967,
116.23071869607,116.308447496046,116.383657693371,116.458861918069,116.534071728334,
116.60929868332,116.684581572929,116.7598976198,116.835284529057,116.852549095875,
116.929140996276,117.005667698218,117.08213889411,117.158555754371,117.234939793206,
117.311299956619,117.351918963807,117.430038232286,117.50820253576,117.586416612749,
117.664721735438,117.743075162037,117.821514251804,117.851288831738,117.933267610324,
118.015174359564,118.09904544459,118.180710857104,118.265684778387,118.350658699669,
118.424270373775,118.497876740628,118.571490792531,118.64515708506,118.718850613084,
118.79262608615,118.8500285676,118.926529292406,119.002974059587,119.079373779167,
119.155739328773,119.232081560963,119.309167403776,119.385509217152,119.461861304794,
119.538233528902,119.615867222542,119.692338899535,119.770553601498,119.848768303462,
119.923450118151,119.998051970303,120.072586253877,120.147054811412,120.221485027006,
120.295889938807,120.348138171393,120.421620020599,120.495149820344,120.504169542556),
 .UNSPECIFIED.);
#3541=B_SPLINE_CURVE_WITH_KNOTS('',3,(#220837,#220838,#220839,#220840,#220841,
#220842,#220843,#220844,#220845,#220846,#220847,#220848),.UNSPECIFIED.,
 .F.,.F.,(4,1,1,1,1,1,1,1,1,4),(120.504170804088,120.847508039324,121.846247775186,
122.844987511049,123.843727246911,124.343097114842,124.842466982773,125.341836850704,
125.841206718635,126.787354849736),.UNSPECIFIED.);
#3542=B_SPLINE_CURVE_WITH_KNOTS('',3,(#220850,#220851,#220852,#220853,#220854,
#220855,#220856,#220857,#220858,#220859,#220860,#220861,#220862,#220863,
#220864,#220865,#220866,#220867,#220868,#220869,#220870,#220871,#220872,
#220873,#220874,#220875,#220876,#220877,#220878,#220879,#220880,#220881,
#220882,#220883,#220884,#220885,#220886,#220887,#220888,#220889,#220890,
#220891,#220892,#220893,#220894,#220895,#220896,#220897,#220898,#220899,
#220900,#220901,#220902,#220903,#220904,#220905,#220906,#220907,#220908,
#220909,#220910,#220911,#220912,#220913,#220914,#220915,#220916,#220917,
#220918,#220919,#220920,#220921,#220922,#220923,#220924,#220925,#220926,
#220927,#220928,#220929,#220930,#220931,#220932,#220933,#220934,#220935,
#220936,#220937,#220938,#220939,#220940,#220941,#220942,#220943,#220944,
#220945,#220946,#220947,#220948,#220949,#220950,#220951,#220952,#220953,
#220954,#220955,#220956,#220957,#220958,#220959,#220960,#220961,#220962,
#220963,#220964,#220965,#220966,#220967,#220968,#220969,#220970,#220971,
#220972,#220973,#220974,#220975,#220976,#220977,#220978,#220979,#220980,
#220981,#220982,#220983,#220984,#220985,#220986,#220987,#220988,#220989,
#220990,#220991,#220992,#220993,#220994,#220995,#220996,#220997,#220998,
#220999,#221000,#221001,#221002,#221003,#221004,#221005,#221006,#221007,
#221008,#221009,#221010,#221011,#221012,#221013,#221014,#221015,#221016,
#221017,#221018,#221019,#221020,#221021,#221022,#221023,#221024,#221025,
#221026,#221027,#221028,#221029,#221030,#221031,#221032,#221033,#221034,
#221035,#221036,#221037,#221038,#221039,#221040,#221041,#221042,#221043,
#221044,#221045,#221046,#221047,#221048,#221049,#221050,#221051,#221052,
#221053,#221054,#221055,#221056,#221057,#221058,#221059,#221060,#221061,
#221062,#221063,#221064,#221065,#221066,#221067,#221068,#221069,#221070,
#221071,#221072,#221073,#221074,#221075,#221076,#221077,#221078,#221079,
#221080,#221081,#221082,#221083,#221084,#221085,#221086,#221087,#221088,
#221089,#221090,#221091,#221092,#221093,#221094,#221095,#221096,#221097,
#221098,#221099,#221100,#221101,#221102,#221103,#221104,#221105,#221106,
#221107,#221108,#221109,#221110,#221111,#221112,#221113,#221114,#221115,
#221116,#221117,#221118,#221119,#221120,#221121,#221122,#221123,#221124,
#221125,#221126,#221127,#221128,#221129,#221130,#221131,#221132,#221133,
#221134,#221135,#221136,#221137,#221138,#221139,#221140,#221141,#221142,
#221143,#221144,#221145,#221146,#221147,#221148,#221149,#221150,#221151,
#221152,#221153,#221154,#221155,#221156,#221157,#221158,#221159,#221160,
#221161,#221162,#221163,#221164,#221165,#221166,#221167,#221168,#221169,
#221170,#221171,#221172,#221173,#221174,#221175,#221176,#221177,#221178,
#221179,#221180,#221181,#221182,#221183,#221184,#221185,#221186,#221187,
#221188,#221189,#221190,#221191,#221192,#221193,#221194,#221195,#221196,
#221197,#221198,#221199,#221200,#221201,#221202,#221203,#221204,#221205,
#221206,#221207,#221208,#221209,#221210,#221211,#221212,#221213,#221214,
#221215,#221216,#221217,#221218,#221219,#221220,#221221,#221222,#221223,
#221224,#221225,#221226,#221227,#221228,#221229,#221230,#221231,#221232,
#221233,#221234,#221235,#221236,#221237,#221238,#221239,#221240,#221241,
#221242,#221243,#221244,#221245,#221246,#221247,#221248,#221249,#221250,
#221251,#221252,#221253,#221254,#221255,#221256,#221257,#221258,#221259,
#221260,#221261,#221262,#221263,#221264,#221265,#221266,#221267,#221268,
#221269,#221270,#221271,#221272,#221273,#221274,#221275,#221276,#221277,
#221278,#221279,#221280,#221281,#221282,#221283,#221284,#221285,#221286,
#221287,#221288,#221289,#221290,#221291,#221292,#221293,#221294,#221295,
#221296,#221297,#221298,#221299,#221300,#221301,#221302,#221303,#221304,
#221305,#221306,#221307,#221308,#221309,#221310,#221311,#221312,#221313,
#221314,#221315,#221316,#221317,#221318,#221319,#221320,#221321,#221322,
#221323,#221324,#221325,#221326,#221327,#221328,#221329,#221330,#221331,
#221332,#221333,#221334,#221335,#221336,#221337,#221338,#221339,#221340,
#221341,#221342,#221343,#221344,#221345,#221346,#221347,#221348,#221349,
#221350,#221351,#221352,#221353,#221354,#221355,#221356,#221357,#221358,
#221359,#221360,#221361,#221362,#221363,#221364,#221365,#221366,#221367,
#221368,#221369,#221370,#221371,#221372,#221373,#221374,#221375,#221376,
#221377,#221378,#221379,#221380,#221381,#221382,#221383,#221384,#221385,
#221386,#221387,#221388,#221389),.UNSPECIFIED.,.F.,.F.,(4,2,2,2,2,2,2,2,
2,2,2,2,2,2,2,2,2,2,2,2,2,2,2,2,2,2,2,2,2,2,2,2,2,2,2,2,2,2,2,2,2,2,2,2,
2,2,2,2,2,2,2,2,2,2,2,2,2,2,2,2,2,2,2,2,2,2,2,2,2,2,2,2,2,2,2,2,2,2,2,2,
2,2,2,2,2,2,2,2,2,2,2,2,2,2,2,2,2,2,2,2,2,2,2,2,2,2,2,2,2,2,2,2,2,2,2,2,
2,2,2,2,2,2,2,2,2,2,2,2,2,2,2,2,2,2,2,2,2,2,2,2,2,2,2,2,2,2,2,2,2,2,2,2,
2,2,2,2,2,2,2,2,2,2,2,2,2,2,2,2,2,2,2,2,2,2,2,2,2,2,2,2,2,2,2,2,2,2,2,2,
2,2,2,2,2,2,2,2,2,2,2,2,2,2,2,2,2,2,2,2,2,2,2,2,2,2,2,2,2,2,2,2,2,2,2,2,
2,2,2,2,2,2,2,2,2,2,2,2,2,2,2,2,2,2,2,2,2,2,2,2,2,2,2,2,2,2,2,2,2,2,2,2,
2,2,2,2,2,2,2,2,2,4),(0.00190372001199662,0.0478014467504751,0.0515987046793617,
0.0538690362872017,0.0554968680757349,0.0569311409708447,0.0584885609762871,
0.0605190974258305,0.0649568043178509,0.0998653319031922,0.111694939859996,
0.121789696784997,0.334545570911788,0.391911534125962,0.405631968002068,
0.416256389217015,0.42127042259101,0.425121226471219,0.428801565723861,
0.434003369235636,0.444803483155246,0.551988386604616,0.700426860411103,
0.762525122245161,0.785881086988788,0.794621043971917,0.798885153758925,
0.802368847880747,0.804374498566845,0.805973795575332,0.808032480248983,
0.811602664083345,0.825313450549338,0.943719966405224,0.954530695091559,
0.966520891886942,0.979995208431586,0.995334756667944,1.01308128280235,
1.03409192175351,1.05992385904713,1.15312596805555,1.19067635209875,1.19582725624681,
1.19842987272194,1.20030954294169,1.20230652010343,1.20512594836215,1.21098601534292,
1.27314098509753,1.47991116819721,1.5612497809114,1.60166180571516,1.61908016711595,
1.62175388831596,1.62287592646669,1.6240133112277,1.62506407795409,1.62649567105522,
1.6293567876305,1.65398201881818,1.72463604636923,1.84051827173563,2.0045064395514,
2.02002008436021,2.02390406786188,2.02617227177171,2.02815835790718,2.03061318171153,
2.03435645970311,2.05066237850186,2.31263760833465,2.37831262379276,2.41284562919197,
2.4187943957808,2.42073158153679,2.42183051281163,2.42300610602772,2.42448549078746,
2.42679195528197,2.43759645850929,2.47479509871719,2.50235015129785,2.71507719902023,
2.82821809505195,2.83686943076858,2.84016836381979,2.84243432121922,2.84464875639419,
2.84731059889031,2.85392008642146,2.91296163152424,3.10607723271175,3.16718566201027,
3.19041142713024,3.23022539778443,3.23596626748258,3.23926402402234,3.24153327329948,
3.24371993197974,3.24570813771416,3.24830837923052,3.25346145107911,3.28515815924116,
3.41943174105194,3.59169782035772,3.67629644569596,3.6894033965237,3.69653438374018,
3.70193245967649,3.70882649745226,3.72050984361697,3.76494841721059,3.76897255286623,
3.97792542616526,3.99142434773547,4.00091886147739,4.00497159761806,4.00804606250772,
4.01095584193143,4.01582572459138,4.02864038780943,4.15070151705689,4.24802021138349,
4.29981686693513,4.31321130681746,4.32129572033366,4.32859113996387,4.33796845864933,
4.35773918125188,4.39982416404737,4.47273269220943,4.74302592758338,4.75983300239487,
4.76359384413405,4.76572010237776,4.76735910887676,4.76948591241028,4.77314926725199,
4.78696847988592,4.98101737441762,5.16558161563544,5.17739938983049,5.18136180545413,
5.18358634300746,5.18561369847494,5.18832125489988,5.19335023114117,5.22035843894141,
5.27326045298571,5.37439563585434,5.58005860617515,5.59213481847676,5.59524968660384,
5.59704893669209,5.59843052497715,5.60021650589705,5.60335667618863,5.61705761770723,
5.82453883876432,5.94526275797642,5.95648364888428,5.96117372787941,5.96507992193408,
5.96908520114785,5.97494251292185,5.9902114594954,6.05778111991776,6.15317653689984,
6.31024172892292,6.33809154781145,6.34260962610404,6.34487979730575,6.34664863636598,
6.34859874066813,6.35177616355349,6.36274016658653,6.42827605828702,6.56235265701554,
6.67415497418702,6.73014367100642,6.73583202834632,6.738609749072,6.74059613447953,
6.74248140872586,6.74511666062975,6.75042338893551,6.79324536349012,6.86084017489016,
6.99643068922566,7.15077154268055,7.16090776949416,7.16309123406323,7.16449530997177,
7.16561334339644,7.1668708803443,7.16900483380658,7.1774837112125,7.24133518760423,
7.4142420867406,7.55314772555149,7.56263848752108,7.56600501203437,7.56794284305434,
7.56973853601016,7.57218130131141,7.57686556793127,7.5827171077293,7.62621886333501,
7.7110296962799,7.8001268369048,7.94979572261828,7.95921812197263,7.96157798184844,
7.96294671294924,7.96400069130473,7.96536633663348,7.96777628539521,7.97839266170175,
8.12768976201616,8.20684312721434,8.36689851981268,8.37731056456854,8.38098891766631,
8.38310250841461,8.38505880746532,8.38771669513652,8.39280244714941,8.42398018514736,
8.4915599645707,8.61424263812748,8.76856000716874,8.77924692897137,8.78281656317761,
8.78481647954515,8.78682098659246,8.78933484415522,8.79423906742558,8.82788074055006,
8.92027696197014,8.96427528803267,9.18571119328004,9.22174880095856,9.23263758814886,
9.2392874529066,9.24510470968616,9.25262605699279,9.26776789106154,9.28723466643923,
9.3323087500676,9.41267182213248,9.52825665043426,9.54078303159781,9.54490906369171,
9.54783292401341,9.55059148983615,9.55355318276258,9.55732613971713,9.56317466939706,
9.61292305907635,9.7696249262346,9.81517981302183,9.84510538447672,9.85650810045179,
9.86339513813875,9.87038522851126,9.87760419649299,9.88711035937725,9.91381911129815,
9.96048377331572),.UNSPECIFIED.);
#3543=B_SPLINE_CURVE_WITH_KNOTS('',3,(#221391,#221392,#221393,#221394,#221395,
#221396,#221397,#221398,#221399,#221400,#221401,#221402,#221403,#221404,
#221405,#221406,#221407,#221408,#221409,#221410,#221411,#221412,#221413,
#221414,#221415,#221416,#221417,#221418,#221419,#221420,#221421,#221422,
#221423,#221424,#221425,#221426,#221427,#221428,#221429,#221430,#221431,
#221432,#221433,#221434,#221435,#221436,#221437,#221438,#221439,#221440,
#221441,#221442,#221443,#221444,#221445,#221446,#221447,#221448,#221449,
#221450,#221451,#221452,#221453,#221454,#221455,#221456,#221457,#221458,
#221459,#221460,#221461,#221462,#221463,#221464,#221465,#221466,#221467,
#221468,#221469,#221470,#221471,#221472,#221473,#221474,#221475,#221476,
#221477,#221478,#221479,#221480,#221481,#221482,#221483,#221484,#221485,
#221486,#221487,#221488,#221489,#221490,#221491,#221492,#221493,#221494,
#221495,#221496,#221497,#221498,#221499,#221500,#221501,#221502,#221503,
#221504,#221505,#221506,#221507,#221508,#221509,#221510,#221511,#221512,
#221513,#221514,#221515,#221516,#221517,#221518,#221519,#221520,#221521,
#221522,#221523,#221524,#221525,#221526,#221527,#221528,#221529,#221530,
#221531,#221532,#221533,#221534,#221535,#221536,#221537,#221538,#221539,
#221540,#221541,#221542,#221543,#221544,#221545,#221546,#221547,#221548,
#221549,#221550,#221551,#221552,#221553,#221554,#221555,#221556,#221557,
#221558,#221559,#221560,#221561,#221562,#221563,#221564,#221565,#221566,
#221567,#221568,#221569,#221570,#221571,#221572,#221573,#221574,#221575,
#221576,#221577,#221578,#221579,#221580,#221581,#221582,#221583,#221584,
#221585,#221586,#221587,#221588,#221589,#221590,#221591,#221592,#221593,
#221594,#221595,#221596,#221597,#221598,#221599,#221600,#221601,#221602,
#221603,#221604,#221605,#221606,#221607,#221608,#221609,#221610,#221611,
#221612,#221613,#221614,#221615,#221616,#221617,#221618,#221619,#221620,
#221621,#221622,#221623,#221624,#221625,#221626,#221627,#221628,#221629,
#221630,#221631,#221632,#221633,#221634,#221635,#221636,#221637,#221638,
#221639,#221640,#221641,#221642,#221643,#221644,#221645,#221646,#221647,
#221648,#221649,#221650,#221651,#221652,#221653,#221654,#221655,#221656,
#221657,#221658,#221659,#221660,#221661,#221662,#221663,#221664,#221665,
#221666,#221667,#221668,#221669,#221670,#221671,#221672,#221673,#221674,
#221675,#221676,#221677,#221678,#221679,#221680,#221681,#221682,#221683,
#221684,#221685,#221686,#221687,#221688,#221689,#221690,#221691,#221692,
#221693,#221694,#221695,#221696,#221697,#221698,#221699,#221700,#221701,
#221702,#221703,#221704,#221705,#221706,#221707,#221708,#221709,#221710,
#221711,#221712,#221713,#221714,#221715,#221716,#221717,#221718,#221719,
#221720,#221721,#221722,#221723,#221724,#221725,#221726,#221727,#221728,
#221729,#221730,#221731,#221732,#221733,#221734,#221735,#221736,#221737,
#221738,#221739,#221740,#221741,#221742,#221743,#221744,#221745,#221746,
#221747,#221748,#221749,#221750,#221751,#221752,#221753,#221754,#221755,
#221756,#221757,#221758,#221759,#221760,#221761,#221762,#221763,#221764,
#221765,#221766,#221767,#221768,#221769,#221770,#221771,#221772,#221773,
#221774,#221775,#221776,#221777,#221778,#221779,#221780,#221781,#221782,
#221783,#221784,#221785,#221786,#221787,#221788,#221789,#221790,#221791,
#221792,#221793,#221794,#221795,#221796,#221797,#221798,#221799,#221800,
#221801,#221802,#221803,#221804,#221805,#221806,#221807,#221808,#221809,
#221810,#221811,#221812,#221813,#221814,#221815,#221816,#221817,#221818,
#221819,#221820,#221821,#221822,#221823,#221824,#221825,#221826,#221827,
#221828,#221829,#221830,#221831,#221832,#221833,#221834,#221835,#221836,
#221837,#221838,#221839,#221840,#221841,#221842,#221843,#221844,#221845,
#221846,#221847,#221848,#221849,#221850,#221851,#221852,#221853,#221854,
#221855,#221856,#221857,#221858,#221859,#221860,#221861,#221862,#221863,
#221864,#221865,#221866,#221867,#221868,#221869,#221870,#221871,#221872,
#221873,#221874,#221875,#221876,#221877,#221878,#221879,#221880,#221881,
#221882,#221883,#221884,#221885,#221886,#221887,#221888,#221889,#221890,
#221891,#221892,#221893,#221894,#221895,#221896,#221897,#221898,#221899,
#221900,#221901,#221902,#221903,#221904,#221905,#221906,#221907,#221908,
#221909,#221910,#221911,#221912,#221913,#221914,#221915,#221916,#221917,
#221918,#221919,#221920,#221921,#221922,#221923,#221924,#221925,#221926,
#221927,#221928,#221929,#221930,#221931,#221932,#221933,#221934,#221935,
#221936,#221937,#221938,#221939,#221940,#221941,#221942,#221943,#221944,
#221945,#221946,#221947,#221948,#221949,#221950,#221951,#221952,#221953,
#221954,#221955,#221956,#221957,#221958,#221959,#221960,#221961,#221962,
#221963,#221964,#221965,#221966,#221967,#221968,#221969,#221970,#221971,
#221972,#221973,#221974,#221975,#221976,#221977,#221978,#221979,#221980,
#221981,#221982,#221983,#221984,#221985,#221986,#221987,#221988,#221989,
#221990,#221991,#221992,#221993,#221994,#221995,#221996,#221997,#221998,
#221999,#222000,#222001,#222002,#222003,#222004),.UNSPECIFIED.,.F.,.F.,
(4,2,2,2,2,2,2,2,2,2,2,2,2,2,2,2,2,2,2,2,2,2,2,2,2,2,2,2,2,2,2,2,2,2,2,
2,2,2,2,2,2,2,2,2,2,2,2,2,2,2,2,2,2,2,2,2,2,2,2,2,2,2,2,2,2,2,2,2,2,2,2,
2,2,2,2,2,2,2,2,2,2,2,2,2,2,2,2,2,2,2,2,2,2,2,2,2,2,2,2,2,2,2,2,2,2,2,2,
2,2,2,2,2,2,2,2,2,2,2,2,2,2,2,2,2,2,2,2,2,2,2,2,2,2,2,2,2,2,2,2,2,2,2,2,
2,2,2,2,2,2,2,2,2,2,2,2,2,2,2,2,2,2,2,2,2,2,2,2,2,2,2,2,2,2,2,2,2,2,2,2,
2,2,2,2,2,2,2,2,2,2,2,2,2,2,2,2,2,2,2,2,2,2,2,2,2,2,2,2,2,2,2,2,2,2,2,2,
2,2,2,2,2,2,2,2,2,2,2,2,2,2,2,2,2,2,2,2,2,2,2,2,2,2,2,2,2,2,2,2,2,2,2,2,
2,2,2,2,2,2,2,2,2,2,2,2,2,2,2,2,2,2,2,2,2,2,2,2,2,2,2,2,2,2,2,2,2,2,2,2,
2,2,2,2,2,2,2,2,2,2,2,2,2,2,2,2,2,2,2,4),(0.00200445933661479,0.257562155059745,
0.316274882700235,0.341574413126625,0.345807148728994,0.348035012614877,
0.349857302511951,0.351960882756546,0.355526363625104,0.368395116683556,
0.532759139362108,0.574442149897183,0.587286486297553,0.605148138983943,
0.754921073955549,0.761703681846437,0.764761431261892,0.767046088233661,
0.769179874062017,0.772112168996419,0.77951926167843,0.869020137795594,
0.980654931082344,1.03865010382674,1.09909585660219,1.16491261869436,1.174708423841,
1.17750808782124,1.17921780549224,1.18076294359186,1.18273806958325,1.18664293058622,
1.20997057423235,1.21825303911419,1.22820064143878,1.22891386269151,1.41087196010116,
1.49061553569335,1.51758453081015,1.5357313333722,1.54192029068296,1.54595627159197,
1.54595733660975,1.5459584021784,1.54595946731916,1.54596053185663,1.54596159731891,
1.54596266374587,1.54596372973979,1.54596479547363,1.54596586141477,1.54596692798112,
1.54596799433288,1.54596906087551,1.54597012751087,1.54597119404546,1.54597226001324,
1.54597332620561,1.54597439292839,1.54597545926682,1.54597652562873,1.54597759221494,
1.54597865941157,1.54597972675294,1.54598079418779,1.54598186128828,1.54598292821321,
1.54598399556114,1.54598506284928,1.54598613069444,1.54598719933944,1.54598826766137,
1.54598933534996,1.54599040346131,1.54599147178244,1.54599253971556,1.54599360756868,
1.54599467601479,1.54987863171109,1.55501595061203,1.56379944330618,1.61386156826146,
1.83972786939599,1.90262466217746,1.92115777257303,1.92493877921191,1.92702228319894,
1.9286036212427,1.93036054009782,1.93355146565727,1.94349208004349,2.08120188211125,
2.23710547049427,2.28741975754036,2.31430639676666,2.31904113969932,2.32155689427955,
2.32342617853064,2.32546296550913,2.32905272656481,2.33950108669311,2.49832925086366,
2.63556079002027,2.74038932741481,2.74415769859847,2.74574654320756,2.74689225997345,
2.74793344460349,2.74932520104005,2.75202811306479,2.77227766855203,2.90679891325944,
3.0269351401939,3.07846506811425,3.13959144144883,3.1455196358291,3.14820849671315,
3.15022402602026,3.15211111284459,3.15471159111842,3.1613176581111,3.24196515857597,
3.27392709476174,3.43861951918611,3.53831774259555,3.54206117452088,3.54368869580022,
3.54488558796346,3.54598989922357,3.54748650815047,3.55115893198215,3.58835073661744,
3.68457627658784,3.84868505509515,3.91309732211954,3.95517812542462,3.96064453750795,
3.96338093778996,3.96534721200938,3.96742693740111,3.97034823442838,3.9763728402556,
4.03829248779477,4.18429186786753,4.34445851041227,4.35963643615124,4.36353239791952,
4.36582793083678,4.36785097408873,4.37036912336293,4.37424826947605,4.39183838641528,
4.40168267924723,4.4327367824747,4.52799371074605,4.70253413940462,4.76759391394344,
4.80334573141613,4.81380397408981,4.82035831299367,4.82642317567252,4.8342774424765,
4.84737840414369,4.98102876442705,5.0499437550147,5.11638298519625,5.12379022516316,
5.12750540482588,5.13054181913247,5.13404722512841,5.14015740530248,5.16662221891198,
5.2207413622884,5.35939993422906,5.37365096605442,5.42130155451077,5.43486760685969,
5.44298825593349,5.44954266096578,5.45847977156309,5.47597232963744,5.57571399612995,
5.65099074577087,5.85357165165343,5.87975480239824,5.88389122758383,5.88632991175477,
5.88818265097178,5.89014852572189,5.89319123313548,5.90238176234558,5.95012347399396,
5.9816168363335,6.28201837390373,6.29802224606703,6.3024324409306,6.30502929367345,
6.30727576369897,6.31001787852728,6.31521278893304,6.34562842023349,6.40155217281647,
6.55976297581316,6.70497822124924,6.71399837732852,6.71683027724222,6.71837489961005,
6.71987976775037,6.72170012714423,6.72366296325356,6.72674218300685,6.73261116721234,
6.94462507295509,7.06632597099788,7.07755306653769,7.08224264953312,7.08614712579224,
7.09014930679843,7.09599962392249,7.11123780317845,7.17860846332306,7.27279030415763,
7.43568959212578,7.45931710530968,7.46323200104254,7.465562003216,7.4673077930834,
7.46916324122535,7.47199502299718,7.47525928277452,7.48123821805066,7.52863975413416,
7.56006660705792,7.83951581558997,7.85476455496277,7.85887944735428,7.86128356957373,
7.86335181254644,7.86586196120119,7.8705740931098,7.89702611390657,7.94551986511262,
7.98887676023074,8.01590077986302,8.03732487544955,8.18257536128988,8.20979173530086,
8.21389035885154,8.27890476410037,8.28299653005717,8.28451921441541,8.28559532550958,
8.28660634317125,8.28768145338652,8.28996704928214,8.30051906358285,8.32039596883359,
8.37608838564092,8.43872892097657,8.52236232126092,8.67275158479116,8.68269592280739,
8.68612593590125,8.68807542390742,8.68986659730358,8.69228019292654,8.69683233013144,
8.72291130557021,8.76231548052929,8.83262914957418,8.85260257459218,8.86903421769268,
8.88290461776496,8.89480487674223,8.90512905407852,8.98816205325646,9.07463893131991,
9.07989220957653,9.08180749768764,9.08293660622949,9.08400010448483,9.08513543316742,
9.08657462669668,9.09206338453848,9.10031640289146,9.12479578442805,9.19883708865226,
9.47824368637398,9.49557089306043,9.50000519443093,9.50254759244992,9.50449034737361,
9.50698979746876,9.51135164416166,9.52989600276192,9.70504086677498,9.85628699878259,
9.86637980922595,9.89599042482016,9.90106993892853,9.90365431863312,9.90560914742451,
9.90750818051455,9.90970720603225,9.91283938594869,9.9182320202591,9.95798028600589),
 .UNSPECIFIED.);
#3544=B_SPLINE_CURVE_WITH_KNOTS('',3,(#222006,#222007,#222008,#222009,#222010,
#222011,#222012,#222013,#222014,#222015,#222016,#222017,#222018),
 .UNSPECIFIED.,.F.,.F.,(4,1,1,1,1,1,1,1,1,1,4),(151.920096078454,152.307809718983,
152.807179586914,153.306549454845,153.805919322776,154.804659058638,155.30402892657,
155.803398794501,156.802138530363,157.800878266225,158.203281385634),
 .UNSPECIFIED.);
#3545=B_SPLINE_CURVE_WITH_KNOTS('',3,(#222020,#222021,#222022,#222023,#222024,
#222025,#222026,#222027,#222028,#222029,#222030,#222031,#222032,#222033,
#222034,#222035,#222036,#222037),.UNSPECIFIED.,.F.,.F.,(4,2,2,2,2,2,2,2,
4),(158.203281385634,159.038198297529,159.873115209424,160.708032121318,
161.542949033213,162.377865945108,163.212782857003,164.047699768898,164.486466692813),
 .UNSPECIFIED.);
#3546=B_SPLINE_CURVE_WITH_KNOTS('',3,(#222039,#222040,#222041,#222042,#222043,
#222044,#222045,#222046,#222047,#222048,#222049,#222050,#222051),
 .UNSPECIFIED.,.F.,.F.,(4,1,1,1,1,1,1,1,1,1,4),(164.486466692813,164.79205641726,
165.790796153122,166.290166021054,166.789535888985,167.288905756916,167.788275624847,
168.787015360709,169.28638522864,169.785755096571,170.769649602841),
 .UNSPECIFIED.);
#3547=B_SPLINE_CURVE_WITH_KNOTS('',3,(#222053,#222054,#222055,#222056,#222057,
#222058,#222059,#222060,#222061,#222062,#222063,#222064,#222065,#222066,
#222067,#222068,#222069,#222070,#222071,#222072,#222073,#222074,#222075,
#222076,#222077,#222078,#222079,#222080,#222081,#222082,#222083,#222084,
#222085,#222086,#222087,#222088,#222089,#222090,#222091,#222092,#222093,
#222094,#222095,#222096,#222097,#222098,#222099,#222100,#222101,#222102,
#222103,#222104,#222105,#222106,#222107,#222108,#222109,#222110,#222111,
#222112,#222113,#222114,#222115,#222116,#222117,#222118,#222119,#222120,
#222121,#222122,#222123,#222124,#222125,#222126,#222127,#222128,#222129,
#222130,#222131,#222132,#222133,#222134,#222135,#222136,#222137,#222138,
#222139,#222140,#222141,#222142,#222143,#222144,#222145,#222146,#222147,
#222148,#222149,#222150,#222151,#222152,#222153,#222154,#222155,#222156,
#222157,#222158,#222159,#222160,#222161,#222162,#222163,#222164,#222165,
#222166,#222167,#222168,#222169,#222170,#222171,#222172,#222173,#222174,
#222175,#222176,#222177,#222178,#222179,#222180,#222181,#222182,#222183,
#222184,#222185,#222186,#222187,#222188,#222189,#222190,#222191,#222192,
#222193,#222194,#222195,#222196,#222197,#222198,#222199,#222200,#222201,
#222202,#222203,#222204,#222205,#222206,#222207,#222208,#222209,#222210,
#222211,#222212,#222213,#222214,#222215,#222216,#222217,#222218,#222219,
#222220,#222221,#222222,#222223,#222224,#222225,#222226,#222227,#222228,
#222229,#222230,#222231,#222232,#222233,#222234,#222235,#222236,#222237,
#222238,#222239,#222240,#222241,#222242,#222243,#222244,#222245,#222246,
#222247,#222248,#222249,#222250,#222251,#222252,#222253,#222254,#222255,
#222256,#222257,#222258,#222259,#222260,#222261,#222262,#222263,#222264,
#222265,#222266,#222267,#222268,#222269,#222270,#222271,#222272,#222273,
#222274,#222275,#222276,#222277,#222278,#222279,#222280,#222281,#222282,
#222283,#222284,#222285,#222286,#222287,#222288,#222289,#222290,#222291,
#222292,#222293,#222294,#222295,#222296,#222297,#222298,#222299,#222300,
#222301,#222302,#222303,#222304,#222305,#222306,#222307,#222308,#222309,
#222310,#222311,#222312,#222313,#222314),.UNSPECIFIED.,.F.,.F.,(4,3,3,3,
3,3,3,3,3,3,3,3,3,3,3,3,3,3,3,3,3,3,3,3,3,3,3,3,3,3,3,3,3,3,3,3,3,3,3,3,
3,3,3,3,3,3,3,3,3,3,3,3,3,3,3,3,3,3,3,3,3,3,3,3,3,3,3,3,3,3,3,3,3,3,3,3,
3,3,3,3,3,3,3,3,3,3,3,4),(170.769651999993,170.784494832433,170.857633776118,
170.930684693425,171.003662517447,171.076582111962,171.149458286939,171.22230581252,
171.29515330968,171.368004458218,171.440872607319,171.513771117372,171.586756558935,
171.659789371711,171.732933795829,171.783234568296,171.858762856963,171.934205052296,
172.009574059991,172.084882737954,172.160143904354,172.23787270433,172.313082901655,
172.388287126354,172.463496936619,172.538723891604,172.614006781214,172.689322828085,
172.764709737342,172.781974304158,172.858566204559,172.935092906499,173.011564102391,
173.087980962652,173.164365001485,173.240725164898,173.281344172089,173.359463440568,
173.437627744043,173.515841821031,173.594146943719,173.672500370318,173.750939460084,
173.78071404002,173.862692818607,173.944599567848,174.028470652873,174.110136065388,
174.195109986669,174.280083907951,174.353695582057,174.42730194891,174.500916000811,
174.57458229334,174.648275821364,174.722051294429,174.779453775882,174.855954500688,
174.932399267869,175.008798987449,175.085164537056,175.161506769247,175.238592612059,
175.314934425435,175.391286513078,175.467658737185,175.545292430825,175.621764107818,
175.699978809781,175.778193511744,175.852875326433,175.927477178584,176.002011462157,
176.076480019692,176.150910235284,176.225315147085,176.277563379675,176.357860628097,
176.438303101,176.522960637651,176.603740784067,176.684622295,176.765639095402,
176.776933247606,176.864827893909,176.952337296125,177.039186513869,177.052837150721),
 .UNSPECIFIED.);
#3548=B_SPLINE_CURVE_WITH_KNOTS('',3,(#222316,#222317,#222318,#222319,#222320,
#222321,#222322,#222323,#222324,#222325,#222326,#222327,#222328),
 .UNSPECIFIED.,.F.,.F.,(4,1,1,1,1,1,1,1,1,1,4),(177.052837307173,177.775672983469,
178.774412719331,179.773152455193,180.272522323124,180.771892191055,181.271262058986,
181.770631926917,182.76937166278,183.268741530711,183.336022614352),
 .UNSPECIFIED.);
#3549=B_SPLINE_CURVE_WITH_KNOTS('',3,(#222330,#222331,#222332,#222333,#222334,
#222335,#222336,#222337,#222338,#222339,#222340,#222341,#222342,#222343,
#222344,#222345,#222346,#222347,#222348,#222349,#222350,#222351,#222352,
#222353,#222354,#222355,#222356,#222357,#222358,#222359,#222360,#222361,
#222362,#222363,#222364,#222365,#222366,#222367,#222368,#222369,#222370,
#222371,#222372,#222373,#222374,#222375,#222376,#222377,#222378,#222379,
#222380,#222381,#222382,#222383,#222384,#222385,#222386,#222387,#222388,
#222389,#222390,#222391,#222392,#222393,#222394,#222395,#222396,#222397,
#222398,#222399,#222400,#222401,#222402,#222403,#222404,#222405,#222406,
#222407,#222408,#222409,#222410,#222411,#222412,#222413,#222414,#222415,
#222416,#222417,#222418,#222419,#222420,#222421,#222422,#222423,#222424,
#222425,#222426,#222427,#222428,#222429,#222430,#222431,#222432,#222433,
#222434,#222435,#222436,#222437,#222438,#222439,#222440,#222441,#222442,
#222443,#222444,#222445,#222446,#222447,#222448,#222449,#222450,#222451,
#222452,#222453,#222454,#222455,#222456,#222457,#222458,#222459,#222460,
#222461,#222462,#222463,#222464,#222465,#222466,#222467,#222468,#222469,
#222470,#222471,#222472,#222473,#222474,#222475,#222476,#222477,#222478,
#222479,#222480,#222481,#222482,#222483,#222484,#222485,#222486,#222487,
#222488,#222489,#222490,#222491,#222492,#222493,#222494,#222495,#222496,
#222497,#222498,#222499,#222500,#222501,#222502,#222503,#222504,#222505,
#222506,#222507,#222508,#222509,#222510,#222511,#222512,#222513,#222514,
#222515,#222516,#222517,#222518,#222519,#222520,#222521,#222522,#222523,
#222524,#222525,#222526,#222527,#222528,#222529,#222530,#222531,#222532,
#222533,#222534,#222535,#222536,#222537,#222538,#222539,#222540,#222541,
#222542,#222543,#222544,#222545,#222546,#222547,#222548,#222549,#222550,
#222551,#222552,#222553,#222554,#222555,#222556,#222557,#222558,#222559,
#222560,#222561,#222562,#222563,#222564,#222565,#222566,#222567,#222568,
#222569,#222570,#222571,#222572,#222573,#222574,#222575,#222576,#222577,
#222578,#222579,#222580,#222581,#222582,#222583,#222584,#222585,#222586,
#222587,#222588,#222589,#222590,#222591),.UNSPECIFIED.,.F.,.F.,(4,3,3,3,
3,3,3,3,3,3,3,3,3,3,3,3,3,3,3,3,3,3,3,3,3,3,3,3,3,3,3,3,3,3,3,3,3,3,3,3,
3,3,3,3,3,3,3,3,3,3,3,3,3,3,3,3,3,3,3,3,3,3,3,3,3,3,3,3,3,3,3,3,3,3,3,3,
3,3,3,3,3,3,3,3,3,3,3,4),(183.336022710285,183.418369237534,183.500946924274,
183.583821518175,183.666843220968,183.750041231153,183.768111398642,183.842640868417,
183.917094196739,183.9914852864,184.065827999059,184.14013616408,184.214423587004,
184.288719132779,184.363023638853,184.43734960221,184.511709528832,184.586155211748,
184.66065006493,184.735247010616,184.766851134504,184.839990078184,184.913040995486,
184.986018819503,185.058938414014,185.131814588985,185.204662114563,185.277509611718,
185.350360760251,185.423228909348,185.496127419396,185.569112860954,185.642145673725,
185.715290097839,185.765590870366,185.841119159016,185.916561354331,185.991930362009,
186.067239039954,186.142500206338,186.220229006324,186.295439203632,186.370643428313,
186.445853238561,186.52108019353,186.596363083123,186.671679129978,186.747066039219,
186.764330606228,186.840922506793,186.917449208897,186.993920404951,187.070337265371,
187.146721304362,187.223081467929,187.263700474159,187.341819742201,187.419984045232,
187.498198121775,187.576503244015,187.654856670165,187.733295759485,187.763070342091,
187.845049121599,187.926955871758,188.010826956324,188.092492369716,188.177466289869,
188.262440210022,188.336051883564,188.40965824985,188.483272301184,188.556938593144,
188.630632120597,188.704407593094,188.761810077953,188.83712615777,188.912381635905,
188.987589440095,189.066503531416,189.141660684109,189.216812290113,189.291970005769,
189.367145488611,189.442379450268,189.517647220403,189.592990271303,189.61890217066),
 .UNSPECIFIED.);
#3550=B_SPLINE_CURVE_WITH_KNOTS('',3,(#222593,#222594,#222595,#222596,#222597,
#222598,#222599,#222600,#222601,#222602,#222603,#222604,#222605,#222606,
#222607,#222608,#222609,#222610,#222611,#222612,#222613,#222614,#222615,
#222616,#222617,#222618,#222619,#222620,#222621,#222622,#222623,#222624,
#222625,#222626,#222627,#222628,#222629,#222630,#222631,#222632,#222633,
#222634,#222635,#222636,#222637,#222638,#222639,#222640,#222641,#222642,
#222643,#222644,#222645,#222646,#222647,#222648,#222649,#222650,#222651,
#222652,#222653,#222654,#222655,#222656,#222657,#222658,#222659,#222660,
#222661,#222662,#222663,#222664,#222665,#222666,#222667,#222668,#222669,
#222670,#222671,#222672,#222673,#222674,#222675,#222676,#222677,#222678,
#222679,#222680,#222681,#222682,#222683,#222684,#222685,#222686,#222687,
#222688,#222689,#222690,#222691,#222692,#222693,#222694,#222695,#222696,
#222697,#222698,#222699,#222700,#222701,#222702,#222703,#222704,#222705,
#222706,#222707,#222708,#222709,#222710,#222711,#222712,#222713,#222714,
#222715,#222716,#222717,#222718,#222719,#222720,#222721,#222722,#222723,
#222724,#222725,#222726,#222727,#222728,#222729,#222730,#222731,#222732,
#222733,#222734,#222735,#222736,#222737,#222738,#222739,#222740,#222741,
#222742,#222743,#222744,#222745,#222746,#222747,#222748,#222749,#222750,
#222751,#222752,#222753,#222754,#222755,#222756,#222757,#222758,#222759,
#222760,#222761,#222762,#222763,#222764,#222765,#222766,#222767,#222768,
#222769,#222770,#222771,#222772,#222773,#222774,#222775,#222776,#222777,
#222778,#222779,#222780,#222781,#222782,#222783,#222784,#222785,#222786,
#222787,#222788,#222789,#222790,#222791,#222792,#222793,#222794,#222795,
#222796,#222797,#222798,#222799,#222800,#222801,#222802,#222803,#222804,
#222805,#222806,#222807,#222808,#222809,#222810,#222811,#222812,#222813,
#222814,#222815,#222816,#222817,#222818,#222819,#222820,#222821,#222822,
#222823,#222824,#222825,#222826,#222827,#222828,#222829,#222830,#222831,
#222832,#222833,#222834,#222835,#222836,#222837,#222838,#222839,#222840,
#222841,#222842,#222843,#222844,#222845,#222846,#222847,#222848,#222849,
#222850,#222851,#222852,#222853,#222854,#222855,#222856,#222857,#222858,
#222859,#222860,#222861,#222862,#222863,#222864,#222865,#222866,#222867,
#222868,#222869,#222870,#222871,#222872,#222873,#222874,#222875,#222876,
#222877,#222878,#222879,#222880,#222881,#222882,#222883,#222884,#222885,
#222886,#222887,#222888,#222889,#222890,#222891,#222892,#222893,#222894,
#222895,#222896,#222897,#222898,#222899,#222900,#222901,#222902,#222903,
#222904,#222905,#222906,#222907,#222908,#222909,#222910,#222911,#222912,
#222913,#222914,#222915,#222916,#222917,#222918,#222919,#222920,#222921,
#222922,#222923,#222924,#222925,#222926,#222927,#222928,#222929,#222930,
#222931,#222932,#222933,#222934,#222935,#222936,#222937,#222938,#222939,
#222940,#222941,#222942,#222943,#222944,#222945,#222946,#222947,#222948,
#222949,#222950,#222951,#222952,#222953,#222954,#222955,#222956,#222957,
#222958,#222959,#222960,#222961,#222962,#222963,#222964,#222965,#222966,
#222967,#222968,#222969,#222970,#222971,#222972,#222973,#222974,#222975,
#222976,#222977,#222978,#222979,#222980,#222981,#222982,#222983,#222984,
#222985,#222986,#222987,#222988,#222989,#222990,#222991,#222992,#222993,
#222994,#222995,#222996,#222997,#222998,#222999,#223000,#223001,#223002,
#223003,#223004,#223005,#223006,#223007,#223008,#223009,#223010,#223011,
#223012,#223013,#223014,#223015,#223016,#223017,#223018,#223019,#223020,
#223021,#223022,#223023,#223024,#223025,#223026,#223027,#223028,#223029,
#223030,#223031,#223032,#223033,#223034,#223035,#223036,#223037,#223038,
#223039,#223040,#223041,#223042,#223043,#223044,#223045,#223046,#223047,
#223048,#223049,#223050,#223051,#223052,#223053,#223054,#223055,#223056,
#223057,#223058,#223059,#223060,#223061,#223062,#223063,#223064,#223065,
#223066,#223067,#223068,#223069,#223070,#223071,#223072,#223073,#223074,
#223075,#223076,#223077,#223078,#223079,#223080,#223081,#223082,#223083,
#223084,#223085,#223086,#223087,#223088,#223089,#223090,#223091,#223092,
#223093,#223094,#223095,#223096,#223097,#223098,#223099,#223100,#223101,
#223102,#223103,#223104,#223105,#223106,#223107,#223108,#223109,#223110,
#223111,#223112,#223113,#223114,#223115,#223116,#223117,#223118,#223119,
#223120,#223121,#223122,#223123,#223124,#223125,#223126,#223127,#223128,
#223129,#223130,#223131,#223132,#223133,#223134),.UNSPECIFIED.,.F.,.F.,
(4,2,2,2,2,2,2,2,2,2,2,2,2,2,2,2,2,2,2,2,2,2,2,2,2,2,2,2,2,2,2,2,2,2,2,
2,2,2,2,2,2,2,2,2,2,2,2,2,2,2,2,2,2,2,2,2,2,2,2,2,2,2,2,2,2,2,2,2,2,2,2,
2,2,2,2,2,2,2,2,2,2,2,2,2,2,2,2,2,2,2,2,2,2,2,2,2,2,2,2,2,2,2,2,2,2,2,2,
2,2,2,2,2,2,2,2,2,2,2,2,2,2,2,2,2,2,2,2,2,2,2,2,2,2,2,2,2,2,2,2,2,2,2,2,
2,2,2,2,2,2,2,2,2,2,2,2,2,2,2,2,2,2,2,2,2,2,2,2,2,2,2,2,2,2,2,2,2,2,2,2,
2,2,2,2,2,2,2,2,2,2,2,2,2,2,2,2,2,2,2,2,2,2,2,2,2,2,2,2,2,2,2,2,2,2,2,2,
2,2,2,2,2,2,2,2,2,2,2,2,2,2,2,2,2,2,2,2,2,2,2,2,2,2,2,2,2,2,2,2,2,2,2,2,
2,2,2,2,2,2,2,2,2,2,2,2,2,2,2,2,2,2,2,4),(0.00141478209296347,0.116359404994446,
0.120713596378298,0.123214540612478,0.124937161336518,0.126623797141894,
0.128174337153862,0.130160235713197,0.133408934317356,0.150951991650534,
0.155749334295669,0.272937339542111,0.298978788255001,0.321770711377344,
0.373371119871339,0.473387650117704,0.481487790296529,0.486559257208962,
0.491316542452597,0.49477628650431,0.498478450251031,0.503759688630404,
0.514873934986964,0.704474471907343,0.773461894469543,0.837295790827264,
0.857270300442468,0.865073774911546,0.870679413777046,0.872621998411138,
0.874523090099118,0.876306419379916,0.878640993518927,0.882561907340408,
0.906034300954475,0.92741173681054,0.98542029462302,1.07896996220131,1.0912915984963,
1.10580264940794,1.12324718155251,1.18374223683944,1.23415143619826,1.2610063247466,
1.2657386548023,1.26825351019186,1.27032248806344,1.27272390408731,1.27682541294864,
1.29193252202704,1.50928071719468,1.60323321708623,1.64914433952348,1.6758190985247,
1.68908655310731,1.69157661288434,1.69291822518187,1.69402096091606,1.69531990823265,
1.69758797984725,1.70662127054167,1.84562906207161,1.99180643756179,2.02136389862685,
2.08005241041187,2.09060325162782,2.09398519473297,2.09614101616721,2.09815177665687,
2.10076760202711,2.1051294183366,2.11465336865836,2.292862221828,2.3977452646824,
2.44254255592615,2.47225966332362,2.48673261002166,2.48932521246531,2.49073025657572,
2.49188960883048,2.49308054306052,2.49530111103813,2.50268360430771,2.61449783213889,
2.7566490473711,2.89395538917891,2.90503701291405,2.90867091643284,2.91100878839675,
2.91320465382772,2.91608342247698,2.92243975105969,2.97355239232443,3.16934045245947,
3.24744999612144,3.27781382061395,3.30484355193634,3.30949127761645,3.31195107996309,
3.31397015828103,3.31600574299151,3.31974731734248,3.33181692527709,3.34186054006806,
3.34415719894622,3.4563422381925,3.63615425134901,3.74346699886949,3.75751928689668,
3.76484696221741,3.77026154518949,3.77615064600599,3.78655948072165,3.81795239455225,
3.98709659398994,4.04062311540851,4.06610994909314,4.07170786820321,4.07508129434783,
4.07813676821402,4.08205623412285,4.09014136897172,4.19101267416699,4.20490129226199,
4.3239442090558,4.35380498803724,4.37607020609286,4.38592139102362,4.39328217418404,
4.40019654021417,4.40982546353891,4.43558488579211,4.60938192688126,4.74921468486974,
4.8032303827859,4.82707226094502,4.83123819953745,4.83345169580967,4.8350963443329,
4.83688866530264,4.8400499951728,4.8492586136554,4.978535670744,5.22735475449493,
5.24420123961521,5.24869788283818,5.25131508635557,5.253539201544,5.25624796656749,
5.26128571005427,5.28848866018707,5.34178805470377,5.44519511585523,5.64808449119481,
5.65992105371258,5.6630140562037,5.66480781563575,5.6661890288924,5.66797909911986,
5.67113967557324,5.68513168809714,5.89233576998291,6.01287253798258,6.02408704939539,
6.02877483801351,6.03267928157106,6.0366829260164,6.0425381396563,6.05780290066231,
6.12536105281249,6.22081382715594,6.37722499988755,6.3920553984691,6.4069658588054,
6.41031449931962,6.41249742674544,6.41425639358635,6.41625762668003,6.41966626074085,
6.43306718102309,6.58931404627895,6.74184465204506,6.797563147668,6.80324253650551,
6.80601751036979,6.80800268087551,6.81009680096605,6.81284658402001,6.81873791247382,
6.89618879935492,7.04940887811756,7.21756355456425,7.22814829856036,7.23036541799864,
7.23177967345,7.23289843764632,7.23414906003042,7.23625205251837,7.24437958209808,
7.30285732956871,7.39807710413337,7.51015359261545,7.55692041408943,7.62447342919497,
7.63079653751478,7.63334877150556,7.63522348075787,7.63724733996519,7.63998498760219,
7.64299607044376,7.64810472380772,7.77661672313094,7.8610655066267,7.98791079850766,
8.02415904802625,8.02738635517798,8.02895612160769,8.03007940539563,8.03114582313132,
8.03263687473307,8.035639404262,8.05965302495922,8.12792990748607,8.26577714132999,
8.36364883022773,8.43834150360216,8.445243363526,8.44802604776885,8.45006898643234,
8.45227351423497,8.45525394017297,8.46199005889707,8.58455271122478,8.67493242463407,
8.83445073387878,8.84560930882574,8.84923788364449,8.85124750205198,8.85326589689574,
8.85575948249289,8.86057839100535,8.89201458938135,8.93912520555978,8.99940659501446,
9.04418114539806,9.2686714225183,9.29097838796148,9.29912743532482,9.30489584624313,
9.31082684438023,9.3152613209626,9.32229933418327,9.33286062879409,9.35205256135841,
9.39623637984588,9.59476159566194,9.60691808190879,9.61096430385776,9.61383759255424,
9.61655847052943,9.61948173177422,9.62321636905001,9.62901963608366,9.68950152708124,
9.88048070961918,9.91187820042959,9.92332779106643,9.93010636852422,9.93696233355684,
9.94394595622972,9.95697286124426),.UNSPECIFIED.);
#3551=B_SPLINE_CURVE_WITH_KNOTS('',3,(#223136,#223137,#223138,#223139,#223140,
#223141,#223142,#223143,#223144,#223145,#223146,#223147,#223148,#223149,
#223150,#223151,#223152,#223153),.UNSPECIFIED.,.F.,.F.,(4,2,2,2,2,2,2,2,
4),(202.185578535891,203.020495447786,203.855412359681,204.690329271575,
205.52524618347,206.360163095365,207.19508000726,208.029996919155,208.46876384307),
 .UNSPECIFIED.);
#3552=B_SPLINE_CURVE_WITH_KNOTS('',3,(#223155,#223156,#223157,#223158,#223159,
#223160,#223161,#223162,#223163,#223164,#223165,#223166,#223167,#223168,
#223169,#223170,#223171,#223172,#223173,#223174,#223175,#223176,#223177,
#223178,#223179,#223180,#223181,#223182,#223183,#223184,#223185,#223186,
#223187,#223188,#223189,#223190,#223191,#223192,#223193,#223194,#223195,
#223196,#223197,#223198,#223199,#223200,#223201,#223202,#223203,#223204,
#223205,#223206,#223207,#223208,#223209,#223210,#223211,#223212,#223213,
#223214,#223215,#223216,#223217,#223218,#223219,#223220,#223221,#223222,
#223223,#223224,#223225,#223226,#223227,#223228,#223229,#223230,#223231,
#223232,#223233,#223234,#223235,#223236,#223237,#223238,#223239,#223240,
#223241,#223242,#223243,#223244,#223245,#223246,#223247,#223248,#223249,
#223250,#223251,#223252,#223253,#223254,#223255,#223256,#223257,#223258,
#223259,#223260,#223261,#223262,#223263,#223264,#223265,#223266,#223267,
#223268,#223269,#223270,#223271,#223272,#223273,#223274,#223275,#223276,
#223277,#223278,#223279,#223280,#223281,#223282,#223283,#223284,#223285,
#223286,#223287,#223288,#223289,#223290,#223291,#223292,#223293,#223294,
#223295,#223296,#223297,#223298,#223299,#223300,#223301,#223302,#223303,
#223304,#223305,#223306,#223307,#223308,#223309,#223310,#223311,#223312,
#223313,#223314,#223315,#223316,#223317,#223318,#223319,#223320,#223321,
#223322,#223323,#223324,#223325,#223326,#223327,#223328,#223329,#223330,
#223331,#223332,#223333,#223334,#223335,#223336,#223337,#223338,#223339,
#223340,#223341,#223342,#223343,#223344,#223345,#223346,#223347,#223348,
#223349,#223350,#223351,#223352,#223353,#223354,#223355,#223356,#223357,
#223358,#223359,#223360,#223361,#223362,#223363,#223364,#223365,#223366,
#223367,#223368,#223369,#223370,#223371,#223372,#223373,#223374,#223375,
#223376,#223377,#223378,#223379,#223380,#223381,#223382,#223383,#223384,
#223385,#223386,#223387,#223388,#223389,#223390,#223391,#223392,#223393,
#223394,#223395,#223396,#223397,#223398,#223399,#223400,#223401,#223402,
#223403,#223404,#223405,#223406,#223407,#223408,#223409,#223410,#223411,
#223412,#223413,#223414,#223415,#223416,#223417,#223418,#223419,#223420,
#223421,#223422,#223423,#223424,#223425,#223426,#223427,#223428,#223429,
#223430,#223431,#223432,#223433,#223434,#223435,#223436,#223437,#223438,
#223439,#223440,#223441,#223442,#223443,#223444,#223445,#223446,#223447,
#223448,#223449,#223450,#223451,#223452,#223453,#223454,#223455,#223456,
#223457,#223458,#223459,#223460,#223461,#223462,#223463,#223464,#223465,
#223466,#223467,#223468,#223469,#223470,#223471,#223472,#223473,#223474,
#223475,#223476,#223477,#223478,#223479,#223480,#223481,#223482,#223483,
#223484,#223485,#223486,#223487,#223488,#223489,#223490,#223491,#223492,
#223493,#223494,#223495,#223496,#223497,#223498,#223499,#223500,#223501,
#223502,#223503,#223504,#223505,#223506,#223507,#223508,#223509,#223510,
#223511,#223512,#223513,#223514,#223515,#223516,#223517,#223518,#223519,
#223520,#223521,#223522,#223523,#223524,#223525,#223526,#223527,#223528,
#223529,#223530,#223531,#223532,#223533,#223534,#223535,#223536,#223537,
#223538,#223539,#223540,#223541,#223542,#223543,#223544,#223545,#223546,
#223547,#223548,#223549,#223550,#223551,#223552,#223553,#223554,#223555,
#223556,#223557,#223558,#223559,#223560,#223561,#223562,#223563,#223564,
#223565,#223566,#223567,#223568,#223569,#223570,#223571,#223572,#223573,
#223574,#223575,#223576,#223577,#223578,#223579,#223580,#223581,#223582,
#223583,#223584,#223585,#223586,#223587,#223588,#223589,#223590,#223591,
#223592,#223593,#223594,#223595,#223596,#223597,#223598,#223599,#223600,
#223601,#223602,#223603,#223604,#223605,#223606,#223607,#223608,#223609,
#223610,#223611,#223612,#223613,#223614,#223615,#223616,#223617,#223618,
#223619,#223620,#223621,#223622,#223623,#223624,#223625,#223626,#223627,
#223628,#223629,#223630,#223631,#223632,#223633,#223634,#223635,#223636,
#223637,#223638,#223639,#223640,#223641,#223642,#223643,#223644,#223645,
#223646,#223647,#223648,#223649,#223650,#223651,#223652,#223653,#223654,
#223655,#223656,#223657,#223658,#223659,#223660,#223661,#223662,#223663,
#223664),.UNSPECIFIED.,.F.,.F.,(4,2,2,2,2,2,2,2,2,2,2,2,2,2,2,2,2,2,2,2,
2,2,2,2,2,2,2,2,2,2,2,2,2,2,2,2,2,2,2,2,2,2,2,2,2,2,2,2,2,2,2,2,2,2,2,2,
2,2,2,2,2,2,2,2,2,2,2,2,2,2,2,2,2,2,2,2,2,2,2,2,2,2,2,2,2,2,2,2,2,2,2,2,
2,2,2,2,2,2,2,2,2,2,2,2,2,2,2,2,2,2,2,2,2,2,2,2,2,2,2,2,2,2,2,2,2,2,2,2,
2,2,2,2,2,2,2,2,2,2,2,2,2,2,2,2,2,2,2,2,2,2,2,2,2,2,2,2,2,2,2,2,2,2,2,2,
2,2,2,2,2,2,2,2,2,2,2,2,2,2,2,2,2,2,2,2,2,2,2,2,2,2,2,2,2,2,2,2,2,2,2,2,
2,2,2,2,2,2,2,2,2,2,2,2,2,2,2,2,2,2,2,2,2,2,2,2,2,2,2,2,2,2,2,2,2,2,2,2,
2,2,2,2,2,2,2,2,2,2,2,2,2,2,2,2,2,2,4),(0.00133830262631356,0.139438357579086,
0.200909927955577,0.209508844580474,0.211752834325512,0.213080352109106,
0.21425700926626,0.215748706974759,0.218098192436531,0.229507013707793,
0.421993595380599,0.451620266910188,0.480376448296373,0.564544135124727,
0.602832587721176,0.606901427897204,0.610432288970518,0.612716015638118,
0.614869745106133,0.617705946905205,0.624020649056565,0.676613099641912,
0.792716358974852,0.863680718094834,0.944020370796353,0.99289578010674,
1.00250355589665,1.00485610951166,1.00623714079598,1.0074604759438,1.00899088934706,
1.01136000470524,1.0221962463077,1.20354130757576,1.30998710672542,1.38605329671361,
1.39215352513267,1.39506367492406,1.39727253011517,1.39936098582232,1.40285072718565,
1.41191520827557,1.54771635385412,1.63867471557651,1.72911277505056,1.78088275114964,
1.78876314347224,1.79098132633146,1.79232785980166,1.79353937140027,1.79508039105697,
1.7982538373683,1.81927056726594,1.96200762844306,2.04847660565329,2.14113543824455,
2.17773569801643,2.18287239840428,2.1854935870463,2.1873835799262,2.18938865687908,
2.19278630229899,2.20186958155214,2.33722773467721,2.50060575595169,2.57149882734751,
2.58060493690987,2.58286362986976,2.58417822291274,2.58532648014708,2.58674195305811,
2.58891753397617,2.59889492988857,2.75135851960496,2.88939193510352,2.96216521301957,
2.99425031221139,2.99916571891074,3.00170106364452,3.00355333098142,3.00554124911303,
3.00896688569999,3.01845745509103,3.16296825385149,3.32543755771256,3.34898711237156,
3.39147184743647,3.39970383932617,3.40244844803796,3.40422617717617,3.40590456287852,
3.40811769542958,3.41187806073602,3.43562639104619,3.54773631740017,3.6676714469246,
3.77225498147016,3.78226586073498,3.78694540533719,3.79051851051431,3.79391491178562,
3.79868197694032,3.80851603030731,3.97441210778706,4.119683924084,4.14888688815871,
4.15269904518385,4.15460964287051,4.1559831629307,4.15743660377674,4.159478642271,
4.16368645322822,4.22050801050266,4.41190400161341,4.55663191296641,4.56336107757395,
4.5663979885925,4.56866838544094,4.57078979759241,4.57370655964312,4.58108207041647,
4.67058351988751,4.89358917796121,4.92474876578906,4.95159199142561,4.97821944055346,
4.98204503443158,4.98438633471492,4.98621324155,4.98819933261065,4.99137447244364,
5.00179405488996,5.0699426278857,5.20808369035609,5.38527053225892,5.41042425222849,
5.41983366614312,5.4265826832077,5.43375681758525,5.44333431888808,5.46484765121972,
5.57996216820587,5.65479128536492,5.68869329771623,5.73185275959319,5.73849672794218,
5.74245231441446,5.74548616777338,5.74873600157766,5.75390634089256,5.77397816222956,
5.9814355572245,6.03130896745828,6.04346455190079,6.05046246516573,6.05584844879478,
6.06285039165623,6.07537423077362,6.14409384998325,6.3143969172455,6.43792305260728,
6.49673122735505,6.50220387745475,6.50488943595653,6.50681843702397,6.50886097308644,
6.51155774593098,6.51739639911708,6.67750525198442,6.75865006920376,6.89476115433202,
6.90322521459539,6.90626100808863,6.90837198088078,6.91032816189779,6.91293558776614,
6.91750399557843,6.92334613241918,7.03760266100932,7.14477910103911,7.31377547487298,
7.32453049265749,7.3268329729917,7.32831102657186,7.32948635398314,7.33080664183205,
7.33301424739902,7.34160235404719,7.40612517014378,7.52037669269505,7.70645039252268,
7.71776743304887,7.72138315458545,7.72337090328877,7.7253562990838,7.72774439402465,
7.73223030956566,7.73783892352537,7.8511828877305,7.97573271879192,8.11408627778447,
8.12309130145391,8.12535733731279,8.1266560321319,8.1277591296147,8.12910190027674,
8.131596215513,8.14493282113219,8.17178604713191,8.21687010570135,8.32019641079246,
8.43758484663809,8.47763935982405,8.54000493457614,8.54587143447741,8.5486928051518,
8.55069064155522,8.55257070465912,8.55457441209143,8.55877803393305,8.5769646127124,
8.60965389586113,8.70652660861874,8.92702254732146,8.9398724682088,8.94335730855871,
8.94539640540007,8.94713553048431,8.94926158894222,8.95323946597728,8.97533210932884,
9.02327082979482,9.17751427222401,9.3061983178575,9.31830290047008,9.32364829341486,
9.32750853216207,9.33151186440182,9.33736322491477,9.35294285029365,9.4268301021248,
9.53506249341463,9.62862823160764,9.64585991443363,9.65710552521339,9.66278829823707,
9.68703810663649,9.69098875590284,9.69297352937588,9.69451972221765,9.69622400684683,
9.698999900928,9.70856667948123,9.77139261896573,9.95633438646292),
 .UNSPECIFIED.);
#3553=B_SPLINE_CURVE_WITH_KNOTS('',3,(#223666,#223667,#223668,#223669,#223670,
#223671,#223672,#223673,#223674,#223675,#223676,#223677,#223678,#223679,
#223680,#223681,#223682,#223683),.UNSPECIFIED.,.F.,.F.,(4,2,2,2,2,2,2,2,
4),(221.03513445743,221.870051369324,222.704968281219,223.539885193114,
224.374802105009,225.209719016904,226.044635928798,226.879552840693,227.318319764609),
 .UNSPECIFIED.);
#3554=B_SPLINE_CURVE_WITH_KNOTS('',3,(#223685,#223686,#223687,#223688,#223689,
#223690,#223691,#223692,#223693,#223694,#223695,#223696,#223697,#223698,
#223699,#223700,#223701,#223702,#223703,#223704,#223705,#223706,#223707,
#223708,#223709,#223710,#223711,#223712,#223713,#223714,#223715,#223716,
#223717,#223718,#223719,#223720,#223721,#223722,#223723,#223724,#223725,
#223726,#223727,#223728,#223729,#223730,#223731,#223732,#223733,#223734,
#223735,#223736,#223737,#223738,#223739,#223740,#223741,#223742,#223743,
#223744,#223745,#223746,#223747,#223748,#223749,#223750,#223751,#223752,
#223753,#223754,#223755,#223756,#223757,#223758,#223759,#223760,#223761,
#223762,#223763,#223764,#223765,#223766,#223767,#223768,#223769,#223770,
#223771,#223772,#223773,#223774,#223775,#223776,#223777,#223778,#223779,
#223780,#223781,#223782,#223783,#223784,#223785,#223786,#223787,#223788,
#223789,#223790,#223791,#223792,#223793,#223794,#223795,#223796,#223797,
#223798,#223799,#223800,#223801,#223802,#223803,#223804,#223805,#223806,
#223807,#223808,#223809,#223810,#223811,#223812,#223813,#223814,#223815,
#223816,#223817,#223818,#223819,#223820,#223821,#223822,#223823,#223824,
#223825,#223826,#223827,#223828,#223829,#223830,#223831,#223832,#223833,
#223834,#223835,#223836,#223837,#223838,#223839,#223840,#223841,#223842,
#223843,#223844,#223845,#223846,#223847,#223848,#223849,#223850,#223851,
#223852,#223853,#223854,#223855,#223856,#223857,#223858,#223859,#223860,
#223861,#223862,#223863,#223864,#223865,#223866,#223867,#223868,#223869,
#223870,#223871,#223872,#223873,#223874,#223875,#223876,#223877,#223878,
#223879,#223880,#223881,#223882,#223883,#223884,#223885,#223886,#223887,
#223888,#223889,#223890,#223891,#223892,#223893,#223894,#223895,#223896,
#223897,#223898,#223899,#223900,#223901,#223902,#223903,#223904,#223905,
#223906,#223907,#223908,#223909,#223910,#223911,#223912,#223913,#223914,
#223915,#223916,#223917,#223918,#223919,#223920,#223921,#223922,#223923,
#223924,#223925,#223926,#223927,#223928,#223929,#223930,#223931,#223932,
#223933,#223934,#223935,#223936,#223937,#223938,#223939,#223940,#223941,
#223942,#223943,#223944,#223945,#223946,#223947,#223948,#223949,#223950,
#223951,#223952,#223953,#223954,#223955,#223956,#223957,#223958,#223959,
#223960,#223961,#223962,#223963,#223964,#223965,#223966,#223967,#223968,
#223969,#223970,#223971,#223972,#223973,#223974,#223975,#223976,#223977,
#223978,#223979,#223980,#223981,#223982,#223983,#223984,#223985,#223986,
#223987,#223988,#223989,#223990,#223991,#223992,#223993,#223994,#223995,
#223996,#223997,#223998,#223999,#224000,#224001,#224002,#224003,#224004,
#224005,#224006,#224007,#224008,#224009,#224010,#224011,#224012,#224013,
#224014,#224015,#224016,#224017,#224018,#224019,#224020,#224021,#224022,
#224023,#224024,#224025,#224026,#224027,#224028,#224029,#224030,#224031,
#224032,#224033,#224034,#224035,#224036,#224037,#224038,#224039,#224040,
#224041,#224042,#224043,#224044,#224045,#224046,#224047,#224048,#224049,
#224050,#224051,#224052,#224053,#224054,#224055,#224056,#224057,#224058,
#224059,#224060,#224061,#224062,#224063,#224064,#224065,#224066,#224067,
#224068,#224069,#224070,#224071,#224072,#224073,#224074,#224075,#224076,
#224077,#224078,#224079,#224080,#224081,#224082,#224083,#224084,#224085,
#224086,#224087,#224088,#224089,#224090,#224091,#224092,#224093,#224094,
#224095,#224096,#224097,#224098,#224099,#224100,#224101,#224102,#224103,
#224104,#224105,#224106,#224107,#224108,#224109,#224110,#224111,#224112,
#224113,#224114,#224115,#224116,#224117,#224118,#224119,#224120,#224121,
#224122,#224123,#224124,#224125,#224126,#224127,#224128,#224129,#224130,
#224131,#224132,#224133,#224134,#224135,#224136,#224137,#224138,#224139,
#224140,#224141,#224142,#224143,#224144,#224145,#224146,#224147,#224148,
#224149,#224150,#224151,#224152,#224153,#224154,#224155,#224156,#224157,
#224158,#224159,#224160,#224161,#224162,#224163,#224164,#224165,#224166,
#224167,#224168,#224169,#224170,#224171,#224172,#224173,#224174,#224175,
#224176,#224177,#224178,#224179,#224180,#224181,#224182,#224183,#224184,
#224185,#224186,#224187,#224188,#224189,#224190,#224191,#224192,#224193,
#224194,#224195,#224196,#224197,#224198,#224199,#224200,#224201,#224202,
#224203,#224204,#224205,#224206,#224207,#224208,#224209,#224210,#224211,
#224212,#224213,#224214,#224215,#224216,#224217,#224218,#224219,#224220,
#224221,#224222),.UNSPECIFIED.,.F.,.F.,(4,2,2,2,2,2,2,2,2,2,2,2,2,2,2,2,
2,2,2,2,2,2,2,2,2,2,2,2,2,2,2,2,2,2,2,2,2,2,2,2,2,2,2,2,2,2,2,2,2,2,2,2,
2,2,2,2,2,2,2,2,2,2,2,2,2,2,2,2,2,2,2,2,2,2,2,2,2,2,2,2,2,2,2,2,2,2,2,2,
2,2,2,2,2,2,2,2,2,2,2,2,2,2,2,2,2,2,2,2,2,2,2,2,2,2,2,2,2,2,2,2,2,2,2,2,
2,2,2,2,2,2,2,2,2,2,2,2,2,2,2,2,2,2,2,2,2,2,2,2,2,2,2,2,2,2,2,2,2,2,2,2,
2,2,2,2,2,2,2,2,2,2,2,2,2,2,2,2,2,2,2,2,2,2,2,2,2,2,2,2,2,2,2,2,2,2,2,2,
2,2,2,2,2,2,2,2,2,2,2,2,2,2,2,2,2,2,2,2,2,2,2,2,2,2,2,2,2,2,2,2,2,2,2,2,
2,2,2,2,2,2,2,2,2,2,2,2,2,2,2,2,2,2,2,2,2,2,2,2,2,2,2,2,2,2,2,2,2,2,2,2,
4),(0.00178360762374811,0.0736416897494022,0.280704762209549,0.294847251336195,
0.298018590754599,0.299811024405146,0.301192311175473,0.302748746647271,
0.305638356977403,0.31513399396247,0.455386698910708,0.500470124117633,
0.53975750666081,0.552003339287543,0.617577443491403,0.702478195068584,
0.708871301398597,0.711855620784236,0.714128620099592,0.716283576240149,
0.719296309366565,0.725463656407434,0.786247841157901,0.909477002392962,
0.968821161715167,1.02765063337858,1.12112766540002,1.12678639674282,1.12929415694603,
1.13115110306628,1.13287419573746,1.1352251344067,1.14107732993314,1.24082199303932,
1.39233488144518,1.48237708782175,1.54803643164556,1.56237107849847,1.56933971001752,
1.57644308820018,1.58461391499729,1.59857291468339,1.65332873119535,1.73312865494947,
1.83842567941408,1.87710508084618,1.88375186659346,1.88678289825031,1.88985952749663,
1.89275838744855,1.89679012052627,1.90852613144818,2.0643159495406,2.16143619777806,
2.18252216858226,2.19114626542794,2.19720987110186,2.20336684917722,2.21226410157583,
2.23457056351268,2.45090867448738,2.53144339999366,2.60206623812774,2.64296605667699,
2.64808616527274,2.65064380431516,2.65247956552519,2.65441984414856,2.65714235344626,
2.6643365673102,2.76574706790368,2.87912583703883,2.97911274856601,3.04192368600478,
3.0487579700802,3.05175610291892,3.05396369446428,3.05600237630447,3.05876841272881,
3.06557451953596,3.13631678757094,3.19054509817067,3.36545170144217,3.42221009471864,
3.45203128295713,3.4687124366621,3.47146286301705,3.47290177434407,3.47396120438062,
3.47510605069817,3.47675459188173,3.48145031775249,3.55916435810003,3.57179704511197,
3.5718481661994,3.57195307728899,3.57216179615365,3.57255335310267,3.57322000969604,
3.57421922007048,3.57554008060686,3.57712951241453,3.57893770370976,3.58096143035843,
3.71064831303396,3.78977211014492,3.8575104584985,3.86389324574107,3.86666455148945,
3.86869394590888,3.87056020058093,3.87308030169292,3.87922155834318,3.93972948997708,
4.14486254416908,4.20490079137044,4.24866398478748,4.26683150647065,4.26949809266037,
4.27086654396646,4.27198121352722,4.27326317744398,4.27542433269413,4.28310280982966,
4.4051648529001,4.57048717128833,4.67360405628189,4.6886572772091,4.6926100711883,
4.69495436119641,4.69702927609223,4.69962307313635,4.70363322164583,4.721932836118,
4.97980010703783,5.07962937050696,5.08622954481,5.08865289916885,5.09035601560706,
5.09194812364498,5.09413575088398,5.09840537651871,5.12743622900781,5.20275215386603,
5.3923091299888,5.45382923546852,5.46424974522926,5.4692295743262,5.47307642985705,
5.47729018828258,5.48410946430728,5.50748062234046,5.73211654119411,5.82971214580383,
5.83520471469364,5.83728016654339,5.83875761614752,5.84015472376008,5.84209932536465,
5.84598634903332,5.88032486338937,5.91637986209933,6.07590018220587,6.23590983347248,
6.24595720324807,6.24966355772437,6.25183656845789,6.25387566667094,6.25668925849661,
6.26222351088608,6.30128005557024,6.39663853102738,6.47831245960531,6.56882542353529,
6.65873728826974,6.66510252912432,6.66753909467498,6.66928457521318,6.67094337565561,
6.67326612782538,6.6779585529885,6.71744729032768,6.79209341809599,6.90977659843109,
7.02932697906653,7.08700850453278,7.10124953606111,7.10951043017779,7.11604987782794,
7.12478871562823,7.14027018361526,7.23233614079705,7.34555775417832,7.41382540140005,
7.42179901554951,7.42570676631063,7.42858182150987,7.43140806069661,7.43608548496645,
7.45052510571772,7.55246393419507,7.69854678042963,7.72044328951425,7.7285645046275,
7.73432868890056,7.74038743963821,7.74833780618792,7.76460761032734,7.91920597578543,
8.14824602837285,8.15749081604834,8.17237111205729,8.18446240003284,8.18820665725569,
8.19024281711461,8.19226190773564,8.19467181496988,8.19913722572664,8.20464093928975,
8.21612682960537,8.24632908749532,8.33565772522918,8.53046241093476,8.58188516983021,
8.58817007197953,8.59081921520617,8.59303018631877,8.59529988927096,8.59861765181704,
8.60739464823482,8.724561640462,8.87406841694435,8.914689766971,8.99114143558169,
9.00762108396818,9.0102825434955,9.01185219694736,9.01304377176556,9.01430678338724,
9.01558831328976,9.01741767249102,9.03134090334122,9.05987685738208,9.11420116947001,
9.15958271476645,9.38623529217457,9.40082711705873,9.40476995133339,9.40707442666774,
9.40905742910072,9.41146469538596,9.41598526871393,9.44139210831433,9.48883454267792,
9.58786856279916,9.62624751959209,9.64524310642237,9.66586810206775,9.74998235635441,
9.7589094337966,9.80434768099741,9.80801623936946,9.80945788783498,9.81051103350733,
9.81164639673706,9.81317896332834,9.81486699567909,9.81773313255874,9.9564473454049),
 .UNSPECIFIED.);
#3555=B_SPLINE_CURVE_WITH_KNOTS('',3,(#224224,#224225,#224226,#224227,#224228,
#224229,#224230,#224231,#224232,#224233,#224234,#224235,#224236,#224237,
#224238,#224239,#224240,#224241,#224242,#224243,#224244,#224245,#224246,
#224247,#224248,#224249,#224250,#224251,#224252,#224253,#224254,#224255,
#224256,#224257,#224258,#224259,#224260,#224261,#224262,#224263,#224264,
#224265,#224266,#224267,#224268,#224269,#224270,#224271,#224272,#224273,
#224274,#224275,#224276,#224277,#224278,#224279,#224280,#224281,#224282,
#224283,#224284,#224285,#224286,#224287,#224288,#224289,#224290,#224291,
#224292,#224293,#224294,#224295,#224296,#224297,#224298,#224299,#224300,
#224301,#224302,#224303,#224304,#224305,#224306,#224307,#224308,#224309,
#224310,#224311,#224312,#224313,#224314,#224315,#224316,#224317,#224318,
#224319,#224320,#224321,#224322,#224323,#224324,#224325,#224326,#224327,
#224328,#224329,#224330,#224331,#224332,#224333,#224334,#224335,#224336,
#224337,#224338,#224339,#224340,#224341,#224342,#224343,#224344,#224345,
#224346,#224347,#224348,#224349,#224350,#224351,#224352,#224353,#224354,
#224355,#224356,#224357,#224358,#224359,#224360,#224361,#224362,#224363,
#224364,#224365,#224366,#224367,#224368,#224369,#224370,#224371,#224372,
#224373,#224374,#224375,#224376,#224377,#224378,#224379,#224380,#224381,
#224382,#224383,#224384,#224385,#224386,#224387,#224388,#224389,#224390,
#224391,#224392,#224393,#224394,#224395,#224396,#224397,#224398,#224399,
#224400,#224401,#224402,#224403,#224404,#224405,#224406,#224407,#224408,
#224409,#224410,#224411,#224412,#224413,#224414,#224415,#224416,#224417,
#224418,#224419,#224420,#224421,#224422,#224423,#224424,#224425,#224426,
#224427,#224428,#224429,#224430,#224431,#224432,#224433,#224434,#224435,
#224436,#224437,#224438,#224439,#224440,#224441,#224442,#224443,#224444,
#224445,#224446,#224447,#224448,#224449,#224450,#224451,#224452,#224453,
#224454,#224455,#224456,#224457,#224458,#224459,#224460,#224461,#224462,
#224463,#224464,#224465,#224466,#224467,#224468,#224469,#224470,#224471,
#224472,#224473,#224474,#224475,#224476,#224477,#224478,#224479,#224480,
#224481,#224482),.UNSPECIFIED.,.F.,.F.,(4,3,3,3,3,3,3,3,3,3,3,3,3,3,3,3,
3,3,3,3,3,3,3,3,3,3,3,3,3,3,3,3,3,3,3,3,3,3,3,3,3,3,3,3,3,3,3,3,3,3,3,3,
3,3,3,3,3,3,3,3,3,3,3,3,3,3,3,3,3,3,3,3,3,3,3,3,3,3,3,3,3,3,3,3,3,3,4),
(239.884690378968,239.957555113344,240.03035368128,240.103101051101,240.177247962562,
240.249945830814,240.322640540092,240.39534554821,240.470578246854,240.54337728036,
240.619826811573,240.696276342786,240.77727032217,240.858147360236,240.942522072856,
241.023080466785,241.103515008765,241.183774426348,241.195646210717,241.270050513933,
241.344471584734,241.418921696184,241.493453731457,241.568030171724,241.642711118493,
241.695016078648,241.771587622015,241.848091514626,241.924538709216,242.000940118241,
242.077306621218,242.15436277038,242.230700160461,242.307037031759,242.383383239976,
242.46097638361,242.53739549535,242.615575654931,242.693755814511,242.767532905335,
242.841247682769,242.914913217055,242.988543362142,243.062151985947,243.135764803752,
243.193125682442,243.274559213523,243.356128208519,243.440220043982,243.522062750477,
243.607279150425,243.692495550373,243.77092849387,243.849291677751,243.927589943029,
244.005809208886,244.083978500391,244.162089825479,244.191865418304,244.268227889387,
244.344607215469,244.42101298111,244.497487653202,244.57399970093,244.650594030156,
244.691235286235,244.766612665172,244.841928498572,244.917195608182,244.992426783265,
245.067634788409,245.14542731762,245.220645493803,245.295880369381,245.371143512926,
245.44644650627,245.521838702226,245.597283601575,245.672826962675,245.689975022097,
245.767187134031,245.844261924242,245.925165364718,246.001941919313,246.078621149182,
246.155182952082,246.167875686148),.UNSPECIFIED.);
#3556=B_SPLINE_CURVE_WITH_KNOTS('',3,(#224484,#224485,#224486,#224487,#224488,
#224489,#224490,#224491,#224492,#224493,#224494,#224495,#224496,#224497,
#224498,#224499,#224500,#224501,#224502,#224503,#224504,#224505,#224506,
#224507,#224508,#224509,#224510,#224511,#224512,#224513,#224514,#224515,
#224516,#224517,#224518,#224519,#224520,#224521,#224522,#224523,#224524,
#224525,#224526,#224527,#224528,#224529,#224530,#224531,#224532,#224533,
#224534,#224535,#224536,#224537,#224538,#224539,#224540,#224541,#224542,
#224543,#224544,#224545,#224546,#224547,#224548,#224549,#224550,#224551,
#224552,#224553,#224554,#224555,#224556,#224557,#224558,#224559,#224560,
#224561,#224562,#224563,#224564,#224565,#224566,#224567,#224568,#224569,
#224570,#224571,#224572,#224573,#224574,#224575,#224576,#224577,#224578,
#224579,#224580,#224581,#224582,#224583,#224584,#224585,#224586,#224587,
#224588,#224589,#224590,#224591,#224592,#224593,#224594,#224595,#224596,
#224597,#224598,#224599,#224600,#224601,#224602,#224603,#224604,#224605,
#224606,#224607,#224608,#224609,#224610,#224611,#224612,#224613,#224614,
#224615,#224616,#224617,#224618,#224619,#224620,#224621,#224622,#224623,
#224624,#224625,#224626,#224627,#224628,#224629,#224630,#224631,#224632,
#224633,#224634,#224635,#224636,#224637,#224638,#224639,#224640,#224641,
#224642,#224643,#224644,#224645,#224646,#224647,#224648,#224649,#224650,
#224651,#224652,#224653,#224654,#224655,#224656,#224657,#224658,#224659,
#224660,#224661,#224662,#224663,#224664,#224665,#224666,#224667,#224668,
#224669,#224670,#224671,#224672,#224673,#224674,#224675,#224676,#224677,
#224678,#224679,#224680,#224681,#224682,#224683,#224684,#224685,#224686,
#224687,#224688,#224689,#224690,#224691,#224692,#224693,#224694,#224695,
#224696,#224697,#224698,#224699,#224700,#224701,#224702,#224703,#224704,
#224705,#224706,#224707,#224708,#224709,#224710,#224711,#224712,#224713,
#224714,#224715,#224716,#224717,#224718,#224719,#224720,#224721,#224722,
#224723,#224724,#224725,#224726,#224727,#224728,#224729,#224730,#224731,
#224732,#224733,#224734,#224735,#224736,#224737,#224738,#224739,#224740,
#224741,#224742,#224743,#224744,#224745,#224746,#224747,#224748,#224749,
#224750,#224751,#224752,#224753,#224754,#224755,#224756,#224757,#224758,
#224759,#224760,#224761,#224762,#224763,#224764,#224765,#224766,#224767,
#224768,#224769,#224770,#224771,#224772,#224773,#224774,#224775,#224776,
#224777,#224778,#224779,#224780,#224781,#224782,#224783,#224784,#224785,
#224786,#224787,#224788,#224789,#224790,#224791,#224792,#224793,#224794,
#224795,#224796,#224797,#224798,#224799,#224800,#224801,#224802,#224803,
#224804,#224805,#224806,#224807,#224808,#224809,#224810,#224811,#224812,
#224813,#224814,#224815,#224816,#224817,#224818,#224819,#224820,#224821,
#224822,#224823,#224824,#224825,#224826,#224827,#224828,#224829,#224830,
#224831,#224832,#224833,#224834,#224835,#224836,#224837,#224838,#224839,
#224840,#224841,#224842,#224843,#224844,#224845,#224846,#224847,#224848,
#224849,#224850,#224851,#224852,#224853,#224854,#224855,#224856,#224857,
#224858,#224859,#224860,#224861,#224862,#224863,#224864,#224865,#224866,
#224867,#224868,#224869,#224870,#224871,#224872,#224873,#224874,#224875,
#224876,#224877,#224878,#224879,#224880,#224881,#224882,#224883,#224884,
#224885,#224886,#224887,#224888,#224889,#224890,#224891,#224892,#224893,
#224894,#224895,#224896,#224897,#224898,#224899,#224900,#224901,#224902,
#224903,#224904,#224905,#224906,#224907,#224908,#224909,#224910,#224911,
#224912,#224913,#224914,#224915,#224916,#224917,#224918,#224919,#224920,
#224921,#224922,#224923,#224924,#224925,#224926,#224927,#224928,#224929,
#224930,#224931,#224932,#224933,#224934,#224935,#224936,#224937,#224938,
#224939,#224940,#224941,#224942,#224943,#224944,#224945,#224946,#224947,
#224948,#224949,#224950,#224951,#224952,#224953,#224954,#224955,#224956,
#224957,#224958,#224959,#224960,#224961,#224962,#224963,#224964,#224965,
#224966,#224967,#224968,#224969,#224970,#224971,#224972,#224973,#224974,
#224975,#224976,#224977,#224978,#224979,#224980,#224981,#224982,#224983,
#224984,#224985,#224986,#224987,#224988,#224989,#224990,#224991,#224992,
#224993,#224994,#224995,#224996,#224997,#224998,#224999,#225000,#225001,
#225002,#225003,#225004,#225005,#225006,#225007,#225008,#225009,#225010,
#225011,#225012,#225013,#225014,#225015,#225016,#225017),.UNSPECIFIED.,
 .F.,.F.,(4,2,2,2,2,2,2,2,2,2,2,2,2,2,2,2,2,2,2,2,2,2,2,2,2,2,2,2,2,2,2,
2,2,2,2,2,2,2,2,2,2,2,2,2,2,2,2,2,2,2,2,2,2,2,2,2,2,2,2,2,2,2,2,2,2,2,2,
2,2,2,2,2,2,2,2,2,2,2,2,2,2,2,2,2,2,2,2,2,2,2,2,2,2,2,2,2,2,2,2,2,2,2,2,
2,2,2,2,2,2,2,2,2,2,2,2,2,2,2,2,2,2,2,2,2,2,2,2,2,2,2,2,2,2,2,2,2,2,2,2,
2,2,2,2,2,2,2,2,2,2,2,2,2,2,2,2,2,2,2,2,2,2,2,2,2,2,2,2,2,2,2,2,2,2,2,2,
2,2,2,2,2,2,2,2,2,2,2,2,2,2,2,2,2,2,2,2,2,2,2,2,2,2,2,2,2,2,2,2,2,2,2,2,
2,2,2,2,2,2,2,2,2,2,2,2,2,2,2,2,2,2,2,2,2,2,2,2,2,2,2,2,2,2,2,2,2,2,2,2,
2,2,2,2,2,2,2,2,2,2,2,2,2,2,2,2,2,2,2,4),(0.00147305716892635,0.00749381998220008,
0.00989642461442405,0.0118079829048873,0.0137693260591038,0.0157355795135307,
0.0192465931573194,0.0297741239825986,0.0873493969891357,0.309696769649157,
0.386917603875351,0.411215935545746,0.41406333181997,0.415467841926669,
0.416480171622895,0.417554622416341,0.419069926507322,0.423112408404172,
0.484956706463286,0.494114742432427,0.515694312418917,0.731820880505203,
0.795121819518333,0.819069490393267,0.82856580696502,0.835511048725812,
0.838441313161028,0.840389133113309,0.842509999797709,0.845062003771217,
0.851412094911848,0.908480833484355,1.01255981481909,1.07729625381323,1.09665701093856,
1.15800091991536,1.20518863666577,1.22785370565823,1.23186240982777,1.23399511384717,
1.23575109661907,1.23752561776291,1.24079921845053,1.25143549274712,1.44446835282154,
1.52631919617496,1.59140646865762,1.60633110121011,1.61213071029591,1.61612296278743,
1.61999114752965,1.6247405785079,1.63588042157662,1.75650378644571,1.96383091052599,
1.97757903204481,1.9807217713994,1.98250785869409,1.98388888945621,1.98568650492903,
1.98879629180428,2.00082420528186,2.19385017145956,2.37693435446593,2.38535666134309,
2.39175036815653,2.39472265470329,2.39686584859117,2.39898135547327,2.4018438854827,
2.40741769515225,2.44979529423293,2.71343498761884,2.73079416994145,2.79736966063391,
2.80854519227524,2.81181812812695,2.81383515324019,2.81567037544692,2.81803395408874,
2.82276617905866,2.8529980196032,2.8612867076133,2.86643381522325,2.98856451763317,
3.1253986752823,3.22601978175105,3.24358587827009,3.25253770714906,3.25909387800418,
3.2661827112549,3.27864194095808,3.31591120605247,3.36710649550511,3.50600031282143,
3.55980969685452,3.56715564594322,3.57092583504954,3.57396604147693,3.57698479251259,
3.58249521420504,3.60296082659404,3.81093646320781,3.85994105138886,3.87160176412624,
3.87842203111497,3.884427704769,3.89192636976483,3.90360007035288,3.97143062851463,
3.97495143564316,3.97649115815609,4.04749999433727,4.06453889821016,4.23757604590462,
4.30596485869173,4.32785746101088,4.33223244725983,4.3346335189519,4.33645174296798,
4.33876671198754,4.34264894769786,4.35627818914582,4.59536721964481,4.69232564877964,
4.72834126061973,4.73361316043832,4.73630940619206,4.73826990626417,4.74036522290009,
4.74395416352845,4.75376908552651,4.90099425833841,4.98010012222836,5.1432563160117,
5.15325930909398,5.15550211296467,5.15696161288984,5.15813521677076,5.15946756770922,
5.16172910941596,5.17098096162955,5.24955585341429,5.42261552657406,5.46667333789819,
5.54137372597943,5.54785422847531,5.55043319534066,5.5523145168499,5.55433317357092,
5.55704228381609,5.56308101046833,5.70276588390827,5.73979259404873,5.77866701934748,
5.92017758878054,5.92576743604786,5.95009656844959,5.95294779902459,5.95437691929121,
5.95542707054886,5.95656490125618,5.95811088801615,5.96163614965713,6.08759608074564,
6.21357425203831,6.36308707052553,6.37341486535841,6.37698732961625,6.37902046657422,
6.38089018312365,6.38341217754772,6.38817720967175,6.41570960466292,6.4475385025929,
6.54687493552076,6.65192631687319,6.76096093250478,6.76886610722654,6.77193070183781,
6.77366200021271,6.77524670633711,6.77732982332109,6.78116610887155,6.78596506843429,
6.88663246451514,7.07183470096642,7.1368856175419,7.14748150659527,7.15244180554368,
7.15629671311951,7.1604781225499,7.16715520691697,7.18921223266523,7.3206039620109,
7.5078200116614,7.51713309276275,7.51999759696788,7.52154940649921,7.52308437729133,
7.52491028987963,7.52817254726477,7.53223476950029,7.6723361719209,7.81595939317523,
7.86455457435632,7.92357175312076,7.93028064328713,7.93306510614329,7.93537081646518,
7.93771924807057,7.94111852466097,7.94992391280861,8.0591076782085,8.0887611135404,
8.13812776786223,8.28657640163204,8.34325019165643,8.34861018147624,8.35103600423687,
8.35288627887708,8.35459858201271,8.3573808967227,8.36455599852038,8.37507745287341,
8.40518381527544,8.53002490562667,8.74637300487212,8.77406955171921,8.78624194839587,
8.79327693428413,8.80058211049047,8.81005414500892,8.82028986324185,8.88235743277589,
8.93346645511187,8.97046170487788,9.02146462883256,9.09666097922066,9.10471071642131,
9.10863262926514,9.11162336737462,9.11491326618468,9.12009970791608,9.13990783198821,
9.17654704045082,9.29281063685616,9.35066906214817,9.39724906810497,9.40911411238741,
9.41604832099134,9.42204197529525,9.42938193625996,9.44349784483151,9.51429789004961,
9.64979844535283,9.76391586292631,9.77979063864637,9.86249121300546,9.86826121530637,
9.87102118310009,9.8729717211139,9.87492256942972,9.87688418705653,9.87939211661189,
9.88325415979244,9.9567376273315),.UNSPECIFIED.);
#3557=B_SPLINE_CURVE_WITH_KNOTS('',3,(#225019,#225020,#225021,#225022,#225023,
#225024,#225025,#225026,#225027,#225028,#225029,#225030),.UNSPECIFIED.,
 .F.,.F.,(4,1,1,1,1,1,1,1,1,4),(258.73438144831,259.672331324168,260.67107106003,
261.669810795892,262.169180663823,262.668550531754,263.667290267616,264.166660135548,
264.666030003479,265.017431607686),.UNSPECIFIED.);
#3558=B_SPLINE_CURVE_WITH_KNOTS('',3,(#225032,#225033,#225034,#225035,#225036,
#225037,#225038,#225039,#225040,#225041,#225042,#225043,#225044,#225045,
#225046,#225047,#225048,#225049,#225050,#225051,#225052,#225053,#225054,
#225055,#225056,#225057,#225058,#225059,#225060,#225061,#225062,#225063,
#225064,#225065,#225066,#225067,#225068,#225069,#225070,#225071,#225072,
#225073,#225074,#225075,#225076,#225077,#225078,#225079,#225080,#225081,
#225082,#225083,#225084,#225085,#225086,#225087,#225088,#225089,#225090,
#225091,#225092,#225093,#225094,#225095,#225096,#225097,#225098,#225099,
#225100,#225101,#225102,#225103,#225104,#225105,#225106,#225107,#225108,
#225109,#225110,#225111,#225112,#225113,#225114,#225115,#225116,#225117,
#225118,#225119,#225120,#225121,#225122,#225123,#225124,#225125,#225126,
#225127,#225128,#225129,#225130,#225131,#225132,#225133,#225134,#225135,
#225136,#225137,#225138,#225139,#225140,#225141,#225142,#225143,#225144,
#225145,#225146,#225147,#225148,#225149,#225150,#225151,#225152,#225153,
#225154,#225155,#225156,#225157,#225158,#225159,#225160,#225161,#225162,
#225163,#225164,#225165,#225166,#225167,#225168,#225169,#225170,#225171,
#225172,#225173,#225174,#225175,#225176,#225177,#225178,#225179,#225180,
#225181,#225182,#225183,#225184,#225185,#225186,#225187,#225188,#225189,
#225190,#225191,#225192,#225193,#225194,#225195,#225196,#225197,#225198,
#225199,#225200,#225201,#225202,#225203,#225204,#225205,#225206,#225207,
#225208,#225209,#225210,#225211,#225212,#225213,#225214,#225215,#225216,
#225217,#225218,#225219,#225220,#225221,#225222,#225223,#225224,#225225,
#225226,#225227,#225228,#225229,#225230,#225231,#225232,#225233,#225234,
#225235,#225236,#225237,#225238,#225239,#225240,#225241,#225242,#225243,
#225244,#225245,#225246,#225247,#225248,#225249,#225250,#225251,#225252,
#225253,#225254,#225255,#225256,#225257,#225258,#225259,#225260,#225261,
#225262,#225263,#225264,#225265,#225266,#225267,#225268,#225269,#225270,
#225271,#225272,#225273,#225274,#225275,#225276,#225277,#225278,#225279,
#225280,#225281,#225282,#225283,#225284,#225285,#225286,#225287,#225288,
#225289,#225290,#225291,#225292,#225293,#225294,#225295,#225296,#225297,
#225298,#225299,#225300,#225301,#225302,#225303,#225304,#225305,#225306,
#225307,#225308,#225309,#225310,#225311,#225312,#225313,#225314,#225315,
#225316,#225317,#225318,#225319,#225320,#225321,#225322,#225323,#225324,
#225325,#225326,#225327,#225328,#225329,#225330,#225331,#225332,#225333,
#225334,#225335,#225336,#225337,#225338,#225339,#225340,#225341,#225342,
#225343,#225344,#225345,#225346,#225347,#225348,#225349,#225350,#225351,
#225352,#225353,#225354,#225355,#225356,#225357,#225358,#225359,#225360,
#225361,#225362,#225363,#225364,#225365,#225366,#225367,#225368,#225369,
#225370,#225371,#225372,#225373,#225374,#225375,#225376,#225377,#225378,
#225379,#225380,#225381,#225382,#225383,#225384,#225385,#225386,#225387,
#225388,#225389,#225390,#225391,#225392,#225393,#225394,#225395,#225396,
#225397,#225398,#225399,#225400,#225401,#225402,#225403,#225404,#225405,
#225406,#225407,#225408,#225409,#225410,#225411,#225412,#225413,#225414,
#225415,#225416,#225417,#225418,#225419,#225420,#225421,#225422,#225423,
#225424,#225425,#225426,#225427,#225428,#225429,#225430,#225431,#225432,
#225433,#225434,#225435,#225436,#225437,#225438,#225439,#225440,#225441,
#225442,#225443,#225444,#225445,#225446,#225447,#225448,#225449,#225450,
#225451,#225452,#225453,#225454,#225455,#225456,#225457,#225458,#225459,
#225460,#225461,#225462,#225463,#225464,#225465,#225466,#225467,#225468,
#225469,#225470,#225471,#225472,#225473,#225474,#225475,#225476,#225477,
#225478,#225479,#225480,#225481,#225482,#225483,#225484,#225485,#225486,
#225487,#225488,#225489,#225490,#225491,#225492,#225493,#225494,#225495,
#225496,#225497,#225498,#225499,#225500,#225501,#225502,#225503,#225504,
#225505,#225506,#225507,#225508,#225509,#225510,#225511,#225512,#225513,
#225514,#225515,#225516,#225517,#225518,#225519,#225520,#225521,#225522,
#225523,#225524,#225525,#225526,#225527,#225528,#225529,#225530,#225531,
#225532,#225533,#225534,#225535,#225536,#225537,#225538,#225539,#225540,
#225541,#225542,#225543,#225544,#225545,#225546,#225547,#225548,#225549,
#225550,#225551,#225552,#225553,#225554,#225555,#225556,#225557,#225558,
#225559),.UNSPECIFIED.,.F.,.F.,(4,2,2,2,2,2,2,2,2,2,2,2,2,2,2,2,2,2,2,2,
2,2,2,2,2,2,2,2,2,2,2,2,2,2,2,2,2,2,2,2,2,2,2,2,2,2,2,2,2,2,2,2,2,2,2,2,
2,2,2,2,2,2,2,2,2,2,2,2,2,2,2,2,2,2,2,2,2,2,2,2,2,2,2,2,2,2,2,2,2,2,2,2,
2,2,2,2,2,2,2,2,2,2,2,2,2,2,2,2,2,2,2,2,2,2,2,2,2,2,2,2,2,2,2,2,2,2,2,2,
2,2,2,2,2,2,2,2,2,2,2,2,2,2,2,2,2,2,2,2,2,2,2,2,2,2,2,2,2,2,2,2,2,2,2,2,
2,2,2,2,2,2,2,2,2,2,2,2,2,2,2,2,2,2,2,2,2,2,2,2,2,2,2,2,2,2,2,2,2,2,2,2,
2,2,2,2,2,2,2,2,2,2,2,2,2,2,2,2,2,2,2,2,2,2,2,2,2,2,2,2,2,2,2,2,2,2,2,2,
2,2,2,2,2,2,2,2,2,2,2,2,2,2,2,2,2,2,2,2,2,2,2,2,2,2,2,4),(0.0013984589909669,
0.00758538319000157,0.0138316523058583,0.0196994110499808,0.0254599733433377,
0.0312029810325234,0.0408521959009723,0.0670506220258798,0.263875818637476,
0.374604171535812,0.442494887563076,0.470980336443651,0.475686080779563,
0.478158061972327,0.480177753916977,0.482204380610581,0.485908081914892,
0.497628898150731,0.670987232608517,0.724939834278448,0.803424167889865,
0.849056130185995,0.864568053748669,0.871496288178267,0.876953491396784,
0.879688091340448,0.881654135300919,0.883734616898646,0.886658491409639,
0.892692402676658,0.954517790180003,1.06719782345678,1.15138318962781,1.18514845399419,
1.23231646350036,1.28885223140284,1.29709014176535,1.29930269250406,1.30062416518764,
1.30179943662341,1.30327593644542,1.30557097117994,1.31695230561336,1.50171553573889,
1.5938543621018,1.65834335694585,1.67763285556883,1.68561494092747,1.68976246383864,
1.69237257390772,1.69482033988358,1.6966161003335,1.6985505366644,1.70190228222598,
1.71129664884711,1.84910727268763,1.99739640916572,2.02100485290848,2.0565939400234,
2.08994215418236,2.0957540899652,2.09761686394535,2.09881621982331,2.09995044159275,
2.10144848376419,2.10480041403386,2.13297363986997,2.2876359039831,2.38723418769212,
2.47826436330779,2.51407056879355,2.51916574942751,2.52175708196898,2.5236354376741,
2.52563740670042,2.5290524710947,2.53831181011983,2.68028656066205,2.8324264657307,
2.90092423575469,2.91214135413812,2.91534425345094,2.91729956497148,2.91906631924886,
2.92132438200619,2.92578812394697,2.95256148843368,3.01423206727539,3.26243012592556,
3.27844658624767,3.29057289505769,3.29588173518521,3.29977948537614,3.30337471127242,
3.30825234064485,3.31780649178716,3.40149477966164,3.53814658106887,3.59989758903079,
3.65270955818973,3.66126772315916,3.66393161015268,3.66561063506772,3.66716358391967,
3.66916538212632,3.67345173202999,3.70998647186018,3.7721878154103,3.94430896203305,
4.06623184297491,4.07382353364534,4.0770250111134,4.07933455863342,4.08143461370161,
4.08423514208219,4.09131604185056,4.16017456317236,4.21543042597559,4.41500376306745,
4.4521538777401,4.48846673739912,4.49302679587756,4.49532275048454,4.49697849173306,
4.49873536850344,4.50171302672694,4.50969788929422,4.5558996031632,4.55818672904746,
4.56651708872552,4.57426148976264,4.77405762967652,4.86244585520452,4.89816258982957,
4.9225221813698,4.93269101177473,4.94010362094912,4.94693270702372,4.95622585494011,
4.97958641694583,5.0863155888876,5.15991929287492,5.24062255944352,5.24887205316262,
5.25282366209976,5.25588313616447,5.25923978573685,5.26475455410025,5.28896928931034,
5.33840611258749,5.49964326902273,5.54206554987833,5.553707258246,5.56052332500533,
5.56647212405472,5.57394869997153,5.58873393812068,5.71364833666406,5.9061894145442,
6.00679675291165,6.01261567146818,6.01538767008321,6.0173416800407,6.01917446491608,
6.02170233049056,6.02667548361257,6.06271202118362,6.09128764979767,6.15084395491074,
6.30478092038589,6.35053978392625,6.40815910863949,6.4140684345446,6.4169608418462,
6.41903241393073,6.42121989791487,6.42409603483496,6.43027284727676,6.51402358647735,
6.63579271745738,6.80402699030117,6.82831240965539,6.8355042153803,6.83770194046944,
6.83888820738784,6.84005890868061,6.84143348485369,6.8439713904554,6.84711217147657,
6.95303621399563,7.05646877155635,7.16537518155188,7.22353235432673,7.22910956974834,
7.23180208113871,7.23371339844825,7.23551589336713,7.23801707150799,7.2429867141531,
7.27998503378046,7.3348989053676,7.53134472478755,7.60492069071673,7.63156229589308,
7.63448822126048,7.63593585331661,7.63699054844077,7.63812500419528,7.63965183604271,
7.64300335547336,7.67947348396097,7.75067837410735,7.82415842626353,8.0390830623178,
8.05400031891449,8.05808222761089,8.06047905128405,8.06254827147825,8.06506867161196,
8.06982713453443,8.09722967526423,8.13885817957425,8.27389320604298,8.43497693338631,
8.44942197315286,8.45273607831524,8.45491005719968,8.45666809466609,8.45863456403046,
8.46194762489439,8.46595644578898,8.47398697322504,8.49476788188291,8.53902296438352,
8.76260942456012,8.81939643524981,8.82955370676513,8.83447962426361,8.83831846655862,
8.84255749072362,8.84949445072087,8.87403410273132,9.09894629367027,9.17057566260111,
9.19692712812516,9.20102682623861,9.20301373803425,9.2045597691785,9.20599530795815,
9.20845855989933,9.2152745407914,9.22522897971901,9.2552425534656,9.29861907247562,
9.59372018011532,9.60981212948134,9.61423054017918,9.61682876017148,9.61907428775765,
9.62181258414712,9.62699222677798,9.65710591683204,9.70170682036863,9.95757013430097),
 .UNSPECIFIED.);
#3559=B_SPLINE_CURVE_WITH_KNOTS('',3,(#225561,#225562,#225563,#225564,#225565,
#225566,#225567,#225568,#225569,#225570,#225571,#225572,#225573,#225574,
#225575,#225576,#225577,#225578,#225579,#225580,#225581,#225582,#225583,
#225584,#225585,#225586,#225587,#225588,#225589,#225590,#225591,#225592,
#225593,#225594,#225595,#225596,#225597,#225598,#225599,#225600,#225601,
#225602,#225603,#225604,#225605,#225606,#225607,#225608,#225609,#225610,
#225611,#225612,#225613,#225614,#225615,#225616,#225617,#225618,#225619,
#225620,#225621,#225622,#225623,#225624,#225625,#225626,#225627,#225628,
#225629,#225630,#225631,#225632,#225633,#225634,#225635,#225636,#225637,
#225638,#225639,#225640,#225641,#225642,#225643,#225644,#225645,#225646,
#225647,#225648,#225649,#225650,#225651,#225652,#225653,#225654,#225655,
#225656,#225657,#225658,#225659,#225660,#225661,#225662,#225663,#225664,
#225665,#225666,#225667,#225668,#225669,#225670,#225671,#225672,#225673,
#225674,#225675,#225676,#225677,#225678,#225679,#225680,#225681,#225682,
#225683,#225684,#225685,#225686,#225687,#225688,#225689,#225690,#225691,
#225692,#225693,#225694,#225695,#225696,#225697,#225698,#225699,#225700,
#225701,#225702,#225703,#225704,#225705,#225706,#225707,#225708,#225709,
#225710,#225711,#225712,#225713,#225714,#225715,#225716,#225717,#225718,
#225719,#225720,#225721,#225722,#225723,#225724,#225725,#225726,#225727,
#225728,#225729,#225730,#225731,#225732,#225733,#225734,#225735,#225736,
#225737,#225738,#225739,#225740,#225741,#225742,#225743,#225744,#225745,
#225746,#225747,#225748,#225749,#225750,#225751,#225752,#225753,#225754,
#225755,#225756,#225757,#225758,#225759,#225760,#225761,#225762,#225763,
#225764,#225765,#225766,#225767,#225768,#225769,#225770,#225771,#225772,
#225773,#225774,#225775,#225776,#225777,#225778,#225779,#225780,#225781,
#225782,#225783,#225784,#225785,#225786,#225787,#225788,#225789,#225790,
#225791,#225792,#225793,#225794,#225795,#225796,#225797,#225798,#225799,
#225800,#225801,#225802,#225803,#225804,#225805,#225806,#225807,#225808,
#225809,#225810,#225811,#225812,#225813,#225814,#225815,#225816,#225817,
#225818,#225819,#225820,#225821,#225822,#225823,#225824,#225825,#225826,
#225827,#225828,#225829,#225830,#225831,#225832,#225833,#225834,#225835,
#225836,#225837,#225838,#225839,#225840,#225841,#225842,#225843,#225844,
#225845,#225846,#225847,#225848,#225849,#225850,#225851,#225852,#225853,
#225854,#225855,#225856,#225857,#225858,#225859,#225860,#225861,#225862,
#225863,#225864,#225865,#225866,#225867,#225868,#225869,#225870,#225871,
#225872,#225873,#225874,#225875,#225876,#225877,#225878,#225879,#225880,
#225881,#225882,#225883,#225884,#225885,#225886,#225887,#225888,#225889,
#225890,#225891,#225892,#225893,#225894,#225895,#225896,#225897,#225898,
#225899,#225900,#225901,#225902,#225903,#225904,#225905,#225906,#225907,
#225908,#225909,#225910,#225911,#225912,#225913,#225914,#225915,#225916,
#225917,#225918,#225919,#225920,#225921,#225922,#225923,#225924,#225925,
#225926,#225927,#225928,#225929,#225930,#225931,#225932,#225933,#225934,
#225935,#225936,#225937,#225938,#225939,#225940,#225941,#225942,#225943,
#225944,#225945,#225946,#225947,#225948,#225949,#225950,#225951,#225952,
#225953,#225954,#225955,#225956,#225957,#225958,#225959,#225960,#225961,
#225962,#225963,#225964,#225965,#225966,#225967,#225968,#225969,#225970,
#225971,#225972,#225973,#225974,#225975,#225976,#225977,#225978,#225979,
#225980,#225981,#225982,#225983,#225984,#225985,#225986,#225987,#225988,
#225989,#225990,#225991,#225992,#225993,#225994,#225995,#225996,#225997,
#225998,#225999,#226000,#226001,#226002,#226003,#226004,#226005,#226006,
#226007,#226008,#226009,#226010,#226011,#226012,#226013,#226014,#226015,
#226016,#226017,#226018,#226019,#226020,#226021,#226022,#226023,#226024,
#226025,#226026,#226027,#226028,#226029,#226030,#226031,#226032,#226033,
#226034,#226035,#226036,#226037,#226038,#226039,#226040,#226041,#226042,
#226043,#226044,#226045,#226046,#226047,#226048,#226049,#226050,#226051,
#226052,#226053,#226054,#226055,#226056,#226057,#226058,#226059,#226060,
#226061,#226062,#226063,#226064,#226065,#226066,#226067,#226068,#226069,
#226070,#226071,#226072,#226073,#226074,#226075,#226076,#226077,#226078,
#226079,#226080,#226081,#226082,#226083,#226084),.UNSPECIFIED.,.F.,.F.,
(4,2,2,2,2,2,2,2,2,2,2,2,2,2,2,2,2,2,2,2,2,2,2,2,2,2,2,2,2,2,2,2,2,2,2,
2,2,2,2,2,2,2,2,2,2,2,2,2,2,2,2,2,2,2,2,2,2,2,2,2,2,2,2,2,2,2,2,2,2,2,2,
2,2,2,2,2,2,2,2,2,2,2,2,2,2,2,2,2,2,2,2,2,2,2,2,2,2,2,2,2,2,2,2,2,2,2,2,
2,2,2,2,2,2,2,2,2,2,2,2,2,2,2,2,2,2,2,2,2,2,2,2,2,2,2,2,2,2,2,2,2,2,2,2,
2,2,2,2,2,2,2,2,2,2,2,2,2,2,2,2,2,2,2,2,2,2,2,2,2,2,2,2,2,2,2,2,2,2,2,2,
2,2,2,2,2,2,2,2,2,2,2,2,2,2,2,2,2,2,2,2,2,2,2,2,2,2,2,2,2,2,2,2,2,2,2,2,
2,2,2,2,2,2,2,2,2,2,2,2,2,2,2,2,2,2,2,2,2,2,2,2,2,2,2,2,2,2,2,2,2,2,2,2,
2,2,2,2,2,2,2,2,2,2,4),(0.00178286918103071,0.0702116732403354,0.0739134554827725,
0.0762686171690966,0.0780700941729444,0.0798031318675091,0.0815216676358921,
0.0838550823887649,0.0896065993021719,0.164469550269398,0.178374533877773,
0.32160563258876,0.386827762891506,0.471904890444151,0.492986723116284,
0.504735745040343,0.515147997854299,0.522603509386662,0.529380986753213,
0.538466808477913,0.560604650320051,0.72824374638507,0.822365739799538,
0.831373276795891,0.83546871079109,0.838387196001289,0.841558656577101,
0.846304169102604,0.86079626188838,0.92306555897299,1.08366895181813,1.12580905683544,
1.13698457916237,1.14369764165037,1.14971967740729,1.15738911520198,1.16963031667308,
1.25324542117658,1.25487205590743,1.39735445259342,1.47469279260515,1.55911341679864,
1.58100622837593,1.58961063169148,1.59398013506102,1.59762491862314,1.59984586309468,
1.60187285632001,1.60443498701174,1.6094090575242,1.6369315135227,1.8156866689287,
1.87671167317494,1.91310114619797,1.96632370158965,1.99343841542587,1.99833378850852,
2.00095017198125,2.00290087211242,2.00534253579087,2.0094424247477,2.02309515423683,
2.22704446612452,2.30613662411913,2.373741475614,2.40300492833247,2.41736952844954,
2.42000225318346,2.42142741260923,2.42248509982681,2.42363625727691,2.42530804519999,
2.43016758672025,2.51068593651509,2.70447576402168,2.80682032781053,2.81269252436261,
2.81537023123019,2.8173832629407,2.81927227527447,2.82188213036766,2.82854786113356,
2.91191490271624,3.01271061770623,3.12311267126745,3.18301569140295,3.21124211130723,
3.21481530627825,3.21758566695507,3.21898720138829,3.21999875576205,3.22107363425176,
3.22259160035302,3.22665321282433,3.28975829054167,3.44758266392114,3.55216454587476,
3.62484020195874,3.63714335469069,3.64082044972755,3.64310237917082,3.64518882801826,
3.64784534149745,3.65215436380811,3.66370874320673,3.86275202736945,4.01883048364631,
4.03229557406914,4.03570901908868,4.03771092228346,4.03946916457513,4.04164948561655,
4.04499095415936,4.05684111953118,4.22391385832158,4.32492680588544,4.39384547204995,
4.40929249818887,4.4151757713194,4.41918410156414,4.42308195796013,4.42774849343317,
4.43929718819992,4.58447487048618,4.71058063202622,4.75772221719597,4.77958681927027,
4.78318388134995,4.78506764999755,4.7866033255218,4.78837005230441,4.79134980813085,
4.80200481725375,4.97779453670051,5.17919466977863,5.19193290207189,5.19601480620525,
5.19826197228476,5.20050861069068,5.20326969184945,5.2085579321487,5.24113649814398,
5.31216611815138,5.51390710740312,5.60617790989111,5.61201333075414,5.61435999222778,
5.61608108423327,5.61793680196753,5.62044239385927,5.62609476488107,5.73810651998382,
5.83440217112809,5.92774913980307,6.00090088418838,6.03741721456688,6.04956461018117,
6.05659241272413,6.06389520351191,6.07337240929874,6.09359147351263,6.19529800053409,
6.26635008247157,6.35988397980786,6.36806909588673,6.37200663194041,6.37506265450251,
6.37842301211415,6.38396335201921,6.40860049569881,6.45939283193589,6.56747742286012,
6.61312086246876,6.61454182808589,6.63883833883263,6.66484242091535,6.67451670989531,
6.68025971480296,6.68632245567479,6.69432221923568,6.71185458909553,6.95204534382295,
7.11855733567308,7.12223529097698,7.13100900399951,7.13429529143143,7.13623889121713,
7.13807372463758,7.14062309868737,7.14570585888688,7.18611676571545,7.20738929120618,
7.26066915850748,7.40385925154798,7.46892479873277,7.52673788303649,7.53264978817835,
7.53554193863534,7.5376126280315,7.53979854117012,7.54267154541657,7.54842206898336,
7.58748227248819,7.6863002975352,7.77193864881608,7.91578203645863,7.95128191182783,
7.95498001168649,7.95644115954674,7.95753591908568,7.95873883296929,7.96040438186014,
7.96437843887609,8.06121820142061,8.21491708697904,8.33897543486416,8.34687856333327,
8.34968353266834,8.35162496278071,8.35341694022077,8.35584397420615,8.36005641699285,
8.38237386617808,8.42543011028978,8.52690141301026,8.73814164392687,8.75049573626578,
8.75280294918174,8.7542336798369,8.7553531958431,8.75659362495449,8.75862812913511,
8.76576542221671,8.81155263273582,8.87000187257926,8.99840624358182,9.03326004324483,
9.15513213718595,9.17116561220399,9.17535803919379,9.17777971444962,9.17963975728071,
9.18204404358492,9.18627184663985,9.20371922922874,9.2335846971396,9.31254852452438,
9.3700428151602,9.55479697246631,9.56697239860403,9.57038454765662,9.5724055450048,
9.57416101670328,9.57631295710055,9.58041811658988,9.60531436375194,9.66071275428514,
9.92178683662287,9.94215160107944,9.9484448831181,9.95135769407405,9.95208945193033),
 .UNSPECIFIED.);
#3560=B_SPLINE_CURVE_WITH_KNOTS('',3,(#226086,#226087,#226088,#226089,#226090,
#226091,#226092,#226093,#226094,#226095,#226096,#226097,#226098,#226099,
#226100,#226101,#226102,#226103,#226104,#226105,#226106,#226107,#226108,
#226109,#226110,#226111,#226112,#226113,#226114,#226115,#226116,#226117,
#226118,#226119,#226120,#226121,#226122,#226123,#226124,#226125,#226126,
#226127,#226128,#226129,#226130,#226131,#226132,#226133,#226134,#226135,
#226136,#226137,#226138,#226139,#226140,#226141,#226142,#226143,#226144,
#226145,#226146,#226147,#226148,#226149,#226150,#226151,#226152,#226153,
#226154,#226155,#226156,#226157,#226158,#226159,#226160,#226161,#226162,
#226163,#226164,#226165,#226166,#226167,#226168,#226169,#226170,#226171,
#226172,#226173,#226174,#226175,#226176,#226177,#226178,#226179,#226180,
#226181,#226182,#226183,#226184,#226185,#226186,#226187,#226188,#226189,
#226190,#226191,#226192,#226193,#226194,#226195,#226196,#226197,#226198,
#226199,#226200,#226201,#226202,#226203,#226204,#226205,#226206,#226207,
#226208,#226209,#226210,#226211,#226212,#226213,#226214,#226215,#226216,
#226217,#226218,#226219,#226220,#226221,#226222,#226223,#226224,#226225,
#226226,#226227,#226228,#226229,#226230,#226231,#226232,#226233,#226234,
#226235,#226236,#226237,#226238,#226239,#226240,#226241,#226242,#226243,
#226244,#226245,#226246,#226247,#226248,#226249,#226250,#226251,#226252,
#226253,#226254,#226255,#226256,#226257,#226258,#226259,#226260,#226261,
#226262,#226263,#226264,#226265,#226266,#226267,#226268,#226269,#226270,
#226271,#226272,#226273,#226274,#226275,#226276,#226277,#226278,#226279,
#226280,#226281,#226282,#226283,#226284,#226285,#226286,#226287,#226288,
#226289,#226290,#226291,#226292,#226293,#226294,#226295,#226296,#226297,
#226298,#226299,#226300,#226301,#226302,#226303,#226304,#226305,#226306,
#226307,#226308,#226309,#226310,#226311,#226312,#226313,#226314,#226315,
#226316,#226317,#226318,#226319,#226320,#226321,#226322,#226323,#226324,
#226325,#226326,#226327,#226328,#226329,#226330,#226331,#226332,#226333,
#226334,#226335,#226336,#226337,#226338,#226339,#226340,#226341,#226342,
#226343,#226344,#226345,#226346,#226347,#226348,#226349,#226350,#226351,
#226352,#226353,#226354,#226355,#226356,#226357,#226358,#226359,#226360,
#226361,#226362,#226363,#226364,#226365,#226366,#226367,#226368,#226369,
#226370,#226371,#226372,#226373,#226374,#226375,#226376,#226377,#226378,
#226379,#226380,#226381,#226382,#226383,#226384,#226385,#226386,#226387,
#226388,#226389,#226390,#226391,#226392,#226393,#226394,#226395,#226396,
#226397,#226398,#226399,#226400,#226401,#226402,#226403,#226404,#226405,
#226406,#226407,#226408,#226409,#226410,#226411,#226412,#226413,#226414,
#226415,#226416,#226417,#226418,#226419,#226420,#226421,#226422,#226423,
#226424,#226425,#226426,#226427,#226428,#226429,#226430,#226431,#226432,
#226433,#226434,#226435,#226436,#226437,#226438,#226439,#226440,#226441,
#226442,#226443,#226444,#226445,#226446,#226447,#226448,#226449,#226450,
#226451,#226452,#226453,#226454,#226455,#226456,#226457,#226458,#226459,
#226460,#226461,#226462,#226463,#226464,#226465,#226466,#226467,#226468,
#226469,#226470,#226471,#226472,#226473,#226474,#226475,#226476,#226477,
#226478,#226479,#226480,#226481,#226482,#226483,#226484,#226485,#226486,
#226487,#226488,#226489,#226490,#226491,#226492,#226493,#226494,#226495,
#226496,#226497,#226498,#226499,#226500,#226501,#226502,#226503,#226504,
#226505,#226506,#226507,#226508,#226509,#226510,#226511,#226512,#226513,
#226514,#226515,#226516,#226517,#226518,#226519,#226520,#226521,#226522,
#226523,#226524,#226525,#226526,#226527,#226528,#226529,#226530,#226531,
#226532,#226533,#226534,#226535,#226536,#226537,#226538,#226539,#226540,
#226541,#226542,#226543,#226544,#226545,#226546,#226547,#226548,#226549,
#226550,#226551,#226552,#226553,#226554,#226555,#226556,#226557,#226558,
#226559,#226560,#226561,#226562,#226563,#226564,#226565,#226566,#226567,
#226568,#226569,#226570,#226571,#226572,#226573,#226574,#226575,#226576,
#226577,#226578,#226579,#226580,#226581,#226582,#226583,#226584,#226585,
#226586,#226587,#226588,#226589,#226590,#226591,#226592,#226593,#226594,
#226595,#226596,#226597,#226598,#226599,#226600,#226601,#226602,#226603,
#226604,#226605,#226606,#226607,#226608,#226609,#226610,#226611,#226612,
#226613,#226614,#226615,#226616,#226617,#226618,#226619),.UNSPECIFIED.,
 .F.,.F.,(4,2,2,2,2,2,2,2,2,2,2,2,2,2,2,2,2,2,2,2,2,2,2,2,2,2,2,2,2,2,2,
2,2,2,2,2,2,2,2,2,2,2,2,2,2,2,2,2,2,2,2,2,2,2,2,2,2,2,2,2,2,2,2,2,2,2,2,
2,2,2,2,2,2,2,2,2,2,2,2,2,2,2,2,2,2,2,2,2,2,2,2,2,2,2,2,2,2,2,2,2,2,2,2,
2,2,2,2,2,2,2,2,2,2,2,2,2,2,2,2,2,2,2,2,2,2,2,2,2,2,2,2,2,2,2,2,2,2,2,2,
2,2,2,2,2,2,2,2,2,2,2,2,2,2,2,2,2,2,2,2,2,2,2,2,2,2,2,2,2,2,2,2,2,2,2,2,
2,2,2,2,2,2,2,2,2,2,2,2,2,2,2,2,2,2,2,2,2,2,2,2,2,2,2,2,2,2,2,2,2,2,2,2,
2,2,2,2,2,2,2,2,2,2,2,2,2,2,2,2,2,2,2,2,2,2,2,2,2,2,2,2,2,2,2,2,2,2,2,2,
2,2,2,2,2,2,2,2,2,2,2,2,2,2,2,2,2,2,2,4),(0.00234020634155756,0.0027510816593974,
0.00551666244128114,0.00960651587262544,0.015988039053587,0.034709088262484,
0.0487890063522092,0.298800863107575,0.344565586174986,0.365421925911194,
0.368975910792349,0.37085125084883,0.372387305170986,0.374162580527031,
0.377176090405291,0.388159462689479,0.572357328461512,0.596799345510092,
0.648110740262354,0.731805891957862,0.774921877363855,0.780612143318704,
0.78345762638049,0.785501125101516,0.787661491073668,0.791303999476934,
0.80094218796162,0.946683184463535,0.973280832551976,1.05209220156824,1.0788670978043,
1.11860737335751,1.18527413803429,1.19645764841932,1.19973138775093,1.20174856430344,
1.20358369678438,1.20594684048276,1.20974273635202,1.22976469973963,1.4196872550323,
1.58620370649975,1.62426033872084,1.63621069661681,1.64303996562399,1.64936279581738,
1.65808096700916,1.67443605317583,1.79797767843293,1.87897483675758,1.926105216938,
1.95020944640804,1.95613923727781,1.95963150463417,1.9626687341535,1.96640041163289,
1.97390276119606,2.04999442128266,2.15757843334392,2.23620418547095,2.25503206188746,
2.26327588537184,2.26869624063672,2.2747953808667,2.28359753911647,2.30532834570571,
2.5676610715653,2.67852344161176,2.71503694047112,2.72003333407314,2.72256580956398,
2.72439813298371,2.72634841073006,2.729670863345,2.73865032547288,2.83976376572276,
2.9551196832462,3.05433574594742,3.09547300106072,3.11732491861376,3.1206393505533,
3.12364584529936,3.12585505198356,3.12789202681393,3.13065087876145,3.13741510773507,
3.20645352418863,3.25260723367752,3.4387062212664,3.49512619324314,3.5258289055587,
3.5408214416601,3.54349361777068,3.54491600232031,3.5460872255496,3.54727012421086,
3.54945174029345,3.5567892729209,3.67653313056764,3.81568535251143,3.87129584491105,
3.92478241940949,3.93471742191485,3.93802319206267,3.94016244725309,3.94218066509392,
3.9448393924993,3.95076245520002,3.99990826628503,4.22359519879862,4.28373841163122,
4.32227091207181,4.33908595569833,4.34170184654556,4.34306010170982,4.34417431215424,
4.34546442504321,4.34766006975108,4.35566255940737,4.47654171720973,4.64038946849911,
4.75667794043611,4.76321816704555,4.76608841835433,4.76820219842565,4.77015453181233,
4.77280381456673,4.77932423148728,4.84748642893328,4.87037140727346,4.8788673160922,
4.98139134278997,5.14531532735059,5.15665336676671,5.16001447698011,5.1620052242881,
5.16374892828331,5.16593969809426,5.17022485130362,5.19970443713107,5.27726514978158,
5.44431443312162,5.52431215092603,5.53553307700073,5.5406149550474,5.54448974281139,
5.54862003062171,5.55506312165651,5.57507980679941,5.68661065923917,5.89651443824823,
5.90569785796369,5.90854715407342,5.91009615043434,5.91147849042039,5.9132828273197,
5.91650832437957,5.93174749687171,5.96149087625891,5.9922912685522,6.11077851938026,
6.23715942429661,6.23927010688217,6.24793280342784,6.31190386383668,6.31815557364956,
6.32118908665647,6.32334959657339,6.32539296555707,6.32823784484381,6.33392535460176,
6.37796842523448,6.47450432278688,6.56816988174891,6.72501553541103,6.73532904805074,
6.73857161284296,6.74057147259473,6.7423623258137,6.74464164425599,6.74912177160998,
6.78099553177467,6.87147850064111,6.95099692710767,7.13967902450119,7.16577493780009,
7.17544117848804,7.18236514832674,7.18972046648128,7.19953733853387,7.22160814647065,
7.3945903814351,7.48542570592058,7.49347161362858,7.49739272407579,7.50046569330726,
7.50377792092347,7.5090728477986,7.53023393725348,7.73913262105028,7.78620643959158,
7.79811272042643,7.80505675117524,7.81105029350359,7.81837926069913,7.83243985840723,
7.93996851827831,8.04576189461681,8.18657821314542,8.25188675567935,8.25796481255288,
8.26072294080131,8.26275174612017,8.26463997345015,8.26762458904398,8.27509840482735,
8.36834042332271,8.59722044716719,8.65326895592211,8.65978641275396,8.66243275510679,
8.66464292865305,8.66691339757199,8.67023519796964,8.67903966178091,8.79618114460997,
8.82774313442611,8.85243375918805,8.87282024726062,8.89016240359095,8.90519918130994,
8.91841622666362,8.95818791685082,9.04711978092511,9.05480762654373,9.07014273108751,
9.0799142995929,9.08213772613291,9.08359105855612,9.08469443705782,9.085979975628,
9.08808227811472,9.09557441444737,9.1081063990997,9.12993190802072,9.17381503759162,
9.45608280641075,9.47227975825498,9.47601290693852,9.47846407155866,9.48044920279866,
9.48271851362884,9.48660984712489,9.50222223923292,9.66609898221339,9.80467429081347,
9.8120493494853,9.87572038823951,9.87971391329847,9.88120808578717,9.88227448145145,
9.88335046319597,9.88444533578335,9.8858612038,9.88807395688612,9.90387815808587,
9.95827008045819),.UNSPECIFIED.);
#3561=B_SPLINE_CURVE_WITH_KNOTS('',3,(#226621,#226622,#226623,#226624,#226625,
#226626,#226627,#226628,#226629,#226630,#226631,#226632,#226633,#226634,
#226635,#226636,#226637,#226638,#226639,#226640,#226641,#226642,#226643,
#226644,#226645,#226646,#226647,#226648,#226649,#226650,#226651,#226652,
#226653,#226654,#226655,#226656,#226657,#226658,#226659,#226660,#226661,
#226662,#226663,#226664,#226665,#226666,#226667,#226668,#226669,#226670,
#226671,#226672,#226673,#226674,#226675,#226676,#226677,#226678,#226679,
#226680,#226681,#226682,#226683,#226684,#226685,#226686,#226687,#226688,
#226689,#226690,#226691,#226692,#226693,#226694,#226695,#226696,#226697,
#226698,#226699,#226700,#226701,#226702,#226703,#226704,#226705,#226706,
#226707,#226708,#226709,#226710,#226711,#226712,#226713,#226714,#226715,
#226716,#226717,#226718,#226719,#226720,#226721,#226722,#226723,#226724,
#226725,#226726,#226727,#226728,#226729,#226730,#226731,#226732,#226733,
#226734,#226735,#226736,#226737,#226738,#226739,#226740,#226741,#226742,
#226743,#226744,#226745,#226746,#226747,#226748,#226749,#226750,#226751,
#226752,#226753,#226754,#226755,#226756,#226757,#226758,#226759,#226760,
#226761,#226762,#226763,#226764,#226765,#226766,#226767,#226768,#226769,
#226770,#226771,#226772,#226773,#226774,#226775,#226776,#226777,#226778,
#226779,#226780,#226781,#226782,#226783,#226784,#226785,#226786,#226787,
#226788,#226789,#226790,#226791,#226792,#226793,#226794,#226795,#226796,
#226797,#226798,#226799,#226800,#226801,#226802,#226803,#226804,#226805,
#226806,#226807,#226808,#226809,#226810,#226811,#226812,#226813,#226814,
#226815,#226816,#226817,#226818,#226819,#226820,#226821,#226822,#226823,
#226824,#226825,#226826,#226827,#226828,#226829,#226830,#226831,#226832,
#226833,#226834,#226835,#226836,#226837,#226838,#226839,#226840,#226841,
#226842,#226843,#226844,#226845,#226846,#226847,#226848,#226849,#226850,
#226851,#226852,#226853,#226854,#226855,#226856,#226857,#226858,#226859,
#226860,#226861,#226862,#226863,#226864,#226865,#226866,#226867,#226868,
#226869,#226870,#226871,#226872,#226873,#226874,#226875,#226876,#226877,
#226878,#226879),.UNSPECIFIED.,.F.,.F.,(4,3,3,3,3,3,3,3,3,3,3,3,3,3,3,3,
3,3,3,3,3,3,3,3,3,3,3,3,3,3,3,3,3,3,3,3,3,3,3,3,3,3,3,3,3,3,3,3,3,3,3,3,
3,3,3,3,3,3,3,3,3,3,3,3,3,3,3,3,3,3,3,3,3,3,3,3,3,3,3,3,3,3,3,3,3,3,4),
(302.716543450764,302.789903215031,302.863182747746,302.936396853066,303.009560278126,
303.085475206124,303.158589582007,303.23170097055,303.304822643183,303.377967876696,
303.451183102599,303.524439931745,303.597783837003,303.616879702104,303.697873681488,
303.778750719554,303.863125432175,303.943683826104,304.024118368083,304.104377785666,
304.116249570035,304.190653873251,304.265074944053,304.339525055503,304.414057090776,
304.488633531045,304.563314477813,304.615619437966,304.692190981333,304.768694873943,
304.845142068533,304.921543477559,304.997909980536,305.074966129697,305.151303519778,
305.227640391075,305.303986599292,305.381579742926,305.457998854666,305.536179014247,
305.614359173828,305.688136264652,305.761851042085,305.835516576372,305.909146721459,
305.982755345264,306.056368163069,306.113729041759,306.19516257284,306.276731567837,
306.3608234033,306.442666109795,306.527882509743,306.61309890969,306.691531853187,
306.769895037067,306.848193302346,306.926412568203,307.004581859708,307.082693184795,
307.112468777621,307.188831248704,307.265210574786,307.341616340427,307.418091012518,
307.494603060247,307.571197389472,307.611838645552,307.68721602449,307.762531857889,
307.8377989675,307.913030142583,307.988238147729,308.066030676939,308.141248853122,
308.2164837287,308.291746872247,308.367049865591,308.442442061547,308.517886960896,
308.593430321996,308.610578381415,308.691791755436,308.772652942617,308.853304139261,
308.933615080475,308.999728757943),.UNSPECIFIED.);
#3562=B_SPLINE_CURVE_WITH_KNOTS('',3,(#226881,#226882,#226883,#226884,#226885,
#226886,#226887,#226888,#226889,#226890,#226891,#226892,#226893,#226894,
#226895,#226896,#226897,#226898),.UNSPECIFIED.,.F.,.F.,(4,2,2,2,2,2,2,2,
4),(308.999728757943,309.834645669838,310.669562581733,311.504479493628,
312.339396405523,313.174313317418,314.009230229313,314.844147141208,315.282914065123),
 .UNSPECIFIED.);
#3563=B_SPLINE_CURVE_WITH_KNOTS('',3,(#226900,#226901,#226902,#226903,#226904,
#226905,#226906,#226907,#226908,#226909,#226910,#226911,#226912),
 .UNSPECIFIED.,.F.,.F.,(4,1,1,1,1,1,1,1,1,1,4),(315.282914065123,315.60175653245,
316.600496268312,317.599236004174,318.098605872105,318.597975740036,319.596715475899,
320.09608534383,320.595455211761,321.094825079692,321.566099372303),
 .UNSPECIFIED.);
#3564=B_SPLINE_CURVE_WITH_KNOTS('',3,(#226914,#226915,#226916,#226917,#226918,
#226919,#226920,#226921,#226922,#226923,#226924,#226925,#226926,#226927),
 .UNSPECIFIED.,.F.,.F.,(4,2,1,1,1,1,1,1,1,1,4),(321.566099372303,321.594194947623,
322.592934683485,323.591674419347,324.59041415521,325.089784023141,325.589153891072,
326.587893626934,327.087263494865,327.586633362796,327.849284679482),
 .UNSPECIFIED.);
#3565=B_SPLINE_CURVE_WITH_KNOTS('',3,(#226929,#226930,#226931,#226932,#226933,
#226934,#226935,#226936,#226937,#226938,#226939,#226940,#226941,#226942,
#226943,#226944,#226945,#226946,#226947,#226948,#226949,#226950,#226951,
#226952,#226953,#226954,#226955,#226956,#226957,#226958,#226959,#226960,
#226961,#226962,#226963,#226964,#226965,#226966,#226967,#226968,#226969,
#226970,#226971,#226972,#226973,#226974,#226975,#226976,#226977,#226978,
#226979,#226980,#226981,#226982,#226983,#226984,#226985,#226986,#226987,
#226988,#226989,#226990,#226991,#226992,#226993,#226994,#226995,#226996,
#226997,#226998,#226999,#227000,#227001,#227002,#227003,#227004,#227005,
#227006,#227007,#227008,#227009,#227010,#227011,#227012,#227013,#227014,
#227015,#227016,#227017,#227018,#227019,#227020,#227021,#227022,#227023,
#227024,#227025,#227026,#227027,#227028,#227029,#227030,#227031,#227032,
#227033,#227034,#227035,#227036,#227037,#227038,#227039,#227040,#227041,
#227042,#227043,#227044,#227045,#227046,#227047,#227048,#227049,#227050,
#227051,#227052,#227053,#227054,#227055,#227056,#227057,#227058,#227059,
#227060,#227061,#227062,#227063,#227064,#227065,#227066,#227067,#227068,
#227069,#227070,#227071,#227072,#227073,#227074,#227075,#227076,#227077,
#227078,#227079,#227080,#227081,#227082,#227083,#227084,#227085,#227086,
#227087,#227088,#227089,#227090,#227091,#227092,#227093,#227094,#227095,
#227096,#227097,#227098,#227099,#227100,#227101,#227102,#227103,#227104,
#227105,#227106,#227107,#227108,#227109,#227110,#227111,#227112,#227113,
#227114,#227115,#227116,#227117,#227118,#227119,#227120,#227121,#227122,
#227123,#227124,#227125,#227126,#227127,#227128,#227129,#227130,#227131,
#227132,#227133,#227134,#227135,#227136,#227137,#227138,#227139,#227140,
#227141,#227142,#227143,#227144,#227145,#227146,#227147,#227148,#227149,
#227150,#227151,#227152,#227153,#227154,#227155,#227156,#227157,#227158,
#227159,#227160,#227161,#227162,#227163,#227164,#227165,#227166,#227167,
#227168,#227169,#227170,#227171,#227172,#227173,#227174,#227175,#227176,
#227177,#227178,#227179,#227180,#227181,#227182,#227183,#227184,#227185,
#227186,#227187,#227188,#227189,#227190,#227191,#227192,#227193,#227194,
#227195,#227196,#227197,#227198,#227199,#227200,#227201,#227202,#227203,
#227204,#227205,#227206,#227207,#227208,#227209,#227210,#227211,#227212,
#227213,#227214,#227215,#227216,#227217,#227218,#227219,#227220,#227221,
#227222,#227223,#227224,#227225,#227226,#227227,#227228,#227229,#227230,
#227231,#227232,#227233,#227234,#227235,#227236,#227237,#227238,#227239,
#227240,#227241,#227242,#227243,#227244,#227245,#227246,#227247,#227248,
#227249,#227250,#227251,#227252,#227253,#227254,#227255,#227256,#227257,
#227258,#227259,#227260,#227261,#227262,#227263,#227264,#227265,#227266,
#227267,#227268,#227269,#227270,#227271,#227272,#227273,#227274,#227275,
#227276,#227277,#227278,#227279,#227280,#227281,#227282,#227283,#227284,
#227285,#227286,#227287,#227288,#227289,#227290,#227291,#227292,#227293,
#227294,#227295,#227296,#227297,#227298,#227299,#227300,#227301,#227302,
#227303,#227304,#227305,#227306,#227307,#227308,#227309,#227310,#227311,
#227312,#227313,#227314,#227315,#227316,#227317,#227318,#227319,#227320,
#227321,#227322,#227323,#227324,#227325,#227326,#227327,#227328,#227329,
#227330,#227331,#227332,#227333,#227334,#227335,#227336,#227337,#227338,
#227339,#227340,#227341,#227342,#227343,#227344,#227345,#227346,#227347,
#227348,#227349,#227350,#227351,#227352,#227353,#227354,#227355,#227356,
#227357,#227358,#227359,#227360,#227361,#227362,#227363,#227364,#227365,
#227366,#227367,#227368,#227369,#227370,#227371,#227372,#227373,#227374,
#227375,#227376,#227377,#227378,#227379,#227380,#227381,#227382,#227383,
#227384,#227385,#227386,#227387,#227388,#227389,#227390,#227391,#227392,
#227393,#227394,#227395,#227396,#227397,#227398,#227399,#227400,#227401,
#227402,#227403,#227404,#227405,#227406,#227407,#227408,#227409,#227410,
#227411,#227412,#227413,#227414,#227415,#227416,#227417,#227418,#227419,
#227420,#227421,#227422,#227423,#227424,#227425,#227426,#227427,#227428,
#227429,#227430,#227431,#227432,#227433,#227434,#227435,#227436,#227437,
#227438,#227439,#227440,#227441,#227442,#227443,#227444,#227445,#227446,
#227447,#227448,#227449,#227450,#227451,#227452),.UNSPECIFIED.,.F.,.F.,
(4,2,2,2,2,2,2,2,2,2,2,2,2,2,2,2,2,2,2,2,2,2,2,2,2,2,2,2,2,2,2,2,2,2,2,
2,2,2,2,2,2,2,2,2,2,2,2,2,2,2,2,2,2,2,2,2,2,2,2,2,2,2,2,2,2,2,2,2,2,2,2,
2,2,2,2,2,2,2,2,2,2,2,2,2,2,2,2,2,2,2,2,2,2,2,2,2,2,2,2,2,2,2,2,2,2,2,2,
2,2,2,2,2,2,2,2,2,2,2,2,2,2,2,2,2,2,2,2,2,2,2,2,2,2,2,2,2,2,2,2,2,2,2,2,
2,2,2,2,2,2,2,2,2,2,2,2,2,2,2,2,2,2,2,2,2,2,2,2,2,2,2,2,2,2,2,2,2,2,2,2,
2,2,2,2,2,2,2,2,2,2,2,2,2,2,2,2,2,2,2,2,2,2,2,2,2,2,2,2,2,2,2,2,2,2,2,2,
2,2,2,2,2,2,2,2,2,2,2,2,2,2,2,2,2,2,2,2,2,2,2,2,2,2,2,2,2,2,2,2,2,2,2,2,
2,2,2,2,2,2,2,2,2,2,4),(0.00141745760897423,0.067162311283536,0.0780209552792477,
0.0851854906335986,0.0909210426250336,0.0968707264688579,0.103770083128768,
0.115494274022767,0.16237726379872,0.206207364650622,0.456623595264774,
0.515771718959542,0.541705696762699,0.546296033793239,0.548743640484823,
0.550743266418886,0.552779534906327,0.556530540707647,0.568631379334648,
0.729403105854545,0.782206725727187,0.839959053698312,0.910649773391808,
0.942586920948702,0.947704008334611,0.950368297643282,0.952532398783485,
0.954693798396332,0.958610983339168,0.97076891749642,1.14727277420351,1.23861232553984,
1.25127341753228,1.29295222246926,1.35877106132461,1.36769669441332,1.3699717109283,
1.37130726202381,1.37248079233919,1.3739364354681,1.37616408280461,1.38660790323757,
1.55435250822876,1.62359624571914,1.70728969075542,1.7409323688155,1.7530317453309,
1.75866975621739,1.76321455138327,1.76562750368209,1.76741959033857,1.76937143843708,
1.7728092133636,1.78279952483596,1.93040389735508,2.09480521253811,2.15768215265109,
2.16610157981944,2.16823014245425,2.16948636191472,2.17060432891969,2.17200979688767,
2.17419824471008,2.18440272010436,2.34513614150874,2.43847169427428,2.54388013707765,
2.58478491107501,2.590038248084,2.5926623072679,2.59454558218568,2.59653539051702,
2.59988731414479,2.60873923020928,2.74252500115857,2.86549427911651,2.97956761389034,
2.98492186811423,2.9873216337073,2.98910911048775,2.99077506111053,2.99305918913317,
2.99760158217403,3.03701411894509,3.22612515087694,3.33766817538262,3.35837177010574,
3.36501771431343,3.36919256894291,3.37305095147414,3.37802797119256,3.38873979701807,
3.4757667471831,3.60055926291225,3.702950785543,3.73007942154706,3.7338748728155,
3.73580055193312,3.73719431648433,3.73867797233158,3.74077693905783,3.74641995038451,
3.83459759229004,4.01592119297889,4.13803885224389,4.14501723412619,4.14811057371096,
4.15040092801254,4.15252510392066,4.15542110210616,4.162617729655,4.24217153457634,
4.4358174930071,4.49556434090439,4.53838244230649,4.56023523738886,4.56430251842368,
4.56649519939402,4.56813896253032,4.57020752468113,4.57371001678128,4.5856709199006,
4.59159097026156,4.59331528643355,4.76381405634778,4.88682837056718,4.98028744093667,
4.99556685502615,5.00495325654838,5.0122489791179,5.02032685882555,5.03369440147927,
5.08517552972484,5.18151594937427,5.30495942465799,5.31769911541664,5.32255699349876,
5.32546419180189,5.32853934239581,5.33259872032313,5.34214047037631,5.35572723109848,
5.39412830013317,5.52175314488656,5.56710689104154,5.61258119114196,5.62435653636009,
5.63127137982623,5.63726839234622,5.6446380237003,5.65889228698797,5.770932609268,
5.87746043311761,6.02576122481904,6.07851227678507,6.08445768173807,6.08714766808781,
6.08919904876443,6.0913832968761,6.09477985555712,6.10516305429029,6.15876632597075,
6.24280588310666,6.46947438593558,6.48346970680589,6.48761000085326,6.49006121147773,
6.49201149376827,6.49461691240164,6.49945868165752,6.52550465786664,6.57610237741566,
6.63504187202422,6.78934347291348,6.89954243926188,6.906839317458,6.90904993043202,
6.91023895192103,6.91140975623648,6.9128229400933,6.91545307037718,6.93107247920207,
6.93328937158055,6.97493539267457,7.12297310878393,7.23410455741389,7.29489494242167,
7.30104036424938,7.30356121067752,7.30542765906325,7.30745691844026,7.31022745077674,
7.31660585254173,7.37854628083601,7.41027894943964,7.5559193336004,7.69551565805991,
7.70455618857236,7.70682508324113,7.70812429905798,7.70922714750612,7.71056875669458,
7.71305839952144,7.7263145601904,7.75296164178759,7.80388452792607,7.91448178713277,
8.05145589969884,8.1211847484972,8.1277631866839,8.1304223377097,8.13237700972853,
8.13448857988451,8.13734730496074,8.14382485807563,8.26418415364691,8.40681007728003,
8.51264947398095,8.52188549783611,8.5249830537626,8.52672108417959,8.52846436419277,
8.53065237165202,8.53450719646242,8.55684285072358,8.60567549590081,8.73500394118451,
8.7944338573327,8.88825211858894,8.89875428431989,8.9038805227842,8.90754078777543,
8.91140082415158,8.91516033387907,8.92005701272533,8.94123735031426,8.97412411999817,
9.0572858725404,9.1244380607312,9.24036186541586,9.26775909043428,9.27190596608096,
9.27390233855925,9.27544973540007,9.27714746044654,9.2788859841696,9.28142499662682,
9.30442331369998,9.37414146134346,9.42320007992591,9.60208625751048,9.6104970471058,
9.67612638090174,9.68241991592185,9.6854634356422,9.68762640874013,9.68966831733391,
9.69250513700915,9.69815463790678,9.74091386502713,9.8504320272541,9.95730281891779),
 .UNSPECIFIED.);
#3566=B_SPLINE_CURVE_WITH_KNOTS('',3,(#227454,#227455,#227456,#227457,#227458,
#227459,#227460,#227461,#227462,#227463,#227464,#227465,#227466,#227467,
#227468,#227469,#227470,#227471),.UNSPECIFIED.,.F.,.F.,(4,2,2,2,2,2,2,2,
4),(340.415655293841,341.250572205736,342.085489117631,342.920406029526,
343.755322941421,344.590239853316,345.425156765211,346.260073677105,346.698657753416),
 .UNSPECIFIED.);
#3567=B_SPLINE_CURVE_WITH_KNOTS('',3,(#227473,#227474,#227475,#227476,#227477,
#227478,#227479,#227480,#227481,#227482,#227483,#227484,#227485,#227486,
#227487,#227488,#227489,#227490,#227491,#227492,#227493,#227494,#227495,
#227496,#227497,#227498,#227499,#227500,#227501,#227502,#227503,#227504,
#227505,#227506,#227507,#227508,#227509,#227510,#227511,#227512,#227513,
#227514,#227515,#227516,#227517,#227518,#227519,#227520,#227521,#227522,
#227523,#227524,#227525,#227526,#227527,#227528,#227529,#227530,#227531,
#227532,#227533,#227534,#227535,#227536,#227537,#227538,#227539,#227540,
#227541,#227542,#227543,#227544,#227545,#227546,#227547,#227548,#227549,
#227550,#227551,#227552,#227553,#227554,#227555,#227556,#227557,#227558,
#227559,#227560,#227561,#227562,#227563,#227564,#227565,#227566,#227567,
#227568,#227569,#227570,#227571,#227572,#227573,#227574,#227575,#227576,
#227577,#227578,#227579,#227580,#227581,#227582,#227583,#227584,#227585,
#227586,#227587,#227588,#227589,#227590,#227591,#227592,#227593,#227594,
#227595,#227596,#227597,#227598,#227599,#227600,#227601,#227602,#227603,
#227604,#227605,#227606,#227607,#227608,#227609,#227610,#227611,#227612,
#227613,#227614,#227615,#227616,#227617,#227618,#227619,#227620,#227621,
#227622,#227623,#227624,#227625,#227626,#227627,#227628,#227629,#227630,
#227631,#227632,#227633,#227634,#227635,#227636,#227637,#227638,#227639,
#227640,#227641,#227642,#227643,#227644,#227645,#227646,#227647,#227648,
#227649,#227650,#227651,#227652,#227653,#227654,#227655,#227656,#227657,
#227658,#227659,#227660,#227661,#227662,#227663,#227664,#227665,#227666,
#227667,#227668,#227669,#227670,#227671,#227672,#227673,#227674,#227675,
#227676,#227677,#227678,#227679,#227680,#227681,#227682,#227683,#227684,
#227685,#227686,#227687,#227688,#227689,#227690,#227691,#227692,#227693,
#227694,#227695,#227696,#227697,#227698,#227699,#227700,#227701,#227702,
#227703,#227704,#227705,#227706,#227707,#227708,#227709,#227710,#227711,
#227712,#227713,#227714,#227715,#227716,#227717,#227718,#227719,#227720,
#227721,#227722,#227723,#227724,#227725,#227726,#227727,#227728,#227729,
#227730,#227731,#227732,#227733,#227734),.UNSPECIFIED.,.F.,.F.,(4,3,3,3,
3,3,3,3,3,3,3,3,3,3,3,3,3,3,3,3,3,3,3,3,3,3,3,3,3,3,3,3,3,3,3,3,3,3,3,3,
3,3,3,3,3,3,3,3,3,3,3,3,3,3,3,3,3,3,3,3,3,3,3,3,3,3,3,3,3,3,3,3,3,3,3,3,
3,3,3,3,3,3,3,3,3,3,3,4),(346.698953041191,346.774312894999,346.849606692114,
346.924847356439,347.000047776703,347.075224878317,347.150390746122,347.22555702008,
347.300735338305,347.375965001418,347.451223462602,347.526553270498,347.56142808004,
347.635205170864,347.708919948298,347.782585482584,347.856215627671,347.929824251476,
348.003437069281,348.060797947971,348.142231479052,348.223800474049,348.307892309512,
348.389735016008,348.474951415955,348.560167815902,348.638600759399,348.716963943279,
348.795262208557,348.873481474414,348.951650765919,349.029762091005,349.059537683833,
349.135900154916,349.212279480999,349.288685246639,349.365159918731,349.441671966459,
349.518266295685,349.558907551764,349.634284930701,349.709600764101,349.784867873711,
349.860099048794,349.935307053938,350.013099583149,350.088317759332,350.163552634909,
350.238815778455,350.314118771799,350.389510967755,350.464955867104,350.540499228203,
350.557647287626,350.630791096602,350.703846109716,350.776827264111,350.849749426759,
350.922627410056,350.995475985878,351.068323386895,351.141173733045,351.214040373102,
351.286936666527,351.359918806511,351.432947707244,351.506087260815,351.556387023489,
351.630975642714,351.705478613094,351.779909870854,351.854283304733,351.928612765146,
352.002912072902,352.077205434053,352.151498983122,352.225805213731,352.300136623861,
352.374540666731,352.448986319046,352.523522877136,352.555126759351,352.63852443211,
352.724399776288,352.807379818993,352.89017442231,352.972685446835,352.982025808824),
 .UNSPECIFIED.);
#3568=B_SPLINE_CURVE_WITH_KNOTS('',3,(#227736,#227737,#227738,#227739,#227740,
#227741,#227742,#227743,#227744,#227745,#227746,#227747,#227748),
 .UNSPECIFIED.,.F.,.F.,(4,1,1,1,1,1,1,1,1,1,4),(352.9820259082,353.054496627282,
353.553866495213,354.552606231075,355.051976099006,355.551345966937,356.050715834868,
356.550085702799,357.548825438662,358.547565174524,359.26521121538),
 .UNSPECIFIED.);
#3569=B_SPLINE_CURVE_WITH_KNOTS('',3,(#227750,#227751,#227752,#227753,#227754,
#227755,#227756,#227757,#227758,#227759,#227760,#227761,#227762,#227763,
#227764,#227765,#227766,#227767,#227768,#227769,#227770,#227771,#227772,
#227773,#227774,#227775,#227776,#227777,#227778,#227779,#227780,#227781,
#227782,#227783,#227784,#227785,#227786,#227787,#227788,#227789,#227790,
#227791,#227792,#227793,#227794,#227795,#227796,#227797,#227798,#227799,
#227800,#227801,#227802,#227803,#227804,#227805,#227806,#227807,#227808,
#227809,#227810,#227811,#227812,#227813,#227814,#227815,#227816,#227817,
#227818,#227819,#227820,#227821,#227822,#227823,#227824,#227825,#227826,
#227827,#227828,#227829,#227830,#227831,#227832,#227833,#227834,#227835,
#227836,#227837,#227838,#227839,#227840,#227841,#227842,#227843,#227844,
#227845,#227846,#227847,#227848,#227849,#227850,#227851,#227852,#227853,
#227854,#227855,#227856,#227857,#227858,#227859,#227860,#227861,#227862,
#227863,#227864,#227865,#227866,#227867,#227868,#227869,#227870,#227871,
#227872,#227873,#227874,#227875,#227876,#227877,#227878,#227879,#227880,
#227881,#227882,#227883,#227884,#227885,#227886,#227887,#227888,#227889,
#227890,#227891,#227892,#227893,#227894,#227895,#227896,#227897,#227898,
#227899,#227900,#227901,#227902,#227903,#227904,#227905,#227906,#227907,
#227908,#227909,#227910,#227911,#227912,#227913,#227914,#227915,#227916,
#227917,#227918,#227919,#227920,#227921,#227922,#227923,#227924,#227925,
#227926,#227927,#227928,#227929,#227930,#227931,#227932,#227933,#227934,
#227935,#227936,#227937,#227938,#227939,#227940,#227941,#227942,#227943,
#227944,#227945,#227946,#227947,#227948,#227949,#227950,#227951,#227952,
#227953,#227954,#227955,#227956,#227957,#227958,#227959,#227960,#227961,
#227962,#227963,#227964,#227965,#227966,#227967,#227968,#227969,#227970,
#227971,#227972,#227973,#227974,#227975,#227976,#227977,#227978,#227979,
#227980,#227981,#227982,#227983,#227984,#227985,#227986,#227987,#227988,
#227989,#227990,#227991,#227992,#227993,#227994,#227995,#227996,#227997,
#227998,#227999,#228000,#228001,#228002,#228003,#228004,#228005,#228006,
#228007,#228008,#228009,#228010,#228011),.UNSPECIFIED.,.F.,.F.,(4,3,3,3,
3,3,3,3,3,3,3,3,3,3,3,3,3,3,3,3,3,3,3,3,3,3,3,3,3,3,3,3,3,3,3,3,3,3,3,3,
3,3,3,3,3,3,3,3,3,3,3,3,3,3,3,3,3,3,3,3,3,3,3,3,3,3,3,3,3,3,3,3,3,3,3,3,
3,3,3,3,3,3,3,3,3,3,3,4),(359.265211374834,359.351771246646,359.438775330765,
359.526288962694,359.546304910386,359.62729888977,359.708175927836,359.792550640457,
359.873109034386,359.953543576365,360.033802993948,360.045674778317,360.120079081534,
360.194500152335,360.268950263786,360.343482299059,360.418058739327,360.492739686096,
360.545044646248,360.621616189615,360.698120082225,360.774567276814,360.850968685839,
360.927335188816,361.004391337978,361.080728728059,361.157065599356,361.233411807572,
361.311004951207,361.387424062947,361.465604222528,361.54378438211,361.617561472934,
361.691276250369,361.764941784655,361.838571929742,361.912180553548,361.985793371353,
362.043154250042,362.124587781123,362.20615677612,362.290248611583,362.372091318079,
362.457307718026,362.542524117973,362.620957061469,362.699320245349,362.777618510626,
362.855837776482,362.934007067986,363.012118393073,363.041893985904,363.118256456988,
363.19463578307,363.271041548711,363.347516220803,363.424028268532,363.500622597758,
363.541263853835,363.616641232772,363.691957066172,363.767224175782,363.842455350865,
363.91766335601,363.995455885221,364.070674061403,364.145908936981,364.221172080526,
364.29647507387,364.371867269826,364.447312169175,364.522855530275,364.540003589697,
364.613147398672,364.686202411787,364.759183566181,364.832105728829,364.904983712125,
364.977832287947,365.050679688963,365.123530035113,365.19639667517,365.269292968596,
365.342275108579,365.415304009312,365.488443562883,365.538743325559,365.54839652256),
 .UNSPECIFIED.);
#3570=B_SPLINE_CURVE_WITH_KNOTS('',3,(#228013,#228014,#228015,#228016,#228017,
#228018,#228019,#228020,#228021,#228022,#228023,#228024,#228025),
 .UNSPECIFIED.,.F.,.F.,(4,1,1,1,1,1,1,1,1,1,4),(365.548397871087,366.537483061421,
367.036852929352,367.536222797283,368.534962533146,369.034332401077,369.533702269008,
370.033072136939,370.53244200487,371.531181740732,371.831581829739),
 .UNSPECIFIED.);
#3571=B_SPLINE_CURVE_WITH_KNOTS('',3,(#228027,#228028,#228029,#228030,#228031,
#228032,#228033,#228034,#228035,#228036,#228037,#228038,#228039,#228040,
#228041,#228042,#228043,#228044),.UNSPECIFIED.,.F.,.F.,(4,2,2,2,2,2,2,2,
4),(371.831581829739,372.666498741634,373.501415653529,374.336332565424,
375.171249477319,376.006166389214,376.841083301109,377.676000213004,378.114767136919),
 .UNSPECIFIED.);
#3572=B_SPLINE_CURVE_WITH_KNOTS('',3,(#228046,#228047,#228048,#228049,#228050,
#228051,#228052,#228053,#228054,#228055,#228056,#228057,#228058,#228059,
#228060,#228061,#228062,#228063,#228064,#228065,#228066,#228067,#228068,
#228069,#228070,#228071,#228072,#228073,#228074,#228075,#228076,#228077,
#228078,#228079,#228080,#228081,#228082,#228083,#228084,#228085,#228086,
#228087,#228088,#228089,#228090,#228091,#228092,#228093,#228094,#228095,
#228096,#228097,#228098,#228099,#228100,#228101,#228102,#228103,#228104,
#228105,#228106,#228107,#228108,#228109,#228110,#228111,#228112,#228113,
#228114,#228115,#228116,#228117,#228118,#228119,#228120,#228121,#228122,
#228123,#228124,#228125,#228126,#228127,#228128,#228129,#228130,#228131,
#228132,#228133,#228134,#228135,#228136,#228137,#228138,#228139,#228140,
#228141,#228142,#228143,#228144,#228145,#228146,#228147,#228148,#228149,
#228150,#228151,#228152,#228153,#228154,#228155,#228156,#228157,#228158,
#228159,#228160,#228161,#228162,#228163,#228164,#228165,#228166,#228167,
#228168,#228169,#228170,#228171,#228172,#228173,#228174,#228175,#228176,
#228177,#228178,#228179,#228180,#228181,#228182,#228183,#228184,#228185,
#228186,#228187,#228188,#228189,#228190,#228191,#228192,#228193,#228194,
#228195,#228196,#228197,#228198,#228199,#228200,#228201,#228202,#228203,
#228204,#228205,#228206,#228207,#228208,#228209,#228210,#228211,#228212,
#228213,#228214,#228215,#228216,#228217,#228218,#228219,#228220,#228221,
#228222,#228223,#228224,#228225,#228226,#228227,#228228,#228229,#228230,
#228231,#228232,#228233,#228234,#228235,#228236,#228237,#228238,#228239,
#228240,#228241,#228242,#228243,#228244,#228245,#228246,#228247,#228248,
#228249,#228250,#228251,#228252,#228253,#228254,#228255,#228256,#228257,
#228258,#228259,#228260,#228261,#228262,#228263,#228264,#228265,#228266,
#228267,#228268,#228269,#228270,#228271,#228272,#228273,#228274,#228275,
#228276,#228277,#228278,#228279,#228280,#228281,#228282,#228283,#228284,
#228285,#228286,#228287,#228288,#228289,#228290,#228291,#228292,#228293,
#228294,#228295,#228296,#228297,#228298,#228299,#228300,#228301,#228302,
#228303,#228304,#228305,#228306,#228307,#228308,#228309,#228310,#228311,
#228312,#228313,#228314,#228315,#228316,#228317,#228318,#228319,#228320,
#228321,#228322,#228323,#228324,#228325,#228326,#228327,#228328,#228329,
#228330,#228331,#228332,#228333,#228334,#228335,#228336,#228337,#228338,
#228339,#228340,#228341,#228342,#228343,#228344,#228345,#228346,#228347,
#228348,#228349,#228350,#228351,#228352,#228353,#228354,#228355,#228356,
#228357,#228358,#228359,#228360,#228361,#228362,#228363,#228364,#228365,
#228366,#228367,#228368,#228369,#228370,#228371,#228372,#228373,#228374,
#228375,#228376,#228377,#228378,#228379,#228380,#228381,#228382,#228383,
#228384,#228385,#228386,#228387,#228388,#228389,#228390,#228391,#228392,
#228393,#228394,#228395,#228396,#228397,#228398,#228399,#228400,#228401,
#228402,#228403,#228404,#228405,#228406,#228407,#228408,#228409,#228410,
#228411,#228412,#228413,#228414,#228415,#228416,#228417,#228418,#228419,
#228420,#228421,#228422,#228423,#228424,#228425,#228426,#228427,#228428,
#228429,#228430,#228431,#228432,#228433,#228434,#228435,#228436,#228437,
#228438,#228439,#228440,#228441,#228442,#228443,#228444,#228445,#228446,
#228447,#228448,#228449,#228450,#228451,#228452,#228453,#228454,#228455,
#228456,#228457,#228458,#228459,#228460,#228461,#228462,#228463,#228464,
#228465,#228466,#228467,#228468,#228469,#228470,#228471,#228472,#228473,
#228474,#228475,#228476,#228477,#228478,#228479,#228480,#228481,#228482,
#228483,#228484,#228485,#228486,#228487,#228488,#228489,#228490,#228491,
#228492,#228493,#228494,#228495,#228496,#228497,#228498,#228499,#228500,
#228501,#228502,#228503,#228504,#228505,#228506,#228507,#228508,#228509,
#228510,#228511,#228512,#228513,#228514,#228515,#228516,#228517,#228518,
#228519,#228520,#228521,#228522,#228523,#228524,#228525,#228526,#228527,
#228528,#228529,#228530,#228531,#228532,#228533,#228534,#228535,#228536,
#228537,#228538,#228539,#228540,#228541,#228542,#228543,#228544,#228545,
#228546,#228547,#228548,#228549,#228550,#228551,#228552,#228553,#228554,
#228555,#228556,#228557,#228558,#228559,#228560,#228561,#228562,#228563,
#228564,#228565,#228566,#228567,#228568,#228569,#228570,#228571,#228572,
#228573,#228574,#228575,#228576,#228577),.UNSPECIFIED.,.F.,.F.,(4,2,2,2,
2,2,2,2,2,2,2,2,2,2,2,2,2,2,2,2,2,2,2,2,2,2,2,2,2,2,2,2,2,2,2,2,2,2,2,2,
2,2,2,2,2,2,2,2,2,2,2,2,2,2,2,2,2,2,2,2,2,2,2,2,2,2,2,2,2,2,2,2,2,2,2,2,
2,2,2,2,2,2,2,2,2,2,2,2,2,2,2,2,2,2,2,2,2,2,2,2,2,2,2,2,2,2,2,2,2,2,2,2,
2,2,2,2,2,2,2,2,2,2,2,2,2,2,2,2,2,2,2,2,2,2,2,2,2,2,2,2,2,2,2,2,2,2,2,2,
2,2,2,2,2,2,2,2,2,2,2,2,2,2,2,2,2,2,2,2,2,2,2,2,2,2,2,2,2,2,2,2,2,2,2,2,
2,2,2,2,2,2,2,2,2,2,2,2,2,2,2,2,2,2,2,2,2,2,2,2,2,2,2,2,2,2,2,2,2,2,2,2,
2,2,2,2,2,2,2,2,2,2,2,2,2,2,2,2,2,2,2,2,2,2,2,2,2,2,2,2,2,2,2,2,2,2,2,2,
2,2,2,2,2,2,2,2,2,4),(0.00193034970426769,0.251769396345977,0.307891382236222,
0.316094863725038,0.318304129568899,0.319624845655523,0.320800202296045,
0.322277821764209,0.324576538969347,0.336011088366562,0.526210819881589,
0.627146546913494,0.679015458140233,0.697261508663907,0.704918787823994,
0.708942333462824,0.71236269399982,0.714508820411928,0.716422074763476,
0.71896165887763,0.724119115451281,0.754827416334772,0.855377445575457,
0.913468041963251,1.02182672019539,1.06417651461188,1.10754885551415,1.1143892613705,
1.1163676333868,1.11759151760635,1.11871635257558,1.12015632429706,1.12319993798314,
1.14340608252472,1.39324747618811,1.47245014954148,1.51280083785537,1.52686501275496,
1.5332437090269,1.53828118864638,1.54084079689098,1.54272164275102,1.54471464758234,
1.54752003513558,1.553324502198,1.61384341876806,1.74665762394975,1.85129426279119,
1.919846964539,1.93106700551334,1.93426960922784,1.93622449476669,1.93799070418438,
1.9402478494948,1.94470907225781,1.97145037102271,2.03268553921962,2.15004691225555,
2.22624741731643,2.29263519605128,2.30773765786598,2.31356555778627,2.31756287220201,
2.32144540522662,2.32614384381588,2.33715087961591,2.44894720632182,2.5774752340157,
2.67388587805365,2.68025247428209,2.68262848223882,2.68424450269457,2.68581142784186,
2.68767951432188,2.69224364650306,2.74067282460147,2.86836179220626,2.99440542087378,
3.07663044854312,3.0856210707495,3.09235955996217,3.09539870362877,3.0976899824399,
3.0998114797624,3.1026983944094,3.10984494589131,3.18724710976461,3.3234455339535,
3.43528251243566,3.48450070172673,3.50722820752353,3.51133755057011,3.51353887845412,
3.51535951598177,3.51720663445849,3.5206354633706,3.53196523777127,3.57280785946028,
3.70178657267434,3.83030678424797,3.92673972889401,3.94394864184916,3.95282829890369,
3.95937563719589,3.96753230187217,3.98126635160781,4.03067859941869,4.03852950046107,
4.07821319859314,4.1939951579044,4.25943941532161,4.26705086177669,4.27087517692903,
4.27363155463765,4.27655745285908,4.28069402265697,4.29331673539156,4.40451960396545,
4.55042695309604,4.5677947601653,4.57577536386716,4.58183807353924,4.58759456358594,
4.5956897185081,4.61758145167919,4.87590566985032,4.9788856913442,5.02579199541689,
5.03100494687026,5.0336272507417,5.03554120493761,5.03759635654019,5.04035902402382,
5.04654081505736,5.13814868412498,5.35684901036038,5.42593205335334,5.43267919995992,
5.43543473533897,5.43747058301688,5.43967985397271,5.44268886356742,5.44958518670571,
5.56854474825664,5.74935865021088,5.7825841352723,5.79748994768594,5.82805126021636,
5.84537470010864,5.85356447532792,5.85584884176459,5.85719941702674,5.85837099742916,
5.85980492261539,5.86253385625708,5.8806626475182,5.92398864901478,5.97913633837282,
6.14508326446712,6.19695932396676,6.24245218713914,6.24824589412459,6.25088032426205,
6.25289404541378,6.25504201828088,6.25838886946113,6.26865441706738,6.32486041346161,
6.37007819592485,6.51717304195755,6.57869895642406,6.5971396361932,6.62540158775356,
6.64983137868104,6.65268563856773,6.65411539495785,6.65516558565209,6.6563030623871,
6.65784786335825,6.6613673856847,6.78306040763654,6.91113060472586,7.06276880506085,
7.07308796367761,7.07665884709422,7.07869144382003,7.0805608844206,7.08308283750937,
7.08784887893496,7.11541533358484,7.14128200980715,7.23600266099889,7.3645336356411,
7.46206803261948,7.46911323842904,7.47160394636142,7.47332526822798,7.47491171580678,
7.47705711388727,7.48112806873204,7.50474857740392,7.55733803551137,7.7887734298149,
7.83801727121392,7.84675394090786,7.85187659955578,7.85575699457646,7.85931865811554,
7.86509484915785,7.88029003323125,7.90186502312458,7.97149602376957,8.09422951602577,
8.19207187906817,8.21474939099986,8.21861894205266,8.22058577526896,8.22212908958517,
8.22384158163449,8.22665672402663,8.23638169109511,8.25214869671166,8.30547477782331,
8.41041806471349,8.61388659578707,8.62734289951141,8.63151489439541,8.63378031166291,
8.63602531746479,8.6387555178748,8.64389753281159,8.67321829032837,8.72373655599779,
8.77479711312779,8.83908782135329,8.89667911150504,9.03614580348131,9.04600034025412,
9.04924834682371,9.05105731419524,9.05288065000309,9.05514287557664,9.0595444188461,
9.08863504615795,9.16146252377471,9.23946999706734,9.35493909019988,9.45736964677849,
9.47836148118326,9.48799961413974,9.49534889681019,9.50209872504978,9.50977756025845,
9.53034451817732,9.60822593396827,9.67004957467597,9.78815339424313,9.80113588441011,
9.80602918058808,9.80894172562362,9.81185242129976,9.8148046621534,9.81859783202482,
9.82469671079591,9.83705628883101,9.95375202500103),.UNSPECIFIED.);
#3573=B_SPLINE_CURVE_WITH_KNOTS('',3,(#228579,#228580,#228581,#228582,#228583,
#228584,#228585,#228586,#228587,#228588,#228589,#228590),.UNSPECIFIED.,
 .F.,.F.,(4,1,1,1,1,1,1,1,1,4),(390.681137751278,391.006606590045,391.505976457976,
392.504716193838,393.5034559297,394.502195665562,395.001565533494,395.500935401425,
396.499675137287,396.964023113174),.UNSPECIFIED.);
#3574=B_SPLINE_CURVE_WITH_KNOTS('',3,(#228592,#228593,#228594,#228595,#228596,
#228597,#228598,#228599,#228600,#228601,#228602,#228603,#228604,#228605,
#228606,#228607,#228608,#228609,#228610,#228611,#228612,#228613,#228614,
#228615,#228616,#228617,#228618,#228619,#228620,#228621,#228622,#228623,
#228624,#228625,#228626,#228627,#228628,#228629,#228630,#228631,#228632,
#228633,#228634,#228635,#228636,#228637,#228638,#228639,#228640,#228641,
#228642,#228643,#228644,#228645,#228646,#228647,#228648,#228649,#228650,
#228651,#228652,#228653,#228654,#228655,#228656,#228657,#228658,#228659,
#228660,#228661,#228662,#228663,#228664,#228665,#228666,#228667,#228668,
#228669,#228670,#228671,#228672,#228673,#228674,#228675,#228676,#228677,
#228678,#228679,#228680,#228681,#228682,#228683,#228684,#228685,#228686,
#228687,#228688,#228689,#228690,#228691,#228692,#228693,#228694,#228695,
#228696,#228697,#228698,#228699,#228700,#228701,#228702,#228703,#228704,
#228705,#228706,#228707,#228708,#228709,#228710,#228711,#228712,#228713,
#228714,#228715,#228716,#228717,#228718,#228719,#228720,#228721,#228722,
#228723,#228724,#228725,#228726,#228727,#228728,#228729,#228730,#228731,
#228732,#228733,#228734,#228735,#228736,#228737,#228738,#228739,#228740,
#228741,#228742,#228743,#228744,#228745,#228746,#228747,#228748,#228749,
#228750,#228751,#228752,#228753,#228754,#228755,#228756,#228757,#228758,
#228759,#228760,#228761,#228762,#228763,#228764,#228765,#228766,#228767,
#228768,#228769,#228770,#228771,#228772,#228773,#228774,#228775,#228776,
#228777,#228778,#228779,#228780,#228781,#228782,#228783,#228784,#228785,
#228786,#228787,#228788,#228789,#228790,#228791,#228792,#228793,#228794,
#228795,#228796,#228797,#228798,#228799,#228800,#228801,#228802,#228803,
#228804,#228805,#228806,#228807,#228808,#228809,#228810,#228811,#228812,
#228813,#228814,#228815,#228816,#228817,#228818,#228819,#228820,#228821,
#228822,#228823,#228824,#228825,#228826,#228827,#228828,#228829,#228830,
#228831,#228832,#228833,#228834,#228835,#228836,#228837,#228838,#228839,
#228840,#228841,#228842,#228843,#228844,#228845,#228846,#228847,#228848,
#228849,#228850,#228851,#228852,#228853,#228854,#228855,#228856,#228857,
#228858,#228859,#228860,#228861,#228862,#228863,#228864,#228865,#228866,
#228867,#228868,#228869,#228870,#228871,#228872,#228873,#228874,#228875,
#228876,#228877,#228878,#228879,#228880,#228881,#228882,#228883,#228884,
#228885,#228886,#228887,#228888,#228889,#228890,#228891,#228892,#228893,
#228894,#228895,#228896,#228897,#228898,#228899,#228900,#228901,#228902,
#228903,#228904,#228905,#228906,#228907,#228908,#228909,#228910,#228911,
#228912,#228913,#228914,#228915,#228916,#228917,#228918,#228919,#228920,
#228921,#228922,#228923,#228924,#228925,#228926,#228927,#228928,#228929,
#228930,#228931,#228932,#228933,#228934,#228935,#228936,#228937,#228938,
#228939,#228940,#228941,#228942,#228943,#228944,#228945,#228946,#228947,
#228948,#228949,#228950,#228951,#228952,#228953,#228954,#228955,#228956,
#228957,#228958,#228959,#228960,#228961,#228962,#228963,#228964,#228965,
#228966,#228967,#228968,#228969,#228970,#228971,#228972,#228973,#228974,
#228975,#228976,#228977,#228978,#228979,#228980,#228981,#228982,#228983,
#228984,#228985,#228986,#228987,#228988,#228989,#228990,#228991,#228992,
#228993,#228994,#228995,#228996,#228997,#228998,#228999,#229000,#229001,
#229002,#229003,#229004,#229005,#229006,#229007,#229008,#229009,#229010,
#229011,#229012,#229013,#229014,#229015,#229016,#229017,#229018,#229019,
#229020,#229021,#229022,#229023,#229024,#229025,#229026,#229027,#229028,
#229029,#229030,#229031,#229032,#229033,#229034,#229035,#229036,#229037,
#229038,#229039,#229040,#229041,#229042,#229043,#229044,#229045,#229046,
#229047,#229048,#229049,#229050,#229051,#229052,#229053,#229054,#229055,
#229056,#229057,#229058,#229059,#229060,#229061,#229062,#229063,#229064,
#229065,#229066,#229067,#229068,#229069,#229070,#229071),.UNSPECIFIED.,
 .F.,.F.,(4,2,2,2,2,2,2,2,2,2,2,2,2,2,2,2,2,2,2,2,2,2,2,2,2,2,2,2,2,2,2,
2,2,2,2,2,2,2,2,2,2,2,2,2,2,2,2,2,2,2,2,2,2,2,2,2,2,2,2,2,2,2,2,2,2,2,2,
2,2,2,2,2,2,2,2,2,2,2,2,2,2,2,2,2,2,2,2,2,2,2,2,2,2,2,2,2,2,2,2,2,2,2,2,
2,2,2,2,2,2,2,2,2,2,2,2,2,2,2,2,2,2,2,2,2,2,2,2,2,2,2,2,2,2,2,2,2,2,2,2,
2,2,2,2,2,2,2,2,2,2,2,2,2,2,2,2,2,2,2,2,2,2,2,2,2,2,2,2,2,2,2,2,2,2,2,2,
2,2,2,2,2,2,2,2,2,2,2,2,2,2,2,2,2,2,2,2,2,2,2,2,2,2,2,2,2,2,2,2,2,2,2,2,
2,2,2,2,2,2,2,2,2,2,2,2,2,2,2,2,2,2,2,2,2,2,2,2,2,2,2,2,4),(0.00169205085482047,
0.0516099663871825,0.0798090565293214,0.0891707982109067,0.096340521663136,
0.103370345146304,0.110316766529791,0.122039124148549,0.154045623255705,
0.199450145104775,0.353781929219954,0.403283886548112,0.409093062442713,
0.412849415832662,0.415805636931924,0.418561124198566,0.421491016970439,
0.425641897335404,0.438363213028286,0.554983080822192,0.638713628781982,
0.68090256455011,0.699476433871832,0.714050513036348,0.721456710782671,
0.727315814748324,0.734047324736872,0.745313900310716,0.785114221009155,
1.00357245087222,1.04761250334487,1.13942944891135,1.17198906773006,1.1768543131915,
1.17935968392888,1.18138158373093,1.18338972935964,1.18700192890167,1.19801217960724,
1.34975889907847,1.45789445194702,1.56823039798511,1.57681266588377,1.58010115173553,
1.58236505154398,1.58458147064734,1.58725038594849,1.59390271461916,1.65396136578439,
1.76932457583323,1.87446507875747,1.96820307840433,1.99687870674681,1.99999355308001,
2.00150729794154,2.00257739143659,2.00369324071564,2.00523466152933,2.00920649664411,
2.06822484936667,2.16043087939128,2.24455315911634,2.33601800746862,2.38259425680721,
2.38868310746353,2.39352068023074,2.3959951439471,2.3977944652624,2.39971754566394,
2.40301136705745,2.41201730801419,2.54599334559463,2.68860124462997,2.74644694630033,
2.78992843393922,2.796780015887,2.79875986784698,2.79998442182562,2.80110961256146,
2.80254968195062,2.80559215980666,2.82575592392835,2.94230832732665,3.04325453255975,
3.13297422592285,3.1877040790232,3.21579561287667,3.22058845230548,3.22311697265912,
3.22498809850428,3.22701940325989,3.22996143505291,3.2382979667065,3.36691408924803,
3.53002676926141,3.56006497810949,3.60519250149703,3.61396440857074,3.61688695375515,
3.61877959428914,3.62056630268876,3.62292214983633,3.62692545398737,3.65229271754626,
3.86288736341471,3.96882935111336,3.98889605681299,3.99546087660878,3.99961881417096,
4.00348508343925,4.00850549666663,4.01944267341708,4.11556215359659,4.24926291488605,
4.35883983892365,4.36375999285221,4.3659022883867,4.36747353595603,4.36891989842782,
4.37087516544998,4.37565165326645,4.44129639557311,4.53439098440493,4.6159743625376,
4.76440532157646,4.77399485349962,4.77763015256483,4.77978944611996,4.78183404615547,
4.78468444478042,4.79039692381932,4.83528978497999,4.90567479643752,5.02894123160039,
5.18197858425998,5.19177283842955,5.19500209179651,5.19680085854632,5.19861405584541,
5.20086391275691,5.20524199459982,5.23471931015002,5.31145832329827,5.4822875129227,
5.59765658539371,5.6200898725517,5.62920955406716,5.63667764823094,5.64425562432676,
5.65525977505159,5.68478217560014,5.70912829025556,5.79856907016586,5.93369004963465,
5.94669266683466,5.95147818627327,5.95465323394181,5.95765913623308,5.96173914461121,
5.97127653124005,5.98490766243149,6.18360091571373,6.24212040727959,6.25349825754496,
6.26078910284963,6.26659972486131,6.2731652238429,6.28431050105973,6.33098608008638,
6.42812006358124,6.63880564684559,6.65298822910695,6.68475963113383,6.70983956493742,
6.71423093404109,6.71688453325539,6.71893923076202,6.72098015170416,6.72429580549374,
6.72809487812411,6.73506101182642,6.78987042190301,6.88957101610736,6.96524381164446,
7.10296469311381,7.11207099643112,7.11553065717512,7.11758779122784,7.11953704145349,
7.12225667141412,7.12771491975124,7.17091031333986,7.23834425990563,7.33122250358557,
7.42268257061352,7.52922124307661,7.53627501946933,7.53843568540303,7.53960298146341,
7.54075560770922,7.54215143854955,7.54471007200515,7.55924933355297,7.58824594726097,
7.64636410566151,7.70209763132859,7.81776208415526,7.93142598930088,7.93850332430317,
7.94115271053839,7.9430305681646,7.9447991813057,7.94724964662972,7.95210507907004,
7.98766888158887,8.07638244655228,8.14951401847776,8.21967654325857,8.33350159578396,
8.3406609092546,8.34285561667671,8.34404942846161,8.34523388079835,8.34667583364257,
8.34821027262679,8.35479519898447,8.41406181631397,8.4537309150801,8.48980483970088,
8.65051319258309,8.66039397517519,8.7497739496824,8.75708535369838,8.75996830340157,
8.76206218250745,8.76430035290099,8.76728933837661,8.77389280438359,8.91007170909831,
9.06691452272662),.UNSPECIFIED.);
#3575=B_SPLINE_CURVE_WITH_KNOTS('',3,(#229075,#229076,#229077,#229078,#229079,
#229080,#229081,#229082,#229083,#229084,#229085,#229086,#229087,#229088,
#229089,#229090,#229091,#229092,#229093,#229094,#229095,#229096,#229097,
#229098,#229099,#229100,#229101,#229102,#229103,#229104,#229105,#229106,
#229107,#229108,#229109,#229110,#229111,#229112,#229113,#229114,#229115,
#229116,#229117,#229118,#229119,#229120,#229121,#229122,#229123,#229124,
#229125,#229126,#229127,#229128,#229129,#229130,#229131,#229132,#229133,
#229134,#229135,#229136,#229137,#229138,#229139,#229140,#229141,#229142,
#229143,#229144,#229145,#229146,#229147,#229148,#229149,#229150,#229151,
#229152,#229153,#229154,#229155,#229156,#229157,#229158,#229159,#229160,
#229161,#229162,#229163,#229164,#229165,#229166,#229167,#229168,#229169,
#229170,#229171,#229172,#229173,#229174,#229175,#229176,#229177,#229178,
#229179,#229180,#229181,#229182,#229183,#229184,#229185,#229186,#229187,
#229188,#229189,#229190,#229191,#229192,#229193,#229194,#229195,#229196,
#229197,#229198,#229199,#229200,#229201,#229202,#229203,#229204,#229205,
#229206,#229207,#229208,#229209,#229210,#229211,#229212,#229213,#229214,
#229215,#229216,#229217,#229218,#229219,#229220,#229221,#229222,#229223,
#229224,#229225,#229226,#229227,#229228,#229229,#229230,#229231,#229232,
#229233,#229234,#229235,#229236,#229237,#229238,#229239,#229240,#229241,
#229242,#229243,#229244,#229245,#229246),.UNSPECIFIED.,.F.,.F.,(4,3,3,3,
3,3,3,3,3,3,3,3,3,3,3,3,3,3,3,3,3,3,3,3,3,3,3,3,3,3,3,3,3,3,3,3,3,3,3,3,
3,3,3,3,3,3,3,3,3,3,3,3,3,3,3,3,3,4),(-410.482031439357,-410.40051557623,
-410.318975660214,-410.234897138017,-410.153354592523,-410.068008081974,
-409.982661571426,-409.908581990859,-409.834525645462,-409.760479759459,
-409.686410655311,-409.612330240246,-409.538194979741,-409.483291703495,
-409.39912997051,-409.314950786704,-409.230830079807,-409.14678551264,-409.062932700955,
-408.983921835564,-408.908993513659,-408.834071857824,-408.759144941605,
-408.684173917891,-408.609179509688,-408.534115640984,-408.484551967633,
-408.409077454774,-408.333661595445,-408.258291743711,-408.182955284671,
-408.107639626691,-408.029911202326,-407.954580371603,-407.879231192739,
-407.803852246168,-407.728432097994,-407.652921369643,-407.57735703147,
-407.501693797513,-407.485812231771,-407.412829970114,-407.339936403889,
-407.26711651233,-407.194355349297,-407.121638026441,-407.048949698084,
-406.976261565061,-406.90356994441,-406.830861420205,-406.758122564272,
-406.685296111268,-406.612422218906,-406.539435187989,-406.487072495908,
-406.38181871027,-406.280243949839,-406.216790079623),.UNSPECIFIED.);
#3576=B_SPLINE_CURVE_WITH_KNOTS('',3,(#229248,#229249,#229250,#229251,#229252,
#229253,#229254,#229255,#229256,#229257,#229258,#229259,#229260,#229261,
#229262,#229263,#229264,#229265),.UNSPECIFIED.,.F.,.F.,(4,2,2,2,2,2,2,2,
4),(-406.216790079623,-405.381873167729,-404.546956255834,-403.712039343939,
-402.877122432044,-402.042205520149,-401.207288608255,-400.37237169636,
-399.933604772444),.UNSPECIFIED.);
#3577=B_SPLINE_CURVE_WITH_KNOTS('',3,(#229267,#229268,#229269,#229270,#229271,
#229272,#229273,#229274,#229275,#229276,#229277,#229278,#229279,#229280,
#229281,#229282,#229283,#229284,#229285,#229286,#229287,#229288,#229289,
#229290,#229291,#229292,#229293,#229294,#229295,#229296,#229297,#229298,
#229299,#229300,#229301,#229302,#229303,#229304,#229305,#229306,#229307,
#229308,#229309,#229310,#229311,#229312,#229313,#229314,#229315,#229316,
#229317,#229318,#229319,#229320,#229321,#229322,#229323,#229324,#229325,
#229326,#229327,#229328,#229329,#229330,#229331,#229332,#229333,#229334,
#229335,#229336,#229337,#229338,#229339,#229340,#229341,#229342,#229343,
#229344,#229345,#229346,#229347,#229348,#229349,#229350,#229351,#229352,
#229353,#229354,#229355,#229356,#229357,#229358,#229359,#229360,#229361,
#229362,#229363,#229364,#229365,#229366,#229367,#229368,#229369,#229370,
#229371,#229372,#229373,#229374,#229375,#229376,#229377,#229378,#229379,
#229380,#229381,#229382,#229383,#229384,#229385,#229386,#229387,#229388,
#229389,#229390,#229391,#229392,#229393,#229394,#229395,#229396,#229397,
#229398,#229399,#229400,#229401,#229402,#229403,#229404,#229405,#229406,
#229407,#229408,#229409,#229410,#229411,#229412,#229413,#229414,#229415,
#229416,#229417,#229418,#229419,#229420,#229421,#229422,#229423,#229424,
#229425,#229426,#229427,#229428,#229429,#229430,#229431,#229432,#229433,
#229434,#229435,#229436,#229437,#229438,#229439,#229440,#229441,#229442,
#229443,#229444,#229445,#229446,#229447,#229448,#229449,#229450,#229451,
#229452,#229453,#229454,#229455,#229456,#229457,#229458,#229459,#229460,
#229461,#229462,#229463,#229464,#229465,#229466,#229467,#229468,#229469,
#229470,#229471,#229472,#229473,#229474,#229475,#229476,#229477,#229478,
#229479,#229480,#229481,#229482,#229483,#229484,#229485,#229486,#229487,
#229488,#229489,#229490,#229491,#229492,#229493,#229494,#229495,#229496,
#229497,#229498,#229499,#229500,#229501,#229502,#229503,#229504,#229505,
#229506,#229507,#229508,#229509,#229510,#229511,#229512,#229513,#229514,
#229515,#229516,#229517,#229518,#229519,#229520,#229521,#229522,#229523,
#229524,#229525,#229526,#229527,#229528,#229529,#229530,#229531,#229532,
#229533,#229534,#229535,#229536,#229537,#229538,#229539,#229540,#229541,
#229542,#229543,#229544,#229545,#229546,#229547,#229548,#229549,#229550,
#229551,#229552,#229553,#229554,#229555,#229556,#229557,#229558,#229559,
#229560,#229561,#229562,#229563,#229564,#229565,#229566,#229567,#229568,
#229569,#229570,#229571,#229572,#229573,#229574,#229575,#229576,#229577,
#229578,#229579,#229580,#229581,#229582,#229583,#229584,#229585,#229586,
#229587,#229588,#229589,#229590,#229591,#229592,#229593,#229594,#229595,
#229596,#229597,#229598,#229599,#229600,#229601,#229602,#229603,#229604,
#229605,#229606,#229607,#229608,#229609,#229610,#229611,#229612,#229613,
#229614,#229615,#229616,#229617,#229618,#229619,#229620,#229621,#229622,
#229623,#229624,#229625,#229626,#229627,#229628,#229629,#229630,#229631,
#229632,#229633,#229634,#229635,#229636,#229637,#229638,#229639,#229640,
#229641,#229642,#229643,#229644,#229645,#229646,#229647,#229648,#229649,
#229650,#229651,#229652,#229653,#229654,#229655,#229656,#229657,#229658,
#229659,#229660,#229661,#229662,#229663,#229664,#229665,#229666,#229667,
#229668,#229669,#229670,#229671,#229672,#229673,#229674,#229675,#229676,
#229677,#229678,#229679,#229680,#229681,#229682,#229683,#229684,#229685,
#229686,#229687,#229688,#229689,#229690,#229691,#229692,#229693,#229694,
#229695,#229696,#229697,#229698,#229699,#229700,#229701,#229702,#229703,
#229704,#229705,#229706,#229707,#229708,#229709,#229710,#229711,#229712,
#229713,#229714,#229715,#229716,#229717,#229718,#229719,#229720,#229721,
#229722,#229723,#229724,#229725,#229726,#229727,#229728,#229729,#229730,
#229731,#229732,#229733,#229734,#229735,#229736,#229737,#229738,#229739,
#229740,#229741,#229742,#229743,#229744,#229745,#229746,#229747,#229748,
#229749,#229750,#229751,#229752,#229753,#229754,#229755,#229756,#229757,
#229758,#229759,#229760,#229761,#229762,#229763,#229764,#229765,#229766,
#229767,#229768,#229769,#229770,#229771,#229772,#229773,#229774,#229775,
#229776,#229777,#229778,#229779,#229780,#229781,#229782,#229783,#229784,
#229785,#229786,#229787,#229788,#229789,#229790),.UNSPECIFIED.,.F.,.F.,
(4,2,2,2,2,2,2,2,2,2,2,2,2,2,2,2,2,2,2,2,2,2,2,2,2,2,2,2,2,2,2,2,2,2,2,
2,2,2,2,2,2,2,2,2,2,2,2,2,2,2,2,2,2,2,2,2,2,2,2,2,2,2,2,2,2,2,2,2,2,2,2,
2,2,2,2,2,2,2,2,2,2,2,2,2,2,2,2,2,2,2,2,2,2,2,2,2,2,2,2,2,2,2,2,2,2,2,2,
2,2,2,2,2,2,2,2,2,2,2,2,2,2,2,2,2,2,2,2,2,2,2,2,2,2,2,2,2,2,2,2,2,2,2,2,
2,2,2,2,2,2,2,2,2,2,2,2,2,2,2,2,2,2,2,2,2,2,2,2,2,2,2,2,2,2,2,2,2,2,2,2,
2,2,2,2,2,2,2,2,2,2,2,2,2,2,2,2,2,2,2,2,2,2,2,2,2,2,2,2,2,2,2,2,2,2,2,2,
2,2,2,2,2,2,2,2,2,2,2,2,2,2,2,2,2,2,2,2,2,2,2,2,2,2,2,2,2,2,2,2,2,2,2,2,
2,2,2,2,2,2,2,2,2,2,4),(0.0019992779279493,0.297228947054352,0.343206093336844,
0.3503282603909,0.352397935254475,0.353685501401623,0.3548647364931,0.356368710625501,
0.359526680001281,0.379983031318882,0.437800654898626,0.662665731018093,
0.715324353514643,0.748059636914255,0.760178068514997,0.768681673569802,
0.771949177383266,0.773969505821607,0.776163649489694,0.779054042805263,
0.785493405937425,0.839378339458817,0.921165257031632,0.973737674056047,
1.07403941840921,1.16448437909037,1.17121208842534,1.17406815400539,1.17613626449919,
1.17802306984809,1.18054909299143,1.18698989681943,1.29134835881228,1.32664915232754,
1.5997870143185,1.61836009401939,1.62653740906363,1.63261932489516,1.63891506645648,
1.64845069124845,1.67491640221799,1.85513197443603,1.90521009723151,1.92961637905726,
1.93513577982862,1.93848848843592,1.94153997204339,1.945475034328,1.95366711626696,
2.04401426136949,2.15307738077737,2.20282768142618,2.22468886393581,2.24207184232718,
2.25098865782536,2.25815829891227,2.26647546151626,2.28041334313099,2.33806240139658,
2.46055436802008,2.56649374416049,2.65783257485772,2.68983765934622,2.69431446185873,
2.69659007143058,2.69823903237573,2.69999636981616,2.7029953116031,2.71112778664773,
2.82658707030246,2.97984819749147,3.10018735797163,3.10637899983089,3.111348953454,
3.11402616316939,3.11626779025475,3.11886248164798,3.12327724801515,3.13937901070979,
3.39409515319172,3.45553455445926,3.51476141191506,3.52403085918468,3.52677149118404,
3.5284655787969,3.53001012201323,3.53200346106441,3.53614635902375,3.56357680677665,
3.57435733283979,3.58122904603894,3.58535026835805,3.58798373417945,3.74373595078643,
3.87546299879015,3.8873506421484,3.89259351518159,3.89647413767126,3.90007758010477,
3.90500423106867,3.91723138207572,4.08177131512006,4.20291119356008,4.24874216888675,
4.2701361636558,4.27407269269763,4.27618726296623,4.27792247886036,4.27996337786905,
4.28346682811556,4.29654384927286,4.53606304052704,4.59397590020799,4.64991898865479,
4.66525389452868,4.66922646203589,4.67157209062458,4.67364178030088,4.67622061745384,
4.68019127104281,4.69805679702972,4.98308190961803,5.08671613173766,5.09343687248634,
5.09551069425155,5.09663440683052,5.09774609515131,5.09909598980325,5.10167893502373,
5.11777829779163,5.1530080125434,5.21162561518377,5.40110282176406,5.48881648253929,
5.49555928488173,5.49817965419276,5.50006956882661,5.50207734004741,5.50473747379003,
5.51052916903007,5.60198522323136,5.70535856844502,5.75068322388203,5.80504227161934,
5.88711162687489,5.89211316909507,5.89380229969992,5.89495716783776,5.89601199595674,
5.89742402012768,5.90005588350536,5.91433289653597,5.94332463672421,5.99885041524903,
6.15764280351359,6.29966959544904,6.30942061895616,6.31299566695155,6.31508546967096,
6.31704247654236,6.31973651220617,6.32501318429958,6.36139058804319,6.45783807932016,
6.64126789772151,6.70721010371304,6.71317789432634,6.71586853547409,6.71791682725447,
6.72009390011982,6.72340330868569,6.73300407796326,6.78888707700809,6.91051973628635,
7.13545141826491,7.1577854348511,7.16593365678988,7.17169801146943,7.17774215403553,
7.18549655191127,7.20155886401366,7.22269298063199,7.27339432600211,7.37440708273428,
7.46791276261557,7.47534205621098,7.47905704995501,7.48208809077319,7.48536793971601,
7.49106782448146,7.49801744753919,7.5121595850515,7.55102878833044,7.68100662035085,
7.72011479218897,7.77224585818453,7.78621867100486,7.79441832452067,7.80160446698084,
7.810518651449,7.82767807427143,7.85054727836261,7.90668179587075,8.18684462456534,
8.19349108776987,8.20179636992428,8.23183535612473,8.23655325343509,8.23891140316971,
8.24074322508187,8.24275733182213,8.24481927279615,8.25129390476362,8.2602350460732,
8.28287732060411,8.31752193756336,8.41819280867382,8.4970593059251,8.64193316334752,
8.65158179498022,8.65522208733346,8.65737937709897,8.65941880359651,8.66225676051235,
8.66792519488908,8.71157596324893,8.82699719722926,8.9192282925171,8.96002475289104,
9.02690261667247,9.06363893165391,9.06749441673257,9.06946196239184,9.07090904721298,
9.07247303579576,9.07459116081652,9.07693165309151,9.09203175909149,9.12148023812957,
9.19951570275614,9.27169365400701,9.41823718439555,9.42978126939524,9.43444335739657,
9.4383364264765,9.44233870547363,9.44637124726198,9.45199548384072,9.48261243362604,
9.57513842185726,9.60500204001224,9.63839687086317,9.78932144734067,9.81185821182605,
9.81571034804602,9.81801999060946,9.81979676672897,9.82170336747785,9.8236421588566,
9.82643033046538,9.83123731522428,9.96237951771243),.UNSPECIFIED.);
#3578=B_SPLINE_CURVE_WITH_KNOTS('',3,(#229792,#229793,#229794,#229795,#229796,
#229797,#229798,#229799,#229800,#229801,#229802,#229803,#229804,#229805,
#229806,#229807,#229808,#229809,#229810,#229811,#229812,#229813,#229814,
#229815,#229816,#229817,#229818,#229819,#229820,#229821,#229822,#229823,
#229824,#229825,#229826,#229827,#229828,#229829,#229830,#229831,#229832,
#229833,#229834,#229835,#229836,#229837,#229838,#229839,#229840,#229841,
#229842,#229843,#229844,#229845,#229846,#229847,#229848,#229849,#229850,
#229851,#229852,#229853,#229854,#229855,#229856,#229857,#229858,#229859,
#229860,#229861,#229862,#229863,#229864,#229865,#229866,#229867,#229868,
#229869,#229870,#229871,#229872,#229873,#229874,#229875,#229876,#229877,
#229878,#229879,#229880,#229881,#229882,#229883,#229884,#229885,#229886,
#229887,#229888,#229889,#229890,#229891,#229892,#229893,#229894,#229895,
#229896,#229897,#229898,#229899,#229900,#229901,#229902,#229903,#229904,
#229905,#229906,#229907,#229908,#229909,#229910,#229911,#229912,#229913,
#229914,#229915,#229916,#229917,#229918,#229919,#229920,#229921,#229922,
#229923,#229924,#229925,#229926,#229927,#229928,#229929,#229930,#229931,
#229932,#229933,#229934,#229935,#229936,#229937,#229938,#229939,#229940,
#229941,#229942,#229943,#229944,#229945,#229946,#229947,#229948,#229949,
#229950,#229951,#229952,#229953,#229954,#229955,#229956,#229957,#229958,
#229959,#229960,#229961,#229962,#229963,#229964,#229965,#229966,#229967,
#229968,#229969,#229970,#229971,#229972,#229973,#229974,#229975,#229976,
#229977,#229978,#229979,#229980,#229981,#229982,#229983,#229984,#229985,
#229986,#229987,#229988,#229989,#229990,#229991,#229992,#229993,#229994,
#229995,#229996,#229997,#229998,#229999,#230000,#230001,#230002,#230003,
#230004,#230005,#230006,#230007,#230008,#230009,#230010,#230011,#230012,
#230013,#230014,#230015,#230016,#230017,#230018,#230019,#230020,#230021,
#230022,#230023,#230024,#230025,#230026,#230027,#230028,#230029,#230030,
#230031,#230032,#230033,#230034,#230035,#230036,#230037,#230038,#230039,
#230040,#230041,#230042,#230043,#230044,#230045,#230046,#230047,#230048,
#230049,#230050),.UNSPECIFIED.,.F.,.F.,(4,3,3,3,3,3,3,3,3,3,3,3,3,3,3,3,
3,3,3,3,3,3,3,3,3,3,3,3,3,3,3,3,3,3,3,3,3,3,3,3,3,3,3,3,3,3,3,3,3,3,3,3,
3,3,3,3,3,3,3,3,3,3,3,3,3,3,3,3,3,3,3,3,3,3,3,3,3,3,3,3,3,3,3,3,3,3,4),
(-387.367234158085,-387.293462939457,-387.219749263725,-387.146078733845,
-387.07243698482,-386.998797021076,-386.92515438306,-386.851496085639,-386.777809136646,
-386.704040445516,-386.630226409719,-386.556308537467,-386.512277778665,
-386.439138834976,-386.366087917664,-386.293110093637,-386.220190499117,
-386.147314324136,-386.07446679855,-386.001619301385,-385.928768152842,
-385.855900003737,-385.783001493679,-385.710016052112,-385.636983239331,
-385.563838815208,-385.513538042803,-385.438009754137,-385.362567558804,
-385.28719855111,-385.211889873148,-385.136628706748,-385.058899906772,
-384.983689709447,-384.908485484749,-384.833275674485,-384.758048719499,
-384.68276582989,-384.60744978302,-384.532062873763,-384.51479830694,-384.438206406543,
-384.361679704606,-384.285208508718,-384.208791648461,-384.13240760963,
-384.056047446221,-384.015428439009,-383.937309170526,-383.859144867048,
-383.780930790054,-383.702625667362,-383.624272240758,-383.545833150988,
-383.516058571078,-383.434079792495,-383.352173043258,-383.268301958231,
-383.18663654572,-383.101662624433,-383.016688703147,-382.94307702904,-382.869470662186,
-382.795856610283,-382.722190317753,-382.648496789728,-382.574721316661,
-382.517318835216,-382.44081811041,-382.364373343229,-382.287973623649,
-382.211608074043,-382.135265841853,-382.05817999904,-381.981838185664,
-381.905486098022,-381.829113873915,-381.751480180275,-381.675008503282,
-381.596793801318,-381.518579099354,-381.442494174995,-381.366503409665,
-381.290623633396,-381.214808144098,-381.139062747223,-381.084048850905),
 .UNSPECIFIED.);
#3579=B_SPLINE_CURVE_WITH_KNOTS('',3,(#230052,#230053,#230054,#230055,#230056,
#230057,#230058,#230059,#230060,#230061,#230062,#230063,#230064,#230065,
#230066,#230067,#230068,#230069,#230070,#230071,#230072,#230073,#230074,
#230075,#230076,#230077,#230078,#230079,#230080,#230081,#230082,#230083,
#230084,#230085,#230086,#230087,#230088,#230089,#230090,#230091,#230092,
#230093,#230094,#230095,#230096,#230097,#230098,#230099,#230100,#230101,
#230102,#230103,#230104,#230105,#230106,#230107,#230108,#230109,#230110,
#230111,#230112,#230113,#230114,#230115,#230116,#230117,#230118,#230119,
#230120,#230121,#230122,#230123,#230124,#230125,#230126,#230127,#230128,
#230129,#230130,#230131,#230132,#230133,#230134,#230135,#230136,#230137,
#230138,#230139,#230140,#230141,#230142,#230143,#230144,#230145,#230146,
#230147,#230148,#230149,#230150,#230151,#230152,#230153,#230154,#230155,
#230156,#230157,#230158,#230159,#230160,#230161,#230162,#230163,#230164,
#230165,#230166,#230167,#230168,#230169,#230170,#230171,#230172,#230173,
#230174,#230175,#230176,#230177,#230178,#230179,#230180,#230181,#230182,
#230183,#230184,#230185,#230186,#230187,#230188,#230189,#230190,#230191,
#230192,#230193,#230194,#230195,#230196,#230197,#230198,#230199,#230200,
#230201,#230202,#230203,#230204,#230205,#230206,#230207,#230208,#230209,
#230210,#230211,#230212,#230213,#230214,#230215,#230216,#230217,#230218,
#230219,#230220,#230221,#230222,#230223,#230224,#230225,#230226,#230227,
#230228,#230229,#230230,#230231,#230232,#230233,#230234,#230235,#230236,
#230237,#230238,#230239,#230240,#230241,#230242,#230243,#230244,#230245,
#230246,#230247,#230248,#230249,#230250,#230251,#230252,#230253,#230254,
#230255,#230256,#230257,#230258,#230259,#230260,#230261,#230262,#230263,
#230264,#230265,#230266,#230267,#230268,#230269,#230270,#230271,#230272,
#230273,#230274,#230275,#230276,#230277,#230278,#230279,#230280,#230281,
#230282,#230283,#230284,#230285,#230286,#230287,#230288,#230289,#230290,
#230291,#230292,#230293,#230294,#230295,#230296,#230297,#230298,#230299,
#230300,#230301,#230302,#230303,#230304,#230305,#230306,#230307,#230308,
#230309,#230310,#230311,#230312,#230313,#230314,#230315,#230316,#230317,
#230318,#230319,#230320,#230321,#230322,#230323,#230324,#230325,#230326,
#230327,#230328,#230329,#230330,#230331,#230332,#230333,#230334,#230335,
#230336,#230337,#230338,#230339,#230340,#230341,#230342,#230343,#230344,
#230345,#230346,#230347,#230348,#230349,#230350,#230351,#230352,#230353,
#230354,#230355,#230356,#230357,#230358,#230359,#230360,#230361,#230362,
#230363,#230364,#230365,#230366,#230367,#230368,#230369,#230370,#230371,
#230372,#230373,#230374,#230375,#230376,#230377,#230378,#230379,#230380,
#230381,#230382,#230383,#230384,#230385,#230386,#230387,#230388,#230389,
#230390,#230391,#230392,#230393,#230394,#230395,#230396,#230397,#230398,
#230399,#230400,#230401,#230402,#230403,#230404,#230405,#230406,#230407,
#230408,#230409,#230410,#230411,#230412,#230413,#230414,#230415,#230416,
#230417,#230418,#230419,#230420,#230421,#230422,#230423,#230424,#230425,
#230426,#230427,#230428,#230429,#230430,#230431,#230432,#230433,#230434,
#230435,#230436,#230437,#230438,#230439,#230440,#230441,#230442,#230443,
#230444,#230445,#230446,#230447,#230448,#230449,#230450,#230451,#230452,
#230453,#230454,#230455,#230456,#230457,#230458,#230459,#230460,#230461,
#230462,#230463,#230464,#230465,#230466,#230467,#230468,#230469,#230470,
#230471,#230472,#230473,#230474,#230475,#230476,#230477,#230478,#230479,
#230480,#230481,#230482,#230483,#230484,#230485,#230486,#230487,#230488,
#230489,#230490,#230491,#230492,#230493,#230494,#230495,#230496,#230497,
#230498,#230499,#230500,#230501,#230502,#230503,#230504,#230505,#230506,
#230507,#230508,#230509,#230510,#230511,#230512,#230513,#230514,#230515,
#230516,#230517,#230518,#230519,#230520,#230521,#230522,#230523,#230524,
#230525,#230526,#230527,#230528,#230529,#230530,#230531,#230532,#230533,
#230534,#230535,#230536,#230537,#230538,#230539,#230540,#230541,#230542,
#230543,#230544,#230545,#230546,#230547,#230548,#230549,#230550,#230551,
#230552,#230553,#230554,#230555,#230556,#230557,#230558,#230559,#230560,
#230561,#230562,#230563,#230564,#230565,#230566,#230567,#230568,#230569,
#230570,#230571,#230572,#230573,#230574,#230575,#230576,#230577,#230578,
#230579,#230580,#230581,#230582,#230583,#230584,#230585,#230586,#230587),
 .UNSPECIFIED.,.F.,.F.,(4,2,2,2,2,2,2,2,2,2,2,2,2,2,2,2,2,2,2,2,2,2,2,2,
2,2,2,2,2,2,2,2,2,2,2,2,2,2,2,2,2,2,2,2,2,2,2,2,2,2,2,2,2,2,2,2,2,2,2,2,
2,2,2,2,2,2,2,2,2,2,2,2,2,2,2,2,2,2,2,2,2,2,2,2,2,2,2,2,2,2,2,2,2,2,2,2,
2,2,2,2,2,2,2,2,2,2,2,2,2,2,2,2,2,2,2,2,2,2,2,2,2,2,2,2,2,2,2,2,2,2,2,2,
2,2,2,2,2,2,2,2,2,2,2,2,2,2,2,2,2,2,2,2,2,2,2,2,2,2,2,2,2,2,2,2,2,2,2,2,
2,2,2,2,2,2,2,2,2,2,2,2,2,2,2,2,2,2,2,2,2,2,2,2,2,2,2,2,2,2,2,2,2,2,2,2,
2,2,2,2,2,2,2,2,2,2,2,2,2,2,2,2,2,2,2,2,2,2,2,2,2,2,2,2,2,2,2,2,2,2,2,2,
2,2,2,2,2,2,2,2,2,2,2,2,2,2,2,2,2,2,2,2,2,2,2,2,2,2,2,4),(0.00136196530955085,
0.0236124556839763,0.0292659071113713,0.0333084640585915,0.03686252960954,
0.0406110068832381,0.0455738782555038,0.0562154239113908,0.0811176318447605,
0.331754615019365,0.386990162446628,0.411821203394026,0.415919343847642,
0.418067990451346,0.419820968232722,0.421839306700059,0.425247464787378,
0.437413270522316,0.618850537864965,0.675078510992058,0.751521043042145,
0.78695949380261,0.799638694305315,0.805533128507329,0.810278664031603,
0.812793239586447,0.814658691310162,0.816688399968935,0.820258021300029,
0.830598030662721,0.987769148384333,1.06460698171212,1.07436405361475,1.0856285243643,
1.11869579464937,1.17776687034043,1.22687328611878,1.23431620079812,1.23637958406761,
1.23762535416216,1.23874181795397,1.24015764158288,1.24241835223426,1.25409173095658,
1.45080428958484,1.51263164120352,1.58290728550593,1.61573032191407,1.62761190169168,
1.6331722370948,1.63762775506656,1.64003739605459,1.64182525262976,1.64377075150026,
1.64659637438564,1.65465439129887,1.78022263044505,1.9257462280367,1.94732001714936,
1.97689088139107,2.02499312575702,2.03231168265478,2.03440072306649,2.03569249340056,
2.03687034472446,2.03839035470773,2.0415478409083,2.06200134288342,2.21603159948904,
2.30008997083458,2.39102491668349,2.44033203172534,2.4468575824038,2.45205849979095,
2.45473623495933,2.45669059933914,2.4587862938115,2.46177763666948,2.46997709768255,
2.59804147266279,2.75498467654587,2.84632380395221,2.85306703717984,2.85592580350572,
2.8579944293996,2.85988071536277,2.86240457163804,2.86883176248918,2.95647887874079,
3.1553576752948,3.28668265609071,3.30169217464577,3.30920307279823,3.31462902464923,
3.32041336830083,3.33033597675164,3.35816721206757,3.39130941156882,3.53793166220926,
3.58693863800192,3.61100399089153,3.61650029836134,3.6198481238142,3.6229005346247,
3.62684437802611,3.63508246966176,3.71605282590116,3.78962674125273,3.89624006654166,
3.92007374651435,3.93017952969019,3.93756885727421,3.94439560498426,3.95372200436719,
3.97749884868377,4.18380905148408,4.30799040526486,4.36108159670524,4.3691519382429,
4.37504851788863,4.37759514899182,4.37945554635735,4.38116298809323,4.3834637948443,
4.38905029117079,4.4517122648304,4.64304984568877,4.71832975067706,4.77897813507876,
4.79021393804593,4.79394938264702,4.79636615937359,4.79864591963759,4.80164893488286,
4.80833883161805,4.86430167055103,4.97949568178559,5.19214041517499,5.20435864780263,
5.20748027517295,5.20927806586203,5.21065567300716,5.21243312294419,5.21554859833586,
5.22899736664495,5.35655949478621,5.46976260595272,5.55814447031661,5.56887165372405,
5.57384468777813,5.5776952059052,5.58185676427516,5.58847117190765,5.60900897955343,
5.71921882760491,5.90552851287311,5.92623721278161,5.95031689459131,5.95425040163329,
5.95658337968545,5.95836328899277,5.96025888333169,5.9632067183965,5.97220916524013,
6.13376393631706,6.33303116735921,6.34464228060622,6.34892983509415,6.35160610321291,
6.35368616361993,6.35597395612439,6.35968904765886,6.37238250886363,6.44881917279999,
6.53791359041877,6.72231983745179,6.77067658576297,6.77446759438621,6.7759399776664,
6.77700140471194,6.77801586706867,6.77941752830882,6.7823000244874,6.78604953950823,
6.81777620383178,6.89074502905239,7.15632948240258,7.17326913458454,7.17705951533461,
7.17952606945882,7.18150887834564,7.18375950397884,7.18757950328156,7.20242187076909,
7.25761702845799,7.31891429461854,7.51271221383867,7.56891525525163,7.57283425230113,
7.57436483136627,7.57547609651029,7.57666340132407,7.57821557579685,7.58156544577563,
7.58601102578738,7.62630965207514,7.68553923131124,7.6935001771149,7.9705581906164,
7.98820711490774,7.99226898591487,7.99493523144023,7.99709399981822,7.9995612759102,
8.00379099466473,8.02075594260699,8.19597357337795,8.26716439171727,8.38433310728232,
8.39243022026517,8.3952888759041,8.39726362528687,8.39924527104867,8.40173176557202,
8.40444550792262,8.40882277174437,8.41745632636344,8.5128419558117,8.68019757327686,
8.75336330516805,8.82955546336615,8.8414311107382,8.8489807385905,8.85497715618765,
8.86173355113897,8.87315396079692,8.91922952813686,9.00581296499531,9.08169880468175,
9.14752245751981,9.15478410073917,9.15845309383498,9.16134085574025,9.16473392303519,
9.17036390343075,9.19111094249666,9.22868379246932,9.34812426892164,9.42006510906791,
9.45516567168477,9.46727904885301,9.47428817319761,9.48084393399812,9.48990988194288,
9.50812860241058,9.61741479843833,9.68401792423951,9.87143384275936,9.88295728658906,
9.9104880277396,9.91467959153884,9.91713096380455,9.91894512436701,9.92064211511499,
9.92253831544743,9.92515013362575,9.92946269899985,9.95805478872874),
 .UNSPECIFIED.);
#3580=B_SPLINE_CURVE_WITH_KNOTS('',3,(#230589,#230590,#230591,#230592,#230593,
#230594,#230595,#230596,#230597,#230598,#230599,#230600,#230601,#230602,
#230603,#230604,#230605,#230606,#230607,#230608,#230609,#230610,#230611,
#230612,#230613,#230614,#230615,#230616,#230617,#230618,#230619,#230620,
#230621,#230622,#230623,#230624,#230625,#230626,#230627,#230628,#230629,
#230630,#230631,#230632,#230633,#230634,#230635,#230636,#230637,#230638,
#230639,#230640,#230641,#230642,#230643,#230644,#230645,#230646,#230647,
#230648,#230649,#230650,#230651,#230652,#230653,#230654,#230655,#230656,
#230657,#230658,#230659,#230660,#230661,#230662,#230663,#230664,#230665,
#230666,#230667,#230668,#230669,#230670,#230671,#230672,#230673,#230674,
#230675,#230676,#230677,#230678,#230679,#230680,#230681,#230682,#230683,
#230684,#230685,#230686,#230687,#230688,#230689,#230690,#230691,#230692,
#230693,#230694,#230695,#230696,#230697,#230698,#230699,#230700,#230701,
#230702,#230703,#230704,#230705,#230706,#230707,#230708,#230709,#230710,
#230711,#230712,#230713,#230714,#230715,#230716,#230717,#230718,#230719,
#230720,#230721,#230722,#230723,#230724,#230725,#230726,#230727,#230728,
#230729,#230730,#230731,#230732,#230733,#230734,#230735,#230736,#230737,
#230738,#230739,#230740,#230741,#230742,#230743,#230744,#230745,#230746,
#230747,#230748,#230749,#230750,#230751,#230752,#230753,#230754,#230755,
#230756,#230757,#230758,#230759,#230760,#230761,#230762,#230763,#230764,
#230765,#230766,#230767,#230768,#230769,#230770,#230771,#230772,#230773,
#230774,#230775,#230776,#230777,#230778,#230779,#230780,#230781,#230782,
#230783,#230784,#230785,#230786,#230787,#230788,#230789,#230790,#230791,
#230792,#230793,#230794,#230795,#230796,#230797,#230798,#230799,#230800,
#230801,#230802,#230803,#230804,#230805,#230806,#230807,#230808,#230809,
#230810,#230811,#230812,#230813,#230814,#230815,#230816,#230817,#230818,
#230819,#230820,#230821,#230822,#230823,#230824,#230825,#230826,#230827,
#230828,#230829,#230830,#230831,#230832,#230833,#230834,#230835,#230836,
#230837,#230838,#230839,#230840,#230841,#230842,#230843,#230844,#230845,
#230846,#230847,#230848,#230849,#230850,#230851,#230852,#230853,#230854,
#230855,#230856,#230857,#230858,#230859,#230860,#230861,#230862,#230863,
#230864,#230865,#230866,#230867,#230868,#230869,#230870,#230871,#230872,
#230873,#230874,#230875,#230876,#230877,#230878,#230879,#230880,#230881,
#230882,#230883,#230884,#230885,#230886,#230887,#230888,#230889,#230890,
#230891,#230892,#230893,#230894,#230895,#230896,#230897,#230898,#230899,
#230900,#230901,#230902,#230903,#230904,#230905,#230906,#230907,#230908,
#230909,#230910,#230911,#230912,#230913,#230914,#230915,#230916,#230917,
#230918,#230919,#230920,#230921,#230922,#230923,#230924,#230925,#230926,
#230927,#230928,#230929,#230930,#230931,#230932,#230933,#230934,#230935,
#230936,#230937,#230938,#230939,#230940,#230941,#230942,#230943,#230944,
#230945,#230946,#230947,#230948,#230949,#230950,#230951,#230952,#230953,
#230954,#230955,#230956,#230957,#230958,#230959,#230960,#230961,#230962,
#230963,#230964,#230965,#230966,#230967,#230968,#230969,#230970,#230971,
#230972,#230973,#230974,#230975,#230976,#230977,#230978,#230979,#230980,
#230981,#230982,#230983,#230984,#230985,#230986,#230987,#230988,#230989,
#230990,#230991,#230992,#230993,#230994,#230995,#230996,#230997,#230998,
#230999,#231000,#231001,#231002,#231003,#231004,#231005,#231006,#231007,
#231008,#231009,#231010,#231011,#231012,#231013,#231014,#231015,#231016,
#231017,#231018,#231019,#231020,#231021,#231022,#231023,#231024,#231025,
#231026,#231027,#231028,#231029,#231030,#231031,#231032,#231033,#231034,
#231035,#231036,#231037,#231038,#231039,#231040,#231041,#231042,#231043,
#231044,#231045,#231046,#231047,#231048,#231049,#231050,#231051,#231052,
#231053,#231054,#231055,#231056,#231057,#231058,#231059,#231060,#231061,
#231062,#231063,#231064,#231065,#231066,#231067,#231068,#231069,#231070,
#231071,#231072,#231073,#231074,#231075,#231076,#231077,#231078,#231079,
#231080,#231081,#231082,#231083,#231084,#231085,#231086,#231087,#231088,
#231089,#231090,#231091,#231092,#231093,#231094,#231095,#231096,#231097,
#231098,#231099,#231100,#231101,#231102),.UNSPECIFIED.,.F.,.F.,(4,2,2,2,
2,2,2,2,2,2,2,2,2,2,2,2,2,2,2,2,2,2,2,2,2,2,2,2,2,2,2,2,2,2,2,2,2,2,2,2,
2,2,2,2,2,2,2,2,2,2,2,2,2,2,2,2,2,2,2,2,2,2,2,2,2,2,2,2,2,2,2,2,2,2,2,2,
2,2,2,2,2,2,2,2,2,2,2,2,2,2,2,2,2,2,2,2,2,2,2,2,2,2,2,2,2,2,2,2,2,2,2,2,
2,2,2,2,2,2,2,2,2,2,2,2,2,2,2,2,2,2,2,2,2,2,2,2,2,2,2,2,2,2,2,2,2,2,2,2,
2,2,2,2,2,2,2,2,2,2,2,2,2,2,2,2,2,2,2,2,2,2,2,2,2,2,2,2,2,2,2,2,2,2,2,2,
2,2,2,2,2,2,2,2,2,2,2,2,2,2,2,2,2,2,2,2,2,2,2,2,2,2,2,2,2,2,2,2,2,2,2,2,
2,2,2,2,2,2,2,2,2,2,2,2,2,2,2,2,2,2,2,2,2,2,2,2,2,2,2,2,2,2,2,2,2,2,2,2,
4),(0.00195160114906104,0.236564753226539,0.335098581850809,0.341349135687907,
0.371066482143385,0.376219658527723,0.378948856434874,0.38118944845288,
0.383784799532088,0.388205161030339,0.404371930212253,0.665359609611313,
0.725025870907951,0.76793502568408,0.780676553610812,0.786183381855492,
0.789145668938059,0.79169772059083,0.7933345024209,0.794835394757625,0.796816015756153,
0.801005766199686,0.829563273344597,0.914924903629073,0.992305247446216,
1.1388234777171,1.15155728784486,1.15694717519968,1.16085261487765,1.16442084567994,
1.16921126430518,1.1809625016166,1.28496037894192,1.43771930148249,1.5062910684478,
1.5340595547071,1.5382753206524,1.54041869218177,1.54214016493648,1.54406633044912,
1.54719580108933,1.55719308137523,1.71076731761959,1.85052170758076,1.90154307399534,
1.92799922432744,1.93270483431189,1.93521076862615,1.93707518688884,1.93910906514032,
1.94270004339742,1.95319321398495,2.112470924865,2.20065729336001,2.29319376660234,
2.34863452435371,2.35659015448224,2.35869824394119,2.35976182573397,2.36076484505819,
2.36186170702233,2.36347530342251,2.36830670246239,2.44448922157615,2.64969227313868,
2.72428476963431,2.75516165586155,2.75991293289239,2.76236565755929,2.76432914529949,
2.76658296889377,2.77041742761224,2.78361358117687,2.98102972464616,3.10160093911351,
3.14775552386405,3.15246923897567,3.15488763139188,3.15695493810197,3.15821435612411,
3.15939037526977,3.16089613709275,3.16329452091367,3.1754174055144,3.37808115115149,
3.48507866512861,3.54071201146672,3.56987697388276,3.57486384442311,3.57749639958538,
3.57965319961953,3.58214645921628,3.58638082255285,3.60174548136215,3.86411377213341,
3.9675644317206,3.97563551736588,3.97870941021309,3.98082052597055,3.98288397233688,
3.98536646692756,3.99130331223031,4.04742376052928,4.19180128647086,4.29841063221591,
4.41085266647841,4.42509696251923,4.43245354526277,4.43843585520245,4.44532906634405,
4.45705585489681,4.50225922775368,4.50462396718772,4.71277304165758,4.73446683720325,
4.73979467280805,4.74310861046367,4.74617131004224,4.750121071576,4.75666154437867,
4.79633375072138,4.87116764325385,4.98086066249085,4.98324526279393,5.03510218389985,
5.04904785292532,5.05723937649996,5.06442310789975,5.07352169310156,5.09189884192763,
5.20324495223863,5.29946033092353,5.42534561773102,5.43381873306651,5.43916676054429,
5.44129494743573,5.444923396478,5.44812923292397,5.47727794521809,5.48096659548021,
5.48935523359825,5.49711748252184,5.50005618930305,5.50180265291852,5.50364017563343,
5.50604646685044,5.51117926205437,5.60703152194068,5.65322938854595,5.69923379864474,
5.83181448302771,5.90727697734319,5.91436915351803,5.91724339111729,5.9193589278411,
5.92164698764888,5.92474963189037,5.93180189113912,6.05417757569404,6.22436290625847,
6.2632633601556,6.32460772526371,6.32930883239099,6.33124751205842,6.33268688636149,
6.33425568919932,6.33640391338538,6.34137859048937,6.47708326990131,6.58813140664802,
6.68088685514166,6.6906372129087,6.69555956984243,6.69916115119682,6.70304037759745,
6.70827900432122,6.71407172541381,6.72395561189804,6.88919429061741,7.00315999926392,
7.04594902308813,7.07294386681487,7.07741187410535,7.07966792545691,7.08143108576343,
7.08338035349883,7.08656866245492,7.09768863143446,7.16515550970892,7.31735428283288,
7.46061729240305,7.46986953050109,7.4732790181967,7.47527689536756,7.47715087854513,
7.4797353415103,7.48481404437227,7.52038975389516,7.61146312801923,7.70978884005364,
7.88436282411656,7.89545187018429,7.89770241904568,7.89912525986586,7.90024272633313,
7.9014835297925,7.90354899742277,7.9113007217569,7.96493268655756,8.07410227886942,
8.1633819232011,8.28895534739201,8.29743218797857,8.30063948584882,8.30254251705441,
8.30434305262912,8.30685084125137,8.31158494177505,8.34429418175278,8.43727304185448,
8.50359607105898,8.68276785122259,8.6934972746029,8.69574253331132,8.69720183500901,
8.69837312675038,8.69970053238662,8.70194805627772,8.71060307247117,8.77262799719312,
8.88931169928874,8.93915506481872,9.10108606007421,9.11164154999792,9.11533508509668,
9.117448210463,9.11939837328633,9.12203929281573,9.12706373092504,9.15647196804778,
9.21916756444585,9.24932204092596,9.26897622435194,9.32650303437604,9.38529166836775,
9.50518047064267,9.51401274780402,9.51730809811315,9.51925011566599,9.52107965123076,
9.52361612295599,9.52864855077965,9.56666039541573,9.70423316355673,9.90844336539317,
9.94319584725104,9.95899229756381),.UNSPECIFIED.);
#3581=B_SPLINE_CURVE_WITH_KNOTS('',3,(#231104,#231105,#231106,#231107,#231108,
#231109,#231110,#231111,#231112,#231113,#231114,#231115,#231116,#231117,
#231118,#231119,#231120,#231121,#231122,#231123,#231124,#231125,#231126,
#231127,#231128,#231129,#231130,#231131,#231132,#231133,#231134,#231135,
#231136,#231137,#231138,#231139,#231140,#231141,#231142,#231143,#231144,
#231145,#231146,#231147,#231148,#231149,#231150,#231151,#231152,#231153,
#231154,#231155,#231156,#231157,#231158,#231159,#231160,#231161,#231162,
#231163,#231164,#231165,#231166,#231167,#231168,#231169,#231170,#231171,
#231172,#231173,#231174,#231175,#231176,#231177,#231178,#231179,#231180,
#231181,#231182,#231183,#231184,#231185,#231186,#231187,#231188,#231189,
#231190,#231191,#231192,#231193,#231194,#231195,#231196,#231197,#231198,
#231199,#231200,#231201,#231202,#231203,#231204,#231205,#231206,#231207,
#231208,#231209,#231210,#231211,#231212,#231213,#231214,#231215,#231216,
#231217,#231218,#231219,#231220,#231221,#231222,#231223,#231224,#231225,
#231226,#231227,#231228,#231229,#231230,#231231,#231232,#231233,#231234,
#231235,#231236,#231237,#231238,#231239,#231240,#231241,#231242,#231243,
#231244,#231245,#231246,#231247,#231248,#231249,#231250,#231251,#231252,
#231253,#231254,#231255,#231256,#231257,#231258,#231259,#231260,#231261,
#231262,#231263,#231264,#231265,#231266,#231267,#231268,#231269,#231270,
#231271,#231272,#231273,#231274,#231275,#231276,#231277,#231278,#231279,
#231280,#231281,#231282,#231283,#231284,#231285,#231286,#231287,#231288,
#231289,#231290,#231291,#231292,#231293,#231294,#231295,#231296,#231297,
#231298,#231299,#231300,#231301,#231302,#231303,#231304,#231305,#231306,
#231307,#231308,#231309,#231310,#231311,#231312,#231313,#231314,#231315,
#231316,#231317,#231318,#231319,#231320,#231321,#231322,#231323,#231324,
#231325,#231326,#231327,#231328,#231329,#231330,#231331,#231332,#231333,
#231334,#231335,#231336,#231337,#231338,#231339,#231340,#231341,#231342,
#231343,#231344,#231345,#231346,#231347,#231348,#231349,#231350,#231351,
#231352,#231353,#231354,#231355,#231356,#231357,#231358,#231359),
 .UNSPECIFIED.,.F.,.F.,(4,3,3,3,3,3,3,3,3,3,3,3,3,3,3,3,3,3,3,3,3,3,3,3,
3,3,3,3,3,3,3,3,3,3,3,3,3,3,3,3,3,3,3,3,3,3,3,3,3,3,3,3,3,3,3,3,3,3,3,3,
3,3,3,3,3,3,3,3,3,3,3,3,3,3,3,3,3,3,3,3,3,3,3,3,3,4),(-355.951307622187,
-355.872214267879,-355.791997192643,-355.712722085922,-355.63203402643,
-355.551345966937,-355.469367188351,-355.387460439111,-355.303589354085,
-355.221923941571,-355.136950020288,-355.051976099006,-354.9783644249,-354.904758058047,
-354.831144006145,-354.757477713616,-354.683784185592,-354.610008712527,
-354.552606231075,-354.476105506269,-354.399660739088,-354.323261019508,
-354.246895469902,-354.170553237711,-354.093467394898,-354.017125581522,
-353.940773493879,-353.864401269772,-353.786767576132,-353.710295899139,
-353.632081197176,-353.553866495213,-353.479184680524,-353.404582828373,
-353.330048544799,-353.255579987264,-353.181149771671,-353.10674485987,
-353.054496627282,-352.974199378859,-352.893756905955,-352.809099369304,
-352.728319222888,-352.647437711954,-352.566420911552,-352.555126759351,
-352.480597289582,-352.406143961265,-352.33175287161,-352.257410158957,
-352.183101993942,-352.108814571024,-352.034519025254,-351.960214519186,
-351.885888555835,-351.811528629219,-351.737082946309,-351.662588093133,
-351.587991147452,-351.556387023488,-351.483248079804,-351.410197162497,
-351.337219338475,-351.264299743959,-351.191423568983,-351.118576043401,
-351.045728546241,-350.972877397704,-350.900009248603,-350.82711073855,
-350.754125296988,-350.681092484212,-350.607948060094,-350.557647287626,
-350.482812503093,-350.408063623116,-350.333386917726,-350.258768704072,
-350.184198468804,-350.109654671839,-350.035124995162,-349.960597130254,
-349.886032136981,-349.811449289414,-349.73679721459,-349.668434343951),
 .UNSPECIFIED.);
#3582=B_SPLINE_CURVE_WITH_KNOTS('',3,(#231361,#231362,#231363,#231364,#231365,
#231366,#231367,#231368,#231369,#231370,#231371,#231372,#231373,#231374,
#231375,#231376,#231377,#231378,#231379,#231380,#231381,#231382,#231383,
#231384,#231385,#231386,#231387,#231388,#231389,#231390,#231391,#231392,
#231393,#231394,#231395,#231396,#231397,#231398,#231399,#231400,#231401,
#231402,#231403,#231404,#231405,#231406,#231407,#231408,#231409,#231410,
#231411,#231412,#231413,#231414,#231415,#231416,#231417,#231418,#231419,
#231420,#231421,#231422,#231423,#231424,#231425,#231426,#231427,#231428,
#231429,#231430,#231431,#231432,#231433,#231434,#231435,#231436,#231437,
#231438,#231439,#231440,#231441,#231442,#231443,#231444,#231445,#231446,
#231447,#231448,#231449,#231450,#231451,#231452,#231453,#231454,#231455,
#231456,#231457,#231458,#231459,#231460,#231461,#231462,#231463,#231464,
#231465,#231466,#231467,#231468,#231469,#231470,#231471,#231472,#231473,
#231474,#231475,#231476,#231477,#231478,#231479,#231480,#231481,#231482,
#231483,#231484,#231485,#231486,#231487,#231488,#231489,#231490,#231491,
#231492,#231493,#231494,#231495,#231496,#231497,#231498,#231499,#231500,
#231501,#231502,#231503,#231504,#231505,#231506,#231507,#231508,#231509,
#231510,#231511,#231512,#231513,#231514,#231515,#231516,#231517,#231518,
#231519,#231520,#231521,#231522,#231523,#231524,#231525,#231526,#231527,
#231528,#231529,#231530,#231531,#231532,#231533,#231534,#231535,#231536,
#231537,#231538,#231539,#231540,#231541,#231542,#231543,#231544,#231545,
#231546,#231547,#231548,#231549,#231550,#231551,#231552,#231553,#231554,
#231555,#231556,#231557,#231558,#231559,#231560,#231561,#231562,#231563,
#231564,#231565,#231566,#231567,#231568,#231569,#231570,#231571,#231572,
#231573,#231574,#231575,#231576,#231577,#231578,#231579,#231580,#231581,
#231582,#231583,#231584,#231585,#231586,#231587,#231588,#231589,#231590,
#231591,#231592,#231593,#231594,#231595,#231596,#231597,#231598,#231599,
#231600,#231601,#231602,#231603,#231604,#231605,#231606,#231607,#231608,
#231609,#231610,#231611,#231612,#231613,#231614,#231615,#231616,#231617,
#231618,#231619,#231620,#231621,#231622,#231623,#231624,#231625,#231626,
#231627,#231628,#231629,#231630,#231631,#231632,#231633,#231634,#231635,
#231636,#231637,#231638,#231639,#231640,#231641,#231642,#231643,#231644,
#231645,#231646,#231647,#231648,#231649,#231650,#231651,#231652,#231653,
#231654,#231655,#231656,#231657,#231658,#231659,#231660,#231661,#231662,
#231663,#231664,#231665,#231666,#231667,#231668,#231669,#231670,#231671,
#231672,#231673,#231674,#231675,#231676,#231677,#231678,#231679,#231680,
#231681,#231682,#231683,#231684,#231685,#231686,#231687,#231688,#231689,
#231690,#231691,#231692,#231693,#231694,#231695,#231696,#231697,#231698,
#231699,#231700,#231701,#231702,#231703,#231704,#231705,#231706,#231707,
#231708,#231709,#231710,#231711,#231712,#231713,#231714,#231715,#231716,
#231717,#231718,#231719,#231720,#231721,#231722,#231723,#231724,#231725,
#231726,#231727,#231728,#231729,#231730,#231731,#231732,#231733,#231734,
#231735,#231736,#231737,#231738,#231739,#231740,#231741,#231742,#231743,
#231744,#231745,#231746,#231747,#231748,#231749,#231750,#231751,#231752,
#231753,#231754,#231755,#231756,#231757,#231758,#231759,#231760,#231761,
#231762,#231763,#231764,#231765,#231766,#231767,#231768,#231769,#231770,
#231771,#231772,#231773,#231774,#231775,#231776,#231777,#231778,#231779,
#231780,#231781,#231782,#231783,#231784,#231785,#231786,#231787,#231788,
#231789,#231790,#231791,#231792,#231793,#231794,#231795,#231796,#231797,
#231798,#231799,#231800,#231801,#231802,#231803,#231804,#231805,#231806,
#231807,#231808,#231809,#231810,#231811,#231812,#231813,#231814,#231815,
#231816,#231817,#231818,#231819,#231820,#231821,#231822,#231823,#231824,
#231825,#231826,#231827,#231828,#231829,#231830,#231831,#231832,#231833,
#231834,#231835,#231836,#231837,#231838,#231839,#231840,#231841,#231842,
#231843,#231844,#231845,#231846,#231847,#231848,#231849,#231850,#231851,
#231852,#231853,#231854,#231855,#231856,#231857,#231858,#231859,#231860,
#231861,#231862,#231863,#231864,#231865,#231866,#231867,#231868,#231869,
#231870),.UNSPECIFIED.,.F.,.F.,(4,2,2,2,2,2,2,2,2,2,2,2,2,2,2,2,2,2,2,2,
2,2,2,2,2,2,2,2,2,2,2,2,2,2,2,2,2,2,2,2,2,2,2,2,2,2,2,2,2,2,2,2,2,2,2,2,
2,2,2,2,2,2,2,2,2,2,2,2,2,2,2,2,2,2,2,2,2,2,2,2,2,2,2,2,2,2,2,2,2,2,2,2,
2,2,2,2,2,2,2,2,2,2,2,2,2,2,2,2,2,2,2,2,2,2,2,2,2,2,2,2,2,2,2,2,2,2,2,2,
2,2,2,2,2,2,2,2,2,2,2,2,2,2,2,2,2,2,2,2,2,2,2,2,2,2,2,2,2,2,2,2,2,2,2,2,
2,2,2,2,2,2,2,2,2,2,2,2,2,2,2,2,2,2,2,2,2,2,2,2,2,2,2,2,2,2,2,2,2,2,2,2,
2,2,2,2,2,2,2,2,2,2,2,2,2,2,2,2,2,2,2,2,2,2,2,2,2,2,2,2,2,2,2,2,2,2,2,2,
2,2,2,2,2,2,2,2,2,2,2,2,2,2,2,2,2,2,4),(0.00112295043593974,0.107857761231311,
0.114052241037512,0.11753262099607,0.119876263535378,0.121786873765044,
0.123780062850454,0.126142361503766,0.130245616857605,0.146206662253084,
0.275373782427591,0.298248501714585,0.481116090907697,0.551258197698067,
0.561954403051901,0.569030521095548,0.575812313285773,0.58180525133378,
0.589315278962869,0.603815309583193,0.727213567684471,0.811149694425183,
0.867790479377148,0.878519070755276,0.882738884083325,0.885764054322842,
0.887785260694388,0.891662747752114,0.899521235632171,0.961118701627771,
0.991983501862881,1.09959451863446,1.15389657070839,1.18264477335284,1.19097144595685,
1.1990663375337,1.20633371589231,1.21562257141657,1.23061280904579,1.30388785569167,
1.39752278481727,1.5260173359784,1.59690886178953,1.62292528742539,1.63716266103208,
1.64075322826951,1.64250785486455,1.64415262475517,1.64592156107976,1.64845460840261,
1.65545593457385,1.7271548492867,1.75184942887734,1.90829040079901,1.93818210128818,
2.00678198508029,2.05092922827064,2.05660833427005,2.05944714554916,2.06148541949694,
2.06363986052975,2.06727140512236,2.07687513308396,2.22018732039301,2.29787265950914,
2.41440600941893,2.46123301989485,2.46930129331774,2.47190908974559,2.47358480724344,
2.47513370139148,2.47712916470635,2.48041827605827,2.49871540572181,2.68896916872065,
2.80850992496078,2.82928211024011,2.83553226289197,2.83975436237766,2.84358602778225,
2.84851409156694,2.85643707689237,2.89396366801267,3.13522414108122,3.20594768434382,
3.21301668193643,3.21825708861012,3.22062456065244,3.22241122187724,3.22406618882445,
3.22631931655624,3.23074323398895,3.26907822257239,3.48483465793414,3.606016289264,
3.61240072429383,3.61523788931165,3.61734126710108,3.61929386823524,3.62195869187147,
3.62859429587152,3.70126098194594,3.75450237641733,3.88486956360218,3.97351805365338,
4.01756102919334,4.03594836859251,4.03865911356981,4.04004520238173,4.04105265575698,
4.0421289104894,4.04398638815591,4.04925626816744,4.13321670647967,4.32706869089585,
4.43356477957858,4.43944980757982,4.44212594332586,4.44413474111292,4.44601756874773,
4.44861539316056,4.45523177561149,4.53708738527925,4.71795624852287,4.7730462506962,
4.82685711183819,4.83466889334435,4.83680424019092,4.83810597188383,4.8392807073837,
4.84077978189214,4.84315755514824,4.85499520050329,4.89548550671736,4.97743828454832,
5.14289378391396,5.24552568332095,5.25296970987121,5.25583947659063,5.25790154105346,
5.26008513331391,5.26296635075888,5.26919361511967,5.36041122273955,5.58784091811462,
5.64983572182749,5.6557462016845,5.65842500768345,5.66047005379632,5.66264924614495,
5.66604149439303,5.67644366504155,5.80844313803825,6.02920781335209,6.03212123698015,
6.03291018219741,6.03962697243758,6.09351236530757,6.1056440790818,6.11262479733669,
6.11859950671055,6.12584225110404,6.13952303010811,6.2330848856891,6.38093547007934,
6.41184455655155,6.41800078969678,6.4215134612741,6.42423651430679,6.42779226694364,
6.434158619028,6.46464776615813,6.68090148649987,6.71743753095939,6.7294823224904,
6.73657986852364,6.74311113862535,6.75197839879513,6.76919525900418,6.86613477588839,
6.9957181482243,7.12636138773892,7.16298460680583,7.17499715609568,7.17849922917028,
7.18056393430239,7.18220262904189,7.18438600597253,7.18842795298414,7.20994954403043,
7.2483432632449,7.38078843922027,7.57889553757676,7.59143892739234,7.5954897233255,
7.59772731538535,7.59996927580979,7.60267619458662,7.60779231263027,7.61420491967219,
7.73416011782752,7.87000006968885,7.99861036794204,8.0066985499553,8.0094043524844,
8.0109208253831,8.01244061825881,8.01434618235529,8.01806049937145,8.0430661105764,
8.10635300393819,8.28753627468491,8.3602344302799,8.37026869583972,8.37517339317417,
8.37894566852037,8.38308013039411,8.38957946152218,8.40926838715509,8.51212648697745,
8.7291806888181,8.7517013395258,8.75554979194496,8.75785709171259,8.75963198644352,
8.76153649070127,8.7645277982498,8.77389350866761,8.82409056768681,8.94394991238551,
9.00072061672186,9.08605060986792,9.14286500119761,9.14919479646023,9.15173921741696,
9.15385400417221,9.15579629143257,9.15871867891198,9.16560485203871,9.17502846607691,
9.1987526885668,9.26190345048189,9.47695637213122,9.50088516645802,9.50885250652798,
9.57084860559634,9.57488558648574,9.57639754210294,9.5774692007131,9.57847856087551,
9.57987837702897,9.58271392282284,9.60678763708164,9.68405601565054,9.95413096362147),
 .UNSPECIFIED.);
#3583=B_SPLINE_CURVE_WITH_KNOTS('',3,(#231872,#231873,#231874,#231875,#231876,
#231877,#231878,#231879,#231880,#231881,#231882,#231883,#231884,#231885,
#231886,#231887,#231888,#231889,#231890,#231891,#231892,#231893,#231894,
#231895,#231896,#231897,#231898,#231899,#231900,#231901,#231902,#231903,
#231904,#231905,#231906,#231907,#231908,#231909,#231910,#231911,#231912,
#231913,#231914,#231915,#231916,#231917,#231918,#231919,#231920,#231921,
#231922,#231923,#231924,#231925,#231926,#231927,#231928,#231929,#231930,
#231931,#231932,#231933,#231934,#231935,#231936,#231937,#231938,#231939,
#231940,#231941,#231942,#231943,#231944,#231945,#231946,#231947,#231948,
#231949,#231950,#231951,#231952,#231953,#231954,#231955,#231956,#231957,
#231958,#231959,#231960,#231961,#231962,#231963,#231964,#231965,#231966,
#231967,#231968,#231969,#231970,#231971,#231972,#231973,#231974,#231975,
#231976,#231977,#231978,#231979,#231980,#231981,#231982,#231983,#231984,
#231985,#231986,#231987,#231988,#231989,#231990,#231991,#231992,#231993,
#231994,#231995,#231996,#231997,#231998,#231999,#232000,#232001,#232002,
#232003,#232004,#232005,#232006,#232007,#232008,#232009,#232010,#232011,
#232012,#232013,#232014,#232015,#232016,#232017,#232018,#232019,#232020,
#232021,#232022,#232023,#232024,#232025,#232026,#232027,#232028,#232029,
#232030,#232031,#232032,#232033,#232034,#232035,#232036,#232037,#232038,
#232039,#232040,#232041,#232042,#232043,#232044,#232045,#232046,#232047,
#232048,#232049,#232050,#232051,#232052,#232053,#232054,#232055,#232056,
#232057,#232058,#232059,#232060,#232061,#232062,#232063,#232064,#232065,
#232066,#232067,#232068,#232069,#232070,#232071,#232072,#232073,#232074,
#232075,#232076,#232077,#232078,#232079,#232080,#232081,#232082,#232083,
#232084,#232085,#232086,#232087,#232088,#232089,#232090,#232091,#232092,
#232093,#232094,#232095,#232096,#232097,#232098,#232099,#232100,#232101,
#232102,#232103,#232104,#232105,#232106,#232107,#232108,#232109,#232110,
#232111,#232112,#232113,#232114,#232115,#232116,#232117,#232118,#232119,
#232120,#232121,#232122,#232123,#232124,#232125,#232126,#232127,#232128,
#232129,#232130,#232131,#232132,#232133,#232134,#232135,#232136,#232137,
#232138,#232139,#232140,#232141,#232142,#232143,#232144,#232145,#232146,
#232147,#232148,#232149,#232150,#232151,#232152,#232153,#232154,#232155,
#232156,#232157,#232158,#232159,#232160,#232161,#232162,#232163,#232164,
#232165,#232166,#232167,#232168,#232169,#232170,#232171,#232172,#232173,
#232174,#232175,#232176,#232177,#232178,#232179,#232180,#232181,#232182,
#232183,#232184,#232185,#232186,#232187,#232188,#232189,#232190,#232191,
#232192,#232193,#232194,#232195,#232196,#232197,#232198,#232199,#232200,
#232201,#232202,#232203,#232204,#232205,#232206,#232207,#232208,#232209,
#232210,#232211,#232212,#232213,#232214,#232215,#232216,#232217,#232218,
#232219,#232220,#232221,#232222,#232223,#232224,#232225,#232226,#232227,
#232228,#232229,#232230,#232231,#232232,#232233,#232234,#232235,#232236,
#232237,#232238,#232239,#232240,#232241,#232242,#232243,#232244,#232245,
#232246,#232247,#232248,#232249,#232250,#232251,#232252,#232253,#232254,
#232255,#232256,#232257,#232258,#232259,#232260,#232261,#232262,#232263,
#232264,#232265,#232266,#232267,#232268,#232269,#232270,#232271,#232272,
#232273,#232274,#232275,#232276,#232277,#232278,#232279,#232280,#232281,
#232282,#232283,#232284,#232285,#232286,#232287,#232288,#232289,#232290,
#232291,#232292,#232293,#232294,#232295,#232296,#232297,#232298,#232299,
#232300,#232301,#232302,#232303,#232304,#232305,#232306,#232307,#232308,
#232309,#232310,#232311,#232312,#232313,#232314,#232315,#232316,#232317,
#232318,#232319,#232320,#232321,#232322,#232323,#232324,#232325,#232326,
#232327,#232328,#232329,#232330,#232331,#232332,#232333,#232334,#232335,
#232336,#232337,#232338,#232339,#232340,#232341,#232342,#232343,#232344,
#232345,#232346,#232347,#232348,#232349,#232350,#232351,#232352,#232353,
#232354,#232355,#232356,#232357,#232358,#232359,#232360,#232361,#232362,
#232363,#232364,#232365,#232366,#232367,#232368,#232369,#232370,#232371,
#232372,#232373,#232374,#232375,#232376,#232377,#232378,#232379,#232380,
#232381,#232382,#232383,#232384,#232385,#232386,#232387,#232388,#232389,
#232390,#232391,#232392,#232393,#232394,#232395,#232396,#232397,#232398,
#232399,#232400,#232401,#232402,#232403,#232404,#232405,#232406,#232407,
#232408,#232409,#232410,#232411,#232412,#232413,#232414,#232415,#232416,
#232417,#232418,#232419,#232420,#232421,#232422,#232423,#232424,#232425,
#232426,#232427,#232428,#232429,#232430,#232431,#232432,#232433,#232434,
#232435),.UNSPECIFIED.,.F.,.F.,(4,2,2,2,2,2,2,2,2,2,2,2,2,2,2,2,2,2,2,2,
2,2,2,2,2,2,2,2,2,2,2,2,2,2,2,2,2,2,2,2,2,2,2,2,2,2,2,2,2,2,2,2,2,2,2,2,
2,2,2,2,2,2,2,2,2,2,2,2,2,2,2,2,2,2,2,2,2,2,2,2,2,2,2,2,2,2,2,2,2,2,2,2,
2,2,2,2,2,2,2,2,2,2,2,2,2,2,2,2,2,2,2,2,2,2,2,2,2,2,2,2,2,2,2,2,2,2,2,2,
2,2,2,2,2,2,2,2,2,2,2,2,2,2,2,2,2,2,2,2,2,2,2,2,2,2,2,2,2,2,2,2,2,2,2,2,
2,2,2,2,2,2,2,2,2,2,2,2,2,2,2,2,2,2,2,2,2,2,2,2,2,2,2,2,2,2,2,2,2,2,2,2,
2,2,2,2,2,2,2,2,2,2,2,2,2,2,2,2,2,2,2,2,2,2,2,2,2,2,2,2,2,2,2,2,2,2,2,2,
2,2,2,2,2,2,2,2,2,2,2,2,2,2,2,2,2,2,2,2,2,2,2,2,2,2,2,2,2,2,2,2,2,2,2,2,
2,2,2,2,2,2,2,2,2,4),(0.0032206418046776,0.0210815066455308,0.0247042507456413,
0.0270909668341338,0.0289948856039576,0.030956571544407,0.033214350708931,
0.0370668490571024,0.050425706038174,0.0620697250116354,0.353057957478074,
0.385273656061949,0.405409759524707,0.421049422028272,0.423676422408627,
0.425087103529002,0.426141876280886,0.427297560028865,0.428990064128685,
0.433907907077473,0.515931179852567,0.73650149141895,0.800117252920412,
0.824252461611661,0.833899344259589,0.840885907074259,0.8439551733344,0.845984027311522,
0.848190726433849,0.850836312029805,0.857119975050606,0.908794956654506,
1.01523386745463,1.07849304557427,1.09715152519909,1.15506181007503,1.22874672678773,
1.24123594825736,1.24486812448472,1.24710134196542,1.24912998606215,1.25173825949375,
1.25694708520209,1.29009327122796,1.49492160947072,1.62439221179749,1.68165307843147,
1.69366231132888,1.70054652176404,1.70652974236568,1.71368481878407,1.72457364687925,
1.76331773546716,1.77132589907341,1.81691928737767,1.92389715881651,1.97576795349413,
2.00073405597256,2.00629000915767,2.00964992742166,2.01269944769531,2.01662002904365,
2.02473876563319,2.12246582381584,2.22612994589353,2.27471633215386,2.30699490280657,
2.31835159170384,2.32598326567893,2.33336024675526,2.34346546601538,2.36696470916073,
2.40068737829753,2.47660581004675,2.63053530187008,2.74870457837365,2.76266715475535,
2.76619991018831,2.76827197933312,2.7700922094825,2.77235008735283,2.77580480011788,
2.79106481552979,3.03152603787664,3.11878106124968,3.17028949982466,3.17707609948838,
3.18243269440358,3.18519324082447,3.18722854893409,3.18939162628324,3.19244695733074,
3.19880297860454,3.26739163782652,3.42013159838122,3.52398098310493,3.55901338400802,
3.5928386585894,3.5967075923737,3.59864550039752,3.6000387254337,3.60151292431991,
3.60358520317242,3.60907664869178,3.61342172824158,3.61947896731472,3.62682603539969,
3.62892996612677,3.76689450369097,3.94803417659746,3.95867418631668,3.96368432408664,
3.96752724255743,3.9711963136118,3.97742221081651,3.9937553964033,4.03033585854662,
4.2383565476632,4.31164769041488,4.34025402838042,4.34450033823187,4.34667980305043,
4.34841863255329,4.35015418631263,4.35325262327839,4.36252836817173,4.50748641265443,
4.62861042566123,4.7017140133385,4.73377783731544,4.73872804177424,4.74128560384759,
4.74333410019072,4.74568674279962,4.74969242080386,4.76350594980729,4.96944792107184,
4.98269894529362,5.14102443446203,5.16146583148092,5.1645153245062,5.16595452310382,
5.16707719543242,5.16829715355923,5.17026541232617,5.17703635336674,5.21975295382772,
5.27732771800372,5.44132576940524,5.55696655520913,5.56465362800154,5.56742371587753,
5.56935380460868,5.57114531401955,5.57358695461421,5.57828453803244,5.60780233278795,
5.67303390219221,5.7386473075883,5.7959334123614,5.93580992220177,5.95915834182736,
5.96201723540035,5.96349428641046,5.96459182050953,5.96578879146311,5.96742916049262,
5.97123147063057,6.03429608349821,6.18486740598433,6.36544184241586,6.37793733696198,
6.38189171012615,6.38405704260124,6.38599866751159,6.38854623492465,6.39313825259284,
6.41503353879074,6.45619640237481,6.55842925719197,6.66059367903474,6.77163237177265,
6.78071813420437,6.7840521485203,6.78600158142916,6.78799101681612,6.79053907128206,
6.79333878228997,6.79792316627911,6.80712543683528,6.91514253963537,7.07405388093739,
7.08430748019835,7.21121244470401,7.22863055207428,7.23663913729507,7.24271621870402,
7.24918221776059,7.2592793271078,7.27108715926858,7.41103220822256,7.52897613667893,
7.54147668653348,7.54596300330288,7.54907122568415,7.55213369856453,7.55647370570668,
7.56690092774815,7.58165456246179,7.62305917260627,7.69306944835078,7.79580074871121,
7.84153941857464,7.85492986694404,7.86299948143802,7.86954336113563,7.87850707924674,
7.89620010989325,7.99645834816143,8.13318567781716,8.28191368613601,8.2836649203808,
8.28497876142606,8.29351949998282,8.3022314808724,8.30531407847945,8.3070888558898,
8.308858960583,8.31111149245552,8.31549247171402,8.32101189585491,8.33294845516719,
8.36637850472788,8.44503178625175,8.61744580600723,8.64896195620345,8.71307323156934,
8.71931714347526,8.72234488298367,8.7245003765125,8.72653826396476,8.72937433306842,
8.73503992202204,8.77871120401351,8.89525715032246,8.91541235140057,8.93235780893388,
8.94690265630715,8.95956117281509,8.97068929231293,9.06712488805322,9.12964381189146,
9.13436217075744,9.13630347640733,9.13774314035973,9.13920704466464,9.14073816984089,
9.14429134384458,9.16554268333411,9.21218503153921,9.2614649244329,9.39844391353661,
9.4859834721567,9.49668735608423,9.50165514882539,9.50550397493303,9.50966606207296,
9.51628637525377,9.53687817624927,9.64758675553711,9.79655125727371,9.80873977005857,
9.85039853072301,9.87763383153486,9.88211261691432,9.88437049508769,9.88613333962904,
9.88777133884977,9.88967301624833,9.89237281830234,9.8969677328629,9.95836513107871),
 .UNSPECIFIED.);
#3584=B_SPLINE_CURVE_WITH_KNOTS('',3,(#232437,#232438,#232439,#232440,#232441,
#232442,#232443,#232444,#232445,#232446,#232447,#232448,#232449,#232450,
#232451,#232452,#232453,#232454,#232455,#232456,#232457,#232458,#232459,
#232460,#232461,#232462,#232463,#232464,#232465,#232466,#232467,#232468,
#232469,#232470,#232471,#232472,#232473,#232474,#232475,#232476,#232477,
#232478,#232479,#232480,#232481,#232482,#232483,#232484,#232485,#232486,
#232487,#232488,#232489,#232490,#232491,#232492,#232493,#232494,#232495,
#232496,#232497,#232498,#232499,#232500,#232501,#232502,#232503,#232504,
#232505,#232506,#232507,#232508,#232509,#232510,#232511,#232512,#232513,
#232514,#232515,#232516,#232517,#232518,#232519,#232520,#232521,#232522,
#232523,#232524,#232525,#232526,#232527,#232528,#232529,#232530,#232531,
#232532,#232533,#232534,#232535,#232536,#232537,#232538,#232539,#232540,
#232541,#232542,#232543,#232544,#232545,#232546,#232547,#232548,#232549,
#232550,#232551,#232552,#232553,#232554,#232555,#232556,#232557,#232558,
#232559,#232560,#232561,#232562,#232563,#232564,#232565,#232566,#232567,
#232568,#232569,#232570,#232571,#232572,#232573,#232574,#232575,#232576,
#232577,#232578,#232579,#232580,#232581,#232582,#232583,#232584,#232585,
#232586,#232587,#232588,#232589,#232590,#232591,#232592,#232593,#232594,
#232595,#232596,#232597,#232598,#232599,#232600,#232601,#232602,#232603,
#232604,#232605,#232606,#232607,#232608,#232609,#232610,#232611,#232612,
#232613,#232614,#232615,#232616,#232617,#232618,#232619,#232620,#232621,
#232622,#232623,#232624,#232625,#232626,#232627,#232628,#232629,#232630,
#232631,#232632,#232633,#232634,#232635,#232636,#232637,#232638,#232639,
#232640,#232641,#232642,#232643,#232644,#232645,#232646,#232647,#232648,
#232649,#232650,#232651,#232652,#232653,#232654,#232655,#232656,#232657,
#232658,#232659,#232660,#232661,#232662,#232663,#232664,#232665,#232666,
#232667,#232668,#232669,#232670,#232671,#232672,#232673,#232674,#232675,
#232676,#232677,#232678,#232679,#232680,#232681,#232682,#232683,#232684,
#232685,#232686,#232687,#232688,#232689,#232690,#232691,#232692,#232693,
#232694,#232695),.UNSPECIFIED.,.F.,.F.,(4,3,3,3,3,3,3,3,3,3,3,3,3,3,3,3,
3,3,3,3,3,3,3,3,3,3,3,3,3,3,3,3,3,3,3,3,3,3,3,3,3,3,3,3,3,3,3,3,3,3,3,3,
3,3,3,3,3,3,3,3,3,3,3,3,3,3,3,3,3,3,3,3,3,3,3,3,3,3,3,3,3,3,3,3,3,3,4),
(-324.535381086289,-324.461322539534,-324.387335999405,-324.313407189673,
-324.239521874744,-324.165665849949,-324.091812204043,-324.017956628568,
-323.944086283212,-323.870188321613,-323.796208072316,-323.722183693228,
-323.648051467166,-323.591674419347,-323.518535475663,-323.445484558356,
-323.372506734333,-323.299587139818,-323.226710964842,-323.15386343926,
-323.0810159421,-323.008164793562,-322.935296644461,-322.862398134409,-322.789412692846,
-322.71637988007,-322.643235455953,-322.592934683485,-322.517406394818,
-322.441964199485,-322.36659519179,-322.291286513827,-322.216025347427,
-322.138296547451,-322.063086350126,-321.987882125428,-321.912672315163,
-321.837445360177,-321.762162470567,-321.686846423697,-321.61145951444,
-321.594194947623,-321.517603047222,-321.441076345282,-321.36460514939,
-321.288188289129,-321.211804250295,-321.135444086883,-321.094825079692,
-321.016705811213,-320.938541507739,-320.860327430751,-320.782022308062,
-320.703668881464,-320.625229791698,-320.595455211761,-320.513476433175,
-320.431569683936,-320.347698598909,-320.266033186396,-320.181059265113,
-320.09608534383,-320.022473669723,-319.948867302869,-319.875253250966,
-319.801586958436,-319.727893430411,-319.654117957344,-319.596715475898,
-319.520214751092,-319.443769983911,-319.367370264331,-319.291004714725,
-319.214662482534,-319.137576639722,-319.061234826346,-318.984882738703,
-318.908510514596,-318.830876820956,-318.754405143963,-318.676190441999,
-318.597975740036,-318.518993131618,-318.440204240229,-318.361532828754,
-318.283021502504,-318.252195779109),.UNSPECIFIED.);
#3585=B_SPLINE_CURVE_WITH_KNOTS('',3,(#232697,#232698,#232699,#232700,#232701,
#232702,#232703,#232704,#232705,#232706,#232707,#232708,#232709,#232710,
#232711,#232712,#232713,#232714,#232715,#232716,#232717,#232718,#232719,
#232720,#232721,#232722,#232723,#232724,#232725,#232726,#232727,#232728,
#232729,#232730,#232731,#232732,#232733,#232734,#232735,#232736,#232737,
#232738,#232739,#232740,#232741,#232742,#232743,#232744,#232745,#232746,
#232747,#232748,#232749,#232750,#232751,#232752,#232753,#232754,#232755,
#232756,#232757,#232758,#232759,#232760,#232761,#232762,#232763,#232764,
#232765,#232766,#232767,#232768,#232769,#232770,#232771,#232772,#232773,
#232774,#232775,#232776,#232777,#232778,#232779,#232780,#232781,#232782,
#232783,#232784,#232785,#232786,#232787,#232788,#232789,#232790,#232791,
#232792,#232793,#232794,#232795,#232796,#232797,#232798,#232799,#232800,
#232801,#232802,#232803,#232804,#232805,#232806,#232807,#232808,#232809,
#232810,#232811,#232812,#232813,#232814,#232815,#232816,#232817,#232818,
#232819,#232820,#232821,#232822,#232823,#232824,#232825,#232826,#232827,
#232828,#232829,#232830,#232831,#232832,#232833,#232834,#232835,#232836,
#232837,#232838,#232839,#232840,#232841,#232842,#232843,#232844,#232845,
#232846,#232847,#232848,#232849,#232850,#232851,#232852,#232853,#232854,
#232855,#232856,#232857,#232858,#232859,#232860,#232861,#232862,#232863,
#232864,#232865,#232866,#232867,#232868,#232869,#232870,#232871,#232872,
#232873,#232874,#232875,#232876,#232877,#232878,#232879,#232880,#232881,
#232882,#232883,#232884,#232885,#232886,#232887,#232888,#232889,#232890,
#232891,#232892,#232893,#232894,#232895,#232896,#232897,#232898,#232899,
#232900,#232901,#232902,#232903,#232904,#232905,#232906,#232907,#232908,
#232909,#232910,#232911,#232912,#232913,#232914,#232915,#232916,#232917,
#232918,#232919,#232920,#232921,#232922,#232923,#232924,#232925,#232926,
#232927,#232928,#232929,#232930,#232931,#232932,#232933,#232934,#232935,
#232936,#232937,#232938,#232939,#232940,#232941,#232942,#232943,#232944,
#232945,#232946,#232947,#232948,#232949,#232950,#232951,#232952,#232953,
#232954,#232955,#232956,#232957,#232958,#232959,#232960,#232961,#232962,
#232963,#232964,#232965,#232966,#232967,#232968,#232969,#232970,#232971,
#232972,#232973,#232974,#232975,#232976,#232977,#232978,#232979,#232980,
#232981,#232982,#232983,#232984,#232985,#232986,#232987,#232988,#232989,
#232990,#232991,#232992,#232993,#232994,#232995,#232996,#232997,#232998,
#232999,#233000,#233001,#233002,#233003,#233004,#233005,#233006,#233007,
#233008,#233009,#233010,#233011,#233012,#233013,#233014,#233015,#233016,
#233017,#233018,#233019,#233020,#233021,#233022,#233023,#233024,#233025,
#233026,#233027,#233028,#233029,#233030,#233031,#233032,#233033,#233034,
#233035,#233036,#233037,#233038,#233039,#233040,#233041,#233042,#233043,
#233044,#233045,#233046,#233047,#233048,#233049,#233050,#233051,#233052,
#233053,#233054,#233055,#233056,#233057,#233058,#233059,#233060,#233061,
#233062,#233063,#233064,#233065,#233066,#233067,#233068,#233069,#233070,
#233071,#233072,#233073,#233074,#233075,#233076,#233077,#233078,#233079,
#233080,#233081,#233082,#233083,#233084,#233085,#233086,#233087,#233088,
#233089,#233090,#233091,#233092,#233093,#233094,#233095,#233096,#233097,
#233098,#233099,#233100,#233101,#233102,#233103,#233104,#233105,#233106,
#233107,#233108,#233109,#233110,#233111,#233112,#233113,#233114,#233115,
#233116,#233117,#233118,#233119,#233120,#233121,#233122,#233123,#233124,
#233125,#233126,#233127,#233128,#233129,#233130,#233131,#233132,#233133,
#233134,#233135,#233136,#233137,#233138,#233139,#233140,#233141,#233142,
#233143,#233144,#233145,#233146,#233147,#233148,#233149,#233150,#233151,
#233152,#233153,#233154,#233155,#233156,#233157,#233158,#233159,#233160,
#233161,#233162,#233163,#233164,#233165,#233166,#233167,#233168,#233169,
#233170,#233171,#233172,#233173,#233174,#233175,#233176,#233177,#233178,
#233179,#233180,#233181,#233182,#233183,#233184,#233185,#233186,#233187,
#233188,#233189,#233190,#233191,#233192,#233193,#233194,#233195,#233196,
#233197,#233198),.UNSPECIFIED.,.F.,.F.,(4,2,2,2,2,2,2,2,2,2,2,2,2,2,2,2,
2,2,2,2,2,2,2,2,2,2,2,2,2,2,2,2,2,2,2,2,2,2,2,2,2,2,2,2,2,2,2,2,2,2,2,2,
2,2,2,2,2,2,2,2,2,2,2,2,2,2,2,2,2,2,2,2,2,2,2,2,2,2,2,2,2,2,2,2,2,2,2,2,
2,2,2,2,2,2,2,2,2,2,2,2,2,2,2,2,2,2,2,2,2,2,2,2,2,2,2,2,2,2,2,2,2,2,2,2,
2,2,2,2,2,2,2,2,2,2,2,2,2,2,2,2,2,2,2,2,2,2,2,2,2,2,2,2,2,2,2,2,2,2,2,2,
2,2,2,2,2,2,2,2,2,2,2,2,2,2,2,2,2,2,2,2,2,2,2,2,2,2,2,2,2,2,2,2,2,2,2,2,
2,2,2,2,2,2,2,2,2,2,2,2,2,2,2,2,2,2,2,2,2,2,2,2,2,2,2,2,2,2,2,2,2,2,2,2,
2,2,2,2,2,2,2,2,2,2,2,2,2,2,2,2,2,2,4),(0.00121348254971357,0.0844218198558422,
0.0938908223239574,0.0995313570605865,0.103568722924125,0.107122786700612,
0.110982982662361,0.116020140960127,0.127045063186039,0.202337357354917,
0.223548934817849,0.41236865835311,0.45999701856791,0.481978766425379,0.485944302503179,
0.488064681781256,0.489645790598398,0.49162592270192,0.494952698098768,
0.506037432433198,0.664169816120028,0.703088453675587,0.740702436756285,
0.873118102024691,0.879345226483091,0.882154392177681,0.884253945898625,
0.886215218605446,0.888910923892993,0.89572233686709,0.976101250752053,
0.995824217702251,1.07690379222896,1.16463032242153,1.19717713056531,1.24822317687767,
1.29674388054704,1.30413339346925,1.3061914227682,1.30743595353808,1.30855258424657,
1.30997039499775,1.31223788006559,1.32401417485332,1.5147928207457,1.61981545740611,
1.67543314668045,1.7027385224526,1.70736475114492,1.70979125675229,1.71158089231656,
1.71351789017113,1.71689768993709,1.72651793240158,1.86784129999972,1.9934495171053,
2.04361259485488,2.09218373487637,2.10171270357673,2.10399199124184,2.10532632758646,
2.10649652235821,2.10794508851437,2.11015868318238,2.11985027955127,2.1631622147198,
2.29159962793086,2.43201702828084,2.51511024396737,2.52126904679386,2.52413803445429,
2.52632060264184,2.52838790489381,2.53185090819893,2.54089181687515,2.67737341746246,
2.8106270386984,2.86104786617758,2.89671188749953,2.91960222083244,2.92403151039003,
2.92644104182935,2.92843475022784,2.93079920729671,2.93491007149538,2.95094460912242,
2.96234391471357,3.1473631002315,3.35333733438873,3.37040884544617,3.37831617020363,
3.38435726405786,3.39092492367593,3.40148312175346,3.43419333811076,3.55957373021619,
3.66762151305439,3.67753608564849,3.68500610339691,3.68872712527851,3.69146762592415,
3.69443200852598,3.69871470392511,3.7108461594919,3.84368802674237,3.97746397191585,
3.99393622541746,4.00266612862714,4.00919111258611,4.01742321659748,4.03158679962271,
4.08882938149597,4.20846239901833,4.35636008293556,4.43222836102517,4.43958541959908,
4.44506498827798,4.44753647773335,4.44938407780453,4.45111000103136,4.45348249100253,
4.45948207722142,4.52180264480049,4.73219138048668,4.85463960363688,4.86165294335743,
4.86474824260393,4.86703472227711,4.86915151742863,4.87203163315172,4.87915931552144,
4.9562021062755,4.97915154849782,5.2164716270247,5.27196792397129,5.27619282034345,
5.27825313742188,5.2797241668528,5.2811180557192,5.28306300437236,5.28696581014438,
5.31794020020128,5.37693092113321,5.52774652357561,5.62780566875286,5.63881662368138,
5.64384260131559,5.6477013461789,5.65183958277373,5.65834876045442,5.67809379822284,
5.78139445040959,5.99765580472344,6.02062611636122,6.02450058699412,6.02681624756777,
6.02859331986864,6.0304960005705,6.03347577957996,6.04273725223415,6.09201848481516,
6.12393150813305,6.21285647196616,6.40411712068135,6.41426258337349,6.41877916301148,
6.42149502674862,6.42358711170371,6.42583451083396,6.42936935642802,6.44047140390451,
6.61494864815417,6.7980135238467,6.84099059839442,6.84466713048314,6.84612022645114,
6.84717652714774,6.84830635187796,6.84978949672812,6.85308692451535,6.85752214496301,
6.89956960595399,6.9653520553536,7.22669244407188,7.2434030572105,7.24717452648218,
7.24963511532834,7.25161734319513,7.25387187510414,7.25770966595411,7.27275648340527,
7.38230629116713,7.5857184956636,7.60453891713797,7.63970880731287,7.64290495321987,
7.64446553837621,7.64558474774064,7.6466493550247,7.64811107488101,7.65100963953831,
7.65472859020836,7.81070683397365,7.89530111916282,8.04959797527249,8.05965722849809,
8.06327786963883,8.06537617756431,8.06732962022545,8.07000093913175,8.07517143403037,
8.10869624201312,8.18539530231802,8.30659516009491,8.44729962888903,8.46069265125458,
8.46451083249091,8.46677694187205,8.46875075720316,8.47114132612438,8.4756432653729,
8.49997497170848,8.5537482984691,8.6693217340446,8.79155088950859,8.8161934538348,
8.89872537445595,8.91088729507275,8.91852372787577,8.92452995178897,8.93123572432224,
8.94242321553105,8.9856041182205,9.20142749733787,9.22097401063266,9.22625472040813,
9.22954080256217,9.23228094579009,9.2360213794865,9.24325038851341,9.29347785845239,
9.38529183628633,9.51708001320053,9.5320192117991,9.54132473617372,9.54859554383567,
9.55668236514666,9.57017550939193,9.6266678921445,9.71456334555599,9.9583219418317),
 .UNSPECIFIED.);
#3586=B_SPLINE_CURVE_WITH_KNOTS('',3,(#233200,#233201,#233202,#233203,#233204,
#233205,#233206,#233207,#233208,#233209,#233210,#233211,#233212,#233213,
#233214,#233215,#233216,#233217,#233218,#233219,#233220,#233221,#233222,
#233223,#233224,#233225,#233226,#233227,#233228,#233229,#233230,#233231,
#233232,#233233,#233234,#233235,#233236,#233237,#233238,#233239,#233240,
#233241,#233242,#233243,#233244,#233245,#233246,#233247,#233248,#233249,
#233250,#233251,#233252,#233253,#233254,#233255,#233256,#233257,#233258,
#233259,#233260,#233261,#233262,#233263,#233264,#233265,#233266,#233267,
#233268,#233269,#233270,#233271,#233272,#233273,#233274,#233275,#233276,
#233277,#233278,#233279,#233280,#233281,#233282,#233283,#233284,#233285,
#233286,#233287,#233288,#233289,#233290,#233291,#233292,#233293,#233294,
#233295,#233296,#233297,#233298,#233299,#233300,#233301,#233302,#233303,
#233304,#233305,#233306,#233307,#233308,#233309,#233310,#233311,#233312,
#233313,#233314,#233315,#233316,#233317,#233318,#233319,#233320,#233321,
#233322,#233323,#233324,#233325,#233326,#233327,#233328,#233329,#233330,
#233331,#233332,#233333,#233334,#233335,#233336,#233337,#233338,#233339,
#233340,#233341,#233342,#233343,#233344,#233345,#233346,#233347,#233348,
#233349,#233350,#233351,#233352,#233353,#233354,#233355,#233356,#233357,
#233358,#233359,#233360,#233361,#233362,#233363,#233364,#233365,#233366,
#233367,#233368,#233369,#233370,#233371,#233372,#233373,#233374,#233375,
#233376,#233377,#233378,#233379,#233380,#233381,#233382,#233383,#233384,
#233385,#233386,#233387,#233388,#233389,#233390,#233391,#233392,#233393,
#233394,#233395,#233396,#233397,#233398,#233399,#233400,#233401,#233402,
#233403,#233404,#233405,#233406,#233407,#233408,#233409,#233410,#233411,
#233412,#233413,#233414,#233415,#233416,#233417,#233418,#233419,#233420,
#233421,#233422,#233423,#233424,#233425,#233426,#233427,#233428,#233429,
#233430,#233431,#233432,#233433,#233434,#233435,#233436,#233437,#233438,
#233439,#233440,#233441,#233442,#233443,#233444,#233445,#233446,#233447,
#233448,#233449,#233450,#233451,#233452,#233453,#233454,#233455,#233456,
#233457,#233458,#233459,#233460,#233461,#233462,#233463,#233464,#233465,
#233466,#233467,#233468,#233469,#233470,#233471,#233472,#233473,#233474,
#233475,#233476,#233477,#233478,#233479,#233480,#233481,#233482,#233483,
#233484,#233485,#233486,#233487,#233488,#233489,#233490,#233491,#233492,
#233493,#233494,#233495,#233496,#233497,#233498,#233499,#233500,#233501,
#233502,#233503,#233504,#233505,#233506,#233507,#233508,#233509,#233510,
#233511,#233512,#233513,#233514,#233515,#233516,#233517,#233518,#233519,
#233520,#233521,#233522,#233523,#233524,#233525,#233526,#233527,#233528,
#233529,#233530,#233531,#233532,#233533,#233534,#233535,#233536,#233537,
#233538,#233539,#233540,#233541,#233542,#233543,#233544,#233545,#233546,
#233547,#233548,#233549,#233550,#233551,#233552,#233553,#233554,#233555,
#233556,#233557,#233558,#233559,#233560,#233561,#233562,#233563,#233564,
#233565,#233566,#233567,#233568,#233569,#233570,#233571,#233572,#233573,
#233574,#233575,#233576,#233577,#233578,#233579,#233580,#233581,#233582,
#233583,#233584,#233585,#233586,#233587,#233588,#233589,#233590,#233591,
#233592,#233593,#233594,#233595,#233596,#233597,#233598,#233599,#233600,
#233601,#233602,#233603,#233604,#233605,#233606,#233607,#233608,#233609,
#233610,#233611,#233612,#233613,#233614,#233615,#233616,#233617,#233618,
#233619,#233620,#233621,#233622,#233623,#233624,#233625,#233626,#233627,
#233628,#233629,#233630,#233631,#233632,#233633,#233634,#233635,#233636,
#233637,#233638,#233639,#233640,#233641,#233642,#233643,#233644,#233645,
#233646,#233647,#233648,#233649,#233650,#233651,#233652,#233653,#233654,
#233655,#233656,#233657,#233658,#233659,#233660,#233661,#233662,#233663,
#233664,#233665,#233666,#233667,#233668,#233669,#233670,#233671,#233672,
#233673,#233674,#233675,#233676,#233677,#233678,#233679,#233680,#233681,
#233682,#233683,#233684,#233685,#233686,#233687,#233688,#233689,#233690,
#233691,#233692,#233693,#233694,#233695,#233696,#233697,#233698,#233699,
#233700,#233701,#233702,#233703,#233704,#233705,#233706,#233707,#233708,
#233709,#233710,#233711,#233712,#233713,#233714,#233715,#233716,#233717,
#233718,#233719,#233720,#233721,#233722,#233723,#233724,#233725,#233726,
#233727,#233728,#233729),.UNSPECIFIED.,.F.,.F.,(4,2,2,2,2,2,2,2,2,2,2,2,
2,2,2,2,2,2,2,2,2,2,2,2,2,2,2,2,2,2,2,2,2,2,2,2,2,2,2,2,2,2,2,2,2,2,2,2,
2,2,2,2,2,2,2,2,2,2,2,2,2,2,2,2,2,2,2,2,2,2,2,2,2,2,2,2,2,2,2,2,2,2,2,2,
2,2,2,2,2,2,2,2,2,2,2,2,2,2,2,2,2,2,2,2,2,2,2,2,2,2,2,2,2,2,2,2,2,2,2,2,
2,2,2,2,2,2,2,2,2,2,2,2,2,2,2,2,2,2,2,2,2,2,2,2,2,2,2,2,2,2,2,2,2,2,2,2,
2,2,2,2,2,2,2,2,2,2,2,2,2,2,2,2,2,2,2,2,2,2,2,2,2,2,2,2,2,2,2,2,2,2,2,2,
2,2,2,2,2,2,2,2,2,2,2,2,2,2,2,2,2,2,2,2,2,2,2,2,2,2,2,2,2,2,2,2,2,2,2,2,
2,2,2,2,2,2,2,2,2,2,2,2,2,2,2,2,2,2,2,2,2,2,2,2,2,2,2,2,2,2,2,2,2,2,2,2,
4),(0.00198884727365615,0.0171463707040567,0.0256750116657391,0.0285743152075191,
0.0305866372870217,0.0322993945240548,0.0340195300615396,0.0362724063238345,
0.0397113804947701,0.0547865144684803,0.0645103343802238,0.339946689773468,
0.438496089949156,0.445648012664128,0.448767624582792,0.451057800839298,
0.453167975412984,0.456023790731331,0.463015146236112,0.534410202560947,
0.663414367777973,0.781945904415294,0.816553468401073,0.843738551184968,
0.853013901187956,0.85737159961459,0.859872133056049,0.861592841285253,
0.863249291791709,0.864758552761795,0.866733820356451,0.870789238402392,
0.89632099829748,0.999804598008103,1.07998952121405,1.21001057913817,1.22185351716905,
1.22708650650142,1.23096366351171,1.23456663790031,1.23949692087691,1.24926504030501,
1.32028598747467,1.36023160900097,1.48807763203879,1.60040933539202,1.60692629772314,
1.60952169020636,1.61131058988051,1.61309256735427,1.61559167289823,1.62141855944166,
1.69726813511767,1.80495645909475,1.81444926508167,1.82472222017144,1.83592778297765,
1.86583974181973,1.94738375994934,1.98016180636644,1.99842068553729,2.00263008699332,
2.00502771032156,2.00688439860489,2.00930426391325,2.01349991396267,2.02961421801231,
2.2751727379974,2.37781057022431,2.41991444269915,2.42439616841689,2.42773598930991,
2.42924167604163,2.43037581271755,2.43142478027466,2.43285578139489,2.43572132969231,
2.46062740154547,2.4872096705856,2.50739463983733,2.69427950051916,2.81104590060132,
2.82645764099631,2.83032669765709,2.83258813120023,2.83456946622926,2.83701993548203,
2.84075936335307,2.85708823751138,3.11896859020952,3.22101295715412,3.224122329879,
3.22663225561638,3.22800275638513,3.22905757435155,3.23021203204805,3.23225973071354,
3.23830593948605,3.26140641444881,3.50785970597717,3.63168381495137,3.64273248754689,
3.64635703997747,3.64868926688715,3.65088009198266,3.65375262778956,3.66009670594612,
3.7111551285214,3.90697201860214,4.04084444490444,4.0465966752032,4.04927525244862,
4.05131321204736,4.05324474820864,4.05648195626984,4.0649647837136,4.06738218615224,
4.08362869955827,4.27695943649482,4.4767814234358,4.49374047659829,4.50162583718784,
4.50766270131223,4.51342676625764,4.52324848705835,4.5503816094235,4.72584019635343,
4.80151275330677,4.80854801537686,4.81219114061619,4.81521704842281,4.81876577335425,
4.82493202384562,4.84942811029881,4.98058111098711,5.10032363114756,5.11532613117836,
5.12464987561789,5.13192191358108,5.13999675390767,5.15343804759686,5.2093274977759,
5.29726575778849,5.50169861115414,5.51417552653281,5.55316339279786,5.56592534514112,
5.56946716002764,5.57156148416652,5.57337924684139,5.57560598448812,5.57984974886658,
5.6058721421834,5.63549664847498,5.69924491139167,5.75326929445897,5.83321316984002,
5.97387554835989,5.98333153742395,5.98693941643972,5.9890891201945,5.99135574236815,
5.99433029162459,6.0006971050468,6.08447378271113,6.19173283708081,6.35057534276617,
6.35276396250618,6.39487236110566,6.39928948434063,6.40131295177347,6.40286612313846,
6.40452909361055,6.40713335771399,6.41522597832415,6.53779729423936,6.66650677623621,
6.75076037147215,6.76137828678529,6.76632962933164,6.77017575196176,6.77394659486115,
6.7801561052831,6.78738276233063,6.80064288660128,6.90528395347411,7.11882343087342,
7.14275321813219,7.14667747078748,7.14900735035899,7.15078628566553,7.15268218683037,
7.15563325837464,7.16466650933385,7.21202251169895,7.26047709391965,7.38658358420473,
7.52995863424854,7.53920387679239,7.54261147842525,7.54460844175146,7.54648169127216,
7.54906533578278,7.55414311384868,7.58973821287799,7.68074153179939,7.78113081675769,
7.93081272570395,7.96301871081334,7.96614438211233,7.96765291296083,7.96872372892792,
7.96973357871389,7.97113614977494,7.973985159641,7.99860481526616,8.07535028583002,
8.21109717850274,8.35600223288823,8.36595202447255,8.36937830018627,8.37132423484702,
8.37311126671674,8.37551797012166,8.38005280963434,8.40542663700932,8.44020910999858,
8.5124599738622,8.57647449677435,8.73229627854706,8.76081629940044,8.76417665051739,
8.76571616156273,8.76690033082439,8.76817048983073,8.77016390757077,8.77638447316304,
8.81210312745829,8.84027971198559,8.92017256287157,8.99311816982852,9.16843772328873,
9.179908002401,9.18372764738194,9.18586543128531,9.18780977047556,9.19040065179808,
9.1951942912154,9.22051898846983,9.27020543496659,9.31009548091169,9.33439906163638,
9.35107034385852,9.40167657937295,9.56852906458665,9.5813534354853,9.58518418670587,
9.58746115849259,9.58927774551977,9.59171256628152,9.59626289846381,9.62157075763454,
9.67863810718868,9.78800941450442,9.95698214585812),.UNSPECIFIED.);
#3587=B_SPLINE_CURVE_WITH_KNOTS('',3,(#233731,#233732,#233733,#233734,#233735,
#233736,#233737,#233738,#233739,#233740,#233741,#233742,#233743,#233744,
#233745,#233746,#233747,#233748,#233749,#233750,#233751,#233752,#233753,
#233754,#233755,#233756,#233757,#233758,#233759,#233760,#233761,#233762,
#233763,#233764,#233765,#233766,#233767,#233768,#233769,#233770,#233771,
#233772,#233773,#233774,#233775,#233776,#233777,#233778,#233779,#233780,
#233781,#233782,#233783,#233784,#233785,#233786,#233787,#233788,#233789,
#233790,#233791,#233792,#233793,#233794,#233795,#233796,#233797,#233798,
#233799,#233800,#233801,#233802,#233803,#233804,#233805,#233806,#233807,
#233808,#233809,#233810,#233811,#233812,#233813,#233814,#233815,#233816,
#233817,#233818,#233819,#233820,#233821,#233822,#233823,#233824,#233825,
#233826,#233827,#233828,#233829,#233830,#233831,#233832,#233833,#233834,
#233835,#233836,#233837,#233838,#233839,#233840,#233841,#233842,#233843,
#233844,#233845,#233846,#233847,#233848,#233849,#233850,#233851,#233852,
#233853,#233854,#233855,#233856,#233857,#233858,#233859,#233860,#233861,
#233862,#233863,#233864,#233865,#233866,#233867,#233868,#233869,#233870,
#233871,#233872,#233873,#233874,#233875,#233876,#233877,#233878,#233879,
#233880,#233881,#233882,#233883,#233884,#233885,#233886,#233887,#233888,
#233889,#233890,#233891,#233892,#233893,#233894,#233895,#233896,#233897,
#233898,#233899,#233900,#233901,#233902,#233903,#233904,#233905,#233906,
#233907,#233908,#233909,#233910,#233911,#233912,#233913,#233914,#233915,
#233916,#233917,#233918,#233919,#233920,#233921,#233922,#233923,#233924,
#233925,#233926,#233927,#233928,#233929,#233930,#233931,#233932,#233933,
#233934,#233935,#233936,#233937,#233938,#233939,#233940,#233941,#233942,
#233943,#233944,#233945,#233946,#233947,#233948,#233949,#233950,#233951,
#233952,#233953,#233954,#233955,#233956,#233957,#233958,#233959,#233960,
#233961,#233962,#233963,#233964,#233965,#233966,#233967,#233968,#233969,
#233970,#233971,#233972,#233973,#233974,#233975,#233976,#233977,#233978,
#233979,#233980,#233981,#233982,#233983,#233984,#233985,#233986,#233987,
#233988,#233989,#233990,#233991,#233992,#233993,#233994,#233995,#233996,
#233997,#233998,#233999,#234000,#234001,#234002,#234003,#234004,#234005,
#234006,#234007,#234008,#234009,#234010,#234011,#234012,#234013,#234014,
#234015,#234016,#234017,#234018,#234019,#234020,#234021,#234022,#234023,
#234024,#234025,#234026,#234027,#234028,#234029,#234030,#234031,#234032,
#234033,#234034,#234035,#234036,#234037,#234038,#234039,#234040,#234041,
#234042,#234043,#234044,#234045,#234046,#234047,#234048,#234049,#234050,
#234051,#234052,#234053,#234054,#234055,#234056,#234057,#234058,#234059,
#234060,#234061,#234062,#234063,#234064,#234065,#234066,#234067,#234068,
#234069,#234070,#234071,#234072,#234073,#234074,#234075,#234076,#234077,
#234078,#234079,#234080,#234081,#234082,#234083,#234084,#234085,#234086,
#234087,#234088,#234089,#234090,#234091,#234092,#234093,#234094,#234095,
#234096,#234097,#234098,#234099,#234100,#234101,#234102,#234103,#234104,
#234105,#234106,#234107,#234108,#234109,#234110,#234111,#234112,#234113,
#234114,#234115,#234116,#234117,#234118,#234119,#234120,#234121,#234122,
#234123,#234124,#234125,#234126,#234127,#234128,#234129,#234130,#234131,
#234132,#234133,#234134,#234135,#234136,#234137,#234138,#234139,#234140,
#234141,#234142,#234143,#234144,#234145,#234146,#234147,#234148,#234149,
#234150,#234151,#234152,#234153,#234154,#234155,#234156,#234157,#234158,
#234159,#234160,#234161,#234162,#234163,#234164,#234165,#234166,#234167,
#234168,#234169,#234170,#234171,#234172,#234173,#234174,#234175,#234176,
#234177,#234178,#234179,#234180,#234181,#234182,#234183,#234184,#234185,
#234186,#234187,#234188,#234189,#234190,#234191,#234192,#234193,#234194,
#234195,#234196,#234197,#234198,#234199,#234200,#234201,#234202,#234203,
#234204,#234205,#234206,#234207,#234208,#234209,#234210,#234211,#234212,
#234213,#234214,#234215,#234216,#234217,#234218,#234219,#234220,#234221,
#234222,#234223,#234224,#234225,#234226,#234227,#234228,#234229,#234230,
#234231,#234232,#234233,#234234,#234235,#234236,#234237,#234238,#234239,
#234240,#234241,#234242,#234243,#234244,#234245,#234246,#234247,#234248,
#234249,#234250,#234251,#234252,#234253,#234254,#234255,#234256,#234257,
#234258,#234259,#234260,#234261,#234262,#234263,#234264,#234265,#234266,
#234267,#234268,#234269,#234270),.UNSPECIFIED.,.F.,.F.,(4,2,2,2,2,2,2,2,
2,2,2,2,2,2,2,2,2,2,2,2,2,2,2,2,2,2,2,2,2,2,2,2,2,2,2,2,2,2,2,2,2,2,2,2,
2,2,2,2,2,2,2,2,2,2,2,2,2,2,2,2,2,2,2,2,2,2,2,2,2,2,2,2,2,2,2,2,2,2,2,2,
2,2,2,2,2,2,2,2,2,2,2,2,2,2,2,2,2,2,2,2,2,2,2,2,2,2,2,2,2,2,2,2,2,2,2,2,
2,2,2,2,2,2,2,2,2,2,2,2,2,2,2,2,2,2,2,2,2,2,2,2,2,2,2,2,2,2,2,2,2,2,2,2,
2,2,2,2,2,2,2,2,2,2,2,2,2,2,2,2,2,2,2,2,2,2,2,2,2,2,2,2,2,2,2,2,2,2,2,2,
2,2,2,2,2,2,2,2,2,2,2,2,2,2,2,2,2,2,2,2,2,2,2,2,2,2,2,2,2,2,2,2,2,2,2,2,
2,2,2,2,2,2,2,2,2,2,2,2,2,2,2,2,2,2,2,2,2,2,2,2,2,2,2,2,2,2,2,2,2,2,2,2,
2,2,2,2,2,2,2,2,2,4),(0.00205360525305213,0.0593773831792553,0.0709500426668551,
0.078387278285601,0.0842101463919144,0.0900833689727588,0.0967768172356078,
0.107906200022069,0.145521832312656,0.183512161887853,0.331647921885141,
0.380309783067713,0.386610574941088,0.390475557176331,0.393449185361408,
0.396513321521263,0.399420247524142,0.404301921621275,0.417240578218173,
0.537201828279952,0.635946020232279,0.670160334207074,0.686942760904269,
0.697107784863918,0.70639267951786,0.713552708210863,0.720528995699381,
0.730433139607536,0.758236895515654,0.966234212694743,1.01196019163004,
1.07540724372314,1.12473622823872,1.14713744478909,1.15122571308088,1.15341944632182,
1.15521863703423,1.15705682449771,1.16045990331156,1.17156797294044,1.32805796697757,
1.40356860481657,1.4937897370052,1.55412833393993,1.56532848468822,1.56905961121908,
1.57147559582088,1.57375605124961,1.57676208927215,1.58346749925563,1.63989676132955,
1.76949086823613,1.87701698099182,1.97723449858227,1.98163453464158,1.9836772509676,
1.98522828585988,1.98669558037854,1.98874187253823,1.99407399428787,2.09022757991063,
2.31426091890442,2.33083116572251,2.33926705995999,2.34447590037582,2.34904311461777,
2.35281533125918,2.35646991147333,2.3615953388166,2.37211816715402,2.46745545288722,
2.5284496864162,2.6460567307181,2.70100867185602,2.72565193418798,2.72974133771406,
2.73188788440267,2.73364041348433,2.73539782756739,2.73860491692891,2.74870976159622,
2.76637992867256,2.784918640935,2.82649458631348,2.85496790901447,2.98881103843157,
3.08335170830491,3.11857882984537,3.12364332606152,3.12622421688244,3.12809703732692,
3.13009503490561,3.13350821274674,3.14278858630628,3.27745952538948,3.43163516002308,
3.54546352338192,3.54896410693957,3.55050330045609,3.55163770428469,3.55268580471725,
3.55411384607153,3.5569680805554,3.5815431018535,3.60872192624215,3.77629372366884,
3.94407473016478,3.95016500657277,3.95287931387753,3.9548946862876,3.95676781534534,
3.9593275971224,3.96571887143421,4.03693816836897,4.17164512195338,4.27806269168589,
4.32522137383842,4.34434074334756,4.34709905676227,4.34853695790378,4.34970606435603,
4.35087475178229,4.35299452002735,4.35958585464541,4.46691401580334,4.65500045602485,
4.72757700092795,4.7601521669558,4.76528444894179,4.76794721403573,4.77010533766783,
4.77225691637946,4.77614527253955,4.78813940258596,4.97925228940441,5.15242881733038,
5.164390961761,5.1681183727177,5.1701461628033,5.17214017817843,5.17458482360079,
5.17918130914651,5.20544650410065,5.26579687621784,5.44815445466409,5.56141184189628,
5.60540178023497,5.61701461854046,5.62381041672618,5.62920234273582,5.63640900534867,
5.64991971182084,5.7376414434567,5.85141717861117,5.92048737470507,5.92791808783788,
5.93163108123368,5.93465938434876,5.93814835399665,5.94421169093895,5.97019259428511,
6.2022969742365,6.23056432947623,6.24170856281142,6.24853279283878,6.25591319113084,
6.26598870398649,6.28987618720666,6.51211520319966,6.65871075563774,6.68407446407058,
6.68816276990672,6.6905837778307,6.69242926316786,6.69439338345106,6.69744550481796,
6.70675527511992,6.75558513419176,6.78733789871383,7.08599480269894,7.10202595954001,
7.10643092943572,7.1090219341054,7.11126164476541,7.11399337028287,7.11916214303216,
7.14925243638016,7.19748962008518,7.35580622802623,7.50835243907473,7.51771672213975,
7.52052779970833,7.52222904553766,7.52373140904439,7.52484952617282,7.52751956766254,
7.53617325522243,7.59008738779717,7.65238041551183,7.77511719782402,7.87042876030836,
7.88132075575424,7.88632264737826,7.89017554013963,7.89431993812796,7.90086509899404,
7.92089791876676,8.02672945398436,8.0744434782342,8.23913441652531,8.26258080509861,
8.26682324146756,8.26900355767995,8.27072786402079,8.27236472539724,8.27522732987946,
8.28357721238536,8.32536162479298,8.34057933791867,8.39991510481678,8.57260632285271,
8.6530124525068,8.6597895352244,8.66247818182678,8.66443660328259,8.6665352689038,
8.66934713098162,8.67559609546932,8.81153970653139,8.83747737210576,8.85839597324602,
8.87589268648235,8.89084831779175,8.90381590562649,8.91517429517758,8.92520088161523,
9.0109191707375,9.02032151786773,9.08151202355462,9.08553477902998,9.08704417909839,
9.08811492807227,9.08912416099025,9.09019815694449,9.09249645058799,9.10329677071956,
9.12382449830058,9.18563346055924,9.41119241550355,9.41965029178766,9.48058705346492,
9.48672574858062,9.48924076892925,9.49110177736394,9.49312402626457,9.49588299084781,
9.50222599674433,9.61700966967578,9.81664443196399,9.82402160762228,9.87924801352412,
9.88314845096017,9.88467527486454,9.88578497181194,9.88690754280314,9.88806219203879,
9.88956622787327,9.89193273604794,9.9010358693165,9.95458350454511),
 .UNSPECIFIED.);
#3588=B_SPLINE_CURVE_WITH_KNOTS('',3,(#234272,#234273,#234274,#234275,#234276,
#234277,#234278,#234279,#234280,#234281,#234282,#234283,#234284,#234285,
#234286,#234287,#234288,#234289,#234290,#234291,#234292,#234293,#234294,
#234295,#234296,#234297,#234298,#234299,#234300,#234301,#234302,#234303,
#234304,#234305,#234306,#234307,#234308,#234309,#234310,#234311,#234312,
#234313,#234314,#234315,#234316,#234317,#234318,#234319,#234320,#234321,
#234322,#234323,#234324,#234325,#234326,#234327,#234328,#234329,#234330,
#234331,#234332,#234333,#234334,#234335,#234336,#234337,#234338,#234339,
#234340,#234341,#234342,#234343,#234344,#234345,#234346,#234347,#234348,
#234349,#234350,#234351,#234352,#234353,#234354,#234355,#234356,#234357,
#234358,#234359,#234360,#234361,#234362,#234363,#234364,#234365,#234366,
#234367,#234368,#234369,#234370,#234371,#234372,#234373,#234374,#234375,
#234376,#234377,#234378,#234379,#234380,#234381,#234382,#234383,#234384,
#234385,#234386,#234387,#234388,#234389,#234390,#234391,#234392,#234393,
#234394,#234395,#234396,#234397,#234398,#234399,#234400,#234401,#234402,
#234403,#234404,#234405,#234406,#234407,#234408,#234409,#234410,#234411,
#234412,#234413,#234414,#234415,#234416,#234417,#234418,#234419,#234420,
#234421,#234422,#234423,#234424,#234425,#234426,#234427,#234428,#234429,
#234430,#234431,#234432,#234433,#234434,#234435,#234436,#234437,#234438,
#234439,#234440,#234441,#234442,#234443,#234444,#234445,#234446,#234447,
#234448,#234449,#234450,#234451,#234452,#234453,#234454,#234455,#234456,
#234457,#234458,#234459,#234460,#234461,#234462,#234463,#234464,#234465,
#234466,#234467,#234468,#234469,#234470,#234471,#234472,#234473,#234474,
#234475,#234476,#234477,#234478,#234479,#234480,#234481,#234482,#234483,
#234484,#234485,#234486,#234487,#234488,#234489,#234490,#234491,#234492,
#234493,#234494,#234495,#234496,#234497,#234498,#234499,#234500,#234501,
#234502,#234503,#234504,#234505,#234506,#234507,#234508,#234509,#234510,
#234511,#234512,#234513,#234514,#234515,#234516,#234517,#234518,#234519,
#234520,#234521,#234522,#234523,#234524,#234525,#234526,#234527,#234528,
#234529,#234530,#234531,#234532,#234533,#234534,#234535,#234536,#234537,
#234538,#234539,#234540,#234541,#234542,#234543,#234544,#234545,#234546,
#234547,#234548,#234549,#234550,#234551,#234552,#234553,#234554,#234555,
#234556,#234557,#234558,#234559,#234560,#234561,#234562,#234563,#234564,
#234565,#234566,#234567,#234568,#234569,#234570,#234571,#234572,#234573,
#234574,#234575,#234576,#234577,#234578,#234579,#234580,#234581,#234582,
#234583,#234584,#234585,#234586,#234587,#234588,#234589,#234590,#234591,
#234592,#234593,#234594,#234595,#234596,#234597,#234598,#234599,#234600,
#234601,#234602,#234603,#234604,#234605,#234606,#234607,#234608,#234609,
#234610,#234611,#234612,#234613,#234614,#234615,#234616,#234617,#234618,
#234619,#234620,#234621,#234622,#234623,#234624,#234625,#234626,#234627,
#234628,#234629,#234630,#234631,#234632,#234633,#234634,#234635,#234636,
#234637,#234638,#234639,#234640,#234641,#234642,#234643,#234644,#234645,
#234646,#234647,#234648,#234649,#234650,#234651,#234652,#234653,#234654,
#234655,#234656,#234657,#234658,#234659,#234660,#234661,#234662,#234663,
#234664,#234665,#234666,#234667,#234668,#234669,#234670,#234671,#234672,
#234673,#234674,#234675,#234676,#234677,#234678,#234679,#234680,#234681,
#234682,#234683,#234684,#234685,#234686,#234687,#234688,#234689,#234690,
#234691,#234692,#234693,#234694,#234695,#234696,#234697,#234698,#234699,
#234700,#234701,#234702,#234703,#234704,#234705,#234706,#234707,#234708,
#234709,#234710,#234711,#234712,#234713,#234714,#234715,#234716,#234717,
#234718,#234719,#234720,#234721,#234722,#234723,#234724,#234725,#234726,
#234727,#234728,#234729,#234730,#234731,#234732,#234733,#234734,#234735,
#234736,#234737,#234738,#234739,#234740,#234741,#234742,#234743,#234744,
#234745,#234746,#234747,#234748,#234749,#234750,#234751,#234752,#234753,
#234754,#234755,#234756,#234757,#234758,#234759,#234760,#234761,#234762,
#234763,#234764,#234765,#234766,#234767,#234768,#234769,#234770,#234771,
#234772,#234773,#234774,#234775,#234776,#234777,#234778,#234779,#234780,
#234781,#234782,#234783,#234784,#234785,#234786,#234787,#234788,#234789,
#234790,#234791,#234792,#234793,#234794,#234795,#234796,#234797,#234798,
#234799,#234800,#234801,#234802,#234803,#234804,#234805,#234806,#234807,
#234808,#234809,#234810,#234811,#234812,#234813,#234814,#234815,#234816,
#234817,#234818,#234819,#234820,#234821,#234822,#234823,#234824,#234825,
#234826,#234827,#234828,#234829,#234830,#234831,#234832,#234833,#234834,
#234835,#234836,#234837,#234838,#234839,#234840,#234841,#234842,#234843,
#234844,#234845,#234846,#234847,#234848,#234849,#234850,#234851,#234852,
#234853,#234854,#234855,#234856,#234857,#234858,#234859,#234860,#234861,
#234862,#234863,#234864,#234865,#234866,#234867,#234868,#234869,#234870,
#234871,#234872,#234873,#234874,#234875,#234876,#234877),.UNSPECIFIED.,
 .F.,.F.,(4,2,2,2,2,2,2,2,2,2,2,2,2,2,2,2,2,2,2,2,2,2,2,2,2,2,2,2,2,2,2,
2,2,2,2,2,2,2,2,2,2,2,2,2,2,2,2,2,2,2,2,2,2,2,2,2,2,2,2,2,2,2,2,2,2,2,2,
2,2,2,2,2,2,2,2,2,2,2,2,2,2,2,2,2,2,2,2,2,2,2,2,2,2,2,2,2,2,2,2,2,2,2,2,
2,2,2,2,2,2,2,2,2,2,2,2,2,2,2,2,2,2,2,2,2,2,2,2,2,2,2,2,2,2,2,2,2,2,2,2,
2,2,2,2,2,2,2,2,2,2,2,2,2,2,2,2,2,2,2,2,2,2,2,2,2,2,2,2,2,2,2,2,2,2,2,2,
2,2,2,2,2,2,2,2,2,2,2,2,2,2,2,2,2,2,2,2,2,2,2,2,2,2,2,2,2,2,2,2,2,2,2,2,
2,2,2,2,2,2,2,2,2,2,2,2,2,2,2,2,2,2,2,2,2,2,2,2,2,2,2,2,2,2,2,2,2,2,2,2,
2,2,2,2,2,2,2,2,2,2,2,2,2,2,2,2,2,2,2,2,2,2,2,2,2,2,2,2,2,2,2,2,2,2,2,2,
2,2,2,2,2,2,2,2,2,2,2,2,2,2,2,2,2,2,2,4),(0.00298799696991318,0.284548765783284,
0.324998927055044,0.346725222155488,0.351305191664363,0.353849462103799,
0.355790169769175,0.358278477046583,0.362493946379329,0.377687442785345,
0.66059392337514,0.692141903033456,0.74376107945835,0.751799365416695,0.754868007480455,
0.756748203307425,0.75875736883098,0.761424396136439,0.767062140285104,
0.813045040613457,0.851696620085529,0.966681559443179,1.18248503247399,
1.19970929428457,1.20764425203756,1.21368870322025,1.21943727358696,1.22753303494866,
1.24933838462884,1.39644278402009,1.49756032582151,1.50718066805563,1.51447769270129,
1.51816799080709,1.52119605835027,1.52461057865531,1.528486301843,1.54176519756824,
1.64990297845833,1.76907429410024,1.81353878448344,1.82626300613302,1.83418715327372,
1.84150036838553,1.85097416731601,1.87191821243426,1.91125857047846,2.00269496746611,
2.15544490963139,2.21564526546191,2.26959544567536,2.27454803620845,2.27691910327582,
2.27871753272058,2.28066213035479,2.28368242512681,2.29237227960743,2.41431295984751,
2.52924991619505,2.64228407850674,2.68569748934479,2.69135654976542,2.69419162031758,
2.69622968291942,2.69838618730555,2.70141668921914,2.70767060469526,2.77212923676101,
3.00228363882309,3.10122818216294,3.10573712412653,3.10780052101499,3.10932669216269,
3.11094032735715,3.11337516754345,3.11995516740608,3.12909479836546,3.13647279354061,
3.32450255266738,3.45563082949889,3.46750153588689,3.47274025719392,3.47661910396445,
3.48022182328744,3.48514892266501,3.49738398487739,3.65955108685084,3.78189312907216,
3.82847781518075,3.85011695632573,3.85406506303475,3.85618166033255,3.85791637276539,
3.85995415785783,3.8634461258874,3.87641739633784,4.11471652493715,4.17295090954306,
4.21998032789621,4.24401684337691,4.24859622282434,4.25107487411233,4.25311851524632,
4.25553322655929,4.25970597316534,4.27558213461076,4.56266753812426,4.62094811823215,
4.66614181437333,4.67321956954466,4.67524610460064,4.67648363998103,4.67760182436175,
4.67903262957894,4.68202531574454,4.70216719251704,4.87116396568071,4.98214133931871,
5.06837894972334,5.07509185703591,5.07770673777867,5.07959479344217,5.08160253718232,
5.08426594247148,5.09007785230583,5.18458896375922,5.36353426498577,5.46450593290116,
5.47120978641427,5.47331677306128,5.47448291547406,5.47565289450548,5.47709636506131,
5.47987739632411,5.49738898961177,5.53660580707938,5.60359509018789,5.68135984876374,
5.72282644617998,5.77733392846139,5.78255071137604,5.79752027473821,5.8826017497064,
5.88972222839802,5.89253898445213,5.89458793407069,5.89678101119802,5.89971480069819,
5.90621649758936,6.04659169101303,6.1880630934402,6.22382424185533,6.28644160115385,
6.29236817336843,6.29505089337251,6.29709753693096,6.29927708753388,6.30266713472379,
6.31304151492471,6.44373525924046,6.66293617186134,6.72930784022965,6.74195126360323,
6.74896039003915,6.75474814701651,6.76168794798178,6.77393682564694,6.83220505472201,
6.963394911328,7.0086240185794,7.04809320969585,7.05412042887509,7.0579068482803,
7.06094252491028,7.06438300306789,7.07010359180137,7.09075113572629,7.12870279050102,
7.25112988858497,7.29508607544355,7.30174672313976,7.35156376228543,7.36504335588487,
7.37309971220848,7.3801985505715,7.38913573684223,7.40668576792219,7.50750554505508,
7.64480123736787,7.76762089597334,7.77480722676958,7.80973069737468,7.81471279126246,
7.81706468222407,7.81890038753219,7.82089693743581,7.82409069312295,7.83458325074647,
7.89411208133,8.0649478922328,8.21990728815591,8.2297296047366,8.23339632818336,
8.23555827492464,8.23759491135854,8.24041759155522,8.24601435703751,8.28654843353863,
8.38716979905904,8.45819940578936,8.63253257031194,8.6438349884074,8.64687495326056,
8.64865401811518,8.65017146464981,8.65202655136355,8.65549716417568,8.67472986534528,
8.71597425739663,8.74999292881849,8.77587831713415,8.83529161266237,8.99640837878672,
9.00768371203758,9.01284299678956,9.01666126575537,9.01685702865119,9.01688451776892,
9.01691093381246,9.01693631941594,9.01696071608408,9.01698416361527,9.01700670017908,
9.01702836231571,9.01704918504256,9.01706920194387,9.01708844520265,9.01710229598491,
9.01711601142003,9.01712959720982,9.01714305477671,9.0171563855366,9.01716959082916,
9.01718267195316,9.01719563028769,9.01720846710627,9.0172211837034,9.01723378135626,
9.01724626132437,9.0172586248577,9.01727087321867,9.01728300759856,9.01729502927146,
9.01730693938076,9.01731873917141,9.01733042971497,9.01734201220508,9.0173534878348,
9.01736485761211,9.01737612271136,9.01738728428401,9.01739834328824,9.01740930083484,
9.01742015799366,9.01743091585589,9.01744157542675,9.01745213774419,9.01746260383416,
9.01747297469172,9.01748325129263,9.01749343469561,9.01750352578474,9.01751352550644,
9.01752343481792,9.01753325468627,9.02173162943359,9.02879505359289,9.05298730611816,
9.22099259945438,9.31932129227878,9.3622738721429,9.38969638335723,9.39418775108313,
9.39644971286767,9.3982146578637,9.40016301155353,9.40334330437531,9.4143720901834,
9.48073396554205,9.55247242503873,9.58468629245607,9.60168085315791,9.6213175865944,
9.77629978667344,9.78656475456521,9.79012509040459,9.79215399775925,9.79402142642433,
9.79654271237396,9.79922118703221,9.80344490315052,9.83479378676887,9.96256522287139),
 .UNSPECIFIED.);
#3589=B_SPLINE_CURVE_WITH_KNOTS('',3,(#234879,#234880,#234881,#234882,#234883,
#234884,#234885,#234886,#234887,#234888,#234889,#234890,#234891,#234892,
#234893,#234894,#234895,#234896,#234897,#234898,#234899,#234900,#234901,
#234902,#234903,#234904,#234905,#234906,#234907,#234908,#234909,#234910,
#234911,#234912,#234913,#234914,#234915,#234916,#234917,#234918,#234919,
#234920,#234921,#234922,#234923,#234924,#234925,#234926,#234927,#234928,
#234929,#234930,#234931,#234932,#234933,#234934,#234935,#234936,#234937,
#234938,#234939,#234940,#234941,#234942,#234943,#234944,#234945,#234946,
#234947,#234948,#234949,#234950,#234951,#234952,#234953,#234954,#234955,
#234956,#234957,#234958,#234959,#234960,#234961,#234962,#234963,#234964,
#234965,#234966,#234967,#234968,#234969,#234970,#234971,#234972,#234973,
#234974,#234975,#234976,#234977,#234978,#234979,#234980,#234981,#234982,
#234983,#234984,#234985,#234986,#234987,#234988,#234989,#234990,#234991,
#234992,#234993,#234994,#234995,#234996,#234997,#234998,#234999,#235000,
#235001,#235002,#235003,#235004,#235005,#235006,#235007,#235008,#235009,
#235010,#235011,#235012,#235013,#235014,#235015,#235016,#235017,#235018,
#235019,#235020,#235021,#235022,#235023,#235024,#235025,#235026,#235027,
#235028,#235029,#235030,#235031,#235032,#235033,#235034,#235035,#235036,
#235037,#235038,#235039,#235040,#235041,#235042,#235043,#235044,#235045,
#235046,#235047,#235048,#235049,#235050,#235051,#235052,#235053,#235054,
#235055,#235056,#235057,#235058,#235059,#235060,#235061,#235062,#235063,
#235064,#235065,#235066,#235067,#235068,#235069,#235070,#235071,#235072,
#235073,#235074,#235075,#235076,#235077,#235078,#235079,#235080,#235081,
#235082,#235083,#235084,#235085,#235086,#235087,#235088,#235089,#235090,
#235091,#235092,#235093,#235094,#235095,#235096,#235097,#235098,#235099,
#235100,#235101,#235102,#235103,#235104,#235105,#235106,#235107,#235108,
#235109,#235110,#235111,#235112,#235113,#235114,#235115,#235116,#235117,
#235118,#235119,#235120,#235121,#235122,#235123,#235124,#235125,#235126,
#235127,#235128,#235129,#235130,#235131,#235132,#235133,#235134),
 .UNSPECIFIED.,.F.,.F.,(4,3,3,3,3,3,3,3,3,3,3,3,3,3,3,3,3,3,3,3,3,3,3,3,
3,3,3,3,3,3,3,3,3,3,3,3,3,3,3,3,3,3,3,3,3,3,3,3,3,3,3,3,3,3,3,3,3,3,3,3,
3,3,3,3,3,3,3,3,3,3,3,3,3,3,3,3,3,3,3,3,3,3,3,3,3,4),(-267.986713186487,
-267.895065432478,-267.802448421134,-267.708773505748,-267.662249211065,
-267.589110267381,-267.516059350074,-267.443081526052,-267.370161931536,
-267.29728575656,-267.224438230978,-267.151590733819,-267.078739585281,
-267.00587143618,-266.932972926128,-266.859987484565,-266.786954671789,
-266.713810247672,-266.663509475203,-266.587981186536,-266.512538991203,
-266.437169983508,-266.361861305545,-266.286600139145,-266.208871339169,
-266.133661141844,-266.058456917146,-265.983247106881,-265.908020151895,
-265.832737262285,-265.757421215414,-265.682034306157,-265.664769739341,
-265.588177838941,-265.511651137,-265.435179941109,-265.358763080849,-265.282379042015,
-265.206018878603,-265.16539987141,-265.087280602929,-265.009116299454,
-264.930902222464,-264.852597099774,-264.774243673173,-264.695804583406,
-264.666030003478,-264.584051224892,-264.502144475652,-264.418273390626,
-264.336607978112,-264.251634056829,-264.166660135547,-264.093048461441,
-264.019442094588,-263.945828042687,-263.872161750158,-263.798468222134,
-263.724692749069,-263.667290267616,-263.59078954281,-263.514344775629,
-263.437945056048,-263.361579506442,-263.285237274251,-263.208151431439,
-263.131809618062,-263.05545753042,-262.979085306312,-262.901451612672,
-262.824979935679,-262.746765233717,-262.668550531754,-262.593868717066,
-262.519266864914,-262.444732581341,-262.370264023807,-262.295833808213,
-262.221428896414,-262.169180663823,-262.090168152782,-262.011043352256,
-261.931733613374,-261.852330853427,-261.772764020692,-261.703528014493),
 .UNSPECIFIED.);
#3590=B_SPLINE_CURVE_WITH_KNOTS('',3,(#235136,#235137,#235138,#235139,#235140,
#235141,#235142,#235143,#235144,#235145,#235146,#235147,#235148,#235149),
 .UNSPECIFIED.,.F.,.F.,(4,2,1,1,1,1,1,1,1,1,4),(-261.703527798163,-261.669810795892,
-260.67107106003,-259.672331324168,-258.673591588305,-258.174221720374,
-257.674851852443,-257.175481984512,-256.676112116581,-255.677372380719,
-255.420342707314),.UNSPECIFIED.);
#3591=B_SPLINE_CURVE_WITH_KNOTS('',3,(#235151,#235152,#235153,#235154,#235155,
#235156,#235157,#235158,#235159,#235160,#235161,#235162,#235163,#235164,
#235165,#235166,#235167,#235168),.UNSPECIFIED.,.F.,.F.,(4,2,2,2,2,2,2,2,
4),(-255.420342707314,-254.585425795419,-253.750508883524,-252.915591971629,
-252.080675059734,-251.245758147839,-250.410841235945,-249.57592432405,
-249.137157400134),.UNSPECIFIED.);
#3592=B_SPLINE_CURVE_WITH_KNOTS('',3,(#235170,#235171,#235172,#235173,#235174,
#235175,#235176,#235177,#235178,#235179,#235180,#235181,#235182,#235183,
#235184,#235185,#235186,#235187),.UNSPECIFIED.,.F.,.F.,(4,2,2,2,2,2,2,2,
4),(-249.137157400134,-248.302240488239,-247.467323576345,-246.63240666445,
-245.797489752555,-244.96257284066,-244.127655928765,-243.29273901687,-242.853972092955),
 .UNSPECIFIED.);
#3593=B_SPLINE_CURVE_WITH_KNOTS('',3,(#235189,#235190,#235191,#235192,#235193,
#235194,#235195,#235196,#235197,#235198,#235199,#235200,#235201,#235202,
#235203,#235204,#235205,#235206),.UNSPECIFIED.,.F.,.F.,(4,2,2,2,2,2,2,2,
4),(-242.853972092955,-242.01905518106,-241.184138269165,-240.34922135727,
-239.514304445375,-238.67938753348,-237.844470621585,-237.009553709691,
-236.570786785775),.UNSPECIFIED.);
#3594=B_SPLINE_CURVE_WITH_KNOTS('',3,(#235208,#235209,#235210,#235211,#235212,
#235213,#235214,#235215,#235216,#235217,#235218,#235219,#235220,#235221,
#235222,#235223,#235224,#235225),.UNSPECIFIED.,.F.,.F.,(4,2,2,2,2,2,2,2,
4),(-236.570786785775,-235.73586987388,-234.900952961985,-234.066036050091,
-233.231119138196,-232.396202226301,-231.561285314406,-230.726368402511,
-230.287602016329),.UNSPECIFIED.);
#3595=B_SPLINE_CURVE_WITH_KNOTS('',3,(#235227,#235228,#235229,#235230,#235231,
#235232,#235233,#235234,#235235,#235236,#235237,#235238,#235239,#235240,
#235241,#235242,#235243,#235244,#235245,#235246,#235247,#235248,#235249,
#235250,#235251,#235252,#235253,#235254,#235255,#235256,#235257,#235258,
#235259,#235260,#235261,#235262,#235263,#235264,#235265,#235266,#235267,
#235268,#235269,#235270,#235271,#235272,#235273,#235274,#235275,#235276,
#235277,#235278,#235279,#235280,#235281,#235282,#235283,#235284,#235285,
#235286,#235287,#235288,#235289,#235290,#235291,#235292,#235293,#235294,
#235295,#235296,#235297,#235298,#235299,#235300,#235301,#235302,#235303,
#235304,#235305,#235306,#235307,#235308,#235309,#235310,#235311,#235312,
#235313,#235314,#235315,#235316,#235317,#235318,#235319,#235320,#235321,
#235322,#235323,#235324,#235325,#235326,#235327,#235328,#235329,#235330,
#235331,#235332,#235333,#235334,#235335,#235336,#235337,#235338,#235339,
#235340,#235341,#235342,#235343,#235344,#235345,#235346,#235347,#235348,
#235349,#235350,#235351,#235352,#235353,#235354,#235355,#235356,#235357,
#235358,#235359,#235360,#235361,#235362,#235363,#235364,#235365,#235366,
#235367,#235368,#235369,#235370,#235371,#235372,#235373,#235374,#235375,
#235376,#235377,#235378,#235379,#235380,#235381,#235382,#235383,#235384,
#235385,#235386,#235387,#235388,#235389,#235390,#235391,#235392,#235393,
#235394,#235395,#235396,#235397,#235398,#235399,#235400,#235401,#235402,
#235403,#235404,#235405,#235406,#235407,#235408,#235409,#235410,#235411,
#235412,#235413,#235414,#235415,#235416,#235417,#235418,#235419,#235420,
#235421,#235422,#235423,#235424,#235425,#235426,#235427,#235428,#235429,
#235430,#235431,#235432,#235433,#235434,#235435,#235436,#235437,#235438,
#235439,#235440,#235441,#235442,#235443,#235444,#235445,#235446,#235447,
#235448,#235449,#235450,#235451,#235452,#235453,#235454,#235455,#235456,
#235457,#235458,#235459,#235460,#235461,#235462,#235463,#235464,#235465,
#235466,#235467,#235468,#235469,#235470,#235471,#235472,#235473,#235474,
#235475,#235476,#235477,#235478,#235479,#235480,#235481,#235482,#235483,
#235484,#235485,#235486,#235487,#235488,#235489,#235490,#235491,#235492,
#235493,#235494,#235495,#235496,#235497,#235498,#235499,#235500,#235501,
#235502,#235503,#235504,#235505,#235506,#235507,#235508,#235509,#235510,
#235511,#235512,#235513,#235514,#235515,#235516,#235517,#235518,#235519,
#235520,#235521,#235522,#235523,#235524,#235525,#235526,#235527,#235528,
#235529,#235530,#235531,#235532,#235533,#235534,#235535,#235536,#235537,
#235538,#235539,#235540,#235541,#235542,#235543,#235544,#235545,#235546,
#235547,#235548,#235549,#235550,#235551,#235552,#235553,#235554,#235555,
#235556,#235557,#235558,#235559,#235560,#235561,#235562,#235563,#235564,
#235565,#235566,#235567,#235568,#235569,#235570,#235571,#235572,#235573,
#235574,#235575,#235576,#235577,#235578,#235579,#235580,#235581,#235582,
#235583,#235584,#235585,#235586,#235587,#235588,#235589,#235590,#235591,
#235592,#235593,#235594,#235595,#235596,#235597,#235598,#235599,#235600,
#235601,#235602,#235603,#235604,#235605,#235606,#235607,#235608,#235609,
#235610,#235611,#235612,#235613,#235614,#235615,#235616,#235617,#235618,
#235619,#235620,#235621,#235622,#235623,#235624,#235625,#235626,#235627,
#235628,#235629,#235630,#235631,#235632,#235633,#235634,#235635,#235636,
#235637,#235638,#235639,#235640,#235641,#235642,#235643,#235644,#235645,
#235646,#235647,#235648,#235649,#235650,#235651,#235652,#235653,#235654,
#235655,#235656,#235657,#235658,#235659,#235660,#235661,#235662,#235663,
#235664,#235665,#235666,#235667,#235668,#235669,#235670,#235671,#235672,
#235673,#235674,#235675,#235676,#235677,#235678,#235679,#235680,#235681,
#235682,#235683,#235684,#235685,#235686,#235687,#235688,#235689,#235690,
#235691,#235692,#235693,#235694,#235695,#235696,#235697,#235698,#235699,
#235700,#235701,#235702,#235703,#235704,#235705,#235706,#235707,#235708,
#235709,#235710,#235711,#235712,#235713,#235714,#235715,#235716,#235717,
#235718,#235719,#235720,#235721,#235722,#235723,#235724,#235725,#235726,
#235727,#235728,#235729,#235730,#235731,#235732,#235733,#235734,#235735,
#235736,#235737,#235738,#235739,#235740,#235741,#235742,#235743,#235744,
#235745,#235746,#235747,#235748,#235749,#235750,#235751,#235752,#235753,
#235754),.UNSPECIFIED.,.F.,.F.,(4,2,2,2,2,2,2,2,2,2,2,2,2,2,2,2,2,2,2,2,
2,2,2,2,2,2,2,2,2,2,2,2,2,2,2,2,2,2,2,2,2,2,2,2,2,2,2,2,2,2,2,2,2,2,2,2,
2,2,2,2,2,2,2,2,2,2,2,2,2,2,2,2,2,2,2,2,2,2,2,2,2,2,2,2,2,2,2,2,2,2,2,2,
2,2,2,2,2,2,2,2,2,2,2,2,2,2,2,2,2,2,2,2,2,2,2,2,2,2,2,2,2,2,2,2,2,2,2,2,
2,2,2,2,2,2,2,2,2,2,2,2,2,2,2,2,2,2,2,2,2,2,2,2,2,2,2,2,2,2,2,2,2,2,2,2,
2,2,2,2,2,2,2,2,2,2,2,2,2,2,2,2,2,2,2,2,2,2,2,2,2,2,2,2,2,2,2,2,2,2,2,2,
2,2,2,2,2,2,2,2,2,2,2,2,2,2,2,2,2,2,2,2,2,2,2,2,2,2,2,2,2,2,2,2,2,2,2,2,
2,2,2,2,2,2,2,2,2,2,2,2,2,2,2,2,2,2,2,2,2,2,2,2,2,2,2,4),(0.00169204175923553,
0.128820729549866,0.140683025697351,0.148239355435246,0.154099751533378,
0.159924582078469,0.165707733094985,0.175623411871471,0.203402886356974,
0.263964772043401,0.302904995997001,0.40067121699731,0.448936386886242,
0.458962870963235,0.462230108879606,0.46505189696762,0.468101290201929,
0.4720210615819,0.480135792335445,0.547890937157175,0.584005929628486,0.678993742421287,
0.729124166352655,0.751100998364294,0.768396438538095,0.777259485312679,
0.784349980201744,0.792546544477399,0.806545531812426,0.862443329299604,
1.05576876431122,1.12858114708919,1.18912499742063,1.21670182157923,1.22104091711757,
1.22328782371271,1.22510716381907,1.22691905878811,1.23019139750927,1.24025612684883,
1.38650270824074,1.48438440875138,1.59010145705835,1.63193953570891,1.63755223969695,
1.64037795327922,1.64241478874154,1.64457509822983,1.647619307508,1.65392866794775,
1.72056071707936,1.72798325846529,1.83832078293851,1.91810726604842,1.9938072517963,
2.00811599113056,2.03504711049864,2.04911690525961,2.05233998483585,2.05414124676916,
2.0555204334066,2.05706506452728,2.05990392965606,2.06903323549553,2.2694105348947,
2.38950596251023,2.40329786963805,2.4138757783152,2.41885878175748,2.42249017097881,
2.42609434920214,2.43102647218762,2.44079878655823,2.51187178886177,2.55180317775188,
2.68459742272682,2.76524027888333,2.79529881490304,2.79961307049101,2.80180679976827,
2.80339658996465,2.805090871918,2.80749110791666,2.81396474196005,2.89957851414183,
3.02964073147012,3.12935166732212,3.16144850191309,3.18924472845449,3.19401451073827,
3.19653421577097,3.19840018891676,3.20042725333625,3.20398378810365,3.21423167167558,
3.36141446846769,3.51863597739258,3.57398848603187,3.61202332116103,3.61838305501683,
3.62033162805872,3.62155169738221,3.62267442709653,3.62411604503934,3.6272487747198,
3.65080155909433,3.75795219330761,3.91884444431871,4.01486876972315,4.02069258082322,
4.02335823456778,4.02536634283641,4.027253780909,4.02986628694234,4.03656467908008,
4.12247782165953,4.3118803869199,4.39221401883121,4.41487996418079,4.41774571437491,
4.41920619622363,4.42026667955683,4.42139854218053,4.42333276780259,4.42859603003401,
4.51319801795877,4.69466099315154,4.79137056726509,4.83066288951878,4.83603576457255,
4.8387492661589,4.84070860666857,4.84278985202896,4.84572781629199,4.85358660094087,
4.97971560591509,5.22203897867044,5.23532474586461,5.23920967770097,5.24149947805944,
5.2434986370988,5.24600236257967,5.25087576676225,5.28389372599522,5.37147028218351,
5.44957751348197,5.59368552850528,5.67368575373751,5.68572240553988,5.69332205030121,
5.69932544446027,5.70605532303809,5.71734813236724,5.76178475147623,5.84356915572153,
5.98565499882068,5.99744099848249,6.0014733544957,6.00436836048662,6.00743696770192,
6.01149238485903,6.02031287945392,6.10682909705381,6.27746254598682,6.3030915218253,
6.31273421121391,6.31964289014398,6.32697732741801,6.33675018470292,6.35880962872048,
6.54833670380946,6.74727039439894,6.74998377749953,6.75857061786715,6.76157403299604,
6.76351437709716,6.76526586662232,6.76762039591887,6.77248700424533,6.82837164971718,
6.86031354783463,7.15807473009532,7.17413169191457,7.1785411150683,7.18113416937885,
7.18337530307501,7.18610832659734,7.1912782385094,7.22134050042427,7.26688401961591,
7.38764540583095,7.49218527626971,7.54778505620299,7.58744352305227,7.59171346905189,
7.59352115934466,7.59507465946784,7.59652145567753,7.59872843975061,7.60404536907063,
7.61142088518676,7.69569447150197,7.85616488913764,7.94322063727004,7.95391394755627,
7.95887997287957,7.96272876548692,7.96689214700736,7.97351737711832,7.99414433217313,
8.10515945361295,8.29427107004716,8.33066535288816,8.33810378391215,8.34087396869458,
8.3424528111761,8.34416494034495,8.34636985810621,8.35073968853788,8.38373367652693,
8.41328961371291,8.47258339069487,8.6430064111253,8.72588262336472,8.73271165494646,
8.73540978983135,8.73737122634909,8.73946946073971,8.74227442225615,8.74848222362601,
8.87346131447097,8.90295973531925,8.92832892186743,8.94926142702981,8.96706624758196,
8.98250506767304,8.99607309430263,9.04305659958386,9.12973743231144,9.1557935455754,
9.15906608125554,9.16054714558957,9.16167610861934,9.16271540183624,9.16389057355239,
9.16719897728497,9.1716457970705,9.18253256765766,9.21969436889805,9.27912567786901,
9.54063424822291,9.55730314222564,9.56107039710376,9.56352925890164,9.5655107761421,
9.56776523854358,9.57160472181438,9.5866803364728,9.69681320649013,9.92869023299713,
9.93814457512901,9.95463105348814,9.95744203340321,9.958588076165),
 .UNSPECIFIED.);
#3596=B_SPLINE_CURVE_WITH_KNOTS('',3,(#235756,#235757,#235758,#235759,#235760,
#235761,#235762,#235763,#235764,#235765,#235766,#235767,#235768),
 .UNSPECIFIED.,.F.,.F.,(4,1,1,1,1,1,1,1,1,1,4),(-217.721230864236,-216.726522682094,
-216.227152814163,-215.727782946231,-215.2284130783,-214.729043210369,-213.730303474507,
-213.230933606576,-212.731563738645,-211.732824002783,-211.438045557057),
 .UNSPECIFIED.);
#3597=B_SPLINE_CURVE_WITH_KNOTS('',3,(#235770,#235771,#235772,#235773,#235774,
#235775,#235776,#235777,#235778,#235779,#235780,#235781,#235782,#235783,
#235784,#235785,#235786,#235787),.UNSPECIFIED.,.F.,.F.,(4,2,2,2,2,2,2,2,
4),(-211.438045557057,-210.603128645162,-209.768211733267,-208.933294821372,
-208.098377909477,-207.263460997582,-206.428544085688,-205.593627173793,
-205.154860249877),.UNSPECIFIED.);
#3598=B_SPLINE_CURVE_WITH_KNOTS('',3,(#235789,#235790,#235791,#235792,#235793,
#235794,#235795,#235796,#235797,#235798,#235799,#235800,#235801),
 .UNSPECIFIED.,.F.,.F.,(4,1,1,1,1,1,1,1,1,1,4),(-205.154860249877,-204.741645851748,
-204.242275983816,-203.742906115885,-202.744166380023,-202.244796512092,
-201.745426644161,-201.24605677623,-200.746686908299,-199.747947172437,
-198.872317216215),.UNSPECIFIED.);
#3599=B_SPLINE_CURVE_WITH_KNOTS('',3,(#235803,#235804,#235805,#235806,#235807,
#235808,#235809,#235810,#235811,#235812,#235813,#235814,#235815,#235816,
#235817,#235818,#235819,#235820,#235821,#235822,#235823,#235824,#235825,
#235826,#235827,#235828,#235829,#235830,#235831,#235832,#235833,#235834,
#235835,#235836,#235837,#235838,#235839,#235840,#235841,#235842,#235843,
#235844,#235845,#235846,#235847,#235848,#235849,#235850,#235851,#235852,
#235853,#235854,#235855,#235856,#235857,#235858,#235859,#235860,#235861,
#235862,#235863,#235864,#235865,#235866,#235867,#235868,#235869,#235870,
#235871,#235872,#235873,#235874,#235875,#235876,#235877,#235878,#235879,
#235880,#235881,#235882,#235883,#235884,#235885,#235886,#235887,#235888,
#235889,#235890,#235891,#235892,#235893,#235894,#235895,#235896,#235897,
#235898,#235899,#235900,#235901,#235902,#235903,#235904,#235905,#235906,
#235907,#235908,#235909,#235910,#235911,#235912,#235913,#235914,#235915,
#235916,#235917,#235918,#235919,#235920,#235921,#235922,#235923,#235924,
#235925,#235926,#235927,#235928,#235929,#235930,#235931,#235932,#235933,
#235934,#235935,#235936,#235937,#235938,#235939,#235940,#235941,#235942,
#235943,#235944,#235945,#235946,#235947,#235948,#235949,#235950,#235951,
#235952,#235953,#235954,#235955,#235956,#235957,#235958,#235959,#235960,
#235961,#235962,#235963,#235964,#235965,#235966,#235967,#235968,#235969,
#235970,#235971,#235972,#235973,#235974,#235975,#235976,#235977,#235978,
#235979,#235980,#235981,#235982,#235983,#235984,#235985,#235986,#235987,
#235988,#235989,#235990,#235991,#235992,#235993,#235994,#235995,#235996,
#235997,#235998,#235999,#236000,#236001,#236002,#236003,#236004,#236005,
#236006,#236007,#236008,#236009,#236010,#236011,#236012,#236013,#236014,
#236015,#236016,#236017,#236018,#236019,#236020,#236021,#236022,#236023,
#236024,#236025,#236026,#236027,#236028,#236029,#236030,#236031,#236032,
#236033,#236034,#236035,#236036,#236037,#236038,#236039,#236040,#236041,
#236042,#236043,#236044,#236045,#236046,#236047,#236048,#236049,#236050,
#236051,#236052,#236053,#236054,#236055,#236056,#236057,#236058,#236059,
#236060,#236061,#236062,#236063,#236064,#236065,#236066,#236067,#236068,
#236069,#236070,#236071,#236072,#236073,#236074,#236075,#236076,#236077,
#236078,#236079,#236080,#236081,#236082,#236083,#236084,#236085,#236086,
#236087,#236088,#236089,#236090,#236091,#236092,#236093,#236094,#236095,
#236096,#236097,#236098,#236099,#236100,#236101,#236102,#236103,#236104,
#236105,#236106,#236107,#236108,#236109,#236110,#236111,#236112,#236113,
#236114,#236115,#236116,#236117,#236118,#236119,#236120,#236121,#236122,
#236123,#236124,#236125,#236126,#236127,#236128,#236129,#236130,#236131,
#236132,#236133,#236134,#236135,#236136,#236137,#236138,#236139,#236140,
#236141,#236142,#236143,#236144,#236145,#236146,#236147,#236148,#236149,
#236150,#236151,#236152,#236153,#236154,#236155,#236156,#236157,#236158,
#236159,#236160,#236161,#236162,#236163,#236164,#236165,#236166,#236167,
#236168,#236169,#236170,#236171,#236172,#236173,#236174,#236175,#236176,
#236177,#236178,#236179,#236180,#236181,#236182,#236183,#236184,#236185,
#236186,#236187,#236188,#236189,#236190,#236191,#236192,#236193,#236194,
#236195,#236196,#236197,#236198,#236199,#236200,#236201,#236202,#236203,
#236204,#236205,#236206,#236207,#236208,#236209,#236210,#236211,#236212,
#236213,#236214,#236215,#236216,#236217,#236218,#236219,#236220,#236221,
#236222,#236223,#236224,#236225,#236226,#236227,#236228,#236229,#236230,
#236231,#236232,#236233,#236234,#236235,#236236,#236237,#236238,#236239,
#236240,#236241,#236242,#236243,#236244,#236245,#236246,#236247,#236248,
#236249,#236250,#236251,#236252,#236253,#236254,#236255,#236256,#236257,
#236258,#236259,#236260,#236261,#236262,#236263,#236264,#236265,#236266,
#236267,#236268,#236269,#236270,#236271,#236272,#236273,#236274,#236275,
#236276,#236277,#236278,#236279,#236280,#236281,#236282,#236283,#236284,
#236285,#236286,#236287,#236288,#236289,#236290,#236291,#236292,#236293,
#236294,#236295,#236296,#236297,#236298,#236299,#236300,#236301,#236302,
#236303,#236304,#236305,#236306,#236307,#236308,#236309,#236310,#236311,
#236312,#236313,#236314),.UNSPECIFIED.,.F.,.F.,(4,2,2,2,2,2,2,2,2,2,2,2,
2,2,2,2,2,2,2,2,2,2,2,2,2,2,2,2,2,2,2,2,2,2,2,2,2,2,2,2,2,2,2,2,2,2,2,2,
2,2,2,2,2,2,2,2,2,2,2,2,2,2,2,2,2,2,2,2,2,2,2,2,2,2,2,2,2,2,2,2,2,2,2,2,
2,2,2,2,2,2,2,2,2,2,2,2,2,2,2,2,2,2,2,2,2,2,2,2,2,2,2,2,2,2,2,2,2,2,2,2,
2,2,2,2,2,2,2,2,2,2,2,2,2,2,2,2,2,2,2,2,2,2,2,2,2,2,2,2,2,2,2,2,2,2,2,2,
2,2,2,2,2,2,2,2,2,2,2,2,2,2,2,2,2,2,2,2,2,2,2,2,2,2,2,2,2,2,2,2,2,2,2,2,
2,2,2,2,2,2,2,2,2,2,2,2,2,2,2,2,2,2,2,2,2,2,2,2,2,2,2,2,2,2,2,2,2,2,2,2,
2,2,2,2,2,2,2,2,2,2,2,2,2,2,2,2,2,2,2,2,2,2,2,2,2,2,2,4),(0.00191394602328637,
0.0944684754693169,0.0968787543811911,0.0983665318117488,0.0994814529629017,
0.100615559975077,0.101664719732112,0.103090817090912,0.105887054240193,
0.12763755181692,0.173614383098775,0.17623185663861,0.193988745972456,0.201991997469711,
0.388809479155954,0.47888957738054,0.515488743238011,0.520600192581283,
0.523190882670798,0.525065193613106,0.527059499253994,0.530453206829348,
0.539607289044027,0.677360939269346,0.7531359649222,0.90944661516137,0.9151363597031,
0.917592281779398,0.919353568118223,0.921167383202567,0.923815197944702,
0.930498814302529,1.05802998502632,1.1640079236285,1.26878048960929,1.28869166797053,
1.29522135334016,1.29936283769931,1.30321780059319,1.30822916199294,1.31916900526404,
1.41650018840158,1.52664256844806,1.65582814407429,1.66257437105731,1.66500177368406,
1.66659914332189,1.66813226846972,1.67019231135599,1.67463451426253,1.72186110719343,
1.72725618031526,1.85890588313987,1.86822966012696,1.87826647274652,2.06808767085959,
2.07493643224757,2.07800103869861,2.08028159700849,2.08240491975219,2.08531250857926,
2.09260349276629,2.17717654891765,2.39425704232891,2.48671387608953,2.4929571512927,
2.49556329862019,2.49740115479434,2.49926630033228,2.50194414333719,2.50847537381707,
2.64116885546442,2.79842118967124,2.90781414322716,2.92603832800423,2.93510416525806,
2.94165874948799,2.94866558159823,2.96077233530204,2.99583534854256,3.04933207070088,
3.18906711428707,3.24256420034153,3.24988582910731,3.2536445606738,3.25638604252864,
3.25974654629061,3.26531076330751,3.28640744456579,3.50096403718671,3.54353952171919,
3.55467284200496,3.56136498471022,3.56737092888208,3.5750233776465,3.58724403358075,
3.67089698022099,3.67229479695662,3.69652306667407,3.73224316255104,3.90006502780105,
3.99828908783521,4.01150396856832,4.01520806888163,4.0174565765314,4.01948041085218,
4.02205670610179,4.02728895523267,4.05904036458754,4.31149141491449,4.40807605909275,
4.41497567782393,4.41797987270617,4.4201832066768,4.42221182842074,4.4249549063649,
4.43165841026875,4.49894569756243,4.73629255702961,4.79177956105173,4.82979520809024,
4.83625982116579,4.83828178316545,4.83955792139589,4.84073921720697,4.842263121934,
4.84554111627787,4.8717099444164,4.97796292638631,5.17124535684743,5.22414262022017,
5.22956778117636,5.23221889861133,5.23411550747943,5.23591615060921,5.23843400958516,
5.24350742287998,5.28456962391348,5.39337520753743,5.62013413645552,5.63289458858313,
5.63522372982776,5.63664390185122,5.63776289188969,5.63899187619111,5.64098328075268,
5.647738916276,5.6896753863514,5.74704872772061,5.79449560458504,5.98324166854546,
6.04997186947067,6.05646035763179,6.05909913621516,6.06104463750869,6.0631518844749,
6.06601465780526,6.07254389980024,6.19222131088364,6.43637942348593,6.44972212081554,
6.45324982083382,6.45529507648987,6.45686966735421,6.45891015731025,6.46251251544456,
6.47847045918395,6.70231210933929,6.74753686779607,6.81828248311108,6.82079214391801,
6.82447663327616,6.83123142445203,6.83560875042149,6.83941382748229,6.84408867267543,
6.85306472269427,6.91199682482521,6.98738355365248,7.17263047638213,7.19669960705479,
7.20063259858052,7.20260991379666,7.20415097122904,7.20585027845178,7.20861959596037,
7.21817817962904,7.28104625864239,7.39422308208374,7.53039313982771,7.60419540394855,
7.61124294065932,7.61410775528786,7.61621950505469,7.61835784101097,7.62131220791434,
7.62457555280662,7.63001528465736,7.74539429994104,7.87017344689481,8.01845555064868,
8.02791098626311,8.03109972669997,8.03289373647992,8.03469665518467,8.03696485644724,
8.04141233842279,8.07262492204533,8.15960006128387,8.21796695152772,8.28532783371875,
8.34142091704411,8.40023665798033,8.43938515023859,8.46039441767353,8.46987493623481,
8.47718428717912,8.48509528725677,8.49777872530006,8.54189264333745,8.66107099817978,
8.76937339949178,8.78263913865442,8.78756893471798,8.79048344157793,8.79354019513237,
8.79753191479276,8.80667652505242,8.81954730929483,8.83966168945805,8.94515289856989,
9.03216271589456,9.0774422303577,9.08917558159987,9.09606649866031,9.10204307168555,
9.10938782529794,9.12359396995231,9.23533418761744,9.34172038092684,9.48797904483556,
9.51998810048555,9.53574774787381,9.54678259175826,9.55038573202943,9.55238917562775,
9.55420350498837,9.55661002644198,9.56103172804729,9.58383993125126,9.62028933910265,
9.75430381301949,9.94182413716274,9.94912265785832,9.95188999567882,9.95197847831517),
 .UNSPECIFIED.);
#3600=B_SPLINE_CURVE_WITH_KNOTS('',3,(#236316,#236317,#236318,#236319,#236320,
#236321,#236322,#236323,#236324,#236325,#236326,#236327,#236328,#236329,
#236330,#236331,#236332,#236333,#236334,#236335,#236336,#236337,#236338,
#236339,#236340,#236341,#236342,#236343,#236344,#236345,#236346,#236347,
#236348,#236349,#236350,#236351,#236352,#236353,#236354,#236355,#236356,
#236357,#236358,#236359,#236360,#236361,#236362,#236363,#236364,#236365,
#236366,#236367,#236368,#236369,#236370,#236371,#236372,#236373,#236374,
#236375,#236376,#236377,#236378,#236379,#236380,#236381,#236382,#236383,
#236384,#236385,#236386,#236387,#236388,#236389,#236390,#236391,#236392,
#236393,#236394,#236395,#236396,#236397,#236398,#236399,#236400,#236401,
#236402,#236403,#236404,#236405,#236406,#236407,#236408,#236409,#236410,
#236411,#236412,#236413,#236414,#236415,#236416,#236417,#236418,#236419,
#236420,#236421,#236422,#236423,#236424,#236425,#236426,#236427,#236428,
#236429,#236430,#236431,#236432,#236433,#236434,#236435,#236436,#236437,
#236438,#236439,#236440,#236441,#236442,#236443,#236444,#236445,#236446,
#236447,#236448,#236449,#236450,#236451,#236452,#236453,#236454,#236455,
#236456,#236457,#236458,#236459,#236460,#236461,#236462,#236463,#236464,
#236465,#236466,#236467,#236468,#236469,#236470,#236471,#236472,#236473,
#236474,#236475,#236476,#236477,#236478,#236479,#236480,#236481,#236482,
#236483,#236484,#236485,#236486,#236487,#236488,#236489,#236490,#236491,
#236492,#236493,#236494,#236495,#236496,#236497,#236498,#236499,#236500,
#236501,#236502,#236503,#236504,#236505,#236506,#236507,#236508,#236509,
#236510,#236511,#236512,#236513,#236514,#236515,#236516,#236517,#236518,
#236519,#236520,#236521,#236522,#236523,#236524,#236525,#236526,#236527,
#236528,#236529,#236530,#236531,#236532,#236533,#236534,#236535,#236536,
#236537,#236538,#236539,#236540,#236541,#236542,#236543,#236544,#236545,
#236546,#236547,#236548,#236549,#236550,#236551,#236552,#236553,#236554,
#236555,#236556,#236557,#236558,#236559,#236560,#236561,#236562,#236563,
#236564,#236565,#236566,#236567,#236568,#236569,#236570,#236571,#236572,
#236573,#236574,#236575,#236576,#236577,#236578,#236579,#236580,#236581,
#236582,#236583,#236584,#236585,#236586,#236587,#236588,#236589,#236590,
#236591,#236592,#236593,#236594,#236595,#236596,#236597,#236598,#236599,
#236600,#236601,#236602,#236603,#236604,#236605,#236606,#236607,#236608,
#236609,#236610,#236611,#236612,#236613,#236614,#236615,#236616,#236617,
#236618,#236619,#236620,#236621,#236622,#236623,#236624,#236625,#236626,
#236627,#236628,#236629,#236630,#236631,#236632,#236633,#236634,#236635,
#236636,#236637,#236638,#236639,#236640,#236641,#236642,#236643,#236644,
#236645,#236646,#236647,#236648,#236649,#236650,#236651,#236652,#236653,
#236654,#236655,#236656,#236657,#236658,#236659,#236660,#236661,#236662,
#236663,#236664,#236665,#236666,#236667,#236668,#236669,#236670,#236671,
#236672,#236673,#236674,#236675,#236676,#236677,#236678,#236679,#236680,
#236681,#236682,#236683,#236684,#236685,#236686,#236687,#236688,#236689,
#236690,#236691,#236692,#236693,#236694,#236695,#236696,#236697,#236698,
#236699,#236700,#236701,#236702,#236703,#236704,#236705,#236706,#236707,
#236708,#236709,#236710,#236711,#236712,#236713,#236714,#236715,#236716,
#236717,#236718,#236719,#236720,#236721,#236722,#236723,#236724,#236725,
#236726,#236727,#236728,#236729,#236730,#236731,#236732,#236733,#236734,
#236735,#236736,#236737,#236738,#236739,#236740,#236741,#236742,#236743,
#236744,#236745,#236746,#236747,#236748,#236749,#236750,#236751,#236752,
#236753,#236754,#236755,#236756,#236757,#236758,#236759,#236760,#236761,
#236762,#236763,#236764,#236765,#236766,#236767,#236768,#236769,#236770,
#236771,#236772,#236773,#236774,#236775,#236776,#236777,#236778,#236779,
#236780,#236781,#236782,#236783,#236784,#236785,#236786,#236787,#236788,
#236789,#236790,#236791,#236792,#236793,#236794,#236795,#236796,#236797,
#236798,#236799,#236800,#236801,#236802,#236803,#236804,#236805,#236806,
#236807,#236808,#236809,#236810,#236811,#236812,#236813,#236814,#236815,
#236816,#236817,#236818,#236819,#236820,#236821,#236822,#236823,#236824,
#236825,#236826,#236827,#236828,#236829,#236830,#236831,#236832,#236833,
#236834,#236835,#236836,#236837,#236838,#236839,#236840,#236841,#236842,
#236843,#236844,#236845,#236846,#236847,#236848,#236849,#236850,#236851),
 .UNSPECIFIED.,.F.,.F.,(4,2,2,2,2,2,2,2,2,2,2,2,2,2,2,2,2,2,2,2,2,2,2,2,
2,2,2,2,2,2,2,2,2,2,2,2,2,2,2,2,2,2,2,2,2,2,2,2,2,2,2,2,2,2,2,2,2,2,2,2,
2,2,2,2,2,2,2,2,2,2,2,2,2,2,2,2,2,2,2,2,2,2,2,2,2,2,2,2,2,2,2,2,2,2,2,2,
2,2,2,2,2,2,2,2,2,2,2,2,2,2,2,2,2,2,2,2,2,2,2,2,2,2,2,2,2,2,2,2,2,2,2,2,
2,2,2,2,2,2,2,2,2,2,2,2,2,2,2,2,2,2,2,2,2,2,2,2,2,2,2,2,2,2,2,2,2,2,2,2,
2,2,2,2,2,2,2,2,2,2,2,2,2,2,2,2,2,2,2,2,2,2,2,2,2,2,2,2,2,2,2,2,2,2,2,2,
2,2,2,2,2,2,2,2,2,2,2,2,2,2,2,2,2,2,2,2,2,2,2,2,2,2,2,2,2,2,2,2,2,2,2,2,
2,2,2,2,2,2,2,2,2,2,2,2,2,2,2,2,2,2,2,2,2,2,2,2,2,2,2,4),(0.00339948482433297,
0.00455387327914176,0.00664996712160906,0.00873724952909339,0.0121709021781368,
0.0214685783812223,0.135307833821441,0.314182684490307,0.353627606970092,
0.419655465577952,0.42338951960139,0.425017653679891,0.426212325674946,
0.427312396922012,0.42879988447454,0.432460253131873,0.475177802971346,
0.714150741962386,0.809465072885502,0.816427375995736,0.819294158830642,
0.8211561069453,0.823158041344754,0.825927199254051,0.832221943478852,0.899169337230051,
0.953950646209046,1.0316465729292,1.06073320793195,1.12383170898784,1.18641361564054,
1.20839122098479,1.21420268843468,1.22055901103832,1.22248176157527,1.22369166755149,
1.22481705384346,1.22627654792165,1.22870111687558,1.24250521349936,1.49320134560417,
1.59815341710021,1.62519463167248,1.63558829475165,1.64067998302065,1.64372058023638,
1.64642918211452,1.64849292367045,1.65044114577943,1.65308949870639,1.65963092718299,
1.72928979630668,1.8748814370295,1.88449478561483,1.90851723324041,1.9368652742486,
1.98371305418456,2.02876788713024,2.03752331401305,2.04043890103097,2.04232663972898,
2.04410843317757,2.04645737595751,2.05044797667661,2.07570506531668,2.31290595027982,
2.39588274065368,2.4131551307623,2.41931173633497,2.42337112885412,2.42721933887109,
2.4323420122959,2.44346155433415,2.56457920699647,2.77132998387571,2.7850154786549,
2.788147280369,2.78992769532024,2.79130459612038,2.79309719544224,2.79619919424374,
2.80820442811209,3.00036542393493,3.10911235752052,3.18387398114573,3.19235306518527,
3.19683164100235,3.19969238903921,3.20235615643741,3.2045515636765,3.20713767022418,
3.2115212344762,3.22734602892659,3.48484718086632,3.54586704482024,3.60503996033402,
3.61549323086494,3.61868094259353,3.62067511073813,3.62250957416612,3.62486118362018,
3.62984762871348,3.66496249138946,3.81066625069469,3.93773126464987,4.03333530711437,
4.05043489394663,4.05927749241149,4.06580499482296,4.07394629437169,4.08767649875489,
4.13730063433213,4.14453138502757,4.33868139139739,4.36812197195588,4.3744218540239,
4.37796260732031,4.38098763802104,4.38463695972295,4.39148420262095,4.43794992964713,
4.47341912094612,4.57773625520793,4.63410204604303,4.65684022046811,4.67410962621323,
4.68205892720294,4.68810342082402,4.69384667174326,4.70192970705974,4.72383430911374,
4.98043653009428,5.07306595565444,5.13145371522956,5.13691219763676,5.13959223446717,
5.14151792584327,5.14355755994882,5.14625151499181,5.15208802552767,5.29876817117258,
5.52255160090704,5.53646301250632,5.54058638021093,5.54302940697211,5.54497419972363,
5.54757358691066,5.55240828907908,5.57850914157836,5.62919703557433,5.73237414372841,
5.77357598384598,5.81877303674438,5.93807333948164,5.95795685134136,5.96108610969121,
5.96260003528448,5.96377654538478,5.96507024593164,5.96716997594589,5.97460594262434,
6.12801696243354,6.19382477862986,6.34258553306811,6.35228112607749,6.35567063568027,
6.35760888796711,6.35939701072369,6.36181743138727,6.36641863258125,6.39373414244521,
6.44924464588058,6.60652997609976,6.74810102696531,6.75699148042267,6.75924234210572,
6.7605352809782,6.7616350542402,6.76297566634959,6.7654715243006,6.77894044147464,
6.80615055495681,6.85895994488177,6.98639084190845,7.09404343482521,7.17308281239266,
7.17986195381161,7.18255119101633,7.18450997547661,7.18660895510604,7.18942096964188,
7.19566923139514,7.33550696751887,7.48979875668508,7.53349611221558,7.57034088976368,
7.57549970457562,7.57765762229547,7.57945218726998,7.58128714669426,7.58390255074102,
7.59053882180874,7.71666253032761,7.87975650779436,7.94217139571655,7.95261903061846,
7.95754280623525,7.96138444121906,7.96556664780587,7.97214482226862,7.99355206650326,
8.02691021788937,8.09098127821539,8.21834836765874,8.31740099175191,8.32305608362912,
8.32515381340454,8.32663465380853,8.32802493142828,8.32994421681633,8.33364882798252,
8.3383076883155,8.34845993152279,8.37930991719329,8.43980061647463,8.50192482997755,
8.58010934834867,8.72405182152072,8.73367410871813,8.73730809197383,8.73946267492432,
8.74150022302738,8.74433665155944,8.75000598526771,8.79384511977416,8.91776982214926,
8.94710239846476,9.02559809895208,9.14452052881674,9.15205892038015,9.15496340560512,
9.15670153875358,9.15835648129549,9.16067888481514,9.16319386113808,9.17573134821778,
9.19747221331567,9.28844273291446,9.37170794198734,9.55559744081383,9.58153997804678,
9.59117084718496,9.59807315161972,9.60540858640614,9.61256505958894,9.62197872987209,
9.63695150711152,9.72650206571606,9.86572588617263,9.88743509752931,9.90541988793216,
9.910985433902,9.91402747613791,9.91702868902569,9.91991051144495,9.92348634666446,
9.92899640776304,9.95507935882116),.UNSPECIFIED.);
#3601=B_SPLINE_CURVE_WITH_KNOTS('',3,(#236853,#236854,#236855,#236856,#236857,
#236858,#236859,#236860,#236861,#236862,#236863,#236864),.UNSPECIFIED.,
 .F.,.F.,(4,1,1,1,1,1,1,1,1,4),(-173.738933713979,-173.281344172089,-172.781974304158,
-171.783234568295,-170.784494832433,-169.785755096571,-169.28638522864,
-168.787015360709,-167.788275624847,-167.4557484068),.UNSPECIFIED.);
#3602=B_SPLINE_CURVE_WITH_KNOTS('',3,(#236866,#236867,#236868,#236869,#236870,
#236871,#236872,#236873,#236874,#236875,#236876,#236877,#236878,#236879,
#236880,#236881,#236882,#236883),.UNSPECIFIED.,.F.,.F.,(4,2,2,2,2,2,2,2,
4),(-167.4557484068,-166.620831494905,-165.78591458301,-164.950997671115,
-164.11608075922,-163.281163847326,-162.446246935431,-161.611330023536,
-161.17256309962),.UNSPECIFIED.);
#3603=B_SPLINE_CURVE_WITH_KNOTS('',3,(#236885,#236886,#236887,#236888,#236889,
#236890,#236891,#236892,#236893,#236894,#236895,#236896,#236897,#236898,
#236899,#236900,#236901,#236902,#236903,#236904,#236905,#236906,#236907,
#236908,#236909,#236910,#236911,#236912,#236913,#236914,#236915,#236916,
#236917,#236918,#236919,#236920,#236921,#236922,#236923,#236924,#236925,
#236926,#236927,#236928,#236929,#236930,#236931,#236932,#236933,#236934,
#236935,#236936,#236937,#236938,#236939,#236940,#236941,#236942,#236943,
#236944,#236945,#236946,#236947,#236948,#236949,#236950,#236951,#236952,
#236953,#236954,#236955,#236956,#236957,#236958,#236959,#236960,#236961,
#236962,#236963,#236964,#236965,#236966,#236967,#236968,#236969,#236970,
#236971,#236972,#236973,#236974,#236975,#236976,#236977,#236978,#236979,
#236980,#236981,#236982,#236983,#236984,#236985,#236986,#236987,#236988,
#236989,#236990,#236991,#236992,#236993,#236994,#236995,#236996,#236997,
#236998,#236999,#237000,#237001,#237002,#237003,#237004,#237005,#237006,
#237007,#237008,#237009,#237010,#237011,#237012,#237013,#237014,#237015,
#237016,#237017,#237018,#237019,#237020,#237021,#237022,#237023,#237024,
#237025,#237026,#237027,#237028,#237029,#237030,#237031,#237032,#237033,
#237034,#237035,#237036,#237037,#237038,#237039,#237040,#237041,#237042,
#237043,#237044,#237045,#237046,#237047,#237048,#237049,#237050,#237051,
#237052,#237053,#237054,#237055,#237056,#237057,#237058,#237059,#237060,
#237061,#237062,#237063,#237064,#237065,#237066,#237067,#237068,#237069,
#237070,#237071,#237072,#237073,#237074,#237075,#237076,#237077,#237078,
#237079,#237080,#237081,#237082,#237083,#237084,#237085,#237086,#237087,
#237088,#237089,#237090,#237091,#237092,#237093,#237094,#237095,#237096,
#237097,#237098,#237099,#237100,#237101,#237102,#237103,#237104,#237105,
#237106,#237107,#237108,#237109,#237110,#237111,#237112,#237113,#237114,
#237115,#237116,#237117,#237118,#237119,#237120,#237121,#237122,#237123,
#237124,#237125,#237126,#237127,#237128,#237129,#237130,#237131,#237132,
#237133,#237134,#237135,#237136,#237137,#237138,#237139,#237140,#237141,
#237142,#237143,#237144,#237145,#237146),.UNSPECIFIED.,.F.,.F.,(4,3,3,3,
3,3,3,3,3,3,3,3,3,3,3,3,3,3,3,3,3,3,3,3,3,3,3,3,3,3,3,3,3,3,3,3,3,3,3,3,
3,3,3,3,3,3,3,3,3,3,3,3,3,3,3,3,3,3,3,3,3,3,3,3,3,3,3,3,3,3,3,3,3,3,3,3,
3,3,3,3,3,3,3,3,3,3,3,4),(-161.17256309962,-161.086963947609,-161.000905088157,
-160.91465001931,-160.828218360044,-160.797097473811,-160.723320382987,
-160.649605605553,-160.575940071267,-160.502309926181,-160.428701302376,
-160.355088484571,-160.29772760588,-160.216294074799,-160.134725079803,
-160.050633244339,-159.968790537844,-159.883574137897,-159.798357737949,
-159.719924794452,-159.641561610572,-159.563263345294,-159.485044079437,
-159.406874787932,-159.328763462845,-159.298987870018,-159.222625398935,
-159.146246072852,-159.069840307211,-158.99336563512,-158.916853587391,
-158.840259258165,-158.799618002087,-158.72424062315,-158.64892478975,-158.57365768014,
-158.498426505057,-158.423218499912,-158.345425970701,-158.270207794519,
-158.194972918941,-158.119709775396,-158.044406782052,-157.969014586096,
-157.893569686747,-157.818026325647,-157.800878266225,-157.727734457249,
-157.654679444135,-157.58169828974,-157.508776127093,-157.435898143796,
-157.363049567974,-157.290202166957,-157.217351820808,-157.14448518075,
-157.071588887325,-156.998606747341,-156.925577846609,-156.852438293037,
-156.802138530363,-156.727549911139,-156.653046940759,-156.578615682998,
-156.50424224912,-156.429912788706,-156.355613480951,-156.2813201198,-156.207026570731,
-156.132720340123,-156.058388929992,-155.983984887122,-155.909539234808,
-155.835002676717,-155.803398794501,-155.722404815116,-155.641527777048,
-155.557153064428,-155.476594670498,-155.396160128518,-155.315900710935,
-155.304028926569,-155.231802226745,-155.159571043702,-155.08729105622,
-155.014985614552,-154.942600493689,-154.889377792441),.UNSPECIFIED.);
#3604=B_SPLINE_CURVE_WITH_KNOTS('',3,(#237148,#237149,#237150,#237151,#237152,
#237153,#237154,#237155,#237156,#237157,#237158,#237159,#237160,#237161),
 .UNSPECIFIED.,.F.,.F.,(4,2,1,1,1,1,1,1,1,1,4),(-154.889377792441,-154.804659058638,
-153.805919322776,-153.306549454845,-152.807179586914,-152.307809718983,
-151.808439851052,-150.80970011519,-149.810960379327,-148.812220643465,
-148.606192485261),.UNSPECIFIED.);
#3605=B_SPLINE_CURVE_WITH_KNOTS('',3,(#237163,#237164,#237165,#237166,#237167,
#237168,#237169,#237170,#237171,#237172,#237173,#237174,#237175),
 .UNSPECIFIED.,.F.,.F.,(4,1,1,1,1,1,1,1,1,1,4),(-148.606192485261,-148.312850775534,
-147.813480907603,-146.814741171741,-146.31537130381,-145.816001435879,
-145.316631567948,-144.817261700017,-143.818521964154,-142.819782228292,
-142.323011474765),.UNSPECIFIED.);
#3606=B_SPLINE_CURVE_WITH_KNOTS('',3,(#237177,#237178,#237179,#237180,#237181,
#237182,#237183,#237184,#237185,#237186,#237187,#237188,#237189,#237190,
#237191,#237192,#237193,#237194,#237195,#237196,#237197,#237198,#237199,
#237200,#237201,#237202,#237203,#237204,#237205,#237206,#237207,#237208,
#237209,#237210,#237211,#237212,#237213,#237214,#237215,#237216,#237217,
#237218,#237219,#237220,#237221,#237222,#237223,#237224,#237225,#237226,
#237227,#237228,#237229,#237230,#237231,#237232,#237233,#237234,#237235,
#237236,#237237,#237238,#237239,#237240,#237241,#237242,#237243,#237244,
#237245,#237246,#237247,#237248,#237249,#237250,#237251,#237252,#237253,
#237254,#237255,#237256,#237257,#237258,#237259,#237260,#237261,#237262,
#237263,#237264,#237265,#237266,#237267,#237268,#237269,#237270,#237271,
#237272,#237273,#237274,#237275,#237276,#237277,#237278,#237279,#237280,
#237281,#237282,#237283,#237284,#237285,#237286,#237287,#237288,#237289,
#237290,#237291,#237292,#237293,#237294,#237295,#237296,#237297,#237298,
#237299,#237300,#237301,#237302,#237303,#237304,#237305,#237306,#237307,
#237308,#237309,#237310,#237311,#237312,#237313,#237314,#237315,#237316,
#237317,#237318,#237319,#237320,#237321,#237322,#237323,#237324,#237325,
#237326,#237327,#237328,#237329,#237330,#237331,#237332,#237333,#237334,
#237335,#237336,#237337,#237338,#237339,#237340,#237341,#237342,#237343,
#237344,#237345,#237346,#237347,#237348,#237349,#237350,#237351,#237352,
#237353,#237354,#237355,#237356,#237357,#237358,#237359,#237360,#237361,
#237362,#237363,#237364,#237365,#237366,#237367,#237368,#237369,#237370,
#237371,#237372,#237373,#237374,#237375,#237376,#237377,#237378,#237379,
#237380,#237381,#237382,#237383,#237384,#237385,#237386,#237387,#237388,
#237389,#237390,#237391,#237392,#237393,#237394,#237395,#237396,#237397,
#237398,#237399,#237400,#237401,#237402,#237403,#237404,#237405,#237406,
#237407,#237408,#237409,#237410,#237411,#237412,#237413,#237414,#237415,
#237416,#237417,#237418,#237419,#237420,#237421,#237422,#237423,#237424,
#237425,#237426,#237427,#237428,#237429,#237430,#237431,#237432,#237433,
#237434,#237435,#237436,#237437,#237438,#237439,#237440,#237441,#237442,
#237443,#237444,#237445,#237446,#237447,#237448,#237449,#237450,#237451,
#237452,#237453,#237454,#237455,#237456,#237457,#237458,#237459,#237460,
#237461,#237462,#237463,#237464,#237465,#237466,#237467,#237468,#237469,
#237470,#237471,#237472,#237473,#237474,#237475,#237476,#237477,#237478,
#237479,#237480,#237481,#237482,#237483,#237484,#237485,#237486,#237487,
#237488,#237489,#237490,#237491,#237492,#237493,#237494,#237495,#237496,
#237497,#237498,#237499,#237500,#237501,#237502,#237503,#237504,#237505,
#237506,#237507,#237508,#237509,#237510,#237511,#237512,#237513,#237514,
#237515,#237516,#237517,#237518,#237519,#237520,#237521,#237522,#237523,
#237524,#237525,#237526,#237527,#237528,#237529,#237530,#237531,#237532,
#237533,#237534,#237535,#237536,#237537,#237538,#237539,#237540,#237541,
#237542,#237543,#237544,#237545,#237546,#237547,#237548,#237549,#237550,
#237551,#237552,#237553,#237554,#237555,#237556,#237557,#237558,#237559,
#237560,#237561,#237562,#237563,#237564,#237565,#237566,#237567,#237568,
#237569,#237570,#237571,#237572,#237573,#237574,#237575,#237576,#237577,
#237578,#237579,#237580,#237581,#237582,#237583,#237584,#237585,#237586,
#237587,#237588,#237589,#237590,#237591,#237592,#237593,#237594,#237595,
#237596,#237597,#237598,#237599,#237600,#237601,#237602,#237603,#237604,
#237605,#237606,#237607,#237608,#237609,#237610,#237611,#237612,#237613,
#237614,#237615,#237616,#237617,#237618,#237619,#237620,#237621,#237622,
#237623,#237624,#237625,#237626,#237627,#237628,#237629,#237630,#237631,
#237632,#237633,#237634,#237635,#237636,#237637,#237638,#237639,#237640,
#237641,#237642,#237643,#237644,#237645,#237646,#237647,#237648,#237649,
#237650,#237651,#237652,#237653,#237654,#237655,#237656,#237657,#237658,
#237659,#237660,#237661,#237662,#237663,#237664,#237665,#237666,#237667,
#237668,#237669,#237670,#237671,#237672,#237673,#237674,#237675,#237676,
#237677,#237678,#237679,#237680,#237681,#237682,#237683,#237684,#237685,
#237686,#237687,#237688,#237689,#237690,#237691,#237692,#237693,#237694,
#237695,#237696,#237697,#237698,#237699,#237700,#237701,#237702,#237703,
#237704),.UNSPECIFIED.,.F.,.F.,(4,2,2,2,2,2,2,2,2,2,2,2,2,2,2,2,2,2,2,2,
2,2,2,2,2,2,2,2,2,2,2,2,2,2,2,2,2,2,2,2,2,2,2,2,2,2,2,2,2,2,2,2,2,2,2,2,
2,2,2,2,2,2,2,2,2,2,2,2,2,2,2,2,2,2,2,2,2,2,2,2,2,2,2,2,2,2,2,2,2,2,2,2,
2,2,2,2,2,2,2,2,2,2,2,2,2,2,2,2,2,2,2,2,2,2,2,2,2,2,2,2,2,2,2,2,2,2,2,2,
2,2,2,2,2,2,2,2,2,2,2,2,2,2,2,2,2,2,2,2,2,2,2,2,2,2,2,2,2,2,2,2,2,2,2,2,
2,2,2,2,2,2,2,2,2,2,2,2,2,2,2,2,2,2,2,2,2,2,2,2,2,2,2,2,2,2,2,2,2,2,2,2,
2,2,2,2,2,2,2,2,2,2,2,2,2,2,2,2,2,2,2,2,2,2,2,2,2,2,2,2,2,2,2,2,2,2,2,2,
2,2,2,2,2,2,2,2,2,2,2,2,2,2,2,2,2,2,2,2,2,2,2,2,2,2,2,4),(0.0021989709022817,
0.0174738004725367,0.0266728755051898,0.0299382247501041,0.0322134910204027,
0.0341521217674839,0.0360942225102894,0.0386454182923098,0.0425298197095983,
0.0593724824131793,0.0713825199188557,0.347097866130202,0.368030873495306,
0.415799838349878,0.4248840106627,0.427842081983253,0.429739993881052,0.431519050973966,
0.433846547561474,0.437761180144164,0.461486819034567,0.664991788550958,
0.778735926505257,0.799669477603781,0.806335194698198,0.810508145377708,
0.81435498729063,0.819232439769835,0.828320947708939,0.885068479635379,
1.0805050027113,1.13853363449481,1.17135912758122,1.17531027967798,1.17726509952547,
1.17866054829179,1.18012818425219,1.18217562692914,1.18751470151173,1.27391376687694,
1.48849605253348,1.54189020753851,1.56832628035386,1.57873831866527,1.58394503756975,
1.58711228818103,1.58999789805207,1.59221915989653,1.59437129957261,1.59798919177949,
1.60750353409201,1.76031121766192,1.80896726801298,1.82385355094814,1.84502469574128,
1.868941032755,1.94823196004474,1.97737628860025,2.00160931358989,2.0057809029104,
2.00799278732535,2.00963505208825,2.01142336245892,2.0145720214624,2.02374636291436,
2.06763821673483,2.16449978428803,2.31389660910018,2.42013999978783,2.43812779283363,
2.44715128100224,2.45370419203812,2.46073650583,2.47295762087248,2.50882860657318,
2.62186693306429,2.73434336006735,2.75731589412689,2.76314506974697,2.76658354771801,
2.76930668750305,2.77295163022944,2.7797670796623,2.82513029934676,2.97263428312689,
3.02492738605399,3.05759168321795,3.06776254529853,3.07424598824688,3.0803185391646,
3.08829070033247,3.10618911176577,3.23578322706014,3.26269325353364,3.42237870678029,
3.49281121943322,3.52214049901602,3.52687410283799,3.52934873690492,3.53136451293,
3.5336823032336,3.53758955315858,3.55149730201945,3.78888827893873,3.90640055085566,
3.92492608801512,3.92928222306655,3.93177816618775,3.93371808020571,3.93625659422768,
3.94068369022375,3.95797752250563,4.22572829481897,4.28997352849309,4.34160438303979,
4.34941165000115,4.3515796492766,4.35288939424111,4.35406372663174,4.35555187563319,
4.35788993530852,4.36999889449647,4.62186277568004,4.73789099874759,4.74416639418397,
4.74691487771793,4.74893678386463,4.75080264529649,4.75333208479401,4.75954490870874,
4.82311051877275,4.90635095761544,4.98335325688672,5.13758966274805,5.14745750765565,
5.14958862503011,5.15096544073365,5.15207830464268,5.15334886035637,5.15552310436134,
5.16417522289751,5.22935264471346,5.38943195538701,5.49567112458791,5.56437151347006,
5.57091331971715,5.57356262390711,5.57551184801385,5.57761924885999,5.58047536034238,
5.58695991826877,5.70701839025305,5.78223496458913,5.85756767548642,5.95843458726013,
5.96562440013223,5.96841324242663,5.97008746599995,5.97168493076239,5.97393193038925,
5.9785086244463,6.01875108526842,6.09571659667715,6.22558332806175,6.33099790155063,
6.3417463338379,6.34692924796671,6.35059940071529,6.35444236212084,6.35945076597468,
6.37008032567029,6.38381590989211,6.50305248595167,6.61033121327096,6.68899932446522,
6.6911439401827,6.69846682299931,6.70786823658444,6.71406355422338,6.71643746471502,
6.71803706399938,6.71956934880039,6.72167313368793,6.72640120639067,6.83881363264207,
7.04473471356267,7.11920234201839,7.12627043538521,7.12914008036274,7.13125411132866,
7.13354234508795,7.13664841839845,7.14372219769389,7.26609364661515,7.44406763241697,
7.5384124957183,7.54450139382672,7.54710177529751,7.54895192314209,7.55080436873359,
7.55348766333007,7.56019521650181,7.67766519208207,7.75680515859896,7.94751727124192,
7.97358688586004,7.98323481317064,7.99014324066107,7.99747961903742,8.00726669782614,
8.02924906752106,8.04568397594722,8.09814082665305,8.25654388848295,8.29478093100519,
8.30119871952584,8.30511084035366,8.30817615833971,8.31148049848513,8.31676268781673,
8.33786466406911,8.54600766504765,8.54929210693049,8.59426347079943,8.60597363108527,
8.61286233817759,8.61884395812064,8.62620380444695,8.64046760361987,8.75340891515095,
8.92470453324758,9.03948258503262,9.04930177842657,9.05439046548154,9.06428347330626,
9.06766430407698,9.06982713677481,9.0717737907459,9.07436189944925,9.07965057076832,
9.13153347095929,9.161839032087,9.45082576697285,9.46514098011268,9.4693102371038,
9.47176348756786,9.47390240231286,9.47657653534121,9.48176433342541,9.51577736270638,
9.61169624415625,9.82139515579529,9.82891527249432,9.8444090272567,9.87642326666226,
9.88782640812077,9.8901731141985,9.89166265333087,9.89283630844183,9.89393097241329,
9.89520994627623,9.89703664572866,9.90018424157577,9.95940165500043),
 .UNSPECIFIED.);
#3607=B_SPLINE_CURVE_WITH_KNOTS('',3,(#237706,#237707,#237708,#237709,#237710,
#237711,#237712,#237713,#237714,#237715,#237716,#237717,#237718,#237719,
#237720,#237721,#237722,#237723,#237724,#237725,#237726,#237727,#237728,
#237729,#237730,#237731,#237732,#237733,#237734,#237735,#237736,#237737,
#237738,#237739,#237740,#237741,#237742,#237743,#237744,#237745,#237746,
#237747,#237748,#237749,#237750,#237751,#237752,#237753,#237754,#237755,
#237756,#237757,#237758,#237759,#237760,#237761,#237762,#237763,#237764,
#237765,#237766,#237767,#237768,#237769,#237770,#237771,#237772,#237773,
#237774,#237775,#237776,#237777,#237778,#237779,#237780,#237781,#237782,
#237783,#237784,#237785,#237786,#237787,#237788,#237789,#237790,#237791,
#237792,#237793,#237794,#237795,#237796,#237797,#237798,#237799,#237800,
#237801,#237802,#237803,#237804,#237805,#237806,#237807,#237808,#237809,
#237810,#237811,#237812,#237813,#237814,#237815,#237816,#237817,#237818,
#237819,#237820,#237821,#237822,#237823,#237824,#237825,#237826,#237827,
#237828,#237829,#237830,#237831,#237832,#237833,#237834,#237835,#237836,
#237837,#237838,#237839,#237840,#237841,#237842,#237843,#237844,#237845,
#237846,#237847,#237848,#237849,#237850,#237851,#237852,#237853,#237854,
#237855,#237856,#237857,#237858,#237859,#237860,#237861,#237862,#237863,
#237864,#237865,#237866,#237867,#237868,#237869,#237870,#237871,#237872,
#237873,#237874,#237875,#237876,#237877,#237878,#237879,#237880,#237881,
#237882,#237883,#237884,#237885,#237886,#237887,#237888,#237889,#237890,
#237891,#237892,#237893,#237894,#237895,#237896,#237897,#237898,#237899,
#237900,#237901,#237902,#237903,#237904,#237905,#237906,#237907,#237908,
#237909,#237910,#237911,#237912,#237913,#237914,#237915,#237916,#237917,
#237918,#237919,#237920,#237921,#237922,#237923,#237924,#237925,#237926,
#237927,#237928,#237929,#237930,#237931,#237932,#237933,#237934,#237935,
#237936,#237937,#237938,#237939,#237940,#237941,#237942,#237943,#237944,
#237945,#237946,#237947,#237948,#237949,#237950,#237951,#237952,#237953,
#237954,#237955,#237956,#237957,#237958,#237959,#237960,#237961,#237962,
#237963,#237964,#237965,#237966,#237967,#237968,#237969,#237970,#237971,
#237972,#237973,#237974,#237975,#237976,#237977,#237978,#237979,#237980,
#237981,#237982,#237983,#237984,#237985,#237986,#237987,#237988,#237989,
#237990,#237991,#237992,#237993,#237994,#237995,#237996,#237997,#237998,
#237999,#238000,#238001,#238002,#238003,#238004,#238005,#238006,#238007,
#238008,#238009,#238010,#238011,#238012,#238013,#238014,#238015,#238016,
#238017,#238018,#238019,#238020,#238021,#238022,#238023,#238024,#238025,
#238026,#238027,#238028,#238029,#238030,#238031,#238032,#238033,#238034,
#238035,#238036,#238037,#238038,#238039,#238040,#238041,#238042,#238043,
#238044,#238045,#238046,#238047,#238048,#238049,#238050,#238051,#238052,
#238053,#238054,#238055,#238056,#238057,#238058,#238059,#238060,#238061,
#238062,#238063,#238064,#238065,#238066,#238067,#238068,#238069,#238070,
#238071,#238072,#238073,#238074,#238075,#238076,#238077,#238078,#238079,
#238080,#238081,#238082,#238083,#238084,#238085,#238086,#238087,#238088,
#238089,#238090,#238091,#238092,#238093,#238094,#238095,#238096,#238097,
#238098,#238099,#238100,#238101,#238102,#238103,#238104,#238105,#238106,
#238107,#238108,#238109,#238110,#238111,#238112,#238113,#238114,#238115,
#238116,#238117,#238118,#238119,#238120,#238121,#238122,#238123,#238124,
#238125,#238126,#238127,#238128,#238129,#238130,#238131,#238132,#238133,
#238134,#238135,#238136,#238137,#238138,#238139,#238140,#238141,#238142,
#238143,#238144,#238145,#238146,#238147,#238148,#238149,#238150,#238151,
#238152,#238153,#238154,#238155,#238156,#238157,#238158,#238159,#238160,
#238161,#238162,#238163,#238164,#238165,#238166,#238167,#238168,#238169,
#238170,#238171,#238172,#238173,#238174,#238175,#238176,#238177,#238178,
#238179,#238180,#238181,#238182,#238183,#238184,#238185,#238186,#238187,
#238188,#238189,#238190,#238191,#238192,#238193,#238194,#238195,#238196,
#238197,#238198,#238199,#238200,#238201,#238202,#238203,#238204,#238205,
#238206,#238207,#238208,#238209,#238210,#238211,#238212,#238213,#238214,
#238215,#238216,#238217,#238218,#238219,#238220,#238221,#238222,#238223,
#238224,#238225,#238226,#238227),.UNSPECIFIED.,.F.,.F.,(4,2,2,2,2,2,2,2,
2,2,2,2,2,2,2,2,2,2,2,2,2,2,2,2,2,2,2,2,2,2,2,2,2,2,2,2,2,2,2,2,2,2,2,2,
2,2,2,2,2,2,2,2,2,2,2,2,2,2,2,2,2,2,2,2,2,2,2,2,2,2,2,2,2,2,2,2,2,2,2,2,
2,2,2,2,2,2,2,2,2,2,2,2,2,2,2,2,2,2,2,2,2,2,2,2,2,2,2,2,2,2,2,2,2,2,2,2,
2,2,2,2,2,2,2,2,2,2,2,2,2,2,2,2,2,2,2,2,2,2,2,2,2,2,2,2,2,2,2,2,2,2,2,2,
2,2,2,2,2,2,2,2,2,2,2,2,2,2,2,2,2,2,2,2,2,2,2,2,2,2,2,2,2,2,2,2,2,2,2,2,
2,2,2,2,2,2,2,2,2,2,2,2,2,2,2,2,2,2,2,2,2,2,2,2,2,2,2,2,2,2,2,2,2,2,2,2,
2,2,2,2,2,2,2,2,2,2,2,2,2,2,2,2,2,2,2,2,2,2,2,2,2,2,2,2,2,2,2,2,2,2,2,2,
4),(0.00299195565914869,0.204304804266415,0.320244810562324,0.326542787206419,
0.329294687620281,0.331316600490947,0.333180703415817,0.335705074651995,
0.34189213052287,0.404553223481172,0.411592970530418,0.636928067218467,
0.674866396373037,0.728274714773573,0.731687948662123,0.732873622492273,
0.733912975580605,0.735038047081858,0.736494562585654,0.739635667112466,
0.762236700674419,0.806638273444298,0.869735799451805,0.91887819108263,
1.02262490578281,1.11641133873917,1.14926879989619,1.15424935112239,1.15681302471986,
1.15886177128647,1.16090992805181,1.16457281483211,1.17559656731536,1.34926890633361,
1.46912408925914,1.49973481648366,1.53975517059341,1.54788366995576,1.55071756100016,
1.55235466775212,1.55408252452801,1.55628243085285,1.56061205819994,1.58560172998946,
1.66252762168121,1.79568348466412,1.90226210779061,1.92238455881232,1.92894392654275,
1.93309306340189,1.93694741598128,1.94194703248927,1.95281741083261,2.04698630083693,
2.21071082270353,2.28518518395986,2.29562800539406,2.29848758286372,2.2999467967776,
2.30136522088102,2.30309272570482,2.30601238542521,2.31635510723129,2.47928496179845,
2.62718255999014,2.69509861694944,2.70716634289075,2.71100439381433,2.71344376059045,
2.71571406445084,2.71866068503036,2.72355965343022,2.75169282693605,3.04145885928254,
3.07215039366537,3.11771733149536,3.12663957863907,3.12964350296555,3.13156610184395,
3.13337316435036,3.13574480587359,3.14066074606192,3.17648501260328,3.18151930501821,
3.18343929898297,3.18942585848539,3.31437803155712,3.44601130397284,3.54401305514848,
3.56132449412585,3.57021313896487,3.57674923932828,3.58486885880461,3.59848440236222,
3.64683823566358,3.74302040705679,3.8539846184391,3.87964297138532,3.88568451176497,
3.88916977206863,3.8922000838631,3.89592219022888,3.90339785463276,3.97654938184403,
4.08913883278223,4.14540363197154,4.16811808311313,4.18537536277887,4.1933253522458,
4.19937296409566,4.20512111748317,4.21484449495481,4.24159794094126,4.45351757539433,
4.55123789040861,4.61707546128271,4.6449395881812,4.64961039396671,4.65207151252482,
4.65389151514154,4.65615187015555,4.65990548931065,4.6720731238729,4.93219920390064,
4.9822409057344,5.04390151203434,5.049909093815,5.05282270517774,5.0548972157326,
5.05685876769572,5.05958892498399,5.06504405211841,5.10708895782481,5.17148858104234,
5.38383565645856,5.46715989685606,5.47224009107114,5.47414590115759,5.47527209333453,
5.47633441526766,5.47780871336862,5.48074296883495,5.50618455166452,5.58375004322157,
5.76076495864503,5.8586879061462,5.86559558604784,5.86824256080507,5.87013907252819,
5.87214230079071,5.87477704441215,5.88043824110462,5.95700090597055,6.01606562736595,
6.16564617843788,6.20207302889519,6.26669839135053,6.2707014702226,6.272195380661,
6.27326040581108,6.27427264350614,6.27568974477782,6.27855000631779,6.30173179414512,
6.38026173374556,6.5231089037454,6.66045998095707,6.68852872213931,6.69316443745879,
6.69591560048796,6.69801338715346,6.70024605382043,6.70371473257594,6.7142784953503,
6.77214132597164,6.82731308083084,6.99953481505245,7.03955011865145,7.08358112310091,
7.08861547926961,7.09092686011959,7.09270333393783,7.09460772762128,7.09753502127016,
7.10629747161386,7.15748911108523,7.21600591603339,7.3424301977461,7.36685990934665,
7.37535349354944,7.45410193372041,7.46525987960156,7.47032297712433,7.4741878668301,
7.47831184533427,7.48462591674326,7.50378758916066,7.60845244672014,7.75106830074242,
7.83131352684389,7.83650839589159,7.83853242610142,7.83999396334239,7.84154835255648,
7.84361147349523,7.8478751366821,7.88960619378119,7.93361538749365,8.03018348146863,
8.16687972144069,8.16897151929548,8.17729834377345,8.24152544979838,8.24777404933818,
8.25080347503001,8.25295989749751,8.25499844048672,8.25783506763205,8.26350047360152,
8.3071104767254,8.42184149937684,8.53106033194356,8.58667991039619,8.66114829700223,
8.66668485039674,8.66895620704304,8.67065650039618,8.67252363375266,8.67510603784243,
8.68093741241986,8.76275052773776,8.9334985521694,8.99432166999402,9.08041593852909,
9.09935036586209,9.10855623680853,9.1158165916179,9.12257464338248,9.1305186875639,
9.15441069112099,9.18778239639276,9.28245288027419,9.38920598611402,9.41767991291176,
9.42359865913288,9.42740270733699,9.43026453163843,9.43308749145909,9.43802689747503,
9.45453695458353,9.48325429475277,9.55419608272797,9.69982830507318,9.72174693294451,
9.72986082076731,9.73561480151826,9.74165822659727,9.74757750191515,9.75531173530273,
9.76760694038484,9.96019807358396),.UNSPECIFIED.);
#3608=B_SPLINE_CURVE_WITH_KNOTS('',3,(#238229,#238230,#238231,#238232,#238233,
#238234,#238235,#238236,#238237,#238238,#238239,#238240),.UNSPECIFIED.,
 .F.,.F.,(4,1,1,1,1,1,1,1,1,4),(-117.190265949363,-116.852549095875,-115.853809360013,
-114.855069624151,-113.856329888289,-113.356960020358,-112.857590152427,
-111.858850416564,-111.359480548633,-110.907173562223),.UNSPECIFIED.);
#3609=B_SPLINE_CURVE_WITH_KNOTS('',3,(#238242,#238243,#238244,#238245,#238246,
#238247,#238248,#238249,#238250,#238251,#238252,#238253,#238254,#238255,
#238256,#238257,#238258,#238259,#238260,#238261,#238262,#238263,#238264,
#238265,#238266,#238267,#238268,#238269,#238270,#238271,#238272,#238273,
#238274,#238275,#238276,#238277,#238278,#238279,#238280,#238281,#238282,
#238283,#238284,#238285,#238286,#238287,#238288,#238289,#238290,#238291,
#238292,#238293,#238294,#238295,#238296,#238297,#238298,#238299,#238300,
#238301,#238302,#238303,#238304,#238305,#238306,#238307,#238308,#238309,
#238310,#238311,#238312,#238313,#238314,#238315,#238316,#238317,#238318,
#238319,#238320,#238321,#238322,#238323,#238324,#238325,#238326,#238327,
#238328,#238329,#238330,#238331,#238332,#238333,#238334,#238335,#238336,
#238337,#238338,#238339,#238340,#238341,#238342,#238343,#238344,#238345,
#238346,#238347,#238348,#238349,#238350,#238351,#238352,#238353,#238354,
#238355,#238356,#238357,#238358,#238359,#238360,#238361,#238362,#238363,
#238364,#238365,#238366,#238367,#238368,#238369,#238370,#238371,#238372,
#238373,#238374,#238375,#238376,#238377,#238378,#238379,#238380,#238381,
#238382,#238383,#238384,#238385,#238386,#238387,#238388,#238389,#238390,
#238391,#238392,#238393,#238394,#238395,#238396,#238397,#238398,#238399,
#238400,#238401,#238402,#238403,#238404,#238405,#238406,#238407,#238408,
#238409,#238410,#238411,#238412,#238413,#238414,#238415,#238416,#238417,
#238418,#238419,#238420,#238421,#238422,#238423,#238424,#238425,#238426,
#238427,#238428,#238429,#238430,#238431,#238432,#238433,#238434,#238435,
#238436,#238437,#238438,#238439,#238440,#238441,#238442,#238443,#238444,
#238445,#238446,#238447,#238448,#238449,#238450,#238451,#238452,#238453,
#238454,#238455,#238456,#238457,#238458,#238459,#238460,#238461,#238462,
#238463,#238464,#238465,#238466,#238467,#238468,#238469,#238470,#238471,
#238472,#238473,#238474,#238475,#238476,#238477,#238478,#238479,#238480,
#238481,#238482,#238483,#238484,#238485,#238486,#238487,#238488,#238489,
#238490,#238491,#238492,#238493,#238494,#238495,#238496,#238497,#238498,
#238499,#238500,#238501,#238502,#238503,#238504,#238505,#238506,#238507,
#238508,#238509,#238510,#238511,#238512,#238513,#238514,#238515,#238516,
#238517,#238518,#238519,#238520,#238521,#238522,#238523,#238524,#238525,
#238526,#238527,#238528,#238529,#238530,#238531,#238532,#238533,#238534,
#238535,#238536,#238537,#238538,#238539,#238540,#238541,#238542,#238543,
#238544,#238545,#238546,#238547,#238548,#238549,#238550,#238551,#238552,
#238553,#238554,#238555,#238556,#238557,#238558,#238559,#238560,#238561,
#238562,#238563,#238564,#238565,#238566,#238567,#238568,#238569,#238570,
#238571,#238572,#238573,#238574,#238575,#238576,#238577,#238578,#238579,
#238580,#238581,#238582,#238583,#238584,#238585,#238586,#238587,#238588,
#238589,#238590,#238591,#238592,#238593,#238594,#238595,#238596,#238597,
#238598,#238599,#238600,#238601,#238602,#238603,#238604,#238605,#238606,
#238607,#238608,#238609,#238610,#238611,#238612,#238613,#238614,#238615,
#238616,#238617,#238618,#238619,#238620,#238621,#238622,#238623,#238624,
#238625,#238626,#238627,#238628,#238629,#238630,#238631,#238632,#238633,
#238634,#238635,#238636,#238637,#238638,#238639,#238640,#238641,#238642,
#238643,#238644,#238645,#238646,#238647,#238648,#238649,#238650,#238651,
#238652,#238653,#238654,#238655,#238656,#238657,#238658,#238659,#238660,
#238661,#238662,#238663,#238664,#238665,#238666,#238667,#238668,#238669,
#238670,#238671,#238672,#238673,#238674,#238675,#238676,#238677,#238678,
#238679,#238680,#238681,#238682,#238683,#238684,#238685,#238686,#238687,
#238688,#238689,#238690,#238691,#238692,#238693,#238694,#238695,#238696,
#238697,#238698,#238699,#238700,#238701,#238702,#238703,#238704,#238705,
#238706,#238707,#238708,#238709,#238710,#238711,#238712,#238713,#238714,
#238715,#238716,#238717,#238718,#238719,#238720,#238721,#238722,#238723,
#238724,#238725,#238726,#238727,#238728,#238729,#238730,#238731,#238732,
#238733,#238734,#238735,#238736,#238737,#238738,#238739,#238740,#238741,
#238742,#238743,#238744,#238745,#238746,#238747,#238748,#238749,#238750,
#238751,#238752,#238753,#238754,#238755,#238756,#238757,#238758,#238759,
#238760,#238761,#238762,#238763,#238764,#238765,#238766,#238767,#238768,
#238769,#238770,#238771,#238772,#238773),.UNSPECIFIED.,.F.,.F.,(4,2,2,2,
2,2,2,2,2,2,2,2,2,2,2,2,2,2,2,2,2,2,2,2,2,2,2,2,2,2,2,2,2,2,2,2,2,2,2,2,
2,2,2,2,2,2,2,2,2,2,2,2,2,2,2,2,2,2,2,2,2,2,2,2,2,2,2,2,2,2,2,2,2,2,2,2,
2,2,2,2,2,2,2,2,2,2,2,2,2,2,2,2,2,2,2,2,2,2,2,2,2,2,2,2,2,2,2,2,2,2,2,2,
2,2,2,2,2,2,2,2,2,2,2,2,2,2,2,2,2,2,2,2,2,2,2,2,2,2,2,2,2,2,2,2,2,2,2,2,
2,2,2,2,2,2,2,2,2,2,2,2,2,2,2,2,2,2,2,2,2,2,2,2,2,2,2,2,2,2,2,2,2,2,2,2,
2,2,2,2,2,2,2,2,2,2,2,2,2,2,2,2,2,2,2,2,2,2,2,2,2,2,2,2,2,2,2,2,2,2,2,2,
2,2,2,2,2,2,2,2,2,2,2,2,2,2,2,2,2,2,2,2,2,2,2,2,2,2,2,2,2,2,2,2,2,2,2,2,
2,2,2,2,2,2,2,2,2,4),(0.00169228455310972,0.0208076269905666,0.0253450676512967,
0.028578787775409,0.0314337004501233,0.0344443448113954,0.038454885536899,
0.0472928164606967,0.0676712750305325,0.222564681765073,0.313584499892351,
0.323952755739825,0.330905989705942,0.337640572908688,0.343642230693239,
0.351231648228265,0.3632360314278,0.442557054241769,0.455688197628108,0.586744997765805,
0.690920919657209,0.758036552953802,0.776820279838839,0.788331717801715,
0.790967179565189,0.793431903208939,0.795252200090675,0.797225314918757,
0.800077186140425,0.808129421379954,0.920323387521312,1.00928009993188,
1.03197721228674,1.07611124159112,1.15343357722061,1.18712921290333,1.19230671378435,
1.19497966880917,1.19693349108771,1.19903142785402,1.20264945607814,1.21268970641155,
1.35854381573034,1.43676116437018,1.55776425527931,1.59433205669564,1.61139695277517,
1.61415929065484,1.61559878379946,1.61676842347332,1.61810957967311,1.62036069398205,
1.62865214230122,1.76175622680944,1.87950054449306,1.93305524260216,1.97954626927877,
2.00334533803057,2.00777689856845,2.01016203636926,2.01212151155541,2.01412670253363,
2.01784484117802,2.03003463628287,2.20610779653977,2.31332088712653,2.4083246153947,
2.41183163265305,2.41335669410116,2.41448827944028,2.41554171415283,2.41698384425655,
2.41984225800678,2.44327430915916,2.56101213228956,2.71742644390102,2.82484555380525,
2.83310698266921,2.83625776692704,2.83842203236919,2.84053709857879,2.84307946885111,
2.84939172199921,2.90553149848208,2.94267724921543,2.9474590867901,3.01941150883196,
3.14739623827848,3.20002360362122,3.2167685300442,3.22383622191268,3.22917713514963,
3.23156450679453,3.23335512552312,3.23500704905952,3.23724595120155,3.2416207474191,
3.27612070593001,3.41987860763695,3.52016687370595,3.58886499066643,3.60427151014516,
3.61014193184447,3.61414277597609,3.61803429467319,3.62269433790107,3.63423239363179,
3.78394630907534,3.90780218299441,3.95387866748268,3.97487437816231,3.97842863793518,
3.98030141090392,3.98183396814278,3.98360363767069,3.98660389098188,3.99749576972629,
4.23922173720676,4.34334398942954,4.38479330531526,4.39039362823808,4.39321661640452,
4.39525288334908,4.3974138877732,4.40046121041333,4.40859415404207,4.53508409308175,
4.7280846798277,4.78147015467643,4.80481267547004,4.80894458182232,4.81114795898351,
4.81296503373147,4.81480403383221,4.81820463144641,4.82933357975924,4.83068598413479,
4.93244088232358,4.97959955842857,5.2115747076536,5.23720597040815,5.24680704476339,
5.25370468666267,5.26105045543184,5.27088604405945,5.29313366319661,5.48935994625193,
5.55700391340357,5.56511838418575,5.56903859757746,5.57208859002595,5.57544979738637,
5.58100989282558,5.60602751137852,5.65806073355562,5.81309836040524,5.85793712897173,
5.86963851818398,5.87652674884228,5.88251081746369,5.88987733632125,5.9041658123057,
6.01761112622703,6.12439057893242,6.27537940762288,6.32397338177412,6.32980036219826,
6.33246470724888,6.33450816038374,6.33669527817769,6.34011969931916,6.35076906884506,
6.40666787173508,6.48385107286157,6.66964267094354,6.72478816321071,6.73113790592886,
6.73405765829006,6.73622044784171,6.73804013832393,6.74111495239306,6.74840795149835,
6.8668242706869,6.99071742597146,7.14196370014696,7.1516794128272,7.15389525291374,
7.15534464068133,7.15651506553866,7.15784919170866,7.16012695650551,7.16963249840598,
7.21817697075377,7.33881573120204,7.53193293115088,7.54449433845744,7.54818121967568,
7.55039306320065,7.55233415854644,7.55475191927114,7.5593361462241,7.58622963422652,
7.6377810628483,7.69746167566451,7.93676797303654,7.9498855680596,7.95223786817523,
7.95366549810445,7.95478635074989,7.95601335864582,7.95799267409618,7.96462642168007,
8.0053286665715,8.06381251433966,8.12397765349998,8.14629453413927,8.17093619392347,
8.17899959373945,8.21661780854425,8.36294588747713,8.37257863718179,8.3759768179475,
8.37817903062541,8.38022574589198,8.3828842390018,8.38850258874395,8.44665309134468,
8.54610240447915,8.65619970976153,8.722040668501,8.76462846072826,8.76913501639208,
8.771409862585,8.77307097752536,8.77485496533041,8.77725130282303,8.78260350901246,
8.8665284594664,9.09788295166691,9.13877535851554,9.14768687169815,9.15244662830048,
9.15626185421358,9.16058702776937,9.16793282344946,9.19703446173512,9.42066559124138,
9.51279039668691,9.51816002007446,9.52021292130714,9.52168233687259,9.52307842345449,
9.52503216348626,9.52897642995906,9.56674891862977,9.61277441818467,9.90812336478384,
9.9220811786498,9.9301983200311,9.93324339390951,9.93540400980293,9.93757600224356,
9.9397668989649,9.94258125256913,9.9495742293905,9.95986201202622),
 .UNSPECIFIED.);
#3610=B_SPLINE_CURVE_WITH_KNOTS('',3,(#238775,#238776,#238777,#238778,#238779,
#238780,#238781,#238782,#238783,#238784,#238785,#238786,#238787,#238788,
#238789,#238790,#238791,#238792,#238793,#238794,#238795,#238796,#238797,
#238798,#238799,#238800,#238801,#238802,#238803,#238804,#238805,#238806,
#238807,#238808,#238809,#238810,#238811,#238812,#238813,#238814,#238815,
#238816,#238817,#238818,#238819,#238820,#238821,#238822,#238823,#238824,
#238825,#238826,#238827,#238828,#238829,#238830,#238831,#238832,#238833,
#238834,#238835,#238836,#238837,#238838,#238839,#238840,#238841,#238842,
#238843,#238844,#238845,#238846,#238847,#238848,#238849,#238850,#238851,
#238852,#238853,#238854,#238855,#238856,#238857,#238858,#238859,#238860,
#238861,#238862,#238863,#238864,#238865,#238866,#238867,#238868,#238869,
#238870,#238871,#238872,#238873,#238874,#238875,#238876,#238877,#238878,
#238879,#238880,#238881,#238882,#238883,#238884,#238885,#238886,#238887,
#238888,#238889,#238890,#238891,#238892,#238893,#238894,#238895,#238896,
#238897,#238898,#238899,#238900,#238901,#238902,#238903,#238904,#238905,
#238906,#238907,#238908,#238909,#238910,#238911,#238912,#238913,#238914,
#238915,#238916,#238917,#238918,#238919,#238920,#238921,#238922,#238923,
#238924,#238925,#238926,#238927,#238928,#238929,#238930,#238931,#238932,
#238933,#238934,#238935,#238936,#238937,#238938,#238939,#238940,#238941,
#238942,#238943,#238944,#238945,#238946,#238947,#238948,#238949,#238950,
#238951,#238952,#238953,#238954,#238955,#238956,#238957,#238958,#238959,
#238960,#238961,#238962,#238963,#238964,#238965,#238966,#238967,#238968,
#238969,#238970,#238971,#238972,#238973,#238974,#238975,#238976,#238977,
#238978,#238979,#238980,#238981,#238982,#238983,#238984,#238985,#238986,
#238987,#238988,#238989,#238990,#238991,#238992,#238993,#238994,#238995,
#238996,#238997,#238998,#238999,#239000,#239001,#239002,#239003,#239004,
#239005,#239006,#239007,#239008,#239009,#239010,#239011,#239012,#239013,
#239014,#239015,#239016,#239017,#239018,#239019,#239020,#239021,#239022,
#239023,#239024,#239025,#239026,#239027,#239028,#239029,#239030,#239031,
#239032,#239033,#239034,#239035,#239036),.UNSPECIFIED.,.F.,.F.,(4,3,3,3,
3,3,3,3,3,3,3,3,3,3,3,3,3,3,3,3,3,3,3,3,3,3,3,3,3,3,3,3,3,3,3,3,3,3,3,3,
3,3,3,3,3,3,3,3,3,3,3,3,3,3,3,3,3,3,3,3,3,3,3,3,3,3,3,3,3,3,3,3,3,3,3,3,
3,3,3,3,3,3,3,3,3,3,3,4),(-98.3406346348103,-98.2595400399228,-98.1783170760883,
-98.0969160050002,-98.0154335325594,-97.9338358821689,-97.8764941144939,
-97.8027170236699,-97.7290022462361,-97.6553367119498,-97.5817065668627,
-97.5080979430576,-97.4344851252523,-97.3771242465628,-97.2956907154816,
-97.2141217204853,-97.1300298850219,-97.0481871785268,-96.9629707785793,
-96.8777543786317,-96.7993214351354,-96.7209582512547,-96.6426599859769,
-96.56444072012,-96.4862714286153,-96.4081601035283,-96.3783845107007,-96.3020220396171,
-96.2256427135349,-96.1492369478946,-96.0727622758028,-95.9962502280743,
-95.919655898848,-95.8790146427695,-95.803637263832,-95.7283214304325,-95.6530543208225,
-95.5778231457396,-95.5026151405947,-95.4248226113838,-95.3496044352015,
-95.2743695596237,-95.1991064160779,-95.1238034227342,-95.0484112267784,
-94.9729663274293,-94.8974229663296,-94.8802749069074,-94.8071310979317,
-94.7340760848174,-94.6610949304227,-94.5881727677748,-94.5152947844789,
-94.4424462086562,-94.3695988076401,-94.2967484614904,-94.2238818214328,
-94.1509855280076,-94.0780033880236,-94.0049744872913,-93.93183493372,-93.8815351710452,
-93.8069465518206,-93.7324435814405,-93.6580123236801,-93.5836388898013,
-93.5093094293879,-93.4350101216312,-93.3607167604803,-93.2864232114111,
-93.212116980803,-93.1377855706714,-93.063381527802,-92.9889358754876,-92.9143993173973,
-92.882795435183,-92.8018014557991,-92.7209244177331,-92.6365497051128,
-92.5559913111839,-92.4755567692027,-92.3952973516194,-92.3834255672519,
-92.3127120478732,-92.2419793657373,-92.1712373965128,-92.100443561887,
-92.0575247206449),.UNSPECIFIED.);
#3611=B_SPLINE_CURVE_WITH_KNOTS('',3,(#239038,#239039,#239040,#239041,#239042,
#239043,#239044,#239045,#239046,#239047,#239048,#239049,#239050,#239051,
#239052,#239053,#239054,#239055,#239056,#239057,#239058,#239059,#239060,
#239061,#239062,#239063,#239064,#239065,#239066,#239067,#239068,#239069,
#239070,#239071,#239072,#239073,#239074,#239075,#239076,#239077,#239078,
#239079,#239080,#239081,#239082,#239083,#239084,#239085,#239086,#239087,
#239088,#239089,#239090,#239091,#239092,#239093,#239094,#239095,#239096,
#239097,#239098,#239099,#239100,#239101,#239102,#239103,#239104,#239105,
#239106,#239107,#239108,#239109,#239110,#239111,#239112,#239113,#239114,
#239115,#239116,#239117,#239118,#239119,#239120,#239121,#239122,#239123,
#239124,#239125,#239126,#239127,#239128,#239129,#239130,#239131,#239132,
#239133,#239134,#239135,#239136,#239137,#239138,#239139,#239140,#239141,
#239142,#239143,#239144,#239145,#239146,#239147,#239148,#239149,#239150,
#239151,#239152,#239153,#239154,#239155,#239156,#239157,#239158,#239159,
#239160,#239161,#239162,#239163,#239164,#239165,#239166,#239167,#239168,
#239169,#239170,#239171,#239172,#239173,#239174,#239175,#239176,#239177,
#239178,#239179,#239180,#239181,#239182,#239183,#239184,#239185,#239186,
#239187,#239188,#239189,#239190,#239191,#239192,#239193,#239194,#239195,
#239196,#239197,#239198,#239199,#239200,#239201,#239202,#239203,#239204,
#239205,#239206,#239207,#239208,#239209,#239210,#239211,#239212,#239213,
#239214,#239215,#239216,#239217,#239218,#239219,#239220,#239221,#239222,
#239223,#239224,#239225,#239226,#239227,#239228,#239229,#239230,#239231,
#239232,#239233,#239234,#239235,#239236,#239237,#239238,#239239,#239240,
#239241,#239242,#239243,#239244,#239245,#239246,#239247,#239248,#239249,
#239250,#239251,#239252,#239253,#239254,#239255,#239256,#239257,#239258,
#239259,#239260,#239261,#239262,#239263,#239264,#239265,#239266,#239267,
#239268,#239269,#239270,#239271,#239272,#239273,#239274,#239275,#239276,
#239277,#239278,#239279,#239280,#239281,#239282,#239283,#239284,#239285,
#239286,#239287,#239288,#239289,#239290,#239291,#239292,#239293,#239294,
#239295,#239296,#239297,#239298,#239299,#239300,#239301,#239302,#239303,
#239304,#239305,#239306,#239307,#239308,#239309,#239310,#239311,#239312,
#239313,#239314,#239315,#239316,#239317,#239318,#239319,#239320,#239321,
#239322,#239323,#239324,#239325,#239326,#239327,#239328,#239329,#239330,
#239331,#239332,#239333,#239334,#239335,#239336,#239337,#239338,#239339,
#239340,#239341,#239342,#239343,#239344,#239345,#239346,#239347,#239348,
#239349,#239350,#239351,#239352,#239353,#239354,#239355,#239356,#239357,
#239358,#239359,#239360,#239361,#239362,#239363,#239364,#239365,#239366,
#239367,#239368,#239369,#239370,#239371,#239372,#239373,#239374,#239375,
#239376,#239377,#239378,#239379,#239380,#239381,#239382,#239383,#239384,
#239385,#239386,#239387,#239388,#239389,#239390,#239391,#239392,#239393,
#239394,#239395,#239396,#239397,#239398,#239399,#239400,#239401,#239402,
#239403,#239404,#239405,#239406,#239407,#239408,#239409,#239410,#239411,
#239412,#239413,#239414,#239415,#239416,#239417,#239418,#239419,#239420,
#239421,#239422,#239423,#239424,#239425,#239426,#239427,#239428,#239429,
#239430,#239431,#239432,#239433,#239434,#239435,#239436,#239437,#239438,
#239439,#239440,#239441,#239442,#239443,#239444,#239445,#239446,#239447,
#239448,#239449,#239450,#239451,#239452,#239453,#239454,#239455,#239456,
#239457,#239458,#239459,#239460,#239461,#239462,#239463,#239464,#239465,
#239466,#239467,#239468,#239469,#239470,#239471,#239472,#239473,#239474,
#239475,#239476,#239477,#239478,#239479,#239480,#239481,#239482,#239483,
#239484,#239485,#239486,#239487,#239488,#239489,#239490,#239491,#239492,
#239493,#239494,#239495,#239496,#239497,#239498,#239499,#239500,#239501,
#239502,#239503,#239504,#239505,#239506,#239507,#239508,#239509,#239510,
#239511,#239512,#239513,#239514,#239515,#239516,#239517,#239518,#239519,
#239520,#239521,#239522,#239523,#239524,#239525,#239526,#239527,#239528,
#239529,#239530,#239531,#239532,#239533,#239534,#239535,#239536,#239537,
#239538,#239539,#239540,#239541,#239542,#239543,#239544,#239545,#239546,
#239547,#239548,#239549,#239550,#239551,#239552,#239553,#239554,#239555,
#239556,#239557,#239558,#239559,#239560,#239561,#239562,#239563,#239564,
#239565,#239566,#239567,#239568,#239569),.UNSPECIFIED.,.F.,.F.,(4,2,2,2,
2,2,2,2,2,2,2,2,2,2,2,2,2,2,2,2,2,2,2,2,2,2,2,2,2,2,2,2,2,2,2,2,2,2,2,2,
2,2,2,2,2,2,2,2,2,2,2,2,2,2,2,2,2,2,2,2,2,2,2,2,2,2,2,2,2,2,2,2,2,2,2,2,
2,2,2,2,2,2,2,2,2,2,2,2,2,2,2,2,2,2,2,2,2,2,2,2,2,2,2,2,2,2,2,2,2,2,2,2,
2,2,2,2,2,2,2,2,2,2,2,2,2,2,2,2,2,2,2,2,2,2,2,2,2,2,2,2,2,2,2,2,2,2,2,2,
2,2,2,2,2,2,2,2,2,2,2,2,2,2,2,2,2,2,2,2,2,2,2,2,2,2,2,2,2,2,2,2,2,2,2,2,
2,2,2,2,2,2,2,2,2,2,2,2,2,2,2,2,2,2,2,2,2,2,2,2,2,2,2,2,2,2,2,2,2,2,2,2,
2,2,2,2,2,2,2,2,2,2,2,2,2,2,2,2,2,2,2,2,2,2,2,2,2,2,2,2,2,2,2,2,2,2,2,2,
2,2,2,2,2,2,2,2,2,4),(0.00168853654697166,0.103339731779065,0.116709103368618,
0.119909819402091,0.121921927725409,0.123450686793796,0.125005944841013,
0.12646436286641,0.128477680641417,0.132515065212291,0.177689730312591,
0.228623367850564,0.249036582934583,0.268445607615176,0.303450819898069,
0.374741801445695,0.484928277307592,0.527814364491861,0.533458032260693,
0.536289952263605,0.538327552940703,0.540485236988003,0.543520125587614,
0.549791950905152,0.61495115622597,0.831600933000776,0.906641884417419,
0.933284008908887,0.948747815085201,0.952405588095498,0.954155556065803,
0.955805456194687,0.957564232907861,0.960565088326756,0.96872739470707,
1.01488825339754,1.02098415546149,1.10356382417768,1.3277152707527,1.37527288312188,
1.38490143914292,1.39382965514626,1.40037061669404,1.40846560719594,1.42196674955635,
1.46898226310315,1.58285488841581,1.64103889779607,1.68191669357966,1.70389993752507,
1.70964361566064,1.7125441444328,1.71549165590169,1.71859027738407,1.72424135909924,
1.74799894038754,1.93308197397957,1.99880602126494,2.01127147313891,2.01853235860103,
2.02451028080824,2.03148133259751,2.04356235634708,2.09646940527705,2.10398228705012,
2.10490186330515,2.10587811737234,2.10854866602033,2.3290771378131,2.46349727660132,
2.47181110792954,2.47491926149835,2.47681356345735,2.47885612828041,2.48151546511217,
2.48731761399358,2.54145516429396,2.7652313972412,2.8377069473607,2.87007967974646,
2.87520429309674,2.87786585918399,2.8800244111254,2.88217749645447,2.88607186763164,
2.89810235538176,3.08116099681484,3.19950167804142,3.24734514166295,3.2788950104216,
3.29439130645193,3.29708304165713,3.29850744990815,3.29956309069247,3.30071056266545,
3.30237447278133,3.30719192326801,3.38260961457423,3.55985410753927,3.65239015410068,
3.68556094803072,3.69039635096814,3.69286646711469,3.69466131221872,3.69657836676933,
3.6998587646696,3.70880991178198,3.84228172598022,3.98236506457672,4.05625028332767,
4.08053406073973,4.09280075552887,4.09519521565728,4.09650557507375,4.09750598523813,
4.09862346252664,4.10066859228941,4.10716399529996,4.2100660153807,4.41703773010512,
4.51076886249678,4.51679478019851,4.5195658435748,4.52165877740946,4.52362998002922,
4.52636489079275,4.53189764305847,4.58282917182821,4.63692616519046,4.82942715706796,
4.89896505390662,4.91025439857647,4.91345940811302,4.91541200134376,4.9171736932817,
4.91942168872401,4.92385406422193,4.95016294717397,4.97897029083771,5.036575624393,
5.12685406664593,5.16867720942107,5.27631099976005,5.28829590462778,5.29304485042576,
5.29695758346708,5.30093033201643,5.30666871558552,5.32155851700503,5.39021514263851,
5.48803571729544,5.65017830051696,5.65875447732786,5.66152321278846,5.66305339979902,
5.66457194136063,5.66645483831327,5.67005879372544,5.69379770098295,5.72471854317786,
5.76343072559383,5.97135389644435,5.99512276541605,6.064694695965,6.07163974256652,
6.07448754261534,6.07659580077471,6.0788877827083,6.08201681604806,6.08922084850348,
6.19287285235846,6.34176514002606,6.47990495044213,6.48870401131937,6.49180150205578,
6.49357792703083,6.49522056462194,6.49745034302472,6.50171003325252,6.5278425942545,
6.58887115706061,6.6913161784719,6.89253921815124,6.91862129425685,6.92914893333392,
6.93593619220506,6.94335382702288,6.9536284980989,6.97849892936106,7.09448146098816,
7.17109372123003,7.2383000085443,7.24640418032512,7.25032117506468,7.25336944989762,
7.25672956132128,7.26228993755151,7.28734330302029,7.33950737510419,7.50053846524446,
7.54002157104421,7.55016741781575,7.55707834179827,7.56245209498876,7.56931978872469,
7.58125956322892,7.637273796907,7.76266390317901,7.98173145793878,7.99701380263632,
8.00066057287301,8.00949775476811,8.01279011218912,8.01473234487359,8.01656264501494,
8.01910058157145,8.02414191891868,8.06313402520017,8.08316012605268,8.2061315746236,
8.35853773941729,8.40601511165231,8.41160863972868,8.41441819759993,8.41646443728593,
8.41853123151786,8.42133640741034,8.42721010458581,8.43487546995718,8.452623324503,
8.50440190469988,8.57372475598848,8.81842456013667,8.83201697021729,8.83451051409028,
8.83602848572844,8.83720922687333,8.83848890813283,8.84052533983301,8.8473323555643,
8.89005019233614,8.93182688192965,9.0390439423254,9.09698435937286,9.20580204566911,
9.22396924230918,9.22785583344512,9.23035189577089,9.23224036131919,9.23439597264157,
9.23785350294356,9.24194676519544,9.24979245494232,9.26864661996942,9.32277930518578,
9.42944215632464,9.61843082928927,9.63014555805185,9.63240842327018,9.63382458804416,
9.63494069532217,9.6361854288512,9.63824561408103,9.64566164813229,9.69449048739954,
9.95574806259247),.UNSPECIFIED.);
#3612=B_SPLINE_CURVE_WITH_KNOTS('',3,(#239571,#239572,#239573,#239574,#239575,
#239576,#239577,#239578,#239579,#239580,#239581,#239582,#239583,#239584,
#239585,#239586,#239587,#239588,#239589,#239590,#239591,#239592,#239593,
#239594,#239595,#239596,#239597,#239598,#239599,#239600,#239601,#239602,
#239603,#239604,#239605,#239606,#239607,#239608,#239609,#239610,#239611,
#239612,#239613,#239614,#239615,#239616,#239617,#239618,#239619,#239620,
#239621,#239622,#239623,#239624,#239625,#239626,#239627,#239628,#239629,
#239630,#239631,#239632,#239633,#239634,#239635,#239636,#239637,#239638,
#239639,#239640,#239641,#239642,#239643,#239644,#239645,#239646,#239647,
#239648,#239649,#239650,#239651,#239652,#239653,#239654,#239655,#239656,
#239657,#239658,#239659,#239660,#239661,#239662,#239663,#239664,#239665,
#239666,#239667,#239668,#239669,#239670,#239671,#239672,#239673,#239674,
#239675,#239676,#239677,#239678,#239679,#239680,#239681,#239682,#239683,
#239684,#239685,#239686,#239687,#239688,#239689,#239690,#239691,#239692,
#239693,#239694,#239695,#239696,#239697,#239698,#239699,#239700,#239701,
#239702,#239703,#239704,#239705,#239706,#239707,#239708,#239709,#239710,
#239711,#239712,#239713,#239714,#239715,#239716,#239717,#239718,#239719,
#239720,#239721,#239722,#239723,#239724,#239725,#239726,#239727,#239728,
#239729,#239730,#239731,#239732,#239733,#239734,#239735,#239736,#239737,
#239738,#239739,#239740,#239741,#239742,#239743,#239744,#239745,#239746,
#239747,#239748,#239749,#239750,#239751,#239752,#239753,#239754,#239755,
#239756,#239757,#239758,#239759,#239760,#239761,#239762,#239763,#239764,
#239765,#239766,#239767,#239768,#239769,#239770,#239771,#239772,#239773,
#239774,#239775,#239776,#239777,#239778,#239779,#239780,#239781,#239782,
#239783,#239784,#239785,#239786,#239787,#239788,#239789,#239790,#239791,
#239792,#239793,#239794,#239795,#239796,#239797,#239798,#239799,#239800,
#239801,#239802,#239803,#239804,#239805,#239806,#239807,#239808,#239809,
#239810,#239811,#239812,#239813,#239814,#239815,#239816,#239817,#239818,
#239819,#239820,#239821,#239822,#239823,#239824,#239825,#239826,#239827,
#239828,#239829),.UNSPECIFIED.,.F.,.F.,(4,3,3,3,3,3,3,3,3,3,3,3,3,3,3,3,
3,3,3,3,3,3,3,3,3,3,3,3,3,3,3,3,3,3,3,3,3,3,3,3,3,3,3,3,3,3,3,3,3,3,3,3,
3,3,3,3,3,3,3,3,3,3,3,3,3,3,3,3,3,3,3,3,3,3,3,3,3,3,3,3,3,3,3,3,3,3,4),
(-79.4911541062857,-79.4169417776376,-79.3427292477536,-79.2685040476418,
-79.1942537038747,-79.119923121499,-79.0455512581999,-78.9710699178442,
-78.9004391331125,-78.8194451537285,-78.738568115662,-78.6541934030418,
-78.5736350091126,-78.4932004671337,-78.412941049551,-78.4010692651813,
-78.3266649619649,-78.252243891163,-78.177793779712,-78.103261744439,-78.0286853041711,
-77.9540043574025,-77.9016993972503,-77.8251278538832,-77.7486239612732,
-77.6721767666834,-77.5957753576583,-77.5194088546811,-77.4423527055195,
-77.3660153154383,-77.2896784441415,-77.2133322359245,-77.1357390922904,
-77.0593199805502,-76.9811398209692,-76.9029596613881,-76.8291825705641,
-76.7554677931303,-76.6818022588445,-76.6081721137573,-76.5345634899521,
-76.4609506721469,-76.403589793457,-76.3221562623758,-76.2405872673796,
-76.1564954319162,-76.074652725421,-75.9894363254734,-75.9042199255259,
-75.8257869820293,-75.7474237981485,-75.6691255328703,-75.5909062670135,
-75.5127369755081,-75.434625650421,-75.4048500575948,-75.3284875865113,
-75.2521082604288,-75.1757024947876,-75.0992278226961,-75.0227157749675,
-74.9461214457415,-74.9054801896637,-74.8301028107262,-74.7547869773266,
-74.6795198677163,-74.6042886926334,-74.5290806874893,-74.4512881582783,
-74.3760699820961,-74.3008351065181,-74.2255719629728,-74.1502689696294,
-74.0748767736736,-73.9994318743241,-73.9238885132244,-73.9067404538015,
-73.8341485820666,-73.7616487829755,-73.6892437432365,-73.616893345192,
-73.5445839604959,-73.4723019987726,-73.4000210509366,-73.3277420649391,
-73.2554289082589,-73.2079687991061),.UNSPECIFIED.);
#3613=B_SPLINE_CURVE_WITH_KNOTS('',3,(#239831,#239832,#239833,#239834,#239835,
#239836,#239837,#239838,#239839,#239840,#239841,#239842,#239843),
 .UNSPECIFIED.,.F.,.F.,(4,1,1,1,1,1,1,1,1,1,4),(-73.2079630106607,-72.9080007179394,
-71.9092609820772,-71.4098911141461,-70.910521246215,-69.9117815103528,
-69.4124116424217,-68.9130417744906,-68.4136719065595,-67.9143020386284,
-66.9247834919266),.UNSPECIFIED.);
#3614=B_SPLINE_CURVE_WITH_KNOTS('',3,(#239845,#239846,#239847,#239848,#239849,
#239850,#239851,#239852,#239853,#239854,#239855,#239856,#239857,#239858,
#239859,#239860,#239861,#239862,#239863,#239864,#239865,#239866,#239867,
#239868,#239869,#239870,#239871,#239872,#239873,#239874,#239875,#239876,
#239877,#239878,#239879,#239880,#239881,#239882,#239883,#239884,#239885,
#239886,#239887,#239888,#239889,#239890,#239891,#239892,#239893,#239894,
#239895,#239896,#239897,#239898,#239899,#239900,#239901,#239902,#239903,
#239904,#239905,#239906,#239907,#239908,#239909,#239910,#239911,#239912,
#239913,#239914,#239915,#239916,#239917,#239918,#239919,#239920,#239921,
#239922,#239923,#239924,#239925,#239926,#239927,#239928,#239929,#239930,
#239931,#239932,#239933,#239934,#239935,#239936,#239937,#239938,#239939,
#239940,#239941,#239942,#239943,#239944,#239945,#239946,#239947,#239948,
#239949,#239950,#239951,#239952,#239953,#239954,#239955,#239956,#239957,
#239958,#239959,#239960,#239961,#239962,#239963,#239964,#239965,#239966,
#239967,#239968,#239969,#239970,#239971,#239972,#239973,#239974,#239975,
#239976,#239977,#239978,#239979,#239980,#239981,#239982,#239983,#239984,
#239985,#239986,#239987,#239988,#239989,#239990,#239991,#239992,#239993,
#239994,#239995,#239996,#239997,#239998,#239999,#240000,#240001,#240002,
#240003,#240004,#240005,#240006,#240007,#240008,#240009,#240010,#240011,
#240012,#240013,#240014,#240015,#240016,#240017,#240018,#240019,#240020,
#240021,#240022,#240023,#240024,#240025,#240026,#240027,#240028,#240029,
#240030,#240031,#240032,#240033,#240034,#240035,#240036,#240037,#240038,
#240039,#240040,#240041,#240042,#240043,#240044,#240045,#240046,#240047,
#240048,#240049,#240050,#240051,#240052,#240053,#240054,#240055,#240056,
#240057,#240058,#240059,#240060,#240061,#240062,#240063,#240064,#240065,
#240066,#240067,#240068,#240069,#240070,#240071,#240072,#240073,#240074,
#240075,#240076,#240077,#240078,#240079,#240080,#240081,#240082,#240083,
#240084,#240085,#240086,#240087,#240088,#240089,#240090,#240091,#240092,
#240093,#240094,#240095,#240096,#240097,#240098,#240099,#240100,#240101,
#240102,#240103,#240104,#240105,#240106,#240107,#240108,#240109,#240110,
#240111,#240112,#240113,#240114,#240115,#240116,#240117,#240118,#240119,
#240120,#240121,#240122,#240123,#240124,#240125,#240126,#240127,#240128,
#240129,#240130,#240131,#240132,#240133,#240134,#240135,#240136,#240137,
#240138,#240139,#240140,#240141,#240142,#240143,#240144,#240145,#240146,
#240147,#240148,#240149,#240150,#240151,#240152,#240153,#240154,#240155,
#240156,#240157,#240158,#240159,#240160,#240161,#240162,#240163,#240164,
#240165,#240166,#240167,#240168,#240169,#240170,#240171,#240172,#240173,
#240174,#240175,#240176,#240177,#240178,#240179,#240180,#240181,#240182,
#240183,#240184,#240185,#240186,#240187,#240188,#240189,#240190,#240191,
#240192,#240193,#240194,#240195,#240196,#240197,#240198,#240199,#240200,
#240201,#240202,#240203,#240204,#240205,#240206,#240207,#240208,#240209,
#240210,#240211,#240212,#240213,#240214,#240215,#240216,#240217,#240218,
#240219,#240220,#240221,#240222,#240223,#240224,#240225,#240226,#240227,
#240228,#240229,#240230,#240231,#240232,#240233,#240234,#240235,#240236,
#240237,#240238,#240239,#240240,#240241,#240242,#240243,#240244,#240245,
#240246,#240247,#240248,#240249,#240250,#240251,#240252,#240253,#240254,
#240255,#240256,#240257,#240258,#240259,#240260,#240261,#240262,#240263,
#240264,#240265,#240266,#240267,#240268,#240269,#240270,#240271,#240272,
#240273,#240274,#240275,#240276,#240277,#240278,#240279,#240280,#240281,
#240282,#240283,#240284,#240285,#240286,#240287,#240288,#240289,#240290,
#240291,#240292,#240293,#240294,#240295,#240296,#240297,#240298,#240299,
#240300,#240301,#240302,#240303,#240304,#240305,#240306,#240307,#240308,
#240309,#240310,#240311,#240312,#240313,#240314,#240315,#240316,#240317,
#240318,#240319,#240320,#240321,#240322,#240323,#240324,#240325,#240326,
#240327,#240328,#240329,#240330,#240331,#240332,#240333,#240334,#240335,
#240336,#240337,#240338,#240339,#240340,#240341,#240342,#240343,#240344,
#240345,#240346,#240347,#240348,#240349,#240350,#240351,#240352,#240353,
#240354,#240355,#240356,#240357,#240358,#240359,#240360,#240361,#240362,
#240363,#240364,#240365,#240366,#240367,#240368,#240369,#240370,#240371,
#240372,#240373,#240374,#240375,#240376,#240377,#240378,#240379,#240380),
 .UNSPECIFIED.,.F.,.F.,(4,2,2,2,2,2,2,2,2,2,2,2,2,2,2,2,2,2,2,2,2,2,2,2,
2,2,2,2,2,2,2,2,2,2,2,2,2,2,2,2,2,2,2,2,2,2,2,2,2,2,2,2,2,2,2,2,2,2,2,2,
2,2,2,2,2,2,2,2,2,2,2,2,2,2,2,2,2,2,2,2,2,2,2,2,2,2,2,2,2,2,2,2,2,2,2,2,
2,2,2,2,2,2,2,2,2,2,2,2,2,2,2,2,2,2,2,2,2,2,2,2,2,2,2,2,2,2,2,2,2,2,2,2,
2,2,2,2,2,2,2,2,2,2,2,2,2,2,2,2,2,2,2,2,2,2,2,2,2,2,2,2,2,2,2,2,2,2,2,2,
2,2,2,2,2,2,2,2,2,2,2,2,2,2,2,2,2,2,2,2,2,2,2,2,2,2,2,2,2,2,2,2,2,2,2,2,
2,2,2,2,2,2,2,2,2,2,2,2,2,2,2,2,2,2,2,2,2,2,2,2,2,2,2,2,2,2,2,2,2,2,2,2,
2,2,2,2,2,2,2,2,2,2,2,2,2,2,2,2,2,2,2,2,2,2,2,2,2,2,2,4),(0.00169193791497629,
0.00269170506770563,0.00382150025259507,0.00497529633340349,0.00612871498677458,
0.00781404984112232,0.0127998102560316,0.0992952071431597,0.241006483008384,
0.322626394132003,0.377792672142896,0.392612611969002,0.396430301496517,
0.398680227178473,0.40066282537986,0.403129648395394,0.406921427368932,
0.423882088545111,0.720344176276257,0.761999575993357,0.786495003610549,
0.794610060402936,0.798187028584304,0.800148816717977,0.801850918525245,
0.802890651810846,0.804020129466061,0.805502025233649,0.808777036101699,
0.834874903823989,0.920904233879457,0.967500913020852,0.980912714031539,
0.996157536723248,1.01371285205981,1.03430642778889,1.05917268435567,1.1462898639267,
1.19419078706825,1.21892152272548,1.22353968531524,1.22602709661673,1.22807158792978,
1.2304798192881,1.23462312763094,1.25019882037846,1.50776471703766,1.61170323614546,
1.61806083577225,1.62063131590095,1.62244712727404,1.62408777752376,1.62653484005037,
1.63208333747967,1.69733399475308,1.71453434540894,1.77072893152393,1.82607377245994,
1.86883958206715,1.97233102078528,1.99209917900411,1.99861236331483,2.00275211594448,
2.00661155462139,2.01163740824028,2.02223697865391,2.11094795066746,2.2521701178907,
2.31149739673316,2.34706474246649,2.36436910993395,2.36773658355138,2.36956942002404,
2.37094074793797,2.37263899443585,2.37543340819382,2.38464280408234,2.52136993519002,
2.66382753941995,2.69168124697717,2.74567494986017,2.77453042838392,2.77964388032204,
2.78236530897271,2.7846064282369,2.78721020996672,2.79166387605688,2.80814413952905,
3.0723007112816,3.19249748446832,3.19770148117874,3.20012160946691,3.20192793370995,
3.20385213158838,3.20678705274988,3.21490666489957,3.26058563038,3.45696833731933,
3.60858174425896,3.62933295423243,3.6388758473337,3.64617743203437,3.6531596255548,
3.66512330126049,3.69907632554344,3.72244135797862,3.9207261316018,3.94939208378295,
3.95564501118944,3.95917706738549,3.96220477585861,3.96586978785082,3.97278949746997,
4.02143038678407,4.16594232237504,4.21793371071668,4.25046108114024,4.26061642479772,
4.26709636139357,4.27317011279584,4.28115037057796,4.29909527338847,4.42922029695093,
4.45532200989663,4.6151098573033,4.68561020734812,4.71496503238116,4.71969958685053,
4.72217437990107,4.72419011427012,4.72650766679617,4.73041406749951,4.7443145311256,
4.9817770008264,5.11136280130468,5.11975512578225,5.12277618835428,5.12488027268926,
5.12683269665446,5.12949280737777,5.13460835220472,5.166719266993,5.23760724695966,
5.43608360217353,5.51880128110111,5.54007577545144,5.54327138229398,5.54478268616827,
5.54596300416593,5.54724703090316,5.54930075443546,5.55626618434596,5.60059970139283,
5.71391934567529,5.76770393658139,5.83765198534363,5.86655691376328,5.92976267005913,
5.93596224009174,5.93848959361659,5.9403551204055,5.94237782829179,5.94512950614628,
5.95142129764205,6.06660831633939,6.21447673287528,6.33258252053735,6.33996131170891,
6.34208622879112,6.3432143380281,6.34421423220962,6.34550979973154,6.34779606258712,
6.35786515280854,6.50209947308295,6.63022997193524,6.68385855991787,6.75636680479173,
6.76300222428483,6.76566786760625,6.76762152277431,6.76972646836974,6.77256650816992,
6.77896061103927,6.90010161075822,7.04944354150552,7.11024052719992,7.13157422536459,
7.15503633824202,7.15895189951689,7.16128266915803,7.16306272759256,7.16495997673894,
7.16791350023821,7.17629680272853,7.22445722843781,7.27171794556602,7.38298996736577,
7.52272654605282,7.53492211562209,7.53984331999971,7.54344558705204,7.5470762183348,
7.55207062557926,7.56270376977997,7.57658146530835,7.6979480214644,7.89693516338263,
7.90608691397582,7.90892907885227,7.91047472319245,7.91185436953749,7.91365560717128,
7.91687678948814,7.93211474533385,7.96186624535493,7.98775288882021,8.11227883685769,
8.29696385425935,8.31608660193267,8.32037354804583,8.32316558670998,8.32541176434123,
8.32796330222301,8.33229917487821,8.34921812148471,8.47198196962048,8.57770487934709,
8.72604339770952,8.73626234349374,8.73955529783358,8.7413717060368,8.74300872228565,
8.74516883785471,8.74909927208373,8.76861747392223,8.84327724321625,8.8922336851052,
9.10085744071271,9.15955384252156,9.17374138775755,9.18206044321826,9.18921735449683,
9.19795299470797,9.21462684093077,9.23562578246183,9.2825854315289,9.37911520275485,
9.44521762658215,9.48781279647693,9.49448894292639,9.49847904204394,9.50154865086394,
9.50436835791005,9.50757441393806,9.51205835446919,9.55249840557096,9.66752902267458,
9.70622078553479,9.78400107516521,9.7965135759874,9.80418665527794,9.81021515008504,
9.81583977894261,9.82236785490708,9.83171345803354,9.86860524257916,9.96114864333145),
 .UNSPECIFIED.);
#3615=B_SPLINE_CURVE_WITH_KNOTS('',3,(#240382,#240383,#240384,#240385,#240386,
#240387,#240388,#240389,#240390,#240391,#240392,#240393,#240394,#240395,
#240396,#240397,#240398,#240399),.UNSPECIFIED.,.F.,.F.,(4,2,2,2,2,2,2,2,
4),(-54.3584128775674,-53.5234959656725,-52.6885790537777,-51.8536621418828,
-51.018745229988,-50.1838283180931,-49.3489114061983,-48.5139944943034,
-48.0752275703878),.UNSPECIFIED.);
#3616=B_SPLINE_CURVE_WITH_KNOTS('',3,(#240401,#240402,#240403,#240404,#240405,
#240406,#240407,#240408,#240409,#240410,#240411,#240412,#240413,#240414,
#240415,#240416,#240417,#240418,#240419,#240420,#240421,#240422,#240423,
#240424,#240425,#240426,#240427,#240428,#240429,#240430,#240431,#240432,
#240433,#240434,#240435,#240436,#240437,#240438,#240439,#240440,#240441,
#240442,#240443,#240444,#240445,#240446,#240447,#240448,#240449,#240450,
#240451,#240452,#240453,#240454,#240455,#240456,#240457,#240458,#240459,
#240460,#240461,#240462,#240463,#240464,#240465,#240466,#240467,#240468,
#240469,#240470,#240471,#240472,#240473,#240474,#240475,#240476,#240477,
#240478,#240479,#240480,#240481,#240482,#240483,#240484,#240485,#240486,
#240487,#240488,#240489,#240490,#240491,#240492,#240493,#240494,#240495,
#240496,#240497,#240498,#240499,#240500,#240501,#240502,#240503,#240504,
#240505,#240506,#240507,#240508,#240509,#240510,#240511,#240512,#240513,
#240514,#240515,#240516,#240517,#240518,#240519,#240520,#240521,#240522,
#240523,#240524,#240525,#240526,#240527,#240528,#240529,#240530,#240531,
#240532,#240533,#240534,#240535,#240536,#240537,#240538,#240539,#240540,
#240541,#240542,#240543,#240544,#240545,#240546,#240547,#240548,#240549,
#240550,#240551,#240552,#240553,#240554,#240555,#240556,#240557,#240558,
#240559,#240560,#240561,#240562,#240563,#240564,#240565,#240566,#240567,
#240568,#240569,#240570,#240571,#240572,#240573,#240574,#240575,#240576,
#240577,#240578,#240579,#240580,#240581,#240582,#240583,#240584,#240585,
#240586,#240587,#240588,#240589,#240590,#240591,#240592,#240593,#240594,
#240595,#240596,#240597,#240598,#240599,#240600,#240601,#240602,#240603,
#240604,#240605,#240606,#240607,#240608,#240609,#240610,#240611,#240612,
#240613,#240614,#240615,#240616,#240617,#240618,#240619,#240620,#240621,
#240622,#240623,#240624,#240625,#240626,#240627,#240628,#240629,#240630,
#240631,#240632,#240633,#240634,#240635,#240636,#240637,#240638,#240639,
#240640,#240641,#240642,#240643,#240644,#240645,#240646,#240647,#240648,
#240649,#240650,#240651,#240652,#240653,#240654,#240655,#240656,#240657,
#240658,#240659,#240660,#240661,#240662,#240663,#240664,#240665,#240666,
#240667,#240668,#240669,#240670,#240671,#240672,#240673,#240674,#240675,
#240676,#240677,#240678,#240679,#240680,#240681,#240682,#240683,#240684,
#240685,#240686,#240687,#240688,#240689,#240690,#240691,#240692,#240693,
#240694,#240695,#240696,#240697,#240698,#240699,#240700,#240701,#240702,
#240703,#240704,#240705,#240706,#240707,#240708,#240709,#240710,#240711,
#240712,#240713,#240714,#240715,#240716,#240717,#240718,#240719,#240720,
#240721,#240722,#240723,#240724,#240725,#240726,#240727,#240728,#240729,
#240730,#240731,#240732,#240733,#240734,#240735,#240736,#240737,#240738,
#240739,#240740,#240741,#240742,#240743,#240744,#240745,#240746,#240747,
#240748,#240749,#240750,#240751,#240752,#240753,#240754,#240755,#240756,
#240757,#240758,#240759,#240760,#240761,#240762,#240763,#240764,#240765,
#240766,#240767,#240768,#240769,#240770,#240771,#240772,#240773,#240774,
#240775,#240776,#240777,#240778,#240779,#240780,#240781,#240782,#240783,
#240784,#240785,#240786,#240787,#240788,#240789,#240790,#240791,#240792,
#240793,#240794,#240795,#240796,#240797,#240798,#240799,#240800,#240801,
#240802,#240803,#240804,#240805,#240806,#240807,#240808,#240809,#240810,
#240811,#240812,#240813,#240814,#240815,#240816,#240817,#240818,#240819,
#240820,#240821,#240822,#240823,#240824,#240825,#240826,#240827,#240828,
#240829,#240830,#240831,#240832,#240833,#240834,#240835,#240836,#240837,
#240838,#240839,#240840,#240841,#240842,#240843,#240844,#240845,#240846,
#240847,#240848,#240849,#240850,#240851,#240852,#240853,#240854,#240855,
#240856,#240857,#240858,#240859,#240860,#240861,#240862,#240863,#240864,
#240865,#240866,#240867,#240868,#240869,#240870,#240871,#240872,#240873,
#240874,#240875,#240876,#240877,#240878,#240879,#240880,#240881,#240882,
#240883,#240884,#240885,#240886,#240887,#240888,#240889,#240890,#240891,
#240892,#240893,#240894,#240895,#240896,#240897,#240898,#240899,#240900,
#240901,#240902,#240903,#240904,#240905,#240906,#240907,#240908,#240909,
#240910,#240911,#240912,#240913,#240914,#240915,#240916,#240917,#240918,
#240919,#240920,#240921,#240922,#240923,#240924,#240925,#240926,#240927,
#240928,#240929,#240930,#240931,#240932,#240933,#240934),.UNSPECIFIED.,
 .F.,.F.,(4,2,2,2,2,2,2,2,2,2,2,2,2,2,2,2,2,2,2,2,2,2,2,2,2,2,2,2,2,2,2,
2,2,2,2,2,2,2,2,2,2,2,2,2,2,2,2,2,2,2,2,2,2,2,2,2,2,2,2,2,2,2,2,2,2,2,2,
2,2,2,2,2,2,2,2,2,2,2,2,2,2,2,2,2,2,2,2,2,2,2,2,2,2,2,2,2,2,2,2,2,2,2,2,
2,2,2,2,2,2,2,2,2,2,2,2,2,2,2,2,2,2,2,2,2,2,2,2,2,2,2,2,2,2,2,2,2,2,2,2,
2,2,2,2,2,2,2,2,2,2,2,2,2,2,2,2,2,2,2,2,2,2,2,2,2,2,2,2,2,2,2,2,2,2,2,2,
2,2,2,2,2,2,2,2,2,2,2,2,2,2,2,2,2,2,2,2,2,2,2,2,2,2,2,2,2,2,2,2,2,2,2,2,
2,2,2,2,2,2,2,2,2,2,2,2,2,2,2,2,2,2,2,2,2,2,2,2,2,2,2,2,2,2,2,2,2,2,2,2,
2,2,2,2,2,2,2,2,2,2,2,2,2,2,2,2,2,2,2,4),(0.00146851476906278,0.0692655499922215,
0.089400024040553,0.0944724269859721,0.0979216631136692,0.10079614387533,
0.103826040131627,0.107544923500693,0.115003199896438,0.186094811208884,
0.224090798072318,0.247835106160534,0.308925425060645,0.385911850393577,
0.395396505367879,0.401983996719065,0.40758372284573,0.413584498335929,
0.421163537381088,0.43313302811207,0.511650111852883,0.533885271508265,
0.550653768842362,0.610088844507437,0.695342960668452,0.763872207393003,
0.828673286310461,0.846988381638754,0.858255087048304,0.860883916315355,
0.863343919807208,0.865358432888645,0.867383740437143,0.871096100778068,
0.882928927181664,1.00570375849612,1.0949202422572,1.10725360276171,1.12203587807812,
1.14024040144564,1.17665250669679,1.22959135477994,1.2574577685711,1.26238349373266,
1.26500332067486,1.26695109340906,1.26938195387707,1.27344676632077,1.28684307039591,
1.48953822268046,1.59429653067734,1.64722436496261,1.67001914779108,1.68193156982673,
1.68442587582703,1.68580788963179,1.68686010553232,1.68820667708916,1.69048067620084,
1.699007592445,1.83320636878154,1.91433248206823,2.00116412607974,2.04758138321328,
2.07327093689801,2.07779856366154,2.08020438118668,2.08199201583473,2.08393984632913,
2.08737273939037,2.09736311776734,2.25035853958936,2.34086219951431,2.42334381656648,
2.47124487084906,2.48045694180497,2.48264705455828,2.48391445301725,2.48502773023013,
2.48640815062321,2.48852180057692,2.49783469281014,2.64027236954451,2.78661456731993,
2.89790777159325,2.90405032128404,2.90684380022263,2.9089408203341,2.91090649083658,
2.91361889860019,2.9205288124644,3.00746342268466,3.08094752984613,3.21696487836916,
3.28628447779599,3.29366639353152,3.2992417040133,3.30167813007679,3.30346861096541,
3.30512016524016,3.30735819810807,3.3117302047703,3.34616255928018,3.48102229500202,
3.66470672226491,3.67616166560683,3.68133677937927,3.68520523450572,3.68882296825786,
3.69380834510445,3.70380937046665,3.80930176243178,3.95469563085087,4.01412049204915,
4.04445109559307,4.04833620637309,4.05027756287007,4.05167092904741,4.05314329642527,
4.05520855719195,4.05945341164996,4.11624426606879,4.35259196524155,4.45173974255662,
4.45942928899073,4.46264309909995,4.46495101407759,4.46704243310408,4.4698209430599,
4.47651653444533,4.53544696527002,4.58686524887046,4.78434186162305,4.81647525970919,
4.86725545082275,4.8767945511091,4.87987594964872,4.88184718000565,4.88369104798299,
4.88609800726606,4.89118138658488,4.93073369506005,4.93397829819044,4.9424219841965,
4.94746081248866,4.96182761578438,4.97931403108478,5.13232177972035,5.19767445793448,
5.29017099030379,5.30814170620958,5.31726645604533,5.32404357307894,5.33147412144347,
5.34181122439952,5.36705810810029,5.48654600837033,5.62010697718058,5.63243770025018,
5.63674947375852,5.63972184210742,5.64246037319347,5.64616461509851,5.65353944431,
5.65891213165663,5.75702947264751,5.81745184643111,5.8900276791472,5.92842317402104,
5.93963986723146,5.94635255651402,5.95175639700145,5.95908673606465,5.97320283754696,
6.08260894230299,6.18869458790093,6.33186130138922,6.39275686151867,6.39886911788521,
6.40158565431815,6.40363759916557,6.40580370646485,6.40913420829052,6.41903724095087,
6.58242591113428,6.64124548791066,6.78932858486455,6.79899146336551,6.80248121211969,
6.80476739780165,6.80690958549081,6.80971868068372,6.81575512173777,6.88803267113628,
6.94634842367095,7.15777823880518,7.21826760452027,7.22242266133639,7.2239985759794,
7.22512208375423,7.22618560398163,7.22766751009316,7.23063917424668,7.25778159710836,
7.3405378102815,7.42141909464429,7.60213831654654,7.61198270719985,7.61667453197753,
7.61911681233593,7.62106469069747,7.62292166189652,7.62620201937552,7.63597445512227,
7.68802905016287,7.74398652575734,7.86691034088456,7.99386296446121,8.01799387513124,
8.02083409728693,8.02225893514415,8.02330653245235,8.024442106603,8.0259859358551,
8.02951019481616,8.16114626072756,8.26532140583614,8.43049623128637,8.44129483081343,
8.44485577421308,8.44709601763168,8.44913169165893,8.45170803553229,8.45692585819034,
8.49696761798772,8.60010556517228,8.67224933983917,8.82674969048819,8.83676331148724,
8.83995907297507,8.8417143463864,8.84346735621258,8.84561833100048,8.84972792404426,
8.87483099212183,8.93025937475379,9.16046590934478,9.20700970330384,9.21578324258158,
9.22077446923018,9.22462722643471,9.22878029181728,9.2353563898159,9.25659352010707,
9.37988075886679,9.56244294581531,9.56877658684074,9.57689514520887,9.58298516814561,
9.5873987079952,9.5894219755417,9.59097540622986,9.59263928113368,9.59524623506897,
9.60335540458085,9.65004831824916,9.95823180089409),.UNSPECIFIED.);
#3617=B_SPLINE_CURVE_WITH_KNOTS('',3,(#240936,#240937,#240938,#240939,#240940,
#240941,#240942,#240943,#240944,#240945,#240946,#240947,#240948,#240949,
#240950,#240951,#240952,#240953),.UNSPECIFIED.,.F.,.F.,(4,2,2,2,2,2,2,2,
4),(-35.5088569560286,-34.6739400441337,-33.8390231322389,-33.004106220344,
-32.1691893084491,-31.3342723965543,-30.4993554846594,-29.6644385727646,
-29.225671648849),.UNSPECIFIED.);
#3618=B_SPLINE_CURVE_WITH_KNOTS('',3,(#240955,#240956,#240957,#240958,#240959,
#240960,#240961,#240962,#240963,#240964,#240965,#240966,#240967),
 .UNSPECIFIED.,.F.,.F.,(4,1,1,1,1,1,1,1,1,1,4),(-29.225671648849,-28.9634523400033,
-27.9647126041411,-27.46534273621,-26.9659728682789,-26.4666030003479,-25.9672331324168,
-24.9684933965546,-23.9697536606924,-22.9710139248302,-22.9424868718849),
 .UNSPECIFIED.);
#3619=B_SPLINE_CURVE_WITH_KNOTS('',3,(#240969,#240970,#240971,#240972,#240973,
#240974,#240975,#240976,#240977,#240978,#240979,#240980,#240981,#240982,
#240983,#240984,#240985,#240986,#240987,#240988,#240989,#240990,#240991,
#240992,#240993,#240994,#240995,#240996,#240997,#240998,#240999,#241000,
#241001,#241002,#241003,#241004,#241005,#241006,#241007,#241008,#241009,
#241010,#241011,#241012,#241013,#241014,#241015,#241016,#241017,#241018,
#241019,#241020,#241021,#241022,#241023,#241024,#241025,#241026,#241027,
#241028,#241029,#241030,#241031,#241032,#241033,#241034,#241035,#241036,
#241037,#241038,#241039,#241040,#241041,#241042,#241043,#241044,#241045,
#241046,#241047,#241048,#241049,#241050,#241051,#241052,#241053,#241054,
#241055,#241056,#241057,#241058,#241059,#241060,#241061,#241062,#241063,
#241064,#241065,#241066,#241067,#241068,#241069,#241070,#241071,#241072,
#241073,#241074,#241075,#241076,#241077,#241078,#241079,#241080,#241081,
#241082,#241083,#241084,#241085,#241086,#241087,#241088,#241089,#241090,
#241091,#241092,#241093,#241094,#241095,#241096,#241097,#241098,#241099,
#241100,#241101,#241102,#241103,#241104,#241105,#241106,#241107,#241108,
#241109,#241110,#241111,#241112,#241113,#241114,#241115,#241116,#241117,
#241118,#241119,#241120,#241121,#241122,#241123,#241124,#241125,#241126,
#241127,#241128,#241129,#241130,#241131,#241132,#241133,#241134,#241135,
#241136,#241137,#241138,#241139,#241140,#241141,#241142,#241143,#241144,
#241145,#241146,#241147,#241148,#241149,#241150,#241151,#241152,#241153,
#241154,#241155,#241156,#241157,#241158,#241159,#241160,#241161,#241162,
#241163,#241164,#241165,#241166,#241167,#241168,#241169,#241170,#241171,
#241172,#241173,#241174,#241175,#241176,#241177,#241178,#241179,#241180,
#241181,#241182,#241183,#241184,#241185,#241186,#241187,#241188,#241189,
#241190,#241191,#241192,#241193,#241194,#241195,#241196,#241197,#241198,
#241199,#241200,#241201,#241202,#241203,#241204,#241205,#241206,#241207,
#241208,#241209,#241210,#241211,#241212,#241213,#241214,#241215,#241216,
#241217,#241218,#241219,#241220,#241221,#241222,#241223,#241224),
 .UNSPECIFIED.,.F.,.F.,(4,3,3,3,3,3,3,3,3,3,3,3,3,3,3,3,3,3,3,3,3,3,3,3,
3,3,3,3,3,3,3,3,3,3,3,3,3,3,3,3,3,3,3,3,3,3,3,3,3,3,3,3,3,3,3,3,3,3,3,3,
3,3,3,3,3,3,3,3,3,3,3,3,3,3,3,3,3,3,3,3,3,3,3,3,3,4),(-22.9424863416694,
-22.8626944275539,-22.7830199127632,-22.7035200632596,-22.6241260056474,
-22.544893840185,-22.4716440568991,-22.3972397536512,-22.3228186828177,
-22.2483685713348,-22.1738365360289,-22.0992600957276,-22.0245791489254,
-21.972274188968,-21.8957026457029,-21.8191987531952,-21.7427515587079,
-21.6663501497856,-21.5899836469113,-21.5129274976856,-21.4365901077061,
-21.3602532365099,-21.2839070283929,-21.2063138845711,-21.1298947729273,
-21.0517146130165,-20.9735344531058,-20.8997573618599,-20.826042584007,
-20.752377049305,-20.6787469038082,-20.6051382795967,-20.5315254613912,
-20.4741645851747,-20.3927310551976,-20.311162061333,-20.2270702253107,
-20.1452275199713,-20.0600111186075,-19.9747947172437,-19.8963617729823,
-19.8179985883438,-19.7397003223178,-19.6614810557322,-19.5833117635119,
-19.5052004377325,-19.4754248493126,-19.3990623781506,-19.322683051983,
-19.2462772862505,-19.169802614058,-19.0932905662234,-19.0166962368841,
-18.9760549813815,-18.9006776035735,-18.8253617713139,-18.7500946628522,
-18.6748634889253,-18.5996554849425,-18.5218629550146,-18.4466447799998,
-18.3714099055896,-18.2961467632106,-18.2208437710307,-18.1454515762295,
-18.0700066780304,-17.994463318066,-17.9773152455193,-17.904171434713,-17.831116419771,
-17.7581352635524,-17.6852130990856,-17.6123351139755,-17.5394865363451,
-17.466639133535,-17.393788785599,-17.3209221437638,-17.2480258485698,-17.1750437068389,
-17.1020148043683,-17.0288752490888,-16.9785755096571,-16.884308028905,
-16.7907763237038,-16.6987671708473,-16.6593011630521),.UNSPECIFIED.);
#3620=B_SPLINE_CURVE_WITH_KNOTS('',3,(#241226,#241227,#241228,#241229,#241230,
#241231,#241232,#241233,#241234,#241235,#241236,#241237,#241238),
 .UNSPECIFIED.,.F.,.F.,(4,1,1,1,1,1,1,1,1,1,4),(-16.6593010344898,-15.9798357737949,
-15.4804659058638,-14.9810960379327,-13.9823563020706,-13.4829864341395,
-12.9836165662084,-12.4842466982773,-11.9848768303462,-10.986137094484,
-10.3761157273102),.UNSPECIFIED.);
#3621=B_SPLINE_CURVE_WITH_KNOTS('',3,(#241239,#241240,#241241,#241242,#241243,
#241244,#241245,#241246,#241247,#241248,#241249,#241250,#241251,#241252,
#241253,#241254,#241255,#241256,#241257,#241258,#241259,#241260,#241261,
#241262,#241263,#241264,#241265,#241266,#241267,#241268,#241269,#241270,
#241271,#241272,#241273,#241274,#241275,#241276,#241277,#241278,#241279,
#241280,#241281,#241282,#241283,#241284,#241285,#241286,#241287,#241288,
#241289,#241290,#241291,#241292,#241293,#241294,#241295,#241296,#241297,
#241298,#241299,#241300,#241301,#241302,#241303,#241304,#241305,#241306,
#241307,#241308,#241309,#241310,#241311,#241312,#241313,#241314,#241315,
#241316,#241317,#241318,#241319,#241320,#241321,#241322,#241323,#241324,
#241325,#241326,#241327,#241328,#241329,#241330,#241331,#241332,#241333,
#241334,#241335,#241336,#241337,#241338,#241339,#241340,#241341,#241342,
#241343,#241344,#241345,#241346,#241347,#241348,#241349,#241350,#241351,
#241352,#241353,#241354,#241355,#241356,#241357,#241358,#241359,#241360,
#241361,#241362,#241363,#241364,#241365,#241366,#241367,#241368,#241369,
#241370,#241371,#241372,#241373,#241374,#241375,#241376,#241377,#241378,
#241379,#241380,#241381,#241382,#241383,#241384,#241385,#241386,#241387,
#241388,#241389,#241390,#241391,#241392,#241393,#241394,#241395,#241396,
#241397,#241398,#241399,#241400,#241401,#241402,#241403,#241404,#241405,
#241406,#241407,#241408,#241409,#241410,#241411,#241412,#241413,#241414,
#241415,#241416,#241417,#241418,#241419,#241420,#241421,#241422,#241423,
#241424,#241425,#241426,#241427,#241428,#241429,#241430,#241431,#241432,
#241433,#241434,#241435,#241436,#241437,#241438,#241439,#241440,#241441,
#241442,#241443,#241444,#241445,#241446,#241447,#241448,#241449,#241450,
#241451,#241452,#241453,#241454,#241455,#241456,#241457,#241458,#241459,
#241460,#241461,#241462,#241463,#241464,#241465,#241466,#241467,#241468,
#241469,#241470,#241471,#241472,#241473,#241474,#241475,#241476,#241477,
#241478,#241479,#241480,#241481,#241482,#241483,#241484,#241485,#241486,
#241487,#241488,#241489,#241490,#241491,#241492,#241493,#241494,#241495,
#241496,#241497),.UNSPECIFIED.,.F.,.F.,(4,3,3,3,3,3,3,3,3,3,3,3,3,3,3,3,
3,3,3,3,3,3,3,3,3,3,3,3,3,3,3,3,3,3,3,3,3,3,3,3,3,3,3,3,3,3,3,3,3,3,3,3,
3,3,3,3,3,3,3,3,3,3,3,3,3,3,3,3,3,3,3,3,3,3,3,3,3,3,3,3,3,3,3,3,3,3,4),
(-10.3761155919908,-10.2949452678718,-10.2133195299643,-10.1314591778195,
-10.0492442106362,-9.98739735862183,-9.91280691640399,-9.83830212093258,
-9.76386903770048,-9.68949377967818,-9.61516249815242,-9.54086137401722,
-9.46656620911823,-9.3922708644428,-9.3179628479057,-9.24362966306445,-9.16922387076276,
-9.09477648114597,-9.02023821787867,-8.98865762275964,-8.90768234806484,
-8.82682378339225,-8.74243977625133,-8.66189879816705,-8.58148114198779,
-8.50123776391101,-8.48928775482855,-8.41486188710567,-8.34041906846526,
-8.26594704683611,-8.19139293979972,-8.11679432384346,-8.0420911626425,
-7.98991788689746,-7.91335494065555,-7.83685968219422,-7.76042114153417,
-7.68402838897576,-7.60767052774935,-7.53060898066009,-7.45428011123147,
-7.37795169077802,-7.30161384817896,-7.22400492389304,-7.14759387543904,
-7.06938601323716,-6.99117815103528,-6.91742310966251,-6.84373039576828,
-6.77008692443867,-6.6964787878574,-6.62289214969108,-6.54930120466727,
-6.49180828310419,-6.41019566437374,-6.32844180433781,-6.24444095704664,
-6.16240671975315,-6.07742256746312,-5.9924384151731,-5.91439691633121,
-5.8364239239298,-5.75851331313484,-5.6806752626253,-5.60288259323826,-5.5251391570527,
-5.49306854724201,-5.41619341909099,-5.3392952721306,-5.26236564969255,
-5.1853627112488,-5.10832015885976,-5.03119535881957,-4.99369867931092,
-4.91974063918843,-4.84584806684379,-4.77200666060005,-4.69820215528429,
-4.6225431926378,-4.54875584762045,-4.47496019497449,-4.40114335197271,
-4.32409012750761,-4.25015428000783,-4.17616787206064,-4.10208725131818,
-4.09293045411233),.UNSPECIFIED.);
#3622=B_SPLINE_CURVE_WITH_KNOTS('',3,(#241500,#241501,#241502,#241503,#241504,
#241505,#241506,#241507,#241508,#241509,#241510,#241511,#241512,#241513,
#241514,#241515,#241516,#241517,#241518,#241519,#241520,#241521,#241522,
#241523,#241524,#241525,#241526,#241527,#241528,#241529,#241530,#241531,
#241532,#241533,#241534,#241535,#241536,#241537,#241538,#241539,#241540,
#241541,#241542,#241543,#241544,#241545,#241546,#241547,#241548,#241549,
#241550,#241551,#241552,#241553,#241554,#241555,#241556,#241557,#241558,
#241559,#241560,#241561,#241562,#241563,#241564,#241565,#241566,#241567,
#241568,#241569,#241570,#241571,#241572,#241573,#241574,#241575),
 .UNSPECIFIED.,.F.,.F.,(4,3,3,3,3,3,3,3,3,3,3,3,3,3,3,3,3,3,3,3,3,3,3,3,
3,4),(415.785312438574,415.867774042332,415.950234980212,416.03269527961,
416.115154967923,416.197614072545,416.280072620868,416.362530640282,416.444988158175,
416.531665331254,416.614132116863,416.696597229994,416.779060780301,416.861522877415,
416.943983630947,417.026443150489,417.108901545616,417.191358925887,417.273825311706,
417.35628851333,417.438748969279,417.521207117915,417.603672721927,417.686132600504,
417.768596712241,417.831822927442),.UNSPECIFIED.);
#3623=B_SPLINE_CURVE_WITH_KNOTS('',3,(#241577,#241578,#241579,#241580,#241581,
#241582,#241583,#241584,#241585,#241586,#241587,#241588,#241589,#241590,
#241591,#241592,#241593,#241594,#241595,#241596,#241597,#241598,#241599,
#241600,#241601,#241602,#241603,#241604,#241605,#241606,#241607,#241608,
#241609,#241610,#241611,#241612,#241613,#241614,#241615,#241616,#241617,
#241618,#241619,#241620,#241621,#241622,#241623,#241624,#241625,#241626,
#241627,#241628,#241629,#241630,#241631,#241632,#241633,#241634,#241635,
#241636,#241637,#241638,#241639,#241640,#241641,#241642,#241643,#241644,
#241645,#241646,#241647,#241648,#241649,#241650,#241651,#241652,#241653,
#241654,#241655,#241656,#241657,#241658,#241659,#241660,#241661,#241662,
#241663,#241664),.UNSPECIFIED.,.F.,.F.,(4,3,3,3,3,3,3,3,3,3,3,3,3,3,3,3,
3,3,3,3,3,3,3,3,3,3,3,3,3,4),(417.831822927442,417.936862277953,418.045946800198,
418.102105343728,418.177999062294,418.25379634993,418.329514096796,418.405169105709,
418.480778112549,418.558286483429,418.633868479123,418.709457603604,418.785068942452,
418.864012976737,418.939757279917,419.015558616832,419.091467379743,419.10084507959,
419.178871624819,419.256804913119,419.334660133074,419.412452418422,419.490194251559,
419.567908427544,419.645608569675,419.72330829071,419.801050685512,419.878814189843,
419.956654054945,420.022062012856),.UNSPECIFIED.);
#3624=B_SPLINE_CURVE_WITH_KNOTS('',3,(#241668,#241669,#241670,#241671,#241672,
#241673,#241674,#241675,#241676,#241677,#241678,#241679,#241680,#241681,
#241682,#241683,#241684,#241685,#241686,#241687,#241688,#241689,#241690,
#241691,#241692,#241693,#241694,#241695,#241696,#241697,#241698,#241699,
#241700,#241701,#241702,#241703,#241704),.UNSPECIFIED.,.F.,.F.,(4,3,3,3,
3,3,3,3,3,3,3,3,4),(417.832158352677,417.908872951564,417.985549119717,
418.062212442549,418.138866002223,418.215550066432,418.283790826053,418.368525197013,
418.453296162334,418.538099097117,418.622896862441,418.707669660275,418.783160693984),
 .UNSPECIFIED.);
#3625=B_SPLINE_CURVE_WITH_KNOTS('',3,(#241705,#241706,#241707,#241708,#241709,
#241710,#241711,#241712,#241713,#241714,#241715,#241716,#241717,#241718,
#241719,#241720,#241721,#241722,#241723,#241724,#241725,#241726,#241727,
#241728,#241729,#241730,#241731,#241732,#241733,#241734,#241735,#241736,
#241737,#241738,#241739,#241740,#241741,#241742,#241743,#241744,#241745,
#241746,#241747,#241748,#241749,#241750,#241751,#241752,#241753,#241754,
#241755,#241756,#241757,#241758,#241759,#241760,#241761,#241762,#241763,
#241764,#241765,#241766,#241767,#241768,#241769,#241770,#241771,#241772,
#241773,#241774,#241775,#241776,#241777,#241778,#241779,#241780),
 .UNSPECIFIED.,.F.,.F.,(4,3,3,3,3,3,3,3,3,3,3,3,3,3,3,3,3,3,3,3,3,3,3,3,
3,4),(415.785312438575,415.867774042333,415.950234980212,416.03269527961,
416.115154967923,416.197614072545,416.280072620869,416.362530640283,416.444988158176,
416.531665331255,416.614132116864,416.696597229995,416.779060780302,416.861522877416,
416.943983630948,417.02644315049,417.108901545617,417.191358925888,417.273825311707,
417.356288513331,417.43874896928,417.521207117916,417.603672721928,417.686132600505,
417.768596712242,417.831822927443),.UNSPECIFIED.);
#3626=B_SPLINE_CURVE_WITH_KNOTS('',3,(#241784,#241785,#241786,#241787,#241788,
#241789,#241790,#241791,#241792,#241793),.UNSPECIFIED.,.F.,.F.,(4,2,2,2,
4),(0.911640176190889,0.987592569311299,1.06354496243171,1.13953259867645,
1.21552023492119),.UNSPECIFIED.);
#3627=B_SPLINE_CURVE_WITH_KNOTS('',3,(#241795,#241796,#241797,#241798,#241799,
#241800,#241801,#241802,#241803,#241804,#241805,#241806,#241807,#241808,
#241809,#241810,#241811,#241812),.UNSPECIFIED.,.F.,.F.,(4,2,2,2,2,2,2,2,
4),(0.303880058730296,0.379832451850707,0.455784844971118,0.531772481215855,
0.607760117460592,0.68374775370533,0.759735389950067,0.835687783070478,
0.911640176190889),.UNSPECIFIED.);
#3628=B_SPLINE_CURVE_WITH_KNOTS('',3,(#241813,#241814,#241815,#241816,#241817,
#241818,#241819,#241820,#241821,#241822),.UNSPECIFIED.,.F.,.F.,(4,2,2,2,
4),(1.21552023492119,1.29150787116592,1.36749550741066,1.44344790053107,
1.51940029365148),.UNSPECIFIED.);
#3629=B_SPLINE_CURVE_WITH_KNOTS('',3,(#241826,#241827,#241828,#241829,#241830,
#241831,#241832,#241833,#241834,#241835),.UNSPECIFIED.,.F.,.F.,(4,2,2,2,
4),(0.911640176190889,0.9875925693113,1.06354496243171,1.13953259867645,
1.21552023492119),.UNSPECIFIED.);
#3630=B_SPLINE_CURVE_WITH_KNOTS('',3,(#241837,#241838,#241839,#241840,#241841,
#241842,#241843,#241844,#241845,#241846,#241847,#241848,#241849,#241850,
#241851,#241852,#241853,#241854),.UNSPECIFIED.,.F.,.F.,(4,2,2,2,2,2,2,2,
4),(0.303880058730296,0.379832451850707,0.455784844971118,0.531772481215856,
0.607760117460593,0.68374775370533,0.759735389950067,0.835687783070478,
0.911640176190889),.UNSPECIFIED.);
#3631=B_SPLINE_CURVE_WITH_KNOTS('',3,(#241855,#241856,#241857,#241858,#241859,
#241860,#241861,#241862,#241863,#241864),.UNSPECIFIED.,.F.,.F.,(4,2,2,2,
4),(1.21552023492119,1.29150787116592,1.36749550741066,1.44344790053107,
1.51940029365148),.UNSPECIFIED.);
#3632=B_SPLINE_CURVE_WITH_KNOTS('',3,(#244221,#244222,#244223,#244224,#244225,
#244226,#244227,#244228,#244229,#244230,#244231,#244232,#244233,#244234,
#244235,#244236,#244237,#244238,#244239,#244240,#244241,#244242,#244243,
#244244,#244245,#244246,#244247,#244248,#244249,#244250,#244251,#244252,
#244253,#244254,#244255,#244256,#244257,#244258,#244259,#244260,#244261,
#244262,#244263,#244264,#244265,#244266,#244267,#244268,#244269,#244270,
#244271,#244272,#244273,#244274,#244275,#244276,#244277,#244278,#244279,
#244280,#244281,#244282,#244283,#244284,#244285,#244286,#244287,#244288,
#244289,#244290,#244291,#244292,#244293,#244294,#244295,#244296,#244297,
#244298,#244299,#244300,#244301,#244302,#244303,#244304,#244305,#244306,
#244307,#244308,#244309,#244310,#244311,#244312,#244313,#244314,#244315,
#244316,#244317,#244318,#244319,#244320,#244321,#244322,#244323,#244324,
#244325,#244326,#244327,#244328,#244329,#244330,#244331,#244332),
 .UNSPECIFIED.,.F.,.F.,(4,3,3,3,3,3,3,3,3,3,3,3,3,3,3,3,3,3,3,3,3,3,3,3,
3,3,3,3,3,3,3,3,3,3,3,3,3,4),(0.,0.0614070448361033,0.123000388029202,0.185032164943811,
0.246804846791042,0.29762099995536,0.305065160573997,0.365696235832332,
0.426395934638525,0.449954325750456,0.510788416315891,0.571039794968828,
0.588887633948557,0.599629016443718,0.607143367867252,0.666657656805943,
0.725941079523381,0.784345238663423,0.825028657709657,0.870198948105793,
0.888116253859817,0.894842574301577,0.952699129950469,1.01087631965265,
1.06867337830243,1.12531084762339,1.15700566255158,1.16650423523313,1.1732896249373,
1.18639098087874,1.24342851224962,1.30047172399187,1.34989027008284,1.35816107472823,
1.41436027386202,1.46989172561496,1.52521609801738,1.53373699248706),
 .UNSPECIFIED.);
#3633=B_SPLINE_CURVE_WITH_KNOTS('',3,(#244333,#244334,#244335,#244336,#244337,
#244338,#244339,#244340,#244341,#244342,#244343,#244344,#244345,#244346,
#244347,#244348,#244349,#244350,#244351,#244352,#244353,#244354,#244355,
#244356,#244357,#244358,#244359,#244360,#244361,#244362,#244363,#244364,
#244365,#244366,#244367,#244368,#244369,#244370,#244371,#244372,#244373,
#244374,#244375,#244376,#244377,#244378,#244379,#244380,#244381,#244382,
#244383,#244384,#244385,#244386,#244387,#244388,#244389,#244390,#244391,
#244392,#244393,#244394,#244395,#244396,#244397,#244398,#244399,#244400,
#244401,#244402,#244403,#244404,#244405,#244406,#244407,#244408,#244409,
#244410,#244411,#244412,#244413,#244414,#244415,#244416,#244417,#244418,
#244419,#244420,#244421,#244422,#244423,#244424,#244425,#244426,#244427,
#244428,#244429,#244430,#244431,#244432,#244433,#244434,#244435,#244436,
#244437,#244438,#244439,#244440,#244441),.UNSPECIFIED.,.F.,.F.,(4,3,3,3,
3,3,3,3,3,3,3,3,3,3,3,3,3,3,3,3,3,3,3,3,3,3,3,3,3,3,3,3,3,3,3,3,4),(-1.53373699248736,
-1.48074492111914,-1.42597430957864,-1.38913925044945,-1.35382340313308,
-1.34128955619904,-1.284953556331,-1.22801001408438,-1.17965192531475,-1.16822998829084,
-1.15948917603948,-1.13129383654512,-1.07393261892752,-1.01569915500957,
-0.957333826688686,-0.899346117127988,-0.88926600173786,-0.882672214977545,
-0.823092924494319,-0.767660588719696,-0.7089616547114,-0.649590264476471,
-0.604729941843312,-0.595476697221127,-0.535516633819567,-0.474961154894728,
-0.414241537401714,-0.390466188696484,-0.329920792589955,-0.320304295415085,
-0.310066000769442,-0.297802242924248,-0.237064747296051,-0.175222188325058,
-0.113179732983841,-0.0515754651466952,0.),.UNSPECIFIED.);
#3634=B_SPLINE_CURVE_WITH_KNOTS('',3,(#246798,#246799,#246800,#246801,#246802,
#246803,#246804,#246805,#246806,#246807,#246808,#246809,#246810,#246811,
#246812,#246813,#246814,#246815,#246816,#246817,#246818,#246819,#246820,
#246821,#246822,#246823,#246824,#246825,#246826,#246827,#246828,#246829,
#246830,#246831,#246832,#246833,#246834,#246835,#246836,#246837,#246838,
#246839,#246840,#246841,#246842,#246843,#246844,#246845,#246846,#246847,
#246848,#246849,#246850,#246851,#246852,#246853,#246854,#246855,#246856,
#246857,#246858,#246859,#246860,#246861,#246862,#246863,#246864,#246865,
#246866,#246867,#246868,#246869,#246870,#246871,#246872,#246873,#246874,
#246875,#246876,#246877,#246878,#246879,#246880,#246881,#246882,#246883,
#246884,#246885,#246886,#246887,#246888,#246889,#246890,#246891,#246892,
#246893,#246894,#246895,#246896,#246897,#246898,#246899,#246900,#246901,
#246902,#246903,#246904,#246905,#246906,#246907,#246908,#246909),
 .UNSPECIFIED.,.F.,.F.,(4,3,3,3,3,3,3,3,3,3,3,3,3,3,3,3,3,3,3,3,3,3,3,3,
3,3,3,3,3,3,3,3,3,3,3,3,3,4),(0.,0.0528697059263613,0.107325934667311,0.162613932174076,
0.218756404443508,0.264210921238665,0.272319408785509,0.329151478442084,
0.385983548098659,0.401883732982838,0.459384745316969,0.517029025796296,
0.532644921841707,0.541940475471059,0.54873148511669,0.607427868628937,
0.666405972188839,0.72513755497834,0.764359179612553,0.822926923794845,
0.826792889734822,0.83378661030972,0.892090379582624,0.951786196051419,
1.01185326841918,1.07167856199159,1.10858072873138,1.11899067792923,1.12650652923598,
1.1400296903362,1.20015177784907,1.26114459016009,1.31842175654699,1.32779114489853,
1.38958900979801,1.45163430952323,1.51340906521101,1.52870610664523),
 .UNSPECIFIED.);
#3635=B_SPLINE_CURVE_WITH_KNOTS('',3,(#246910,#246911,#246912,#246913,#246914,
#246915,#246916,#246917,#246918,#246919,#246920,#246921,#246922,#246923,
#246924,#246925,#246926,#246927,#246928,#246929,#246930,#246931,#246932,
#246933,#246934,#246935,#246936,#246937,#246938,#246939,#246940,#246941,
#246942,#246943,#246944,#246945,#246946,#246947,#246948,#246949,#246950,
#246951,#246952,#246953,#246954,#246955,#246956,#246957,#246958,#246959,
#246960,#246961,#246962,#246963,#246964,#246965,#246966,#246967,#246968,
#246969,#246970,#246971,#246972,#246973,#246974,#246975,#246976,#246977,
#246978,#246979,#246980,#246981,#246982,#246983,#246984,#246985,#246986,
#246987,#246988,#246989,#246990,#246991,#246992,#246993,#246994,#246995,
#246996,#246997,#246998,#246999,#247000,#247001,#247002,#247003,#247004,
#247005,#247006,#247007,#247008,#247009,#247010,#247011,#247012,#247013,
#247014,#247015,#247016,#247017,#247018,#247019,#247020,#247021),
 .UNSPECIFIED.,.F.,.F.,(4,3,3,3,3,3,3,3,3,3,3,3,3,3,3,3,3,3,3,3,3,3,3,3,
3,3,3,3,3,3,3,3,3,3,3,3,3,4),(-1.52870610664522,-1.46751956777301,-1.4056757019945,
-1.34361550157725,-1.33048902574182,-1.32126641659285,-1.28497700231689,
-1.22375459820483,-1.16284546373868,-1.14061554159086,-1.12299841173653,
-1.11207164330468,-1.08095498548466,-1.02082441436179,-0.960638340272262,
-0.900842120772938,-0.852426264160289,-0.833346966102961,-0.821061892466914,
-0.762469470452377,-0.707178694322342,-0.648327099083374,-0.589945955835236,
-0.547705085953817,-0.537342986300492,-0.479826857793964,-0.422459929680001,
-0.365926586536747,-0.346773440319137,-0.303426760279258,-0.283727392684925,
-0.271794967690972,-0.261530163865359,-0.205492049525167,-0.149273616827515,
-0.0934113811589646,-0.0385977154833653,-1.01138585612593E-13),
 .UNSPECIFIED.);
#4374=LINE('',#185304,#5011);
#4375=LINE('',#185526,#5012);
#4376=LINE('',#186025,#5013);
#4377=LINE('',#186521,#5014);
#4378=LINE('',#187032,#5015);
#4379=LINE('',#187540,#5016);
#4380=LINE('',#188033,#5017);
#4381=LINE('',#188535,#5018);
#4382=LINE('',#189028,#5019);
#4383=LINE('',#189530,#5020);
#4384=LINE('',#190041,#5021);
#4385=LINE('',#190552,#5022);
#4386=LINE('',#191051,#5023);
#4387=LINE('',#191553,#5024);
#4388=LINE('',#192058,#5025);
#4389=LINE('',#192566,#5026);
#4390=LINE('',#193068,#5027);
#4391=LINE('',#193558,#5028);
#4392=LINE('',#194045,#5029);
#4393=LINE('',#194547,#5030);
#4394=LINE('',#195055,#5031);
#4395=LINE('',#195569,#5032);
#4396=LINE('',#196062,#5033);
#4397=LINE('',#196558,#5034);
#4398=LINE('',#197063,#5035);
#4399=LINE('',#197574,#5036);
#4400=LINE('',#198073,#5037);
#4401=LINE('',#198560,#5038);
#4402=LINE('',#199065,#5039);
#4403=LINE('',#199576,#5040);
#4404=LINE('',#200087,#5041);
#4405=LINE('',#200586,#5042);
#4406=LINE('',#201085,#5043);
#4407=LINE('',#201578,#5044);
#4408=LINE('',#202053,#5045);
#4409=LINE('',#202537,#5046);
#4410=LINE('',#203033,#5047);
#4411=LINE('',#203532,#5048);
#4412=LINE('',#204037,#5049);
#4413=LINE('',#204536,#5050);
#4414=LINE('',#205029,#5051);
#4415=LINE('',#205519,#5052);
#4416=LINE('',#206018,#5053);
#4417=LINE('',#206520,#5054);
#4418=LINE('',#207022,#5055);
#4419=LINE('',#207518,#5056);
#4420=LINE('',#208008,#5057);
#4421=LINE('',#208510,#5058);
#4422=LINE('',#209003,#5059);
#4423=LINE('',#209493,#5060);
#4424=LINE('',#209983,#5061);
#4425=LINE('',#210470,#5062);
#4426=LINE('',#210813,#5063);
#4427=LINE('',#211230,#5064);
#4428=LINE('',#211735,#5065);
#4429=LINE('',#212234,#5066);
#4430=LINE('',#212733,#5067);
#4431=LINE('',#213241,#5068);
#4432=LINE('',#213737,#5069);
#4433=LINE('',#214230,#5070);
#4434=LINE('',#214708,#5071);
#4435=LINE('',#215192,#5072);
#4436=LINE('',#215694,#5073);
#4437=LINE('',#216202,#5074);
#4438=LINE('',#216698,#5075);
#4439=LINE('',#241824,#5076);
#4440=LINE('',#247031,#5077);
#4441=LINE('',#247033,#5078);
#4442=LINE('',#247035,#5079);
#5011=VECTOR('',#19402,6.767);
#5012=VECTOR('',#19407,6.767);
#5013=VECTOR('',#19410,6.767);
#5014=VECTOR('',#19413,6.767);
#5015=VECTOR('',#19416,6.767);
#5016=VECTOR('',#19419,6.767);
#5017=VECTOR('',#19422,6.767);
#5018=VECTOR('',#19425,6.767);
#5019=VECTOR('',#19428,6.767);
#5020=VECTOR('',#19431,6.767);
#5021=VECTOR('',#19434,6.767);
#5022=VECTOR('',#19437,6.767);
#5023=VECTOR('',#19440,6.767);
#5024=VECTOR('',#19443,6.767);
#5025=VECTOR('',#19446,6.767);
#5026=VECTOR('',#19449,6.767);
#5027=VECTOR('',#19452,6.767);
#5028=VECTOR('',#19455,6.767);
#5029=VECTOR('',#19458,6.767);
#5030=VECTOR('',#19461,6.767);
#5031=VECTOR('',#19464,6.767);
#5032=VECTOR('',#19467,6.767);
#5033=VECTOR('',#19470,6.767);
#5034=VECTOR('',#19473,6.767);
#5035=VECTOR('',#19476,6.767);
#5036=VECTOR('',#19479,6.767);
#5037=VECTOR('',#19482,6.767);
#5038=VECTOR('',#19485,6.767);
#5039=VECTOR('',#19488,6.767);
#5040=VECTOR('',#19491,6.767);
#5041=VECTOR('',#19494,6.767);
#5042=VECTOR('',#19497,6.767);
#5043=VECTOR('',#19500,6.767);
#5044=VECTOR('',#19503,6.767);
#5045=VECTOR('',#19506,6.767);
#5046=VECTOR('',#19509,6.767);
#5047=VECTOR('',#19512,6.767);
#5048=VECTOR('',#19515,6.767);
#5049=VECTOR('',#19518,6.767);
#5050=VECTOR('',#19521,6.767);
#5051=VECTOR('',#19524,6.767);
#5052=VECTOR('',#19527,6.767);
#5053=VECTOR('',#19530,6.767);
#5054=VECTOR('',#19533,6.767);
#5055=VECTOR('',#19536,6.767);
#5056=VECTOR('',#19539,6.767);
#5057=VECTOR('',#19542,6.767);
#5058=VECTOR('',#19545,6.767);
#5059=VECTOR('',#19548,6.767);
#5060=VECTOR('',#19551,6.767);
#5061=VECTOR('',#19554,6.767);
#5062=VECTOR('',#19557,6.767);
#5063=VECTOR('',#19560,6.767);
#5064=VECTOR('',#19563,6.767);
#5065=VECTOR('',#19566,6.767);
#5066=VECTOR('',#19569,6.767);
#5067=VECTOR('',#19572,6.767);
#5068=VECTOR('',#19575,6.767);
#5069=VECTOR('',#19578,6.767);
#5070=VECTOR('',#19581,6.767);
#5071=VECTOR('',#19584,6.767);
#5072=VECTOR('',#19587,6.767);
#5073=VECTOR('',#19590,6.767);
#5074=VECTOR('',#19593,6.767);
#5075=VECTOR('',#19596,6.767);
#5076=VECTOR('',#19609,2.);
#5077=VECTOR('',#19622,10.);
#5078=VECTOR('',#19625,6.);
#5079=VECTOR('',#19626,6.);
#6622=VERTEX_POINT('',#185302);
#6623=VERTEX_POINT('',#185303);
#6624=VERTEX_POINT('',#185305);
#6625=VERTEX_POINT('',#185439);
#6626=VERTEX_POINT('',#185524);
#6627=VERTEX_POINT('',#185525);
#6628=VERTEX_POINT('',#185527);
#6629=VERTEX_POINT('',#185767);
#6630=VERTEX_POINT('',#186023);
#6631=VERTEX_POINT('',#186024);
#6632=VERTEX_POINT('',#186026);
#6633=VERTEX_POINT('',#186272);
#6634=VERTEX_POINT('',#186519);
#6635=VERTEX_POINT('',#186520);
#6636=VERTEX_POINT('',#186522);
#6637=VERTEX_POINT('',#186777);
#6638=VERTEX_POINT('',#187030);
#6639=VERTEX_POINT('',#187031);
#6640=VERTEX_POINT('',#187033);
#6641=VERTEX_POINT('',#187282);
#6642=VERTEX_POINT('',#187538);
#6643=VERTEX_POINT('',#187539);
#6644=VERTEX_POINT('',#187541);
#6645=VERTEX_POINT('',#187790);
#6646=VERTEX_POINT('',#188031);
#6647=VERTEX_POINT('',#188032);
#6648=VERTEX_POINT('',#188034);
#6649=VERTEX_POINT('',#188286);
#6650=VERTEX_POINT('',#188533);
#6651=VERTEX_POINT('',#188534);
#6652=VERTEX_POINT('',#188536);
#6653=VERTEX_POINT('',#188785);
#6654=VERTEX_POINT('',#189026);
#6655=VERTEX_POINT('',#189027);
#6656=VERTEX_POINT('',#189029);
#6657=VERTEX_POINT('',#189281);
#6658=VERTEX_POINT('',#189528);
#6659=VERTEX_POINT('',#189529);
#6660=VERTEX_POINT('',#189531);
#6661=VERTEX_POINT('',#189786);
#6662=VERTEX_POINT('',#190039);
#6663=VERTEX_POINT('',#190040);
#6664=VERTEX_POINT('',#190042);
#6665=VERTEX_POINT('',#190297);
#6666=VERTEX_POINT('',#190550);
#6667=VERTEX_POINT('',#190551);
#6668=VERTEX_POINT('',#190553);
#6669=VERTEX_POINT('',#190790);
#6670=VERTEX_POINT('',#191049);
#6671=VERTEX_POINT('',#191050);
#6672=VERTEX_POINT('',#191052);
#6673=VERTEX_POINT('',#191298);
#6674=VERTEX_POINT('',#191551);
#6675=VERTEX_POINT('',#191552);
#6676=VERTEX_POINT('',#191554);
#6677=VERTEX_POINT('',#191803);
#6678=VERTEX_POINT('',#192056);
#6679=VERTEX_POINT('',#192057);
#6680=VERTEX_POINT('',#192059);
#6681=VERTEX_POINT('',#192308);
#6682=VERTEX_POINT('',#192564);
#6683=VERTEX_POINT('',#192565);
#6684=VERTEX_POINT('',#192567);
#6685=VERTEX_POINT('',#192810);
#6686=VERTEX_POINT('',#193066);
#6687=VERTEX_POINT('',#193067);
#6688=VERTEX_POINT('',#193069);
#6689=VERTEX_POINT('',#193315);
#6690=VERTEX_POINT('',#193556);
#6691=VERTEX_POINT('',#193557);
#6692=VERTEX_POINT('',#193559);
#6693=VERTEX_POINT('',#193808);
#6694=VERTEX_POINT('',#194043);
#6695=VERTEX_POINT('',#194044);
#6696=VERTEX_POINT('',#194046);
#6697=VERTEX_POINT('',#194298);
#6698=VERTEX_POINT('',#194545);
#6699=VERTEX_POINT('',#194546);
#6700=VERTEX_POINT('',#194548);
#6701=VERTEX_POINT('',#194800);
#6702=VERTEX_POINT('',#195053);
#6703=VERTEX_POINT('',#195054);
#6704=VERTEX_POINT('',#195056);
#6705=VERTEX_POINT('',#195311);
#6706=VERTEX_POINT('',#195567);
#6707=VERTEX_POINT('',#195568);
#6708=VERTEX_POINT('',#195570);
#6709=VERTEX_POINT('',#195807);
#6710=VERTEX_POINT('',#196060);
#6711=VERTEX_POINT('',#196061);
#6712=VERTEX_POINT('',#196063);
#6713=VERTEX_POINT('',#196306);
#6714=VERTEX_POINT('',#196556);
#6715=VERTEX_POINT('',#196557);
#6716=VERTEX_POINT('',#196559);
#6717=VERTEX_POINT('',#196808);
#6718=VERTEX_POINT('',#197061);
#6719=VERTEX_POINT('',#197062);
#6720=VERTEX_POINT('',#197064);
#6721=VERTEX_POINT('',#197316);
#6722=VERTEX_POINT('',#197572);
#6723=VERTEX_POINT('',#197573);
#6724=VERTEX_POINT('',#197575);
#6725=VERTEX_POINT('',#197818);
#6726=VERTEX_POINT('',#198071);
#6727=VERTEX_POINT('',#198072);
#6728=VERTEX_POINT('',#198074);
#6729=VERTEX_POINT('',#198317);
#6730=VERTEX_POINT('',#198558);
#6731=VERTEX_POINT('',#198559);
#6732=VERTEX_POINT('',#198561);
#6733=VERTEX_POINT('',#198816);
#6734=VERTEX_POINT('',#199063);
#6735=VERTEX_POINT('',#199064);
#6736=VERTEX_POINT('',#199066);
#6737=VERTEX_POINT('',#199318);
#6738=VERTEX_POINT('',#199574);
#6739=VERTEX_POINT('',#199575);
#6740=VERTEX_POINT('',#199577);
#6741=VERTEX_POINT('',#199832);
#6742=VERTEX_POINT('',#200085);
#6743=VERTEX_POINT('',#200086);
#6744=VERTEX_POINT('',#200088);
#6745=VERTEX_POINT('',#200328);
#6746=VERTEX_POINT('',#200584);
#6747=VERTEX_POINT('',#200585);
#6748=VERTEX_POINT('',#200587);
#6749=VERTEX_POINT('',#200833);
#6750=VERTEX_POINT('',#201083);
#6751=VERTEX_POINT('',#201084);
#6752=VERTEX_POINT('',#201086);
#6753=VERTEX_POINT('',#201326);
#6754=VERTEX_POINT('',#201576);
#6755=VERTEX_POINT('',#201577);
#6756=VERTEX_POINT('',#201579);
#6757=VERTEX_POINT('',#201813);
#6758=VERTEX_POINT('',#202051);
#6759=VERTEX_POINT('',#202052);
#6760=VERTEX_POINT('',#202054);
#6761=VERTEX_POINT('',#202288);
#6762=VERTEX_POINT('',#202535);
#6763=VERTEX_POINT('',#202536);
#6764=VERTEX_POINT('',#202538);
#6765=VERTEX_POINT('',#202772);
#6766=VERTEX_POINT('',#203031);
#6767=VERTEX_POINT('',#203032);
#6768=VERTEX_POINT('',#203034);
#6769=VERTEX_POINT('',#203277);
#6770=VERTEX_POINT('',#203530);
#6771=VERTEX_POINT('',#203531);
#6772=VERTEX_POINT('',#203533);
#6773=VERTEX_POINT('',#203785);
#6774=VERTEX_POINT('',#204035);
#6775=VERTEX_POINT('',#204036);
#6776=VERTEX_POINT('',#204038);
#6777=VERTEX_POINT('',#204290);
#6778=VERTEX_POINT('',#204534);
#6779=VERTEX_POINT('',#204535);
#6780=VERTEX_POINT('',#204537);
#6781=VERTEX_POINT('',#204777);
#6782=VERTEX_POINT('',#205027);
#6783=VERTEX_POINT('',#205028);
#6784=VERTEX_POINT('',#205030);
#6785=VERTEX_POINT('',#205276);
#6786=VERTEX_POINT('',#205517);
#6787=VERTEX_POINT('',#205518);
#6788=VERTEX_POINT('',#205520);
#6789=VERTEX_POINT('',#205772);
#6790=VERTEX_POINT('',#206016);
#6791=VERTEX_POINT('',#206017);
#6792=VERTEX_POINT('',#206019);
#6793=VERTEX_POINT('',#206259);
#6794=VERTEX_POINT('',#206518);
#6795=VERTEX_POINT('',#206519);
#6796=VERTEX_POINT('',#206521);
#6797=VERTEX_POINT('',#206767);
#6798=VERTEX_POINT('',#207020);
#6799=VERTEX_POINT('',#207021);
#6800=VERTEX_POINT('',#207023);
#6801=VERTEX_POINT('',#207263);
#6802=VERTEX_POINT('',#207516);
#6803=VERTEX_POINT('',#207517);
#6804=VERTEX_POINT('',#207519);
#6805=VERTEX_POINT('',#207753);
#6806=VERTEX_POINT('',#208006);
#6807=VERTEX_POINT('',#208007);
#6808=VERTEX_POINT('',#208009);
#6809=VERTEX_POINT('',#208255);
#6810=VERTEX_POINT('',#208508);
#6811=VERTEX_POINT('',#208509);
#6812=VERTEX_POINT('',#208511);
#6813=VERTEX_POINT('',#208763);
#6814=VERTEX_POINT('',#209001);
#6815=VERTEX_POINT('',#209002);
#6816=VERTEX_POINT('',#209004);
#6817=VERTEX_POINT('',#209256);
#6818=VERTEX_POINT('',#209491);
#6819=VERTEX_POINT('',#209492);
#6820=VERTEX_POINT('',#209494);
#6821=VERTEX_POINT('',#209734);
#6822=VERTEX_POINT('',#209981);
#6823=VERTEX_POINT('',#209982);
#6824=VERTEX_POINT('',#209984);
#6825=VERTEX_POINT('',#210230);
#6826=VERTEX_POINT('',#210468);
#6827=VERTEX_POINT('',#210469);
#6828=VERTEX_POINT('',#210471);
#6829=VERTEX_POINT('',#210723);
#6830=VERTEX_POINT('',#210811);
#6831=VERTEX_POINT('',#210812);
#6832=VERTEX_POINT('',#210814);
#6833=VERTEX_POINT('',#211051);
#6834=VERTEX_POINT('',#211228);
#6835=VERTEX_POINT('',#211229);
#6836=VERTEX_POINT('',#211231);
#6837=VERTEX_POINT('',#211480);
#6838=VERTEX_POINT('',#211733);
#6839=VERTEX_POINT('',#211734);
#6840=VERTEX_POINT('',#211736);
#6841=VERTEX_POINT('',#211976);
#6842=VERTEX_POINT('',#212232);
#6843=VERTEX_POINT('',#212233);
#6844=VERTEX_POINT('',#212235);
#6845=VERTEX_POINT('',#212478);
#6846=VERTEX_POINT('',#212731);
#6847=VERTEX_POINT('',#212732);
#6848=VERTEX_POINT('',#212734);
#6849=VERTEX_POINT('',#212986);
#6850=VERTEX_POINT('',#213239);
#6851=VERTEX_POINT('',#213240);
#6852=VERTEX_POINT('',#213242);
#6853=VERTEX_POINT('',#213497);
#6854=VERTEX_POINT('',#213735);
#6855=VERTEX_POINT('',#213736);
#6856=VERTEX_POINT('',#213738);
#6857=VERTEX_POINT('',#213993);
#6858=VERTEX_POINT('',#214228);
#6859=VERTEX_POINT('',#214229);
#6860=VERTEX_POINT('',#214231);
#6861=VERTEX_POINT('',#214471);
#6862=VERTEX_POINT('',#214706);
#6863=VERTEX_POINT('',#214707);
#6864=VERTEX_POINT('',#214709);
#6865=VERTEX_POINT('',#214955);
#6866=VERTEX_POINT('',#215190);
#6867=VERTEX_POINT('',#215191);
#6868=VERTEX_POINT('',#215193);
#6869=VERTEX_POINT('',#215445);
#6870=VERTEX_POINT('',#215692);
#6871=VERTEX_POINT('',#215693);
#6872=VERTEX_POINT('',#215695);
#6873=VERTEX_POINT('',#215944);
#6874=VERTEX_POINT('',#216200);
#6875=VERTEX_POINT('',#216201);
#6876=VERTEX_POINT('',#216203);
#6877=VERTEX_POINT('',#216443);
#6878=VERTEX_POINT('',#216696);
#6879=VERTEX_POINT('',#216697);
#6880=VERTEX_POINT('',#216699);
#6881=VERTEX_POINT('',#216933);
#6882=VERTEX_POINT('',#217177);
#6883=VERTEX_POINT('',#217178);
#6884=VERTEX_POINT('',#217187);
#6885=VERTEX_POINT('',#217189);
#6886=VERTEX_POINT('',#217530);
#6887=VERTEX_POINT('',#217549);
#6888=VERTEX_POINT('',#217562);
#6889=VERTEX_POINT('',#218121);
#6890=VERTEX_POINT('',#218662);
#6891=VERTEX_POINT('',#219193);
#6892=VERTEX_POINT('',#219453);
#6893=VERTEX_POINT('',#219467);
#6894=VERTEX_POINT('',#219486);
#6895=VERTEX_POINT('',#219749);
#6896=VERTEX_POINT('',#219763);
#6897=VERTEX_POINT('',#220020);
#6898=VERTEX_POINT('',#220559);
#6899=VERTEX_POINT('',#220573);
#6900=VERTEX_POINT('',#220836);
#6901=VERTEX_POINT('',#220849);
#6902=VERTEX_POINT('',#221390);
#6903=VERTEX_POINT('',#222005);
#6904=VERTEX_POINT('',#222019);
#6905=VERTEX_POINT('',#222038);
#6906=VERTEX_POINT('',#222052);
#6907=VERTEX_POINT('',#222315);
#6908=VERTEX_POINT('',#222329);
#6909=VERTEX_POINT('',#222592);
#6910=VERTEX_POINT('',#223135);
#6911=VERTEX_POINT('',#223154);
#6912=VERTEX_POINT('',#223665);
#6913=VERTEX_POINT('',#223684);
#6914=VERTEX_POINT('',#224223);
#6915=VERTEX_POINT('',#224483);
#6916=VERTEX_POINT('',#225018);
#6917=VERTEX_POINT('',#225031);
#6918=VERTEX_POINT('',#225560);
#6919=VERTEX_POINT('',#226085);
#6920=VERTEX_POINT('',#226620);
#6921=VERTEX_POINT('',#226880);
#6922=VERTEX_POINT('',#226899);
#6923=VERTEX_POINT('',#226913);
#6924=VERTEX_POINT('',#226928);
#6925=VERTEX_POINT('',#227453);
#6926=VERTEX_POINT('',#227472);
#6927=VERTEX_POINT('',#227735);
#6928=VERTEX_POINT('',#227749);
#6929=VERTEX_POINT('',#228012);
#6930=VERTEX_POINT('',#228026);
#6931=VERTEX_POINT('',#228045);
#6932=VERTEX_POINT('',#228578);
#6933=VERTEX_POINT('',#228591);
#6934=VERTEX_POINT('',#229072);
#6935=VERTEX_POINT('',#229074);
#6936=VERTEX_POINT('',#229247);
#6937=VERTEX_POINT('',#229266);
#6938=VERTEX_POINT('',#229791);
#6939=VERTEX_POINT('',#230051);
#6940=VERTEX_POINT('',#230588);
#6941=VERTEX_POINT('',#231103);
#6942=VERTEX_POINT('',#231360);
#6943=VERTEX_POINT('',#231871);
#6944=VERTEX_POINT('',#232436);
#6945=VERTEX_POINT('',#232696);
#6946=VERTEX_POINT('',#233199);
#6947=VERTEX_POINT('',#233730);
#6948=VERTEX_POINT('',#234271);
#6949=VERTEX_POINT('',#234878);
#6950=VERTEX_POINT('',#235135);
#6951=VERTEX_POINT('',#235150);
#6952=VERTEX_POINT('',#235169);
#6953=VERTEX_POINT('',#235188);
#6954=VERTEX_POINT('',#235207);
#6955=VERTEX_POINT('',#235226);
#6956=VERTEX_POINT('',#235755);
#6957=VERTEX_POINT('',#235769);
#6958=VERTEX_POINT('',#235788);
#6959=VERTEX_POINT('',#235802);
#6960=VERTEX_POINT('',#236315);
#6961=VERTEX_POINT('',#236852);
#6962=VERTEX_POINT('',#236865);
#6963=VERTEX_POINT('',#236884);
#6964=VERTEX_POINT('',#237147);
#6965=VERTEX_POINT('',#237162);
#6966=VERTEX_POINT('',#237176);
#6967=VERTEX_POINT('',#237705);
#6968=VERTEX_POINT('',#238228);
#6969=VERTEX_POINT('',#238241);
#6970=VERTEX_POINT('',#238774);
#6971=VERTEX_POINT('',#239037);
#6972=VERTEX_POINT('',#239570);
#6973=VERTEX_POINT('',#239830);
#6974=VERTEX_POINT('',#239844);
#6975=VERTEX_POINT('',#240381);
#6976=VERTEX_POINT('',#240400);
#6977=VERTEX_POINT('',#240935);
#6978=VERTEX_POINT('',#240954);
#6979=VERTEX_POINT('',#240968);
#6980=VERTEX_POINT('',#241225);
#6981=VERTEX_POINT('',#241499);
#6982=VERTEX_POINT('',#241576);
#6983=VERTEX_POINT('',#241665);
#6984=VERTEX_POINT('',#241667);
#6985=VERTEX_POINT('',#241782);
#6986=VERTEX_POINT('',#241783);
#6987=VERTEX_POINT('',#241794);
#6988=VERTEX_POINT('',#241823);
#6989=VERTEX_POINT('',#241825);
#6990=VERTEX_POINT('',#241836);
#6991=VERTEX_POINT('',#247024);
#6992=VERTEX_POINT('',#247026);
#6993=VERTEX_POINT('',#247029);
#6994=VERTEX_POINT('',#247034);
#9211=EDGE_CURVE('',#6622,#6623,#4374,.T.);
#9212=EDGE_CURVE('',#6624,#6622,#3267,.T.);
#9213=EDGE_CURVE('',#6625,#6624,#1917,.T.);
#9214=EDGE_CURVE('',#6625,#6623,#3268,.T.);
#9215=EDGE_CURVE('',#6626,#6627,#4375,.T.);
#9216=EDGE_CURVE('',#6628,#6626,#3269,.T.);
#9217=EDGE_CURVE('',#6622,#6628,#3270,.T.);
#9218=EDGE_CURVE('',#6623,#6629,#3271,.T.);
#9219=EDGE_CURVE('',#6629,#6627,#3272,.T.);
#9220=EDGE_CURVE('',#6630,#6631,#4376,.T.);
#9221=EDGE_CURVE('',#6632,#6630,#3273,.T.);
#9222=EDGE_CURVE('',#6626,#6632,#3274,.T.);
#9223=EDGE_CURVE('',#6627,#6633,#3275,.T.);
#9224=EDGE_CURVE('',#6633,#6631,#3276,.T.);
#9225=EDGE_CURVE('',#6634,#6635,#4377,.T.);
#9226=EDGE_CURVE('',#6636,#6634,#3277,.T.);
#9227=EDGE_CURVE('',#6630,#6636,#3278,.T.);
#9228=EDGE_CURVE('',#6631,#6637,#3279,.T.);
#9229=EDGE_CURVE('',#6637,#6635,#3280,.T.);
#9230=EDGE_CURVE('',#6638,#6639,#4378,.T.);
#9231=EDGE_CURVE('',#6640,#6638,#3281,.T.);
#9232=EDGE_CURVE('',#6634,#6640,#3282,.T.);
#9233=EDGE_CURVE('',#6635,#6641,#3283,.T.);
#9234=EDGE_CURVE('',#6641,#6639,#3284,.T.);
#9235=EDGE_CURVE('',#6642,#6643,#4379,.T.);
#9236=EDGE_CURVE('',#6644,#6642,#3285,.T.);
#9237=EDGE_CURVE('',#6638,#6644,#3286,.T.);
#9238=EDGE_CURVE('',#6639,#6645,#3287,.T.);
#9239=EDGE_CURVE('',#6645,#6643,#3288,.T.);
#9240=EDGE_CURVE('',#6646,#6647,#4380,.T.);
#9241=EDGE_CURVE('',#6648,#6646,#3289,.T.);
#9242=EDGE_CURVE('',#6642,#6648,#3290,.T.);
#9243=EDGE_CURVE('',#6643,#6649,#3291,.T.);
#9244=EDGE_CURVE('',#6649,#6647,#3292,.T.);
#9245=EDGE_CURVE('',#6650,#6651,#4381,.T.);
#9246=EDGE_CURVE('',#6652,#6650,#3293,.T.);
#9247=EDGE_CURVE('',#6646,#6652,#3294,.T.);
#9248=EDGE_CURVE('',#6647,#6653,#3295,.T.);
#9249=EDGE_CURVE('',#6653,#6651,#3296,.T.);
#9250=EDGE_CURVE('',#6654,#6655,#4382,.T.);
#9251=EDGE_CURVE('',#6656,#6654,#3297,.T.);
#9252=EDGE_CURVE('',#6650,#6656,#3298,.T.);
#9253=EDGE_CURVE('',#6651,#6657,#3299,.T.);
#9254=EDGE_CURVE('',#6657,#6655,#3300,.T.);
#9255=EDGE_CURVE('',#6658,#6659,#4383,.T.);
#9256=EDGE_CURVE('',#6660,#6658,#3301,.T.);
#9257=EDGE_CURVE('',#6654,#6660,#3302,.T.);
#9258=EDGE_CURVE('',#6655,#6661,#3303,.T.);
#9259=EDGE_CURVE('',#6661,#6659,#3304,.T.);
#9260=EDGE_CURVE('',#6662,#6663,#4384,.T.);
#9261=EDGE_CURVE('',#6664,#6662,#3305,.T.);
#9262=EDGE_CURVE('',#6658,#6664,#3306,.T.);
#9263=EDGE_CURVE('',#6659,#6665,#3307,.T.);
#9264=EDGE_CURVE('',#6665,#6663,#3308,.T.);
#9265=EDGE_CURVE('',#6666,#6667,#4385,.T.);
#9266=EDGE_CURVE('',#6668,#6666,#3309,.T.);
#9267=EDGE_CURVE('',#6662,#6668,#3310,.T.);
#9268=EDGE_CURVE('',#6663,#6669,#3311,.T.);
#9269=EDGE_CURVE('',#6669,#6667,#3312,.T.);
#9270=EDGE_CURVE('',#6670,#6671,#4386,.T.);
#9271=EDGE_CURVE('',#6672,#6670,#3313,.T.);
#9272=EDGE_CURVE('',#6666,#6672,#3314,.T.);
#9273=EDGE_CURVE('',#6667,#6673,#3315,.T.);
#9274=EDGE_CURVE('',#6673,#6671,#3316,.T.);
#9275=EDGE_CURVE('',#6674,#6675,#4387,.T.);
#9276=EDGE_CURVE('',#6676,#6674,#3317,.T.);
#9277=EDGE_CURVE('',#6670,#6676,#3318,.T.);
#9278=EDGE_CURVE('',#6671,#6677,#3319,.T.);
#9279=EDGE_CURVE('',#6677,#6675,#3320,.T.);
#9280=EDGE_CURVE('',#6678,#6679,#4388,.T.);
#9281=EDGE_CURVE('',#6680,#6678,#3321,.T.);
#9282=EDGE_CURVE('',#6674,#6680,#3322,.T.);
#9283=EDGE_CURVE('',#6675,#6681,#3323,.T.);
#9284=EDGE_CURVE('',#6681,#6679,#3324,.T.);
#9285=EDGE_CURVE('',#6682,#6683,#4389,.T.);
#9286=EDGE_CURVE('',#6684,#6682,#3325,.T.);
#9287=EDGE_CURVE('',#6678,#6684,#3326,.T.);
#9288=EDGE_CURVE('',#6679,#6685,#3327,.T.);
#9289=EDGE_CURVE('',#6685,#6683,#3328,.T.);
#9290=EDGE_CURVE('',#6686,#6687,#4390,.T.);
#9291=EDGE_CURVE('',#6688,#6686,#3329,.T.);
#9292=EDGE_CURVE('',#6682,#6688,#3330,.T.);
#9293=EDGE_CURVE('',#6683,#6689,#3331,.T.);
#9294=EDGE_CURVE('',#6689,#6687,#3332,.T.);
#9295=EDGE_CURVE('',#6690,#6691,#4391,.T.);
#9296=EDGE_CURVE('',#6692,#6690,#3333,.T.);
#9297=EDGE_CURVE('',#6686,#6692,#3334,.T.);
#9298=EDGE_CURVE('',#6687,#6693,#3335,.T.);
#9299=EDGE_CURVE('',#6693,#6691,#3336,.T.);
#9300=EDGE_CURVE('',#6694,#6695,#4392,.T.);
#9301=EDGE_CURVE('',#6696,#6694,#3337,.T.);
#9302=EDGE_CURVE('',#6690,#6696,#3338,.T.);
#9303=EDGE_CURVE('',#6691,#6697,#3339,.T.);
#9304=EDGE_CURVE('',#6697,#6695,#3340,.T.);
#9305=EDGE_CURVE('',#6698,#6699,#4393,.T.);
#9306=EDGE_CURVE('',#6700,#6698,#3341,.T.);
#9307=EDGE_CURVE('',#6694,#6700,#3342,.T.);
#9308=EDGE_CURVE('',#6695,#6701,#3343,.T.);
#9309=EDGE_CURVE('',#6701,#6699,#3344,.T.);
#9310=EDGE_CURVE('',#6702,#6703,#4394,.T.);
#9311=EDGE_CURVE('',#6704,#6702,#3345,.T.);
#9312=EDGE_CURVE('',#6698,#6704,#3346,.T.);
#9313=EDGE_CURVE('',#6699,#6705,#3347,.T.);
#9314=EDGE_CURVE('',#6705,#6703,#3348,.T.);
#9315=EDGE_CURVE('',#6706,#6707,#4395,.T.);
#9316=EDGE_CURVE('',#6708,#6706,#3349,.T.);
#9317=EDGE_CURVE('',#6702,#6708,#3350,.T.);
#9318=EDGE_CURVE('',#6703,#6709,#3351,.T.);
#9319=EDGE_CURVE('',#6709,#6707,#3352,.T.);
#9320=EDGE_CURVE('',#6710,#6711,#4396,.T.);
#9321=EDGE_CURVE('',#6712,#6710,#3353,.T.);
#9322=EDGE_CURVE('',#6706,#6712,#3354,.T.);
#9323=EDGE_CURVE('',#6707,#6713,#3355,.T.);
#9324=EDGE_CURVE('',#6713,#6711,#3356,.T.);
#9325=EDGE_CURVE('',#6714,#6715,#4397,.T.);
#9326=EDGE_CURVE('',#6716,#6714,#3357,.T.);
#9327=EDGE_CURVE('',#6710,#6716,#3358,.T.);
#9328=EDGE_CURVE('',#6711,#6717,#3359,.T.);
#9329=EDGE_CURVE('',#6717,#6715,#3360,.T.);
#9330=EDGE_CURVE('',#6718,#6719,#4398,.T.);
#9331=EDGE_CURVE('',#6720,#6718,#3361,.T.);
#9332=EDGE_CURVE('',#6714,#6720,#3362,.T.);
#9333=EDGE_CURVE('',#6715,#6721,#3363,.T.);
#9334=EDGE_CURVE('',#6721,#6719,#3364,.T.);
#9335=EDGE_CURVE('',#6722,#6723,#4399,.T.);
#9336=EDGE_CURVE('',#6724,#6722,#3365,.T.);
#9337=EDGE_CURVE('',#6718,#6724,#3366,.T.);
#9338=EDGE_CURVE('',#6719,#6725,#3367,.T.);
#9339=EDGE_CURVE('',#6725,#6723,#3368,.T.);
#9340=EDGE_CURVE('',#6726,#6727,#4400,.T.);
#9341=EDGE_CURVE('',#6728,#6726,#3369,.T.);
#9342=EDGE_CURVE('',#6722,#6728,#3370,.T.);
#9343=EDGE_CURVE('',#6723,#6729,#3371,.T.);
#9344=EDGE_CURVE('',#6729,#6727,#3372,.T.);
#9345=EDGE_CURVE('',#6730,#6731,#4401,.T.);
#9346=EDGE_CURVE('',#6732,#6730,#3373,.T.);
#9347=EDGE_CURVE('',#6726,#6732,#3374,.T.);
#9348=EDGE_CURVE('',#6727,#6733,#3375,.T.);
#9349=EDGE_CURVE('',#6733,#6731,#3376,.T.);
#9350=EDGE_CURVE('',#6734,#6735,#4402,.T.);
#9351=EDGE_CURVE('',#6736,#6734,#3377,.T.);
#9352=EDGE_CURVE('',#6730,#6736,#3378,.T.);
#9353=EDGE_CURVE('',#6731,#6737,#3379,.T.);
#9354=EDGE_CURVE('',#6737,#6735,#3380,.T.);
#9355=EDGE_CURVE('',#6738,#6739,#4403,.T.);
#9356=EDGE_CURVE('',#6740,#6738,#3381,.T.);
#9357=EDGE_CURVE('',#6734,#6740,#3382,.T.);
#9358=EDGE_CURVE('',#6735,#6741,#3383,.T.);
#9359=EDGE_CURVE('',#6741,#6739,#3384,.T.);
#9360=EDGE_CURVE('',#6742,#6743,#4404,.T.);
#9361=EDGE_CURVE('',#6744,#6742,#3385,.T.);
#9362=EDGE_CURVE('',#6738,#6744,#3386,.T.);
#9363=EDGE_CURVE('',#6739,#6745,#3387,.T.);
#9364=EDGE_CURVE('',#6745,#6743,#3388,.T.);
#9365=EDGE_CURVE('',#6746,#6747,#4405,.T.);
#9366=EDGE_CURVE('',#6748,#6746,#3389,.T.);
#9367=EDGE_CURVE('',#6742,#6748,#3390,.T.);
#9368=EDGE_CURVE('',#6743,#6749,#3391,.T.);
#9369=EDGE_CURVE('',#6749,#6747,#3392,.T.);
#9370=EDGE_CURVE('',#6750,#6751,#4406,.T.);
#9371=EDGE_CURVE('',#6752,#6750,#3393,.T.);
#9372=EDGE_CURVE('',#6746,#6752,#3394,.T.);
#9373=EDGE_CURVE('',#6747,#6753,#3395,.T.);
#9374=EDGE_CURVE('',#6753,#6751,#3396,.T.);
#9375=EDGE_CURVE('',#6754,#6755,#4407,.T.);
#9376=EDGE_CURVE('',#6756,#6754,#3397,.T.);
#9377=EDGE_CURVE('',#6750,#6756,#3398,.T.);
#9378=EDGE_CURVE('',#6751,#6757,#3399,.T.);
#9379=EDGE_CURVE('',#6757,#6755,#3400,.T.);
#9380=EDGE_CURVE('',#6758,#6759,#4408,.T.);
#9381=EDGE_CURVE('',#6760,#6758,#3401,.T.);
#9382=EDGE_CURVE('',#6754,#6760,#3402,.T.);
#9383=EDGE_CURVE('',#6755,#6761,#3403,.T.);
#9384=EDGE_CURVE('',#6761,#6759,#3404,.T.);
#9385=EDGE_CURVE('',#6762,#6763,#4409,.T.);
#9386=EDGE_CURVE('',#6764,#6762,#3405,.T.);
#9387=EDGE_CURVE('',#6758,#6764,#3406,.T.);
#9388=EDGE_CURVE('',#6759,#6765,#3407,.T.);
#9389=EDGE_CURVE('',#6765,#6763,#3408,.T.);
#9390=EDGE_CURVE('',#6766,#6767,#4410,.T.);
#9391=EDGE_CURVE('',#6768,#6766,#3409,.T.);
#9392=EDGE_CURVE('',#6762,#6768,#3410,.T.);
#9393=EDGE_CURVE('',#6763,#6769,#3411,.T.);
#9394=EDGE_CURVE('',#6769,#6767,#3412,.T.);
#9395=EDGE_CURVE('',#6770,#6771,#4411,.T.);
#9396=EDGE_CURVE('',#6772,#6770,#3413,.T.);
#9397=EDGE_CURVE('',#6766,#6772,#3414,.T.);
#9398=EDGE_CURVE('',#6767,#6773,#3415,.T.);
#9399=EDGE_CURVE('',#6773,#6771,#3416,.T.);
#9400=EDGE_CURVE('',#6774,#6775,#4412,.T.);
#9401=EDGE_CURVE('',#6776,#6774,#3417,.T.);
#9402=EDGE_CURVE('',#6770,#6776,#3418,.T.);
#9403=EDGE_CURVE('',#6771,#6777,#3419,.T.);
#9404=EDGE_CURVE('',#6777,#6775,#3420,.T.);
#9405=EDGE_CURVE('',#6778,#6779,#4413,.T.);
#9406=EDGE_CURVE('',#6780,#6778,#3421,.T.);
#9407=EDGE_CURVE('',#6774,#6780,#3422,.T.);
#9408=EDGE_CURVE('',#6775,#6781,#3423,.T.);
#9409=EDGE_CURVE('',#6781,#6779,#3424,.T.);
#9410=EDGE_CURVE('',#6782,#6783,#4414,.T.);
#9411=EDGE_CURVE('',#6784,#6782,#3425,.T.);
#9412=EDGE_CURVE('',#6778,#6784,#3426,.T.);
#9413=EDGE_CURVE('',#6779,#6785,#3427,.T.);
#9414=EDGE_CURVE('',#6785,#6783,#3428,.T.);
#9415=EDGE_CURVE('',#6786,#6787,#4415,.T.);
#9416=EDGE_CURVE('',#6788,#6786,#3429,.T.);
#9417=EDGE_CURVE('',#6782,#6788,#3430,.T.);
#9418=EDGE_CURVE('',#6783,#6789,#3431,.T.);
#9419=EDGE_CURVE('',#6789,#6787,#3432,.T.);
#9420=EDGE_CURVE('',#6790,#6791,#4416,.T.);
#9421=EDGE_CURVE('',#6792,#6790,#3433,.T.);
#9422=EDGE_CURVE('',#6786,#6792,#3434,.T.);
#9423=EDGE_CURVE('',#6787,#6793,#3435,.T.);
#9424=EDGE_CURVE('',#6793,#6791,#3436,.T.);
#9425=EDGE_CURVE('',#6794,#6795,#4417,.T.);
#9426=EDGE_CURVE('',#6796,#6794,#3437,.T.);
#9427=EDGE_CURVE('',#6790,#6796,#3438,.T.);
#9428=EDGE_CURVE('',#6791,#6797,#3439,.T.);
#9429=EDGE_CURVE('',#6797,#6795,#3440,.T.);
#9430=EDGE_CURVE('',#6798,#6799,#4418,.T.);
#9431=EDGE_CURVE('',#6800,#6798,#3441,.T.);
#9432=EDGE_CURVE('',#6794,#6800,#3442,.T.);
#9433=EDGE_CURVE('',#6795,#6801,#3443,.T.);
#9434=EDGE_CURVE('',#6801,#6799,#3444,.T.);
#9435=EDGE_CURVE('',#6802,#6803,#4419,.T.);
#9436=EDGE_CURVE('',#6804,#6802,#3445,.T.);
#9437=EDGE_CURVE('',#6798,#6804,#3446,.T.);
#9438=EDGE_CURVE('',#6799,#6805,#3447,.T.);
#9439=EDGE_CURVE('',#6805,#6803,#3448,.T.);
#9440=EDGE_CURVE('',#6806,#6807,#4420,.T.);
#9441=EDGE_CURVE('',#6808,#6806,#3449,.T.);
#9442=EDGE_CURVE('',#6802,#6808,#3450,.T.);
#9443=EDGE_CURVE('',#6803,#6809,#3451,.T.);
#9444=EDGE_CURVE('',#6809,#6807,#3452,.T.);
#9445=EDGE_CURVE('',#6810,#6811,#4421,.T.);
#9446=EDGE_CURVE('',#6812,#6810,#3453,.T.);
#9447=EDGE_CURVE('',#6806,#6812,#3454,.T.);
#9448=EDGE_CURVE('',#6807,#6813,#3455,.T.);
#9449=EDGE_CURVE('',#6813,#6811,#3456,.T.);
#9450=EDGE_CURVE('',#6814,#6815,#4422,.T.);
#9451=EDGE_CURVE('',#6816,#6814,#3457,.T.);
#9452=EDGE_CURVE('',#6810,#6816,#3458,.T.);
#9453=EDGE_CURVE('',#6811,#6817,#3459,.T.);
#9454=EDGE_CURVE('',#6817,#6815,#3460,.T.);
#9455=EDGE_CURVE('',#6818,#6819,#4423,.T.);
#9456=EDGE_CURVE('',#6820,#6818,#3461,.T.);
#9457=EDGE_CURVE('',#6814,#6820,#3462,.T.);
#9458=EDGE_CURVE('',#6815,#6821,#3463,.T.);
#9459=EDGE_CURVE('',#6821,#6819,#3464,.T.);
#9460=EDGE_CURVE('',#6822,#6823,#4424,.T.);
#9461=EDGE_CURVE('',#6824,#6822,#3465,.T.);
#9462=EDGE_CURVE('',#6818,#6824,#3466,.T.);
#9463=EDGE_CURVE('',#6819,#6825,#3467,.T.);
#9464=EDGE_CURVE('',#6825,#6823,#3468,.T.);
#9465=EDGE_CURVE('',#6826,#6827,#4425,.T.);
#9466=EDGE_CURVE('',#6828,#6826,#3469,.T.);
#9467=EDGE_CURVE('',#6822,#6828,#3470,.T.);
#9468=EDGE_CURVE('',#6823,#6829,#3471,.T.);
#9469=EDGE_CURVE('',#6829,#6827,#3472,.T.);
#9470=EDGE_CURVE('',#6830,#6831,#4426,.T.);
#9471=EDGE_CURVE('',#6832,#6830,#3473,.T.);
#9472=EDGE_CURVE('',#6826,#6832,#3474,.T.);
#9473=EDGE_CURVE('',#6827,#6833,#3475,.T.);
#9474=EDGE_CURVE('',#6833,#6831,#3476,.T.);
#9475=EDGE_CURVE('',#6834,#6835,#4427,.T.);
#9476=EDGE_CURVE('',#6836,#6834,#3477,.T.);
#9477=EDGE_CURVE('',#6830,#6836,#3478,.T.);
#9478=EDGE_CURVE('',#6831,#6837,#3479,.T.);
#9479=EDGE_CURVE('',#6837,#6835,#3480,.T.);
#9480=EDGE_CURVE('',#6838,#6839,#4428,.T.);
#9481=EDGE_CURVE('',#6840,#6838,#3481,.T.);
#9482=EDGE_CURVE('',#6834,#6840,#3482,.T.);
#9483=EDGE_CURVE('',#6835,#6841,#3483,.T.);
#9484=EDGE_CURVE('',#6841,#6839,#3484,.T.);
#9485=EDGE_CURVE('',#6842,#6843,#4429,.T.);
#9486=EDGE_CURVE('',#6844,#6842,#3485,.T.);
#9487=EDGE_CURVE('',#6838,#6844,#3486,.T.);
#9488=EDGE_CURVE('',#6839,#6845,#3487,.T.);
#9489=EDGE_CURVE('',#6845,#6843,#3488,.T.);
#9490=EDGE_CURVE('',#6846,#6847,#4430,.T.);
#9491=EDGE_CURVE('',#6848,#6846,#3489,.T.);
#9492=EDGE_CURVE('',#6842,#6848,#3490,.T.);
#9493=EDGE_CURVE('',#6843,#6849,#3491,.T.);
#9494=EDGE_CURVE('',#6849,#6847,#3492,.T.);
#9495=EDGE_CURVE('',#6850,#6851,#4431,.T.);
#9496=EDGE_CURVE('',#6852,#6850,#3493,.T.);
#9497=EDGE_CURVE('',#6846,#6852,#3494,.T.);
#9498=EDGE_CURVE('',#6847,#6853,#3495,.T.);
#9499=EDGE_CURVE('',#6853,#6851,#3496,.T.);
#9500=EDGE_CURVE('',#6854,#6855,#4432,.T.);
#9501=EDGE_CURVE('',#6856,#6854,#3497,.T.);
#9502=EDGE_CURVE('',#6850,#6856,#3498,.T.);
#9503=EDGE_CURVE('',#6851,#6857,#3499,.T.);
#9504=EDGE_CURVE('',#6857,#6855,#3500,.T.);
#9505=EDGE_CURVE('',#6858,#6859,#4433,.T.);
#9506=EDGE_CURVE('',#6860,#6858,#3501,.T.);
#9507=EDGE_CURVE('',#6854,#6860,#3502,.T.);
#9508=EDGE_CURVE('',#6855,#6861,#3503,.T.);
#9509=EDGE_CURVE('',#6861,#6859,#3504,.T.);
#9510=EDGE_CURVE('',#6862,#6863,#4434,.T.);
#9511=EDGE_CURVE('',#6864,#6862,#3505,.T.);
#9512=EDGE_CURVE('',#6858,#6864,#3506,.T.);
#9513=EDGE_CURVE('',#6859,#6865,#3507,.T.);
#9514=EDGE_CURVE('',#6865,#6863,#3508,.T.);
#9515=EDGE_CURVE('',#6866,#6867,#4435,.T.);
#9516=EDGE_CURVE('',#6868,#6866,#3509,.T.);
#9517=EDGE_CURVE('',#6862,#6868,#3510,.T.);
#9518=EDGE_CURVE('',#6863,#6869,#3511,.T.);
#9519=EDGE_CURVE('',#6869,#6867,#3512,.T.);
#9520=EDGE_CURVE('',#6870,#6871,#4436,.T.);
#9521=EDGE_CURVE('',#6872,#6870,#3513,.T.);
#9522=EDGE_CURVE('',#6866,#6872,#3514,.T.);
#9523=EDGE_CURVE('',#6867,#6873,#3515,.T.);
#9524=EDGE_CURVE('',#6873,#6871,#3516,.T.);
#9525=EDGE_CURVE('',#6874,#6875,#4437,.T.);
#9526=EDGE_CURVE('',#6876,#6874,#3517,.T.);
#9527=EDGE_CURVE('',#6870,#6876,#3518,.T.);
#9528=EDGE_CURVE('',#6871,#6877,#3519,.T.);
#9529=EDGE_CURVE('',#6877,#6875,#3520,.T.);
#9530=EDGE_CURVE('',#6878,#6879,#4438,.T.);
#9531=EDGE_CURVE('',#6880,#6878,#3521,.T.);
#9532=EDGE_CURVE('',#6874,#6880,#3522,.T.);
#9533=EDGE_CURVE('',#6875,#6881,#3523,.T.);
#9534=EDGE_CURVE('',#6881,#6879,#3524,.T.);
#9535=EDGE_CURVE('',#6882,#6883,#3525,.T.);
#9536=EDGE_CURVE('',#6884,#6883,#1918,.T.);
#9537=EDGE_CURVE('',#6884,#6885,#3526,.T.);
#9538=EDGE_CURVE('',#6885,#6886,#3527,.T.);
#9539=EDGE_CURVE('',#6886,#6887,#3528,.T.);
#9540=EDGE_CURVE('',#6887,#6888,#3529,.T.);
#9541=EDGE_CURVE('',#6888,#6889,#3530,.T.);
#9542=EDGE_CURVE('',#6889,#6890,#3531,.T.);
#9543=EDGE_CURVE('',#6890,#6891,#3532,.T.);
#9544=EDGE_CURVE('',#6891,#6892,#3533,.T.);
#9545=EDGE_CURVE('',#6892,#6893,#3534,.T.);
#9546=EDGE_CURVE('',#6893,#6894,#3535,.T.);
#9547=EDGE_CURVE('',#6894,#6895,#3536,.T.);
#9548=EDGE_CURVE('',#6895,#6896,#3537,.T.);
#9549=EDGE_CURVE('',#6896,#6897,#3538,.T.);
#9550=EDGE_CURVE('',#6897,#6898,#3539,.T.);
#9551=EDGE_CURVE('',#6898,#6899,#3540,.T.);
#9552=EDGE_CURVE('',#6899,#6900,#3541,.T.);
#9553=EDGE_CURVE('',#6900,#6901,#3542,.T.);
#9554=EDGE_CURVE('',#6901,#6902,#3543,.T.);
#9555=EDGE_CURVE('',#6902,#6903,#3544,.T.);
#9556=EDGE_CURVE('',#6903,#6904,#3545,.T.);
#9557=EDGE_CURVE('',#6904,#6905,#3546,.T.);
#9558=EDGE_CURVE('',#6905,#6906,#3547,.T.);
#9559=EDGE_CURVE('',#6906,#6907,#3548,.T.);
#9560=EDGE_CURVE('',#6907,#6908,#3549,.T.);
#9561=EDGE_CURVE('',#6908,#6909,#3550,.T.);
#9562=EDGE_CURVE('',#6909,#6910,#3551,.T.);
#9563=EDGE_CURVE('',#6910,#6911,#3552,.T.);
#9564=EDGE_CURVE('',#6911,#6912,#3553,.T.);
#9565=EDGE_CURVE('',#6912,#6913,#3554,.T.);
#9566=EDGE_CURVE('',#6913,#6914,#3555,.T.);
#9567=EDGE_CURVE('',#6914,#6915,#3556,.T.);
#9568=EDGE_CURVE('',#6915,#6916,#3557,.T.);
#9569=EDGE_CURVE('',#6916,#6917,#3558,.T.);
#9570=EDGE_CURVE('',#6917,#6918,#3559,.T.);
#9571=EDGE_CURVE('',#6918,#6919,#3560,.T.);
#9572=EDGE_CURVE('',#6919,#6920,#3561,.T.);
#9573=EDGE_CURVE('',#6920,#6921,#3562,.T.);
#9574=EDGE_CURVE('',#6921,#6922,#3563,.T.);
#9575=EDGE_CURVE('',#6922,#6923,#3564,.T.);
#9576=EDGE_CURVE('',#6923,#6924,#3565,.T.);
#9577=EDGE_CURVE('',#6924,#6925,#3566,.T.);
#9578=EDGE_CURVE('',#6925,#6926,#3567,.T.);
#9579=EDGE_CURVE('',#6926,#6927,#3568,.T.);
#9580=EDGE_CURVE('',#6927,#6928,#3569,.T.);
#9581=EDGE_CURVE('',#6928,#6929,#3570,.T.);
#9582=EDGE_CURVE('',#6929,#6930,#3571,.T.);
#9583=EDGE_CURVE('',#6930,#6931,#3572,.T.);
#9584=EDGE_CURVE('',#6931,#6932,#3573,.T.);
#9585=EDGE_CURVE('',#6932,#6933,#3574,.T.);
#9586=EDGE_CURVE('',#6934,#6933,#1919,.F.);
#9587=EDGE_CURVE('',#6934,#6935,#3575,.T.);
#9588=EDGE_CURVE('',#6935,#6936,#3576,.T.);
#9589=EDGE_CURVE('',#6936,#6937,#3577,.T.);
#9590=EDGE_CURVE('',#6937,#6938,#3578,.T.);
#9591=EDGE_CURVE('',#6938,#6939,#3579,.T.);
#9592=EDGE_CURVE('',#6939,#6940,#3580,.T.);
#9593=EDGE_CURVE('',#6940,#6941,#3581,.T.);
#9594=EDGE_CURVE('',#6941,#6942,#3582,.T.);
#9595=EDGE_CURVE('',#6942,#6943,#3583,.T.);
#9596=EDGE_CURVE('',#6943,#6944,#3584,.T.);
#9597=EDGE_CURVE('',#6944,#6945,#3585,.T.);
#9598=EDGE_CURVE('',#6945,#6946,#3586,.T.);
#9599=EDGE_CURVE('',#6946,#6947,#3587,.T.);
#9600=EDGE_CURVE('',#6947,#6948,#3588,.T.);
#9601=EDGE_CURVE('',#6948,#6949,#3589,.T.);
#9602=EDGE_CURVE('',#6949,#6950,#3590,.T.);
#9603=EDGE_CURVE('',#6950,#6951,#3591,.T.);
#9604=EDGE_CURVE('',#6951,#6952,#3592,.T.);
#9605=EDGE_CURVE('',#6952,#6953,#3593,.T.);
#9606=EDGE_CURVE('',#6953,#6954,#3594,.T.);
#9607=EDGE_CURVE('',#6954,#6955,#3595,.T.);
#9608=EDGE_CURVE('',#6955,#6956,#3596,.T.);
#9609=EDGE_CURVE('',#6956,#6957,#3597,.T.);
#9610=EDGE_CURVE('',#6957,#6958,#3598,.T.);
#9611=EDGE_CURVE('',#6958,#6959,#3599,.T.);
#9612=EDGE_CURVE('',#6959,#6960,#3600,.T.);
#9613=EDGE_CURVE('',#6960,#6961,#3601,.T.);
#9614=EDGE_CURVE('',#6961,#6962,#3602,.T.);
#9615=EDGE_CURVE('',#6962,#6963,#3603,.T.);
#9616=EDGE_CURVE('',#6963,#6964,#3604,.T.);
#9617=EDGE_CURVE('',#6964,#6965,#3605,.T.);
#9618=EDGE_CURVE('',#6965,#6966,#3606,.T.);
#9619=EDGE_CURVE('',#6966,#6967,#3607,.T.);
#9620=EDGE_CURVE('',#6967,#6968,#3608,.T.);
#9621=EDGE_CURVE('',#6968,#6969,#3609,.T.);
#9622=EDGE_CURVE('',#6969,#6970,#3610,.T.);
#9623=EDGE_CURVE('',#6970,#6971,#3611,.T.);
#9624=EDGE_CURVE('',#6971,#6972,#3612,.T.);
#9625=EDGE_CURVE('',#6972,#6973,#3613,.T.);
#9626=EDGE_CURVE('',#6973,#6974,#3614,.T.);
#9627=EDGE_CURVE('',#6974,#6975,#3615,.T.);
#9628=EDGE_CURVE('',#6975,#6976,#3616,.T.);
#9629=EDGE_CURVE('',#6976,#6977,#3617,.T.);
#9630=EDGE_CURVE('',#6977,#6978,#3618,.T.);
#9631=EDGE_CURVE('',#6978,#6979,#3619,.T.);
#9632=EDGE_CURVE('',#6979,#6980,#3620,.T.);
#9633=EDGE_CURVE('',#6980,#6882,#3621,.T.);
#9634=EDGE_CURVE('',#6879,#6981,#3622,.T.);
#9635=EDGE_CURVE('',#6981,#6982,#3623,.T.);
#9636=EDGE_CURVE('',#6983,#6982,#1920,.T.);
#9637=EDGE_CURVE('',#6984,#6983,#3624,.T.);
#9638=EDGE_CURVE('',#6878,#6984,#3625,.T.);
#9639=EDGE_CURVE('',#6985,#6986,#3626,.T.);
#9640=EDGE_CURVE('',#6987,#6985,#3627,.T.);
#9641=EDGE_CURVE('',#6986,#6987,#3628,.T.);
#9642=EDGE_CURVE('',#6986,#6988,#4439,.T.);
#9643=EDGE_CURVE('',#6989,#6988,#3629,.T.);
#9644=EDGE_CURVE('',#6990,#6989,#3630,.T.);
#9645=EDGE_CURVE('',#6988,#6990,#3631,.T.);
#9646=EDGE_CURVE('',#6933,#6983,#3632,.T.);
#9647=EDGE_CURVE('',#6624,#6884,#3633,.T.);
#9648=EDGE_CURVE('',#6982,#6934,#3634,.T.);
#9649=EDGE_CURVE('',#6883,#6625,#3635,.T.);
#9650=EDGE_CURVE('',#6991,#6991,#1921,.T.);
#9651=EDGE_CURVE('',#6992,#6992,#1922,.T.);
#9652=EDGE_CURVE('',#6993,#6993,#1923,.T.);
#9653=EDGE_CURVE('',#6993,#6991,#4440,.T.);
#9654=EDGE_CURVE('',#6992,#6989,#4441,.T.);
#9655=EDGE_CURVE('',#6990,#6994,#4442,.T.);
#9656=EDGE_CURVE('',#6994,#6994,#1924,.T.);
#13799=ORIENTED_EDGE('',*,*,#9211,.F.);
#13800=ORIENTED_EDGE('',*,*,#9212,.F.);
#13801=ORIENTED_EDGE('',*,*,#9213,.F.);
#13802=ORIENTED_EDGE('',*,*,#9214,.T.);
#13803=ORIENTED_EDGE('',*,*,#9215,.F.);
#13804=ORIENTED_EDGE('',*,*,#9216,.F.);
#13805=ORIENTED_EDGE('',*,*,#9217,.F.);
#13806=ORIENTED_EDGE('',*,*,#9211,.T.);
#13807=ORIENTED_EDGE('',*,*,#9218,.T.);
#13808=ORIENTED_EDGE('',*,*,#9219,.T.);
#13809=ORIENTED_EDGE('',*,*,#9220,.F.);
#13810=ORIENTED_EDGE('',*,*,#9221,.F.);
#13811=ORIENTED_EDGE('',*,*,#9222,.F.);
#13812=ORIENTED_EDGE('',*,*,#9215,.T.);
#13813=ORIENTED_EDGE('',*,*,#9223,.T.);
#13814=ORIENTED_EDGE('',*,*,#9224,.T.);
#13815=ORIENTED_EDGE('',*,*,#9225,.F.);
#13816=ORIENTED_EDGE('',*,*,#9226,.F.);
#13817=ORIENTED_EDGE('',*,*,#9227,.F.);
#13818=ORIENTED_EDGE('',*,*,#9220,.T.);
#13819=ORIENTED_EDGE('',*,*,#9228,.T.);
#13820=ORIENTED_EDGE('',*,*,#9229,.T.);
#13821=ORIENTED_EDGE('',*,*,#9230,.F.);
#13822=ORIENTED_EDGE('',*,*,#9231,.F.);
#13823=ORIENTED_EDGE('',*,*,#9232,.F.);
#13824=ORIENTED_EDGE('',*,*,#9225,.T.);
#13825=ORIENTED_EDGE('',*,*,#9233,.T.);
#13826=ORIENTED_EDGE('',*,*,#9234,.T.);
#13827=ORIENTED_EDGE('',*,*,#9235,.F.);
#13828=ORIENTED_EDGE('',*,*,#9236,.F.);
#13829=ORIENTED_EDGE('',*,*,#9237,.F.);
#13830=ORIENTED_EDGE('',*,*,#9230,.T.);
#13831=ORIENTED_EDGE('',*,*,#9238,.T.);
#13832=ORIENTED_EDGE('',*,*,#9239,.T.);
#13833=ORIENTED_EDGE('',*,*,#9240,.F.);
#13834=ORIENTED_EDGE('',*,*,#9241,.F.);
#13835=ORIENTED_EDGE('',*,*,#9242,.F.);
#13836=ORIENTED_EDGE('',*,*,#9235,.T.);
#13837=ORIENTED_EDGE('',*,*,#9243,.T.);
#13838=ORIENTED_EDGE('',*,*,#9244,.T.);
#13839=ORIENTED_EDGE('',*,*,#9245,.F.);
#13840=ORIENTED_EDGE('',*,*,#9246,.F.);
#13841=ORIENTED_EDGE('',*,*,#9247,.F.);
#13842=ORIENTED_EDGE('',*,*,#9240,.T.);
#13843=ORIENTED_EDGE('',*,*,#9248,.T.);
#13844=ORIENTED_EDGE('',*,*,#9249,.T.);
#13845=ORIENTED_EDGE('',*,*,#9250,.F.);
#13846=ORIENTED_EDGE('',*,*,#9251,.F.);
#13847=ORIENTED_EDGE('',*,*,#9252,.F.);
#13848=ORIENTED_EDGE('',*,*,#9245,.T.);
#13849=ORIENTED_EDGE('',*,*,#9253,.T.);
#13850=ORIENTED_EDGE('',*,*,#9254,.T.);
#13851=ORIENTED_EDGE('',*,*,#9255,.F.);
#13852=ORIENTED_EDGE('',*,*,#9256,.F.);
#13853=ORIENTED_EDGE('',*,*,#9257,.F.);
#13854=ORIENTED_EDGE('',*,*,#9250,.T.);
#13855=ORIENTED_EDGE('',*,*,#9258,.T.);
#13856=ORIENTED_EDGE('',*,*,#9259,.T.);
#13857=ORIENTED_EDGE('',*,*,#9260,.F.);
#13858=ORIENTED_EDGE('',*,*,#9261,.F.);
#13859=ORIENTED_EDGE('',*,*,#9262,.F.);
#13860=ORIENTED_EDGE('',*,*,#9255,.T.);
#13861=ORIENTED_EDGE('',*,*,#9263,.T.);
#13862=ORIENTED_EDGE('',*,*,#9264,.T.);
#13863=ORIENTED_EDGE('',*,*,#9265,.F.);
#13864=ORIENTED_EDGE('',*,*,#9266,.F.);
#13865=ORIENTED_EDGE('',*,*,#9267,.F.);
#13866=ORIENTED_EDGE('',*,*,#9260,.T.);
#13867=ORIENTED_EDGE('',*,*,#9268,.T.);
#13868=ORIENTED_EDGE('',*,*,#9269,.T.);
#13869=ORIENTED_EDGE('',*,*,#9270,.F.);
#13870=ORIENTED_EDGE('',*,*,#9271,.F.);
#13871=ORIENTED_EDGE('',*,*,#9272,.F.);
#13872=ORIENTED_EDGE('',*,*,#9265,.T.);
#13873=ORIENTED_EDGE('',*,*,#9273,.T.);
#13874=ORIENTED_EDGE('',*,*,#9274,.T.);
#13875=ORIENTED_EDGE('',*,*,#9275,.F.);
#13876=ORIENTED_EDGE('',*,*,#9276,.F.);
#13877=ORIENTED_EDGE('',*,*,#9277,.F.);
#13878=ORIENTED_EDGE('',*,*,#9270,.T.);
#13879=ORIENTED_EDGE('',*,*,#9278,.T.);
#13880=ORIENTED_EDGE('',*,*,#9279,.T.);
#13881=ORIENTED_EDGE('',*,*,#9280,.F.);
#13882=ORIENTED_EDGE('',*,*,#9281,.F.);
#13883=ORIENTED_EDGE('',*,*,#9282,.F.);
#13884=ORIENTED_EDGE('',*,*,#9275,.T.);
#13885=ORIENTED_EDGE('',*,*,#9283,.T.);
#13886=ORIENTED_EDGE('',*,*,#9284,.T.);
#13887=ORIENTED_EDGE('',*,*,#9285,.F.);
#13888=ORIENTED_EDGE('',*,*,#9286,.F.);
#13889=ORIENTED_EDGE('',*,*,#9287,.F.);
#13890=ORIENTED_EDGE('',*,*,#9280,.T.);
#13891=ORIENTED_EDGE('',*,*,#9288,.T.);
#13892=ORIENTED_EDGE('',*,*,#9289,.T.);
#13893=ORIENTED_EDGE('',*,*,#9290,.F.);
#13894=ORIENTED_EDGE('',*,*,#9291,.F.);
#13895=ORIENTED_EDGE('',*,*,#9292,.F.);
#13896=ORIENTED_EDGE('',*,*,#9285,.T.);
#13897=ORIENTED_EDGE('',*,*,#9293,.T.);
#13898=ORIENTED_EDGE('',*,*,#9294,.T.);
#13899=ORIENTED_EDGE('',*,*,#9295,.F.);
#13900=ORIENTED_EDGE('',*,*,#9296,.F.);
#13901=ORIENTED_EDGE('',*,*,#9297,.F.);
#13902=ORIENTED_EDGE('',*,*,#9290,.T.);
#13903=ORIENTED_EDGE('',*,*,#9298,.T.);
#13904=ORIENTED_EDGE('',*,*,#9299,.T.);
#13905=ORIENTED_EDGE('',*,*,#9300,.F.);
#13906=ORIENTED_EDGE('',*,*,#9301,.F.);
#13907=ORIENTED_EDGE('',*,*,#9302,.F.);
#13908=ORIENTED_EDGE('',*,*,#9295,.T.);
#13909=ORIENTED_EDGE('',*,*,#9303,.T.);
#13910=ORIENTED_EDGE('',*,*,#9304,.T.);
#13911=ORIENTED_EDGE('',*,*,#9305,.F.);
#13912=ORIENTED_EDGE('',*,*,#9306,.F.);
#13913=ORIENTED_EDGE('',*,*,#9307,.F.);
#13914=ORIENTED_EDGE('',*,*,#9300,.T.);
#13915=ORIENTED_EDGE('',*,*,#9308,.T.);
#13916=ORIENTED_EDGE('',*,*,#9309,.T.);
#13917=ORIENTED_EDGE('',*,*,#9310,.F.);
#13918=ORIENTED_EDGE('',*,*,#9311,.F.);
#13919=ORIENTED_EDGE('',*,*,#9312,.F.);
#13920=ORIENTED_EDGE('',*,*,#9305,.T.);
#13921=ORIENTED_EDGE('',*,*,#9313,.T.);
#13922=ORIENTED_EDGE('',*,*,#9314,.T.);
#13923=ORIENTED_EDGE('',*,*,#9315,.F.);
#13924=ORIENTED_EDGE('',*,*,#9316,.F.);
#13925=ORIENTED_EDGE('',*,*,#9317,.F.);
#13926=ORIENTED_EDGE('',*,*,#9310,.T.);
#13927=ORIENTED_EDGE('',*,*,#9318,.T.);
#13928=ORIENTED_EDGE('',*,*,#9319,.T.);
#13929=ORIENTED_EDGE('',*,*,#9320,.F.);
#13930=ORIENTED_EDGE('',*,*,#9321,.F.);
#13931=ORIENTED_EDGE('',*,*,#9322,.F.);
#13932=ORIENTED_EDGE('',*,*,#9315,.T.);
#13933=ORIENTED_EDGE('',*,*,#9323,.T.);
#13934=ORIENTED_EDGE('',*,*,#9324,.T.);
#13935=ORIENTED_EDGE('',*,*,#9325,.F.);
#13936=ORIENTED_EDGE('',*,*,#9326,.F.);
#13937=ORIENTED_EDGE('',*,*,#9327,.F.);
#13938=ORIENTED_EDGE('',*,*,#9320,.T.);
#13939=ORIENTED_EDGE('',*,*,#9328,.T.);
#13940=ORIENTED_EDGE('',*,*,#9329,.T.);
#13941=ORIENTED_EDGE('',*,*,#9330,.F.);
#13942=ORIENTED_EDGE('',*,*,#9331,.F.);
#13943=ORIENTED_EDGE('',*,*,#9332,.F.);
#13944=ORIENTED_EDGE('',*,*,#9325,.T.);
#13945=ORIENTED_EDGE('',*,*,#9333,.T.);
#13946=ORIENTED_EDGE('',*,*,#9334,.T.);
#13947=ORIENTED_EDGE('',*,*,#9335,.F.);
#13948=ORIENTED_EDGE('',*,*,#9336,.F.);
#13949=ORIENTED_EDGE('',*,*,#9337,.F.);
#13950=ORIENTED_EDGE('',*,*,#9330,.T.);
#13951=ORIENTED_EDGE('',*,*,#9338,.T.);
#13952=ORIENTED_EDGE('',*,*,#9339,.T.);
#13953=ORIENTED_EDGE('',*,*,#9340,.F.);
#13954=ORIENTED_EDGE('',*,*,#9341,.F.);
#13955=ORIENTED_EDGE('',*,*,#9342,.F.);
#13956=ORIENTED_EDGE('',*,*,#9335,.T.);
#13957=ORIENTED_EDGE('',*,*,#9343,.T.);
#13958=ORIENTED_EDGE('',*,*,#9344,.T.);
#13959=ORIENTED_EDGE('',*,*,#9345,.F.);
#13960=ORIENTED_EDGE('',*,*,#9346,.F.);
#13961=ORIENTED_EDGE('',*,*,#9347,.F.);
#13962=ORIENTED_EDGE('',*,*,#9340,.T.);
#13963=ORIENTED_EDGE('',*,*,#9348,.T.);
#13964=ORIENTED_EDGE('',*,*,#9349,.T.);
#13965=ORIENTED_EDGE('',*,*,#9350,.F.);
#13966=ORIENTED_EDGE('',*,*,#9351,.F.);
#13967=ORIENTED_EDGE('',*,*,#9352,.F.);
#13968=ORIENTED_EDGE('',*,*,#9345,.T.);
#13969=ORIENTED_EDGE('',*,*,#9353,.T.);
#13970=ORIENTED_EDGE('',*,*,#9354,.T.);
#13971=ORIENTED_EDGE('',*,*,#9355,.F.);
#13972=ORIENTED_EDGE('',*,*,#9356,.F.);
#13973=ORIENTED_EDGE('',*,*,#9357,.F.);
#13974=ORIENTED_EDGE('',*,*,#9350,.T.);
#13975=ORIENTED_EDGE('',*,*,#9358,.T.);
#13976=ORIENTED_EDGE('',*,*,#9359,.T.);
#13977=ORIENTED_EDGE('',*,*,#9360,.F.);
#13978=ORIENTED_EDGE('',*,*,#9361,.F.);
#13979=ORIENTED_EDGE('',*,*,#9362,.F.);
#13980=ORIENTED_EDGE('',*,*,#9355,.T.);
#13981=ORIENTED_EDGE('',*,*,#9363,.T.);
#13982=ORIENTED_EDGE('',*,*,#9364,.T.);
#13983=ORIENTED_EDGE('',*,*,#9365,.F.);
#13984=ORIENTED_EDGE('',*,*,#9366,.F.);
#13985=ORIENTED_EDGE('',*,*,#9367,.F.);
#13986=ORIENTED_EDGE('',*,*,#9360,.T.);
#13987=ORIENTED_EDGE('',*,*,#9368,.T.);
#13988=ORIENTED_EDGE('',*,*,#9369,.T.);
#13989=ORIENTED_EDGE('',*,*,#9370,.F.);
#13990=ORIENTED_EDGE('',*,*,#9371,.F.);
#13991=ORIENTED_EDGE('',*,*,#9372,.F.);
#13992=ORIENTED_EDGE('',*,*,#9365,.T.);
#13993=ORIENTED_EDGE('',*,*,#9373,.T.);
#13994=ORIENTED_EDGE('',*,*,#9374,.T.);
#13995=ORIENTED_EDGE('',*,*,#9375,.F.);
#13996=ORIENTED_EDGE('',*,*,#9376,.F.);
#13997=ORIENTED_EDGE('',*,*,#9377,.F.);
#13998=ORIENTED_EDGE('',*,*,#9370,.T.);
#13999=ORIENTED_EDGE('',*,*,#9378,.T.);
#14000=ORIENTED_EDGE('',*,*,#9379,.T.);
#14001=ORIENTED_EDGE('',*,*,#9380,.F.);
#14002=ORIENTED_EDGE('',*,*,#9381,.F.);
#14003=ORIENTED_EDGE('',*,*,#9382,.F.);
#14004=ORIENTED_EDGE('',*,*,#9375,.T.);
#14005=ORIENTED_EDGE('',*,*,#9383,.T.);
#14006=ORIENTED_EDGE('',*,*,#9384,.T.);
#14007=ORIENTED_EDGE('',*,*,#9385,.F.);
#14008=ORIENTED_EDGE('',*,*,#9386,.F.);
#14009=ORIENTED_EDGE('',*,*,#9387,.F.);
#14010=ORIENTED_EDGE('',*,*,#9380,.T.);
#14011=ORIENTED_EDGE('',*,*,#9388,.T.);
#14012=ORIENTED_EDGE('',*,*,#9389,.T.);
#14013=ORIENTED_EDGE('',*,*,#9390,.F.);
#14014=ORIENTED_EDGE('',*,*,#9391,.F.);
#14015=ORIENTED_EDGE('',*,*,#9392,.F.);
#14016=ORIENTED_EDGE('',*,*,#9385,.T.);
#14017=ORIENTED_EDGE('',*,*,#9393,.T.);
#14018=ORIENTED_EDGE('',*,*,#9394,.T.);
#14019=ORIENTED_EDGE('',*,*,#9395,.F.);
#14020=ORIENTED_EDGE('',*,*,#9396,.F.);
#14021=ORIENTED_EDGE('',*,*,#9397,.F.);
#14022=ORIENTED_EDGE('',*,*,#9390,.T.);
#14023=ORIENTED_EDGE('',*,*,#9398,.T.);
#14024=ORIENTED_EDGE('',*,*,#9399,.T.);
#14025=ORIENTED_EDGE('',*,*,#9400,.F.);
#14026=ORIENTED_EDGE('',*,*,#9401,.F.);
#14027=ORIENTED_EDGE('',*,*,#9402,.F.);
#14028=ORIENTED_EDGE('',*,*,#9395,.T.);
#14029=ORIENTED_EDGE('',*,*,#9403,.T.);
#14030=ORIENTED_EDGE('',*,*,#9404,.T.);
#14031=ORIENTED_EDGE('',*,*,#9405,.F.);
#14032=ORIENTED_EDGE('',*,*,#9406,.F.);
#14033=ORIENTED_EDGE('',*,*,#9407,.F.);
#14034=ORIENTED_EDGE('',*,*,#9400,.T.);
#14035=ORIENTED_EDGE('',*,*,#9408,.T.);
#14036=ORIENTED_EDGE('',*,*,#9409,.T.);
#14037=ORIENTED_EDGE('',*,*,#9410,.F.);
#14038=ORIENTED_EDGE('',*,*,#9411,.F.);
#14039=ORIENTED_EDGE('',*,*,#9412,.F.);
#14040=ORIENTED_EDGE('',*,*,#9405,.T.);
#14041=ORIENTED_EDGE('',*,*,#9413,.T.);
#14042=ORIENTED_EDGE('',*,*,#9414,.T.);
#14043=ORIENTED_EDGE('',*,*,#9415,.F.);
#14044=ORIENTED_EDGE('',*,*,#9416,.F.);
#14045=ORIENTED_EDGE('',*,*,#9417,.F.);
#14046=ORIENTED_EDGE('',*,*,#9410,.T.);
#14047=ORIENTED_EDGE('',*,*,#9418,.T.);
#14048=ORIENTED_EDGE('',*,*,#9419,.T.);
#14049=ORIENTED_EDGE('',*,*,#9420,.F.);
#14050=ORIENTED_EDGE('',*,*,#9421,.F.);
#14051=ORIENTED_EDGE('',*,*,#9422,.F.);
#14052=ORIENTED_EDGE('',*,*,#9415,.T.);
#14053=ORIENTED_EDGE('',*,*,#9423,.T.);
#14054=ORIENTED_EDGE('',*,*,#9424,.T.);
#14055=ORIENTED_EDGE('',*,*,#9425,.F.);
#14056=ORIENTED_EDGE('',*,*,#9426,.F.);
#14057=ORIENTED_EDGE('',*,*,#9427,.F.);
#14058=ORIENTED_EDGE('',*,*,#9420,.T.);
#14059=ORIENTED_EDGE('',*,*,#9428,.T.);
#14060=ORIENTED_EDGE('',*,*,#9429,.T.);
#14061=ORIENTED_EDGE('',*,*,#9430,.F.);
#14062=ORIENTED_EDGE('',*,*,#9431,.F.);
#14063=ORIENTED_EDGE('',*,*,#9432,.F.);
#14064=ORIENTED_EDGE('',*,*,#9425,.T.);
#14065=ORIENTED_EDGE('',*,*,#9433,.T.);
#14066=ORIENTED_EDGE('',*,*,#9434,.T.);
#14067=ORIENTED_EDGE('',*,*,#9435,.F.);
#14068=ORIENTED_EDGE('',*,*,#9436,.F.);
#14069=ORIENTED_EDGE('',*,*,#9437,.F.);
#14070=ORIENTED_EDGE('',*,*,#9430,.T.);
#14071=ORIENTED_EDGE('',*,*,#9438,.T.);
#14072=ORIENTED_EDGE('',*,*,#9439,.T.);
#14073=ORIENTED_EDGE('',*,*,#9440,.F.);
#14074=ORIENTED_EDGE('',*,*,#9441,.F.);
#14075=ORIENTED_EDGE('',*,*,#9442,.F.);
#14076=ORIENTED_EDGE('',*,*,#9435,.T.);
#14077=ORIENTED_EDGE('',*,*,#9443,.T.);
#14078=ORIENTED_EDGE('',*,*,#9444,.T.);
#14079=ORIENTED_EDGE('',*,*,#9445,.F.);
#14080=ORIENTED_EDGE('',*,*,#9446,.F.);
#14081=ORIENTED_EDGE('',*,*,#9447,.F.);
#14082=ORIENTED_EDGE('',*,*,#9440,.T.);
#14083=ORIENTED_EDGE('',*,*,#9448,.T.);
#14084=ORIENTED_EDGE('',*,*,#9449,.T.);
#14085=ORIENTED_EDGE('',*,*,#9450,.F.);
#14086=ORIENTED_EDGE('',*,*,#9451,.F.);
#14087=ORIENTED_EDGE('',*,*,#9452,.F.);
#14088=ORIENTED_EDGE('',*,*,#9445,.T.);
#14089=ORIENTED_EDGE('',*,*,#9453,.T.);
#14090=ORIENTED_EDGE('',*,*,#9454,.T.);
#14091=ORIENTED_EDGE('',*,*,#9455,.F.);
#14092=ORIENTED_EDGE('',*,*,#9456,.F.);
#14093=ORIENTED_EDGE('',*,*,#9457,.F.);
#14094=ORIENTED_EDGE('',*,*,#9450,.T.);
#14095=ORIENTED_EDGE('',*,*,#9458,.T.);
#14096=ORIENTED_EDGE('',*,*,#9459,.T.);
#14097=ORIENTED_EDGE('',*,*,#9460,.F.);
#14098=ORIENTED_EDGE('',*,*,#9461,.F.);
#14099=ORIENTED_EDGE('',*,*,#9462,.F.);
#14100=ORIENTED_EDGE('',*,*,#9455,.T.);
#14101=ORIENTED_EDGE('',*,*,#9463,.T.);
#14102=ORIENTED_EDGE('',*,*,#9464,.T.);
#14103=ORIENTED_EDGE('',*,*,#9465,.F.);
#14104=ORIENTED_EDGE('',*,*,#9466,.F.);
#14105=ORIENTED_EDGE('',*,*,#9467,.F.);
#14106=ORIENTED_EDGE('',*,*,#9460,.T.);
#14107=ORIENTED_EDGE('',*,*,#9468,.T.);
#14108=ORIENTED_EDGE('',*,*,#9469,.T.);
#14109=ORIENTED_EDGE('',*,*,#9470,.F.);
#14110=ORIENTED_EDGE('',*,*,#9471,.F.);
#14111=ORIENTED_EDGE('',*,*,#9472,.F.);
#14112=ORIENTED_EDGE('',*,*,#9465,.T.);
#14113=ORIENTED_EDGE('',*,*,#9473,.T.);
#14114=ORIENTED_EDGE('',*,*,#9474,.T.);
#14115=ORIENTED_EDGE('',*,*,#9475,.F.);
#14116=ORIENTED_EDGE('',*,*,#9476,.F.);
#14117=ORIENTED_EDGE('',*,*,#9477,.F.);
#14118=ORIENTED_EDGE('',*,*,#9470,.T.);
#14119=ORIENTED_EDGE('',*,*,#9478,.T.);
#14120=ORIENTED_EDGE('',*,*,#9479,.T.);
#14121=ORIENTED_EDGE('',*,*,#9480,.F.);
#14122=ORIENTED_EDGE('',*,*,#9481,.F.);
#14123=ORIENTED_EDGE('',*,*,#9482,.F.);
#14124=ORIENTED_EDGE('',*,*,#9475,.T.);
#14125=ORIENTED_EDGE('',*,*,#9483,.T.);
#14126=ORIENTED_EDGE('',*,*,#9484,.T.);
#14127=ORIENTED_EDGE('',*,*,#9485,.F.);
#14128=ORIENTED_EDGE('',*,*,#9486,.F.);
#14129=ORIENTED_EDGE('',*,*,#9487,.F.);
#14130=ORIENTED_EDGE('',*,*,#9480,.T.);
#14131=ORIENTED_EDGE('',*,*,#9488,.T.);
#14132=ORIENTED_EDGE('',*,*,#9489,.T.);
#14133=ORIENTED_EDGE('',*,*,#9490,.F.);
#14134=ORIENTED_EDGE('',*,*,#9491,.F.);
#14135=ORIENTED_EDGE('',*,*,#9492,.F.);
#14136=ORIENTED_EDGE('',*,*,#9485,.T.);
#14137=ORIENTED_EDGE('',*,*,#9493,.T.);
#14138=ORIENTED_EDGE('',*,*,#9494,.T.);
#14139=ORIENTED_EDGE('',*,*,#9495,.F.);
#14140=ORIENTED_EDGE('',*,*,#9496,.F.);
#14141=ORIENTED_EDGE('',*,*,#9497,.F.);
#14142=ORIENTED_EDGE('',*,*,#9490,.T.);
#14143=ORIENTED_EDGE('',*,*,#9498,.T.);
#14144=ORIENTED_EDGE('',*,*,#9499,.T.);
#14145=ORIENTED_EDGE('',*,*,#9500,.F.);
#14146=ORIENTED_EDGE('',*,*,#9501,.F.);
#14147=ORIENTED_EDGE('',*,*,#9502,.F.);
#14148=ORIENTED_EDGE('',*,*,#9495,.T.);
#14149=ORIENTED_EDGE('',*,*,#9503,.T.);
#14150=ORIENTED_EDGE('',*,*,#9504,.T.);
#14151=ORIENTED_EDGE('',*,*,#9505,.F.);
#14152=ORIENTED_EDGE('',*,*,#9506,.F.);
#14153=ORIENTED_EDGE('',*,*,#9507,.F.);
#14154=ORIENTED_EDGE('',*,*,#9500,.T.);
#14155=ORIENTED_EDGE('',*,*,#9508,.T.);
#14156=ORIENTED_EDGE('',*,*,#9509,.T.);
#14157=ORIENTED_EDGE('',*,*,#9510,.F.);
#14158=ORIENTED_EDGE('',*,*,#9511,.F.);
#14159=ORIENTED_EDGE('',*,*,#9512,.F.);
#14160=ORIENTED_EDGE('',*,*,#9505,.T.);
#14161=ORIENTED_EDGE('',*,*,#9513,.T.);
#14162=ORIENTED_EDGE('',*,*,#9514,.T.);
#14163=ORIENTED_EDGE('',*,*,#9515,.F.);
#14164=ORIENTED_EDGE('',*,*,#9516,.F.);
#14165=ORIENTED_EDGE('',*,*,#9517,.F.);
#14166=ORIENTED_EDGE('',*,*,#9510,.T.);
#14167=ORIENTED_EDGE('',*,*,#9518,.T.);
#14168=ORIENTED_EDGE('',*,*,#9519,.T.);
#14169=ORIENTED_EDGE('',*,*,#9520,.F.);
#14170=ORIENTED_EDGE('',*,*,#9521,.F.);
#14171=ORIENTED_EDGE('',*,*,#9522,.F.);
#14172=ORIENTED_EDGE('',*,*,#9515,.T.);
#14173=ORIENTED_EDGE('',*,*,#9523,.T.);
#14174=ORIENTED_EDGE('',*,*,#9524,.T.);
#14175=ORIENTED_EDGE('',*,*,#9525,.F.);
#14176=ORIENTED_EDGE('',*,*,#9526,.F.);
#14177=ORIENTED_EDGE('',*,*,#9527,.F.);
#14178=ORIENTED_EDGE('',*,*,#9520,.T.);
#14179=ORIENTED_EDGE('',*,*,#9528,.T.);
#14180=ORIENTED_EDGE('',*,*,#9529,.T.);
#14181=ORIENTED_EDGE('',*,*,#9530,.F.);
#14182=ORIENTED_EDGE('',*,*,#9531,.F.);
#14183=ORIENTED_EDGE('',*,*,#9532,.F.);
#14184=ORIENTED_EDGE('',*,*,#9525,.T.);
#14185=ORIENTED_EDGE('',*,*,#9533,.T.);
#14186=ORIENTED_EDGE('',*,*,#9534,.T.);
#14187=ORIENTED_EDGE('',*,*,#9535,.T.);
#14188=ORIENTED_EDGE('',*,*,#9536,.F.);
#14189=ORIENTED_EDGE('',*,*,#9537,.T.);
#14190=ORIENTED_EDGE('',*,*,#9538,.T.);
#14191=ORIENTED_EDGE('',*,*,#9539,.T.);
#14192=ORIENTED_EDGE('',*,*,#9540,.T.);
#14193=ORIENTED_EDGE('',*,*,#9541,.T.);
#14194=ORIENTED_EDGE('',*,*,#9542,.T.);
#14195=ORIENTED_EDGE('',*,*,#9543,.T.);
#14196=ORIENTED_EDGE('',*,*,#9544,.T.);
#14197=ORIENTED_EDGE('',*,*,#9545,.T.);
#14198=ORIENTED_EDGE('',*,*,#9546,.T.);
#14199=ORIENTED_EDGE('',*,*,#9547,.T.);
#14200=ORIENTED_EDGE('',*,*,#9548,.T.);
#14201=ORIENTED_EDGE('',*,*,#9549,.T.);
#14202=ORIENTED_EDGE('',*,*,#9550,.T.);
#14203=ORIENTED_EDGE('',*,*,#9551,.T.);
#14204=ORIENTED_EDGE('',*,*,#9552,.T.);
#14205=ORIENTED_EDGE('',*,*,#9553,.T.);
#14206=ORIENTED_EDGE('',*,*,#9554,.T.);
#14207=ORIENTED_EDGE('',*,*,#9555,.T.);
#14208=ORIENTED_EDGE('',*,*,#9556,.T.);
#14209=ORIENTED_EDGE('',*,*,#9557,.T.);
#14210=ORIENTED_EDGE('',*,*,#9558,.T.);
#14211=ORIENTED_EDGE('',*,*,#9559,.T.);
#14212=ORIENTED_EDGE('',*,*,#9560,.T.);
#14213=ORIENTED_EDGE('',*,*,#9561,.T.);
#14214=ORIENTED_EDGE('',*,*,#9562,.T.);
#14215=ORIENTED_EDGE('',*,*,#9563,.T.);
#14216=ORIENTED_EDGE('',*,*,#9564,.T.);
#14217=ORIENTED_EDGE('',*,*,#9565,.T.);
#14218=ORIENTED_EDGE('',*,*,#9566,.T.);
#14219=ORIENTED_EDGE('',*,*,#9567,.T.);
#14220=ORIENTED_EDGE('',*,*,#9568,.T.);
#14221=ORIENTED_EDGE('',*,*,#9569,.T.);
#14222=ORIENTED_EDGE('',*,*,#9570,.T.);
#14223=ORIENTED_EDGE('',*,*,#9571,.T.);
#14224=ORIENTED_EDGE('',*,*,#9572,.T.);
#14225=ORIENTED_EDGE('',*,*,#9573,.T.);
#14226=ORIENTED_EDGE('',*,*,#9574,.T.);
#14227=ORIENTED_EDGE('',*,*,#9575,.T.);
#14228=ORIENTED_EDGE('',*,*,#9576,.T.);
#14229=ORIENTED_EDGE('',*,*,#9577,.T.);
#14230=ORIENTED_EDGE('',*,*,#9578,.T.);
#14231=ORIENTED_EDGE('',*,*,#9579,.T.);
#14232=ORIENTED_EDGE('',*,*,#9580,.T.);
#14233=ORIENTED_EDGE('',*,*,#9581,.T.);
#14234=ORIENTED_EDGE('',*,*,#9582,.T.);
#14235=ORIENTED_EDGE('',*,*,#9583,.T.);
#14236=ORIENTED_EDGE('',*,*,#9584,.T.);
#14237=ORIENTED_EDGE('',*,*,#9585,.T.);
#14238=ORIENTED_EDGE('',*,*,#9586,.F.);
#14239=ORIENTED_EDGE('',*,*,#9587,.T.);
#14240=ORIENTED_EDGE('',*,*,#9588,.T.);
#14241=ORIENTED_EDGE('',*,*,#9589,.T.);
#14242=ORIENTED_EDGE('',*,*,#9590,.T.);
#14243=ORIENTED_EDGE('',*,*,#9591,.T.);
#14244=ORIENTED_EDGE('',*,*,#9592,.T.);
#14245=ORIENTED_EDGE('',*,*,#9593,.T.);
#14246=ORIENTED_EDGE('',*,*,#9594,.T.);
#14247=ORIENTED_EDGE('',*,*,#9595,.T.);
#14248=ORIENTED_EDGE('',*,*,#9596,.T.);
#14249=ORIENTED_EDGE('',*,*,#9597,.T.);
#14250=ORIENTED_EDGE('',*,*,#9598,.T.);
#14251=ORIENTED_EDGE('',*,*,#9599,.T.);
#14252=ORIENTED_EDGE('',*,*,#9600,.T.);
#14253=ORIENTED_EDGE('',*,*,#9601,.T.);
#14254=ORIENTED_EDGE('',*,*,#9602,.T.);
#14255=ORIENTED_EDGE('',*,*,#9603,.T.);
#14256=ORIENTED_EDGE('',*,*,#9604,.T.);
#14257=ORIENTED_EDGE('',*,*,#9605,.T.);
#14258=ORIENTED_EDGE('',*,*,#9606,.T.);
#14259=ORIENTED_EDGE('',*,*,#9607,.T.);
#14260=ORIENTED_EDGE('',*,*,#9608,.T.);
#14261=ORIENTED_EDGE('',*,*,#9609,.T.);
#14262=ORIENTED_EDGE('',*,*,#9610,.T.);
#14263=ORIENTED_EDGE('',*,*,#9611,.T.);
#14264=ORIENTED_EDGE('',*,*,#9612,.T.);
#14265=ORIENTED_EDGE('',*,*,#9613,.T.);
#14266=ORIENTED_EDGE('',*,*,#9614,.T.);
#14267=ORIENTED_EDGE('',*,*,#9615,.T.);
#14268=ORIENTED_EDGE('',*,*,#9616,.T.);
#14269=ORIENTED_EDGE('',*,*,#9617,.T.);
#14270=ORIENTED_EDGE('',*,*,#9618,.T.);
#14271=ORIENTED_EDGE('',*,*,#9619,.T.);
#14272=ORIENTED_EDGE('',*,*,#9620,.T.);
#14273=ORIENTED_EDGE('',*,*,#9621,.T.);
#14274=ORIENTED_EDGE('',*,*,#9622,.T.);
#14275=ORIENTED_EDGE('',*,*,#9623,.T.);
#14276=ORIENTED_EDGE('',*,*,#9624,.T.);
#14277=ORIENTED_EDGE('',*,*,#9625,.T.);
#14278=ORIENTED_EDGE('',*,*,#9626,.T.);
#14279=ORIENTED_EDGE('',*,*,#9627,.T.);
#14280=ORIENTED_EDGE('',*,*,#9628,.T.);
#14281=ORIENTED_EDGE('',*,*,#9629,.T.);
#14282=ORIENTED_EDGE('',*,*,#9630,.T.);
#14283=ORIENTED_EDGE('',*,*,#9631,.T.);
#14284=ORIENTED_EDGE('',*,*,#9632,.T.);
#14285=ORIENTED_EDGE('',*,*,#9633,.T.);
#14286=ORIENTED_EDGE('',*,*,#9530,.T.);
#14287=ORIENTED_EDGE('',*,*,#9634,.T.);
#14288=ORIENTED_EDGE('',*,*,#9635,.T.);
#14289=ORIENTED_EDGE('',*,*,#9636,.F.);
#14290=ORIENTED_EDGE('',*,*,#9637,.F.);
#14291=ORIENTED_EDGE('',*,*,#9638,.F.);
#14292=ORIENTED_EDGE('',*,*,#9639,.F.);
#14293=ORIENTED_EDGE('',*,*,#9640,.F.);
#14294=ORIENTED_EDGE('',*,*,#9641,.F.);
#14295=ORIENTED_EDGE('',*,*,#9642,.T.);
#14296=ORIENTED_EDGE('',*,*,#9643,.F.);
#14297=ORIENTED_EDGE('',*,*,#9644,.F.);
#14298=ORIENTED_EDGE('',*,*,#9645,.F.);
#14299=ORIENTED_EDGE('',*,*,#9642,.F.);
#14300=ORIENTED_EDGE('',*,*,#9646,.F.);
#14301=ORIENTED_EDGE('',*,*,#9585,.F.);
#14302=ORIENTED_EDGE('',*,*,#9584,.F.);
#14303=ORIENTED_EDGE('',*,*,#9583,.F.);
#14304=ORIENTED_EDGE('',*,*,#9582,.F.);
#14305=ORIENTED_EDGE('',*,*,#9581,.F.);
#14306=ORIENTED_EDGE('',*,*,#9580,.F.);
#14307=ORIENTED_EDGE('',*,*,#9579,.F.);
#14308=ORIENTED_EDGE('',*,*,#9578,.F.);
#14309=ORIENTED_EDGE('',*,*,#9577,.F.);
#14310=ORIENTED_EDGE('',*,*,#9576,.F.);
#14311=ORIENTED_EDGE('',*,*,#9575,.F.);
#14312=ORIENTED_EDGE('',*,*,#9574,.F.);
#14313=ORIENTED_EDGE('',*,*,#9573,.F.);
#14314=ORIENTED_EDGE('',*,*,#9572,.F.);
#14315=ORIENTED_EDGE('',*,*,#9571,.F.);
#14316=ORIENTED_EDGE('',*,*,#9570,.F.);
#14317=ORIENTED_EDGE('',*,*,#9569,.F.);
#14318=ORIENTED_EDGE('',*,*,#9568,.F.);
#14319=ORIENTED_EDGE('',*,*,#9567,.F.);
#14320=ORIENTED_EDGE('',*,*,#9566,.F.);
#14321=ORIENTED_EDGE('',*,*,#9565,.F.);
#14322=ORIENTED_EDGE('',*,*,#9564,.F.);
#14323=ORIENTED_EDGE('',*,*,#9563,.F.);
#14324=ORIENTED_EDGE('',*,*,#9562,.F.);
#14325=ORIENTED_EDGE('',*,*,#9561,.F.);
#14326=ORIENTED_EDGE('',*,*,#9560,.F.);
#14327=ORIENTED_EDGE('',*,*,#9559,.F.);
#14328=ORIENTED_EDGE('',*,*,#9558,.F.);
#14329=ORIENTED_EDGE('',*,*,#9557,.F.);
#14330=ORIENTED_EDGE('',*,*,#9556,.F.);
#14331=ORIENTED_EDGE('',*,*,#9555,.F.);
#14332=ORIENTED_EDGE('',*,*,#9554,.F.);
#14333=ORIENTED_EDGE('',*,*,#9553,.F.);
#14334=ORIENTED_EDGE('',*,*,#9552,.F.);
#14335=ORIENTED_EDGE('',*,*,#9551,.F.);
#14336=ORIENTED_EDGE('',*,*,#9550,.F.);
#14337=ORIENTED_EDGE('',*,*,#9549,.F.);
#14338=ORIENTED_EDGE('',*,*,#9548,.F.);
#14339=ORIENTED_EDGE('',*,*,#9547,.F.);
#14340=ORIENTED_EDGE('',*,*,#9546,.F.);
#14341=ORIENTED_EDGE('',*,*,#9545,.F.);
#14342=ORIENTED_EDGE('',*,*,#9544,.F.);
#14343=ORIENTED_EDGE('',*,*,#9543,.F.);
#14344=ORIENTED_EDGE('',*,*,#9542,.F.);
#14345=ORIENTED_EDGE('',*,*,#9541,.F.);
#14346=ORIENTED_EDGE('',*,*,#9540,.F.);
#14347=ORIENTED_EDGE('',*,*,#9539,.F.);
#14348=ORIENTED_EDGE('',*,*,#9538,.F.);
#14349=ORIENTED_EDGE('',*,*,#9537,.F.);
#14350=ORIENTED_EDGE('',*,*,#9647,.F.);
#14351=ORIENTED_EDGE('',*,*,#9212,.T.);
#14352=ORIENTED_EDGE('',*,*,#9217,.T.);
#14353=ORIENTED_EDGE('',*,*,#9216,.T.);
#14354=ORIENTED_EDGE('',*,*,#9222,.T.);
#14355=ORIENTED_EDGE('',*,*,#9221,.T.);
#14356=ORIENTED_EDGE('',*,*,#9227,.T.);
#14357=ORIENTED_EDGE('',*,*,#9226,.T.);
#14358=ORIENTED_EDGE('',*,*,#9232,.T.);
#14359=ORIENTED_EDGE('',*,*,#9231,.T.);
#14360=ORIENTED_EDGE('',*,*,#9237,.T.);
#14361=ORIENTED_EDGE('',*,*,#9236,.T.);
#14362=ORIENTED_EDGE('',*,*,#9242,.T.);
#14363=ORIENTED_EDGE('',*,*,#9241,.T.);
#14364=ORIENTED_EDGE('',*,*,#9247,.T.);
#14365=ORIENTED_EDGE('',*,*,#9246,.T.);
#14366=ORIENTED_EDGE('',*,*,#9252,.T.);
#14367=ORIENTED_EDGE('',*,*,#9251,.T.);
#14368=ORIENTED_EDGE('',*,*,#9257,.T.);
#14369=ORIENTED_EDGE('',*,*,#9256,.T.);
#14370=ORIENTED_EDGE('',*,*,#9262,.T.);
#14371=ORIENTED_EDGE('',*,*,#9261,.T.);
#14372=ORIENTED_EDGE('',*,*,#9267,.T.);
#14373=ORIENTED_EDGE('',*,*,#9266,.T.);
#14374=ORIENTED_EDGE('',*,*,#9272,.T.);
#14375=ORIENTED_EDGE('',*,*,#9271,.T.);
#14376=ORIENTED_EDGE('',*,*,#9277,.T.);
#14377=ORIENTED_EDGE('',*,*,#9276,.T.);
#14378=ORIENTED_EDGE('',*,*,#9282,.T.);
#14379=ORIENTED_EDGE('',*,*,#9281,.T.);
#14380=ORIENTED_EDGE('',*,*,#9287,.T.);
#14381=ORIENTED_EDGE('',*,*,#9286,.T.);
#14382=ORIENTED_EDGE('',*,*,#9292,.T.);
#14383=ORIENTED_EDGE('',*,*,#9291,.T.);
#14384=ORIENTED_EDGE('',*,*,#9297,.T.);
#14385=ORIENTED_EDGE('',*,*,#9296,.T.);
#14386=ORIENTED_EDGE('',*,*,#9302,.T.);
#14387=ORIENTED_EDGE('',*,*,#9301,.T.);
#14388=ORIENTED_EDGE('',*,*,#9307,.T.);
#14389=ORIENTED_EDGE('',*,*,#9306,.T.);
#14390=ORIENTED_EDGE('',*,*,#9312,.T.);
#14391=ORIENTED_EDGE('',*,*,#9311,.T.);
#14392=ORIENTED_EDGE('',*,*,#9317,.T.);
#14393=ORIENTED_EDGE('',*,*,#9316,.T.);
#14394=ORIENTED_EDGE('',*,*,#9322,.T.);
#14395=ORIENTED_EDGE('',*,*,#9321,.T.);
#14396=ORIENTED_EDGE('',*,*,#9327,.T.);
#14397=ORIENTED_EDGE('',*,*,#9326,.T.);
#14398=ORIENTED_EDGE('',*,*,#9332,.T.);
#14399=ORIENTED_EDGE('',*,*,#9331,.T.);
#14400=ORIENTED_EDGE('',*,*,#9337,.T.);
#14401=ORIENTED_EDGE('',*,*,#9336,.T.);
#14402=ORIENTED_EDGE('',*,*,#9342,.T.);
#14403=ORIENTED_EDGE('',*,*,#9341,.T.);
#14404=ORIENTED_EDGE('',*,*,#9347,.T.);
#14405=ORIENTED_EDGE('',*,*,#9346,.T.);
#14406=ORIENTED_EDGE('',*,*,#9352,.T.);
#14407=ORIENTED_EDGE('',*,*,#9351,.T.);
#14408=ORIENTED_EDGE('',*,*,#9357,.T.);
#14409=ORIENTED_EDGE('',*,*,#9356,.T.);
#14410=ORIENTED_EDGE('',*,*,#9362,.T.);
#14411=ORIENTED_EDGE('',*,*,#9361,.T.);
#14412=ORIENTED_EDGE('',*,*,#9367,.T.);
#14413=ORIENTED_EDGE('',*,*,#9366,.T.);
#14414=ORIENTED_EDGE('',*,*,#9372,.T.);
#14415=ORIENTED_EDGE('',*,*,#9371,.T.);
#14416=ORIENTED_EDGE('',*,*,#9377,.T.);
#14417=ORIENTED_EDGE('',*,*,#9376,.T.);
#14418=ORIENTED_EDGE('',*,*,#9382,.T.);
#14419=ORIENTED_EDGE('',*,*,#9381,.T.);
#14420=ORIENTED_EDGE('',*,*,#9387,.T.);
#14421=ORIENTED_EDGE('',*,*,#9386,.T.);
#14422=ORIENTED_EDGE('',*,*,#9392,.T.);
#14423=ORIENTED_EDGE('',*,*,#9391,.T.);
#14424=ORIENTED_EDGE('',*,*,#9397,.T.);
#14425=ORIENTED_EDGE('',*,*,#9396,.T.);
#14426=ORIENTED_EDGE('',*,*,#9402,.T.);
#14427=ORIENTED_EDGE('',*,*,#9401,.T.);
#14428=ORIENTED_EDGE('',*,*,#9407,.T.);
#14429=ORIENTED_EDGE('',*,*,#9406,.T.);
#14430=ORIENTED_EDGE('',*,*,#9412,.T.);
#14431=ORIENTED_EDGE('',*,*,#9411,.T.);
#14432=ORIENTED_EDGE('',*,*,#9417,.T.);
#14433=ORIENTED_EDGE('',*,*,#9416,.T.);
#14434=ORIENTED_EDGE('',*,*,#9422,.T.);
#14435=ORIENTED_EDGE('',*,*,#9421,.T.);
#14436=ORIENTED_EDGE('',*,*,#9427,.T.);
#14437=ORIENTED_EDGE('',*,*,#9426,.T.);
#14438=ORIENTED_EDGE('',*,*,#9432,.T.);
#14439=ORIENTED_EDGE('',*,*,#9431,.T.);
#14440=ORIENTED_EDGE('',*,*,#9437,.T.);
#14441=ORIENTED_EDGE('',*,*,#9436,.T.);
#14442=ORIENTED_EDGE('',*,*,#9442,.T.);
#14443=ORIENTED_EDGE('',*,*,#9441,.T.);
#14444=ORIENTED_EDGE('',*,*,#9447,.T.);
#14445=ORIENTED_EDGE('',*,*,#9446,.T.);
#14446=ORIENTED_EDGE('',*,*,#9452,.T.);
#14447=ORIENTED_EDGE('',*,*,#9451,.T.);
#14448=ORIENTED_EDGE('',*,*,#9457,.T.);
#14449=ORIENTED_EDGE('',*,*,#9456,.T.);
#14450=ORIENTED_EDGE('',*,*,#9462,.T.);
#14451=ORIENTED_EDGE('',*,*,#9461,.T.);
#14452=ORIENTED_EDGE('',*,*,#9467,.T.);
#14453=ORIENTED_EDGE('',*,*,#9466,.T.);
#14454=ORIENTED_EDGE('',*,*,#9472,.T.);
#14455=ORIENTED_EDGE('',*,*,#9471,.T.);
#14456=ORIENTED_EDGE('',*,*,#9477,.T.);
#14457=ORIENTED_EDGE('',*,*,#9476,.T.);
#14458=ORIENTED_EDGE('',*,*,#9482,.T.);
#14459=ORIENTED_EDGE('',*,*,#9481,.T.);
#14460=ORIENTED_EDGE('',*,*,#9487,.T.);
#14461=ORIENTED_EDGE('',*,*,#9486,.T.);
#14462=ORIENTED_EDGE('',*,*,#9492,.T.);
#14463=ORIENTED_EDGE('',*,*,#9491,.T.);
#14464=ORIENTED_EDGE('',*,*,#9497,.T.);
#14465=ORIENTED_EDGE('',*,*,#9496,.T.);
#14466=ORIENTED_EDGE('',*,*,#9502,.T.);
#14467=ORIENTED_EDGE('',*,*,#9501,.T.);
#14468=ORIENTED_EDGE('',*,*,#9507,.T.);
#14469=ORIENTED_EDGE('',*,*,#9506,.T.);
#14470=ORIENTED_EDGE('',*,*,#9512,.T.);
#14471=ORIENTED_EDGE('',*,*,#9511,.T.);
#14472=ORIENTED_EDGE('',*,*,#9517,.T.);
#14473=ORIENTED_EDGE('',*,*,#9516,.T.);
#14474=ORIENTED_EDGE('',*,*,#9522,.T.);
#14475=ORIENTED_EDGE('',*,*,#9521,.T.);
#14476=ORIENTED_EDGE('',*,*,#9527,.T.);
#14477=ORIENTED_EDGE('',*,*,#9526,.T.);
#14478=ORIENTED_EDGE('',*,*,#9532,.T.);
#14479=ORIENTED_EDGE('',*,*,#9531,.T.);
#14480=ORIENTED_EDGE('',*,*,#9638,.T.);
#14481=ORIENTED_EDGE('',*,*,#9637,.T.);
#14482=ORIENTED_EDGE('',*,*,#9648,.F.);
#14483=ORIENTED_EDGE('',*,*,#9635,.F.);
#14484=ORIENTED_EDGE('',*,*,#9634,.F.);
#14485=ORIENTED_EDGE('',*,*,#9534,.F.);
#14486=ORIENTED_EDGE('',*,*,#9533,.F.);
#14487=ORIENTED_EDGE('',*,*,#9529,.F.);
#14488=ORIENTED_EDGE('',*,*,#9528,.F.);
#14489=ORIENTED_EDGE('',*,*,#9524,.F.);
#14490=ORIENTED_EDGE('',*,*,#9523,.F.);
#14491=ORIENTED_EDGE('',*,*,#9519,.F.);
#14492=ORIENTED_EDGE('',*,*,#9518,.F.);
#14493=ORIENTED_EDGE('',*,*,#9514,.F.);
#14494=ORIENTED_EDGE('',*,*,#9513,.F.);
#14495=ORIENTED_EDGE('',*,*,#9509,.F.);
#14496=ORIENTED_EDGE('',*,*,#9508,.F.);
#14497=ORIENTED_EDGE('',*,*,#9504,.F.);
#14498=ORIENTED_EDGE('',*,*,#9503,.F.);
#14499=ORIENTED_EDGE('',*,*,#9499,.F.);
#14500=ORIENTED_EDGE('',*,*,#9498,.F.);
#14501=ORIENTED_EDGE('',*,*,#9494,.F.);
#14502=ORIENTED_EDGE('',*,*,#9493,.F.);
#14503=ORIENTED_EDGE('',*,*,#9489,.F.);
#14504=ORIENTED_EDGE('',*,*,#9488,.F.);
#14505=ORIENTED_EDGE('',*,*,#9484,.F.);
#14506=ORIENTED_EDGE('',*,*,#9483,.F.);
#14507=ORIENTED_EDGE('',*,*,#9479,.F.);
#14508=ORIENTED_EDGE('',*,*,#9478,.F.);
#14509=ORIENTED_EDGE('',*,*,#9474,.F.);
#14510=ORIENTED_EDGE('',*,*,#9473,.F.);
#14511=ORIENTED_EDGE('',*,*,#9469,.F.);
#14512=ORIENTED_EDGE('',*,*,#9468,.F.);
#14513=ORIENTED_EDGE('',*,*,#9464,.F.);
#14514=ORIENTED_EDGE('',*,*,#9463,.F.);
#14515=ORIENTED_EDGE('',*,*,#9459,.F.);
#14516=ORIENTED_EDGE('',*,*,#9458,.F.);
#14517=ORIENTED_EDGE('',*,*,#9454,.F.);
#14518=ORIENTED_EDGE('',*,*,#9453,.F.);
#14519=ORIENTED_EDGE('',*,*,#9449,.F.);
#14520=ORIENTED_EDGE('',*,*,#9448,.F.);
#14521=ORIENTED_EDGE('',*,*,#9444,.F.);
#14522=ORIENTED_EDGE('',*,*,#9443,.F.);
#14523=ORIENTED_EDGE('',*,*,#9439,.F.);
#14524=ORIENTED_EDGE('',*,*,#9438,.F.);
#14525=ORIENTED_EDGE('',*,*,#9434,.F.);
#14526=ORIENTED_EDGE('',*,*,#9433,.F.);
#14527=ORIENTED_EDGE('',*,*,#9429,.F.);
#14528=ORIENTED_EDGE('',*,*,#9428,.F.);
#14529=ORIENTED_EDGE('',*,*,#9424,.F.);
#14530=ORIENTED_EDGE('',*,*,#9423,.F.);
#14531=ORIENTED_EDGE('',*,*,#9419,.F.);
#14532=ORIENTED_EDGE('',*,*,#9418,.F.);
#14533=ORIENTED_EDGE('',*,*,#9414,.F.);
#14534=ORIENTED_EDGE('',*,*,#9413,.F.);
#14535=ORIENTED_EDGE('',*,*,#9409,.F.);
#14536=ORIENTED_EDGE('',*,*,#9408,.F.);
#14537=ORIENTED_EDGE('',*,*,#9404,.F.);
#14538=ORIENTED_EDGE('',*,*,#9403,.F.);
#14539=ORIENTED_EDGE('',*,*,#9399,.F.);
#14540=ORIENTED_EDGE('',*,*,#9398,.F.);
#14541=ORIENTED_EDGE('',*,*,#9394,.F.);
#14542=ORIENTED_EDGE('',*,*,#9393,.F.);
#14543=ORIENTED_EDGE('',*,*,#9389,.F.);
#14544=ORIENTED_EDGE('',*,*,#9388,.F.);
#14545=ORIENTED_EDGE('',*,*,#9384,.F.);
#14546=ORIENTED_EDGE('',*,*,#9383,.F.);
#14547=ORIENTED_EDGE('',*,*,#9379,.F.);
#14548=ORIENTED_EDGE('',*,*,#9378,.F.);
#14549=ORIENTED_EDGE('',*,*,#9374,.F.);
#14550=ORIENTED_EDGE('',*,*,#9373,.F.);
#14551=ORIENTED_EDGE('',*,*,#9369,.F.);
#14552=ORIENTED_EDGE('',*,*,#9368,.F.);
#14553=ORIENTED_EDGE('',*,*,#9364,.F.);
#14554=ORIENTED_EDGE('',*,*,#9363,.F.);
#14555=ORIENTED_EDGE('',*,*,#9359,.F.);
#14556=ORIENTED_EDGE('',*,*,#9358,.F.);
#14557=ORIENTED_EDGE('',*,*,#9354,.F.);
#14558=ORIENTED_EDGE('',*,*,#9353,.F.);
#14559=ORIENTED_EDGE('',*,*,#9349,.F.);
#14560=ORIENTED_EDGE('',*,*,#9348,.F.);
#14561=ORIENTED_EDGE('',*,*,#9344,.F.);
#14562=ORIENTED_EDGE('',*,*,#9343,.F.);
#14563=ORIENTED_EDGE('',*,*,#9339,.F.);
#14564=ORIENTED_EDGE('',*,*,#9338,.F.);
#14565=ORIENTED_EDGE('',*,*,#9334,.F.);
#14566=ORIENTED_EDGE('',*,*,#9333,.F.);
#14567=ORIENTED_EDGE('',*,*,#9329,.F.);
#14568=ORIENTED_EDGE('',*,*,#9328,.F.);
#14569=ORIENTED_EDGE('',*,*,#9324,.F.);
#14570=ORIENTED_EDGE('',*,*,#9323,.F.);
#14571=ORIENTED_EDGE('',*,*,#9319,.F.);
#14572=ORIENTED_EDGE('',*,*,#9318,.F.);
#14573=ORIENTED_EDGE('',*,*,#9314,.F.);
#14574=ORIENTED_EDGE('',*,*,#9313,.F.);
#14575=ORIENTED_EDGE('',*,*,#9309,.F.);
#14576=ORIENTED_EDGE('',*,*,#9308,.F.);
#14577=ORIENTED_EDGE('',*,*,#9304,.F.);
#14578=ORIENTED_EDGE('',*,*,#9303,.F.);
#14579=ORIENTED_EDGE('',*,*,#9299,.F.);
#14580=ORIENTED_EDGE('',*,*,#9298,.F.);
#14581=ORIENTED_EDGE('',*,*,#9294,.F.);
#14582=ORIENTED_EDGE('',*,*,#9293,.F.);
#14583=ORIENTED_EDGE('',*,*,#9289,.F.);
#14584=ORIENTED_EDGE('',*,*,#9288,.F.);
#14585=ORIENTED_EDGE('',*,*,#9284,.F.);
#14586=ORIENTED_EDGE('',*,*,#9283,.F.);
#14587=ORIENTED_EDGE('',*,*,#9279,.F.);
#14588=ORIENTED_EDGE('',*,*,#9278,.F.);
#14589=ORIENTED_EDGE('',*,*,#9274,.F.);
#14590=ORIENTED_EDGE('',*,*,#9273,.F.);
#14591=ORIENTED_EDGE('',*,*,#9269,.F.);
#14592=ORIENTED_EDGE('',*,*,#9268,.F.);
#14593=ORIENTED_EDGE('',*,*,#9264,.F.);
#14594=ORIENTED_EDGE('',*,*,#9263,.F.);
#14595=ORIENTED_EDGE('',*,*,#9259,.F.);
#14596=ORIENTED_EDGE('',*,*,#9258,.F.);
#14597=ORIENTED_EDGE('',*,*,#9254,.F.);
#14598=ORIENTED_EDGE('',*,*,#9253,.F.);
#14599=ORIENTED_EDGE('',*,*,#9249,.F.);
#14600=ORIENTED_EDGE('',*,*,#9248,.F.);
#14601=ORIENTED_EDGE('',*,*,#9244,.F.);
#14602=ORIENTED_EDGE('',*,*,#9243,.F.);
#14603=ORIENTED_EDGE('',*,*,#9239,.F.);
#14604=ORIENTED_EDGE('',*,*,#9238,.F.);
#14605=ORIENTED_EDGE('',*,*,#9234,.F.);
#14606=ORIENTED_EDGE('',*,*,#9233,.F.);
#14607=ORIENTED_EDGE('',*,*,#9229,.F.);
#14608=ORIENTED_EDGE('',*,*,#9228,.F.);
#14609=ORIENTED_EDGE('',*,*,#9224,.F.);
#14610=ORIENTED_EDGE('',*,*,#9223,.F.);
#14611=ORIENTED_EDGE('',*,*,#9219,.F.);
#14612=ORIENTED_EDGE('',*,*,#9218,.F.);
#14613=ORIENTED_EDGE('',*,*,#9214,.F.);
#14614=ORIENTED_EDGE('',*,*,#9649,.F.);
#14615=ORIENTED_EDGE('',*,*,#9535,.F.);
#14616=ORIENTED_EDGE('',*,*,#9633,.F.);
#14617=ORIENTED_EDGE('',*,*,#9632,.F.);
#14618=ORIENTED_EDGE('',*,*,#9631,.F.);
#14619=ORIENTED_EDGE('',*,*,#9630,.F.);
#14620=ORIENTED_EDGE('',*,*,#9629,.F.);
#14621=ORIENTED_EDGE('',*,*,#9628,.F.);
#14622=ORIENTED_EDGE('',*,*,#9627,.F.);
#14623=ORIENTED_EDGE('',*,*,#9626,.F.);
#14624=ORIENTED_EDGE('',*,*,#9625,.F.);
#14625=ORIENTED_EDGE('',*,*,#9624,.F.);
#14626=ORIENTED_EDGE('',*,*,#9623,.F.);
#14627=ORIENTED_EDGE('',*,*,#9622,.F.);
#14628=ORIENTED_EDGE('',*,*,#9621,.F.);
#14629=ORIENTED_EDGE('',*,*,#9620,.F.);
#14630=ORIENTED_EDGE('',*,*,#9619,.F.);
#14631=ORIENTED_EDGE('',*,*,#9618,.F.);
#14632=ORIENTED_EDGE('',*,*,#9617,.F.);
#14633=ORIENTED_EDGE('',*,*,#9616,.F.);
#14634=ORIENTED_EDGE('',*,*,#9615,.F.);
#14635=ORIENTED_EDGE('',*,*,#9614,.F.);
#14636=ORIENTED_EDGE('',*,*,#9613,.F.);
#14637=ORIENTED_EDGE('',*,*,#9612,.F.);
#14638=ORIENTED_EDGE('',*,*,#9611,.F.);
#14639=ORIENTED_EDGE('',*,*,#9610,.F.);
#14640=ORIENTED_EDGE('',*,*,#9609,.F.);
#14641=ORIENTED_EDGE('',*,*,#9608,.F.);
#14642=ORIENTED_EDGE('',*,*,#9607,.F.);
#14643=ORIENTED_EDGE('',*,*,#9606,.F.);
#14644=ORIENTED_EDGE('',*,*,#9605,.F.);
#14645=ORIENTED_EDGE('',*,*,#9604,.F.);
#14646=ORIENTED_EDGE('',*,*,#9603,.F.);
#14647=ORIENTED_EDGE('',*,*,#9602,.F.);
#14648=ORIENTED_EDGE('',*,*,#9601,.F.);
#14649=ORIENTED_EDGE('',*,*,#9600,.F.);
#14650=ORIENTED_EDGE('',*,*,#9599,.F.);
#14651=ORIENTED_EDGE('',*,*,#9598,.F.);
#14652=ORIENTED_EDGE('',*,*,#9597,.F.);
#14653=ORIENTED_EDGE('',*,*,#9596,.F.);
#14654=ORIENTED_EDGE('',*,*,#9595,.F.);
#14655=ORIENTED_EDGE('',*,*,#9594,.F.);
#14656=ORIENTED_EDGE('',*,*,#9593,.F.);
#14657=ORIENTED_EDGE('',*,*,#9592,.F.);
#14658=ORIENTED_EDGE('',*,*,#9591,.F.);
#14659=ORIENTED_EDGE('',*,*,#9590,.F.);
#14660=ORIENTED_EDGE('',*,*,#9589,.F.);
#14661=ORIENTED_EDGE('',*,*,#9588,.F.);
#14662=ORIENTED_EDGE('',*,*,#9587,.F.);
#14663=ORIENTED_EDGE('',*,*,#9648,.T.);
#14664=ORIENTED_EDGE('',*,*,#9586,.T.);
#14665=ORIENTED_EDGE('',*,*,#9646,.T.);
#14666=ORIENTED_EDGE('',*,*,#9636,.T.);
#14667=ORIENTED_EDGE('',*,*,#9650,.F.);
#14668=ORIENTED_EDGE('',*,*,#9651,.F.);
#14669=ORIENTED_EDGE('',*,*,#9652,.F.);
#14670=ORIENTED_EDGE('',*,*,#9653,.T.);
#14671=ORIENTED_EDGE('',*,*,#9650,.T.);
#14672=ORIENTED_EDGE('',*,*,#9653,.F.);
#14673=ORIENTED_EDGE('',*,*,#9651,.T.);
#14674=ORIENTED_EDGE('',*,*,#9654,.T.);
#14675=ORIENTED_EDGE('',*,*,#9643,.T.);
#14676=ORIENTED_EDGE('',*,*,#9645,.T.);
#14677=ORIENTED_EDGE('',*,*,#9655,.T.);
#14678=ORIENTED_EDGE('',*,*,#9656,.T.);
#14679=ORIENTED_EDGE('',*,*,#9655,.F.);
#14680=ORIENTED_EDGE('',*,*,#9644,.T.);
#14681=ORIENTED_EDGE('',*,*,#9654,.F.);
#14682=ORIENTED_EDGE('',*,*,#9640,.T.);
#14683=ORIENTED_EDGE('',*,*,#9639,.T.);
#14684=ORIENTED_EDGE('',*,*,#9641,.T.);
#14685=ORIENTED_EDGE('',*,*,#9652,.T.);
#14686=ORIENTED_EDGE('',*,*,#9536,.T.);
#14687=ORIENTED_EDGE('',*,*,#9649,.T.);
#14688=ORIENTED_EDGE('',*,*,#9213,.T.);
#14689=ORIENTED_EDGE('',*,*,#9647,.T.);
#14690=ORIENTED_EDGE('',*,*,#9656,.F.);
#16047=CYLINDRICAL_SURFACE('',#17585,6.767);
#16048=CYLINDRICAL_SURFACE('',#17587,6.767);
#16049=CYLINDRICAL_SURFACE('',#17588,6.767);
#16050=CYLINDRICAL_SURFACE('',#17589,6.767);
#16051=CYLINDRICAL_SURFACE('',#17590,6.767);
#16052=CYLINDRICAL_SURFACE('',#17591,6.767);
#16053=CYLINDRICAL_SURFACE('',#17592,6.767);
#16054=CYLINDRICAL_SURFACE('',#17593,6.767);
#16055=CYLINDRICAL_SURFACE('',#17594,6.767);
#16056=CYLINDRICAL_SURFACE('',#17595,6.767);
#16057=CYLINDRICAL_SURFACE('',#17596,6.767);
#16058=CYLINDRICAL_SURFACE('',#17597,6.767);
#16059=CYLINDRICAL_SURFACE('',#17598,6.767);
#16060=CYLINDRICAL_SURFACE('',#17599,6.767);
#16061=CYLINDRICAL_SURFACE('',#17600,6.767);
#16062=CYLINDRICAL_SURFACE('',#17601,6.767);
#16063=CYLINDRICAL_SURFACE('',#17602,6.767);
#16064=CYLINDRICAL_SURFACE('',#17603,6.767);
#16065=CYLINDRICAL_SURFACE('',#17604,6.767);
#16066=CYLINDRICAL_SURFACE('',#17605,6.767);
#16067=CYLINDRICAL_SURFACE('',#17606,6.767);
#16068=CYLINDRICAL_SURFACE('',#17607,6.767);
#16069=CYLINDRICAL_SURFACE('',#17608,6.767);
#16070=CYLINDRICAL_SURFACE('',#17609,6.767);
#16071=CYLINDRICAL_SURFACE('',#17610,6.767);
#16072=CYLINDRICAL_SURFACE('',#17611,6.767);
#16073=CYLINDRICAL_SURFACE('',#17612,6.767);
#16074=CYLINDRICAL_SURFACE('',#17613,6.767);
#16075=CYLINDRICAL_SURFACE('',#17614,6.767);
#16076=CYLINDRICAL_SURFACE('',#17615,6.767);
#16077=CYLINDRICAL_SURFACE('',#17616,6.767);
#16078=CYLINDRICAL_SURFACE('',#17617,6.767);
#16079=CYLINDRICAL_SURFACE('',#17618,6.767);
#16080=CYLINDRICAL_SURFACE('',#17619,6.767);
#16081=CYLINDRICAL_SURFACE('',#17620,6.767);
#16082=CYLINDRICAL_SURFACE('',#17621,6.767);
#16083=CYLINDRICAL_SURFACE('',#17622,6.767);
#16084=CYLINDRICAL_SURFACE('',#17623,6.767);
#16085=CYLINDRICAL_SURFACE('',#17624,6.767);
#16086=CYLINDRICAL_SURFACE('',#17625,6.767);
#16087=CYLINDRICAL_SURFACE('',#17626,6.767);
#16088=CYLINDRICAL_SURFACE('',#17627,6.767);
#16089=CYLINDRICAL_SURFACE('',#17628,6.767);
#16090=CYLINDRICAL_SURFACE('',#17629,6.767);
#16091=CYLINDRICAL_SURFACE('',#17630,6.767);
#16092=CYLINDRICAL_SURFACE('',#17631,6.767);
#16093=CYLINDRICAL_SURFACE('',#17632,6.767);
#16094=CYLINDRICAL_SURFACE('',#17633,6.767);
#16095=CYLINDRICAL_SURFACE('',#17634,6.767);
#16096=CYLINDRICAL_SURFACE('',#17635,6.767);
#16097=CYLINDRICAL_SURFACE('',#17636,6.767);
#16098=CYLINDRICAL_SURFACE('',#17637,6.767);
#16099=CYLINDRICAL_SURFACE('',#17638,6.767);
#16100=CYLINDRICAL_SURFACE('',#17639,6.767);
#16101=CYLINDRICAL_SURFACE('',#17640,6.767);
#16102=CYLINDRICAL_SURFACE('',#17641,6.767);
#16103=CYLINDRICAL_SURFACE('',#17642,6.767);
#16104=CYLINDRICAL_SURFACE('',#17643,6.767);
#16105=CYLINDRICAL_SURFACE('',#17644,6.767);
#16106=CYLINDRICAL_SURFACE('',#17645,6.767);
#16107=CYLINDRICAL_SURFACE('',#17646,6.767);
#16108=CYLINDRICAL_SURFACE('',#17647,6.767);
#16109=CYLINDRICAL_SURFACE('',#17648,6.767);
#16110=CYLINDRICAL_SURFACE('',#17649,6.767);
#16111=CYLINDRICAL_SURFACE('',#17650,6.767);
#16112=CYLINDRICAL_SURFACE('',#17651,7.911);
#16113=CYLINDRICAL_SURFACE('',#17654,6.767);
#16114=CYLINDRICAL_SURFACE('',#17656,2.);
#16115=CYLINDRICAL_SURFACE('',#17661,10.);
#16116=CYLINDRICAL_SURFACE('',#17663,6.);
#16634=ADVANCED_FACE('',(#866),#16047,.T.);
#16635=ADVANCED_FACE('',(#867),#16048,.T.);
#16636=ADVANCED_FACE('',(#868),#16049,.T.);
#16637=ADVANCED_FACE('',(#869),#16050,.T.);
#16638=ADVANCED_FACE('',(#870),#16051,.T.);
#16639=ADVANCED_FACE('',(#871),#16052,.T.);
#16640=ADVANCED_FACE('',(#872),#16053,.T.);
#16641=ADVANCED_FACE('',(#873),#16054,.T.);
#16642=ADVANCED_FACE('',(#874),#16055,.T.);
#16643=ADVANCED_FACE('',(#875),#16056,.T.);
#16644=ADVANCED_FACE('',(#876),#16057,.T.);
#16645=ADVANCED_FACE('',(#877),#16058,.T.);
#16646=ADVANCED_FACE('',(#878),#16059,.T.);
#16647=ADVANCED_FACE('',(#879),#16060,.T.);
#16648=ADVANCED_FACE('',(#880),#16061,.T.);
#16649=ADVANCED_FACE('',(#881),#16062,.T.);
#16650=ADVANCED_FACE('',(#882),#16063,.T.);
#16651=ADVANCED_FACE('',(#883),#16064,.T.);
#16652=ADVANCED_FACE('',(#884),#16065,.T.);
#16653=ADVANCED_FACE('',(#885),#16066,.T.);
#16654=ADVANCED_FACE('',(#886),#16067,.T.);
#16655=ADVANCED_FACE('',(#887),#16068,.T.);
#16656=ADVANCED_FACE('',(#888),#16069,.T.);
#16657=ADVANCED_FACE('',(#889),#16070,.T.);
#16658=ADVANCED_FACE('',(#890),#16071,.T.);
#16659=ADVANCED_FACE('',(#891),#16072,.T.);
#16660=ADVANCED_FACE('',(#892),#16073,.T.);
#16661=ADVANCED_FACE('',(#893),#16074,.T.);
#16662=ADVANCED_FACE('',(#894),#16075,.T.);
#16663=ADVANCED_FACE('',(#895),#16076,.T.);
#16664=ADVANCED_FACE('',(#896),#16077,.T.);
#16665=ADVANCED_FACE('',(#897),#16078,.T.);
#16666=ADVANCED_FACE('',(#898),#16079,.T.);
#16667=ADVANCED_FACE('',(#899),#16080,.T.);
#16668=ADVANCED_FACE('',(#900),#16081,.T.);
#16669=ADVANCED_FACE('',(#901),#16082,.T.);
#16670=ADVANCED_FACE('',(#902),#16083,.T.);
#16671=ADVANCED_FACE('',(#903),#16084,.T.);
#16672=ADVANCED_FACE('',(#904),#16085,.T.);
#16673=ADVANCED_FACE('',(#905),#16086,.T.);
#16674=ADVANCED_FACE('',(#906),#16087,.T.);
#16675=ADVANCED_FACE('',(#907),#16088,.T.);
#16676=ADVANCED_FACE('',(#908),#16089,.T.);
#16677=ADVANCED_FACE('',(#909),#16090,.T.);
#16678=ADVANCED_FACE('',(#910),#16091,.T.);
#16679=ADVANCED_FACE('',(#911),#16092,.T.);
#16680=ADVANCED_FACE('',(#912),#16093,.T.);
#16681=ADVANCED_FACE('',(#913),#16094,.T.);
#16682=ADVANCED_FACE('',(#914),#16095,.T.);
#16683=ADVANCED_FACE('',(#915),#16096,.T.);
#16684=ADVANCED_FACE('',(#916),#16097,.T.);
#16685=ADVANCED_FACE('',(#917),#16098,.T.);
#16686=ADVANCED_FACE('',(#918),#16099,.T.);
#16687=ADVANCED_FACE('',(#919),#16100,.T.);
#16688=ADVANCED_FACE('',(#920),#16101,.T.);
#16689=ADVANCED_FACE('',(#921),#16102,.T.);
#16690=ADVANCED_FACE('',(#922),#16103,.T.);
#16691=ADVANCED_FACE('',(#923),#16104,.T.);
#16692=ADVANCED_FACE('',(#924),#16105,.T.);
#16693=ADVANCED_FACE('',(#925),#16106,.T.);
#16694=ADVANCED_FACE('',(#926),#16107,.T.);
#16695=ADVANCED_FACE('',(#927),#16108,.T.);
#16696=ADVANCED_FACE('',(#928),#16109,.T.);
#16697=ADVANCED_FACE('',(#929),#16110,.T.);
#16698=ADVANCED_FACE('',(#930),#16111,.T.);
#16699=ADVANCED_FACE('',(#931),#16112,.T.);
#16700=ADVANCED_FACE('',(#932),#16113,.T.);
#16701=ADVANCED_FACE('',(#933),#16114,.F.);
#16702=ADVANCED_FACE('',(#934),#295,.F.);
#16703=ADVANCED_FACE('',(#935),#296,.F.);
#16704=ADVANCED_FACE('',(#936),#373,.T.);
#16705=ADVANCED_FACE('',(#937,#240),#374,.F.);
#16706=ADVANCED_FACE('',(#938),#16115,.T.);
#16707=ADVANCED_FACE('',(#939,#241),#16116,.T.);
#16708=ADVANCED_FACE('',(#940,#242),#375,.T.);
#16709=ADVANCED_FACE('',(#941),#376,.F.);
#16849=CLOSED_SHELL('',(#16634,#16635,#16636,#16637,#16638,#16639,#16640,
#16641,#16642,#16643,#16644,#16645,#16646,#16647,#16648,#16649,#16650,#16651,
#16652,#16653,#16654,#16655,#16656,#16657,#16658,#16659,#16660,#16661,#16662,
#16663,#16664,#16665,#16666,#16667,#16668,#16669,#16670,#16671,#16672,#16673,
#16674,#16675,#16676,#16677,#16678,#16679,#16680,#16681,#16682,#16683,#16684,
#16685,#16686,#16687,#16688,#16689,#16690,#16691,#16692,#16693,#16694,#16695,
#16696,#16697,#16698,#16699,#16700,#16701,#16702,#16703,#16704,#16705,#16706,
#16707,#16708,#16709));
#17584=AXIS2_PLACEMENT_3D('',#185300,#19398,#19399);
#17585=AXIS2_PLACEMENT_3D('',#185301,#19400,#19401);
#17586=AXIS2_PLACEMENT_3D('',#185440,#19403,#19404);
#17587=AXIS2_PLACEMENT_3D('',#185523,#19405,#19406);
#17588=AXIS2_PLACEMENT_3D('',#186022,#19408,#19409);
#17589=AXIS2_PLACEMENT_3D('',#186518,#19411,#19412);
#17590=AXIS2_PLACEMENT_3D('',#187029,#19414,#19415);
#17591=AXIS2_PLACEMENT_3D('',#187537,#19417,#19418);
#17592=AXIS2_PLACEMENT_3D('',#188030,#19420,#19421);
#17593=AXIS2_PLACEMENT_3D('',#188532,#19423,#19424);
#17594=AXIS2_PLACEMENT_3D('',#189025,#19426,#19427);
#17595=AXIS2_PLACEMENT_3D('',#189527,#19429,#19430);
#17596=AXIS2_PLACEMENT_3D('',#190038,#19432,#19433);
#17597=AXIS2_PLACEMENT_3D('',#190549,#19435,#19436);
#17598=AXIS2_PLACEMENT_3D('',#191048,#19438,#19439);
#17599=AXIS2_PLACEMENT_3D('',#191550,#19441,#19442);
#17600=AXIS2_PLACEMENT_3D('',#192055,#19444,#19445);
#17601=AXIS2_PLACEMENT_3D('',#192563,#19447,#19448);
#17602=AXIS2_PLACEMENT_3D('',#193065,#19450,#19451);
#17603=AXIS2_PLACEMENT_3D('',#193555,#19453,#19454);
#17604=AXIS2_PLACEMENT_3D('',#194042,#19456,#19457);
#17605=AXIS2_PLACEMENT_3D('',#194544,#19459,#19460);
#17606=AXIS2_PLACEMENT_3D('',#195052,#19462,#19463);
#17607=AXIS2_PLACEMENT_3D('',#195566,#19465,#19466);
#17608=AXIS2_PLACEMENT_3D('',#196059,#19468,#19469);
#17609=AXIS2_PLACEMENT_3D('',#196555,#19471,#19472);
#17610=AXIS2_PLACEMENT_3D('',#197060,#19474,#19475);
#17611=AXIS2_PLACEMENT_3D('',#197571,#19477,#19478);
#17612=AXIS2_PLACEMENT_3D('',#198070,#19480,#19481);
#17613=AXIS2_PLACEMENT_3D('',#198557,#19483,#19484);
#17614=AXIS2_PLACEMENT_3D('',#199062,#19486,#19487);
#17615=AXIS2_PLACEMENT_3D('',#199573,#19489,#19490);
#17616=AXIS2_PLACEMENT_3D('',#200084,#19492,#19493);
#17617=AXIS2_PLACEMENT_3D('',#200583,#19495,#19496);
#17618=AXIS2_PLACEMENT_3D('',#201082,#19498,#19499);
#17619=AXIS2_PLACEMENT_3D('',#201575,#19501,#19502);
#17620=AXIS2_PLACEMENT_3D('',#202050,#19504,#19505);
#17621=AXIS2_PLACEMENT_3D('',#202534,#19507,#19508);
#17622=AXIS2_PLACEMENT_3D('',#203030,#19510,#19511);
#17623=AXIS2_PLACEMENT_3D('',#203529,#19513,#19514);
#17624=AXIS2_PLACEMENT_3D('',#204034,#19516,#19517);
#17625=AXIS2_PLACEMENT_3D('',#204533,#19519,#19520);
#17626=AXIS2_PLACEMENT_3D('',#205026,#19522,#19523);
#17627=AXIS2_PLACEMENT_3D('',#205516,#19525,#19526);
#17628=AXIS2_PLACEMENT_3D('',#206015,#19528,#19529);
#17629=AXIS2_PLACEMENT_3D('',#206517,#19531,#19532);
#17630=AXIS2_PLACEMENT_3D('',#207019,#19534,#19535);
#17631=AXIS2_PLACEMENT_3D('',#207515,#19537,#19538);
#17632=AXIS2_PLACEMENT_3D('',#208005,#19540,#19541);
#17633=AXIS2_PLACEMENT_3D('',#208507,#19543,#19544);
#17634=AXIS2_PLACEMENT_3D('',#209000,#19546,#19547);
#17635=AXIS2_PLACEMENT_3D('',#209490,#19549,#19550);
#17636=AXIS2_PLACEMENT_3D('',#209980,#19552,#19553);
#17637=AXIS2_PLACEMENT_3D('',#210467,#19555,#19556);
#17638=AXIS2_PLACEMENT_3D('',#210810,#19558,#19559);
#17639=AXIS2_PLACEMENT_3D('',#211227,#19561,#19562);
#17640=AXIS2_PLACEMENT_3D('',#211732,#19564,#19565);
#17641=AXIS2_PLACEMENT_3D('',#212231,#19567,#19568);
#17642=AXIS2_PLACEMENT_3D('',#212730,#19570,#19571);
#17643=AXIS2_PLACEMENT_3D('',#213238,#19573,#19574);
#17644=AXIS2_PLACEMENT_3D('',#213734,#19576,#19577);
#17645=AXIS2_PLACEMENT_3D('',#214227,#19579,#19580);
#17646=AXIS2_PLACEMENT_3D('',#214705,#19582,#19583);
#17647=AXIS2_PLACEMENT_3D('',#215189,#19585,#19586);
#17648=AXIS2_PLACEMENT_3D('',#215691,#19588,#19589);
#17649=AXIS2_PLACEMENT_3D('',#216199,#19591,#19592);
#17650=AXIS2_PLACEMENT_3D('',#216695,#19594,#19595);
#17651=AXIS2_PLACEMENT_3D('',#217176,#19597,#19598);
#17652=AXIS2_PLACEMENT_3D('',#217188,#19599,#19600);
#17653=AXIS2_PLACEMENT_3D('',#229073,#19601,#19602);
#17654=AXIS2_PLACEMENT_3D('',#241498,#19603,#19604);
#17655=AXIS2_PLACEMENT_3D('',#241666,#19605,#19606);
#17656=AXIS2_PLACEMENT_3D('',#241781,#19607,#19608);
#17657=AXIS2_PLACEMENT_3D('',#247022,#19610,#19611);
#17658=AXIS2_PLACEMENT_3D('',#247023,#19612,#19613);
#17659=AXIS2_PLACEMENT_3D('',#247025,#19614,#19615);
#17660=AXIS2_PLACEMENT_3D('',#247027,#19616,#19617);
#17661=AXIS2_PLACEMENT_3D('',#247028,#19618,#19619);
#17662=AXIS2_PLACEMENT_3D('',#247030,#19620,#19621);
#17663=AXIS2_PLACEMENT_3D('',#247032,#19623,#19624);
#17664=AXIS2_PLACEMENT_3D('',#247036,#19627,#19628);
#17665=AXIS2_PLACEMENT_3D('',#247037,#19629,#19630);
#17666=AXIS2_PLACEMENT_3D('',#247038,#19631,#19632);
#19398=DIRECTION('axis',(0.,0.,1.));
#19399=DIRECTION('refdir',(1.,0.,0.));
#19400=DIRECTION('center_axis',(0.,0.,1.));
#19401=DIRECTION('ref_axis',(-0.457973429632235,-0.888965881094932,0.));
#19402=DIRECTION('',(0.,0.,-1.));
#19403=DIRECTION('center_axis',(0.,0.,-1.));
#19404=DIRECTION('ref_axis',(1.,-1.02558375769811E-12,0.));
#19405=DIRECTION('center_axis',(0.,0.,1.));
#19406=DIRECTION('ref_axis',(-0.457973429632235,-0.888965881094932,0.));
#19407=DIRECTION('',(0.,0.,-1.));
#19408=DIRECTION('center_axis',(0.,0.,1.));
#19409=DIRECTION('ref_axis',(-0.457973429632235,-0.888965881094932,0.));
#19410=DIRECTION('',(0.,0.,-1.));
#19411=DIRECTION('center_axis',(0.,0.,1.));
#19412=DIRECTION('ref_axis',(-0.457973429632235,-0.888965881094932,0.));
#19413=DIRECTION('',(0.,0.,-1.));
#19414=DIRECTION('center_axis',(0.,0.,1.));
#19415=DIRECTION('ref_axis',(-0.457973429632235,-0.888965881094932,0.));
#19416=DIRECTION('',(0.,0.,-1.));
#19417=DIRECTION('center_axis',(0.,0.,1.));
#19418=DIRECTION('ref_axis',(-0.457973429632235,-0.888965881094932,0.));
#19419=DIRECTION('',(0.,0.,-1.));
#19420=DIRECTION('center_axis',(0.,0.,1.));
#19421=DIRECTION('ref_axis',(-0.457973429632235,-0.888965881094932,0.));
#19422=DIRECTION('',(0.,0.,-1.));
#19423=DIRECTION('center_axis',(0.,0.,1.));
#19424=DIRECTION('ref_axis',(-0.457973429632235,-0.888965881094932,0.));
#19425=DIRECTION('',(0.,0.,-1.));
#19426=DIRECTION('center_axis',(0.,0.,1.));
#19427=DIRECTION('ref_axis',(-0.457973429632235,-0.888965881094932,0.));
#19428=DIRECTION('',(0.,0.,-1.));
#19429=DIRECTION('center_axis',(0.,0.,1.));
#19430=DIRECTION('ref_axis',(-0.457973429632235,-0.888965881094932,0.));
#19431=DIRECTION('',(0.,0.,-1.));
#19432=DIRECTION('center_axis',(0.,0.,1.));
#19433=DIRECTION('ref_axis',(-0.457973429632235,-0.888965881094932,0.));
#19434=DIRECTION('',(0.,0.,-1.));
#19435=DIRECTION('center_axis',(0.,0.,1.));
#19436=DIRECTION('ref_axis',(-0.457973429632235,-0.888965881094932,0.));
#19437=DIRECTION('',(0.,0.,-1.));
#19438=DIRECTION('center_axis',(0.,0.,1.));
#19439=DIRECTION('ref_axis',(-0.457973429632235,-0.888965881094932,0.));
#19440=DIRECTION('',(0.,0.,-1.));
#19441=DIRECTION('center_axis',(0.,0.,1.));
#19442=DIRECTION('ref_axis',(-0.457973429632235,-0.888965881094932,0.));
#19443=DIRECTION('',(0.,0.,-1.));
#19444=DIRECTION('center_axis',(0.,0.,1.));
#19445=DIRECTION('ref_axis',(-0.457973429632235,-0.888965881094932,0.));
#19446=DIRECTION('',(0.,0.,-1.));
#19447=DIRECTION('center_axis',(0.,0.,1.));
#19448=DIRECTION('ref_axis',(-0.457973429632235,-0.888965881094932,0.));
#19449=DIRECTION('',(0.,0.,-1.));
#19450=DIRECTION('center_axis',(0.,0.,1.));
#19451=DIRECTION('ref_axis',(-0.457973429632235,-0.888965881094932,0.));
#19452=DIRECTION('',(0.,0.,-1.));
#19453=DIRECTION('center_axis',(0.,0.,1.));
#19454=DIRECTION('ref_axis',(-0.457973429632235,-0.888965881094932,0.));
#19455=DIRECTION('',(0.,0.,-1.));
#19456=DIRECTION('center_axis',(0.,0.,1.));
#19457=DIRECTION('ref_axis',(-0.457973429632235,-0.888965881094932,0.));
#19458=DIRECTION('',(0.,0.,-1.));
#19459=DIRECTION('center_axis',(0.,0.,1.));
#19460=DIRECTION('ref_axis',(-0.457973429632235,-0.888965881094932,0.));
#19461=DIRECTION('',(0.,0.,-1.));
#19462=DIRECTION('center_axis',(0.,0.,1.));
#19463=DIRECTION('ref_axis',(-0.457973429632235,-0.888965881094932,0.));
#19464=DIRECTION('',(0.,0.,-1.));
#19465=DIRECTION('center_axis',(0.,0.,1.));
#19466=DIRECTION('ref_axis',(-0.457973429632235,-0.888965881094932,0.));
#19467=DIRECTION('',(0.,0.,-1.));
#19468=DIRECTION('center_axis',(0.,0.,1.));
#19469=DIRECTION('ref_axis',(-0.457973429632235,-0.888965881094932,0.));
#19470=DIRECTION('',(0.,0.,-1.));
#19471=DIRECTION('center_axis',(0.,0.,1.));
#19472=DIRECTION('ref_axis',(-0.457973429632235,-0.888965881094932,0.));
#19473=DIRECTION('',(0.,0.,-1.));
#19474=DIRECTION('center_axis',(0.,0.,1.));
#19475=DIRECTION('ref_axis',(-0.457973429632235,-0.888965881094932,0.));
#19476=DIRECTION('',(0.,0.,-1.));
#19477=DIRECTION('center_axis',(0.,0.,1.));
#19478=DIRECTION('ref_axis',(-0.457973429632235,-0.888965881094932,0.));
#19479=DIRECTION('',(0.,0.,-1.));
#19480=DIRECTION('center_axis',(0.,0.,1.));
#19481=DIRECTION('ref_axis',(-0.457973429632235,-0.888965881094932,0.));
#19482=DIRECTION('',(0.,0.,-1.));
#19483=DIRECTION('center_axis',(0.,0.,1.));
#19484=DIRECTION('ref_axis',(-0.457973429632235,-0.888965881094932,0.));
#19485=DIRECTION('',(0.,0.,-1.));
#19486=DIRECTION('center_axis',(0.,0.,1.));
#19487=DIRECTION('ref_axis',(-0.457973429632235,-0.888965881094932,0.));
#19488=DIRECTION('',(0.,0.,-1.));
#19489=DIRECTION('center_axis',(0.,0.,1.));
#19490=DIRECTION('ref_axis',(-0.457973429632235,-0.888965881094932,0.));
#19491=DIRECTION('',(0.,0.,-1.));
#19492=DIRECTION('center_axis',(0.,0.,1.));
#19493=DIRECTION('ref_axis',(-0.457973429632235,-0.888965881094932,0.));
#19494=DIRECTION('',(0.,0.,-1.));
#19495=DIRECTION('center_axis',(0.,0.,1.));
#19496=DIRECTION('ref_axis',(-0.457973429632235,-0.888965881094932,0.));
#19497=DIRECTION('',(0.,0.,-1.));
#19498=DIRECTION('center_axis',(0.,0.,1.));
#19499=DIRECTION('ref_axis',(-0.457973429632235,-0.888965881094932,0.));
#19500=DIRECTION('',(0.,0.,-1.));
#19501=DIRECTION('center_axis',(0.,0.,1.));
#19502=DIRECTION('ref_axis',(-0.457973429632235,-0.888965881094932,0.));
#19503=DIRECTION('',(0.,0.,-1.));
#19504=DIRECTION('center_axis',(0.,0.,1.));
#19505=DIRECTION('ref_axis',(-0.457973429632235,-0.888965881094932,0.));
#19506=DIRECTION('',(0.,0.,-1.));
#19507=DIRECTION('center_axis',(0.,0.,1.));
#19508=DIRECTION('ref_axis',(-0.457973429632235,-0.888965881094932,0.));
#19509=DIRECTION('',(0.,0.,-1.));
#19510=DIRECTION('center_axis',(0.,0.,1.));
#19511=DIRECTION('ref_axis',(-0.457973429632235,-0.888965881094932,0.));
#19512=DIRECTION('',(0.,0.,-1.));
#19513=DIRECTION('center_axis',(0.,0.,1.));
#19514=DIRECTION('ref_axis',(-0.457973429632235,-0.888965881094932,0.));
#19515=DIRECTION('',(0.,0.,-1.));
#19516=DIRECTION('center_axis',(0.,0.,1.));
#19517=DIRECTION('ref_axis',(-0.457973429632235,-0.888965881094932,0.));
#19518=DIRECTION('',(0.,0.,-1.));
#19519=DIRECTION('center_axis',(0.,0.,1.));
#19520=DIRECTION('ref_axis',(-0.457973429632235,-0.888965881094932,0.));
#19521=DIRECTION('',(0.,0.,-1.));
#19522=DIRECTION('center_axis',(0.,0.,1.));
#19523=DIRECTION('ref_axis',(-0.457973429632235,-0.888965881094932,0.));
#19524=DIRECTION('',(0.,0.,-1.));
#19525=DIRECTION('center_axis',(0.,0.,1.));
#19526=DIRECTION('ref_axis',(-0.457973429632235,-0.888965881094932,0.));
#19527=DIRECTION('',(0.,0.,-1.));
#19528=DIRECTION('center_axis',(0.,0.,1.));
#19529=DIRECTION('ref_axis',(-0.457973429632235,-0.888965881094932,0.));
#19530=DIRECTION('',(0.,0.,-1.));
#19531=DIRECTION('center_axis',(0.,0.,1.));
#19532=DIRECTION('ref_axis',(-0.457973429632235,-0.888965881094932,0.));
#19533=DIRECTION('',(0.,0.,-1.));
#19534=DIRECTION('center_axis',(0.,0.,1.));
#19535=DIRECTION('ref_axis',(-0.457973429632235,-0.888965881094932,0.));
#19536=DIRECTION('',(0.,0.,-1.));
#19537=DIRECTION('center_axis',(0.,0.,1.));
#19538=DIRECTION('ref_axis',(-0.457973429632235,-0.888965881094932,0.));
#19539=DIRECTION('',(0.,0.,-1.));
#19540=DIRECTION('center_axis',(0.,0.,1.));
#19541=DIRECTION('ref_axis',(-0.457973429632235,-0.888965881094932,0.));
#19542=DIRECTION('',(0.,0.,-1.));
#19543=DIRECTION('center_axis',(0.,0.,1.));
#19544=DIRECTION('ref_axis',(-0.457973429632235,-0.888965881094932,0.));
#19545=DIRECTION('',(0.,0.,-1.));
#19546=DIRECTION('center_axis',(0.,0.,1.));
#19547=DIRECTION('ref_axis',(-0.457973429632235,-0.888965881094932,0.));
#19548=DIRECTION('',(0.,0.,-1.));
#19549=DIRECTION('center_axis',(0.,0.,1.));
#19550=DIRECTION('ref_axis',(-0.457973429632235,-0.888965881094932,0.));
#19551=DIRECTION('',(0.,0.,-1.));
#19552=DIRECTION('center_axis',(0.,0.,1.));
#19553=DIRECTION('ref_axis',(-0.457973429632235,-0.888965881094932,0.));
#19554=DIRECTION('',(0.,0.,-1.));
#19555=DIRECTION('center_axis',(0.,0.,1.));
#19556=DIRECTION('ref_axis',(-0.457973429632235,-0.888965881094932,0.));
#19557=DIRECTION('',(0.,0.,-1.));
#19558=DIRECTION('center_axis',(0.,0.,1.));
#19559=DIRECTION('ref_axis',(-0.457973429632235,-0.888965881094932,0.));
#19560=DIRECTION('',(0.,0.,-1.));
#19561=DIRECTION('center_axis',(0.,0.,1.));
#19562=DIRECTION('ref_axis',(-0.457973429632235,-0.888965881094932,0.));
#19563=DIRECTION('',(0.,0.,-1.));
#19564=DIRECTION('center_axis',(0.,0.,1.));
#19565=DIRECTION('ref_axis',(-0.457973429632235,-0.888965881094932,0.));
#19566=DIRECTION('',(0.,0.,-1.));
#19567=DIRECTION('center_axis',(0.,0.,1.));
#19568=DIRECTION('ref_axis',(-0.457973429632235,-0.888965881094932,0.));
#19569=DIRECTION('',(0.,0.,-1.));
#19570=DIRECTION('center_axis',(0.,0.,1.));
#19571=DIRECTION('ref_axis',(-0.457973429632235,-0.888965881094932,0.));
#19572=DIRECTION('',(0.,0.,-1.));
#19573=DIRECTION('center_axis',(0.,0.,1.));
#19574=DIRECTION('ref_axis',(-0.457973429632235,-0.888965881094932,0.));
#19575=DIRECTION('',(0.,0.,-1.));
#19576=DIRECTION('center_axis',(0.,0.,1.));
#19577=DIRECTION('ref_axis',(-0.457973429632235,-0.888965881094932,0.));
#19578=DIRECTION('',(0.,0.,-1.));
#19579=DIRECTION('center_axis',(0.,0.,1.));
#19580=DIRECTION('ref_axis',(-0.457973429632235,-0.888965881094932,0.));
#19581=DIRECTION('',(0.,0.,-1.));
#19582=DIRECTION('center_axis',(0.,0.,1.));
#19583=DIRECTION('ref_axis',(-0.457973429632235,-0.888965881094932,0.));
#19584=DIRECTION('',(0.,0.,-1.));
#19585=DIRECTION('center_axis',(0.,0.,1.));
#19586=DIRECTION('ref_axis',(-0.457973429632235,-0.888965881094932,0.));
#19587=DIRECTION('',(0.,0.,-1.));
#19588=DIRECTION('center_axis',(0.,0.,1.));
#19589=DIRECTION('ref_axis',(-0.457973429632235,-0.888965881094932,0.));
#19590=DIRECTION('',(0.,0.,-1.));
#19591=DIRECTION('center_axis',(0.,0.,1.));
#19592=DIRECTION('ref_axis',(-0.457973429632235,-0.888965881094932,0.));
#19593=DIRECTION('',(0.,0.,-1.));
#19594=DIRECTION('center_axis',(0.,0.,1.));
#19595=DIRECTION('ref_axis',(-0.457973429632235,-0.888965881094932,0.));
#19596=DIRECTION('',(0.,0.,-1.));
#19597=DIRECTION('center_axis',(0.,0.,1.));
#19598=DIRECTION('ref_axis',(1.,0.,0.));
#19599=DIRECTION('center_axis',(0.,0.,-1.));
#19600=DIRECTION('ref_axis',(1.,0.,0.));
#19601=DIRECTION('center_axis',(0.,0.,-1.));
#19602=DIRECTION('ref_axis',(1.,0.,0.));
#19603=DIRECTION('center_axis',(0.,0.,1.));
#19604=DIRECTION('ref_axis',(-0.457973429632235,-0.888965881094932,0.));
#19605=DIRECTION('center_axis',(0.,0.,1.));
#19606=DIRECTION('ref_axis',(1.,-1.02558375769811E-12,0.));
#19607=DIRECTION('center_axis',(-1.,0.,0.));
#19608=DIRECTION('ref_axis',(0.,1.,0.));
#19609=DIRECTION('',(-1.,0.,0.));
#19610=DIRECTION('center_axis',(0.,0.,1.));
#19611=DIRECTION('ref_axis',(1.,0.,0.));
#19612=DIRECTION('center_axis',(0.,0.,1.));
#19613=DIRECTION('ref_axis',(1.,0.,0.));
#19614=DIRECTION('center_axis',(0.,0.,1.));
#19615=DIRECTION('ref_axis',(1.,0.,0.));
#19616=DIRECTION('center_axis',(0.,0.,-1.));
#19617=DIRECTION('ref_axis',(1.,0.,0.));
#19618=DIRECTION('center_axis',(0.,0.,1.));
#19619=DIRECTION('ref_axis',(1.,0.,0.));
#19620=DIRECTION('center_axis',(0.,0.,1.));
#19621=DIRECTION('ref_axis',(1.,0.,0.));
#19622=DIRECTION('',(0.,0.,-1.));
#19623=DIRECTION('center_axis',(0.,0.,1.));
#19624=DIRECTION('ref_axis',(1.,0.,0.));
#19625=DIRECTION('',(0.,0.,-1.));
#19626=DIRECTION('',(0.,0.,-1.));
#19627=DIRECTION('center_axis',(0.,0.,1.));
#19628=DIRECTION('ref_axis',(1.,0.,0.));
#19629=DIRECTION('center_axis',(0.,0.,1.));
#19630=DIRECTION('ref_axis',(1.,0.,0.));
#19631=DIRECTION('center_axis',(0.,0.,1.));
#19632=DIRECTION('ref_axis',(1.,0.,0.));
#185300=CARTESIAN_POINT('',(0.,0.,0.));
#185301=CARTESIAN_POINT('Origin',(0.,0.,4.30282021618968));
#185302=CARTESIAN_POINT('',(3.09910619832133,6.0156321173694,9.04578901356831));
#185303=CARTESIAN_POINT('',(3.09910619832133,6.0156321173694,8.6514415183394));
#185304=CARTESIAN_POINT('',(3.09910619832133,6.0156321173694,4.30282021618968));
#185305=CARTESIAN_POINT('',(-3.92879376257849,-5.50970675908658,8.00008340518918));
#185306=CARTESIAN_POINT('Ctrl Pts',(-3.92879376257849,-5.50970675908658,
8.00008340518918));
#185307=CARTESIAN_POINT('Ctrl Pts',(-3.78617121598613,-5.61140628611332,
8.00834306925214));
#185308=CARTESIAN_POINT('Ctrl Pts',(-3.63945998519003,-5.7076623902655,
8.01660273331509));
#185309=CARTESIAN_POINT('Ctrl Pts',(-3.48911231632171,-5.79813627332889,
8.02486239737804));
#185310=CARTESIAN_POINT('Ctrl Pts',(-3.33888110786677,-5.88854007465504,
8.03311566344428));
#185311=CARTESIAN_POINT('Ctrl Pts',(-3.18501937441404,-5.97317039562586,
8.04136892951052));
#185312=CARTESIAN_POINT('Ctrl Pts',(-3.02800917015506,-6.05173111311606,
8.04962219557676));
#185313=CARTESIAN_POINT('Ctrl Pts',(-2.87109023696789,-6.13024616274076,
8.05787066396477));
#185314=CARTESIAN_POINT('Ctrl Pts',(-2.71102679497344,-6.20269848060912,
8.06611913235277));
#185315=CARTESIAN_POINT('Ctrl Pts',(-2.54832651194958,-6.26883729159522,
8.07436760074078));
#185316=CARTESIAN_POINT('Ctrl Pts',(-2.38568936503828,-6.33495043730688,
8.08261286829705));
#185317=CARTESIAN_POINT('Ctrl Pts',(-2.22041774337426,-6.39475482519885,
8.09085813585333));
#185318=CARTESIAN_POINT('Ctrl Pts',(-2.05304049370703,-6.44804728047176,
8.0991034034096));
#185319=CARTESIAN_POINT('Ctrl Pts',(-1.88566464369749,-6.50133929009751,
8.10734860201653));
#185320=CARTESIAN_POINT('Ctrl Pts',(-1.71618353484674,-6.54811935906065,
8.11559380062346));
#185321=CARTESIAN_POINT('Ctrl Pts',(-1.54514286689777,-6.58823364194645,
8.12383899923038));
#185322=CARTESIAN_POINT('Ctrl Pts',(-1.37409597703566,-6.62834938406172,
8.1320844977713));
#185323=CARTESIAN_POINT('Ctrl Pts',(-1.20148975947593,-6.6617987752453,
8.14032999631221));
#185324=CARTESIAN_POINT('Ctrl Pts',(-1.02788174576766,-6.68847875953252,
8.14857549485312));
#185325=CARTESIAN_POINT('Ctrl Pts',(-0.854237005138767,-6.71516438799274,
8.15682273773616));
#185326=CARTESIAN_POINT('Ctrl Pts',(-0.679590395912993,-6.73507770216261,
8.16506998061919));
#185327=CARTESIAN_POINT('Ctrl Pts',(-0.504506353298766,-6.74816733191177,
8.17331722350222));
#185328=CARTESIAN_POINT('Ctrl Pts',(-0.329354600483387,-6.76126202380966,
8.18156765583911));
#185329=CARTESIAN_POINT('Ctrl Pts',(-0.153765429952902,-6.76752774692309,
8.189818088176));
#185330=CARTESIAN_POINT('Ctrl Pts',(0.0216948116684557,-6.76696522343263,
8.19806852051288));
#185331=CARTESIAN_POINT('Ctrl Pts',(0.19735801950094,-6.76640204923487,
8.20632849665853));
#185332=CARTESIAN_POINT('Ctrl Pts',(0.37289164614926,-6.75899484888137,
8.21458847280418));
#185333=CARTESIAN_POINT('Ctrl Pts',(0.547731437659107,-6.74479645891556,
8.22284844894983));
#185334=CARTESIAN_POINT('Ctrl Pts',(0.722677486175284,-6.73058944003067,
8.23111344500731));
#185335=CARTESIAN_POINT('Ctrl Pts',(0.896928507983267,-6.70958304496605,
8.23937844106479));
#185336=CARTESIAN_POINT('Ctrl Pts',(1.06992855532672,-6.6818816127268,8.24764343712227));
#185337=CARTESIAN_POINT('Ctrl Pts',(1.24319209235441,-6.65413798950699,
8.25592102127574));
#185338=CARTESIAN_POINT('Ctrl Pts',(1.41520050044158,-6.61967902065648,
8.2641986054292));
#185339=CARTESIAN_POINT('Ctrl Pts',(1.5854098301569,-6.57865979287893,8.27247618958267));
#185340=CARTESIAN_POINT('Ctrl Pts',(1.72771248155696,-6.54436587443809,
8.27939662205364));
#185341=CARTESIAN_POINT('Ctrl Pts',(1.86875779235141,-6.50548745357604,
8.28631705452462));
#185342=CARTESIAN_POINT('Ctrl Pts',(2.00823823124676,-6.4621411472173,8.2932374869956));
#185343=CARTESIAN_POINT('Ctrl Pts',(2.1705257283394,-6.41170709622862,8.30128950972658));
#185344=CARTESIAN_POINT('Ctrl Pts',(2.33121798580858,-6.3550604691712,8.30934153245757));
#185345=CARTESIAN_POINT('Ctrl Pts',(2.48978960024624,-6.29231569030875,
8.31739355518856));
#185346=CARTESIAN_POINT('Ctrl Pts',(2.6481615005552,-6.22964993579682,8.32543543674321));
#185347=CARTESIAN_POINT('Ctrl Pts',(2.80441772782733,-6.16090144600992,
8.33347731829786));
#185348=CARTESIAN_POINT('Ctrl Pts',(2.95804508144256,-6.086235149594,8.34151919985251));
#185349=CARTESIAN_POINT('Ctrl Pts',(3.11151292919324,-6.01164637656101,
8.34955273180509));
#185350=CARTESIAN_POINT('Ctrl Pts',(3.26235700045555,-5.93115218531975,
8.35758626375767));
#185351=CARTESIAN_POINT('Ctrl Pts',(3.41008134960162,-5.84496656868961,
8.36561979571025));
#185352=CARTESIAN_POINT('Ctrl Pts',(3.55768493839698,-5.7588514062896,8.37364676048455));
#185353=CARTESIAN_POINT('Ctrl Pts',(3.70217355859849,-5.66705426565699,
8.38167372525886));
#185354=CARTESIAN_POINT('Ctrl Pts',(3.84307339962506,-5.56983624939678,
8.38970069003316));
#185355=CARTESIAN_POINT('Ctrl Pts',(3.98388912949794,-5.47267626811692,
8.39772286305424));
#185356=CARTESIAN_POINT('Ctrl Pts',(4.12112003699627,-5.37010206484599,
8.40574503607532));
#185357=CARTESIAN_POINT('Ctrl Pts',(4.25431910137204,-5.26241940401001,
8.4137672090964));
#185358=CARTESIAN_POINT('Ctrl Pts',(4.39087135540917,-5.1520259104312,8.42199133449427));
#185359=CARTESIAN_POINT('Ctrl Pts',(4.52318574229823,-5.03626356696928,
8.43021545989213));
#185360=CARTESIAN_POINT('Ctrl Pts',(4.65081416021784,-4.91550777103619,
8.43843958528999));
#185361=CARTESIAN_POINT('Ctrl Pts',(4.77526750401165,-4.79775607567458,
8.4464591151269));
#185362=CARTESIAN_POINT('Ctrl Pts',(4.89526499102733,-4.67525671345183,
8.45447864496381));
#185363=CARTESIAN_POINT('Ctrl Pts',(5.01042671483032,-4.5483967653795,8.46249817480072));
#185364=CARTESIAN_POINT('Ctrl Pts',(5.12560049249289,-4.42152353900644,
8.47051854403359));
#185365=CARTESIAN_POINT('Ctrl Pts',(5.23593724688707,-4.29028909578871,
8.47853891326647));
#185366=CARTESIAN_POINT('Ctrl Pts',(5.34109607102384,-4.15511513199017,
8.48655928249934));
#185367=CARTESIAN_POINT('Ctrl Pts',(5.44628688845443,-4.01990004315647,
8.49458209183206));
#185368=CARTESIAN_POINT('Ctrl Pts',(5.54629640999215,-3.8807433442112,8.50260490116477));
#185369=CARTESIAN_POINT('Ctrl Pts',(5.64082603077095,-3.73809720186311,
8.51062771049748));
#185370=CARTESIAN_POINT('Ctrl Pts',(5.73952354912554,-3.5891616604252,8.51900425284312));
#185371=CARTESIAN_POINT('Ctrl Pts',(5.83224671071703,-3.43642236636971,
8.52738079518875));
#185372=CARTESIAN_POINT('Ctrl Pts',(5.91870864162228,-3.28042329823238,
8.53575733753439));
#185373=CARTESIAN_POINT('Ctrl Pts',(6.00166713683383,-3.1307453091847,8.54379446255339));
#185374=CARTESIAN_POINT('Ctrl Pts',(6.07886173514008,-2.97806688554535,
8.5518315875724));
#185375=CARTESIAN_POINT('Ctrl Pts',(6.15008830340139,-2.82288909813429,
8.5598687125914));
#185376=CARTESIAN_POINT('Ctrl Pts',(6.22136913836607,-2.66759308255128,
8.56791196100354));
#185377=CARTESIAN_POINT('Ctrl Pts',(6.28667274832479,-2.50979425618822,
8.57595520941568));
#185378=CARTESIAN_POINT('Ctrl Pts',(6.3458446220462,-2.35000958143735,8.58399845782782));
#185379=CARTESIAN_POINT('Ctrl Pts',(6.4051010791394,-2.18999650211348,8.59205320368002));
#185380=CARTESIAN_POINT('Ctrl Pts',(6.45820819723198,-2.02799226391842,
8.60010794953221));
#185381=CARTESIAN_POINT('Ctrl Pts',(6.50506220907525,-1.8645253165514,8.6081626953844));
#185382=CARTESIAN_POINT('Ctrl Pts',(6.51084720576157,-1.84434229034639,
8.60915720313797));
#185383=CARTESIAN_POINT('Ctrl Pts',(6.51653694186991,-1.82413697333543,
8.61015171089155));
#185384=CARTESIAN_POINT('Ctrl Pts',(6.52213127688102,-1.80391036560313,
8.61114621864512));
#185385=CARTESIAN_POINT('Ctrl Pts',(6.56888345588548,-1.63487544304732,
8.61945737706236));
#185386=CARTESIAN_POINT('Ctrl Pts',(6.60912320732425,-1.46379381995098,
8.62776853547959));
#185387=CARTESIAN_POINT('Ctrl Pts',(6.64267135078699,-1.29120344076129,
8.63607969389682));
#185388=CARTESIAN_POINT('Ctrl Pts',(6.67617888760101,-1.11882196484241,
8.64438079249389));
#185389=CARTESIAN_POINT('Ctrl Pts',(6.70301088339192,-0.944935711135553,
8.65268189109096));
#185390=CARTESIAN_POINT('Ctrl Pts',(6.7230378912973,-0.770097728980386,
8.66098298968802));
#185391=CARTESIAN_POINT('Ctrl Pts',(6.74304441839381,-0.595438546539786,
8.66927559908817));
#185392=CARTESIAN_POINT('Ctrl Pts',(6.75625978152564,-0.419829920320681,
8.67756820848831));
#185393=CARTESIAN_POINT('Ctrl Pts',(6.76260551695485,-0.243835235459976,
8.68586081788846));
#185394=CARTESIAN_POINT('Ctrl Pts',(6.76894595353476,-0.0679875106046658,
8.69414650275038));
#185395=CARTESIAN_POINT('Ctrl Pts',(6.76842817879555,0.108245282101846,
8.7024321876123));
#185396=CARTESIAN_POINT('Ctrl Pts',(6.7610254959682,0.284294289193273,8.71071787247422));
#185397=CARTESIAN_POINT('Ctrl Pts',(6.75362760620306,0.460229308712769,
8.71899819255099));
#185398=CARTESIAN_POINT('Ctrl Pts',(6.73935370606844,0.635980430749615,
8.72727851262777));
#185399=CARTESIAN_POINT('Ctrl Pts',(6.71822917679434,0.810978253758559,
8.73555883270454));
#185400=CARTESIAN_POINT('Ctrl Pts',(6.6971135375181,0.985902431089819,8.74383566811063));
#185401=CARTESIAN_POINT('Ctrl Pts',(6.66915305511013,1.16007359379113,8.75211250351671));
#185402=CARTESIAN_POINT('Ctrl Pts',(6.6344250344493,1.33292665299801,8.7603893389228));
#185403=CARTESIAN_POINT('Ctrl Pts',(6.59970459738207,1.50574196610449,8.76866436690782));
#185404=CARTESIAN_POINT('Ctrl Pts',(6.55821963485177,1.67723940584398,8.77693939489285));
#185405=CARTESIAN_POINT('Ctrl Pts',(6.51009875741734,1.84686306170035,8.78521442287787));
#185406=CARTESIAN_POINT('Ctrl Pts',(6.46198020926171,2.01647850696694,8.79348905031228));
#185407=CARTESIAN_POINT('Ctrl Pts',(6.4072264819389,2.18422001211556,8.80176367774668));
#185408=CARTESIAN_POINT('Ctrl Pts',(6.34601639486469,2.34954568291588,8.81003830518109));
#185409=CARTESIAN_POINT('Ctrl Pts',(6.28479886740995,2.51489144984675,8.81831393843627));
#185410=CARTESIAN_POINT('Ctrl Pts',(6.21712353870525,2.6778204690414,8.82658957169144));
#185411=CARTESIAN_POINT('Ctrl Pts',(6.14321787351347,2.83780957052172,8.83486520494662));
#185412=CARTESIAN_POINT('Ctrl Pts',(6.06925881749105,2.99791425111225,8.84314681667357));
#185413=CARTESIAN_POINT('Ctrl Pts',(5.98906057847584,3.15507445174475,8.85142842840052));
#185414=CARTESIAN_POINT('Ctrl Pts',(5.90289761555557,3.30878961861712,8.85971004012748));
#185415=CARTESIAN_POINT('Ctrl Pts',(5.81670262731503,3.46256191882476,8.86799472998985));
#185416=CARTESIAN_POINT('Ctrl Pts',(5.7245386747233,3.61288633158087,8.87627941985222));
#185417=CARTESIAN_POINT('Ctrl Pts',(5.62672438706186,3.75929004893787,8.88456410971459));
#185418=CARTESIAN_POINT('Ctrl Pts',(5.52880186651922,3.90585576406153,8.89285796670249));
#185419=CARTESIAN_POINT('Ctrl Pts',(5.42521672004798,4.04849182860883,8.90115182369039));
#185420=CARTESIAN_POINT('Ctrl Pts',(5.31632948052648,4.18675648378133,8.9094456806783));
#185421=CARTESIAN_POINT('Ctrl Pts',(5.23051499394649,4.29572343388429,8.91598210388374));
#185422=CARTESIAN_POINT('Ctrl Pts',(5.14140818171798,4.4019758686728,8.92251852708918));
#185423=CARTESIAN_POINT('Ctrl Pts',(5.0492019292571,4.50531340503482,8.92905495029462));
#185424=CARTESIAN_POINT('Ctrl Pts',(4.9291557516156,4.63985174615666,8.93756492223598));
#185425=CARTESIAN_POINT('Ctrl Pts',(4.80363577572484,4.76969374884127,8.94607489417734));
#185426=CARTESIAN_POINT('Ctrl Pts',(4.67303313686358,4.89438967612663,8.95458486611871));
#185427=CARTESIAN_POINT('Ctrl Pts',(4.54258179068798,5.0189411531781,8.96308497993989));
#185428=CARTESIAN_POINT('Ctrl Pts',(4.40705976086991,5.13835822431179,8.97158509376107));
#185429=CARTESIAN_POINT('Ctrl Pts',(4.26689595798769,5.25222694518319,8.98008520758225));
#185430=CARTESIAN_POINT('Ctrl Pts',(4.12682955979059,5.36601653473343,8.9885794143797));
#185431=CARTESIAN_POINT('Ctrl Pts',(3.98212806882856,5.47426525584026,8.99707362117715));
#185432=CARTESIAN_POINT('Ctrl Pts',(3.83325529781371,5.57659778196197,9.0055678279746));
#185433=CARTESIAN_POINT('Ctrl Pts',(3.6844893612837,5.67885687193658,9.01405593913615));
#185434=CARTESIAN_POINT('Ctrl Pts',(3.53155838193464,5.77520805237895,9.0225440502977));
#185435=CARTESIAN_POINT('Ctrl Pts',(3.3749573045159,5.86531774013095,9.03103216145925));
#185436=CARTESIAN_POINT('Ctrl Pts',(3.28420531444393,5.91753726264669,9.03595111216227));
#185437=CARTESIAN_POINT('Ctrl Pts',(3.19222136425885,5.96766146652434,9.04087006286529));
#185438=CARTESIAN_POINT('Ctrl Pts',(3.09910619832133,6.0156321173694,9.04578901356831));
#185439=CARTESIAN_POINT('',(3.92888236737287,-5.50964357679755,8.));
#185440=CARTESIAN_POINT('Origin',(0.,0.,8.));
#185441=CARTESIAN_POINT('Ctrl Pts',(3.92888236737205,-5.50964357679814,
8.));
#185442=CARTESIAN_POINT('Ctrl Pts',(4.08455174303594,-5.39863700138894,
8.00899352209616));
#185443=CARTESIAN_POINT('Ctrl Pts',(4.23547548564298,-5.28105696228342,
8.01798704419231));
#185444=CARTESIAN_POINT('Ctrl Pts',(4.38113219096226,-5.15732195284667,
8.02698056628847));
#185445=CARTESIAN_POINT('Ctrl Pts',(4.52683306677746,-5.03354942068334,
8.03597681567637));
#185446=CARTESIAN_POINT('Ctrl Pts',(4.66726353054798,-4.90361834910203,
8.04497306506428));
#185447=CARTESIAN_POINT('Ctrl Pts',(4.80193642306303,-4.76798653404775,
8.05396931445219));
#185448=CARTESIAN_POINT('Ctrl Pts',(4.93663304510132,-4.63233082050693,
8.0629671489899));
#185449=CARTESIAN_POINT('Ctrl Pts',(5.06556989731732,-4.49097252926221,
8.07196498352761));
#185450=CARTESIAN_POINT('Ctrl Pts',(5.18829690835927,-4.34440608031865,
8.08096281806532));
#185451=CARTESIAN_POINT('Ctrl Pts',(5.31100285047716,-4.19786479288889,
8.08995910791705));
#185452=CARTESIAN_POINT('Ctrl Pts',(5.42750092637609,-4.04611732175522,
8.09895539776879));
#185453=CARTESIAN_POINT('Ctrl Pts',(5.53738107052083,-3.88969148903067,
8.10795168762053));
#185454=CARTESIAN_POINT('Ctrl Pts',(5.64720908640168,-3.7333398663206,8.11694370954037));
#185455=CARTESIAN_POINT('Ctrl Pts',(5.75042530410842,-3.57231451577492,
8.12593573146022));
#185456=CARTESIAN_POINT('Ctrl Pts',(5.84666223591746,-3.40717327107041,
8.13492775338006));
#185457=CARTESIAN_POINT('Ctrl Pts',(5.93237701301114,-3.26008789841009,
8.14293662419496));
#185458=CARTESIAN_POINT('Ctrl Pts',(6.01255575491793,-3.10973797526773,
8.15094549500986));
#185459=CARTESIAN_POINT('Ctrl Pts',(6.08696823580306,-2.95653626670206,
8.15895436582476));
#185460=CARTESIAN_POINT('Ctrl Pts',(6.16290650334216,-2.80019324206262,
8.16712745409428));
#185461=CARTESIAN_POINT('Ctrl Pts',(6.23286194654829,-2.64083088712788,
8.17530054236379));
#185462=CARTESIAN_POINT('Ctrl Pts',(6.29659359585751,-2.47895100568894,
8.18347363063331));
#185463=CARTESIAN_POINT('Ctrl Pts',(6.36030468714056,-2.31712334211782,
8.19164408249589));
#185464=CARTESIAN_POINT('Ctrl Pts',(6.41779585019016,-2.15278010606025,
8.19981453435846));
#185465=CARTESIAN_POINT('Ctrl Pts',(6.46887395681812,-1.98644373965142,
8.20798498622104));
#185466=CARTESIAN_POINT('Ctrl Pts',(6.51994510918165,-1.82013001987444,
8.21615432567976));
#185467=CARTESIAN_POINT('Ctrl Pts',(6.56460483900829,-1.65182405680871,
8.22432366513848));
#185468=CARTESIAN_POINT('Ctrl Pts',(6.60270966236539,-1.48206413980866,
8.2324930045972));
#185469=CARTESIAN_POINT('Ctrl Pts',(6.64082696565672,-1.31224862374234,
8.24066501964422));
#185470=CARTESIAN_POINT('Ctrl Pts',(6.67238499141571,-1.1409785555763,8.24883703469122));
#185471=CARTESIAN_POINT('Ctrl Pts',(6.69729114048687,-0.968803581514901,
8.25700904973823));
#185472=CARTESIAN_POINT('Ctrl Pts',(6.72220180218756,-0.796597411869245,
8.26518254543471));
#185473=CARTESIAN_POINT('Ctrl Pts',(6.74045814160945,-0.623486369340189,
8.2733560411312));
#185474=CARTESIAN_POINT('Ctrl Pts',(6.75201938147832,-0.450025857191645,
8.28152953682767));
#185475=CARTESIAN_POINT('Ctrl Pts',(6.76358901971194,-0.276439339124579,
8.28970896994945));
#185476=CARTESIAN_POINT('Ctrl Pts',(6.76845382921612,-0.10250320643135,
8.29788840307123));
#185477=CARTESIAN_POINT('Ctrl Pts',(6.76662514637511,0.0712258972851174,
8.306067836193));
#185478=CARTESIAN_POINT('Ctrl Pts',(6.76574272000883,0.155058445100922,
8.31001480134518));
#185479=CARTESIAN_POINT('Ctrl Pts',(6.76330247670826,0.23884281946348,8.31396176649735));
#185480=CARTESIAN_POINT('Ctrl Pts',(6.75931001498592,0.322516854305433,
8.31790873164953));
#185481=CARTESIAN_POINT('Ctrl Pts',(6.74991754506057,0.51936429091016,8.327194168572));
#185482=CARTESIAN_POINT('Ctrl Pts',(6.73192447125622,0.715743860383588,
8.33647960549447));
#185483=CARTESIAN_POINT('Ctrl Pts',(6.7054056754185,0.910946610985172,8.34576504241694));
#185484=CARTESIAN_POINT('Ctrl Pts',(6.6788814416537,1.10618938973627,8.35505238340509));
#185485=CARTESIAN_POINT('Ctrl Pts',(6.64382801984104,1.30025468391843,8.36433972439324));
#185486=CARTESIAN_POINT('Ctrl Pts',(6.6003718822135,1.49244095912886,8.37362706538139));
#185487=CARTESIAN_POINT('Ctrl Pts',(6.55694837666439,1.68448291784108,8.38290743232039));
#185488=CARTESIAN_POINT('Ctrl Pts',(6.50513480897838,1.87464849745314,8.39218779925939));
#185489=CARTESIAN_POINT('Ctrl Pts',(6.44510829319222,2.06224830925495,8.40146816619839));
#185490=CARTESIAN_POINT('Ctrl Pts',(6.38514056272315,2.24966440034135,8.41073944466531));
#185491=CARTESIAN_POINT('Ctrl Pts',(6.31697600347113,2.43451956542231,8.42001072313222));
#185492=CARTESIAN_POINT('Ctrl Pts',(6.24084145515054,2.61613970033608,8.42928200159913));
#185493=CARTESIAN_POINT('Ctrl Pts',(6.16488429767093,2.79733666667287,8.43853167831073));
#185494=CARTESIAN_POINT('Ctrl Pts',(6.08099430017188,2.97531348152076,8.44778135502232));
#185495=CARTESIAN_POINT('Ctrl Pts',(5.9894460394904,3.14941663487585,8.45703103173391));
#185496=CARTESIAN_POINT('Ctrl Pts',(5.92401704556043,3.27384711645205,8.46364172031403));
#185497=CARTESIAN_POINT('Ctrl Pts',(5.85467733362457,3.39629930313006,8.47025240889415));
#185498=CARTESIAN_POINT('Ctrl Pts',(5.78154241060723,3.51654039566589,8.47686309747428));
#185499=CARTESIAN_POINT('Ctrl Pts',(5.69008649737165,3.66690301960275,8.48512982609403));
#185500=CARTESIAN_POINT('Ctrl Pts',(5.59273632757111,3.81373627669594,8.49339655471379));
#185501=CARTESIAN_POINT('Ctrl Pts',(5.48980022029091,3.95656195974408,8.50166328333354));
#185502=CARTESIAN_POINT('Ctrl Pts',(5.38687329625559,4.09937490087632,8.50992927445316));
#185503=CARTESIAN_POINT('Ctrl Pts',(5.27836163360689,4.23818069531259,8.51819526557278));
#185504=CARTESIAN_POINT('Ctrl Pts',(5.16461605766672,4.37253130084749,8.5264612566924));
#185505=CARTESIAN_POINT('Ctrl Pts',(5.05086105281971,4.50689304333724,8.53472793301897));
#185506=CARTESIAN_POINT('Ctrl Pts',(4.93187149831131,4.63679859343608,8.54299460934555));
#185507=CARTESIAN_POINT('Ctrl Pts',(4.80803765128304,4.76183398953016,8.55126128567213));
#185508=CARTESIAN_POINT('Ctrl Pts',(4.68412876548718,4.88694515248648,8.55953297130124));
#185509=CARTESIAN_POINT('Ctrl Pts',(4.55536997067134,5.00718001583141,8.56780465693035));
#185510=CARTESIAN_POINT('Ctrl Pts',(4.42218796782023,5.12216190463227,8.57607634255946));
#185511=CARTESIAN_POINT('Ctrl Pts',(4.28896000624874,5.23718347162058,8.58435088259892));
#185512=CARTESIAN_POINT('Ctrl Pts',(4.15130606590586,5.34694822772878,8.59262542263838));
#185513=CARTESIAN_POINT('Ctrl Pts',(4.00968498910448,5.45112055344131,8.60089996267783));
#185514=CARTESIAN_POINT('Ctrl Pts',(3.86793510529871,5.55538762582232,8.60918202856541));
#185515=CARTESIAN_POINT('Ctrl Pts',(3.7222111669496,5.65405190789338,8.61746409445299));
#185516=CARTESIAN_POINT('Ctrl Pts',(3.57300063748498,5.74682133396645,8.62574616034057));
#185517=CARTESIAN_POINT('Ctrl Pts',(3.51251876950539,5.78442503526304,8.62910326132673));
#185518=CARTESIAN_POINT('Ctrl Pts',(3.45146432374767,5.82106070438347,8.63246036231289));
#185519=CARTESIAN_POINT('Ctrl Pts',(3.38987086665649,5.85671106572568,8.63581746329905));
#185520=CARTESIAN_POINT('Ctrl Pts',(3.29431822886113,5.91201703855918,8.64102548164583));
#185521=CARTESIAN_POINT('Ctrl Pts',(3.19735717007827,5.96501562526646,8.64623349999262));
#185522=CARTESIAN_POINT('Ctrl Pts',(3.09910619832133,6.0156321173694,8.6514415183394));
#185523=CARTESIAN_POINT('Origin',(0.,0.,4.30282021618968));
#185524=CARTESIAN_POINT('',(3.09910619832133,6.01563211736941,11.0457552630241));
#185525=CARTESIAN_POINT('',(3.09910619832133,6.01563211736941,10.651525285013));
#185526=CARTESIAN_POINT('',(3.09910619832133,6.0156321173694,4.30282021618968));
#185527=CARTESIAN_POINT('',(-6.767,9.95106571471428E-13,9.69717978381004));
#185528=CARTESIAN_POINT('Ctrl Pts',(-6.767,9.95106540770597E-13,9.69717978381004));
#185529=CARTESIAN_POINT('Ctrl Pts',(-6.76700000000003,-0.186007249525989,
9.70592929562122));
#185530=CARTESIAN_POINT('Ctrl Pts',(-6.75932637294525,-0.372014355749146,
9.71467880743241));
#185531=CARTESIAN_POINT('Ctrl Pts',(-6.74400518264186,-0.557389537486834,
9.7234283192436));
#185532=CARTESIAN_POINT('Ctrl Pts',(-6.72868405705092,-0.742763936251198,
9.73217779409927));
#185533=CARTESIAN_POINT('Ctrl Pts',(-6.70571545645732,-0.927506130241735,
9.74092726895495));
#185534=CARTESIAN_POINT('Ctrl Pts',(-6.67517739404809,-1.11098863990114,
9.74967674381062));
#185535=CARTESIAN_POINT('Ctrl Pts',(-6.64463945808679,-1.29447038982067,
9.75842618243764));
#185536=CARTESIAN_POINT('Ctrl Pts',(-6.60653217008324,-1.47669218313825,
9.76717562106466));
#185537=CARTESIAN_POINT('Ctrl Pts',(-6.56098496092636,-1.65703510599448,
9.77592505969168));
#185538=CARTESIAN_POINT('Ctrl Pts',(-6.51543793658249,-1.83737729708868,
9.78467446281685));
#185539=CARTESIAN_POINT('Ctrl Pts',(-6.46245112167367,-2.01584035511099,
9.79342386594202));
#185540=CARTESIAN_POINT('Ctrl Pts',(-6.40220448374193,-2.19181813760969,
9.80217326906719));
#185541=CARTESIAN_POINT('Ctrl Pts',(-6.34195808526434,-2.3677952206733,
9.8109226374173));
#185542=CARTESIAN_POINT('Ctrl Pts',(-6.27445201433025,-2.54128677684361,
9.8196720057674));
#185543=CARTESIAN_POINT('Ctrl Pts',(-6.19991555071813,-2.71170355385015,
9.8284213741175));
#185544=CARTESIAN_POINT('Ctrl Pts',(-6.12537937716595,-2.88211966767684,
9.83717070841928));
#185545=CARTESIAN_POINT('Ctrl Pts',(-6.04381298052414,-3.04946076371996,
9.84592004272107));
#185546=CARTESIAN_POINT('Ctrl Pts',(-5.95549339335716,-3.2131584837476,
9.85466937702285));
#185547=CARTESIAN_POINT('Ctrl Pts',(-5.86717414255289,-3.37685558033701,
9.86341867800303));
#185548=CARTESIAN_POINT('Ctrl Pts',(-5.77210188876474,-3.53690907646959,
9.87216797898322));
#185549=CARTESIAN_POINT('Ctrl Pts',(-5.67059953346867,-3.69277536969484,
9.88091727996341));
#185550=CARTESIAN_POINT('Ctrl Pts',(-5.56909755631257,-3.84864108225107,
9.88966654834868));
#185551=CARTESIAN_POINT('Ctrl Pts',(-5.46116568196725,-4.00031938297687,
9.89841581673395));
#185552=CARTESIAN_POINT('Ctrl Pts',(-5.34717048533482,-4.1472951186001,
9.90716508511923));
#185553=CARTESIAN_POINT('Ctrl Pts',(-5.23317570391725,-4.29427031888051,
9.91591432163626));
#185554=CARTESIAN_POINT('Ctrl Pts',(-5.11311782003413,-4.43654276189662,
9.92466355815329));
#185555=CARTESIAN_POINT('Ctrl Pts',(-4.98740458984665,-4.57362924351948,
9.93341279467033));
#185556=CARTESIAN_POINT('Ctrl Pts',(-4.86169180711645,-4.71071523720369,
9.94216200004577));
#185557=CARTESIAN_POINT('Ctrl Pts',(-4.73032391204063,-4.84261509523345,
9.95091120542122));
#185558=CARTESIAN_POINT('Ctrl Pts',(-4.59374707013479,-4.96888084538441,
9.95966041079667));
#185559=CARTESIAN_POINT('Ctrl Pts',(-4.45717070301335,-5.09514615659559,
9.9684095857571));
#185560=CARTESIAN_POINT('Ctrl Pts',(-4.31538563570942,-5.21577720459608,
9.97715876071754));
#185561=CARTESIAN_POINT('Ctrl Pts',(-4.16887341029423,-5.33036429232954,
9.98590793567797));
#185562=CARTESIAN_POINT('Ctrl Pts',(-4.02236168203631,-5.44495099123671,
9.99465708094999));
#185563=CARTESIAN_POINT('Ctrl Pts',(-3.87112305348101,-5.55349359438646,
10.003406226222));
#185564=CARTESIAN_POINT('Ctrl Pts',(-3.71567117017709,-5.65562346298928,
10.012155371494));
#185565=CARTESIAN_POINT('Ctrl Pts',(-3.56021980145775,-5.75775299351671,
10.0209044878042));
#185566=CARTESIAN_POINT('Ctrl Pts',(-3.40055544538315,-5.85346967463892,
10.0296536041143));
#185567=CARTESIAN_POINT('Ctrl Pts',(-3.23722035986829,-5.94244842986914,
10.0384027204245));
#185568=CARTESIAN_POINT('Ctrl Pts',(-3.07388580147158,-6.0314268979454,
10.0471518084993));
#185569=CARTESIAN_POINT('Ctrl Pts',(-2.90688078896558,-6.11366734656791,
10.0559008965742));
#185570=CARTESIAN_POINT('Ctrl Pts',(-2.73677250721353,-6.18889046952361,
10.064649984649));
#185571=CARTESIAN_POINT('Ctrl Pts',(-2.56666476031449,-6.26411335596341,
10.0733990452151));
#185572=CARTESIAN_POINT('Ctrl Pts',(-2.39345402575116,-6.33231884500575,
10.0821481057811));
#185573=CARTESIAN_POINT('Ctrl Pts',(-2.21772856065524,-6.3932752976275,
10.0908971663471));
#185574=CARTESIAN_POINT('Ctrl Pts',(-2.04200363348448,-6.45423156365132,
10.0996462001308));
#185575=CARTESIAN_POINT('Ctrl Pts',(-1.86376426189216,-6.50793874375676,
10.1083952339145));
#185576=CARTESIAN_POINT('Ctrl Pts',(-1.68361577753094,-6.55421443909557,
10.1171442676982));
#185577=CARTESIAN_POINT('Ctrl Pts',(-1.50346782967715,-6.60048999661888,
10.125893275426));
#185578=CARTESIAN_POINT('Ctrl Pts',(-1.32141105794878,-6.63933404237735,
10.1346422831539));
#185579=CARTESIAN_POINT('Ctrl Pts',(-1.13806375486889,-6.67061465607584,
10.1433912908817));
#185580=CARTESIAN_POINT('Ctrl Pts',(-0.954716982602104,-6.70189517921308,
10.1521402732801));
#185581=CARTESIAN_POINT('Ctrl Pts',(-0.770079968901649,-6.72561226592233,
10.1608892556785));
#185582=CARTESIAN_POINT('Ctrl Pts',(-0.584779765558184,-6.74168536983103,
10.1696382380769));
#185583=CARTESIAN_POINT('Ctrl Pts',(-0.391489830651259,-6.75845151013853,
10.1787644570867));
#185584=CARTESIAN_POINT('Ctrl Pts',(-0.197478578238317,-6.76689983031625,
10.1878906760966));
#185585=CARTESIAN_POINT('Ctrl Pts',(-0.00346287645134736,-6.76699911397118,
10.1970168951065));
#185586=CARTESIAN_POINT('Ctrl Pts',(0.184489834654779,-6.76709529501189,
10.2058579197723));
#185587=CARTESIAN_POINT('Ctrl Pts',(0.372446404250258,-6.75935639738163,
10.2146989444381));
#185588=CARTESIAN_POINT('Ctrl Pts',(0.559755019489222,-6.74380925873179,
10.2235399691039));
#185589=CARTESIAN_POINT('Ctrl Pts',(0.745134705522643,-6.72842222659796,
10.2322899477137));
#185590=CARTESIAN_POINT('Ctrl Pts',(0.929879431229419,-6.70538706057512,
10.2410399263234));
#185591=CARTESIAN_POINT('Ctrl Pts',(1.11336163626909,-6.67478200894113,
10.2497899049331));
#185592=CARTESIAN_POINT('Ctrl Pts',(1.29684196300825,-6.64417727060993,
10.2585397939697));
#185593=CARTESIAN_POINT('Ctrl Pts',(1.47905951217638,-6.60600284890562,
10.2672896830062));
#185594=CARTESIAN_POINT('Ctrl Pts',(1.65939532067234,-6.56038841607193,
10.2760395720427));
#185595=CARTESIAN_POINT('Ctrl Pts',(1.83972934300957,-6.51477443503213,
10.2847893744149));
#185596=CARTESIAN_POINT('Ctrl Pts',(2.01818138406424,-6.46172066062091,
10.2935391767871));
#185597=CARTESIAN_POINT('Ctrl Pts',(2.19414528354364,-6.40140730423422,
10.3022889791592));
#185598=CARTESIAN_POINT('Ctrl Pts',(2.37010749864153,-6.34109452518585,
10.3110386977755));
#185599=CARTESIAN_POINT('Ctrl Pts',(2.54358134866603,-6.27352239616446,
10.3197884163918));
#185600=CARTESIAN_POINT('Ctrl Pts',(2.71397759435689,-6.19892043966761,
10.3285381350082));
#185601=CARTESIAN_POINT('Ctrl Pts',(2.88437226558249,-6.12431917249456,
10.3372877727769));
#185602=CARTESIAN_POINT('Ctrl Pts',(3.05168912681073,-6.04268832278739,
10.3460374105456));
#185603=CARTESIAN_POINT('Ctrl Pts',(3.21535986273964,-5.95430516123275,
10.3547870483143));
#185604=CARTESIAN_POINT('Ctrl Pts',(3.3790291407296,-5.86592278697373,10.3635366081434));
#185605=CARTESIAN_POINT('Ctrl Pts',(3.53905210621699,-5.77078835741864,
10.3722861679724));
#185606=CARTESIAN_POINT('Ctrl Pts',(3.69488522831832,-5.66922500431541,
10.3810357278015));
#185607=CARTESIAN_POINT('Ctrl Pts',(3.85071701407077,-5.56766252216998,
10.3897852125986));
#185608=CARTESIAN_POINT('Ctrl Pts',(4.00235878822544,-5.45967138329268,
10.3985346973957));
#185609=CARTESIAN_POINT('Ctrl Pts',(4.14929549611466,-5.34561838199498,
10.4072841821929));
#185610=CARTESIAN_POINT('Ctrl Pts',(4.29623099276228,-5.23156632086902,
10.4160335948654));
#185611=CARTESIAN_POINT('Ctrl Pts',(4.43846127436164,-5.11145267304846,
10.424783007538));
#185612=CARTESIAN_POINT('Ctrl Pts',(4.57550326054575,-4.98568540049763,
10.4335324202106));
#185613=CARTESIAN_POINT('Ctrl Pts',(4.71254416257903,-4.85991912290241,
10.4422817636659));
#185614=CARTESIAN_POINT('Ctrl Pts',(4.84439664018874,-4.72849950385303,
10.4510311071211));
#185615=CARTESIAN_POINT('Ctrl Pts',(4.97061286794848,-4.59187289860957,
10.4597804505764));
#185616=CARTESIAN_POINT('Ctrl Pts',(5.09682813912776,-4.4552473288458,10.4685297277212));
#185617=CARTESIAN_POINT('Ctrl Pts',(5.21740705147919,-4.31341506235689,
10.477279004866));
#185618=CARTESIAN_POINT('Ctrl Pts',(5.33194007545767,-4.16685781275633,
10.4860282820108));
#185619=CARTESIAN_POINT('Ctrl Pts',(5.44647226944537,-4.0203016252177,10.4947774957519));
#185620=CARTESIAN_POINT('Ctrl Pts',(5.55495848628148,-3.86902074887883,
10.503526709493));
#185621=CARTESIAN_POINT('Ctrl Pts',(5.65703027291807,-3.71352898080634,
10.5122759232341));
#185622=CARTESIAN_POINT('Ctrl Pts',(5.7591013537701,-3.55803828789568,10.521025076478));
#185623=CARTESIAN_POINT('Ctrl Pts',(5.85475793592759,-3.398337001067,10.5297742297219));
#185624=CARTESIAN_POINT('Ctrl Pts',(5.943675144274,-3.23496750823551,10.5385233829658));
#185625=CARTESIAN_POINT('Ctrl Pts',(6.03259176732643,-3.0715990907772,10.5472724786187));
#185626=CARTESIAN_POINT('Ctrl Pts',(6.11476896835928,-2.90456276731427,
10.5560215742716));
#185627=CARTESIAN_POINT('Ctrl Pts',(6.18992765547891,-2.7344258300304,10.5647706699246));
#185628=CARTESIAN_POINT('Ctrl Pts',(6.26508587283059,-2.56428995616159,
10.5735197108926));
#185629=CARTESIAN_POINT('Ctrl Pts',(6.33322554827165,-2.39105376935189,
10.5822687518606));
#185630=CARTESIAN_POINT('Ctrl Pts',(6.39411526733035,-2.21530561054066,
10.5910177928287));
#185631=CARTESIAN_POINT('Ctrl Pts',(6.45500462602846,-2.03955849185101,
10.5997667820177));
#185632=CARTESIAN_POINT('Ctrl Pts',(6.50864402040734,-1.86129970164564,
10.6085157712067));
#185633=CARTESIAN_POINT('Ctrl Pts',(6.55485128368592,-1.68113463136095,
10.6172647603957));
#185634=CARTESIAN_POINT('Ctrl Pts',(6.60199809554315,-1.49730620116918,
10.6261916458672));
#185635=CARTESIAN_POINT('Ctrl Pts',(6.64140720707861,-1.31149343245761,
10.6351185313386));
#185636=CARTESIAN_POINT('Ctrl Pts',(6.67293928722871,-1.12435326697601,
10.64404541681));
#185637=CARTESIAN_POINT('Ctrl Pts',(6.70384625876246,-0.940923067007366,
10.6527953309875));
#185638=CARTESIAN_POINT('Ctrl Pts',(6.72718554579787,-0.756217899522463,
10.6615452451649));
#185639=CARTESIAN_POINT('Ctrl Pts',(6.74287786815321,-0.570865181255318,
10.6702951593424));
#185640=CARTESIAN_POINT('Ctrl Pts',(6.75856988190841,-0.385516108074804,
10.6790449014469));
#185641=CARTESIAN_POINT('Ctrl Pts',(6.766615207734,-0.199519795227242,10.6877946435514));
#185642=CARTESIAN_POINT('Ctrl Pts',(6.76698651789579,-0.0135080204565767,
10.6965443856558));
#185643=CARTESIAN_POINT('Ctrl Pts',(6.76735782124905,0.172500343511997,
10.7052939673208));
#185644=CARTESIAN_POINT('Ctrl Pts',(6.76005538995189,0.358523882209922,
10.7140435489858));
#185645=CARTESIAN_POINT('Ctrl Pts',(6.74510402742369,0.543930748563345,
10.7227931306508));
#185646=CARTESIAN_POINT('Ctrl Pts',(6.73015291918042,0.729334461614151,
10.7315425635074));
#185647=CARTESIAN_POINT('Ctrl Pts',(6.7075531630661,0.914121237633547,10.7402919963641));
#185648=CARTESIAN_POINT('Ctrl Pts',(6.67738151874594,1.09766345166003,10.7490414292208));
#185649=CARTESIAN_POINT('Ctrl Pts',(6.64721034747591,1.28120278799551,10.7577907248983));
#185650=CARTESIAN_POINT('Ctrl Pts',(6.60946757205166,1.4634973186022,10.7665400205758));
#185651=CARTESIAN_POINT('Ctrl Pts',(6.56428138111549,1.64392790278058,10.7752893162534));
#185652=CARTESIAN_POINT('Ctrl Pts',(6.51909583859879,1.82435589778951,10.784038486379));
#185653=CARTESIAN_POINT('Ctrl Pts',(6.46646716392908,2.00291972192159,10.7927876565046));
#185654=CARTESIAN_POINT('Ctrl Pts',(6.4065740987292,2.17901292274557,10.8015368266302));
#185655=CARTESIAN_POINT('Ctrl Pts',(6.34668181342117,2.35510383058867,10.8102858828293));
#185656=CARTESIAN_POINT('Ctrl Pts',(6.27952541914095,2.52872390822468,10.8190349390284));
#185657=CARTESIAN_POINT('Ctrl Pts',(6.20533299175567,2.6992835089017,10.8277839952275));
#185658=CARTESIAN_POINT('Ctrl Pts',(6.12831602991598,2.87633637965519,10.8368661313857));
#185659=CARTESIAN_POINT('Ctrl Pts',(6.04371690605318,3.05009086601368,10.8459482675439));
#185660=CARTESIAN_POINT('Ctrl Pts',(5.95184520316677,3.2199111288265,10.8550304037021));
#185661=CARTESIAN_POINT('Ctrl Pts',(5.8633354950932,3.38351691182938,10.8637801840457));
#185662=CARTESIAN_POINT('Ctrl Pts',(5.76807618099414,3.5434710371193,10.8725299643892));
#185663=CARTESIAN_POINT('Ctrl Pts',(5.66639083309061,3.69923018027626,10.8812797447328));
#185664=CARTESIAN_POINT('Ctrl Pts',(5.56470914082247,3.85498372381983,10.8900292105177));
#185665=CARTESIAN_POINT('Ctrl Pts',(5.45660203372114,4.00654234701933,10.8987786763026));
#185666=CARTESIAN_POINT('Ctrl Pts',(5.34243669839265,4.15339127986607,10.9075281420875));
#185667=CARTESIAN_POINT('Ctrl Pts',(5.22827486050639,4.30023571401221,10.9162773398335));
#185668=CARTESIAN_POINT('Ctrl Pts',(5.10805534167158,4.44237052028415,10.9250265375796));
#185669=CARTESIAN_POINT('Ctrl Pts',(4.98218644339998,4.5793129662867,10.9337757353256));
#185670=CARTESIAN_POINT('Ctrl Pts',(4.85632073219634,4.71625194483312,10.9425247115372));
#185671=CARTESIAN_POINT('Ctrl Pts',(4.72480612170366,4.84799861524462,10.9512736877488));
#185672=CARTESIAN_POINT('Ctrl Pts',(4.58808925235359,4.97410554898441,10.9600226639605));
#185673=CARTESIAN_POINT('Ctrl Pts',(4.45136349474098,5.10022068121163,10.9687722089622));
#185674=CARTESIAN_POINT('Ctrl Pts',(4.30943501210132,5.22069514871791,10.9775217539639));
#185675=CARTESIAN_POINT('Ctrl Pts',(4.16278587431836,5.33511975166214,10.9862712989656));
#185676=CARTESIAN_POINT('Ctrl Pts',(4.01614535740492,5.4495376280781,10.9950203296193));
#185677=CARTESIAN_POINT('Ctrl Pts',(3.86478496657957,5.55790617532761,11.0037693602731));
#185678=CARTESIAN_POINT('Ctrl Pts',(3.70921874747218,5.65985735539341,11.0125183909268));
#185679=CARTESIAN_POINT('Ctrl Pts',(3.55365041605934,5.76180991977025,11.0212675403764));
#185680=CARTESIAN_POINT('Ctrl Pts',(3.39387638174568,5.85734478552786,11.030016689826));
#185681=CARTESIAN_POINT('Ctrl Pts',(3.23043927904597,5.94613749121201,11.0387658392756));
#185682=CARTESIAN_POINT('Ctrl Pts',(3.18691767070467,5.96978206944128,11.0410956471918));
#185683=CARTESIAN_POINT('Ctrl Pts',(3.14313645919646,5.99294880633417,11.043425455108));
#185684=CARTESIAN_POINT('Ctrl Pts',(3.09910619832133,6.01563211736941,11.0457552630241));
#185685=CARTESIAN_POINT('Ctrl Pts',(3.09910619832133,6.0156321173694,9.04578901356831));
#185686=CARTESIAN_POINT('Ctrl Pts',(2.93854643732489,6.09834857023698,9.05427082790305));
#185687=CARTESIAN_POINT('Ctrl Pts',(2.77462202131184,6.17465935559691,9.06275264223778));
#185688=CARTESIAN_POINT('Ctrl Pts',(2.6078694041067,6.244301896219,9.07123445657252));
#185689=CARTESIAN_POINT('Ctrl Pts',(2.49793806071349,6.29021360768847,9.07682607642148));
#185690=CARTESIAN_POINT('Ctrl Pts',(2.38677808018559,6.33322817998522,9.08241769627043));
#185691=CARTESIAN_POINT('Ctrl Pts',(2.27454838086761,6.3732816243355,9.08800931611939));
#185692=CARTESIAN_POINT('Ctrl Pts',(2.10237858916949,6.43472697447443,9.09658733094523));
#185693=CARTESIAN_POINT('Ctrl Pts',(1.92776963553591,6.48917305710021,9.10516534577107));
#185694=CARTESIAN_POINT('Ctrl Pts',(1.75130881270765,6.53645212959848,9.11374336059692));
#185695=CARTESIAN_POINT('Ctrl Pts',(1.57475862025023,6.58375514686313,9.12232571980919));
#185696=CARTESIAN_POINT('Ctrl Pts',(1.39635498702721,6.62388383109445,9.13090807902146));
#185697=CARTESIAN_POINT('Ctrl Pts',(1.21669707763909,6.65672120651485,9.13949043823373));
#185698=CARTESIAN_POINT('Ctrl Pts',(1.02921542872602,6.69098858339106,9.14844654187627));
#185699=CARTESIAN_POINT('Ctrl Pts',(0.840368190626526,6.717315330712,9.1574026455188));
#185700=CARTESIAN_POINT('Ctrl Pts',(0.650843588111725,6.7356285247788,9.16635874916134));
#185701=CARTESIAN_POINT('Ctrl Pts',(0.468914041976044,6.75320783132086,
9.17495594366384));
#185702=CARTESIAN_POINT('Ctrl Pts',(0.286360676529203,6.763403362385,9.18355313816635));
#185703=CARTESIAN_POINT('Ctrl Pts',(0.103793877473092,6.76620394541867,
9.19215033266886));
#185704=CARTESIAN_POINT('Ctrl Pts',(-0.0788866154034073,6.76900627252073,
9.20075288109055));
#185705=CARTESIAN_POINT('Ctrl Pts',(-0.261580248477637,6.76440446413929,
9.20935542951224));
#185706=CARTESIAN_POINT('Ctrl Pts',(-0.443678625344181,6.75243943159898,
9.21795797793393));
#185707=CARTESIAN_POINT('Ctrl Pts',(-0.625968327623834,6.7404618277506,
9.22656956480044));
#185708=CARTESIAN_POINT('Ctrl Pts',(-0.807661215189427,6.72110557014409,
9.23518115166695));
#185709=CARTESIAN_POINT('Ctrl Pts',(-0.988154744929942,6.6944633242757,
9.24379273853346));
#185710=CARTESIAN_POINT('Ctrl Pts',(-1.0103084152377,6.69119327059525,9.24484971967036));
#185711=CARTESIAN_POINT('Ctrl Pts',(-1.03244403022776,6.68781351690102,
9.24590670080725));
#185712=CARTESIAN_POINT('Ctrl Pts',(-1.05456048731491,6.68432428736025,
9.24696368194414));
#185713=CARTESIAN_POINT('Ctrl Pts',(-1.24425019003177,6.65439766250844,
9.25602925862511));
#185714=CARTESIAN_POINT('Ctrl Pts',(-1.43270925910908,6.61638521402429,
9.26509483530608));
#185715=CARTESIAN_POINT('Ctrl Pts',(-1.61927316818519,6.57040663937899,
9.27416041198704));
#185716=CARTESIAN_POINT('Ctrl Pts',(-1.80566893266155,6.5244695038795,9.28321781812865));
#185717=CARTESIAN_POINT('Ctrl Pts',(-1.99017272058708,6.47058063306388,
9.29227522427025));
#185718=CARTESIAN_POINT('Ctrl Pts',(-2.17213145945179,6.40891050981833,
9.30133263041186));
#185719=CARTESIAN_POINT('Ctrl Pts',(-2.35376430771272,6.34735083861166,
9.3103738146145));
#185720=CARTESIAN_POINT('Ctrl Pts',(-2.53286098808698,6.27803781958628,
9.31941499881713));
#185721=CARTESIAN_POINT('Ctrl Pts',(-2.70878498740475,6.20119124781768,
9.32845618301977));
#185722=CARTESIAN_POINT('Ctrl Pts',(-2.88448220283226,6.12444373907953,
9.33748571221835));
#185723=CARTESIAN_POINT('Ctrl Pts',(-3.05701468582643,6.04018215231809,
9.34651524141693));
#185724=CARTESIAN_POINT('Ctrl Pts',(-3.22576480942988,5.9486746754419,9.35554477061551));
#185725=CARTESIAN_POINT('Ctrl Pts',(-3.39411795280301,5.85738246749987,
9.36455305808398));
#185726=CARTESIAN_POINT('Ctrl Pts',(-3.55870629230085,5.75887850510299,
9.37356134555245));
#185727=CARTESIAN_POINT('Ctrl Pts',(-3.71893623776688,5.65347700618162,
9.38256963302093));
#185728=CARTESIAN_POINT('Ctrl Pts',(-3.85736858815834,5.56241427013669,
9.39035243793692));
#185729=CARTESIAN_POINT('Ctrl Pts',(-3.99254793695919,5.46620380645547,
9.39813524285292));
#185730=CARTESIAN_POINT('Ctrl Pts',(-4.1241052636902,5.36507639964267,9.40591804776891));
#185731=CARTESIAN_POINT('Ctrl Pts',(-4.26134633016998,5.2595799327701,9.41403709726176));
#185732=CARTESIAN_POINT('Ctrl Pts',(-4.39458133961908,5.14877973427311,
9.4221561467546));
#185733=CARTESIAN_POINT('Ctrl Pts',(-4.52338049145663,5.03302274279678,
9.43027519624744));
#185734=CARTESIAN_POINT('Ctrl Pts',(-4.65217030132519,4.91727414732468,
9.43839365685513));
#185735=CARTESIAN_POINT('Ctrl Pts',(-4.77652462189025,4.79656971991791,
9.44651211746282));
#185736=CARTESIAN_POINT('Ctrl Pts',(-4.89604821773083,4.67129541451349,
9.4546305780705));
#185737=CARTESIAN_POINT('Ctrl Pts',(-5.0155859867208,4.54600625403854,9.46275000136806));
#185738=CARTESIAN_POINT('Ctrl Pts',(-5.13029163829269,4.41614640248504,
9.47086942466562));
#185739=CARTESIAN_POINT('Ctrl Pts',(-5.23980819879691,4.28213720469355,
9.47898884796318));
#185740=CARTESIAN_POINT('Ctrl Pts',(-5.34940462715595,4.14803027714225,
9.4871141925654));
#185741=CARTESIAN_POINT('Ctrl Pts',(-5.45380417410579,4.00976824360599,
9.49523953716763));
#185742=CARTESIAN_POINT('Ctrl Pts',(-5.55269104690452,3.8678044337358,9.50336488176986));
#185743=CARTESIAN_POINT('Ctrl Pts',(-5.65161816392444,3.72578284852292,
9.51149353316253));
#185744=CARTESIAN_POINT('Ctrl Pts',(-5.74502793731403,3.5800567923771,9.51962218455519));
#185745=CARTESIAN_POINT('Ctrl Pts',(-5.83264917564189,3.43110661359918,
9.52775083594785));
#185746=CARTESIAN_POINT('Ctrl Pts',(-5.92036613308567,3.28199371879828,
9.5358883672347));
#185747=CARTESIAN_POINT('Ctrl Pts',(-6.00228175205012,3.12964998894373,
9.54402589852156));
#185748=CARTESIAN_POINT('Ctrl Pts',(-6.07817152326886,2.97457895066234,
9.55216342980841));
#185749=CARTESIAN_POINT('Ctrl Pts',(-6.11767907733684,2.89385031845155,
9.55639975773683));
#185750=CARTESIAN_POINT('Ctrl Pts',(-6.15555433183113,2.81238286858704,
9.56063608566525));
#185751=CARTESIAN_POINT('Ctrl Pts',(-6.19177088937875,2.73024948556756,
9.56487241359367));
#185752=CARTESIAN_POINT('Ctrl Pts',(-6.2709848012202,2.55060495272671,9.57413823369852));
#185753=CARTESIAN_POINT('Ctrl Pts',(-6.34239258434351,2.36747498292763,
9.58340405380337));
#185754=CARTESIAN_POINT('Ctrl Pts',(-6.40572310947491,2.18151333819876,
9.59266987390822));
#185755=CARTESIAN_POINT('Ctrl Pts',(-6.46892235210657,1.99593718702969,
9.60191648621362));
#185756=CARTESIAN_POINT('Ctrl Pts',(-6.52407771530158,1.80754126517537,
9.61116309851903));
#185757=CARTESIAN_POINT('Ctrl Pts',(-6.57096762095635,1.61699521469397,
9.62040971082443));
#185758=CARTESIAN_POINT('Ctrl Pts',(-6.61777937428698,1.42676675104699,
9.62964091162));
#185759=CARTESIAN_POINT('Ctrl Pts',(-6.65635312271435,1.23439549741426,
9.63887211241557));
#185760=CARTESIAN_POINT('Ctrl Pts',(-6.68651729066465,1.04056500116173,
9.64810331321114));
#185761=CARTESIAN_POINT('Ctrl Pts',(-6.71658029407039,0.84738457335817,
9.65730355441831));
#185762=CARTESIAN_POINT('Ctrl Pts',(-6.73828996916701,0.652754858681284,
9.66650379562548));
#185763=CARTESIAN_POINT('Ctrl Pts',(-6.75152608207339,0.457366989498324,
9.67570403683265));
#185764=CARTESIAN_POINT('Ctrl Pts',(-6.76182492117774,0.305338350736371,
9.68286261915845));
#185765=CARTESIAN_POINT('Ctrl Pts',(-6.76699468300774,0.152851025931063,
9.69002120148424));
#185766=CARTESIAN_POINT('Ctrl Pts',(-6.76699999589956,0.000235574698585379,
9.69717978381004));
#185767=CARTESIAN_POINT('',(-6.7669997504469,0.00183778443585837,9.30282021621592));
#185768=CARTESIAN_POINT('Ctrl Pts',(3.09910619832133,6.0156321173694,8.6514415183394));
#185769=CARTESIAN_POINT('Ctrl Pts',(2.94209720223375,6.09651930320018,8.659764140677));
#185770=CARTESIAN_POINT('Ctrl Pts',(2.78179285456176,6.1713209246991,8.66808676301459));
#185771=CARTESIAN_POINT('Ctrl Pts',(2.6186994290156,6.23976780821798,8.67640938535219));
#185772=CARTESIAN_POINT('Ctrl Pts',(2.45571880527167,6.30816735119083,8.68472625143813));
#185773=CARTESIAN_POINT('Ctrl Pts',(2.28995326589144,6.37022078068447,8.69304311752408));
#185774=CARTESIAN_POINT('Ctrl Pts',(2.12193190900749,6.42570571793759,8.70135998361003));
#185775=CARTESIAN_POINT('Ctrl Pts',(1.95399641886819,6.48116229980169,8.70967259938977));
#185776=CARTESIAN_POINT('Ctrl Pts',(1.78380773696813,6.53005697086354,8.71798521516951));
#185777=CARTESIAN_POINT('Ctrl Pts',(1.61191331302807,6.57221610047044,8.72629783094925));
#185778=CARTESIAN_POINT('Ctrl Pts',(1.44007570477806,6.61436129536098,8.73460769918785));
#185779=CARTESIAN_POINT('Ctrl Pts',(1.26653381432395,6.64977530391236,8.74291756742645));
#185780=CARTESIAN_POINT('Ctrl Pts',(1.09184880431173,6.67833476163954,8.75122743566505));
#185781=CARTESIAN_POINT('Ctrl Pts',(0.914481883555387,6.70733268810837,
8.75966488396853));
#185782=CARTESIAN_POINT('Ctrl Pts',(0.735936808451345,6.72926377155085,
8.76810233227201));
#185783=CARTESIAN_POINT('Ctrl Pts',(0.556810674542134,6.74405300043794,
8.77653978057549));
#185784=CARTESIAN_POINT('Ctrl Pts',(0.380370682180497,6.75862045285219,
8.78485070250368));
#185785=CARTESIAN_POINT('Ctrl Pts',(0.203367291180232,6.7662587470079,8.79316162443186));
#185786=CARTESIAN_POINT('Ctrl Pts',(0.0263751707729974,6.76694859965455,
8.80147254636005));
#185787=CARTESIAN_POINT('Ctrl Pts',(-0.150657686527601,6.7676386110792,
8.8097853811482));
#185788=CARTESIAN_POINT('Ctrl Pts',(-0.327678921432271,6.76137699179026,
8.81809821593635));
#185789=CARTESIAN_POINT('Ctrl Pts',(-0.504114683114431,6.74819660252044,
8.8264110507245));
#185790=CARTESIAN_POINT('Ctrl Pts',(-0.680619953403618,6.73501102070639,
8.83472716043583));
#185791=CARTESIAN_POINT('Ctrl Pts',(-0.856538945274694,6.71490126194879,
8.84304327014717));
#185792=CARTESIAN_POINT('Ctrl Pts',(-1.03130353000278,6.68795200558466,
8.8513593798585));
#185793=CARTESIAN_POINT('Ctrl Pts',(-1.21057499376556,6.660307774099,8.85988994778267));
#185794=CARTESIAN_POINT('Ctrl Pts',(-1.38863132264786,6.62546659988185,
8.86842051570684));
#185795=CARTESIAN_POINT('Ctrl Pts',(-1.56487190523667,6.5835753903332,8.87695108363102));
#185796=CARTESIAN_POINT('Ctrl Pts',(-1.73699120549985,6.54266378207148,
8.88528216924358));
#185797=CARTESIAN_POINT('Ctrl Pts',(-1.9073784162457,6.4950283321297,8.89361325485615));
#185798=CARTESIAN_POINT('Ctrl Pts',(-2.07549093628096,6.44085602799935,
8.90194434046872));
#185799=CARTESIAN_POINT('Ctrl Pts',(-2.2496414702677,6.38473804410611,8.9105746495487));
#185800=CARTESIAN_POINT('Ctrl Pts',(-2.42135049050345,6.32160507907051,
8.91920495862867));
#185801=CARTESIAN_POINT('Ctrl Pts',(-2.59003914532514,6.25171866175082,
8.92783526770865));
#185802=CARTESIAN_POINT('Ctrl Pts',(-2.75872780014682,6.18183224443113,
8.93646557678862));
#185803=CARTESIAN_POINT('Ctrl Pts',(-2.92439574511086,6.10519260033339,
8.9450958858686));
#185804=CARTESIAN_POINT('Ctrl Pts',(-3.08649419652116,6.02211279991011,
8.95372619494857));
#185805=CARTESIAN_POINT('Ctrl Pts',(-3.23773100661891,5.94459988174059,
8.96177821767956));
#185806=CARTESIAN_POINT('Ctrl Pts',(-3.38633099540894,5.8612399075377,8.96983024041054));
#185807=CARTESIAN_POINT('Ctrl Pts',(-3.53179615922495,5.77223569249246,
8.97788226314153));
#185808=CARTESIAN_POINT('Ctrl Pts',(-3.67707811592324,5.68334357442821,
8.98592414469618));
#185809=CARTESIAN_POINT('Ctrl Pts',(-3.81923278735326,5.5888215515979,8.99396602625083));
#185810=CARTESIAN_POINT('Ctrl Pts',(-3.95778285138489,5.48892010337951,
9.00200790780548));
#185811=CARTESIAN_POINT('Ctrl Pts',(-4.09618906377005,5.38912237931247,
9.01004143975806));
#185812=CARTESIAN_POINT('Ctrl Pts',(-4.23099781455493,5.28395656086194,
9.01807497171063));
#185813=CARTESIAN_POINT('Ctrl Pts',(-4.36175719359503,5.17371850646341,
9.02610850366321));
#185814=CARTESIAN_POINT('Ctrl Pts',(-4.49240968065308,5.06357056846203,
9.03413546843751));
#185815=CARTESIAN_POINT('Ctrl Pts',(-4.6190190988995,4.94835888673088,9.04216243321181));
#185816=CARTESIAN_POINT('Ctrl Pts',(-4.74116342286366,4.82842193658547,
9.05018939798611));
#185817=CARTESIAN_POINT('Ctrl Pts',(-4.86323483191242,4.70855658364808,
9.0582115710072));
#185818=CARTESIAN_POINT('Ctrl Pts',(-4.98084618571305,4.58397183896925,
9.06623374402828));
#185819=CARTESIAN_POINT('Ctrl Pts',(-5.09360950959622,4.45504558492402,
9.07425591704936));
#185820=CARTESIAN_POINT('Ctrl Pts',(-5.20921156822271,4.32287370611286,
9.08248004244723));
#185821=CARTESIAN_POINT('Ctrl Pts',(-5.31971797713956,4.18613910650498,
9.09070416784509));
#185822=CARTESIAN_POINT('Ctrl Pts',(-5.42475163585204,4.04528845563832,
9.09892829324295));
#185823=CARTESIAN_POINT('Ctrl Pts',(-5.52717232123493,3.90794181480693,
9.10694782307986));
#185824=CARTESIAN_POINT('Ctrl Pts',(-5.62438910319465,3.76668181360193,
9.11496735291676));
#185825=CARTESIAN_POINT('Ctrl Pts',(-5.71609406999345,3.62195493939194,
9.12298688275367));
#185826=CARTESIAN_POINT('Ctrl Pts',(-5.8078086354572,3.47721291676829,9.13100725198655));
#185827=CARTESIAN_POINT('Ctrl Pts',(-5.89401003617417,3.3290036155374,9.13902762121942));
#185828=CARTESIAN_POINT('Ctrl Pts',(-5.97443471743049,3.17780093888231,
9.1470479904523));
#185829=CARTESIAN_POINT('Ctrl Pts',(-6.05488386691842,3.02655226065091,
9.15507079978502));
#185830=CARTESIAN_POINT('Ctrl Pts',(-6.12955262288142,2.87230872547832,
9.16309360911774));
#185831=CARTESIAN_POINT('Ctrl Pts',(-6.19822433073136,2.7155670026589,9.17111641845046));
#185832=CARTESIAN_POINT('Ctrl Pts',(-6.26992383708833,2.55191439369433,
9.17949296079609));
#185833=CARTESIAN_POINT('Ctrl Pts',(-6.33508527033752,2.38553872161157,
9.18786950314173));
#185834=CARTESIAN_POINT('Ctrl Pts',(-6.39351927512407,2.21702509652395,
9.19624604548737));
#185835=CARTESIAN_POINT('Ctrl Pts',(-6.44958553521713,2.05533964012063,
9.20428317050638));
#185836=CARTESIAN_POINT('Ctrl Pts',(-6.49945880191981,1.89168645707455,
9.21232029552539));
#185837=CARTESIAN_POINT('Ctrl Pts',(-6.54302387842973,1.72659419850132,
9.2203574205444));
#185838=CARTESIAN_POINT('Ctrl Pts',(-6.5866221466704,1.561376158035,9.22840066895652));
#185839=CARTESIAN_POINT('Ctrl Pts',(-6.62390257490159,1.39471722264299,
9.23644391736865));
#185840=CARTESIAN_POINT('Ctrl Pts',(-6.65480157814796,1.22715319152884,
9.24448716578078));
#185841=CARTESIAN_POINT('Ctrl Pts',(-6.68574475004606,1.05934963562248,
9.25254191163297));
#185842=CARTESIAN_POINT('Ctrl Pts',(-6.71028824433949,0.890638770314056,
9.26059665748516));
#185843=CARTESIAN_POINT('Ctrl Pts',(-6.72842043818449,0.721559011461451,
9.26865140333735));
#185844=CARTESIAN_POINT('Ctrl Pts',(-6.73065919378264,0.700682979586886,
9.26964591109093));
#185845=CARTESIAN_POINT('Ctrl Pts',(-6.73280027753,0.679801320340407,9.27064041884451));
#185846=CARTESIAN_POINT('Ctrl Pts',(-6.7348437224623,0.658915043089906,
9.27163492659808));
#185847=CARTESIAN_POINT('Ctrl Pts',(-6.75620283932173,0.440601141158822,
9.2820300231287));
#185848=CARTESIAN_POINT('Ctrl Pts',(-6.76694013810318,0.221339368319224,
9.29242511965931));
#185849=CARTESIAN_POINT('Ctrl Pts',(-6.76699975044675,0.00183778498507086,
9.30282021618991));
#185850=CARTESIAN_POINT('Ctrl Pts',(-6.7669997504469,0.00183778443585837,
9.30282021621592));
#185851=CARTESIAN_POINT('Ctrl Pts',(-6.7670466121356,-0.170714028257617,
9.31099187822504));
#185852=CARTESIAN_POINT('Ctrl Pts',(-6.7604893996205,-0.343535385381546,
9.31916354023416));
#185853=CARTESIAN_POINT('Ctrl Pts',(-6.74729237457982,-0.516076168735846,
9.32733520224329));
#185854=CARTESIAN_POINT('Ctrl Pts',(-6.73411098419024,-0.688412541251919,
9.3354971832005));
#185855=CARTESIAN_POINT('Ctrl Pts',(-6.71430546902278,-0.860468642160045,
9.34365916415771));
#185856=CARTESIAN_POINT('Ctrl Pts',(-6.68789204202812,-1.03169231565278,
9.35182114511491));
#185857=CARTESIAN_POINT('Ctrl Pts',(-6.6615043985982,-1.20274884852148,
9.35997515872413));
#185858=CARTESIAN_POINT('Ctrl Pts',(-6.62852174184835,-1.37297421433712,
9.36812917233336));
#185859=CARTESIAN_POINT('Ctrl Pts',(-6.58901222851907,-1.54181933196669,
9.37628318594258));
#185860=CARTESIAN_POINT('Ctrl Pts',(-6.54953304674473,-1.71053482676543,
9.38443093969459));
#185861=CARTESIAN_POINT('Ctrl Pts',(-6.5035370695623,-1.87787183037223,
9.3925786934466));
#185862=CARTESIAN_POINT('Ctrl Pts',(-6.45114387794042,-2.04328942299221,
9.40072644719861));
#185863=CARTESIAN_POINT('Ctrl Pts',(-6.39877942289436,-2.20861628750336,
9.40886973207717));
#185864=CARTESIAN_POINT('Ctrl Pts',(-6.34002485152426,-2.37202549135048,
9.41701301695572));
#185865=CARTESIAN_POINT('Ctrl Pts',(-6.27505014849156,-2.53298926841708,
9.42515630183427));
#185866=CARTESIAN_POINT('Ctrl Pts',(-6.21009406395858,-2.6939069213169,
9.43329725325473));
#185867=CARTESIAN_POINT('Ctrl Pts',(-6.13892153218648,-2.85238020490531,
9.44143820467518));
#185868=CARTESIAN_POINT('Ctrl Pts',(-6.06175145907753,-3.00789930821686,
9.44957915609563));
#185869=CARTESIAN_POINT('Ctrl Pts',(-5.98458893522756,-3.16340319767749,
9.45771931111732));
#185870=CARTESIAN_POINT('Ctrl Pts',(-5.90143020041023,-3.31595315609132,
9.46585946613901));
#185871=CARTESIAN_POINT('Ctrl Pts',(-5.81254108315226,-3.46506207111318,
9.4739996211607));
#185872=CARTESIAN_POINT('Ctrl Pts',(-5.72364388599234,-3.61418453993612,
9.4821405161116));
#185873=CARTESIAN_POINT('Ctrl Pts',(-5.62901545650814,-3.75986503006738,
9.4902814110625));
#185874=CARTESIAN_POINT('Ctrl Pts',(-5.52896607630542,-3.90164364429452,
9.4984223060134));
#185875=CARTESIAN_POINT('Ctrl Pts',(-5.42884492179168,-4.0435239689204,
9.50656904115167));
#185876=CARTESIAN_POINT('Ctrl Pts',(-5.32329525781112,-4.18149652761971,
9.51471577628994));
#185877=CARTESIAN_POINT('Ctrl Pts',(-5.21266937519114,-4.31513232531106,
9.5228625114282));
#185878=CARTESIAN_POINT('Ctrl Pts',(-5.10200169492407,-4.44881861445864,
9.53101232463782));
#185879=CARTESIAN_POINT('Ctrl Pts',(-4.98625421496092,-4.57816460423707,
9.53916213784745));
#185880=CARTESIAN_POINT('Ctrl Pts',(-4.86581739319278,-4.70277684949037,
9.54731195105707));
#185881=CARTESIAN_POINT('Ctrl Pts',(-4.74524373195729,-4.82753067829775,
9.55547102402697));
#185882=CARTESIAN_POINT('Ctrl Pts',(-4.61997034650439,-4.94753976429741,
9.56363009699687));
#185883=CARTESIAN_POINT('Ctrl Pts',(-4.49042285896871,-5.0624491649449,
9.57178916996678));
#185884=CARTESIAN_POINT('Ctrl Pts',(-4.39645591943421,-5.14579840550515,
9.57770733272705));
#185885=CARTESIAN_POINT('Ctrl Pts',(-4.30024097346765,-5.22646537689021,
9.58362549548732));
#185886=CARTESIAN_POINT('Ctrl Pts',(-4.20195024913151,-5.30432871377931,
9.5895436582476));
#185887=CARTESIAN_POINT('Ctrl Pts',(-4.0606351949001,-5.41627479769963,
9.59805235016198));
#185888=CARTESIAN_POINT('Ctrl Pts',(-3.91473401575087,-5.52265723072521,
9.60656104207637));
#185889=CARTESIAN_POINT('Ctrl Pts',(-3.76470895516439,-5.6231001665367,
9.61506973399076));
#185890=CARTESIAN_POINT('Ctrl Pts',(-3.61481639142518,-5.72345439468645,
9.62357091132826));
#185891=CARTESIAN_POINT('Ctrl Pts',(-3.46080747525354,-5.8178794036784,
9.63207208866576));
#185892=CARTESIAN_POINT('Ctrl Pts',(-3.30317592279674,-5.90604079083915,
9.64057326600325));
#185893=CARTESIAN_POINT('Ctrl Pts',(-3.14566475190075,-5.9941348500746,
9.64906795108092));
#185894=CARTESIAN_POINT('Ctrl Pts',(-2.98453674275637,-6.07597466717417,
9.65756263615859));
#185895=CARTESIAN_POINT('Ctrl Pts',(-2.82031328098179,-6.15126994994674,
9.66605732123625));
#185896=CARTESIAN_POINT('Ctrl Pts',(-2.65621759810112,-6.22650664701027,
9.67454539677438));
#185897=CARTESIAN_POINT('Ctrl Pts',(-2.4890315615849,-6.29520883418608,
9.68303347231251));
#185898=CARTESIAN_POINT('Ctrl Pts',(-2.31929997642462,-6.35713273570379,
9.69152154785064));
#185899=CARTESIAN_POINT('Ctrl Pts',(-2.14964906063651,-6.41902720626879,
9.70000558920901));
#185900=CARTESIAN_POINT('Ctrl Pts',(-1.97745531220279,-6.47414970339247,
9.70848963056739));
#185901=CARTESIAN_POINT('Ctrl Pts',(-1.80328302776581,-6.52230475535848,
9.71697367192576));
#185902=CARTESIAN_POINT('Ctrl Pts',(-1.62918098751762,-6.57044038625199,
9.72545429164559));
#185903=CARTESIAN_POINT('Ctrl Pts',(-1.45310231492341,-6.61161409100884,
9.73393491136541));
#185904=CARTESIAN_POINT('Ctrl Pts',(-1.27562634308607,-6.64568028367487,
9.74241553108523));
#185905=CARTESIAN_POINT('Ctrl Pts',(-1.23319641108622,-6.65382463258785,
9.74444302874761));
#185906=CARTESIAN_POINT('Ctrl Pts',(-1.19068667308345,-6.66156296771806,
9.74647052640999));
#185907=CARTESIAN_POINT('Ctrl Pts',(-1.14810514809912,-6.66889372901595,
9.74849802407237));
#185908=CARTESIAN_POINT('Ctrl Pts',(-0.967949600006465,-6.69990899490988,
9.75707603889821));
#185909=CARTESIAN_POINT('Ctrl Pts',(-0.786591102187406,-6.72361042674612,
9.76565405372405));
#185910=CARTESIAN_POINT('Ctrl Pts',(-0.604637011330119,-6.73993346291562,
9.77423206854989));
#185911=CARTESIAN_POINT('Ctrl Pts',(-0.422590768744204,-6.75626476598362,
9.78281442776222));
#185912=CARTESIAN_POINT('Ctrl Pts',(-0.239948640404219,-6.76521018946188,
9.79139678697455));
#185913=CARTESIAN_POINT('Ctrl Pts',(-0.0573209745920767,-6.76675722232384,
9.79997914618688));
#185914=CARTESIAN_POINT('Ctrl Pts',(0.133259757644712,-6.76837162534605,
9.8089352498294));
#185915=CARTESIAN_POINT('Ctrl Pts',(0.323824359734286,-6.76192884701384,
9.81789135347192));
#185916=CARTESIAN_POINT('Ctrl Pts',(0.513682295249814,-6.74747504623373,
9.82684745711444));
#185917=CARTESIAN_POINT('Ctrl Pts',(0.69593181631616,-6.73360047068539,
9.83544465161694));
#185918=CARTESIAN_POINT('Ctrl Pts',(0.877529900041484,-6.71234450500837,
9.84404184611944));
#185919=CARTESIAN_POINT('Ctrl Pts',(1.05787328418431,-6.68380079854338,
9.85263904062193));
#185920=CARTESIAN_POINT('Ctrl Pts',(1.23832897751235,-6.65523931643094,
9.86124158904365));
#185921=CARTESIAN_POINT('Ctrl Pts',(1.41752810691512,-6.61938109244112,
9.86984413746536));
#185922=CARTESIAN_POINT('Ctrl Pts',(1.59487830026516,-6.57637074740646,
9.87844668588707));
#185923=CARTESIAN_POINT('Ctrl Pts',(1.77241483025084,-6.53331521266639,
9.88705827275358));
#185924=CARTESIAN_POINT('Ctrl Pts',(1.94809824320536,-6.4830926229974,9.89566985962008));
#185925=CARTESIAN_POINT('Ctrl Pts',(2.12135080736073,-6.42589758338164,
9.90428144648658));
#185926=CARTESIAN_POINT('Ctrl Pts',(2.14261572578531,-6.41887749766084,
9.90533842762343));
#185927=CARTESIAN_POINT('Ctrl Pts',(2.16384404715849,-6.41175243221178,
9.90639540876027));
#185928=CARTESIAN_POINT('Ctrl Pts',(2.18503472365863,-6.40452279693078,
9.90745238989712));
#185929=CARTESIAN_POINT('Ctrl Pts',(2.36678413813419,-6.34251524473282,
9.91651796657808));
#185930=CARTESIAN_POINT('Ctrl Pts',(2.54593475176408,-6.27275261438359,
9.92558354325904));
#185931=CARTESIAN_POINT('Ctrl Pts',(2.72185240231887,-6.19546677014662,
9.93464911994));
#185932=CARTESIAN_POINT('Ctrl Pts',(2.89761150343534,-6.11825058138286,
9.94370652608159));
#185933=CARTESIAN_POINT('Ctrl Pts',(3.07014324523132,-6.0335248106319,9.95276393222317));
#185934=CARTESIAN_POINT('Ctrl Pts',(3.23883345735384,-5.94156939162755,
9.96182133836476));
#185935=CARTESIAN_POINT('Ctrl Pts',(3.40722154298656,-5.84977866604324,
9.97086252256739));
#185936=CARTESIAN_POINT('Ctrl Pts',(3.57178163311142,-5.75078426082011,
9.97990370677001));
#185937=CARTESIAN_POINT('Ctrl Pts',(3.73192432653554,-5.64491185236867,
9.98894489097264));
#185938=CARTESIAN_POINT('Ctrl Pts',(3.89186057977518,-5.53917592419656,
9.99797442017125));
#185939=CARTESIAN_POINT('Ctrl Pts',(4.04739060635348,-5.42657981625096,
10.0070039493699));
#185940=CARTESIAN_POINT('Ctrl Pts',(4.19795190901923,-5.30749364291299,
10.0160334785685));
#185941=CARTESIAN_POINT('Ctrl Pts',(4.34815902017713,-5.18868761666828,
10.0250417660369));
#185942=CARTESIAN_POINT('Ctrl Pts',(4.49342055584514,-5.06342214512154,
10.0340500535054));
#185943=CARTESIAN_POINT('Ctrl Pts',(4.63320559190143,-4.93210856968633,
10.0430583409739));
#185944=CARTESIAN_POINT('Ctrl Pts',(4.75397434729608,-4.81865882199413,
10.0508411458899));
#185945=CARTESIAN_POINT('Ctrl Pts',(4.87065564734211,-4.70069533661137,
10.0586239508059));
#185946=CARTESIAN_POINT('Ctrl Pts',(4.98292550652445,-4.57850875246822,
10.0664067557219));
#185947=CARTESIAN_POINT('Ctrl Pts',(5.10004581894295,-4.45104327765228,
10.0745258052147));
#185948=CARTESIAN_POINT('Ctrl Pts',(5.21231002407704,-4.31903948992084,
10.0826448547076));
#185949=CARTESIAN_POINT('Ctrl Pts',(5.31935417212587,-4.18291288356417,
10.0907639042004));
#185950=CARTESIAN_POINT('Ctrl Pts',(5.42639055612429,-4.04679615064619,
10.0988823648081));
#185951=CARTESIAN_POINT('Ctrl Pts',(5.52820741067156,-3.90655748276577,
10.1070008254158));
#185952=CARTESIAN_POINT('Ctrl Pts',(5.6244815288003,-3.76264488520831,10.1151192860235));
#185953=CARTESIAN_POINT('Ctrl Pts',(5.72076706314787,-3.61871522244435,
10.1232387093211));
#185954=CARTESIAN_POINT('Ctrl Pts',(5.81150834959695,-3.47111106775377,
10.1313581326187));
#185955=CARTESIAN_POINT('Ctrl Pts',(5.89642594444674,-3.32030873288244,
10.1394775559163));
#185956=CARTESIAN_POINT('Ctrl Pts',(5.9814054677032,-3.1693964214116,10.1476029005185));
#185957=CARTESIAN_POINT('Ctrl Pts',(6.06055263682131,-3.01528159103643,
10.1557282451207));
#185958=CARTESIAN_POINT('Ctrl Pts',(6.133634063267,-2.85846500379676,10.163853589723));
#185959=CARTESIAN_POINT('Ctrl Pts',(6.20674523183145,-2.70158459654443,
10.1719822411157));
#185960=CARTESIAN_POINT('Ctrl Pts',(6.2737855953791,-2.54200057835911,10.1801108925084));
#185961=CARTESIAN_POINT('Ctrl Pts',(6.33457033879776,-2.38023268249633,
10.1882395439011));
#185962=CARTESIAN_POINT('Ctrl Pts',(6.39542148463189,-2.21828806829228,
10.1963770751879));
#185963=CARTESIAN_POINT('Ctrl Pts',(6.45000324561459,-2.05415515866025,
10.2045146064748));
#185964=CARTESIAN_POINT('Ctrl Pts',(6.49818077163492,-1.88836851783601,
10.2126521377616));
#185965=CARTESIAN_POINT('Ctrl Pts',(6.52326157216328,-1.80206143625145,
10.21688846569));
#185966=CARTESIAN_POINT('Ctrl Pts',(6.54660756825064,-1.71530635134659,
10.2211247936183));
#185967=CARTESIAN_POINT('Ctrl Pts',(6.56820525017969,-1.62817959436664,
10.2253611215467));
#185968=CARTESIAN_POINT('Ctrl Pts',(6.6112308218627,-1.45461103546927,10.2338004731193));
#185969=CARTESIAN_POINT('Ctrl Pts',(6.64740423022982,-1.27920682544239,
10.242239824692));
#185970=CARTESIAN_POINT('Ctrl Pts',(6.67657888614868,-1.10253497769171,
10.2506791762646));
#185971=CARTESIAN_POINT('Ctrl Pts',(6.70573136685457,-0.925997415529906,
10.2591121132143));
#185972=CARTESIAN_POINT('Ctrl Pts',(6.72789564526412,-0.748194464282019,
10.267545050164));
#185973=CARTESIAN_POINT('Ctrl Pts',(6.74297595893689,-0.569705377540964,
10.2759779871137));
#185974=CARTESIAN_POINT('Ctrl Pts',(6.75804713251623,-0.391324472033178,
10.2844058129076));
#185975=CARTESIAN_POINT('Ctrl Pts',(6.76604287311658,-0.21225859168572,
10.2928336387016));
#185976=CARTESIAN_POINT('Ctrl Pts',(6.76691907851943,-0.0330935759595899,
10.3012614644955));
#185977=CARTESIAN_POINT('Ctrl Pts',(6.76779488763841,0.145990408305047,
10.3096854786132));
#185978=CARTESIAN_POINT('Ctrl Pts',(6.7615575801646,0.325173105515606,10.3181094927308));
#185979=CARTESIAN_POINT('Ctrl Pts',(6.74821511557709,0.503866801741148,
10.3265335068485));
#185980=CARTESIAN_POINT('Ctrl Pts',(6.73487663477628,0.682507143688387,
10.334955005728));
#185981=CARTESIAN_POINT('Ctrl Pts',(6.71443725230049,0.860658443502518,
10.3433765046076));
#185982=CARTESIAN_POINT('Ctrl Pts',(6.68695695545498,1.0377358410946,10.3517980034871));
#185983=CARTESIAN_POINT('Ctrl Pts',(6.65947627551724,1.21481570725446,10.3602196197676));
#185984=CARTESIAN_POINT('Ctrl Pts',(6.62495452963571,1.39082131068888,10.368641236048));
#185985=CARTESIAN_POINT('Ctrl Pts',(6.58350332138551,1.56517507560848,10.3770628523284));
#185986=CARTESIAN_POINT('Ctrl Pts',(6.54205075252875,1.73953456356692,10.3854847450424));
#185987=CARTESIAN_POINT('Ctrl Pts',(6.49366834479376,1.91224178021917,10.3939066377564));
#185988=CARTESIAN_POINT('Ctrl Pts',(6.4385184055237,2.08273131770102,10.4023285304705));
#185989=CARTESIAN_POINT('Ctrl Pts',(6.38335894358225,2.25325029339914,10.4107518773822));
#185990=CARTESIAN_POINT('Ctrl Pts',(6.3214297230832,2.42155050901785,10.419175224294));
#185991=CARTESIAN_POINT('Ctrl Pts',(6.25294243045065,2.58708329233327,10.4275985712057));
#185992=CARTESIAN_POINT('Ctrl Pts',(6.18443373173197,2.75266781384539,10.4360245508816));
#185993=CARTESIAN_POINT('Ctrl Pts',(6.10936300174402,2.91548287032578,10.4444505305575));
#185994=CARTESIAN_POINT('Ctrl Pts',(6.027989562113,3.07500094943997,10.4528765102334));
#185995=CARTESIAN_POINT('Ctrl Pts',(5.94654295224503,3.23466246572113,10.4613100664716));
#185996=CARTESIAN_POINT('Ctrl Pts',(5.85878246027435,3.39102078335486,10.4697436227097));
#185997=CARTESIAN_POINT('Ctrl Pts',(5.76501331348837,3.54357312543453,10.4781771789479));
#185998=CARTESIAN_POINT('Ctrl Pts',(5.67119887575865,3.69619915102077,10.4866148086338));
#185999=CARTESIAN_POINT('Ctrl Pts',(5.57137017663366,3.84501525498488,10.4950524383197));
#186000=CARTESIAN_POINT('Ctrl Pts',(5.46587535680585,3.98954829321097,10.5034900680056));
#186001=CARTESIAN_POINT('Ctrl Pts',(5.36026250784733,4.13424303709131,10.5119371378337));
#186002=CARTESIAN_POINT('Ctrl Pts',(5.24897107439376,4.27464487543108,10.5203842076617));
#186003=CARTESIAN_POINT('Ctrl Pts',(5.13238976466265,4.41031340196885,10.5288312774898));
#186004=CARTESIAN_POINT('Ctrl Pts',(5.06596562387541,4.48761280208648,10.5336441360586));
#186005=CARTESIAN_POINT('Ctrl Pts',(4.99782491158918,4.56337625664566,10.5384569946274));
#186006=CARTESIAN_POINT('Ctrl Pts',(4.92804479460896,4.63752773601707,10.5432698531962));
#186007=CARTESIAN_POINT('Ctrl Pts',(4.80851785790511,4.76454241533947,10.5515138382511));
#186008=CARTESIAN_POINT('Ctrl Pts',(4.68391210280518,4.88710868455191,10.559757823306));
#186009=CARTESIAN_POINT('Ctrl Pts',(4.55459000775174,5.00479758444715,10.5680018083609));
#186010=CARTESIAN_POINT('Ctrl Pts',(4.42545716313932,5.12231425796298,10.5762337291371));
#186011=CARTESIAN_POINT('Ctrl Pts',(4.29162199506258,5.2349675498427,10.5844656499132));
#186012=CARTESIAN_POINT('Ctrl Pts',(4.1534854404704,5.34236349341754,10.5926975706893));
#186013=CARTESIAN_POINT('Ctrl Pts',(4.01546585408141,5.44966849864093,10.6009225210225));
#186014=CARTESIAN_POINT('Ctrl Pts',(3.87315241089694,5.5517248007974,10.6091474713556));
#186015=CARTESIAN_POINT('Ctrl Pts',(3.72698151371424,5.6481765018838,10.6173724216887));
#186016=CARTESIAN_POINT('Ctrl Pts',(3.58093181984589,5.74454822627121,10.6255905519827));
#186017=CARTESIAN_POINT('Ctrl Pts',(3.43103134131578,5.83532441488182,10.6338086822767));
#186018=CARTESIAN_POINT('Ctrl Pts',(3.27774791139971,5.9201906750809,10.6420268125707));
#186019=CARTESIAN_POINT('Ctrl Pts',(3.21869317985551,5.95288666978797,10.6451929700514));
#186020=CARTESIAN_POINT('Ctrl Pts',(3.15913664059974,5.98470590510722,10.6483591275322));
#186021=CARTESIAN_POINT('Ctrl Pts',(3.09910619832133,6.01563211736941,10.651525285013));
#186022=CARTESIAN_POINT('Origin',(0.,0.,4.30282021618968));
#186023=CARTESIAN_POINT('',(3.09910619832134,6.0156321173694,13.0454981451509));
#186024=CARTESIAN_POINT('',(3.09910619832132,6.01563211736941,12.6513039064363));
#186025=CARTESIAN_POINT('',(3.09910619832133,6.0156321173694,4.30282021618968));
#186026=CARTESIAN_POINT('',(-6.76699966505605,-0.00196815110624866,11.69717978381));
#186027=CARTESIAN_POINT('Ctrl Pts',(-6.76699960802935,-0.0023032435072958,
11.69717978381));
#186028=CARTESIAN_POINT('Ctrl Pts',(-6.76693681242208,-0.186798651139549,
11.7058298775953));
#186029=CARTESIAN_POINT('Ctrl Pts',(-6.75932464309069,-0.371131808236207,
11.7144799713807));
#186030=CARTESIAN_POINT('Ctrl Pts',(-6.74422821643248,-0.554684382938594,
11.723130065166));
#186031=CARTESIAN_POINT('Ctrl Pts',(-6.72911430810714,-0.738449511584034,
11.7317901757629));
#186032=CARTESIAN_POINT('Ctrl Pts',(-6.70649887319034,-0.92143195827289,
11.7404502863597));
#186033=CARTESIAN_POINT('Ctrl Pts',(-6.67649843439857,-1.10302205575116,
11.7491103969565));
#186034=CARTESIAN_POINT('Ctrl Pts',(-6.64643861478435,-1.28497158028351,
11.7577876487857));
#186035=CARTESIAN_POINT('Ctrl Pts',(-6.60896462059164,-1.46552295301023,
11.7664649006148));
#186036=CARTESIAN_POINT('Ctrl Pts',(-6.56424377347403,-1.64407806457217,
11.7751421524439));
#186037=CARTESIAN_POINT('Ctrl Pts',(-6.53831776864942,-1.74759177198564,
11.7801726133427));
#186038=CARTESIAN_POINT('Ctrl Pts',(-6.50995711894902,-1.85043486796765,
11.7852030742415));
#186039=CARTESIAN_POINT('Ctrl Pts',(-6.47920190307687,-1.95249371296429,
11.7902335351403));
#186040=CARTESIAN_POINT('Ctrl Pts',(-6.42760020303839,-2.12373003033185,
11.7986737403866));
#186041=CARTESIAN_POINT('Ctrl Pts',(-6.36916780679982,-2.29304635343699,
11.8071139456329));
#186042=CARTESIAN_POINT('Ctrl Pts',(-6.30406874060674,-2.45987932909422,
11.8155541508792));
#186043=CARTESIAN_POINT('Ctrl Pts',(-6.23901899736336,-2.62658590210163,
11.8239879613207));
#186044=CARTESIAN_POINT('Ctrl Pts',(-6.16731277392029,-2.79081256881585,
11.8324217717622));
#186045=CARTESIAN_POINT('Ctrl Pts',(-6.08916353704902,-2.95201226607761,
11.8408555822037));
#186046=CARTESIAN_POINT('Ctrl Pts',(-6.0110614969762,-3.11311460973843,
11.8492842992001));
#186047=CARTESIAN_POINT('Ctrl Pts',(-5.9265243461337,-3.27119332916337,
11.8577130161965));
#186048=CARTESIAN_POINT('Ctrl Pts',(-5.83581333221124,-3.42572207739997,
11.8661417331929));
#186049=CARTESIAN_POINT('Ctrl Pts',(-5.74514317202579,-3.58018123015341,
11.8745666541277));
#186050=CARTESIAN_POINT('Ctrl Pts',(-5.64830486138084,-3.73109331244725,
11.8829915750626));
#186051=CARTESIAN_POINT('Ctrl Pts',(-5.54560536888083,-3.87795694827059,
11.8914164959975));
#186052=CARTESIAN_POINT('Ctrl Pts',(-5.44293637211757,-4.02477697419219,
11.8998389152241));
#186053=CARTESIAN_POINT('Ctrl Pts',(-5.33440985519956,-4.16755067799563,
11.9082613344507));
#186054=CARTESIAN_POINT('Ctrl Pts',(-5.22037606490862,-4.30580570171591,
11.9166837536773));
#186055=CARTESIAN_POINT('Ctrl Pts',(-5.10634048214024,-4.444062898643,11.9251063052944));
#186056=CARTESIAN_POINT('Ctrl Pts',(-4.98679766004418,-4.57780101213762,
11.9335288569116));
#186057=CARTESIAN_POINT('Ctrl Pts',(-4.86213850888825,-4.70658030000402,
11.9419514085287));
#186058=CARTESIAN_POINT('Ctrl Pts',(-4.73747514726915,-4.83536393749453,
11.9503742446243));
#186059=CARTESIAN_POINT('Ctrl Pts',(-4.60769534391517,-4.95918817560475,
11.9587970807199));
#186060=CARTESIAN_POINT('Ctrl Pts',(-4.4732273948143,-5.07764962106316,
11.9672199168155));
#186061=CARTESIAN_POINT('Ctrl Pts',(-4.33873613058136,-5.1961316063176,
11.9756442133301));
#186062=CARTESIAN_POINT('Ctrl Pts',(-4.19955535026871,-5.30924872459061,
11.9840685098446));
#186063=CARTESIAN_POINT('Ctrl Pts',(-4.05614726551665,-5.41663718190925,
11.9924928063591));
#186064=CARTESIAN_POINT('Ctrl Pts',(-3.91269428786376,-5.52405925643556,
12.0009197400409));
#186065=CARTESIAN_POINT('Ctrl Pts',(-3.76501163431016,-5.62574889475977,
12.0093466737227));
#186066=CARTESIAN_POINT('Ctrl Pts',(-3.61359167504872,-5.72138481541127,
12.0177736074045));
#186067=CARTESIAN_POINT('Ctrl Pts',(-3.46203557008112,-5.81710672485853,
12.0262081179661));
#186068=CARTESIAN_POINT('Ctrl Pts',(-3.30673572726618,-5.90676386224585,
12.0346426285277));
#186069=CARTESIAN_POINT('Ctrl Pts',(-3.14821136361916,-5.99007964971913,
12.0430771390894));
#186070=CARTESIAN_POINT('Ctrl Pts',(-2.98961043129991,-6.07343567945597,
12.0515157235944));
#186071=CARTESIAN_POINT('Ctrl Pts',(-2.82778217076928,-6.15044410274545,
12.0599543080993));
#186072=CARTESIAN_POINT('Ctrl Pts',(-2.66326757435415,-6.2208757283355,
12.0683928926043));
#186073=CARTESIAN_POINT('Ctrl Pts',(-2.49856908691915,-6.29138608094275,
12.0768409095848));
#186074=CARTESIAN_POINT('Ctrl Pts',(-2.33117857343359,-6.35530482272349,
12.0852889265654));
#186075=CARTESIAN_POINT('Ctrl Pts',(-2.16165519938208,-6.41245162157068,
12.0937369435459));
#186076=CARTESIAN_POINT('Ctrl Pts',(-2.0652996875405,-6.44493333144601,
12.0985387179605));
#186077=CARTESIAN_POINT('Ctrl Pts',(-1.96825538871769,-6.47522815707328,
12.1033404923752));
#186078=CARTESIAN_POINT('Ctrl Pts',(-1.87062672729887,-6.50331028377973,
12.1081422667898));
#186079=CARTESIAN_POINT('Ctrl Pts',(-1.70310221153925,-6.55149741048647,
12.1163818034373));
#186080=CARTESIAN_POINT('Ctrl Pts',(-1.53348245935107,-6.59327404759384,
12.1246213400847));
#186081=CARTESIAN_POINT('Ctrl Pts',(-1.36229741557804,-6.62845643807888,
12.1328608767322));
#186082=CARTESIAN_POINT('Ctrl Pts',(-1.19130237552393,-6.66359977851093,
12.1410912680561));
#186083=CARTESIAN_POINT('Ctrl Pts',(-1.01874584882209,-6.69216337498689,
12.14932165938));
#186084=CARTESIAN_POINT('Ctrl Pts',(-0.845173570896423,-6.7140130052792,
12.157552050704));
#186085=CARTESIAN_POINT('Ctrl Pts',(-0.671762982778306,-6.73584228173067,
12.1657747750755));
#186086=CARTESIAN_POINT('Ctrl Pts',(-0.497338878882295,-6.75097000343168,
12.1739974994471));
#186087=CARTESIAN_POINT('Ctrl Pts',(-0.322457933687271,-6.75931282609424,
12.1822202238186));
#186088=CARTESIAN_POINT('Ctrl Pts',(-0.147731946550763,-6.76764825636994,
12.1904356622197));
#186089=CARTESIAN_POINT('Ctrl Pts',(0.0274497209401242,-6.76921075308692,
12.1986511006208));
#186090=CARTESIAN_POINT('Ctrl Pts',(0.202524641810431,-6.76396871440574,
12.2068665390219));
#186091=CARTESIAN_POINT('Ctrl Pts',(0.377509587208122,-6.75872936974209,
12.2150777552993));
#186092=CARTESIAN_POINT('Ctrl Pts',(0.552387540366576,-6.74669246493872,
12.2232889715768));
#186093=CARTESIAN_POINT('Ctrl Pts',(0.726595016490422,-6.72787846813624,
12.2315001878543));
#186094=CARTESIAN_POINT('Ctrl Pts',(0.900744071880028,-6.70907078063536,
12.2397086504883));
#186095=CARTESIAN_POINT('Ctrl Pts',(1.07422274467752,-6.68349056674038,
12.2479171131223));
#186096=CARTESIAN_POINT('Ctrl Pts',(1.2464715234989,-6.65121024634663,12.2561255757563));
#186097=CARTESIAN_POINT('Ctrl Pts',(1.32321147796168,-6.6368287782514,12.2597825947091));
#186098=CARTESIAN_POINT('Ctrl Pts',(1.39970739264354,-6.62111811727423,
12.2634396136618));
#186099=CARTESIAN_POINT('Ctrl Pts',(1.47591029112141,-6.60408796220659,
12.2670966326146));
#186100=CARTESIAN_POINT('Ctrl Pts',(1.66051062433008,-6.56283267713372,
12.2759557039979));
#186101=CARTESIAN_POINT('Ctrl Pts',(1.84319879724182,-6.51387371439261,
12.2848147753813));
#186102=CARTESIAN_POINT('Ctrl Pts',(2.02335685831665,-6.457423326986,12.2936738467646));
#186103=CARTESIAN_POINT('Ctrl Pts',(2.20385339789918,-6.40086688136156,
12.3025495624504));
#186104=CARTESIAN_POINT('Ctrl Pts',(2.38181007859704,-6.3367909609365,12.3114252781362));
#186105=CARTESIAN_POINT('Ctrl Pts',(2.55662797381253,-6.26545628055286,
12.320300993822));
#186106=CARTESIAN_POINT('Ctrl Pts',(2.7319447475375,-6.19391803211355,12.3292020381723));
#186107=CARTESIAN_POINT('Ctrl Pts',(2.90410456971904,-6.11507966997994,
12.3381030825226));
#186108=CARTESIAN_POINT('Ctrl Pts',(3.07252943976385,-6.02924969144457,
12.3470041268729));
#186109=CARTESIAN_POINT('Ctrl Pts',(3.24118328471917,-5.94330302639106,
12.3559172722616));
#186110=CARTESIAN_POINT('Ctrl Pts',(3.40609180655076,-5.85034588128721,
12.3648304176504));
#186111=CARTESIAN_POINT('Ctrl Pts',(3.5667040062172,-5.75073139105229,12.3737435630391));
#186112=CARTESIAN_POINT('Ctrl Pts',(3.72767280825489,-5.65089572980107,
12.3826764980129));
#186113=CARTESIAN_POINT('Ctrl Pts',(3.88432598718312,-5.54437329570926,
12.3916094329867));
#186114=CARTESIAN_POINT('Ctrl Pts',(4.03614143131697,-5.43156067317733,
12.4005423679605));
#186115=CARTESIAN_POINT('Ctrl Pts',(4.18064802691937,-5.3241791869519,12.4090452447868));
#186116=CARTESIAN_POINT('Ctrl Pts',(4.32077158341717,-5.21109902508388,
12.4175481216131));
#186117=CARTESIAN_POINT('Ctrl Pts',(4.45609154240944,-5.09269448972418,
12.4260509984394));
#186118=CARTESIAN_POINT('Ctrl Pts',(4.58695297837985,-4.97819114788188,
12.4342737224163));
#186119=CARTESIAN_POINT('Ctrl Pts',(4.71357229982678,-4.85848830038076,
12.4424964463933));
#186120=CARTESIAN_POINT('Ctrl Pts',(4.83551168253833,-4.73393237890397,
12.4507191703703));
#186121=CARTESIAN_POINT('Ctrl Pts',(4.95732199654481,-4.60950829564987,
12.4589331908725));
#186122=CARTESIAN_POINT('Ctrl Pts',(5.07446198707429,-4.48024162167048,
12.4671472113747));
#186123=CARTESIAN_POINT('Ctrl Pts',(5.18652721610824,-4.34651865710577,
12.475361231877));
#186124=CARTESIAN_POINT('Ctrl Pts',(5.29849632742207,-4.21291038597981,
12.4835682072598));
#186125=CARTESIAN_POINT('Ctrl Pts',(5.40539911670082,-4.07485370976442,
12.4917751826426));
#186126=CARTESIAN_POINT('Ctrl Pts',(5.5068682599934,-3.93277141047853,12.4999821580254));
#186127=CARTESIAN_POINT('Ctrl Pts',(5.60827074008092,-3.79078245643184,
12.5081837415889));
#186128=CARTESIAN_POINT('Ctrl Pts',(5.70424647705759,-3.6447734382238,12.5163853251524));
#186129=CARTESIAN_POINT('Ctrl Pts',(5.79446863718678,-3.49519988164609,
12.524586908716));
#186130=CARTESIAN_POINT('Ctrl Pts',(5.88464962833072,-3.34569457649945,
12.5327847498411));
#186131=CARTESIAN_POINT('Ctrl Pts',(5.96908208815702,-3.19262827995006,
12.5409825909663));
#186132=CARTESIAN_POINT('Ctrl Pts',(6.04748266452477,-3.03648520863719,
12.5491804320915));
#186133=CARTESIAN_POINT('Ctrl Pts',(6.12587632227628,-2.88035591648308,
12.5573775497817));
#186134=CARTESIAN_POINT('Ctrl Pts',(6.1982389883186,-2.72115070687866,12.5655746674719));
#186135=CARTESIAN_POINT('Ctrl Pts',(6.26433325423851,-2.55937841669448,
12.5737717851621));
#186136=CARTESIAN_POINT('Ctrl Pts',(6.33042678478087,-2.39760792642003,
12.5819688116496));
#186137=CARTESIAN_POINT('Ctrl Pts',(6.39025191740379,-2.23327074422573,
12.5901658381371));
#186138=CARTESIAN_POINT('Ctrl Pts',(6.44361944974623,-2.06689559166691,
12.5983628646246));
#186139=CARTESIAN_POINT('Ctrl Pts',(6.49699609214695,-1.90049203818212,
12.6065612903784));
#186140=CARTESIAN_POINT('Ctrl Pts',(6.54391282847634,-1.73205016292751,
12.6147597161322));
#186141=CARTESIAN_POINT('Ctrl Pts',(6.58423036489251,-1.56211379291891,
12.622958141886));
#186142=CARTESIAN_POINT('Ctrl Pts',(6.62456211470853,-1.39211751415121,
12.6311594578835));
#186143=CARTESIAN_POINT('Ctrl Pts',(6.65828994749948,-1.22062604003942,
12.6393607738809));
#186144=CARTESIAN_POINT('Ctrl Pts',(6.68532569457477,-1.04819337789283,
12.6475620898783));
#186145=CARTESIAN_POINT('Ctrl Pts',(6.71239223083345,-0.875564343852308,
12.6557727457998));
#186146=CARTESIAN_POINT('Ctrl Pts',(6.73275140000822,-0.701992335270251,
12.6639834017212));
#186147=CARTESIAN_POINT('Ctrl Pts',(6.74636682694953,-0.528037532979418,
12.6721940576426));
#186148=CARTESIAN_POINT('Ctrl Pts',(6.75999027713044,-0.353980223358749,
12.6804095519036));
#186149=CARTESIAN_POINT('Ctrl Pts',(6.76686204957201,-0.179540028349648,
12.6886250461647));
#186150=CARTESIAN_POINT('Ctrl Pts',(6.76699794245695,-0.00527700516096534,
12.6968405404257));
#186151=CARTESIAN_POINT('Ctrl Pts',(6.76713404618214,0.169256390256702,
12.7050687811746));
#186152=CARTESIAN_POINT('Ctrl Pts',(6.76051339906589,0.343611706188307,
12.7132970219234));
#186153=CARTESIAN_POINT('Ctrl Pts',(6.74720380957269,0.517232783268677,
12.7215252626722));
#186154=CARTESIAN_POINT('Ctrl Pts',(6.73510751985823,0.675026594262806,
12.7290034184778));
#186155=CARTESIAN_POINT('Ctrl Pts',(6.71748690659344,0.832213821742122,
12.7364815742833));
#186156=CARTESIAN_POINT('Ctrl Pts',(6.69442928804816,0.988385303069121,
12.7439597300889));
#186157=CARTESIAN_POINT('Ctrl Pts',(6.66954798240274,1.15690879357467,12.7520293527126));
#186158=CARTESIAN_POINT('Ctrl Pts',(6.63825329605563,1.32480105408137,12.7600989753363));
#186159=CARTESIAN_POINT('Ctrl Pts',(6.60057929905731,1.49152335444544,12.76816859796));
#186160=CARTESIAN_POINT('Ctrl Pts',(6.56295259957615,1.65803634463562,12.7762280896408));
#186161=CARTESIAN_POINT('Ctrl Pts',(6.51896260661402,1.82338193789948,12.7842875813216));
#186162=CARTESIAN_POINT('Ctrl Pts',(6.46869516395212,1.98702588706401,12.7923470730023));
#186163=CARTESIAN_POINT('Ctrl Pts',(6.41847979680908,2.15050030614881,12.8003982152985));
#186164=CARTESIAN_POINT('Ctrl Pts',(6.36200003066915,2.31227623564346,12.8084493575947));
#186165=CARTESIAN_POINT('Ctrl Pts',(6.29939281912488,2.47182910217473,12.8165004998909));
#186166=CARTESIAN_POINT('Ctrl Pts',(6.23683674710517,2.63125164094448,12.8245450657627));
#186167=CARTESIAN_POINT('Ctrl Pts',(6.16816332754824,2.78845438547341,12.8325896316345));
#186168=CARTESIAN_POINT('Ctrl Pts',(6.09355943013832,2.94292753416941,12.8406341975064));
#186169=CARTESIAN_POINT('Ctrl Pts',(6.01900014046277,3.09730831909588,12.8486739533097));
#186170=CARTESIAN_POINT('Ctrl Pts',(5.93851759428498,3.24896242225308,12.8567137091131));
#186171=CARTESIAN_POINT('Ctrl Pts',(5.85234686621959,3.39739976415048,12.8647534649164));
#186172=CARTESIAN_POINT('Ctrl Pts',(5.76619954440878,3.54579678652997,12.8727910369089));
#186173=CARTESIAN_POINT('Ctrl Pts',(5.67436729919539,3.6909784619495,12.8808286089013));
#186174=CARTESIAN_POINT('Ctrl Pts',(5.57713129273385,3.83247903368158,12.8888661808938));
#186175=CARTESIAN_POINT('Ctrl Pts',(5.47990580844396,3.97396429325349,12.8969028831189));
#186176=CARTESIAN_POINT('Ctrl Pts',(5.37727793763501,4.11176893377874,12.9049395853439));
#186177=CARTESIAN_POINT('Ctrl Pts',(5.26957222086834,4.24545611319358,12.912976287569));
#186178=CARTESIAN_POINT('Ctrl Pts',(5.16185682403204,4.37915530776643,12.921013712094));
#186179=CARTESIAN_POINT('Ctrl Pts',(5.04906290737038,4.50873601391433,12.929051136619));
#186180=CARTESIAN_POINT('Ctrl Pts',(4.93155524625363,4.63379454153379,12.937088561144));
#186181=CARTESIAN_POINT('Ctrl Pts',(4.81401374286677,4.758889086077,12.9451283004517));
#186182=CARTESIAN_POINT('Ctrl Pts',(4.69175604904061,4.8794585882599,12.9531680397593));
#186183=CARTESIAN_POINT('Ctrl Pts',(4.56518360805953,4.99513639700705,12.961207779067));
#186184=CARTESIAN_POINT('Ctrl Pts',(4.43848484523008,5.11092965453992,12.9692555421966));
#186185=CARTESIAN_POINT('Ctrl Pts',(4.30746301304585,5.22182121893857,12.9773033053262));
#186186=CARTESIAN_POINT('Ctrl Pts',(4.172552946396,5.32748448233518,12.9853510684558));
#186187=CARTESIAN_POINT('Ctrl Pts',(4.037566819994,5.43320731668764,12.9934033687625));
#186188=CARTESIAN_POINT('Ctrl Pts',(3.89868839502885,5.53369576138043,13.0014556690692));
#186189=CARTESIAN_POINT('Ctrl Pts',(3.75638081995438,5.62866699454488,13.0095079693759));
#186190=CARTESIAN_POINT('Ctrl Pts',(3.61388392645767,5.7237645723822,13.0175709820343));
#186191=CARTESIAN_POINT('Ctrl Pts',(3.46794909182187,5.81333009010918,13.0256339946927));
#186192=CARTESIAN_POINT('Ctrl Pts',(3.31906400050988,5.89712668682973,13.0336970073511));
#186193=CARTESIAN_POINT('Ctrl Pts',(3.24642723501661,5.93800864278306,13.037630719951));
#186194=CARTESIAN_POINT('Ctrl Pts',(3.17308856489218,5.97751821573234,13.041564432551));
#186195=CARTESIAN_POINT('Ctrl Pts',(3.09910619832134,6.0156321173694,13.0454981451509));
#186196=CARTESIAN_POINT('Ctrl Pts',(3.09910619832133,6.01563211736941,11.0457552630241));
#186197=CARTESIAN_POINT('Ctrl Pts',(2.9337533076482,6.10081787314656,11.0545047109264));
#186198=CARTESIAN_POINT('Ctrl Pts',(2.76488627843059,6.17918207037044,11.0632541588287));
#186199=CARTESIAN_POINT('Ctrl Pts',(2.59307866646686,6.25045854554004,11.072003606731));
#186200=CARTESIAN_POINT('Ctrl Pts',(2.42127244185365,6.32173444515041,11.0807529839813));
#186201=CARTESIAN_POINT('Ctrl Pts',(2.24652594672458,6.3859226274184,11.0895023612316));
#186202=CARTESIAN_POINT('Ctrl Pts',(2.06943269687119,6.44280508110562,11.0982517384819));
#186203=CARTESIAN_POINT('Ctrl Pts',(1.89234081822068,6.49968709436169,11.1070010479873));
#186204=CARTESIAN_POINT('Ctrl Pts',(1.71290249405572,6.54926340459549,11.1157503574927));
#186205=CARTESIAN_POINT('Ctrl Pts',(1.53172716625035,6.59136563150389,11.124499666998));
#186206=CARTESIAN_POINT('Ctrl Pts',(1.35055318107315,6.63346754640714,11.1332489116653));
#186207=CARTESIAN_POINT('Ctrl Pts',(1.16764249714404,6.66809542395778,11.1419981563325));
#186208=CARTESIAN_POINT('Ctrl Pts',(0.983616340614246,6.6951316562467,11.1507474009997));
#186209=CARTESIAN_POINT('Ctrl Pts',(0.79959148671368,6.72216769715963,11.1594965837354));
#186210=CARTESIAN_POINT('Ctrl Pts',(0.614451459526498,6.74161215869373,
11.1682457664711));
#186211=CARTESIAN_POINT('Ctrl Pts',(0.428825047910016,6.75339900185714,
11.1769949492068));
#186212=CARTESIAN_POINT('Ctrl Pts',(0.24319988859665,6.76518576550223,11.1857440729174));
#186213=CARTESIAN_POINT('Ctrl Pts',(0.0570886373913931,6.76931499599835,
11.1944931966279));
#186214=CARTESIAN_POINT('Ctrl Pts',(-0.128876626811801,6.76577266947846,
11.2032423203384));
#186215=CARTESIAN_POINT('Ctrl Pts',(-0.314840698188869,6.7622303656799,
11.21199138793));
#186216=CARTESIAN_POINT('Ctrl Pts',(-0.500658497952018,6.75101660879217,
11.2207404555215));
#186217=CARTESIAN_POINT('Ctrl Pts',(-0.685698951927038,6.7321694829621,
11.2294895231131));
#186218=CARTESIAN_POINT('Ctrl Pts',(-0.870738280460472,6.71332247176285,
11.2382385374916));
#186219=CARTESIAN_POINT('Ctrl Pts',(-1.05499998761293,6.68684221356179,
11.2469875518701));
#186220=CARTESIAN_POINT('Ctrl Pts',(-1.23785829161442,6.65281863948518,
11.2557365662486));
#186221=CARTESIAN_POINT('Ctrl Pts',(-1.43007412917425,6.61705395368857,
11.2649332999478));
#186222=CARTESIAN_POINT('Ctrl Pts',(-1.62073882535812,6.57295372727785,
11.274130033647));
#186223=CARTESIAN_POINT('Ctrl Pts',(-1.80913696091533,6.52068343478274,
11.2833267673462));
#186224=CARTESIAN_POINT('Ctrl Pts',(-1.9883835618613,6.47095219815193,11.2920767650599));
#186225=CARTESIAN_POINT('Ctrl Pts',(-2.16557827572549,6.41382586850885,
11.3008267627735));
#186226=CARTESIAN_POINT('Ctrl Pts',(-2.34011918621715,6.34949849943272,
11.3095767604872));
#186227=CARTESIAN_POINT('Ctrl Pts',(-2.51465655691113,6.28517243495545,
11.3183265807455));
#186228=CARTESIAN_POINT('Ctrl Pts',(-2.68653996295343,6.21364572242368,
11.3270764010038));
#186229=CARTESIAN_POINT('Ctrl Pts',(-2.85518555380003,6.13516132252214,
11.3358262212621));
#186230=CARTESIAN_POINT('Ctrl Pts',(-3.02382794858707,6.05667841000498,
11.3445758756996));
#186231=CARTESIAN_POINT('Ctrl Pts',(-3.18923239109303,5.97123819492069,
11.3533255301372));
#186232=CARTESIAN_POINT('Ctrl Pts',(-3.35083705967724,5.87913088810699,
11.3620751845747));
#186233=CARTESIAN_POINT('Ctrl Pts',(-3.51243888042421,5.7870252044309,11.3708246848236));
#186234=CARTESIAN_POINT('Ctrl Pts',(-3.67024081223708,5.68825280605772,
11.3795741850725));
#186235=CARTESIAN_POINT('Ctrl Pts',(-3.82370687544415,5.58314917682495,
11.3883236853215));
#186236=CARTESIAN_POINT('Ctrl Pts',(-3.97717043817821,5.47804726008016,
11.3970730430119));
#186237=CARTESIAN_POINT('Ctrl Pts',(-4.12629803722459,5.36661448084237,
11.4058224007024));
#186238=CARTESIAN_POINT('Ctrl Pts',(-4.27058317206899,5.24922931204583,
11.4145717583929));
#186239=CARTESIAN_POINT('Ctrl Pts',(-4.4148661477481,5.13184589986811,11.4233209851529));
#186240=CARTESIAN_POINT('Ctrl Pts',(-4.55430658194374,5.0085104572307,11.432070211913));
#186241=CARTESIAN_POINT('Ctrl Pts',(-4.68843089001792,4.8796418710317,11.4408194386731));
#186242=CARTESIAN_POINT('Ctrl Pts',(-4.8225533691777,4.75077504208027,11.449568546129));
#186243=CARTESIAN_POINT('Ctrl Pts',(-4.95135966065056,4.61637541908176,
11.4583176535849));
#186244=CARTESIAN_POINT('Ctrl Pts',(-5.07441230869156,4.47689945401945,
11.4670667610408));
#186245=CARTESIAN_POINT('Ctrl Pts',(-5.19746344226316,4.33742520555636,
11.4758157608172));
#186246=CARTESIAN_POINT('Ctrl Pts',(-5.31476088454655,4.19287495491478,
11.4845647605935));
#186247=CARTESIAN_POINT('Ctrl Pts',(-5.42590627628732,4.04373961586869,
11.4933137603699));
#186248=CARTESIAN_POINT('Ctrl Pts',(-5.53706380672551,3.894587989069,11.5020637156646));
#186249=CARTESIAN_POINT('Ctrl Pts',(-5.64206777071753,3.74085050155452,
11.5108136709593));
#186250=CARTESIAN_POINT('Ctrl Pts',(-5.74056148163902,3.58304938223331,
11.519563626254));
#186251=CARTESIAN_POINT('Ctrl Pts',(-5.83905138951775,3.42525435593466,
11.5283132436951));
#186252=CARTESIAN_POINT('Ctrl Pts',(-5.93103139557543,3.26339625497381,
11.5370628611362));
#186253=CARTESIAN_POINT('Ctrl Pts',(-6.01618907820737,3.09802485065217,
11.5458124785773));
#186254=CARTESIAN_POINT('Ctrl Pts',(-6.10134392544891,2.93265895249834,
11.5545618046932));
#186255=CARTESIAN_POINT('Ctrl Pts',(-6.17967677261754,2.7637802398621,11.563311130809));
#186256=CARTESIAN_POINT('Ctrl Pts',(-6.2509215700916,2.59196229227271,11.5720604569249));
#186257=CARTESIAN_POINT('Ctrl Pts',(-6.32216437407699,2.42014915229234,
11.5808095382274));
#186258=CARTESIAN_POINT('Ctrl Pts',(-6.38631941548876,2.2453972066298,11.5895586195298));
#186259=CARTESIAN_POINT('Ctrl Pts',(-6.443168810375,2.06829994947802,11.5983077008323));
#186260=CARTESIAN_POINT('Ctrl Pts',(-6.5000233452454,1.89118668024558,11.6070575731746));
#186261=CARTESIAN_POINT('Ctrl Pts',(-6.5495708241107,1.71172794807804,11.615807445517));
#186262=CARTESIAN_POINT('Ctrl Pts',(-6.59164294296062,1.53053334250434,
11.6245573178594));
#186263=CARTESIAN_POINT('Ctrl Pts',(-6.63371214082116,1.34935131693688,
11.6333065827143));
#186264=CARTESIAN_POINT('Ctrl Pts',(-6.66830695239675,1.16643393829848,
11.6420558475692));
#186265=CARTESIAN_POINT('Ctrl Pts',(-6.69530988153977,0.982402458341779,
11.6508051124241));
#186266=CARTESIAN_POINT('Ctrl Pts',(-6.72231419690474,0.79836153094786,
11.6595548264311));
#186267=CARTESIAN_POINT('Ctrl Pts',(-6.7417258082927,0.613206671363291,
11.6683045404381));
#186268=CARTESIAN_POINT('Ctrl Pts',(-6.75347878028174,0.427566795114224,
11.6770542544452));
#186269=CARTESIAN_POINT('Ctrl Pts',(-6.76248992368214,0.285234494205681,
11.6837627642334));
#186270=CARTESIAN_POINT('Ctrl Pts',(-6.76699999999998,0.142617266092119,
11.6904712740217));
#186271=CARTESIAN_POINT('Ctrl Pts',(-6.767,1.00878458448079E-12,11.69717978381));
#186272=CARTESIAN_POINT('',(-6.76699818449147,0.00495692335195666,11.3028202161557));
#186273=CARTESIAN_POINT('Ctrl Pts',(3.09910619832133,6.01563211736941,10.651525285013));
#186274=CARTESIAN_POINT('Ctrl Pts',(2.93889730946949,6.09816780950944,10.6599751073476));
#186275=CARTESIAN_POINT('Ctrl Pts',(2.77531112510111,6.17433926859913,10.6684249296823));
#186276=CARTESIAN_POINT('Ctrl Pts',(2.60889777959418,6.24387230615974,10.6768747520169));
#186277=CARTESIAN_POINT('Ctrl Pts',(2.44248443408725,6.31340534372035,10.6853245743516));
#186278=CARTESIAN_POINT('Ctrl Pts',(2.27324429892826,6.37629978527336,10.6937743966863));
#186279=CARTESIAN_POINT('Ctrl Pts',(2.10175175536633,6.43233461185086,10.7022242190209));
#186280=CARTESIAN_POINT('Ctrl Pts',(1.92198972526209,6.49107147569867,10.7110814975086));
#186281=CARTESIAN_POINT('Ctrl Pts',(1.73994024598263,6.54221110080664,10.7199387759964));
#186282=CARTESIAN_POINT('Ctrl Pts',(1.55624274932444,6.58562051026136,10.7287960544841));
#186283=CARTESIAN_POINT('Ctrl Pts',(1.37220179041347,6.6291110830081,10.7376698935722));
#186284=CARTESIAN_POINT('Ctrl Pts',(1.18650690895843,6.6648424965498,10.7465437326602));
#186285=CARTESIAN_POINT('Ctrl Pts',(0.999805918544201,6.69273315807854,
10.7554175717483));
#186286=CARTESIAN_POINT('Ctrl Pts',(0.812574071119657,6.72070312263168,
10.7643166423024));
#186287=CARTESIAN_POINT('Ctrl Pts',(0.624330648419938,6.74078768343343,
10.7732157128564));
#186288=CARTESIAN_POINT('Ctrl Pts',(0.435729855818093,6.75295701842895,
10.7821147834104));
#186289=CARTESIAN_POINT('Ctrl Pts',(0.246873554445342,6.76514283995023,
10.7910259100675));
#186290=CARTESIAN_POINT('Ctrl Pts',(0.0576591754872288,6.76939200528491,
10.7999370367245));
#186291=CARTESIAN_POINT('Ctrl Pts',(-0.131259506601047,6.76572685983752,
10.8088481633815));
#186292=CARTESIAN_POINT('Ctrl Pts',(-0.320596891080043,6.76205359129111,
10.8177790398589));
#186293=CARTESIAN_POINT('Ctrl Pts',(-0.509637007248433,6.75043093280429,
10.8267099163363));
#186294=CARTESIAN_POINT('Ctrl Pts',(-0.697728744206054,6.73093333791894,
10.8356407928137));
#186295=CARTESIAN_POINT('Ctrl Pts',(-0.877011172364044,6.7123489162382,
10.8441533901577));
#186296=CARTESIAN_POINT('Ctrl Pts',(-1.05543183885851,6.68661035022064,
10.8526659875017));
#186297=CARTESIAN_POINT('Ctrl Pts',(-1.23243601784636,6.65382525032894,
10.8611785848456));
#186298=CARTESIAN_POINT('Ctrl Pts',(-1.40341669656413,6.62215583628817,
10.8694014961907));
#186299=CARTESIAN_POINT('Ctrl Pts',(-1.57340328579009,6.58384963638255,
10.8776244075358));
#186300=CARTESIAN_POINT('Ctrl Pts',(-1.74184244167911,6.53898110628601,
10.8858473188808));
#186301=CARTESIAN_POINT('Ctrl Pts',(-1.9101033665741,6.49416005305242,10.8940615292938));
#186302=CARTESIAN_POINT('Ctrl Pts',(-2.07681977496709,6.44279058857545,
10.9022757397067));
#186303=CARTESIAN_POINT('Ctrl Pts',(-2.24144668537069,6.38499849308054,
10.9104899501196));
#186304=CARTESIAN_POINT('Ctrl Pts',(-2.40593244616417,6.32725594800073,
10.9186971177435));
#186305=CARTESIAN_POINT('Ctrl Pts',(-2.56833194039352,6.26310185713325,
10.9269042853675));
#186306=CARTESIAN_POINT('Ctrl Pts',(-2.72811348288888,6.19271231565619,
10.9351114529914));
#186307=CARTESIAN_POINT('Ctrl Pts',(-2.8877900958395,6.12236899943411,10.9433132309166));
#186308=CARTESIAN_POINT('Ctrl Pts',(-3.04485185446441,6.04579853317224,
10.9515150088419));
#186309=CARTESIAN_POINT('Ctrl Pts',(-3.19878518083012,5.9632258356448,10.9597167867672));
#186310=CARTESIAN_POINT('Ctrl Pts',(-3.35264830393675,5.88069079645045,
10.9679148241669));
#186311=CARTESIAN_POINT('Ctrl Pts',(-3.50338552179908,5.79215914876494,
10.9761128615666));
#186312=CARTESIAN_POINT('Ctrl Pts',(-3.65050600445879,5.69790267654778,
10.9843108989663));
#186313=CARTESIAN_POINT('Ctrl Pts',(-3.79761354436566,5.6036544964338,10.9925082151533));
#186314=CARTESIAN_POINT('Ctrl Pts',(-3.94110467640356,5.50368268109398,
11.0007055313402));
#186315=CARTESIAN_POINT('Ctrl Pts',(-4.08051551316418,5.3983036360348,11.0089028475272));
#186316=CARTESIAN_POINT('Ctrl Pts',(-4.21992482153698,5.29292574626635,
11.0171000738454));
#186317=CARTESIAN_POINT('Ctrl Pts',(-4.35525363684475,5.18214096035967,
11.0252973001635));
#186318=CARTESIAN_POINT('Ctrl Pts',(-4.48606937660464,5.06630738786052,
11.0334945264817));
#186319=CARTESIAN_POINT('Ctrl Pts',(-4.61690746497943,4.9504540263061,11.0416931532174));
#186320=CARTESIAN_POINT('Ctrl Pts',(-4.7432306730703,4.82955039760395,11.0498917799532));
#186321=CARTESIAN_POINT('Ctrl Pts',(-4.86464162644933,4.70399307463526,
11.0580904066889));
#186322=CARTESIAN_POINT('Ctrl Pts',(-4.98609539491333,4.578391474381,11.0662919246374));
#186323=CARTESIAN_POINT('Ctrl Pts',(-5.10263320865769,4.4481331685404,11.0744934425859));
#186324=CARTESIAN_POINT('Ctrl Pts',(-5.21389646118121,4.31364957919417,
11.0826949605344));
#186325=CARTESIAN_POINT('Ctrl Pts',(-5.32528642644745,4.17901283250201,
11.0909058188249));
#186326=CARTESIAN_POINT('Ctrl Pts',(-5.43138960068738,4.04014146555799,
11.0991166771154));
#186327=CARTESIAN_POINT('Ctrl Pts',(-5.53188876505622,3.89749864541924,
11.1073275354059));
#186328=CARTESIAN_POINT('Ctrl Pts',(-5.63244715625975,3.75477176206682,
11.115543232574));
#186329=CARTESIAN_POINT('Ctrl Pts',(-5.72739475955337,3.60826929567592,
11.123758929742));
#186330=CARTESIAN_POINT('Ctrl Pts',(-5.8164592843317,3.45848093730638,11.13197462691));
#186331=CARTESIAN_POINT('Ctrl Pts',(-5.9056619794547,3.30846020460872,11.1402030695086));
#186332=CARTESIAN_POINT('Ctrl Pts',(-5.98896318609218,3.15514370804712,
11.1484315121071));
#186333=CARTESIAN_POINT('Ctrl Pts',(-6.06613732808664,2.99904433391604,
11.1566599547056));
#186334=CARTESIAN_POINT('Ctrl Pts',(-6.1362523542124,2.85722336367187,11.1641357419688));
#186335=CARTESIAN_POINT('Ctrl Pts',(-6.20131046664306,2.71310577237175,
11.171611529232));
#186336=CARTESIAN_POINT('Ctrl Pts',(-6.2611780300233,2.56708758642038,11.1790873164952));
#186337=CARTESIAN_POINT('Ctrl Pts',(-6.33388635258981,2.38975053167341,
11.1881665560881));
#186338=CARTESIAN_POINT('Ctrl Pts',(-6.39914195040219,2.20911460084561,
11.1972457956809));
#186339=CARTESIAN_POINT('Ctrl Pts',(-6.45666022227768,2.02579065405515,
11.2063250352738));
#186340=CARTESIAN_POINT('Ctrl Pts',(-6.51389912282271,1.843357127878,11.2153601761975));
#186341=CARTESIAN_POINT('Ctrl Pts',(-6.56347555581142,1.65826183282316,
11.2243953171212));
#186342=CARTESIAN_POINT('Ctrl Pts',(-6.60515402599733,1.4711319766939,11.2334304580448));
#186343=CARTESIAN_POINT('Ctrl Pts',(-6.64670601382407,1.28457000670751,
11.2424381798734));
#186344=CARTESIAN_POINT('Ctrl Pts',(-6.68040777661328,1.09598600498177,
11.2514459017019));
#186345=CARTESIAN_POINT('Ctrl Pts',(-6.70607263333926,0.906023640076943,
11.2604536235304));
#186346=CARTESIAN_POINT('Ctrl Pts',(-6.73161310095464,0.71698196021121,
11.269417687897));
#186347=CARTESIAN_POINT('Ctrl Pts',(-6.74919427707081,0.52657545879325,
11.2783817522635));
#186348=CARTESIAN_POINT('Ctrl Pts',(-6.75868014845368,0.335457375680179,
11.28734581663));
#186349=CARTESIAN_POINT('Ctrl Pts',(-6.76413854164175,0.225483541872191,
11.2925039498053));
#186350=CARTESIAN_POINT('Ctrl Pts',(-6.7669173753356,0.115274427227421,
11.2976620829805));
#186351=CARTESIAN_POINT('Ctrl Pts',(-6.76699818449147,0.00495692335193946,
11.3028202161557));
#186352=CARTESIAN_POINT('Ctrl Pts',(-6.76699818449201,0.00495692262024367,
11.3028202161899));
#186353=CARTESIAN_POINT('Ctrl Pts',(-6.76712508573948,-0.168283730312138,
11.3109204571108));
#186354=CARTESIAN_POINT('Ctrl Pts',(-6.76059500658483,-0.341555143110208,
11.3190206980317));
#186355=CARTESIAN_POINT('Ctrl Pts',(-6.74742764060013,-0.514304612914761,
11.3271209389526));
#186356=CARTESIAN_POINT('Ctrl Pts',(-6.73425896758729,-0.687071230295947,
11.3352219839252));
#186357=CARTESIAN_POINT('Ctrl Pts',(-6.71445172225605,-0.859315435977075,
11.3433230288978));
#186358=CARTESIAN_POINT('Ctrl Pts',(-6.6880775739972,-1.03048889571683,
11.3514240738704));
#186359=CARTESIAN_POINT('Ctrl Pts',(-6.66169577561294,-1.20171200628977,
11.3595274686443));
#186360=CARTESIAN_POINT('Ctrl Pts',(-6.62874333622474,-1.3718633902453,
11.3676308634183));
#186361=CARTESIAN_POINT('Ctrl Pts',(-6.58934320424099,-1.54040421212198,
11.3757342581923));
#186362=CARTESIAN_POINT('Ctrl Pts',(-6.54992412541367,-1.70902608237146,
11.3838415497489));
#186363=CARTESIAN_POINT('Ctrl Pts',(-6.50405126239577,-1.87603549180717,
11.3919488413056));
#186364=CARTESIAN_POINT('Ctrl Pts',(-6.45189762645819,-2.04090813553752,
11.4000561328623));
#186365=CARTESIAN_POINT('Ctrl Pts',(-6.39967184979173,-2.2060088368611,
11.4081746387075));
#186366=CARTESIAN_POINT('Ctrl Pts',(-6.34114805599682,-2.36896651875642,
11.4162931445527));
#186367=CARTESIAN_POINT('Ctrl Pts',(-6.27654808583317,-2.52927521757202,
11.4244116503979));
#186368=CARTESIAN_POINT('Ctrl Pts',(-6.211902004502,-2.68969834401427,11.432535951196));
#186369=CARTESIAN_POINT('Ctrl Pts',(-6.14117125563026,-2.84746838735584,
11.4406602519941));
#186370=CARTESIAN_POINT('Ctrl Pts',(-6.06462381628711,-3.00210375685505,
11.4487845527922));
#186371=CARTESIAN_POINT('Ctrl Pts',(-5.98793678504328,-3.15702111939447,
11.4569236690643));
#186372=CARTESIAN_POINT('Ctrl Pts',(-5.90541204317221,-3.30879206499058,
11.4650627853363));
#186373=CARTESIAN_POINT('Ctrl Pts',(-5.81736185239714,-3.45696255089269,
11.4732019016083));
#186374=CARTESIAN_POINT('Ctrl Pts',(-5.73155896045956,-3.60135129188561,
11.4811332837871));
#186375=CARTESIAN_POINT('Ctrl Pts',(-5.64050946324707,-3.74232091358637,
11.4890646659659));
#186376=CARTESIAN_POINT('Ctrl Pts',(-5.54453817086657,-3.87948262939836,
11.4969960481447));
#186377=CARTESIAN_POINT('Ctrl Pts',(-5.44370899934471,-4.02358720303489,
11.505328901379));
#186378=CARTESIAN_POINT('Ctrl Pts',(-5.33712880616364,-4.16394350491165,
11.5136617546133));
#186379=CARTESIAN_POINT('Ctrl Pts',(-5.22510181678832,-4.30006976736372,
11.5219946078476));
#186380=CARTESIAN_POINT('Ctrl Pts',(-5.11320722602375,-4.43603514958382,
11.5303176129355));
#186381=CARTESIAN_POINT('Ctrl Pts',(-4.99587888182987,-4.56778018490212,
11.5386406180234));
#186382=CARTESIAN_POINT('Ctrl Pts',(-4.87346418341003,-4.69485205869361,
11.5469636231113));
#186383=CARTESIAN_POINT('Ctrl Pts',(-4.75117168868107,-4.82179707964647,
11.5552783195406));
#186384=CARTESIAN_POINT('Ctrl Pts',(-4.62380319581286,-4.94407798442775,
11.5635930159698));
#186385=CARTESIAN_POINT('Ctrl Pts',(-4.49174639335769,-5.06127487277249,
11.5719077123991));
#186386=CARTESIAN_POINT('Ctrl Pts',(-4.35979719460836,-5.17837626569962,
11.580215633773));
#186387=CARTESIAN_POINT('Ctrl Pts',(-4.22316755740045,-5.29040166670229,
11.5885235551469));
#186388=CARTESIAN_POINT('Ctrl Pts',(-4.08228220897734,-5.39696775664512,
11.5968314765208));
#186389=CARTESIAN_POINT('Ctrl Pts',(-3.94148582705851,-5.5034665520637,
11.6051341515953));
#186390=CARTESIAN_POINT('Ctrl Pts',(-3.79643936632356,-5.60451269747081,
11.6134368266698));
#186391=CARTESIAN_POINT('Ctrl Pts',(-3.64760100598947,-5.69976279340681,
11.6217395017442));
#186392=CARTESIAN_POINT('Ctrl Pts',(-3.49882347594604,-5.79497396059482,
11.6300387835125));
#186393=CARTESIAN_POINT('Ctrl Pts',(-3.34625742689429,-5.88439361116354,
11.6383380652807));
#186394=CARTESIAN_POINT('Ctrl Pts',(-3.19039065887923,-5.96772121028925,
11.6466373470489));
#186395=CARTESIAN_POINT('Ctrl Pts',(-3.03455704324672,-6.0510310858907,
11.6549348635854));
#186396=CARTESIAN_POINT('Ctrl Pts',(-2.87542441393954,-6.12825132756268,
11.6632323801219));
#186397=CARTESIAN_POINT('Ctrl Pts',(-2.71350606206983,-6.19912686199519,
11.6715298966584));
#186398=CARTESIAN_POINT('Ctrl Pts',(-2.55159524091372,-6.26999910005427,
11.679827027283));
#186399=CARTESIAN_POINT('Ctrl Pts',(-2.38689927413735,-6.33452707955494,
11.6881241579076));
#186400=CARTESIAN_POINT('Ctrl Pts',(-2.2199525381012,-6.39250340074826,
11.6964212885322));
#186401=CARTESIAN_POINT('Ctrl Pts',(-2.0529858234046,-6.45048666001813,
11.7047194120816));
#186402=CARTESIAN_POINT('Ctrl Pts',(-1.88376813156692,-6.50191658512377,
11.713017535631));
#186403=CARTESIAN_POINT('Ctrl Pts',(-1.71285032473928,-6.5466352246815,
11.7213156591804));
#186404=CARTESIAN_POINT('Ctrl Pts',(-1.54181229773543,-6.59138531843833,
11.7296196194643));
#186405=CARTESIAN_POINT('Ctrl Pts',(-1.36907210323849,-6.62941460582099,
11.7379235797483));
#186406=CARTESIAN_POINT('Ctrl Pts',(-1.19519304639963,-6.66061578097986,
11.7462275400323));
#186407=CARTESIAN_POINT('Ctrl Pts',(-1.02125075704963,-6.69182830269589,
11.7545345201179));
#186408=CARTESIAN_POINT('Ctrl Pts',(-0.846169123591691,-6.71620770889585,
11.7628415002036));
#186409=CARTESIAN_POINT('Ctrl Pts',(-0.67051819155781,-6.73369841578832,
11.7711484802892));
#186410=CARTESIAN_POINT('Ctrl Pts',(-0.494679437028176,-6.75120782538951,
11.7794643429792));
#186411=CARTESIAN_POINT('Ctrl Pts',(-0.318270514757428,-6.76181379111098,
11.7877802056691));
#186412=CARTESIAN_POINT('Ctrl Pts',(-0.141864212426566,-6.76551280726248,
11.7960960683591));
#186413=CARTESIAN_POINT('Ctrl Pts',(-0.00886637605910517,-6.76830160300468,
11.8023656388375));
#186414=CARTESIAN_POINT('Ctrl Pts',(0.124129918561489,-6.76716550414954,
11.8086352093159));
#186415=CARTESIAN_POINT('Ctrl Pts',(0.256880684272667,-6.7621225450333,
11.8149047797942));
#186416=CARTESIAN_POINT('Ctrl Pts',(0.435807109389025,-6.75532545695744,
11.823355140338));
#186417=CARTESIAN_POINT('Ctrl Pts',(0.614615459470383,-6.74141665938708,
11.8318055008817));
#186418=CARTESIAN_POINT('Ctrl Pts',(0.792717641896063,-6.72040830160094,
11.8402558614254));
#186419=CARTESIAN_POINT('Ctrl Pts',(0.970662638890027,-6.69941848490027,
11.8486987640393));
#186420=CARTESIAN_POINT('Ctrl Pts',(1.14790238269182,-6.67134163545978,
11.8571416666532));
#186421=CARTESIAN_POINT('Ctrl Pts',(1.32385153293246,-6.63624186710765,
11.8655845692671));
#186422=CARTESIAN_POINT('Ctrl Pts',(1.49966934960006,-6.60116829824544,
11.8740211698525));
#186423=CARTESIAN_POINT('Ctrl Pts',(1.67419816896492,-6.5590823249825,11.8824577704379));
#186424=CARTESIAN_POINT('Ctrl Pts',(1.846860113013,-6.51009959393569,11.8908943710233));
#186425=CARTESIAN_POINT('Ctrl Pts',(2.01939848651896,-6.46115191880502,
11.8993249337101));
#186426=CARTESIAN_POINT('Ctrl Pts',(2.190072331533,-6.405317421545,11.9077554963969));
#186427=CARTESIAN_POINT('Ctrl Pts',(2.35831606067142,-6.34276236020074,
11.9161860590837));
#186428=CARTESIAN_POINT('Ctrl Pts',(2.52648744799916,-6.28023419642008,
11.9246129967785));
#186429=CARTESIAN_POINT('Ctrl Pts',(2.69223049229545,-6.21099134466006,
11.9330399344733));
#186430=CARTESIAN_POINT('Ctrl Pts',(2.85499618850421,-6.13524944591713,
11.9414668721681));
#186431=CARTESIAN_POINT('Ctrl Pts',(3.01771161748824,-6.05953093868196,
11.9498912073565));
#186432=CARTESIAN_POINT('Ctrl Pts',(3.17745123182088,-5.97731752685017,
11.9583155425449));
#186433=CARTESIAN_POINT('Ctrl Pts',(3.33368704687592,-5.88887252990687,
11.9667398777332));
#186434=CARTESIAN_POINT('Ctrl Pts',(3.37769782421941,-5.86395805644734,
11.9691129670285));
#186435=CARTESIAN_POINT('Ctrl Pts',(3.42143070900545,-5.83854938012263,
11.9714860563238));
#186436=CARTESIAN_POINT('Ctrl Pts',(3.46487424383564,-5.81265304954669,
11.973859145619));
#186437=CARTESIAN_POINT('Ctrl Pts',(3.62265528470566,-5.71860108050327,
11.9824778848755));
#186438=CARTESIAN_POINT('Ctrl Pts',(3.77654702435987,-5.61815541635785,
11.9910966241321));
#186439=CARTESIAN_POINT('Ctrl Pts',(3.92604282991348,-5.51166732465639,
11.9997153633886));
#186440=CARTESIAN_POINT('Ctrl Pts',(4.07562842444101,-5.40511527492981,
12.0083392791633));
#186441=CARTESIAN_POINT('Ctrl Pts',(4.22081256797821,-5.29251373143548,
12.016963194938));
#186442=CARTESIAN_POINT('Ctrl Pts',(4.36112037061277,-5.17425531965967,
12.0255871107127));
#186443=CARTESIAN_POINT('Ctrl Pts',(4.50649807242136,-5.05172374407595,
12.0345226441069));
#186444=CARTESIAN_POINT('Ctrl Pts',(4.64664018478396,-4.92311910217486,
12.0434581775012));
#186445=CARTESIAN_POINT('Ctrl Pts',(4.78105925776186,-4.78892068986005,
12.0523937108955));
#186446=CARTESIAN_POINT('Ctrl Pts',(4.91103314005587,-4.65916017105989,
12.0610337493951));
#186447=CARTESIAN_POINT('Ctrl Pts',(5.03565626845823,-4.52417018231745,
12.0696737878948));
#186448=CARTESIAN_POINT('Ctrl Pts',(5.1545280269216,-4.3844189831356,12.0783138263945));
#186449=CARTESIAN_POINT('Ctrl Pts',(5.2794980217072,-4.23749841210341,12.087397107236));
#186450=CARTESIAN_POINT('Ctrl Pts',(5.39811079960517,-4.08531559718512,
12.0964803880776));
#186451=CARTESIAN_POINT('Ctrl Pts',(5.509951105094,-3.92845107128413,12.1055636689191));
#186452=CARTESIAN_POINT('Ctrl Pts',(5.62179141058283,-3.77158654538314,
12.1146469497607));
#186453=CARTESIAN_POINT('Ctrl Pts',(5.72685906044004,-3.6100406519454,12.1237302306022));
#186454=CARTESIAN_POINT('Ctrl Pts',(5.82479323757426,-3.4444263295227,12.1328135114438));
#186455=CARTESIAN_POINT('Ctrl Pts',(5.92231027499043,-3.27951742285762,
12.1418581030624));
#186456=CARTESIAN_POINT('Ctrl Pts',(6.01284529465068,-3.11042281667467,
12.1509026946811));
#186457=CARTESIAN_POINT('Ctrl Pts',(6.0960680090668,-2.93772766417046,12.1599472862997));
#186458=CARTESIAN_POINT('Ctrl Pts',(6.17921435137585,-2.76519099114829,
12.1689835778464));
#186459=CARTESIAN_POINT('Ctrl Pts',(6.2550616825633,-2.58906058270296,12.1780198693931));
#186460=CARTESIAN_POINT('Ctrl Pts',(6.32332611385161,-2.4099451981077,12.1870561609397));
#186461=CARTESIAN_POINT('Ctrl Pts',(6.39146974364527,-2.23114677808337,
12.1960764617647));
#186462=CARTESIAN_POINT('Ctrl Pts',(6.45205718452823,-2.04937415189009,
12.2050967625896));
#186463=CARTESIAN_POINT('Ctrl Pts',(6.50485306452033,-1.86525483754914,
12.2141170634146));
#186464=CARTESIAN_POINT('Ctrl Pts',(6.55758245756461,-1.68136738848343,
12.2231260047874));
#186465=CARTESIAN_POINT('Ctrl Pts',(6.60253980586729,-1.49513937689381,
12.2321349461602));
#186466=CARTESIAN_POINT('Ctrl Pts',(6.63953905318681,-1.30721465766234,
12.2411438875331));
#186467=CARTESIAN_POINT('Ctrl Pts',(6.67645428235687,-1.11971667919699,
12.2501323713389));
#186468=CARTESIAN_POINT('Ctrl Pts',(6.70544743656993,-0.930529916784176,
12.2591208551446));
#186469=CARTESIAN_POINT('Ctrl Pts',(6.7263832312889,-0.740309142072052,
12.2681093389504));
#186470=CARTESIAN_POINT('Ctrl Pts',(6.74475156096796,-0.573416127088918,
12.2759955183898));
#186471=CARTESIAN_POINT('Ctrl Pts',(6.75691828104992,-0.405727484273719,
12.2838816978292));
#186472=CARTESIAN_POINT('Ctrl Pts',(6.76282418892797,-0.237693057641016,
12.2917678772685));
#186473=CARTESIAN_POINT('Ctrl Pts',(6.76890630704458,-0.0646451111544109,
12.2998893508555));
#186474=CARTESIAN_POINT('Ctrl Pts',(6.76834408385886,0.108692148906018,
12.3080108244426));
#186475=CARTESIAN_POINT('Ctrl Pts',(6.76113132972388,0.281766112629207,
12.3161322980296));
#186476=CARTESIAN_POINT('Ctrl Pts',(6.75391908983964,0.454827736625934,
12.3242531925765));
#186477=CARTESIAN_POINT('Ctrl Pts',(6.74005727872453,0.627625735809023,
12.3323740871235));
#186478=CARTESIAN_POINT('Ctrl Pts',(6.71959179976489,0.799609307432327,
12.3404949816704));
#186479=CARTESIAN_POINT('Ctrl Pts',(6.69912387426174,0.97161343881346,12.3486168470288));
#186480=CARTESIAN_POINT('Ctrl Pts',(6.67205075343001,1.14280258529562,12.3567387123872));
#186481=CARTESIAN_POINT('Ctrl Pts',(6.63846999344241,1.31263290609553,12.3648605777456));
#186482=CARTESIAN_POINT('Ctrl Pts',(6.60486473266487,1.48258713645004,12.3729883688817));
#186483=CARTESIAN_POINT('Ctrl Pts',(6.5647424207357,1.65118020140671,12.3811161600178));
#186484=CARTESIAN_POINT('Ctrl Pts',(6.51825150012339,1.81787963879327,12.3892439511538));
#186485=CARTESIAN_POINT('Ctrl Pts',(6.47174164026241,1.98464698539859,12.3973750533505));
#186486=CARTESIAN_POINT('Ctrl Pts',(6.41885811208877,2.14951881834082,12.4055061555472));
#186487=CARTESIAN_POINT('Ctrl Pts',(6.35979859513314,2.31197985054857,12.4136372577439));
#186488=CARTESIAN_POINT('Ctrl Pts',(6.30067461642269,2.47461820427479,12.4217772348035));
#186489=CARTESIAN_POINT('Ctrl Pts',(6.23536132314184,2.6348401629617,12.4299172118631));
#186490=CARTESIAN_POINT('Ctrl Pts',(6.16410399743514,2.79215166293025,12.4380571889228));
#186491=CARTESIAN_POINT('Ctrl Pts',(6.12714738672581,2.87373906193492,12.4422788736463));
#186492=CARTESIAN_POINT('Ctrl Pts',(6.08859268529131,2.95454400240605,12.4465005583698));
#186493=CARTESIAN_POINT('Ctrl Pts',(6.04847883432448,3.0345004186404,12.4507222430933));
#186494=CARTESIAN_POINT('Ctrl Pts',(5.96828790539243,3.19433995379777,12.4591617424552));
#186495=CARTESIAN_POINT('Ctrl Pts',(5.88169770739263,3.35111725224016,12.4676012418171));
#186496=CARTESIAN_POINT('Ctrl Pts',(5.78896636304306,3.50430555853169,12.476040741179));
#186497=CARTESIAN_POINT('Ctrl Pts',(5.69630145699581,3.65738411152374,12.4844741939768));
#186498=CARTESIAN_POINT('Ctrl Pts',(5.59750434589849,3.80687851312266,12.4929076467747));
#186499=CARTESIAN_POINT('Ctrl Pts',(5.49287909107333,3.95228646366244,12.5013410995726));
#186500=CARTESIAN_POINT('Ctrl Pts',(5.38831415579666,4.09761058222556,12.5097696902359));
#186501=CARTESIAN_POINT('Ctrl Pts',(5.27792796886108,4.23885267598187,12.5181982808992));
#186502=CARTESIAN_POINT('Ctrl Pts',(5.16206813503634,4.37553900328205,12.5266268715625));
#186503=CARTESIAN_POINT('Ctrl Pts',(5.04625890084728,4.51216563536141,12.5350517811951));
#186504=CARTESIAN_POINT('Ctrl Pts',(4.92498100096567,4.64424021375626,12.5434766908276));
#186505=CARTESIAN_POINT('Ctrl Pts',(4.79862281664325,4.77132141692328,12.5519016004601));
#186506=CARTESIAN_POINT('Ctrl Pts',(4.67229083962043,4.89837626283309,12.5603247627256));
#186507=CARTESIAN_POINT('Ctrl Pts',(4.54088091140313,5.02043955963395,12.568747924991));
#186508=CARTESIAN_POINT('Ctrl Pts',(4.40481919147689,5.13710588662497,12.5771710872565));
#186509=CARTESIAN_POINT('Ctrl Pts',(4.26877963526478,5.25375320930587,12.5855928774346));
#186510=CARTESIAN_POINT('Ctrl Pts',(4.12809005261554,5.36500509961155,12.5940146676128));
#186511=CARTESIAN_POINT('Ctrl Pts',(3.98321083474644,5.47049544794241,12.6024364577909));
#186512=CARTESIAN_POINT('Ctrl Pts',(3.83830037511403,5.57600854421835,12.6108600640444));
#186513=CARTESIAN_POINT('Ctrl Pts',(3.68919874271934,5.67575741680091,12.6192836702978));
#186514=CARTESIAN_POINT('Ctrl Pts',(3.53639718849143,5.76941798843089,12.6277072765513));
#186515=CARTESIAN_POINT('Ctrl Pts',(3.39371871989328,5.8568735578177,12.6355728198463));
#186516=CARTESIAN_POINT('Ctrl Pts',(3.24781480299861,5.93902108971557,12.6434383631413));
#186517=CARTESIAN_POINT('Ctrl Pts',(3.09910619832131,6.01563211736941,12.6513039064363));
#186518=CARTESIAN_POINT('Origin',(0.,0.,4.30282021618968));
#186519=CARTESIAN_POINT('',(3.09910619832132,6.01563211736941,15.0460438035976));
#186520=CARTESIAN_POINT('',(3.09910619832135,6.0156321173694,14.6512308626299));
#186521=CARTESIAN_POINT('',(3.09910619832133,6.0156321173694,4.30282021618968));
#186522=CARTESIAN_POINT('',(-6.76699998297921,-0.000479957709509463,13.6971797837721));
#186523=CARTESIAN_POINT('Ctrl Pts',(-6.76699998297915,-0.000479958513274169,
13.69717978381));
#186524=CARTESIAN_POINT('Ctrl Pts',(-6.76699972950591,-0.00405371203792415,
13.6973484975525));
#186525=CARTESIAN_POINT('Ctrl Pts',(-6.76699664500473,-0.00762745138731119,
13.697517211295));
#186526=CARTESIAN_POINT('Ctrl Pts',(-6.76699072954348,-0.0112011728210126,
13.6976859250374));
#186527=CARTESIAN_POINT('Ctrl Pts',(-6.76667360689047,-0.202785222755277,
13.7067305197719));
#186528=CARTESIAN_POINT('Ctrl Pts',(-6.75821599951017,-0.394404825866598,
13.7157751145064));
#186529=CARTESIAN_POINT('Ctrl Pts',(-6.74163256529473,-0.585388208420326,
13.7248197092409));
#186530=CARTESIAN_POINT('Ctrl Pts',(-6.72506434899353,-0.776196333624015,
13.7338560041344));
#186531=CARTESIAN_POINT('Ctrl Pts',(-6.7003852138105,-0.966369167097182,
13.7428922990279));
#186532=CARTESIAN_POINT('Ctrl Pts',(-6.66766176604375,-1.15523831897938,
13.7519285939214));
#186533=CARTESIAN_POINT('Ctrl Pts',(-6.63499622498392,-1.34377325208668,
13.7609488983824));
#186534=CARTESIAN_POINT('Ctrl Pts',(-6.59431483746394,-1.53100887622529,
13.7699692028435));
#186535=CARTESIAN_POINT('Ctrl Pts',(-6.54573550536322,-1.71628543483517,
13.7789895073046));
#186536=CARTESIAN_POINT('Ctrl Pts',(-6.49721734948933,-1.90132867363011,
13.7879984524454));
#186537=CARTESIAN_POINT('Ctrl Pts',(-6.44082115783899,-2.0844175408772,
13.7970073975862));
#186538=CARTESIAN_POINT('Ctrl Pts',(-6.37671557869513,-2.26490340377396,
13.806016342727));
#186539=CARTESIAN_POINT('Ctrl Pts',(-6.31275556972657,-2.44497942155189,
13.815004830464));
#186540=CARTESIAN_POINT('Ctrl Pts',(-6.24112119699352,-2.62246400982848,
13.8239933182009));
#186541=CARTESIAN_POINT('Ctrl Pts',(-6.16203034063119,-2.79672506355929,
13.8329818059378));
#186542=CARTESIAN_POINT('Ctrl Pts',(-6.09263899295528,-2.94961516896424,
13.8408679675793));
#186543=CARTESIAN_POINT('Ctrl Pts',(-6.0175086694995,-3.10002398845393,
13.8487541292207));
#186544=CARTESIAN_POINT('Ctrl Pts',(-5.93681807242098,-3.24753447633365,
13.8566402908622));
#186545=CARTESIAN_POINT('Ctrl Pts',(-5.85371987056364,-3.39944630672915,
13.8647617557625));
#186546=CARTESIAN_POINT('Ctrl Pts',(-5.7647603992845,-3.54821548016966,
13.8728832206629));
#186547=CARTESIAN_POINT('Ctrl Pts',(-5.67021640192898,-3.69336363702461,
13.8810046855632));
#186548=CARTESIAN_POINT('Ctrl Pts',(-5.57567914694529,-3.83850144268993,
13.8891255712842));
#186549=CARTESIAN_POINT('Ctrl Pts',(-5.47555835902103,-3.98001843929452,
13.8972464570051));
#186550=CARTESIAN_POINT('Ctrl Pts',(-5.37017465501147,-4.11746441085682,
13.905367342726));
#186551=CARTESIAN_POINT('Ctrl Pts',(-5.26477835462964,-4.25492681115105,
13.9134891991255));
#186552=CARTESIAN_POINT('Ctrl Pts',(-5.15411810930141,-4.38831692759934,
13.921611055525));
#186553=CARTESIAN_POINT('Ctrl Pts',(-5.03855539966497,-4.51721689588921,
13.9297329119245));
#186554=CARTESIAN_POINT('Ctrl Pts',(-4.92290837689637,-4.64621090801118,
13.9378606939305));
#186555=CARTESIAN_POINT('Ctrl Pts',(-4.8023519907143,-4.77070795606198,
13.9459884759366));
#186556=CARTESIAN_POINT('Ctrl Pts',(-4.6772856720309,-4.89032593414942,
13.9541162579426));
#186557=CARTESIAN_POINT('Ctrl Pts',(-4.55216840597195,-5.00999264016071,
13.9622473509053));
#186558=CARTESIAN_POINT('Ctrl Pts',(-4.42253781936197,-5.12477607187367,
13.970378443868));
#186559=CARTESIAN_POINT('Ctrl Pts',(-4.28882691649475,-5.23433402452978,
13.9785095368308));
#186560=CARTESIAN_POINT('Ctrl Pts',(-4.15497007375995,-5.3440115551168,
13.9866495045419));
#186561=CARTESIAN_POINT('Ctrl Pts',(-4.01702431125062,-5.448451994301,13.9947894722531));
#186562=CARTESIAN_POINT('Ctrl Pts',(-3.8754527347774,-5.54735568541502,
14.0029294399643));
#186563=CARTESIAN_POINT('Ctrl Pts',(-3.80202759922334,-5.59865141233813,
14.0071511788719));
#186564=CARTESIAN_POINT('Ctrl Pts',(-3.72762759464339,-5.6484585394406,
14.0113729177794));
#186565=CARTESIAN_POINT('Ctrl Pts',(-3.65231993181482,-5.69674013060699,
14.015594656687));
#186566=CARTESIAN_POINT('Ctrl Pts',(-3.50176290752131,-5.79326593450448,
14.0240348661343));
#186567=CARTESIAN_POINT('Ctrl Pts',(-3.34726540711925,-5.88389109853242,
14.0324750755817));
#186568=CARTESIAN_POINT('Ctrl Pts',(-3.18931839142901,-5.96829432904349,
14.040915285029));
#186569=CARTESIAN_POINT('Ctrl Pts',(-3.03149104400764,-6.05263361160064,
14.0493490997671));
#186570=CARTESIAN_POINT('Ctrl Pts',(-2.87021968423866,-6.13076020114868,
14.0577829145051));
#186571=CARTESIAN_POINT('Ctrl Pts',(-2.70602223773671,-6.20239733078061,
14.0662167292432));
#186572=CARTESIAN_POINT('Ctrl Pts',(-2.54192395356688,-6.27399119722549,
14.074645450621));
#186573=CARTESIAN_POINT('Ctrl Pts',(-2.37490341057726,-6.33910328406654,
14.0830741719989));
#186574=CARTESIAN_POINT('Ctrl Pts',(-2.20550136003658,-6.39750363429962,
14.0915028933767));
#186575=CARTESIAN_POINT('Ctrl Pts',(-2.03617560196672,-6.45587768315675,
14.0999278187676));
#186576=CARTESIAN_POINT('Ctrl Pts',(-1.86447078962731,-6.50754591386063,
14.1083527441584));
#186577=CARTESIAN_POINT('Ctrl Pts',(-1.69094616812693,-6.55232707184988,
14.1167776695493));
#186578=CARTESIAN_POINT('Ctrl Pts',(-1.51747307193208,-6.59709493280481,
14.125200093296));
#186579=CARTESIAN_POINT('Ctrl Pts',(-1.34218156673801,-6.63497971598868,
14.1336225170427));
#186580=CARTESIAN_POINT('Ctrl Pts',(-1.16564490395299,-6.66585035519764,
14.1420449407894));
#186581=CARTESIAN_POINT('Ctrl Pts',(-0.989105464758191,-6.69672147991223,
14.1504674969964));
#186582=CARTESIAN_POINT('Ctrl Pts',(-0.811321156116721,-6.72057817626419,
14.1588900532034));
#186583=CARTESIAN_POINT('Ctrl Pts',(-0.63287490980961,-6.73734059911873,
14.1673126094104));
#186584=CARTESIAN_POINT('Ctrl Pts',(-0.454422635556327,-6.75410358821091,
14.1757354501328));
#186585=CARTESIAN_POINT('Ctrl Pts',(-0.275308711152397,-6.76377179460825,
14.1841582908553));
#186586=CARTESIAN_POINT('Ctrl Pts',(-0.0961208310274312,-6.76631729863761,
14.1925811315778));
#186587=CARTESIAN_POINT('Ctrl Pts',(0.083098118706693,-6.76886324403509,
14.2010054327471));
#186588=CARTESIAN_POINT('Ctrl Pts',(0.262390716203052,-6.76428402007166,
14.2094297339163));
#186589=CARTESIAN_POINT('Ctrl Pts',(0.441169254230898,-6.7526038451194,
14.2178540350856));
#186590=CARTESIAN_POINT('Ctrl Pts',(0.620003758002324,-6.74092001374573,
14.226280973441));
#186591=CARTESIAN_POINT('Ctrl Pts',(0.798323548744178,-6.72213082122644,
14.2347079117964));
#186592=CARTESIAN_POINT('Ctrl Pts',(0.975545655055304,-6.69631239376589,
14.2431348501518));
#186593=CARTESIAN_POINT('Ctrl Pts',(1.15292710631738,-6.67047075229361,
14.2515693653841));
#186594=CARTESIAN_POINT('Ctrl Pts',(1.32920857065779,-6.63758729532144,
14.2600038806164));
#186595=CARTESIAN_POINT('Ctrl Pts',(1.50381575322244,-6.59778956775374,
14.2684383958486));
#186596=CARTESIAN_POINT('Ctrl Pts',(1.67850727255218,-6.55797261754266,
14.276876985024));
#186597=CARTESIAN_POINT('Ctrl Pts',(1.85152257409379,-6.51123481817353,
14.2853155741994));
#186598=CARTESIAN_POINT('Ctrl Pts',(2.02230163697252,-6.45775387337566,
14.2937541633748));
#186599=CARTESIAN_POINT('Ctrl Pts',(2.19327159220824,-6.40421314898048,
14.3022021849838));
#186600=CARTESIAN_POINT('Ctrl Pts',(2.36199999830811,-6.34391432577537,
14.3106502065929));
#186601=CARTESIAN_POINT('Ctrl Pts',(2.52794480242968,-6.27708404244111,
14.3190982282019));
#186602=CARTESIAN_POINT('Ctrl Pts',(2.62226516868471,-6.23909878080919,
14.3238999482468));
#186603=CARTESIAN_POINT('Ctrl Pts',(2.71568665118124,-6.19900433459048,
14.3287016682916));
#186604=CARTESIAN_POINT('Ctrl Pts',(2.80811313774876,-6.15684899974027,
14.3335033883365));
#186605=CARTESIAN_POINT('Ctrl Pts',(2.96671275895864,-6.08451237430408,
14.341742920191));
#186606=CARTESIAN_POINT('Ctrl Pts',(3.12273526239712,-6.00594335354235,
14.3499824520455));
#186607=CARTESIAN_POINT('Ctrl Pts',(3.27565856692249,-5.92134697116689,
14.3582219839));
#186608=CARTESIAN_POINT('Ctrl Pts',(3.42841213726711,-5.83684448486372,
14.36645237045));
#186609=CARTESIAN_POINT('Ctrl Pts',(3.57807304941933,-5.74632812852416,
14.374682757));
#186610=CARTESIAN_POINT('Ctrl Pts',(3.72413943959445,-5.65005083467902,
14.38291314355));
#186611=CARTESIAN_POINT('Ctrl Pts',(3.87006976318593,-5.55386322691732,
14.3911358631714));
#186612=CARTESIAN_POINT('Ctrl Pts',(4.01241193785822,-5.45192556392291,
14.3993585827928));
#186613=CARTESIAN_POINT('Ctrl Pts',(4.15068887620276,-5.3445365423923,14.4075813024142));
#186614=CARTESIAN_POINT('Ctrl Pts',(4.28884329121644,-5.23724267527265,
14.4157967361136));
#186615=CARTESIAN_POINT('Ctrl Pts',(4.42293936919019,-5.12450729432345,
14.4240121698129));
#186616=CARTESIAN_POINT('Ctrl Pts',(4.55252930136011,-5.00667214427484,
14.4322276035123));
#186617=CARTESIAN_POINT('Ctrl Pts',(4.68205263436727,-4.88889755234371,
14.4404388151166));
#186618=CARTESIAN_POINT('Ctrl Pts',(4.8070741710293,-4.76602864988975,14.4486500267209));
#186619=CARTESIAN_POINT('Ctrl Pts',(4.92717916063223,-4.63844742548964,
14.4568612383253));
#186620=CARTESIAN_POINT('Ctrl Pts',(5.047243873648,-4.51090898479337,14.4650696963422));
#186621=CARTESIAN_POINT('Ctrl Pts',(5.1623950803399,-4.37866162901597,14.4732781543592));
#186622=CARTESIAN_POINT('Ctrl Pts',(5.2722548332316,-4.24212422890538,14.4814866123762));
#186623=CARTESIAN_POINT('Ctrl Pts',(5.32119975171067,-4.18129383613775,
14.4851436596379));
#186624=CARTESIAN_POINT('Ctrl Pts',(5.36909487682439,-4.11961238541116,
14.4888007068995));
#186625=CARTESIAN_POINT('Ctrl Pts',(5.41590930921471,-4.05711909541258,
14.4924577541612));
#186626=CARTESIAN_POINT('Ctrl Pts',(5.52931569949832,-3.90573119912038,
14.501316828337));
#186627=CARTESIAN_POINT('Ctrl Pts',(5.63625969591771,-3.74973455536902,
14.5101759025128));
#186628=CARTESIAN_POINT('Ctrl Pts',(5.73640989029452,-3.58969226682891,
14.5190349766885));
#186629=CARTESIAN_POINT('Ctrl Pts',(5.83674824673813,-3.42934929102628,
14.5279106952824));
#186630=CARTESIAN_POINT('Ctrl Pts',(5.93026715513365,-3.26494570012286,
14.5367864138762));
#186631=CARTESIAN_POINT('Ctrl Pts',(6.01668117519077,-3.09706903960906,
14.5456621324701));
#186632=CARTESIAN_POINT('Ctrl Pts',(6.10334179644595,-2.92871330653758,
14.5545631798571));
#186633=CARTESIAN_POINT('Ctrl Pts',(6.18285683619363,-2.75686490219078,
14.5634642272441));
#186634=CARTESIAN_POINT('Ctrl Pts',(6.2549878243912,-2.58213406249906,14.5723652746311));
#186635=CARTESIAN_POINT('Ctrl Pts',(6.32721687565693,-2.40716567383327,
14.5812784231142));
#186636=CARTESIAN_POINT('Ctrl Pts',(6.39204172953085,-2.22930726402084,
14.5901915715972));
#186637=CARTESIAN_POINT('Ctrl Pts',(6.44927345651298,-2.04918541940869,
14.5991047200803));
#186638=CARTESIAN_POINT('Ctrl Pts',(6.5066322535791,-1.86866365504693,14.6080376581903));
#186639=CARTESIAN_POINT('Ctrl Pts',(6.55636412420428,-1.68586865215733,
14.6169705963003));
#186640=CARTESIAN_POINT('Ctrl Pts',(6.59833033935322,-1.50144121855332,
14.6259035344103));
#186641=CARTESIAN_POINT('Ctrl Pts',(6.63827609132687,-1.32589304262804,
14.6344063962689));
#186642=CARTESIAN_POINT('Ctrl Pts',(6.67118630300886,-1.14886610272031,
14.6429092581274));
#186643=CARTESIAN_POINT('Ctrl Pts',(6.69698490228194,-0.970918234769417,
14.651412119986));
#186644=CARTESIAN_POINT('Ctrl Pts',(6.72193353269149,-0.798833093918143,
14.6596348438513));
#186645=CARTESIAN_POINT('Ctrl Pts',(6.7402782696263,-0.625556742266962,
14.6678575677165));
#186646=CARTESIAN_POINT('Ctrl Pts',(6.75191179983549,-0.451637074698601,
14.6760802915818));
#186647=CARTESIAN_POINT('Ctrl Pts',(6.76353301634702,-0.277901495206955,
14.6842943119723));
#186648=CARTESIAN_POINT('Ctrl Pts',(6.76845714790904,-0.103524310693517,
14.6925083323629));
#186649=CARTESIAN_POINT('Ctrl Pts',(6.7666281705844,0.0709380085259613,
14.7007223527535));
#186650=CARTESIAN_POINT('Ctrl Pts',(6.76480076196337,0.245250692391744,
14.7089293280248));
#186651=CARTESIAN_POINT('Ctrl Pts',(6.75623178366827,0.419648008867386,
14.7171363032961));
#186652=CARTESIAN_POINT('Ctrl Pts',(6.74091713069847,0.593569909156351,
14.7253432785674));
#186653=CARTESIAN_POINT('Ctrl Pts',(6.72561253915008,0.767377546227373,
14.7335448620197));
#186654=CARTESIAN_POINT('Ctrl Pts',(6.7035711318405,0.940710033193421,14.7417464454721));
#186655=CARTESIAN_POINT('Ctrl Pts',(6.67484085652982,1.11300877804275,14.7499480289244));
#186656=CARTESIAN_POINT('Ctrl Pts',(6.64612369103792,1.28522890181048,14.7581458699388));
#186657=CARTESIAN_POINT('Ctrl Pts',(6.61072379710433,1.45641587010172,14.7663437109531));
#186658=CARTESIAN_POINT('Ctrl Pts',(6.56874081204955,1.62601757189602,14.7745415519675));
#186659=CARTESIAN_POINT('Ctrl Pts',(6.52676153186233,1.79560430686884,14.782738669548));
#186660=CARTESIAN_POINT('Ctrl Pts',(6.47820039550589,1.96360570398415,14.7909357871284));
#186661=CARTESIAN_POINT('Ctrl Pts',(6.42320795310195,2.12948082668239,14.7991329047089));
#186662=CARTESIAN_POINT('Ctrl Pts',(6.36821612255023,2.29535410383497,14.8073299310873));
#186663=CARTESIAN_POINT('Ctrl Pts',(6.30679324037308,2.45910081274998,14.8155269574657));
#186664=CARTESIAN_POINT('Ctrl Pts',(6.23913940853569,2.62019625998834,14.823723983844));
#186665=CARTESIAN_POINT('Ctrl Pts',(6.17147402790334,2.78131920690025,14.8319224094895));
#186666=CARTESIAN_POINT('Ctrl Pts',(6.09757571745006,2.93978965960707,14.8401208351349));
#186667=CARTESIAN_POINT('Ctrl Pts',(6.01769231631652,3.09510390554908,14.8483192607803));
#186668=CARTESIAN_POINT('Ctrl Pts',(5.93778075336619,3.25047290543593,14.8565205766702));
#186669=CARTESIAN_POINT('Ctrl Pts',(5.8518800606913,3.40268316318726,14.8647218925602));
#186670=CARTESIAN_POINT('Ctrl Pts',(5.76028353595834,3.55125647980646,14.8729232084501));
#186671=CARTESIAN_POINT('Ctrl Pts',(5.66858269811658,3.69999899656273,14.881133864266));
#186672=CARTESIAN_POINT('Ctrl Pts',(5.5711732576536,3.84509599170721,14.8893445200818));
#186673=CARTESIAN_POINT('Ctrl Pts',(5.46839187287259,3.98609825828479,14.8975551758977));
#186674=CARTESIAN_POINT('Ctrl Pts',(5.36554992151172,4.12718361408185,14.9057706700541));
#186675=CARTESIAN_POINT('Ctrl Pts',(5.25732993785621,4.26416915041607,14.9139861642105));
#186676=CARTESIAN_POINT('Ctrl Pts',(5.14410813426136,4.39663968310187,14.9222016583669));
#186677=CARTESIAN_POINT('Ctrl Pts',(5.03071066495481,4.52931574625675,14.9304298990137));
#186678=CARTESIAN_POINT('Ctrl Pts',(4.91229611070893,4.65746254342381,14.9386581396604));
#186679=CARTESIAN_POINT('Ctrl Pts',(4.7892776596528,4.78070167431002,14.9468863803072));
#186680=CARTESIAN_POINT('Ctrl Pts',(4.67747352753613,4.8927063691607,14.9543645374166));
#186681=CARTESIAN_POINT('Ctrl Pts',(4.56186720603265,5.00065773557728,14.9618426945261));
#186682=CARTESIAN_POINT('Ctrl Pts',(4.44279111096107,5.10430172936175,14.9693208516355));
#186683=CARTESIAN_POINT('Ctrl Pts',(4.31429865585947,5.21614173561904,14.9773903702576));
#186684=CARTESIAN_POINT('Ctrl Pts',(4.18134476669475,5.32333164869652,14.9854598888797));
#186685=CARTESIAN_POINT('Ctrl Pts',(4.04430565237376,5.42548438300007,14.9935294075019));
#186686=CARTESIAN_POINT('Ctrl Pts',(3.90741731585645,5.52752472337146,15.0015900476056));
#186687=CARTESIAN_POINT('Ctrl Pts',(3.76645298746382,5.62453868532145,15.0096506877093));
#186688=CARTESIAN_POINT('Ctrl Pts',(3.62182548495932,5.71617609565164,15.0177113278131));
#186689=CARTESIAN_POINT('Ctrl Pts',(3.47736266831416,5.80770915939901,15.0257627893483));
#186690=CARTESIAN_POINT('Ctrl Pts',(3.32924529483506,5.89387766213528,15.0338142508835));
#186691=CARTESIAN_POINT('Ctrl Pts',(3.17791859704343,5.97437213358571,15.0418657124187));
#186692=CARTESIAN_POINT('Ctrl Pts',(3.15174294605904,5.98829561980201,15.0432584094783));
#186693=CARTESIAN_POINT('Ctrl Pts',(3.1254713474183,6.00204943887579,15.044651106538));
#186694=CARTESIAN_POINT('Ctrl Pts',(3.09910619832132,6.01563211736941,15.0460438035976));
#186695=CARTESIAN_POINT('Ctrl Pts',(3.09910619832134,6.0156321173694,13.0454981451509));
#186696=CARTESIAN_POINT('Ctrl Pts',(2.99647924970002,6.0685030054792,13.0509549173467));
#186697=CARTESIAN_POINT('Ctrl Pts',(2.89261356534081,6.11868781655653,13.0564116895426));
#186698=CARTESIAN_POINT('Ctrl Pts',(2.78766713702072,6.16613338593764,13.0618684617384));
#186699=CARTESIAN_POINT('Ctrl Pts',(2.62740565609552,6.2385865159209,13.0702013836603));
#186700=CARTESIAN_POINT('Ctrl Pts',(2.46411195497162,6.30488082417588,13.0785343055822));
#186701=CARTESIAN_POINT('Ctrl Pts',(2.29829356235286,6.3647573167598,13.0868672275041));
#186702=CARTESIAN_POINT('Ctrl Pts',(2.13267112688792,6.42456304984061,13.0951903019318));
#186703=CARTESIAN_POINT('Ctrl Pts',(1.96453026791125,6.47796595860846,13.1035133763595));
#186704=CARTESIAN_POINT('Ctrl Pts',(1.79440086093049,6.52475398389027,13.1118364507872));
#186705=CARTESIAN_POINT('Ctrl Pts',(1.62444127744431,6.57149530527709,13.1201512171063));
#186706=CARTESIAN_POINT('Ctrl Pts',(1.45249743406288,6.61163480676236,13.1284659834254));
#186707=CARTESIAN_POINT('Ctrl Pts',(1.27911705083958,6.64500929798081,13.1367807497445));
#186708=CARTESIAN_POINT('Ctrl Pts',(1.10587793243847,6.67835659672524,13.1450887414564));
#186709=CARTESIAN_POINT('Ctrl Pts',(0.931204946609093,6.70494980266404,
13.1533967331684));
#186710=CARTESIAN_POINT('Ctrl Pts',(0.755658991091057,6.72467608804939,
13.1617047248803));
#186711=CARTESIAN_POINT('Ctrl Pts',(0.580223881354881,6.74438991757655,
13.1700074706392));
#186712=CARTESIAN_POINT('Ctrl Pts',(0.403917245247942,6.75724542895902,
13.1783102163982));
#186713=CARTESIAN_POINT('Ctrl Pts',(0.227308369897301,6.7631811971124,13.1866129621571));
#186714=CARTESIAN_POINT('Ctrl Pts',(0.0507716689739177,6.76911453950622,
13.194912314848));
#186715=CARTESIAN_POINT('Ctrl Pts',(-0.126066677897103,6.76813376176002,
13.203211667539));
#186716=CARTESIAN_POINT('Ctrl Pts',(-0.3026337917841,6.7602294183016,13.2115110202299));
#186717=CARTESIAN_POINT('Ctrl Pts',(-0.47916335280551,6.75232675596454,
13.2198086077876));
#186718=CARTESIAN_POINT('Ctrl Pts',(-0.655421448412094,6.73750347707007,
13.2281061953454));
#186719=CARTESIAN_POINT('Ctrl Pts',(-0.830836484566319,6.71580224067933,
13.2364037829031));
#186720=CARTESIAN_POINT('Ctrl Pts',(-1.00624336252497,6.69410201356883,
13.244700984557));
#186721=CARTESIAN_POINT('Ctrl Pts',(-1.18080691393567,6.66552450927124,
13.2529981862108));
#186722=CARTESIAN_POINT('Ctrl Pts',(-1.35396174730041,6.63016414478912,
13.2612953878647));
#186723=CARTESIAN_POINT('Ctrl Pts',(-1.52713730035547,6.59479954908926,
13.2695935823609));
#186724=CARTESIAN_POINT('Ctrl Pts',(-1.69890345874809,6.55265054611699,
13.2778917768571));
#186725=CARTESIAN_POINT('Ctrl Pts',(-1.86870589449789,6.50386248931117,
13.2861899713533));
#186726=CARTESIAN_POINT('Ctrl Pts',(-2.03862775430338,6.4550401192896,13.2944940020675));
#186727=CARTESIAN_POINT('Ctrl Pts',(-2.20658279695294,6.39956946139631,
13.3027980327818));
#186728=CARTESIAN_POINT('Ctrl Pts',(-2.3720318454969,6.33764577141612,13.311102063496));
#186729=CARTESIAN_POINT('Ctrl Pts',(-2.53754105587863,6.27569956427416,
13.3194091137849));
#186730=CARTESIAN_POINT('Ctrl Pts',(-2.70054213272634,6.20729577702732,
13.3277161640738));
#186731=CARTESIAN_POINT('Ctrl Pts',(-2.8605165032443,6.13267758280729,13.3360232143626));
#186732=CARTESIAN_POINT('Ctrl Pts',(-3.02066191340138,6.05797960912652,
13.3443391462922));
#186733=CARTESIAN_POINT('Ctrl Pts',(-3.17777383920727,5.97705410703056,
13.3526550782218));
#186734=CARTESIAN_POINT('Ctrl Pts',(-3.33135793194182,5.89019043234498,
13.3609710101514));
#186735=CARTESIAN_POINT('Ctrl Pts',(-3.4471329132116,5.8247107323924,13.3672397378969));
#186736=CARTESIAN_POINT('Ctrl Pts',(-3.5609037198362,5.7558576388238,13.3735084656424));
#186737=CARTESIAN_POINT('Ctrl Pts',(-3.67246982934681,5.68377113829695,
13.3797771933879));
#186738=CARTESIAN_POINT('Ctrl Pts',(-3.82286136738246,5.58659826265044,
13.3882274621237));
#186739=CARTESIAN_POINT('Ctrl Pts',(-3.96952145393238,5.48337026741117,
13.3966777308594));
#186740=CARTESIAN_POINT('Ctrl Pts',(-4.11195058525543,5.3743977694638,13.4051279995952));
#186741=CARTESIAN_POINT('Ctrl Pts',(-4.25425401802717,5.2655214434512,13.4135708106815));
#186742=CARTESIAN_POINT('Ctrl Pts',(-4.39233367591338,5.15091092014112,
13.4220136217678));
#186743=CARTESIAN_POINT('Ctrl Pts',(-4.52571894571774,5.03092009719609,
13.4304564328541));
#186744=CARTESIAN_POINT('Ctrl Pts',(-4.65900465923298,4.9110188331737,13.4388929423829));
#186745=CARTESIAN_POINT('Ctrl Pts',(-4.78760272359501,4.7857454957332,13.4473294519118));
#186746=CARTESIAN_POINT('Ctrl Pts',(-4.91107524620995,4.65549448781371,
13.4557659614406));
#186747=CARTESIAN_POINT('Ctrl Pts',(-5.03445941757595,4.52533668151498,
13.4641964341919));
#186748=CARTESIAN_POINT('Ctrl Pts',(-5.15272513525066,4.39020854936282,
13.4726269069431));
#186749=CARTESIAN_POINT('Ctrl Pts',(-5.26547090893323,4.25054174278737,
13.4810573796944));
#186750=CARTESIAN_POINT('Ctrl Pts',(-5.37816821350532,4.11093497860337,
13.4894842282077));
#186751=CARTESIAN_POINT('Ctrl Pts',(-5.48535009686753,3.96679368724348,
13.497911076721));
#186752=CARTESIAN_POINT('Ctrl Pts',(-5.58665453466185,3.81858352145691,
13.5063379252343));
#186753=CARTESIAN_POINT('Ctrl Pts',(-5.68792770338291,3.67041910287187,
13.5147621726795));
#186754=CARTESIAN_POINT('Ctrl Pts',(-5.78332685750545,3.51818858788166,
13.5231864201247));
#186755=CARTESIAN_POINT('Ctrl Pts',(-5.87253238503921,3.3623878994943,13.5316106675698));
#186756=CARTESIAN_POINT('Ctrl Pts',(-5.89766708894574,3.31848922774924,
13.5339842981174));
#186757=CARTESIAN_POINT('Ctrl Pts',(-5.92231034895509,3.27430729443035,
13.536357928665));
#186758=CARTESIAN_POINT('Ctrl Pts',(-5.94645565075077,3.22985358703058,
13.5387315592127));
#186759=CARTESIAN_POINT('Ctrl Pts',(-6.03409394712244,3.06850347358454,
13.5473469386835));
#186760=CARTESIAN_POINT('Ctrl Pts',(-6.11512962430521,2.90364278619995,
13.5559623181544));
#186761=CARTESIAN_POINT('Ctrl Pts',(-6.18930641017625,2.73583171283455,
13.5645776976252));
#186762=CARTESIAN_POINT('Ctrl Pts',(-6.26352739573469,2.56792064596175,
13.5731982107383));
#186763=CARTESIAN_POINT('Ctrl Pts',(-6.3308812104885,2.39705596330387,13.5818187238514));
#186764=CARTESIAN_POINT('Ctrl Pts',(-6.39115998598896,2.22381722124226,
13.5904392369645));
#186765=CARTESIAN_POINT('Ctrl Pts',(-6.45335842450229,2.04506144598328,
13.5993342825318));
#186766=CARTESIAN_POINT('Ctrl Pts',(-6.50802365181356,1.86377824369163,
13.6082293280991));
#186767=CARTESIAN_POINT('Ctrl Pts',(-6.5549832821678,1.68061987686112,13.6171243736664));
#186768=CARTESIAN_POINT('Ctrl Pts',(-6.60057818246509,1.50278441667421,
13.62576091345));
#186769=CARTESIAN_POINT('Ctrl Pts',(-6.63890906905846,1.32318156436215,
13.6343974532337));
#186770=CARTESIAN_POINT('Ctrl Pts',(-6.66987032856565,1.142417962096,13.6430339930174));
#186771=CARTESIAN_POINT('Ctrl Pts',(-6.70222166989695,0.953538533730723,
13.6520582914765));
#186772=CARTESIAN_POINT('Ctrl Pts',(-6.72652632290179,0.763392101546304,
13.6610825899356));
#186773=CARTESIAN_POINT('Ctrl Pts',(-6.74272428641475,0.572676346108998,
13.6701068883947));
#186774=CARTESIAN_POINT('Ctrl Pts',(-6.7589222499277,0.381960590671692,
13.6791311868538));
#186775=CARTESIAN_POINT('Ctrl Pts',(-6.76701354094034,0.190675889789615,
13.6881554853129));
#186776=CARTESIAN_POINT('Ctrl Pts',(-6.76699998297921,-0.000479957709508635,
13.6971797837721));
#186777=CARTESIAN_POINT('',(-6.76699751798627,-0.00579582329898324,13.3028202162226));
#186778=CARTESIAN_POINT('Ctrl Pts',(3.09910619832131,6.01563211736941,12.6513039064363));
#186779=CARTESIAN_POINT('Ctrl Pts',(2.93978775740063,6.09770907256395,12.6597306285985));
#186780=CARTESIAN_POINT('Ctrl Pts',(2.7772501800563,6.1734306902204,12.6681573507607));
#186781=CARTESIAN_POINT('Ctrl Pts',(2.61203227770273,6.2425616841357,12.676584072923));
#186782=CARTESIAN_POINT('Ctrl Pts',(2.44666622100594,6.31175466925688,12.685018351503));
#186783=CARTESIAN_POINT('Ctrl Pts',(2.27861534458493,6.37434509232258,12.6934526300829));
#186784=CARTESIAN_POINT('Ctrl Pts',(2.10843755082295,6.43014619540487,12.7018869086629));
#186785=CARTESIAN_POINT('Ctrl Pts',(1.93817900638068,6.48597377654246,12.7103251893734));
#186786=CARTESIAN_POINT('Ctrl Pts',(1.76579185105679,6.53500551641699,12.7187634700838));
#186787=CARTESIAN_POINT('Ctrl Pts',(1.59184762273827,6.57710499733603,12.7272017507942));
#186788=CARTESIAN_POINT('Ctrl Pts',(1.41770634921698,6.61925216883287,12.7356495904464));
#186789=CARTESIAN_POINT('Ctrl Pts',(1.24200480411557,6.65445131830971,12.7440974300985));
#186790=CARTESIAN_POINT('Ctrl Pts',(1.06532440572475,6.68261722011423,12.7525452697506));
#186791=CARTESIAN_POINT('Ctrl Pts',(0.953184147250487,6.70049431082314,
12.7579071714147));
#186792=CARTESIAN_POINT('Ctrl Pts',(0.840649698346499,6.71553907890543,
12.7632690730787));
#186793=CARTESIAN_POINT('Ctrl Pts',(0.727870451699451,6.7277406018323,12.7686309747428));
#186794=CARTESIAN_POINT('Ctrl Pts',(0.554564637076018,6.74649045992548,
12.7768705113902));
#186795=CARTESIAN_POINT('Ctrl Pts',(0.380293753517344,6.75856551206301,
12.7851100480377));
#186796=CARTESIAN_POINT('Ctrl Pts',(0.20561140489293,6.76387558653898,12.7933495846851));
#186797=CARTESIAN_POINT('Ctrl Pts',(0.0311229417577409,6.76917976719455,
12.8015799760091));
#186798=CARTESIAN_POINT('Ctrl Pts',(-0.143775724472965,6.76773391047996,
12.809810367333));
#186799=CARTESIAN_POINT('Ctrl Pts',(-0.318523926401962,6.7594993533774,
12.8180407586569));
#186800=CARTESIAN_POINT('Ctrl Pts',(-0.493109343101404,6.75127246710781,
12.8262634830284));
#186801=CARTESIAN_POINT('Ctrl Pts',(-0.667544221215973,6.73626949137306,
12.8344862074));
#186802=CARTESIAN_POINT('Ctrl Pts',(-0.841265839795262,6.71450376325709,
12.8427089317715));
#186803=CARTESIAN_POINT('Ctrl Pts',(-1.01483352756912,6.69275732126156,
12.8509243701726));
#186804=CARTESIAN_POINT('Ctrl Pts',(-1.18768886365077,6.66426011422477,
12.8591398085737));
#186805=CARTESIAN_POINT('Ctrl Pts',(-1.35927233151704,6.62907744175404,
12.8673552469747));
#186806=CARTESIAN_POINT('Ctrl Pts',(-1.53076761825765,6.5939128505571,12.8755664632522));
#186807=CARTESIAN_POINT('Ctrl Pts',(-1.70099199077603,6.55206970800288,
12.8837776795297));
#186808=CARTESIAN_POINT('Ctrl Pts',(-1.86939381828759,6.50366479395642,
12.8919888958072));
#186809=CARTESIAN_POINT('Ctrl Pts',(-2.0377391719983,6.45527611256917,12.9001973584412));
#186810=CARTESIAN_POINT('Ctrl Pts',(-2.20426285656253,6.40033014149029,
12.9084058210752));
#186811=CARTESIAN_POINT('Ctrl Pts',(-2.36842606338852,6.3389941617154,12.9166142837092));
#186812=CARTESIAN_POINT('Ctrl Pts',(-2.44156374890655,6.31166787048091,
12.920271302662));
#186813=CARTESIAN_POINT('Ctrl Pts',(-2.51423310581203,6.2830739131063,12.9239283216148));
#186814=CARTESIAN_POINT('Ctrl Pts',(-2.58638754591579,6.25323024222935,
12.9275853405676));
#186815=CARTESIAN_POINT('Ctrl Pts',(-2.76118055184715,6.18093441493019,
12.9364444119509));
#186816=CARTESIAN_POINT('Ctrl Pts',(-2.93276884545542,6.10137685054242,
12.9453034833343));
#186817=CARTESIAN_POINT('Ctrl Pts',(-3.10058001914121,6.01487261252492,
12.9541625547176));
#186818=CARTESIAN_POINT('Ctrl Pts',(-3.26870647417205,5.9282058515245,12.9630382704035));
#186819=CARTESIAN_POINT('Ctrl Pts',(-3.43304139711229,5.83456645337312,
12.9719139860894));
#186820=CARTESIAN_POINT('Ctrl Pts',(-3.59303943281136,5.73431396369806,
12.9807897017753));
#186821=CARTESIAN_POINT('Ctrl Pts',(-3.75349405552794,5.63377538310285,
12.9896907461256));
#186822=CARTESIAN_POINT('Ctrl Pts',(-3.90958680346882,5.52658608439311,
12.9985917904759));
#186823=CARTESIAN_POINT('Ctrl Pts',(-4.06080113035424,5.41314910008155,
13.0074928348262));
#186824=CARTESIAN_POINT('Ctrl Pts',(-4.21222103428513,5.29955789731357,
13.016405980215));
#186825=CARTESIAN_POINT('Ctrl Pts',(-4.35874906540356,5.17970220284822,
13.0253191256039));
#186826=CARTESIAN_POINT('Ctrl Pts',(-4.49990293266634,5.05402439612047,
13.0342322709927));
#186827=CARTESIAN_POINT('Ctrl Pts',(-4.64137019955671,4.92806755079045,
13.0431652059665));
#186828=CARTESIAN_POINT('Ctrl Pts',(-4.77743924181069,4.79626291060941,
13.0520981409403));
#186829=CARTESIAN_POINT('Ctrl Pts',(-4.90766367778078,4.659090708045,13.061031075914));
#186830=CARTESIAN_POINT('Ctrl Pts',(-5.0316187207818,4.52852238466734,13.0695339527401));
#186831=CARTESIAN_POINT('Ctrl Pts',(-5.15027854017729,4.39309129018316,
13.0780368295662));
#186832=CARTESIAN_POINT('Ctrl Pts',(-5.2632929832141,4.25323829250716,13.0865397063923));
#186833=CARTESIAN_POINT('Ctrl Pts',(-5.37091165595206,4.12006244715601,
13.0946366212104));
#186834=CARTESIAN_POINT('Ctrl Pts',(-5.47364117613993,3.98259047815141,
13.1027335360284));
#186835=CARTESIAN_POINT('Ctrl Pts',(-5.57111288479381,3.84122249093754,
13.1108304508465));
#186836=CARTESIAN_POINT('Ctrl Pts',(-5.66844891615202,3.70005128314268,
13.1189160950351));
#186837=CARTESIAN_POINT('Ctrl Pts',(-5.76054150709384,3.55499516330702,
13.1270017392237));
#186838=CARTESIAN_POINT('Ctrl Pts',(-5.84706149027389,3.40648806382116,
13.1350873834124));
#186839=CARTESIAN_POINT('Ctrl Pts',(-5.93351204297753,3.25810013817573,
13.1431665390407));
#186840=CARTESIAN_POINT('Ctrl Pts',(-6.01439870058324,3.10626706157592,
13.1512456946691));
#186841=CARTESIAN_POINT('Ctrl Pts',(-6.08943463889467,2.95145299448082,
13.1593248502974));
#186842=CARTESIAN_POINT('Ctrl Pts',(-6.1644250602964,2.79673283782478,13.1673991050981));
#186843=CARTESIAN_POINT('Ctrl Pts',(-6.2335716645703,2.63903562198289,13.1754733598989));
#186844=CARTESIAN_POINT('Ctrl Pts',(-6.29663282907075,2.47885135009514,
13.1835476146996));
#186845=CARTESIAN_POINT('Ctrl Pts',(-6.35966808884399,2.31873287987628,
13.1916185526988));
#186846=CARTESIAN_POINT('Ctrl Pts',(-6.41662274988487,2.15612973203305,
13.199689490698));
#186847=CARTESIAN_POINT('Ctrl Pts',(-6.46730278219813,1.99155309328482,
13.2077604286972));
#186848=CARTESIAN_POINT('Ctrl Pts',(-6.51798247269528,1.82697756453877,
13.2158313122612));
#186849=CARTESIAN_POINT('Ctrl Pts',(-6.56238749793609,1.66042892221144,
13.2239021958253));
#186850=CARTESIAN_POINT('Ctrl Pts',(-6.60037323290307,1.49243498564484,
13.2319730793893));
#186851=CARTESIAN_POINT('Ctrl Pts',(-6.63835735458364,1.32444818392333,
13.240043620176));
#186852=CARTESIAN_POINT('Ctrl Pts',(-6.66992265171161,1.1550165732352,13.2481141609628));
#186853=CARTESIAN_POINT('Ctrl Pts',(-6.69497542089426,0.984679193251125,
13.2561847017495));
#186854=CARTESIAN_POINT('Ctrl Pts',(-6.72004235822306,0.81424548200425,
13.2642598066864));
#186855=CARTESIAN_POINT('Ctrl Pts',(-6.73858935704497,0.642905345832317,
13.2723349116234));
#186856=CARTESIAN_POINT('Ctrl Pts',(-6.75057444037095,0.471204546890744,
13.2804100165603));
#186857=CARTESIAN_POINT('Ctrl Pts',(-6.76166152477046,0.312368667526999,
13.2878800831035));
#186858=CARTESIAN_POINT('Ctrl Pts',(-6.76713371623367,0.153224434099281,
13.2953501496467));
#186859=CARTESIAN_POINT('Ctrl Pts',(-6.76699751798686,-0.00579582260286099,
13.3028202161899));
#186860=CARTESIAN_POINT('Ctrl Pts',(-6.76699751798627,-0.00579582329897739,
13.3028202162226));
#186861=CARTESIAN_POINT('Ctrl Pts',(-6.76681198988727,-0.222411844982174,
13.3129958764175));
#186862=CARTESIAN_POINT('Ctrl Pts',(-6.75622188990783,-0.438543524588682,
13.3231715366123));
#186863=CARTESIAN_POINT('Ctrl Pts',(-6.7353881739906,-0.653326216883703,
13.3333471968072));
#186864=CARTESIAN_POINT('Ctrl Pts',(-6.71431012283039,-0.870627854023666,
13.343642195886));
#186865=CARTESIAN_POINT('Ctrl Pts',(-6.68274685485897,-1.08654879994134,
13.3539371949648));
#186866=CARTESIAN_POINT('Ctrl Pts',(-6.64091266108794,-1.30021845387683,
13.3642321940437));
#186867=CARTESIAN_POINT('Ctrl Pts',(-6.5985826378675,-1.51642057461325,
13.3746492120564));
#186868=CARTESIAN_POINT('Ctrl Pts',(-6.54573678032153,-1.73031785842102,
13.3850662300692));
#186869=CARTESIAN_POINT('Ctrl Pts',(-6.48264491585991,-1.9410316573605,
13.3954832480819));
#186870=CARTESIAN_POINT('Ctrl Pts',(-6.46454534874988,-2.00148047397829,
13.3984716447352));
#186871=CARTESIAN_POINT('Ctrl Pts',(-6.44560285358692,-2.06166743370604,
13.4014600413885));
#186872=CARTESIAN_POINT('Ctrl Pts',(-6.42582451980347,-2.12157211536458,
13.4044484380418));
#186873=CARTESIAN_POINT('Ctrl Pts',(-6.37241879311197,-2.28332755397866,
13.4125177474518));
#186874=CARTESIAN_POINT('Ctrl Pts',(-6.3128033732122,-2.44336160887837,
13.4205870568618));
#186875=CARTESIAN_POINT('Ctrl Pts',(-6.247104180371,-2.6011494304617,13.4286563662718));
#186876=CARTESIAN_POINT('Ctrl Pts',(-6.1814869322611,-2.75874044779092,
13.436715611062));
#186877=CARTESIAN_POINT('Ctrl Pts',(-6.10980115115273,-2.91409046625502,
13.4447748558523));
#186878=CARTESIAN_POINT('Ctrl Pts',(-6.03222299244041,-3.06668791523907,
13.4528341006425));
#186879=CARTESIAN_POINT('Ctrl Pts',(-5.95472457035731,-3.21912852102893,
13.4608850619542));
#186880=CARTESIAN_POINT('Ctrl Pts',(-5.87134599053485,-3.36882185760112,
13.468936023266));
#186881=CARTESIAN_POINT('Ctrl Pts',(-5.78231210247125,-3.51527463359758,
13.4769869845777));
#186882=CARTESIAN_POINT('Ctrl Pts',(-5.69335021641091,-3.6616089727439,
13.48503143505));
#186883=CARTESIAN_POINT('Ctrl Pts',(-5.59874231767048,-3.8047076500584,
13.4930758855224));
#186884=CARTESIAN_POINT('Ctrl Pts',(-5.49875990269619,-3.94410047190745,
13.5011203359947));
#186885=CARTESIAN_POINT('Ctrl Pts',(-5.398836458621,-4.08341107809853,13.5091600417479));
#186886=CARTESIAN_POINT('Ctrl Pts',(-5.29354502568335,-4.2190198775832,
13.5171997475012));
#186887=CARTESIAN_POINT('Ctrl Pts',(-5.18320121548749,-4.35048435921439,
13.5252394532544));
#186888=CARTESIAN_POINT('Ctrl Pts',(-5.07047569751661,-4.48478642618439,
13.5334526914393));
#186889=CARTESIAN_POINT('Ctrl Pts',(-4.95247742482353,-4.61476289528958,
13.5416659296241));
#186890=CARTESIAN_POINT('Ctrl Pts',(-4.82958762202021,-4.73997599163004,
13.549879167809));
#186891=CARTESIAN_POINT('Ctrl Pts',(-4.70933300468522,-4.86250408299535,
13.5579162855557));
#186892=CARTESIAN_POINT('Ctrl Pts',(-4.58439479463962,-4.98047074881998,
13.5659534033025));
#186893=CARTESIAN_POINT('Ctrl Pts',(-4.45516846992223,-5.09350202754557,
13.5739905210492));
#186894=CARTESIAN_POINT('Ctrl Pts',(-4.32592847386177,-5.20654526427888,
13.5820284890731));
#186895=CARTESIAN_POINT('Ctrl Pts',(-4.1923997409979,-5.31465182818817,
13.590066457097));
#186896=CARTESIAN_POINT('Ctrl Pts',(-4.05501163878879,-5.41748738893663,
13.5981044251209));
#186897=CARTESIAN_POINT('Ctrl Pts',(-3.91758178012598,-5.5203542045628,
13.6061448361296));
#186898=CARTESIAN_POINT('Ctrl Pts',(-3.77629051625435,-5.61794660447148,
13.6141852471383));
#186899=CARTESIAN_POINT('Ctrl Pts',(-3.63159691743829,-5.70997310232305,
13.6222256581469));
#186900=CARTESIAN_POINT('Ctrl Pts',(-3.48143472688355,-5.80547767626098,
13.6305699507756));
#186901=CARTESIAN_POINT('Ctrl Pts',(-3.32760837488391,-5.89498717056716,
13.6389142434043));
#186902=CARTESIAN_POINT('Ctrl Pts',(-3.17065877865388,-5.97822815802016,
13.647258536033));
#186903=CARTESIAN_POINT('Ctrl Pts',(-3.01915787748253,-6.0585793339164,
13.655313146451));
#186904=CARTESIAN_POINT('Ctrl Pts',(-2.86474731244965,-6.13308984738742,
13.6633677568689));
#186905=CARTESIAN_POINT('Ctrl Pts',(-2.70793328800325,-6.20156321484543,
13.6714223672869));
#186906=CARTESIAN_POINT('Ctrl Pts',(-2.55100055311482,-6.27008841761438,
13.6794830751592));
#186907=CARTESIAN_POINT('Ctrl Pts',(-2.3916610814457,-6.33256723913197,
13.6875437830316));
#186908=CARTESIAN_POINT('Ctrl Pts',(-2.230436169122,-6.38885306572881,13.6956044909039));
#186909=CARTESIAN_POINT('Ctrl Pts',(-2.0689839393402,-6.44521825196582,
13.7036765638909));
#186910=CARTESIAN_POINT('Ctrl Pts',(-1.90564131873512,-6.49537291335649,
13.711748636878));
#186911=CARTESIAN_POINT('Ctrl Pts',(-1.74094027670692,-6.53922135677786,
13.7198207098651));
#186912=CARTESIAN_POINT('Ctrl Pts',(-1.72368912874173,-6.54381413880395,
13.7206661964738));
#186913=CARTESIAN_POINT('Ctrl Pts',(-1.70642308228228,-6.54833778267619,
13.7215116830826));
#186914=CARTESIAN_POINT('Ctrl Pts',(-1.68914275140194,-6.55279221136962,
13.7223571696914));
#186915=CARTESIAN_POINT('Ctrl Pts',(-1.51883177720467,-6.596694037991,13.7306900916133));
#186916=CARTESIAN_POINT('Ctrl Pts',(-1.34658947508686,-6.63400834483046,
13.7390230135352));
#186917=CARTESIAN_POINT('Ctrl Pts',(-1.17296026482133,-6.6645669939727,
13.7473559354571));
#186918=CARTESIAN_POINT('Ctrl Pts',(-0.999536242203163,-6.69508953019757,
13.7556790098848));
#186919=CARTESIAN_POINT('Ctrl Pts',(-0.824728916187795,-6.71887225278418,
13.7640020843125));
#186920=CARTESIAN_POINT('Ctrl Pts',(-0.649096675008562,-6.73579709511004,
13.7723251587402));
#186921=CARTESIAN_POINT('Ctrl Pts',(-0.473639750263407,-6.7527050430264,
13.7806399250593));
#186922=CARTESIAN_POINT('Ctrl Pts',(-0.297359895085378,-6.76276871604712,
13.7889546913784));
#186923=CARTESIAN_POINT('Ctrl Pts',(-0.120824698974208,-6.7659212522847,
13.7972694576975));
#186924=CARTESIAN_POINT('Ctrl Pts',(0.055566661873148,-6.76907121993602,
13.8055774494094));
#186925=CARTESIAN_POINT('Ctrl Pts',(0.232212602718064,-6.7653212648013,
13.8138854411213));
#186926=CARTESIAN_POINT('Ctrl Pts',(0.408541186671082,-6.75465640123859,
13.8221934328333));
#186927=CARTESIAN_POINT('Ctrl Pts',(0.584758430663995,-6.7439982718392,
13.8304961785922));
#186928=CARTESIAN_POINT('Ctrl Pts',(0.760658370785872,-6.7264339564995,
13.8387989243511));
#186929=CARTESIAN_POINT('Ctrl Pts',(0.935669618472968,-6.7020005494678,
13.84710167011));
#186930=CARTESIAN_POINT('Ctrl Pts',(1.11060934463241,-6.67757712759202,
13.855401022801));
#186931=CARTESIAN_POINT('Ctrl Pts',(1.28466075797919,-6.64629025556816,
13.8637003754919));
#186932=CARTESIAN_POINT('Ctrl Pts',(1.45725784371774,-6.6082288532498,13.8719997281828));
#186933=CARTESIAN_POINT('Ctrl Pts',(1.62981822094923,-6.57017554595373,
13.8802973157406));
#186934=CARTESIAN_POINT('Ctrl Pts',(1.80092454724439,-6.5253506536969,13.8885949032983));
#186935=CARTESIAN_POINT('Ctrl Pts',(1.97002100750952,-6.47389420905001,
13.896892490856));
#186936=CARTESIAN_POINT('Ctrl Pts',(2.13910960344286,-6.4224401575375,13.9051896925099));
#186937=CARTESIAN_POINT('Ctrl Pts',(2.30618818685144,-6.36435526966563,
13.9134868941637));
#186938=CARTESIAN_POINT('Ctrl Pts',(2.47071592772062,-6.29982950598726,
13.9217840958176));
#186939=CARTESIAN_POINT('Ctrl Pts',(2.63526335596345,-6.23529602116221,
13.9300822903138));
#186940=CARTESIAN_POINT('Ctrl Pts',(2.79725900980732,-6.16432025236565,
13.93838048481));
#186941=CARTESIAN_POINT('Ctrl Pts',(2.95618169245446,-6.08714044533204,
13.9466786793062));
#186942=CARTESIAN_POINT('Ctrl Pts',(3.11521614729845,-6.00990635682997,
13.9549827100204));
#186943=CARTESIAN_POINT('Ctrl Pts',(3.27117299899495,-5.92645966338178,
13.9632867407347));
#186944=CARTESIAN_POINT('Ctrl Pts',(3.42355453364015,-5.83708517628379,
13.9715907714489));
#186945=CARTESIAN_POINT('Ctrl Pts',(3.57599147841468,-5.74767819015697,
13.9798978217378));
#186946=CARTESIAN_POINT('Ctrl Pts',(3.72485021859095,-5.65233929653858,
13.9882048720267));
#186947=CARTESIAN_POINT('Ctrl Pts',(3.86966155518096,-5.55139698169339,
13.9965119223155));
#186948=CARTESIAN_POINT('Ctrl Pts',(4.01462771956415,-5.45034674245351,
14.0048278542451));
#186949=CARTESIAN_POINT('Ctrl Pts',(4.15553755291809,-5.34368131701438,
14.0131437861747));
#186950=CARTESIAN_POINT('Ctrl Pts',(4.29195364006265,-5.23177053697436,
14.0214597181043));
#186951=CARTESIAN_POINT('Ctrl Pts',(4.3947870107126,-5.14740979210572,14.0277284458498));
#186952=CARTESIAN_POINT('Ctrl Pts',(4.49506748575086,-5.06006924447631,
14.0339971735954));
#186953=CARTESIAN_POINT('Ctrl Pts',(4.59262151425816,-4.96992118919134,
14.0402659013409));
#186954=CARTESIAN_POINT('Ctrl Pts',(4.72412471404781,-4.84840126934609,
14.0487161700766));
#186955=CARTESIAN_POINT('Ctrl Pts',(4.85091351288786,-4.7215556920617,14.0571664388124));
#186956=CARTESIAN_POINT('Ctrl Pts',(4.97254906232811,-4.58977611902147,
14.0656167075482));
#186957=CARTESIAN_POINT('Ctrl Pts',(5.09407726426018,-4.45811284593517,
14.0740595186345));
#186958=CARTESIAN_POINT('Ctrl Pts',(5.2104610577621,-4.32152449875464,14.0825023297208));
#186959=CARTESIAN_POINT('Ctrl Pts',(5.32129747799463,-4.18044042544419,
14.090945140807));
#186960=CARTESIAN_POINT('Ctrl Pts',(5.43205117198079,-4.03946165466683,
14.0993816503359));
#186961=CARTESIAN_POINT('Ctrl Pts',(5.53726554229373,-3.89399410670221,
14.1078181598647));
#186962=CARTESIAN_POINT('Ctrl Pts',(5.63657680515809,-3.74450142469646,
14.1162546693936));
#186963=CARTESIAN_POINT('Ctrl Pts',(5.73581700545794,-3.59511571276694,
14.1246851421449));
#186964=CARTESIAN_POINT('Ctrl Pts',(5.82916234070514,-3.44171088734183,
14.1331156148961));
#186965=CARTESIAN_POINT('Ctrl Pts',(5.91629127695028,-3.28478104693175,
14.1415460876474));
#186966=CARTESIAN_POINT('Ctrl Pts',(6.00338275669556,-3.1279186702461,14.1499729361607));
#186967=CARTESIAN_POINT('Ctrl Pts',(6.08426300432896,-2.9675345889329,14.158399784674));
#186968=CARTESIAN_POINT('Ctrl Pts',(6.15865519724923,-2.80414963249023,
14.1668266331873));
#186969=CARTESIAN_POINT('Ctrl Pts',(6.2330244279481,-2.64081510716667,14.1752508806325));
#186970=CARTESIAN_POINT('Ctrl Pts',(6.30090946041277,-2.47448185532352,
14.1836751280776));
#186971=CARTESIAN_POINT('Ctrl Pts',(6.3620804464561,-2.3056932564461,14.1920993755228));
#186972=CARTESIAN_POINT('Ctrl Pts',(6.37931608940755,-2.25813508855148,
14.1944730060704));
#186973=CARTESIAN_POINT('Ctrl Pts',(6.39601899827916,-2.21038211659263,
14.196846636618));
#186974=CARTESIAN_POINT('Ctrl Pts',(6.41218472486389,-2.16244677488769,
14.1992202671656));
#186975=CARTESIAN_POINT('Ctrl Pts',(6.47088335321927,-1.98839095419338,
14.2078390481797));
#186976=CARTESIAN_POINT('Ctrl Pts',(6.52246944331495,-1.81200728260076,
14.2164578291937));
#186977=CARTESIAN_POINT('Ctrl Pts',(6.56678655545798,-1.6338920818268,14.2250766102078));
#186978=CARTESIAN_POINT('Ctrl Pts',(6.6111302886318,-1.45566988829057,14.2337005684733));
#186979=CARTESIAN_POINT('Ctrl Pts',(6.64819625633659,-1.27571438498409,
14.2423245267389));
#186980=CARTESIAN_POINT('Ctrl Pts',(6.67787902854769,-1.09463266901869,
14.2509484850044));
#186981=CARTESIAN_POINT('Ctrl Pts',(6.70863413762619,-0.907009091037845,
14.2598839973366));
#186982=CARTESIAN_POINT('Ctrl Pts',(6.73146259370863,-0.718176768294806,
14.2688195096687));
#186983=CARTESIAN_POINT('Ctrl Pts',(6.7463057891222,-0.528816792146654,
14.2777550220009));
#186984=CARTESIAN_POINT('Ctrl Pts',(6.76065823142376,-0.345717529746228,
14.2863951039785));
#186985=CARTESIAN_POINT('Ctrl Pts',(6.76754502205472,-0.16212525272967,
14.295035185956));
#186986=CARTESIAN_POINT('Ctrl Pts',(6.76696633971174,0.0213437861759871,
14.3036752679336));
#186987=CARTESIAN_POINT('Ctrl Pts',(6.76635797703756,0.214222861357321,
14.3127584954431));
#186988=CARTESIAN_POINT('Ctrl Pts',(6.7574982435815,0.406965331762482,14.3218417229525));
#186989=CARTESIAN_POINT('Ctrl Pts',(6.74044920709308,0.598860156128475,
14.330924950462));
#186990=CARTESIAN_POINT('Ctrl Pts',(6.72340017060467,0.790754980494468,
14.3400081779715));
#186991=CARTESIAN_POINT('Ctrl Pts',(6.69816191523472,0.981801778793228,
14.3490914054809));
#186992=CARTESIAN_POINT('Ctrl Pts',(6.66485893493886,1.17130029341997,14.3581746329904));
#186993=CARTESIAN_POINT('Ctrl Pts',(6.63169759884853,1.35999283313652,14.3672192277249));
#186994=CARTESIAN_POINT('Ctrl Pts',(6.59051023319254,1.54732463590756,14.3762638224594));
#186995=CARTESIAN_POINT('Ctrl Pts',(6.5414264608003,1.73263638941978,14.3853084171939));
#186996=CARTESIAN_POINT('Ctrl Pts',(6.49238773050414,1.91777809019567,14.3943447120874));
#186997=CARTESIAN_POINT('Ctrl Pts',(6.43546712139934,2.10090321289551,14.4033810069809));
#186998=CARTESIAN_POINT('Ctrl Pts',(6.37084485522845,2.28136468601783,14.4124173018744));
#186999=CARTESIAN_POINT('Ctrl Pts',(6.3063369432251,2.46150681841201,14.4214376063355));
#187000=CARTESIAN_POINT('Ctrl Pts',(6.23415466900139,2.63899448988547,14.4304579107966));
#187001=CARTESIAN_POINT('Ctrl Pts',(6.15452730999182,2.81319792950388,14.4394782152577));
#187002=CARTESIAN_POINT('Ctrl Pts',(6.07500022616442,2.98718199374854,14.4484871603985));
#187003=CARTESIAN_POINT('Ctrl Pts',(5.98804686670153,3.15788986416072,14.4574961055393));
#187004=CARTESIAN_POINT('Ctrl Pts',(5.89394459667191,3.32471142978785,14.4665050506801));
#187005=CARTESIAN_POINT('Ctrl Pts',(5.8000560129413,3.49115417901724,14.475493538417));
#187006=CARTESIAN_POINT('Ctrl Pts',(5.69905103909432,3.6537280320524,14.484482026154));
#187007=CARTESIAN_POINT('Ctrl Pts',(5.59125270914414,3.81184760221187,14.4934705138909));
#187008=CARTESIAN_POINT('Ctrl Pts',(5.49667450204816,3.95057577600994,14.5013566755323));
#187009=CARTESIAN_POINT('Ctrl Pts',(5.39686774681314,4.08587540680076,14.5092428371738));
#187010=CARTESIAN_POINT('Ctrl Pts',(5.29208000568106,4.21736626503683,14.5171289988152));
#187011=CARTESIAN_POINT('Ctrl Pts',(5.18417003098441,4.35277499731603,14.5252501348754));
#187012=CARTESIAN_POINT('Ctrl Pts',(5.07102484814056,4.48408297360082,14.5333712709357));
#187013=CARTESIAN_POINT('Ctrl Pts',(4.95299907767393,4.61086641929271,14.5414924069959));
#187014=CARTESIAN_POINT('Ctrl Pts',(4.83498371114816,4.73763868905696,14.5496128271802));
#187015=CARTESIAN_POINT('Ctrl Pts',(4.71208886415114,4.85988695540559,14.5577332473644));
#187016=CARTESIAN_POINT('Ctrl Pts',(4.5847075292805,4.97722270658634,14.5658536675486));
#187017=CARTESIAN_POINT('Ctrl Pts',(4.45727339209945,5.09460709596643,14.5739774538221));
#187018=CARTESIAN_POINT('Ctrl Pts',(4.32534932020104,5.20707465256417,14.5821012400956));
#187019=CARTESIAN_POINT('Ctrl Pts',(4.1893633935718,5.31427543100662,14.5902250263692));
#187020=CARTESIAN_POINT('Ctrl Pts',(4.05334626534985,5.42150080636957,14.5983506766229));
#187021=CARTESIAN_POINT('Ctrl Pts',(3.9132657186847,5.52345677640222,14.6064763268765));
#187022=CARTESIAN_POINT('Ctrl Pts',(3.76958042428815,5.6198356225804,14.6146019771302));
#187023=CARTESIAN_POINT('Ctrl Pts',(3.62577782930959,5.71629314970361,14.6227342609334));
#187024=CARTESIAN_POINT('Ctrl Pts',(3.47836491883093,5.80716426430875,14.6308665447365));
#187025=CARTESIAN_POINT('Ctrl Pts',(3.32782717117971,5.89218595419035,14.6389988285396));
#187026=CARTESIAN_POINT('Ctrl Pts',(3.2523509209764,5.93481392251282,14.6430761732364));
#187027=CARTESIAN_POINT('Ctrl Pts',(3.17608952358117,5.97597219538194,14.6471535179331));
#187028=CARTESIAN_POINT('Ctrl Pts',(3.09910619832135,6.0156321173694,14.6512308626299));
#187029=CARTESIAN_POINT('Origin',(0.,0.,4.30282021618968));
#187030=CARTESIAN_POINT('',(3.09910619832131,6.01563211736941,17.0457499898821));
#187031=CARTESIAN_POINT('',(3.09910619832134,6.0156321173694,16.6515631567322));
#187032=CARTESIAN_POINT('',(3.09910619832133,6.0156321173694,4.30282021618968));
#187033=CARTESIAN_POINT('',(-6.76699967914366,0.00208385931223479,15.6971797838561));
#187034=CARTESIAN_POINT('Ctrl Pts',(-6.76699967914366,0.0020838593122393,
15.6971797838561));
#187035=CARTESIAN_POINT('Ctrl Pts',(-6.7670521202577,-0.16821026745595,
15.7051773033024));
#187036=CARTESIAN_POINT('Ctrl Pts',(-6.76067197387033,-0.338604812283096,
15.7131748227487));
#187037=CARTESIAN_POINT('Ctrl Pts',(-6.74786284543056,-0.508562699436209,
15.721172342195));
#187038=CARTESIAN_POINT('Ctrl Pts',(-6.73505487207517,-0.678505260355175,
15.7291691404518));
#187039=CARTESIAN_POINT('Ctrl Pts',(-6.71581909033154,-0.848010863801087,
15.7371659387085));
#187040=CARTESIAN_POINT('Ctrl Pts',(-6.690211171013,-1.01654487714655,15.7451627369653));
#187041=CARTESIAN_POINT('Ctrl Pts',(-6.67000489770966,-1.14952890807099,
15.7514727182299));
#187042=CARTESIAN_POINT('Ctrl Pts',(-6.64583223149171,-1.28190798807919,
15.7577826994946));
#187043=CARTESIAN_POINT('Ctrl Pts',(-6.61774319506431,-1.41342279738939,
15.7640926807593));
#187044=CARTESIAN_POINT('Ctrl Pts',(-6.57937648024145,-1.59305840706321,
15.772711461697));
#187045=CARTESIAN_POINT('Ctrl Pts',(-6.53370534698295,-1.77106534870478,
15.7813302426348));
#187046=CARTESIAN_POINT('Ctrl Pts',(-6.48089964856677,-1.94685098176699,
15.7899490235725));
#187047=CARTESIAN_POINT('Ctrl Pts',(-6.42806223008849,-2.12274220819063,
15.7985729817596));
#187048=CARTESIAN_POINT('Ctrl Pts',(-6.36808178102674,-2.29640917181106,
15.8071969399466));
#187049=CARTESIAN_POINT('Ctrl Pts',(-6.30117751899081,-2.46727600283486,
15.8158208981337));
#187050=CARTESIAN_POINT('Ctrl Pts',(-6.23185623424901,-2.64431566945536,
15.8247564105045));
#187051=CARTESIAN_POINT('Ctrl Pts',(-6.15510167929091,-2.81834877879652,
15.8336919228754));
#187052=CARTESIAN_POINT('Ctrl Pts',(-6.07121110395118,-2.98875973126979,
15.8426274352463));
#187053=CARTESIAN_POINT('Ctrl Pts',(-5.99009416167758,-3.15353646976019,
15.8512675171415));
#187054=CARTESIAN_POINT('Ctrl Pts',(-5.90230570237236,-3.31492648760728,
15.8599075990367));
#187055=CARTESIAN_POINT('Ctrl Pts',(-5.80816043205675,-3.47239994751331,
15.868547680932));
#187056=CARTESIAN_POINT('Ctrl Pts',(-5.70918649535935,-3.63795014668964,
15.8776309085406));
#187057=CARTESIAN_POINT('Ctrl Pts',(-5.6031867602438,-3.79917114959769,
15.8867141361493));
#187058=CARTESIAN_POINT('Ctrl Pts',(-5.49057753511751,-3.95548319815202,
15.895797363758));
#187059=CARTESIAN_POINT('Ctrl Pts',(-5.37796830999122,-4.11179524670636,
15.9048805913667));
#187060=CARTESIAN_POINT('Ctrl Pts',(-5.25874986119406,-4.26319805706581,
15.9139638189754));
#187061=CARTESIAN_POINT('Ctrl Pts',(-5.13338667445239,-4.40915300829475,
15.9230470465841));
#187062=CARTESIAN_POINT('Ctrl Pts',(-5.00855668194227,-4.55448718447732,
15.9320916414435));
#187063=CARTESIAN_POINT('Ctrl Pts',(-4.87751949739731,-4.69455452798562,
15.9411362363029));
#187064=CARTESIAN_POINT('Ctrl Pts',(-4.74072311736272,-4.82885424552271,
15.9501808311623));
#187065=CARTESIAN_POINT('Ctrl Pts',(-4.6040522695395,-4.96303072192927,
15.9592171261822));
#187066=CARTESIAN_POINT('Ctrl Pts',(-4.4616329473042,-5.09144997275945,
15.9682534212022));
#187067=CARTESIAN_POINT('Ctrl Pts',(-4.31395041021026,-5.21364755792399,
15.9772897162221));
#187068=CARTESIAN_POINT('Ctrl Pts',(-4.16652920894673,-5.33562890487904,
15.9863100208094));
#187069=CARTESIAN_POINT('Ctrl Pts',(-4.01386357408612,-5.45141041972696,
15.9953303253966));
#187070=CARTESIAN_POINT('Ctrl Pts',(-3.85647211850355,-5.56056757887221,
16.0043506299839));
#187071=CARTESIAN_POINT('Ctrl Pts',(-3.69927886688481,-5.66958727578012,
16.0133595752498));
#187072=CARTESIAN_POINT('Ctrl Pts',(-3.53737186609623,-5.77199912975818,
16.0223685205158));
#187073=CARTESIAN_POINT('Ctrl Pts',(-3.37130104557159,-5.86742006849074,
16.0313774657817));
#187074=CARTESIAN_POINT('Ctrl Pts',(-3.2056073367235,-5.96262432647187,
16.0403659536401));
#187075=CARTESIAN_POINT('Ctrl Pts',(-3.03576888732917,-6.05086923855594,
16.0493544414985));
#187076=CARTESIAN_POINT('Ctrl Pts',(-2.86236227854642,-6.1318163040289,
16.0583429293568));
#187077=CARTESIAN_POINT('Ctrl Pts',(-2.71022184515229,-6.20283621330161,
16.0662290903742));
#187078=CARTESIAN_POINT('Ctrl Pts',(-2.55533529787698,-6.26823905314927,
16.0741152513916));
#187079=CARTESIAN_POINT('Ctrl Pts',(-2.39810960016431,-6.32782421892389,
16.0820014124089));
#187080=CARTESIAN_POINT('Ctrl Pts',(-2.23619267053671,-6.38918726093253,
16.0901228772652));
#187081=CARTESIAN_POINT('Ctrl Pts',(-2.07186682032972,-6.4443512810337,
16.0982443421215));
#187082=CARTESIAN_POINT('Ctrl Pts',(-1.90565336498755,-6.49313285344691,
16.1063658069778));
#187083=CARTESIAN_POINT('Ctrl Pts',(-1.73945176311115,-6.54191094701602,
16.1144866926541));
#187084=CARTESIAN_POINT('Ctrl Pts',(-1.57136317559847,-6.58430739639462,
16.1226075783304));
#187085=CARTESIAN_POINT('Ctrl Pts',(-1.40192394512038,-6.62018868704647,
16.1307284640067));
#187086=CARTESIAN_POINT('Ctrl Pts',(-1.23246446180843,-6.65607426653873,
16.1388503203611));
#187087=CARTESIAN_POINT('Ctrl Pts',(-1.06165437255065,-6.68544306195228,
16.1469721767155));
#187088=CARTESIAN_POINT('Ctrl Pts',(-0.890040024330387,-6.70821270943982,
16.1550940330699));
#187089=CARTESIAN_POINT('Ctrl Pts',(-0.7183004684055,-6.73099896938039,
16.1632218150301));
#187090=CARTESIAN_POINT('Ctrl Pts',(-0.545755844942392,-6.74717641700141,
16.1713495969904));
#187091=CARTESIAN_POINT('Ctrl Pts',(-0.372958076489848,-6.75671453246184,
16.1794773789507));
#187092=CARTESIAN_POINT('Ctrl Pts',(-0.200089916648785,-6.76625653339601,
16.1876084718673));
#187093=CARTESIAN_POINT('Ctrl Pts',(-0.0269687721454283,-6.76915380498501,
16.1957395647838));
#187094=CARTESIAN_POINT('Ctrl Pts',(0.145853877943232,-6.76542797214551,
16.2038706577004));
#187095=CARTESIAN_POINT('Ctrl Pts',(0.318865156731585,-6.76169807271519,
16.212010625365));
#187096=CARTESIAN_POINT('Ctrl Pts',(0.491576925299634,-6.75133065236554,
16.2201505930297));
#187097=CARTESIAN_POINT('Ctrl Pts',(0.663442506852932,-6.73439923379218,
16.2282905606944));
#187098=CARTESIAN_POINT('Ctrl Pts',(0.752579428421628,-6.72561786805402,
16.2325122998741));
#187099=CARTESIAN_POINT('Ctrl Pts',(0.841488875622032,-6.71507169204958,
16.2367340390539));
#187100=CARTESIAN_POINT('Ctrl Pts',(0.930095770580004,-6.70277635443323,
16.2409557782336));
#187101=CARTESIAN_POINT('Ctrl Pts',(1.10724095198241,-6.67819519950748,
16.2493959876912));
#187102=CARTESIAN_POINT('Ctrl Pts',(1.28354234272565,-6.64656898103088,
16.2578361971488));
#187103=CARTESIAN_POINT('Ctrl Pts',(1.45841803467938,-6.60797289916673,
16.2662764066064));
#187104=CARTESIAN_POINT('Ctrl Pts',(1.63316123238882,-6.56940605955255,
16.274710221355));
#187105=CARTESIAN_POINT('Ctrl Pts',(1.80648056009455,-6.52387995489371,
16.2831440361035));
#187106=CARTESIAN_POINT('Ctrl Pts',(1.97780258155493,-6.47152114640713,
16.291577850852));
#187107=CARTESIAN_POINT('Ctrl Pts',(2.14902113800454,-6.41919395851806,
16.3000065722405));
#187108=CARTESIAN_POINT('Ctrl Pts',(2.31824447484924,-6.36004239062506,
16.308435293629));
#187109=CARTESIAN_POINT('Ctrl Pts',(2.48491225687541,-6.29424340772029,
16.3168640150175));
#187110=CARTESIAN_POINT('Ctrl Pts',(2.65150497784993,-6.22847405826234,
16.3252889404193));
#187111=CARTESIAN_POINT('Ctrl Pts',(2.81554412915676,-6.15606338525117,
16.3337138658211));
#187112=CARTESIAN_POINT('Ctrl Pts',(2.97648699809208,-6.07723737813399,
16.3421387912228));
#187113=CARTESIAN_POINT('Ctrl Pts',(3.13738207766922,-5.99843477711309,
16.3505612149805));
#187114=CARTESIAN_POINT('Ctrl Pts',(3.29518240916876,-5.91322078735922,
16.3589836387382));
#187115=CARTESIAN_POINT('Ctrl Pts',(3.44936727774601,-5.82186863328391,
16.3674060624958));
#187116=CARTESIAN_POINT('Ctrl Pts',(3.60355457120818,-5.73051504250173,
16.375828618714));
#187117=CARTESIAN_POINT('Ctrl Pts',(3.75412599791343,-5.63302325874053,
16.3842511749322));
#187118=CARTESIAN_POINT('Ctrl Pts',(3.90058679873038,-5.52971171269989,
16.3926737311504));
#187119=CARTESIAN_POINT('Ctrl Pts',(4.04705254702083,-5.42639667677572,
16.4010965718841));
#187120=CARTESIAN_POINT('Ctrl Pts',(4.18940711987043,-5.31726167872461,
16.4095194126179));
#187121=CARTESIAN_POINT('Ctrl Pts',(4.32718590777588,-5.20266769259251,
16.4179422533516));
#187122=CARTESIAN_POINT('Ctrl Pts',(4.46498858531797,-5.08805383686558,
16.4263665545323));
#187123=CARTESIAN_POINT('Ctrl Pts',(4.59821363965822,-4.96797931922905,
16.4347908557129));
#187124=CARTESIAN_POINT('Ctrl Pts',(4.72643035747701,-4.84284472969346,
16.4432151568935));
#187125=CARTESIAN_POINT('Ctrl Pts',(4.85468721291069,-4.71767096738813,
16.4516420952603));
#187126=CARTESIAN_POINT('Ctrl Pts',(4.97793236736254,-4.58743420794316,
16.4600690336272));
#187127=CARTESIAN_POINT('Ctrl Pts',(5.09577246137279,-4.45257139436469,
16.468495971994));
#187128=CARTESIAN_POINT('Ctrl Pts',(5.21371850843952,-4.31758732216517,
16.4769304872376));
#187129=CARTESIAN_POINT('Ctrl Pts',(5.3262495646675,-4.17796913610944,16.4853650024813));
#187130=CARTESIAN_POINT('Ctrl Pts',(5.43301230000867,-4.03418719793151,
16.4937995177249));
#187131=CARTESIAN_POINT('Ctrl Pts',(5.53982660266573,-3.89033581184556,
16.5022381069117));
#187132=CARTESIAN_POINT('Ctrl Pts',(5.64086683560098,-3.74231693511833,
16.5106766960985));
#187133=CARTESIAN_POINT('Ctrl Pts',(5.73582313106234,-3.59062975105624,
16.5191152852852));
#187134=CARTESIAN_POINT('Ctrl Pts',(5.83088556617843,-3.43877301504117,
16.5275633069055));
#187135=CARTESIAN_POINT('Ctrl Pts',(5.9198503052829,-3.28324006553135,16.5360113285258));
#187136=CARTESIAN_POINT('Ctrl Pts',(6.00245295327843,-3.12455557538654,
16.544459350146));
#187137=CARTESIAN_POINT('Ctrl Pts',(6.049402972765,-3.03436185780838,16.5492610700584));
#187138=CARTESIAN_POINT('Ctrl Pts',(6.09429851404738,-2.94315041219203,
16.5540627899708));
#187139=CARTESIAN_POINT('Ctrl Pts',(6.13709797108092,-2.85102043018889,
16.5588645098832));
#187140=CARTESIAN_POINT('Ctrl Pts',(6.21053988270025,-2.69292959295087,
16.567104041734));
#187141=CARTESIAN_POINT('Ctrl Pts',(6.27797104774454,-2.53178012643929,
16.5753435735848));
#187142=CARTESIAN_POINT('Ctrl Pts',(6.33912819305863,-2.36806730309111,
16.5835831054356));
#187143=CARTESIAN_POINT('Ctrl Pts',(6.40021745821566,-2.20453618953507,
16.5918134919819));
#187144=CARTESIAN_POINT('Ctrl Pts',(6.45504644613494,-2.03844771477305,
16.6000438785282));
#187145=CARTESIAN_POINT('Ctrl Pts',(6.50339839124998,-1.87032039091893,
16.6082742650745));
#187146=CARTESIAN_POINT('Ctrl Pts',(6.55170529462805,-1.70234968427394,
16.6164969846923));
#187147=CARTESIAN_POINT('Ctrl Pts',(6.59354707346849,-1.53234425099341,
16.6247197043101));
#187148=CARTESIAN_POINT('Ctrl Pts',(6.62875554495046,-1.3608412564618,16.632942423928));
#187149=CARTESIAN_POINT('Ctrl Pts',(6.66393281918988,-1.18949022594039,
16.6411578576237));
#187150=CARTESIAN_POINT('Ctrl Pts',(6.69248842935787,-1.0166446262052,16.6493732913195));
#187151=CARTESIAN_POINT('Ctrl Pts',(6.71430442928295,-0.842855284679038,
16.6575887250153));
#187152=CARTESIAN_POINT('Ctrl Pts',(6.73610921747826,-0.669155257378234,
16.6657999366161));
#187153=CARTESIAN_POINT('Ctrl Pts',(6.75118124934669,-0.494512806498292,
16.674011148217));
#187154=CARTESIAN_POINT('Ctrl Pts',(6.75945386287016,-0.319487833461174,
16.6822223598178));
#187155=CARTESIAN_POINT('Ctrl Pts',(6.76772370221547,-0.144521554143462,
16.6904308178313));
#187156=CARTESIAN_POINT('Ctrl Pts',(6.76919864868656,0.0308266366642572,
16.6986392758448));
#187157=CARTESIAN_POINT('Ctrl Pts',(6.76386398338847,0.205992752834478,
16.7068477338583));
#187158=CARTESIAN_POINT('Ctrl Pts',(6.76148727351153,0.284033082478986,
16.7105047811415));
#187159=CARTESIAN_POINT('Ctrl Pts',(6.75775961671522,0.362037242752052,
16.7141618284247));
#187160=CARTESIAN_POINT('Ctrl Pts',(6.75268304404148,0.439955346273543,
16.7178188757079));
#187161=CARTESIAN_POINT('Ctrl Pts',(6.74038521729946,0.628709334201627,
16.7266779498838));
#187162=CARTESIAN_POINT('Ctrl Pts',(6.72018099636176,0.816761881881035,
16.7355370240597));
#187163=CARTESIAN_POINT('Ctrl Pts',(6.6921848122862,1.00346969969496,16.7443960982357));
#187164=CARTESIAN_POINT('Ctrl Pts',(6.66413602901304,1.19052830393664,16.7532718168297));
#187165=CARTESIAN_POINT('Ctrl Pts',(6.6282660647866,1.37623687292825,16.7621475354237));
#187166=CARTESIAN_POINT('Ctrl Pts',(6.58474016644733,1.55996344199958,16.7710232540177));
#187167=CARTESIAN_POINT('Ctrl Pts',(6.5410900574927,1.74421431478603,16.7799243014047));
#187168=CARTESIAN_POINT('Ctrl Pts',(6.48974035393471,1.92647161523584,16.7888253487917));
#187169=CARTESIAN_POINT('Ctrl Pts',(6.43090674026688,2.10611668669852,16.7977263961787));
#187170=CARTESIAN_POINT('Ctrl Pts',(6.37199314149442,2.28600598809953,16.8066395446617));
#187171=CARTESIAN_POINT('Ctrl Pts',(6.30557539532221,2.46327572216089,16.8155526931447));
#187172=CARTESIAN_POINT('Ctrl Pts',(6.23191745348678,2.63732702805831,16.8244658416277));
#187173=CARTESIAN_POINT('Ctrl Pts',(6.15809597087899,2.8117647754485,16.8333987797376));
#187174=CARTESIAN_POINT('Ctrl Pts',(6.07700224068373,2.98296956206476,16.8423317178475));
#187175=CARTESIAN_POINT('Ctrl Pts',(5.98894759872456,3.15036436935973,16.8512646559574));
#187176=CARTESIAN_POINT('Ctrl Pts',(5.90513234697211,3.30969995466581,16.8597675178158));
#187177=CARTESIAN_POINT('Ctrl Pts',(5.81501076015396,3.46558362627804,16.8682703796742));
#187178=CARTESIAN_POINT('Ctrl Pts',(5.71888781512685,3.61754214322289,16.8767732415327));
#187179=CARTESIAN_POINT('Ctrl Pts',(5.62593516252746,3.76448881897351,16.884995665057));
#187180=CARTESIAN_POINT('Ctrl Pts',(5.52719150557644,3.9080460880147,16.8932180885814));
#187181=CARTESIAN_POINT('Ctrl Pts',(5.42293159249036,4.04772799767598,16.9014405121058));
#187182=CARTESIAN_POINT('Ctrl Pts',(5.31877753311522,4.18726809014164,16.9096545875124));
#187183=CARTESIAN_POINT('Ctrl Pts',(5.20911858104267,4.32294037191763,16.9178686629189));
#187184=CARTESIAN_POINT('Ctrl Pts',(5.09427405997421,4.45428566684647,16.9260827383254));
#187185=CARTESIAN_POINT('Ctrl Pts',(4.97952524718653,4.58552150220118,16.9342899683463));
#187186=CARTESIAN_POINT('Ctrl Pts',(4.85959970585535,4.71243726296862,16.9424971983672));
#187187=CARTESIAN_POINT('Ctrl Pts',(4.73485855607681,4.83460478777182,16.9507044283881));
#187188=CARTESIAN_POINT('Ctrl Pts',(4.61020636846293,4.95668518585319,16.9589058052246));
#187189=CARTESIAN_POINT('Ctrl Pts',(4.48074567080274,5.07402384514603,16.9671071820611));
#187190=CARTESIAN_POINT('Ctrl Pts',(4.34687611502017,5.1862276310115,16.9753085588977));
#187191=CARTESIAN_POINT('Ctrl Pts',(4.21306369010708,5.29838353220441,16.9835064356718));
#187192=CARTESIAN_POINT('Ctrl Pts',(4.07484642885521,5.40540869456424,16.991704312446));
#187193=CARTESIAN_POINT('Ctrl Pts',(3.93265907105681,5.5069484863066,16.9999021892202));
#187194=CARTESIAN_POINT('Ctrl Pts',(3.79048911022339,5.60847585441139,17.0080990629645));
#187195=CARTESIAN_POINT('Ctrl Pts',(3.64435030833864,5.70451897517738,17.0162959367087));
#187196=CARTESIAN_POINT('Ctrl Pts',(3.4947087676297,5.79476484677783,17.024492810453));
#187197=CARTESIAN_POINT('Ctrl Pts',(3.36535225195713,5.87277721853478,17.0315785369294));
#187198=CARTESIAN_POINT('Ctrl Pts',(3.23337889068404,5.94645811785487,17.0386642634057));
#187199=CARTESIAN_POINT('Ctrl Pts',(3.09910619832132,6.01563211736941,17.0457499898821));
#187200=CARTESIAN_POINT('Ctrl Pts',(3.09910619832132,6.01563211736941,15.0460438035976));
#187201=CARTESIAN_POINT('Ctrl Pts',(2.94683466579232,6.09407867811004,15.0540873050715));
#187202=CARTESIAN_POINT('Ctrl Pts',(2.79144048604734,6.16681301554515,15.0621308065454));
#187203=CARTESIAN_POINT('Ctrl Pts',(2.63340158188346,6.23357723209825,15.0701743080193));
#187204=CARTESIAN_POINT('Ctrl Pts',(2.47544989763591,6.30030460222159,15.078213370374));
#187205=CARTESIAN_POINT('Ctrl Pts',(2.31485673767434,6.36106826587078,15.0862524327287));
#187206=CARTESIAN_POINT('Ctrl Pts',(2.15212302068412,6.41565705940097,15.0942914950835));
#187207=CARTESIAN_POINT('Ctrl Pts',(1.98938880463277,6.4702460203405,15.1023305820919));
#187208=CARTESIAN_POINT('Ctrl Pts',(1.82451436543312,6.51865993475011,15.1103696691003));
#187209=CARTESIAN_POINT('Ctrl Pts',(1.65801933962676,6.56073630543277,15.1184087561087));
#187210=CARTESIAN_POINT('Ctrl Pts',(1.49156455312839,6.60280250689848,15.1264459001924));
#187211=CARTESIAN_POINT('Ctrl Pts',(1.32349032463615,6.63853413246334,15.1344830442761));
#187212=CARTESIAN_POINT('Ctrl Pts',(1.15432930022063,6.66781919870749,15.1425201883598));
#187213=CARTESIAN_POINT('Ctrl Pts',(0.985145296468844,6.69710824312207,
15.150558424233));
#187214=CARTESIAN_POINT('Ctrl Pts',(0.814874571008829,6.71994892092555,
15.1585966601062));
#187215=CARTESIAN_POINT('Ctrl Pts',(0.644057893040867,6.73628075650145,
15.1666348959795));
#187216=CARTESIAN_POINT('Ctrl Pts',(0.473184164145204,6.75261804673425,
15.1746758165368));
#187217=CARTESIAN_POINT('Ctrl Pts',(0.301764491440067,6.76244213216339,
15.1827167370941));
#187218=CARTESIAN_POINT('Ctrl Pts',(0.130342518113964,6.76574458784632,
15.1907576576514));
#187219=CARTESIAN_POINT('Ctrl Pts',(-0.0412818148417761,6.76905094200093,
15.1988080703273));
#187220=CARTESIAN_POINT('Ctrl Pts',(-0.212908080014956,6.76582028224575,
15.2068584830033));
#187221=CARTESIAN_POINT('Ctrl Pts',(-0.383993985147717,6.75609632993568,
15.2149088956792));
#187222=CARTESIAN_POINT('Ctrl Pts',(-0.555182441695757,6.74636654894516,
15.2229641338912));
#187223=CARTESIAN_POINT('Ctrl Pts',(-0.725829522287586,6.73013575926323,
15.2310193721033));
#187224=CARTESIAN_POINT('Ctrl Pts',(-0.895400813033327,6.707499264556,15.2390746103153));
#187225=CARTESIAN_POINT('Ctrl Pts',(-1.06525494352509,6.68482501286535,
15.2471432844192));
#187226=CARTESIAN_POINT('Ctrl Pts',(-1.23402933192111,6.655723773479,15.2552119585232));
#187227=CARTESIAN_POINT('Ctrl Pts',(-1.40120124622319,6.62034168812929,
15.2632806326271));
#187228=CARTESIAN_POINT('Ctrl Pts',(-1.56659776926395,6.58533536592975,
15.2712636161798));
#187229=CARTESIAN_POINT('Ctrl Pts',(-1.73042538138055,6.54418113218147,
15.2792465997324));
#187230=CARTESIAN_POINT('Ctrl Pts',(-1.89219669410863,6.4970670822152,15.2872295832851));
#187231=CARTESIAN_POINT('Ctrl Pts',(-2.0610593416958,6.44788776184194,15.2955625053317));
#187232=CARTESIAN_POINT('Ctrl Pts',(-2.22822032661907,6.39205789325241,
15.3038954273784));
#187233=CARTESIAN_POINT('Ctrl Pts',(-2.39312566877512,6.3297107780253,15.312228349425));
#187234=CARTESIAN_POINT('Ctrl Pts',(-2.55783613280683,6.26743734196901,
15.3205514239785));
#187235=CARTESIAN_POINT('Ctrl Pts',(-2.72029594151521,6.19866212387286,
15.3288744985321));
#187236=CARTESIAN_POINT('Ctrl Pts',(-2.87996466079607,6.12356861254659,
15.3371975730856));
#187237=CARTESIAN_POINT('Ctrl Pts',(-3.03947399848063,6.04855005969535,
15.3455123395315));
#187238=CARTESIAN_POINT('Ctrl Pts',(-3.19619748457894,5.96722592621008,
15.3538271059774));
#187239=CARTESIAN_POINT('Ctrl Pts',(-3.34961290893504,5.87982842949484,
15.3621418724233));
#187240=CARTESIAN_POINT('Ctrl Pts',(-3.50290333529777,5.79250214147169,
15.3704498642628));
#187241=CARTESIAN_POINT('Ctrl Pts',(-3.65289076950655,5.69911252176903,
15.3787578561022));
#187242=CARTESIAN_POINT('Ctrl Pts',(-3.79907574206022,5.59993861627872,
15.3870658479417));
#187243=CARTESIAN_POINT('Ctrl Pts',(-3.94516840838345,5.5008273326107,15.3953685938287));
#187244=CARTESIAN_POINT('Ctrl Pts',(-4.08746311084286,5.39593923673922,
15.4036713397158));
#187245=CARTESIAN_POINT('Ctrl Pts',(-4.22548743446519,5.28559787925423,
15.4119740856028));
#187246=CARTESIAN_POINT('Ctrl Pts',(-4.36345535194457,5.17530161476604,
15.4202734384222));
#187247=CARTESIAN_POINT('Ctrl Pts',(-4.497156096631,5.05955674617516,15.4285727912416));
#187248=CARTESIAN_POINT('Ctrl Pts',(-4.62614832778306,4.93872864706596,
15.4368721440609));
#187249=CARTESIAN_POINT('Ctrl Pts',(-4.75511312445184,4.81792624606614,
15.4451697317472));
#187250=CARTESIAN_POINT('Ctrl Pts',(-4.87937114888155,4.69204300608057,
15.4534673194335));
#187251=CARTESIAN_POINT('Ctrl Pts',(-4.99851592060525,4.56148304737131,
15.4617649071197));
#187252=CARTESIAN_POINT('Ctrl Pts',(-5.11765515114784,4.4309291607403,15.4700621089021));
#187253=CARTESIAN_POINT('Ctrl Pts',(-5.23168136849243,4.29569924589025,
15.4783593106844));
#187254=CARTESIAN_POINT('Ctrl Pts',(-5.34022646277026,4.15623270839449,
15.4866565124667));
#187255=CARTESIAN_POINT('Ctrl Pts',(-5.44878454554038,4.01674948235046,
15.4949547070912));
#187256=CARTESIAN_POINT('Ctrl Pts',(-5.55185998515246,3.87302889839739,
15.5032529017157));
#187257=CARTESIAN_POINT('Ctrl Pts',(-5.64912620083537,3.72554186220412,
15.5115510963401));
#187258=CARTESIAN_POINT('Ctrl Pts',(-5.74646082498203,3.5779510966584,15.5198551271816));
#187259=CARTESIAN_POINT('Ctrl Pts',(-5.83797786940588,3.42658887645757,
15.5281591580231));
#187260=CARTESIAN_POINT('Ctrl Pts',(-5.92339471510942,3.27195416364806,
15.5364631888646));
#187261=CARTESIAN_POINT('Ctrl Pts',(-6.00884262072878,3.11726322140131,
15.5447702392803));
#187262=CARTESIAN_POINT('Ctrl Pts',(-6.0881857447487,2.95929772285178,15.5530772896959));
#187263=CARTESIAN_POINT('Ctrl Pts',(-6.16118828164667,2.79857963225987,
15.5613843401116));
#187264=CARTESIAN_POINT('Ctrl Pts',(-6.23426887057748,2.63768970690413,
15.5697002721662));
#187265=CARTESIAN_POINT('Ctrl Pts',(-6.30099519032929,2.47404162937591,
15.5780162042207));
#187266=CARTESIAN_POINT('Ctrl Pts',(-6.36117987073296,2.30817669431562,
15.5863321362753));
#187267=CARTESIAN_POINT('Ctrl Pts',(-6.40654836119194,2.18314418316346,
15.592600862495));
#187268=CARTESIAN_POINT('Ctrl Pts',(-6.44820059210438,2.05685234661173,
15.5988695887148));
#187269=CARTESIAN_POINT('Ctrl Pts',(-6.48607526764064,1.92953792979057,
15.6051383149346));
#187270=CARTESIAN_POINT('Ctrl Pts',(-6.54100728234485,1.74488585507684,
15.6142302412945));
#187271=CARTESIAN_POINT('Ctrl Pts',(-6.58807826959424,1.55779126982591,
15.6233221676544));
#187272=CARTESIAN_POINT('Ctrl Pts',(-6.62709478667593,1.36890601883865,
15.6324140940143));
#187273=CARTESIAN_POINT('Ctrl Pts',(-6.6660529089167,1.18030346669301,15.641492412763));
#187274=CARTESIAN_POINT('Ctrl Pts',(-6.69698057155371,0.989915816809847,
15.6505707315118));
#187275=CARTESIAN_POINT('Ctrl Pts',(-6.71973467568172,0.798407720679577,
15.6596490502605));
#187276=CARTESIAN_POINT('Ctrl Pts',(-6.74243203827094,0.607377185168806,
15.6687047305537));
#187277=CARTESIAN_POINT('Ctrl Pts',(-6.75699649243608,0.415232002965931,
15.6777604108468));
#187278=CARTESIAN_POINT('Ctrl Pts',(-6.76333634483653,0.222644305144609,
15.68681609114));
#187279=CARTESIAN_POINT('Ctrl Pts',(-6.76575487404414,0.149175879889805,
15.6902706553633));
#187280=CARTESIAN_POINT('Ctrl Pts',(-6.7669770269594,0.075643168492496,
15.6937252195867));
#187281=CARTESIAN_POINT('Ctrl Pts',(-6.76699967914336,0.00208386029358956,
15.69717978381));
#187282=CARTESIAN_POINT('',(-6.76699999457021,0.000271084328258356,15.3028202162169));
#187283=CARTESIAN_POINT('Ctrl Pts',(3.09910619832135,6.0156321173694,14.6512308626299));
#187284=CARTESIAN_POINT('Ctrl Pts',(2.94269490714649,6.09621138028141,14.6595150299666));
#187285=CARTESIAN_POINT('Ctrl Pts',(2.78330245775587,6.17060202482753,14.6677991973033));
#187286=CARTESIAN_POINT('Ctrl Pts',(2.62147298918087,6.23860307817344,14.6760833646399));
#187287=CARTESIAN_POINT('Ctrl Pts',(2.45659527075519,6.30788501195809,14.6845235740873));
#187288=CARTESIAN_POINT('Ctrl Pts',(2.28884715097256,6.37067805532276,14.6929637835347));
#187289=CARTESIAN_POINT('Ctrl Pts',(2.11876740895101,6.42674985251231,14.701403992982));
#187290=CARTESIAN_POINT('Ctrl Pts',(1.94881652753641,6.48277916700679,14.7098378077201));
#187291=CARTESIAN_POINT('Ctrl Pts',(1.77653786095828,6.53209728252431,14.7182716224581));
#187292=CARTESIAN_POINT('Ctrl Pts',(1.60248911927806,6.57452033403164,14.7267054371961));
#187293=CARTESIAN_POINT('Ctrl Pts',(1.42854548933681,6.61691776535537,14.735134158574));
#187294=CARTESIAN_POINT('Ctrl Pts',(1.25283423865705,6.65242835557688,14.7435628799518));
#187295=CARTESIAN_POINT('Ctrl Pts',(1.07592753892944,6.68091827004142,14.7519916013297));
#187296=CARTESIAN_POINT('Ctrl Pts',(0.899100511491493,6.70939535369333,
14.7604165267205));
#187297=CARTESIAN_POINT('Ctrl Pts',(0.721079437181532,6.73085801303605,
14.7688414521114));
#187298=CARTESIAN_POINT('Ctrl Pts',(0.542446357160277,6.74522356557613,
14.7772663775022));
#187299=CARTESIAN_POINT('Ctrl Pts',(0.36386631931795,6.75958485249974,14.7856888012489));
#187300=CARTESIAN_POINT('Ctrl Pts',(0.184674970220197,6.76685320847487,
14.7941112249956));
#187301=CARTESIAN_POINT('Ctrl Pts',(0.00545954463865506,6.76699779764796,
14.8025336487423));
#187302=CARTESIAN_POINT('Ctrl Pts',(-0.173758699481983,6.76714238909503,
14.8109562049493));
#187303=CARTESIAN_POINT('Ctrl Pts',(-0.353000687448234,6.76016298296884,
14.8193787611563));
#187304=CARTESIAN_POINT('Ctrl Pts',(-0.531678429810775,6.74608086575265,
14.8278013173633));
#187305=CARTESIAN_POINT('Ctrl Pts',(-0.710362207939442,6.73199827284001,
14.8362241580858));
#187306=CARTESIAN_POINT('Ctrl Pts',(-0.88848136990042,6.71081251647774,
14.8446469988082));
#187307=CARTESIAN_POINT('Ctrl Pts',(-1.06545213723992,6.68259685625662,
14.8530698395307));
#187308=CARTESIAN_POINT('Ctrl Pts',(-1.24245358976082,6.65437630368709,
14.8614941407));
#187309=CARTESIAN_POINT('Ctrl Pts',(-1.41830592127252,6.61912346960152,
14.8699184418693));
#187310=CARTESIAN_POINT('Ctrl Pts',(-1.59243428027399,6.57696298172707,
14.8783427430386));
#187311=CARTESIAN_POINT('Ctrl Pts',(-1.76661714930328,6.53478929571891,
14.886769681394));
#187312=CARTESIAN_POINT('Ctrl Pts',(-1.93907464577638,6.48570372313361,
14.8951966197494));
#187313=CARTESIAN_POINT('Ctrl Pts',(-2.10924548398185,6.42988121883307,
14.9036235581048));
#187314=CARTESIAN_POINT('Ctrl Pts',(-2.27956932716175,6.37400852308413,
14.912058073337));
#187315=CARTESIAN_POINT('Ctrl Pts',(-2.44760208662373,6.31138689614873,
14.9204925885693));
#187316=CARTESIAN_POINT('Ctrl Pts',(-2.61279984093959,6.24224046246106,
14.9289271038016));
#187317=CARTESIAN_POINT('Ctrl Pts',(-2.77807738718611,6.17306063045351,
14.937365692977));
#187318=CARTESIAN_POINT('Ctrl Pts',(-2.94051689298704,6.09734984249978,
14.9458042821524));
#187319=CARTESIAN_POINT('Ctrl Pts',(-3.09959709972066,6.01537919165561,
14.9542428713278));
#187320=CARTESIAN_POINT('Ctrl Pts',(-3.25885512213654,5.93331691616809,
14.9626908929368));
#187321=CARTESIAN_POINT('Ctrl Pts',(-3.41474604975449,5.84498095638228,
14.9711389145458));
#187322=CARTESIAN_POINT('Ctrl Pts',(-3.56677471626288,5.75068753484554,
14.9795869361548));
#187323=CARTESIAN_POINT('Ctrl Pts',(-3.65318537300047,5.69709266574515,
14.9843886561997));
#187324=CARTESIAN_POINT('Ctrl Pts',(-3.73834881761911,5.6415739688035,14.9891903762446));
#187325=CARTESIAN_POINT('Ctrl Pts',(-3.822178642059,5.58419550411589,14.9939920962895));
#187326=CARTESIAN_POINT('Ctrl Pts',(-3.96602678446965,5.48573668453899,
15.002231628144));
#187327=CARTESIAN_POINT('Ctrl Pts',(-4.10626736969548,5.38157963553009,
15.0104711599985));
#187328=CARTESIAN_POINT('Ctrl Pts',(-4.24242120299033,5.27201587027373,
15.018710691853));
#187329=CARTESIAN_POINT('Ctrl Pts',(-4.37842391504549,5.16257371313982,
15.026941078403));
#187330=CARTESIAN_POINT('Ctrl Pts',(-4.51034863228934,5.0477370100724,15.035171464953));
#187331=CARTESIAN_POINT('Ctrl Pts',(-4.63774429064585,4.92784099729099,
15.043401851503));
#187332=CARTESIAN_POINT('Ctrl Pts',(-4.76502127493901,4.80805667235828,
15.0516245711244));
#187333=CARTESIAN_POINT('Ctrl Pts',(-4.88777734489452,4.68322266610921,
15.0598472907458));
#187334=CARTESIAN_POINT('Ctrl Pts',(-5.00559369260521,4.55371505306941,
15.0680700103672));
#187335=CARTESIAN_POINT('Ctrl Pts',(-5.12330564654278,4.42432219310621,
15.0762854440665));
#187336=CARTESIAN_POINT('Ctrl Pts',(-5.23608636332162,4.2902642423217,15.0845008777659));
#187337=CARTESIAN_POINT('Ctrl Pts',(-5.34355326109191,4.15195466568145,
15.0927163114652));
#187338=CARTESIAN_POINT('Ctrl Pts',(-5.45096492922155,4.01371616942388,
15.1009275230696));
#187339=CARTESIAN_POINT('Ctrl Pts',(-5.55306799931583,3.87123067929587,
15.1091387346739));
#187340=CARTESIAN_POINT('Ctrl Pts',(-5.64951935821436,3.72494564002767,
15.1173499462783));
#187341=CARTESIAN_POINT('Ctrl Pts',(-5.74593837264833,3.57870965669112,
15.1255584042953));
#187342=CARTESIAN_POINT('Ctrl Pts',(-5.83670925573151,3.42867695926469,
15.1337668623123));
#187343=CARTESIAN_POINT('Ctrl Pts',(-5.92153147632753,3.27532501820237,
15.1419753203293));
#187344=CARTESIAN_POINT('Ctrl Pts',(-5.95932162752477,3.20700338032947,
15.1456323675909));
#187345=CARTESIAN_POINT('Ctrl Pts',(-5.99593160958208,3.138023284743,15.1492894148526));
#187346=CARTESIAN_POINT('Ctrl Pts',(-6.03133770514223,3.06842866733606,
15.1529464621142));
#187347=CARTESIAN_POINT('Ctrl Pts',(-6.11593347616295,2.90214627371737,
15.1616842437833));
#187348=CARTESIAN_POINT('Ctrl Pts',(-6.19357452955852,2.73250963683915,
15.1704220254524));
#187349=CARTESIAN_POINT('Ctrl Pts',(-6.26403344654619,2.5601121031218,15.1791598071215));
#187350=CARTESIAN_POINT('Ctrl Pts',(-6.33460020912402,2.38745069487214,
15.1879109629845));
#187351=CARTESIAN_POINT('Ctrl Pts',(-6.39796277023565,2.21202020841254,
15.1966621188475));
#187352=CARTESIAN_POINT('Ctrl Pts',(-6.4539431889,2.03443021862419,15.2054132747105));
#187353=CARTESIAN_POINT('Ctrl Pts',(-6.51006016205904,1.85640702894389,
15.2141857774962));
#187354=CARTESIAN_POINT('Ctrl Pts',(-6.5587588865186,1.67621406763521,15.2229582802819));
#187355=CARTESIAN_POINT('Ctrl Pts',(-6.599911682748,1.49447475051487,15.2317307830675));
#187356=CARTESIAN_POINT('Ctrl Pts',(-6.64111555804406,1.3125098576003,15.2405141743297));
#187357=CARTESIAN_POINT('Ctrl Pts',(-6.67475474703704,1.12899505147279,
15.2492975655919));
#187358=CARTESIAN_POINT('Ctrl Pts',(-6.7007531753093,0.944561212194508,
15.258080956854));
#187359=CARTESIAN_POINT('Ctrl Pts',(-6.72680535944485,0.759746026776842,
15.2668825091671));
#187360=CARTESIAN_POINT('Ctrl Pts',(-6.74518515453027,0.57400828762247,
15.2756840614802));
#187361=CARTESIAN_POINT('Ctrl Pts',(-6.75586838666445,0.387983687888932,
15.2844856137933));
#187362=CARTESIAN_POINT('Ctrl Pts',(-6.76328650286802,0.258813781233941,
15.2905971479255));
#187363=CARTESIAN_POINT('Ctrl Pts',(-6.76699481745752,0.129505585506803,
15.2967086820577));
#187364=CARTESIAN_POINT('Ctrl Pts',(-6.76699999457019,0.000271084898373194,
15.3028202161899));
#187365=CARTESIAN_POINT('Ctrl Pts',(-6.76699999457022,0.00027108432828991,
15.3028202162169));
#187366=CARTESIAN_POINT('Ctrl Pts',(-6.76700255864279,-0.0637351207553848,
15.3058470867909));
#187367=CARTESIAN_POINT('Ctrl Pts',(-6.76609702024371,-0.127738852254252,
15.3088739573649));
#187368=CARTESIAN_POINT('Ctrl Pts',(-6.76428353672319,-0.191721764063444,
15.3119008279389));
#187369=CARTESIAN_POINT('Ctrl Pts',(-6.75935707096965,-0.365536204764654,
15.3201235518042));
#187370=CARTESIAN_POINT('Ctrl Pts',(-6.74772026327342,-0.539391915402444,
15.3283462756694));
#187371=CARTESIAN_POINT('Ctrl Pts',(-6.72936133136258,-0.712730714900107,
15.3365689995347));
#187372=CARTESIAN_POINT('Ctrl Pts',(-6.71102183175931,-0.885886041149936,
15.3447830199252));
#187373=CARTESIAN_POINT('Ctrl Pts',(-6.68597441393982,-1.0585251920136,
15.3529970403158));
#187374=CARTESIAN_POINT('Ctrl Pts',(-6.65425929575064,-1.23009033201476,
15.3612110607064));
#187375=CARTESIAN_POINT('Ctrl Pts',(-6.62257137944063,-1.40150832155665,
15.3694180359777));
#187376=CARTESIAN_POINT('Ctrl Pts',(-6.58422721718039,-1.57185378408319,
15.3776250112489));
#187377=CARTESIAN_POINT('Ctrl Pts',(-6.53931879045859,-1.74057426062642,
15.3858319865202));
#187378=CARTESIAN_POINT('Ctrl Pts',(-6.49443986767699,-1.90918389118343,
15.3940335699726));
#187379=CARTESIAN_POINT('Ctrl Pts',(-6.44300536253492,-2.07617031684357,
15.4022351534249));
#187380=CARTESIAN_POINT('Ctrl Pts',(-6.38515828866142,-2.24099143879185,
15.4104367368772));
#187381=CARTESIAN_POINT('Ctrl Pts',(-6.32733761079827,-2.40573735174945,
15.4186345778916));
#187382=CARTESIAN_POINT('Ctrl Pts',(-6.26311031225825,-2.56831959163386,
15.426832418906));
#187383=CARTESIAN_POINT('Ctrl Pts',(-6.192669219541,-2.72821130731281,15.4350302599204));
#187384=CARTESIAN_POINT('Ctrl Pts',(-6.12223434303097,-2.88808891304543,
15.4432273775009));
#187385=CARTESIAN_POINT('Ctrl Pts',(-6.045586901243,-3.04527613601308,15.4514244950813));
#187386=CARTESIAN_POINT('Ctrl Pts',(-5.96296796355096,-3.19926586354822,
15.4596216126618));
#187387=CARTESIAN_POINT('Ctrl Pts',(-5.88034994508676,-3.35325387777588,
15.4678186390402));
#187388=CARTESIAN_POINT('Ctrl Pts',(-5.79176073175118,-3.50404415072474,
15.4760156654186));
#187389=CARTESIAN_POINT('Ctrl Pts',(-5.69748742591885,-3.65115406844145,
15.484212691797));
#187390=CARTESIAN_POINT('Ctrl Pts',(-5.60319802723507,-3.79828909844242,
15.4924111174424));
#187391=CARTESIAN_POINT('Ctrl Pts',(-5.50322279654648,-3.94174221941773,
15.5006095430878));
#187392=CARTESIAN_POINT('Ctrl Pts',(-5.3978922690997,-4.08105967258428,
15.5088079687332));
#187393=CARTESIAN_POINT('Ctrl Pts',(-5.29252460879435,-4.22042624024224,
15.5170092846231));
#187394=CARTESIAN_POINT('Ctrl Pts',(-5.18179810721346,-4.355653949734,15.525210600513));
#187395=CARTESIAN_POINT('Ctrl Pts',(-5.06608371039833,-4.48632197231058,
15.533411916403));
#187396=CARTESIAN_POINT('Ctrl Pts',(-4.95023753425529,-4.61713880389165,
15.5416225722188));
#187397=CARTESIAN_POINT('Ctrl Pts',(-4.82939235263694,-4.74338530551013,
15.5498332280347));
#187398=CARTESIAN_POINT('Ctrl Pts',(-4.7039568591392,-4.86467664571421,
15.5580438838505));
#187399=CARTESIAN_POINT('Ctrl Pts',(-4.57844744954418,-4.98603945996645,
15.566259378007));
#187400=CARTESIAN_POINT('Ctrl Pts',(-4.4483426031316,-5.10244105345704,
15.5744748721634));
#187401=CARTESIAN_POINT('Ctrl Pts',(-4.31408414827224,-5.21353689558501,
15.5826903663198));
#187402=CARTESIAN_POINT('Ctrl Pts',(-4.17961738894967,-5.32480510495633,
15.5909186069665));
#187403=CARTESIAN_POINT('Ctrl Pts',(-4.0409844276511,-5.43075089450466,
15.5991468476133));
#187404=CARTESIAN_POINT('Ctrl Pts',(-3.89865721400434,-5.53107231264354,
15.6073750882601));
#187405=CARTESIAN_POINT('Ctrl Pts',(-3.76930449933599,-5.62224846541956,
15.6148532453695));
#187406=CARTESIAN_POINT('Ctrl Pts',(-3.63690088303125,-5.70877939325665,
15.622331402479));
#187407=CARTESIAN_POINT('Ctrl Pts',(-3.5018174165147,-5.79047180991275,
15.6298095595885));
#187408=CARTESIAN_POINT('Ctrl Pts',(-3.35605553343491,-5.87862205355248,
15.6378788688115));
#187409=CARTESIAN_POINT('Ctrl Pts',(-3.20669577456135,-5.96142638875208,
15.6459481780346));
#187410=CARTESIAN_POINT('Ctrl Pts',(-3.0541751126488,-6.03856799094592,
15.6540174872576));
#187411=CARTESIAN_POINT('Ctrl Pts',(-2.9018446854553,-6.11561337659549,
15.6620767318589));
#187412=CARTESIAN_POINT('Ctrl Pts',(-2.74636152851422,-6.1870099163823,
15.6701359764602));
#187413=CARTESIAN_POINT('Ctrl Pts',(-2.58819214117367,-6.25248354179096,
15.6781952210615));
#187414=CARTESIAN_POINT('Ctrl Pts',(-2.43018532403631,-6.31788987187298,
15.6862461821823));
#187415=CARTESIAN_POINT('Ctrl Pts',(-2.26949811273403,-6.37738526072649,
15.6942971433031));
#187416=CARTESIAN_POINT('Ctrl Pts',(-2.10662211081361,-6.43074119229123,
15.7023481044239));
#187417=CARTESIAN_POINT('Ctrl Pts',(-1.94387782730077,-6.48405397472254,
15.7103925547035));
#187418=CARTESIAN_POINT('Ctrl Pts',(-1.77894862901381,-6.53123706628902,
15.7184370049832));
#187419=CARTESIAN_POINT('Ctrl Pts',(-1.61234653503897,-6.5721098325384,
15.7264814552628));
#187420=CARTESIAN_POINT('Ctrl Pts',(-1.44584270513383,-6.61295849150163,
15.7345211608216));
#187421=CARTESIAN_POINT('Ctrl Pts',(-1.27766830523149,-6.64750414568251,
15.7425608663805));
#187422=CARTESIAN_POINT('Ctrl Pts',(-1.10835086511779,-6.6756158786881,
15.7506005719393));
#187423=CARTESIAN_POINT('Ctrl Pts',(-0.935378798600986,-6.70433438841799,
15.7588138102434));
#187424=CARTESIAN_POINT('Ctrl Pts',(-0.7612141661803,-6.72633794998259,
15.7670270485475));
#187425=CARTESIAN_POINT('Ctrl Pts',(-0.586431261825836,-6.74154191377265,
15.7752402868516));
#187426=CARTESIAN_POINT('Ctrl Pts',(-0.415396318507402,-6.75641985103232,
15.7832774044003));
#187427=CARTESIAN_POINT('Ctrl Pts',(-0.2437697384752,-6.76478682785258,
15.7913145219491));
#187428=CARTESIAN_POINT('Ctrl Pts',(-0.0720951450436325,-6.76661594078319,
15.7993516394978));
#187429=CARTESIAN_POINT('Ctrl Pts',(0.0995976104685821,-6.76844524722232,
15.8073896073225));
#187430=CARTESIAN_POINT('Ctrl Pts',(0.271338015873839,-6.7637353084702,
15.8154275751471));
#187431=CARTESIAN_POINT('Ctrl Pts',(0.442582475717851,-6.75251136631309,
15.8234655429718));
#187432=CARTESIAN_POINT('Ctrl Pts',(0.613878981976963,-6.74128401285758,
15.8315059537801));
#187433=CARTESIAN_POINT('Ctrl Pts',(0.78467887003604,-6.7235387396435,15.8395463645884));
#187434=CARTESIAN_POINT('Ctrl Pts',(0.954443842041111,-6.69935265174105,
15.8475867753967));
#187435=CARTESIAN_POINT('Ctrl Pts',(1.13062497246815,-6.67425246613189,
15.8559310683835));
#187436=CARTESIAN_POINT('Ctrl Pts',(1.30569098949103,-6.64221516367928,
15.8642753613702));
#187437=CARTESIAN_POINT('Ctrl Pts',(1.47905316260374,-6.60338479434539,
15.872619654357));
#187438=CARTESIAN_POINT('Ctrl Pts',(1.6463968468264,-6.56590247079471,15.8806742645731));
#187439=CARTESIAN_POINT('Ctrl Pts',(1.81215266868717,-6.52209099479459,
15.8887288747892));
#187440=CARTESIAN_POINT('Ctrl Pts',(1.97580830523767,-6.47213029387959,
15.8967834850054));
#187441=CARTESIAN_POINT('Ctrl Pts',(2.13958783141684,-6.42213177200825,
15.9048441926752));
#187442=CARTESIAN_POINT('Ctrl Pts',(2.30126365622871,-6.36597487819626,
15.912904900345));
#187443=CARTESIAN_POINT('Ctrl Pts',(2.46034442297168,-6.30388723886715,
15.9209656080148));
#187444=CARTESIAN_POINT('Ctrl Pts',(2.61964948406537,-6.24171205968621,
15.9290376807996));
#187445=CARTESIAN_POINT('Ctrl Pts',(2.77635184768708,-6.173589598907,15.9371097535843));
#187446=CARTESIAN_POINT('Ctrl Pts',(2.92998516313957,-6.09979310663747,
15.945181826369));
#187447=CARTESIAN_POINT('Ctrl Pts',(2.9460770855717,-6.09206348480468,15.9460273146587));
#187448=CARTESIAN_POINT('Ctrl Pts',(2.96213536453561,-6.08427165198964,
15.9468728029483));
#187449=CARTESIAN_POINT('Ctrl Pts',(2.97815948344574,-6.07641794901916,
15.947718291238));
#187450=CARTESIAN_POINT('Ctrl Pts',(3.13608920923335,-5.99901380820487,
15.9560512132847));
#187451=CARTESIAN_POINT('Ctrl Pts',(3.29120217217887,-5.91534937231047,
15.9643841353313));
#187452=CARTESIAN_POINT('Ctrl Pts',(3.44297545180372,-5.82565095403741,
15.972717057378));
#187453=CARTESIAN_POINT('Ctrl Pts',(3.59456937221747,-5.73605853754265,
15.9810401319315));
#187454=CARTESIAN_POINT('Ctrl Pts',(3.74283117444873,-5.64044651910953,
15.989363206485));
#187455=CARTESIAN_POINT('Ctrl Pts',(3.88725988849627,-5.53908833286561,
15.9976862810386));
#187456=CARTESIAN_POINT('Ctrl Pts',(4.03154443354709,-5.43783132254171,
16.0060010474844));
#187457=CARTESIAN_POINT('Ctrl Pts',(4.1720032303848,-5.33083977066663,16.0143158139303));
#187458=CARTESIAN_POINT('Ctrl Pts',(4.30816161806241,-5.21843199367912,
16.0226305803762));
#187459=CARTESIAN_POINT('Ctrl Pts',(4.44420906823032,-5.10611580296157,
16.0309385722157));
#187460=CARTESIAN_POINT('Ctrl Pts',(4.57596282375651,-4.98839240089722,
16.0392465640551));
#187461=CARTESIAN_POINT('Ctrl Pts',(4.70297865677638,-4.86562233983546,
16.0475545558946));
#187462=CARTESIAN_POINT('Ctrl Pts',(4.82991428762037,-4.74292980002278,
16.0558573017816));
#187463=CARTESIAN_POINT('Ctrl Pts',(4.95211770855952,-4.61519719293271,
16.0641600476686));
#187464=CARTESIAN_POINT('Ctrl Pts',(5.06917897636533,-4.48282427779361,
16.0724627935556));
#187465=CARTESIAN_POINT('Ctrl Pts',(5.18619240496172,-4.35050545924621,
16.080762146375));
#187466=CARTESIAN_POINT('Ctrl Pts',(5.29806763756567,-4.21355037148143,
16.0890614991944));
#187467=CARTESIAN_POINT('Ctrl Pts',(5.40443251595799,-4.07239464939929,
16.0973608520137));
#187468=CARTESIAN_POINT('Ctrl Pts',(5.51077477232521,-3.93126894877101,
16.1056584397));
#187469=CARTESIAN_POINT('Ctrl Pts',(5.61160880004059,-3.78594467138048,
16.1139560273863));
#187470=CARTESIAN_POINT('Ctrl Pts',(5.70660342840626,-3.63688964788622,
16.1222536150725));
#187471=CARTESIAN_POINT('Ctrl Pts',(5.80159363876482,-3.48784155663819,
16.1305508168549));
#187472=CARTESIAN_POINT('Ctrl Pts',(5.89074480412844,-3.33506335849959,
16.1388480186372));
#187473=CARTESIAN_POINT('Ctrl Pts',(5.97376960617619,-3.17905106790148,
16.1471452204195));
#187474=CARTESIAN_POINT('Ctrl Pts',(6.05680434296129,-3.02302010889235,
16.155443415044));
#187475=CARTESIAN_POINT('Ctrl Pts',(6.13371109278212,-2.86375459368289,
16.1637416096684));
#187476=CARTESIAN_POINT('Ctrl Pts',(6.20424885240915,-2.7017744497607,16.1720398042929));
#187477=CARTESIAN_POINT('Ctrl Pts',(6.27483622206506,-2.53968038331447,
16.1803438351343));
#187478=CARTESIAN_POINT('Ctrl Pts',(6.33904551176145,-2.37486819250092,
16.1886478659758));
#187479=CARTESIAN_POINT('Ctrl Pts',(6.39668383955284,-2.2078779080383,16.1969518968173));
#187480=CARTESIAN_POINT('Ctrl Pts',(6.45434312622656,-2.04082690131227,
16.205258947233));
#187481=CARTESIAN_POINT('Ctrl Pts',(6.50542658214326,-1.87159655358223,
16.2135659976486));
#187482=CARTESIAN_POINT('Ctrl Pts',(6.54979138952807,-1.70074153052836,
16.2218730480643));
#187483=CARTESIAN_POINT('Ctrl Pts',(6.59420363037961,-1.52970383461893,
16.2301889801188));
#187484=CARTESIAN_POINT('Ctrl Pts',(6.63188278992028,-1.35703833151356,
16.2385049121734));
#187485=CARTESIAN_POINT('Ctrl Pts',(6.66273708283519,-1.18331042630952,
16.246820844228));
#187486=CARTESIAN_POINT('Ctrl Pts',(6.68599570420465,-1.05235064124515,
16.2530895704478));
#187487=CARTESIAN_POINT('Ctrl Pts',(6.70537717616939,-0.920787368008855,
16.2593582966677));
#187488=CARTESIAN_POINT('Ctrl Pts',(6.72086170282644,-0.788864355564967,
16.2656270228876));
#187489=CARTESIAN_POINT('Ctrl Pts',(6.74173490843623,-0.611031592291495,
16.2740772916105));
#187490=CARTESIAN_POINT('Ctrl Pts',(6.75556340138393,-0.432218917407917,
16.2825275603333));
#187491=CARTESIAN_POINT('Ctrl Pts',(6.76226850387909,-0.253009251698049,
16.2909778290562));
#187492=CARTESIAN_POINT('Ctrl Pts',(6.7689676888938,-0.0739577445986757,
16.2994206401303));
#187493=CARTESIAN_POINT('Ctrl Pts',(6.76855600151117,0.105489725193847,
16.3078634512043));
#187494=CARTESIAN_POINT('Ctrl Pts',(6.76100653137315,0.284744943290698,
16.3163062622783));
#187495=CARTESIAN_POINT('Ctrl Pts',(6.75346269601888,0.463866368635023,
16.3247427717956));
#187496=CARTESIAN_POINT('Ctrl Pts',(6.7387917119032,0.642795498124919,16.3331792813128));
#187497=CARTESIAN_POINT('Ctrl Pts',(6.7170187358054,0.820943544246058,16.3416157908301));
#187498=CARTESIAN_POINT('Ctrl Pts',(6.69526133944356,0.998964115854307,
16.3500462635708));
#187499=CARTESIAN_POINT('Ctrl Pts',(6.66641212781071,1.17620439058877,16.3584767363116));
#187500=CARTESIAN_POINT('Ctrl Pts',(6.63054815899308,1.3520799204461,16.3669072090523));
#187501=CARTESIAN_POINT('Ctrl Pts',(6.59469960799836,1.52787984189022,16.3753340575557));
#187502=CARTESIAN_POINT('Ctrl Pts',(6.55184237770201,1.70231586376412,16.3837609060591));
#187503=CARTESIAN_POINT('Ctrl Pts',(6.50210487543775,1.8748123076214,16.3921877545625));
#187504=CARTESIAN_POINT('Ctrl Pts',(6.45238272536407,2.04725550798714,16.4006120019987));
#187505=CARTESIAN_POINT('Ctrl Pts',(6.39578463023035,2.21776000601221,16.4090362494349));
#187506=CARTESIAN_POINT('Ctrl Pts',(6.33248934685054,2.38576354067716,16.4174604968711));
#187507=CARTESIAN_POINT('Ctrl Pts',(6.31465515768734,2.43310050888888,16.4198341274848));
#187508=CARTESIAN_POINT('Ctrl Pts',(6.29628958400892,2.48023902117158,16.4222077580986));
#187509=CARTESIAN_POINT('Ctrl Pts',(6.27739733281748,2.52716673884728,16.4245813887123));
#187510=CARTESIAN_POINT('Ctrl Pts',(6.2087985485342,2.69756381588811,16.43320016965));
#187511=CARTESIAN_POINT('Ctrl Pts',(6.13328276638273,2.86510393147769,16.4418189505877));
#187512=CARTESIAN_POINT('Ctrl Pts',(6.05111893817697,3.02923234434667,16.4504377315255));
#187513=CARTESIAN_POINT('Ctrl Pts',(5.96890575465943,3.19345934815483,16.4590616897125));
#187514=CARTESIAN_POINT('Ctrl Pts',(5.88003669155476,3.35427028728933,16.4676856478995));
#187515=CARTESIAN_POINT('Ctrl Pts',(5.78482645847453,3.51113540686386,16.4763096060865));
#187516=CARTESIAN_POINT('Ctrl Pts',(5.68617660453564,3.67366752797623,16.4852451184573));
#187517=CARTESIAN_POINT('Ctrl Pts',(5.58071906132451,3.83196311045958,16.4941806308282));
#187518=CARTESIAN_POINT('Ctrl Pts',(5.46885222716344,3.98546663735246,16.5031161431991));
#187519=CARTESIAN_POINT('Ctrl Pts',(5.36068399143239,4.13389495220571,16.5117562250943));
#187520=CARTESIAN_POINT('Ctrl Pts',(5.24652372156556,4.27784280467942,16.5203963069895));
#187521=CARTESIAN_POINT('Ctrl Pts',(5.12677230880462,4.41684216309278,16.5290363888848));
#187522=CARTESIAN_POINT('Ctrl Pts',(5.00087890272786,4.56297073284985,16.5381196164935));
#187523=CARTESIAN_POINT('Ctrl Pts',(4.86880602404354,4.70362957665082,16.5472028441022));
#187524=CARTESIAN_POINT('Ctrl Pts',(4.73106322116098,4.8383189019925,16.5562860717109));
#187525=CARTESIAN_POINT('Ctrl Pts',(4.5933204182784,4.9730082273342,16.5653692993196));
#187526=CARTESIAN_POINT('Ctrl Pts',(4.44990800226056,5.10172780024531,16.5744525269283));
#187527=CARTESIAN_POINT('Ctrl Pts',(4.30137593202973,5.22402661663926,16.583535754537));
#187528=CARTESIAN_POINT('Ctrl Pts',(4.15346353630972,5.34581520343023,16.5925810869988));
#187529=CARTESIAN_POINT('Ctrl Pts',(4.00033806783277,5.46134965052688,16.6016264194606));
#187530=CARTESIAN_POINT('Ctrl Pts',(3.84252688496662,5.57021329378945,16.6106717519224));
#187531=CARTESIAN_POINT('Ctrl Pts',(3.6848976564009,5.67895141864648,16.6197066552301));
#187532=CARTESIAN_POINT('Ctrl Pts',(3.52259369810313,5.78103396443803,16.6287415585378));
#187533=CARTESIAN_POINT('Ctrl Pts',(3.35617245869314,5.87608674438266,16.6377764618455));
#187534=CARTESIAN_POINT('Ctrl Pts',(3.27152300636822,5.92443493475067,16.6423720268077));
#187535=CARTESIAN_POINT('Ctrl Pts',(3.18580882221027,5.97096505098928,16.64696759177));
#187536=CARTESIAN_POINT('Ctrl Pts',(3.09910619832134,6.0156321173694,16.6515631567322));
#187537=CARTESIAN_POINT('Origin',(0.,0.,4.30282021618968));
#187538=CARTESIAN_POINT('',(3.09910619832135,6.0156321173694,19.0455979788775));
#187539=CARTESIAN_POINT('',(3.09910619832135,6.0156321173694,18.651395695404));
#187540=CARTESIAN_POINT('',(3.09910619832133,6.0156321173694,4.30282021618968));
#187541=CARTESIAN_POINT('',(-6.76699994441487,0.000867346018274939,17.6971797838443));
#187542=CARTESIAN_POINT('Ctrl Pts',(-6.76699994441487,0.000867346018275612,
17.6971797838443));
#187543=CARTESIAN_POINT('Ctrl Pts',(-6.76702404334501,-0.18715157087484,
17.7059864133287));
#187544=CARTESIAN_POINT('Ctrl Pts',(-6.75920775618406,-0.375012429148591,
17.7147930428132));
#187545=CARTESIAN_POINT('Ctrl Pts',(-6.74361644380036,-0.562073179315164,
17.7235996722976));
#187546=CARTESIAN_POINT('Ctrl Pts',(-6.727845109072,-0.751293793514222,
17.7325079859796));
#187547=CARTESIAN_POINT('Ctrl Pts',(-6.70411814837521,-0.939695425552969,
17.7414162996615));
#187548=CARTESIAN_POINT('Ctrl Pts',(-6.67255619747866,-1.12662451219967,
17.7503246133435));
#187549=CARTESIAN_POINT('Ctrl Pts',(-6.64123700124072,-1.31211585798045,
17.7591644098842));
#187550=CARTESIAN_POINT('Ctrl Pts',(-6.60220304049159,-1.4961569841258,
17.768004206425));
#187551=CARTESIAN_POINT('Ctrl Pts',(-6.55562269889953,-1.67812396135485,
17.7768440029657));
#187552=CARTESIAN_POINT('Ctrl Pts',(-6.50850079192844,-1.86220657388466,
17.7857865752183));
#187553=CARTESIAN_POINT('Ctrl Pts',(-6.45365603276216,-2.04416623577394,
17.7947291474709));
#187554=CARTESIAN_POINT('Ctrl Pts',(-6.3913134435766,-2.22337614135733,
17.8036717197235));
#187555=CARTESIAN_POINT('Ctrl Pts',(-6.32897085439105,-2.4025860469407,
17.812614291976));
#187556=CARTESIAN_POINT('Ctrl Pts',(-6.25913057640139,-2.57904594931731,
17.8215568642286));
#187557=CARTESIAN_POINT('Ctrl Pts',(-6.18206664089352,-2.75215207565852,
17.8304994364812));
#187558=CARTESIAN_POINT('Ctrl Pts',(-6.10924520366856,-2.91572842080022,
17.8389497052045));
#187559=CARTESIAN_POINT('Ctrl Pts',(-6.02986569785643,-3.0765515969184,
17.8473999739279));
#187560=CARTESIAN_POINT('Ctrl Pts',(-5.94415800561399,-3.2340801790146,
17.8558502426512));
#187561=CARTESIAN_POINT('Ctrl Pts',(-5.85852595331781,-3.39146973679255,
17.8642930537257));
#187562=CARTESIAN_POINT('Ctrl Pts',(-5.76657700391438,-3.5455702059956,
17.8727358648002));
#187563=CARTESIAN_POINT('Ctrl Pts',(-5.66858825745251,-3.69586203306773,
17.8811786758748));
#187564=CARTESIAN_POINT('Ctrl Pts',(-5.5706726479638,-3.84604168512263,
17.8896151853925));
#187565=CARTESIAN_POINT('Ctrl Pts',(-5.46672640834872,-3.99241808495695,
17.8980516949103));
#187566=CARTESIAN_POINT('Ctrl Pts',(-5.35707170480776,-4.13449776267301,
17.906488204428));
#187567=CARTESIAN_POINT('Ctrl Pts',(-5.24749546510767,-4.2764757747344,
17.9149186771692));
#187568=CARTESIAN_POINT('Ctrl Pts',(-5.13221911119824,-4.41416293547453,
17.9233491499105));
#187569=CARTESIAN_POINT('Ctrl Pts',(-5.01160722528569,-4.54709599848786,
17.9317796226517));
#187570=CARTESIAN_POINT('Ctrl Pts',(-4.89104719009637,-4.67997191393729,
17.9402064711555));
#187571=CARTESIAN_POINT('Ctrl Pts',(-4.76515641793399,-4.80809756087588,
17.9486333196593));
#187572=CARTESIAN_POINT('Ctrl Pts',(-4.63433917106564,-4.9310434440924,
17.9570601681632));
#187573=CARTESIAN_POINT('Ctrl Pts',(-4.50356230280935,-5.0539513783057,
17.9654844155998));
#187574=CARTESIAN_POINT('Ctrl Pts',(-4.36786223367588,-5.17168251038182,
17.9739086630364));
#187575=CARTESIAN_POINT('Ctrl Pts',(-4.22767967387173,-5.28384458279498,
17.9823329104731));
#187576=CARTESIAN_POINT('Ctrl Pts',(-4.18818159198645,-5.31544756341387,
17.9847065410841));
#187577=CARTESIAN_POINT('Ctrl Pts',(-4.14832785889437,-5.34660865436738,
17.987080171695));
#187578=CARTESIAN_POINT('Ctrl Pts',(-4.10812882024542,-5.37731964795371,
17.989453802306));
#187579=CARTESIAN_POINT('Ctrl Pts',(-3.96216393994695,-5.48883292422435,
17.9980725832432));
#187580=CARTESIAN_POINT('Ctrl Pts',(-3.81170926135031,-5.59435881379705,
18.0066913641804));
#187581=CARTESIAN_POINT('Ctrl Pts',(-3.65727921692777,-5.69355756354744,
18.0153101451176));
#187582=CARTESIAN_POINT('Ctrl Pts',(-3.5027564073157,-5.79281590138417,
18.0239341033042));
#187583=CARTESIAN_POINT('Ctrl Pts',(-3.3442537221211,-5.88573935001357,
18.0325580614908));
#187584=CARTESIAN_POINT('Ctrl Pts',(-3.18231218815861,-5.97203299866111,
18.0411820196773));
#187585=CARTESIAN_POINT('Ctrl Pts',(-3.01452025911462,-6.06144414240245,
18.0501175320485));
#187586=CARTESIAN_POINT('Ctrl Pts',(-2.84303670269073,-6.14373736649845,
18.0590530444196));
#187587=CARTESIAN_POINT('Ctrl Pts',(-2.66848766103472,-6.21863832385398,
18.0679885567907));
#187588=CARTESIAN_POINT('Ctrl Pts',(-2.49970964899563,-6.29106286747998,
18.0766286386854));
#187589=CARTESIAN_POINT('Ctrl Pts',(-2.32806591376774,-6.35657606920946,
18.0852687205801));
#187590=CARTESIAN_POINT('Ctrl Pts',(-2.1541400863151,-6.41498008481168,
18.0939088024748));
#187591=CARTESIAN_POINT('Ctrl Pts',(-1.97129368541882,-6.47637961475592,
18.1029920300841));
#187592=CARTESIAN_POINT('Ctrl Pts',(-1.78592532647418,-6.52992144075028,
18.1120752576934));
#187593=CARTESIAN_POINT('Ctrl Pts',(-1.59872828859884,-6.57543586838423,
18.1211584853027));
#187594=CARTESIAN_POINT('Ctrl Pts',(-1.4115312507235,-6.62095029601817,
18.1302417129121));
#187595=CARTESIAN_POINT('Ctrl Pts',(-1.22250592083238,-6.65843728287001,
18.1393249405214));
#187596=CARTESIAN_POINT('Ctrl Pts',(-1.03235542493084,-6.68778971534063,
18.1484081681307));
#187597=CARTESIAN_POINT('Ctrl Pts',(-0.843013676403518,-6.71701730615583,
18.1574527629905));
#187598=CARTESIAN_POINT('Ctrl Pts',(-0.652381594078926,-6.73820724818045,
18.1664973578504));
#187599=CARTESIAN_POINT('Ctrl Pts',(-0.461125177944495,-6.75127044120332,
18.1755419527102));
#187600=CARTESIAN_POINT('Ctrl Pts',(-0.270044269677354,-6.76432164669032,
18.1845782477305));
#187601=CARTESIAN_POINT('Ctrl Pts',(-0.0783404085832252,-6.76926097605705,
18.1936145427508));
#187602=CARTESIAN_POINT('Ctrl Pts',(0.113315738675922,-6.76605117800393,
18.2026508377712));
#187603=CARTESIAN_POINT('Ctrl Pts',(0.304632735353686,-6.76284705994016,
18.2116711423589));
#187604=CARTESIAN_POINT('Ctrl Pts',(0.495901949248468,-6.75152261437507,
18.2206914469466));
#187605=CARTESIAN_POINT('Ctrl Pts',(0.68645333433179,-6.73209260332809,
18.2297117515343));
#187606=CARTESIAN_POINT('Ctrl Pts',(0.876764756961635,-6.71268706060559,
18.2387206968006));
#187607=CARTESIAN_POINT('Ctrl Pts',(1.06635991882635,-6.68519634689232,
18.247729642067));
#187608=CARTESIAN_POINT('Ctrl Pts',(1.25457193988328,-6.64968707892766,
18.2567385873333));
#187609=CARTESIAN_POINT('Ctrl Pts',(1.44235657128392,-6.61425844499342,
18.2657270751921));
#187610=CARTESIAN_POINT('Ctrl Pts',(1.62876409788658,-6.57084764644693,
18.2747155630509));
#187611=CARTESIAN_POINT('Ctrl Pts',(1.81313637854058,-6.5195724915682,18.2837040509097));
#187612=CARTESIAN_POINT('Ctrl Pts',(1.97489767975534,-6.47458560013447,
18.2915902119249));
#187613=CARTESIAN_POINT('Ctrl Pts',(2.13509227952748,-6.4235457708254,18.2994763729402));
#187614=CARTESIAN_POINT('Ctrl Pts',(2.2932805652048,-6.36656526309548,18.3073625339555));
#187615=CARTESIAN_POINT('Ctrl Pts',(2.45618880411828,-6.30788459576963,
18.3154839988117));
#187616=CARTESIAN_POINT('Ctrl Pts',(2.61689573669985,-6.24292817977151,
18.3236054636678));
#187617=CARTESIAN_POINT('Ctrl Pts',(2.77488605225846,-6.17189568908787,
18.331726928524));
#187618=CARTESIAN_POINT('Ctrl Pts',(2.9328651007826,-6.10086826406613,18.3398478142002));
#187619=CARTESIAN_POINT('Ctrl Pts',(3.0881275841925,-6.02376577761723,18.3479686998764));
#187620=CARTESIAN_POINT('Ctrl Pts',(3.24017923388035,-5.94083559209734,
18.3560895855526));
#187621=CARTESIAN_POINT('Ctrl Pts',(3.39224905808847,-5.85789549404877,
18.3642114419069));
#187622=CARTESIAN_POINT('Ctrl Pts',(3.54110696346878,-5.76912648627449,
18.3723332982612));
#187623=CARTESIAN_POINT('Ctrl Pts',(3.68628434527089,-5.67482129461455,
18.3804551546155));
#187624=CARTESIAN_POINT('Ctrl Pts',(3.83156764669412,-5.58044729905385,
18.3885829365756));
#187625=CARTESIAN_POINT('Ctrl Pts',(3.97316475393407,-5.48052925204528,
18.3967107185358));
#187626=CARTESIAN_POINT('Ctrl Pts',(4.11063654134957,-5.37540288954434,
18.4048385004959));
#187627=CARTESIAN_POINT('Ctrl Pts',(4.24816432966186,-5.27023370247055,
18.4129695934124));
#187628=CARTESIAN_POINT('Ctrl Pts',(4.38156316650945,-5.15985220409469,
18.4211006863288));
#187629=CARTESIAN_POINT('Ctrl Pts',(4.51042817341628,-5.04463345471727,
18.4292317792453));
#187630=CARTESIAN_POINT('Ctrl Pts',(4.63943383109268,-4.92928894889007,
18.4373717469098));
#187631=CARTESIAN_POINT('Ctrl Pts',(4.76389551196001,-4.80909690089357,
18.4455117145744));
#187632=CARTESIAN_POINT('Ctrl Pts',(4.88344573534646,-4.68446867317164,
18.453651682239));
#187633=CARTESIAN_POINT('Ctrl Pts',(4.94544965021429,-4.61983108569663,
18.4578734214194));
#187634=CARTESIAN_POINT('Ctrl Pts',(5.00613308562027,-4.55400075606294,
18.4620951605998));
#187635=CARTESIAN_POINT('Ctrl Pts',(5.06544918373611,-4.48703839597871,
18.4663168997802));
#187636=CARTESIAN_POINT('Ctrl Pts',(5.18403545136421,-4.35316552493365,
18.4747571092379));
#187637=CARTESIAN_POINT('Ctrl Pts',(5.29739924020634,-4.21448946552642,
18.4831973186955));
#187638=CARTESIAN_POINT('Ctrl Pts',(5.40514739632277,-4.07144576582142,
18.4916375281531));
#187639=CARTESIAN_POINT('Ctrl Pts',(5.51281391724793,-3.92851044291105,
18.5000713429017));
#187640=CARTESIAN_POINT('Ctrl Pts',(5.61487308693035,-3.78121434165384,
18.5085051576502));
#187641=CARTESIAN_POINT('Ctrl Pts',(5.71097158788152,-3.63002651814144,
18.5169389723987));
#187642=CARTESIAN_POINT('Ctrl Pts',(5.80701205290538,-3.47893000016915,
18.5253676937873));
#187643=CARTESIAN_POINT('Ctrl Pts',(5.89709884742175,-3.32394672632612,
18.5337964151758));
#187644=CARTESIAN_POINT('Ctrl Pts',(5.98092138447731,-3.16557552313983,
18.5422251365644));
#187645=CARTESIAN_POINT('Ctrl Pts',(6.06470617093795,-3.0072756445322,18.5506500619661));
#187646=CARTESIAN_POINT('Ctrl Pts',(6.14223216933314,-2.8455911731076,18.5590749873678));
#187647=CARTESIAN_POINT('Ctrl Pts',(6.2132340610868,-2.68104671763677,18.5674999127695));
#187648=CARTESIAN_POINT('Ctrl Pts',(6.28421486998781,-2.51655112095579,
18.5759223365272));
#187649=CARTESIAN_POINT('Ctrl Pts',(6.34867530351902,-2.34919753963772,
18.5843447602848));
#187650=CARTESIAN_POINT('Ctrl Pts',(6.40639747157322,-2.17953215994173,
18.5927671840425));
#187651=CARTESIAN_POINT('Ctrl Pts',(6.46412054743138,-2.0098641118965,18.6011897402607));
#187652=CARTESIAN_POINT('Ctrl Pts',(6.51510503239564,-1.83788450632087,
18.6096122964789));
#187653=CARTESIAN_POINT('Ctrl Pts',(6.55918215221633,-1.66415699200729,
18.6180348526971));
#187654=CARTESIAN_POINT('Ctrl Pts',(6.60326076097057,-1.490423609145,18.6264576934308));
#187655=CARTESIAN_POINT('Ctrl Pts',(6.64043145714047,-1.31494252310655,
18.6348805341646));
#187656=CARTESIAN_POINT('Ctrl Pts',(6.6705760365812,-1.13829009491813,18.6433033748983));
#187657=CARTESIAN_POINT('Ctrl Pts',(6.70072584282811,-0.96160703674508,
18.6517276760789));
#187658=CARTESIAN_POINT('Ctrl Pts',(6.72384704737116,-0.783752560304833,
18.6601519772595));
#187659=CARTESIAN_POINT('Ctrl Pts',(6.73987295860478,-0.605311078593489,
18.6685762784401));
#187660=CARTESIAN_POINT('Ctrl Pts',(6.75590388667142,-0.426813736650358,
18.677003216807));
#187661=CARTESIAN_POINT('Ctrl Pts',(6.7648350632393,-0.247729355165734,
18.6854301551738));
#187662=CARTESIAN_POINT('Ctrl Pts',(6.76665181398804,-0.0686456717677405,
18.6938570935406));
#187663=CARTESIAN_POINT('Ctrl Pts',(6.76847019822405,0.110599030371753,
18.7022916087843));
#187664=CARTESIAN_POINT('Ctrl Pts',(6.76316137150845,0.289842699303895,
18.7107261240279));
#187665=CARTESIAN_POINT('Ctrl Pts',(6.75076280115442,0.468498241778733,
18.7191606392716));
#187666=CARTESIAN_POINT('Ctrl Pts',(6.73835824218467,0.647240076411422,
18.7275992284584));
#187667=CARTESIAN_POINT('Ctrl Pts',(6.71885714116907,0.825392886096013,
18.7360378176452));
#187668=CARTESIAN_POINT('Ctrl Pts',(6.69234872533146,1.00237594671579,18.7444764068319));
#187669=CARTESIAN_POINT('Ctrl Pts',(6.6658106790824,1.17955683435537,18.7529244284522));
#187670=CARTESIAN_POINT('Ctrl Pts',(6.63224972462385,1.35556503167329,18.7613724500725));
#187671=CARTESIAN_POINT('Ctrl Pts',(6.59180620945051,1.52983002227362,18.7698204716928));
#187672=CARTESIAN_POINT('Ctrl Pts',(6.56881876447694,1.62887944626843,18.7746221916051));
#187673=CARTESIAN_POINT('Ctrl Pts',(6.54360875772431,1.72736595802387,18.7794239115174));
#187674=CARTESIAN_POINT('Ctrl Pts',(6.51620908773702,1.82518714790935,18.7842256314298));
#187675=CARTESIAN_POINT('Ctrl Pts',(6.46919250666082,1.99304383769265,18.7924651632806));
#187676=CARTESIAN_POINT('Ctrl Pts',(6.41562069152411,2.15931522187927,18.8007046951314));
#187677=CARTESIAN_POINT('Ctrl Pts',(6.3556157227279,2.32345384826425,18.8089442269823));
#187678=CARTESIAN_POINT('Ctrl Pts',(6.29567735525339,2.48741029224537,18.8171746135286));
#187679=CARTESIAN_POINT('Ctrl Pts',(6.22932017288087,2.64923836061656,18.8254050000749));
#187680=CARTESIAN_POINT('Ctrl Pts',(6.15671669937133,2.80840319108247,18.8336353866212));
#187681=CARTESIAN_POINT('Ctrl Pts',(6.08418085885108,2.96741975325275,18.841858106239));
#187682=CARTESIAN_POINT('Ctrl Pts',(6.00541046200375,3.12377769638829,18.8500808258568));
#187683=CARTESIAN_POINT('Ctrl Pts',(5.92062706979467,3.27695958174869,18.8583035454745));
#187684=CARTESIAN_POINT('Ctrl Pts',(5.83591880177912,3.43000573692301,18.8665189791703));
#187685=CARTESIAN_POINT('Ctrl Pts',(5.74520832919491,3.57988113311468,18.8747344128661));
#187686=CARTESIAN_POINT('Ctrl Pts',(5.64876426078085,3.72609062237152,18.8829498465619));
#187687=CARTESIAN_POINT('Ctrl Pts',(5.55236975712871,3.8722249713046,18.8911610581628));
#187688=CARTESIAN_POINT('Ctrl Pts',(5.45024772159885,4.01469686907089,18.8993722697636));
#187689=CARTESIAN_POINT('Ctrl Pts',(5.34271162281037,4.15303762509889,18.9075834813644));
#187690=CARTESIAN_POINT('Ctrl Pts',(5.23521158569582,4.29133198927065,18.915791939378));
#187691=CARTESIAN_POINT('Ctrl Pts',(5.12230132030412,4.42549769075964,18.9240003973915));
#187692=CARTESIAN_POINT('Ctrl Pts',(5.00433641114425,4.55509671511988,18.932208855405));
#187693=CARTESIAN_POINT('Ctrl Pts',(4.95178046825714,4.61283591036879,18.9358659026882));
#187694=CARTESIAN_POINT('Ctrl Pts',(4.89822177462262,4.66966909417137,18.9395229499713));
#187695=CARTESIAN_POINT('Ctrl Pts',(4.84369431543715,4.72555968945498,18.9431799972545));
#187696=CARTESIAN_POINT('Ctrl Pts',(4.71153409293054,4.86102379541277,18.9520437182105));
#187697=CARTESIAN_POINT('Ctrl Pts',(4.57381795780396,4.9908074714394,18.9609074391665));
#187698=CARTESIAN_POINT('Ctrl Pts',(4.43105198088476,5.114495805326,18.9697711601225));
#187699=CARTESIAN_POINT('Ctrl Pts',(4.28806313149874,5.23837722950404,18.9786487182643));
#187700=CARTESIAN_POINT('Ctrl Pts',(4.14000889170728,5.3561441374664,18.9875262764061));
#187701=CARTESIAN_POINT('Ctrl Pts',(3.98742611781988,5.46742370362202,18.996403834548));
#187702=CARTESIAN_POINT('Ctrl Pts',(3.83446239597519,5.57898109749263,19.0053035569719));
#187703=CARTESIAN_POINT('Ctrl Pts',(3.67694773369977,5.68401859646539,19.0142032793958));
#187704=CARTESIAN_POINT('Ctrl Pts',(3.51544806098211,5.78220666619044,19.0231030018197));
#187705=CARTESIAN_POINT('Ctrl Pts',(3.37937896955083,5.86493353004133,19.0306013275056));
#187706=CARTESIAN_POINT('Ctrl Pts',(3.240481567078,5.94279899309329,19.0380996531916));
#187707=CARTESIAN_POINT('Ctrl Pts',(3.09910619832135,6.0156321173694,19.0455979788775));
#187708=CARTESIAN_POINT('Ctrl Pts',(3.09910619832132,6.01563211736941,17.0457499898821));
#187709=CARTESIAN_POINT('Ctrl Pts',(2.94375339480714,6.09566607338664,17.0539481383937));
#187710=CARTESIAN_POINT('Ctrl Pts',(2.78532240288702,6.16966581280104,17.0621462869052));
#187711=CARTESIAN_POINT('Ctrl Pts',(2.62432626980797,6.23740335633313,17.0703444354168));
#187712=CARTESIAN_POINT('Ctrl Pts',(2.46327734983215,6.30516310943417,17.0785452719111));
#187713=CARTESIAN_POINT('Ctrl Pts',(2.29966194389878,6.36665643748943,17.0867461084053));
#187714=CARTESIAN_POINT('Ctrl Pts',(2.1340116865812,6.42170406679838,17.0949469448996));
#187715=CARTESIAN_POINT('Ctrl Pts',(1.96613111823765,6.47749285604629,17.1032581972565));
#187716=CARTESIAN_POINT('Ctrl Pts',(1.79616087133529,6.52666100722362,17.1115694496133));
#187717=CARTESIAN_POINT('Ctrl Pts',(1.62466786371038,6.56907476990685,17.1198807019702));
#187718=CARTESIAN_POINT('Ctrl Pts',(1.45516451230489,6.61099644951404,17.1280955274513));
#187719=CARTESIAN_POINT('Ctrl Pts',(1.28417390863389,6.64631961986173,17.1363103529325));
#187720=CARTESIAN_POINT('Ctrl Pts',(1.11225114611088,6.67496714508581,17.1445251784136));
#187721=CARTESIAN_POINT('Ctrl Pts',(0.937301300133083,6.70411907384759,
17.1528846442083));
#187722=CARTESIAN_POINT('Ctrl Pts',(0.761386555647095,6.7263580488944,17.1612441100031));
#187723=CARTESIAN_POINT('Ctrl Pts',(0.585094191029671,6.74165808889945,
17.1696035757979));
#187724=CARTESIAN_POINT('Ctrl Pts',(0.408801826412231,6.7569581289045,17.1779630415926));
#187725=CARTESIAN_POINT('Ctrl Pts',(0.232132228866702,6.76531927755589,
17.1863225073874));
#187726=CARTESIAN_POINT('Ctrl Pts',(0.0556692259077685,6.76677101262388,
17.1946819731822));
#187727=CARTESIAN_POINT('Ctrl Pts',(-0.114668756466932,6.76817235805198,
17.2027512824047));
#187728=CARTESIAN_POINT('Ctrl Pts',(-0.285371928049203,6.76314019090073,
17.2108205916273));
#187729=CARTESIAN_POINT('Ctrl Pts',(-0.4559028109087,6.75162511007576,17.2188899008498));
#187730=CARTESIAN_POINT('Ctrl Pts',(-0.626220995408382,6.74012439168629,
17.2269491454505));
#187731=CARTESIAN_POINT('Ctrl Pts',(-0.796366951182522,6.72215687333881,
17.2350083900513));
#187732=CARTESIAN_POINT('Ctrl Pts',(-0.965799633635627,6.69772499194087,
17.2430676346521));
#187733=CARTESIAN_POINT('Ctrl Pts',(-1.13505816920609,6.67331822220333,
17.2511185957723));
#187734=CARTESIAN_POINT('Ctrl Pts',(-1.30360452418155,6.64246036435025,
17.2591695568926));
#187735=CARTESIAN_POINT('Ctrl Pts',(-1.47089931757245,6.60520584066575,
17.2672205180128));
#187736=CARTESIAN_POINT('Ctrl Pts',(-1.63805881906315,6.56798144484834,
17.2752649682919));
#187737=CARTESIAN_POINT('Ctrl Pts',(-1.8039684111023,6.52437075988779,17.283309418571));
#187738=CARTESIAN_POINT('Ctrl Pts',(-1.96809559704538,6.47447980311087,
17.29135386885));
#187739=CARTESIAN_POINT('Ctrl Pts',(-2.13212597865205,6.42461827266535,
17.2993935744083));
#187740=CARTESIAN_POINT('Ctrl Pts',(-2.29437569085549,6.36848395257984,
17.3074332799666));
#187741=CARTESIAN_POINT('Ctrl Pts',(-2.45432427650537,6.30623353086106,
17.3154729855249));
#187742=CARTESIAN_POINT('Ctrl Pts',(-2.61772526686236,6.24263946707075,
17.3236862238293));
#187743=CARTESIAN_POINT('Ctrl Pts',(-2.77872427492111,6.17266236142368,
17.3318994621338));
#187744=CARTESIAN_POINT('Ctrl Pts',(-2.93678424587852,6.09652255742237,
17.3401127004382));
#187745=CARTESIAN_POINT('Ctrl Pts',(-3.09145485437162,6.02201545898311,
17.3481498179864));
#187746=CARTESIAN_POINT('Ctrl Pts',(-3.24331085003061,5.94160746277927,
17.3561869355346));
#187747=CARTESIAN_POINT('Ctrl Pts',(-3.39187102761633,5.85555291428717,
17.3642240530828));
#187748=CARTESIAN_POINT('Ctrl Pts',(-3.54044692192388,5.76948926177122,
17.3722620209069));
#187749=CARTESIAN_POINT('Ctrl Pts',(-3.6857259805172,5.67777805470077,17.380299988731));
#187750=CARTESIAN_POINT('Ctrl Pts',(-3.82725363847947,5.58071846510337,
17.3883379565551));
#187751=CARTESIAN_POINT('Ctrl Pts',(-3.96882431101462,5.48362937613566,
17.3963783673629));
#187752=CARTESIAN_POINT('Ctrl Pts',(-4.10664100548792,5.38118888022057,
17.4044187781706));
#187753=CARTESIAN_POINT('Ctrl Pts',(-4.24028018494763,5.2737380436594,17.4124591889784));
#187754=CARTESIAN_POINT('Ctrl Pts',(-4.37897017165631,5.16222617150669,
17.4208034819661));
#187755=CARTESIAN_POINT('Ctrl Pts',(-4.51316035369398,5.04531811311258,
17.4291477749539));
#187756=CARTESIAN_POINT('Ctrl Pts',(-4.64241799654051,4.92343824429603,
17.4374920679417));
#187757=CARTESIAN_POINT('Ctrl Pts',(-4.76718829547796,4.80578959055451,
17.4455466781572));
#187758=CARTESIAN_POINT('Ctrl Pts',(-4.88736258487101,4.68350885586968,
17.4536012883728));
#187759=CARTESIAN_POINT('Ctrl Pts',(-5.00259214754638,4.55701226740803,
17.4616558985883));
#187760=CARTESIAN_POINT('Ctrl Pts',(-5.11790894062829,4.43041991924218,
17.4697166062575));
#187761=CARTESIAN_POINT('Ctrl Pts',(-5.2282733145682,4.29960564627444,17.4777773139268));
#187762=CARTESIAN_POINT('Ctrl Pts',(-5.33337892833046,4.16501599118666,
17.485838021596));
#187763=CARTESIAN_POINT('Ctrl Pts',(-5.43863273471159,4.03023657274805,
17.4939100943802));
#187764=CARTESIAN_POINT('Ctrl Pts',(-5.53861277116244,3.89167145183154,
17.5019821671643));
#187765=CARTESIAN_POINT('Ctrl Pts',(-5.63305748741487,3.74979364011931,
17.5100542399485));
#187766=CARTESIAN_POINT('Ctrl Pts',(-5.64294985387348,3.73493301729684,
17.5108997282429));
#187767=CARTESIAN_POINT('Ctrl Pts',(-5.65278153541568,3.72003607051119,
17.5117452165373));
#187768=CARTESIAN_POINT('Ctrl Pts',(-5.66255226178623,3.70510335652593,
17.5125907048317));
#187769=CARTESIAN_POINT('Ctrl Pts',(-5.76270161227652,3.55204394722865,
17.5212569083792));
#187770=CARTESIAN_POINT('Ctrl Pts',(-5.85673922726422,3.39477230473128,
17.5299231119266));
#187771=CARTESIAN_POINT('Ctrl Pts',(-5.94431510077504,3.23379142535474,
17.538589315474));
#187772=CARTESIAN_POINT('Ctrl Pts',(-6.03176681242811,3.07303877875789,
17.5472432323963));
#187773=CARTESIAN_POINT('Ctrl Pts',(-6.11277490536546,2.90858764615479,
17.5558971493186));
#187774=CARTESIAN_POINT('Ctrl Pts',(-6.18703289001532,2.74096935733852,
17.5645510662408));
#187775=CARTESIAN_POINT('Ctrl Pts',(-6.26119068053347,2.57357723098794,
17.5731933066855));
#187776=CARTESIAN_POINT('Ctrl Pts',(-6.32861640146307,2.40302674588132,
17.5818355471302));
#187777=CARTESIAN_POINT('Ctrl Pts',(-6.38904937959031,2.22987376888396,
17.5904777875749));
#187778=CARTESIAN_POINT('Ctrl Pts',(-6.45122769478795,2.05172004032724,
17.5993696205945));
#187779=CARTESIAN_POINT('Ctrl Pts',(-6.506003115993,1.87081150365074,17.6082614536141));
#187780=CARTESIAN_POINT('Ctrl Pts',(-6.55314366955184,1.68777873141376,
17.6171532866337));
#187781=CARTESIAN_POINT('Ctrl Pts',(-6.59882611067744,1.51040737680431,
17.6257700848626));
#187782=CARTESIAN_POINT('Ctrl Pts',(-6.63733882160785,1.33104155455838,
17.6343868830915));
#187783=CARTESIAN_POINT('Ctrl Pts',(-6.66852001686367,1.15027378683886,
17.6430036813205));
#187784=CARTESIAN_POINT('Ctrl Pts',(-6.70119409496568,0.960851280346185,
17.6520330317354));
#187785=CARTESIAN_POINT('Ctrl Pts',(-6.72581725199615,0.76988958644922,
17.6610623821503));
#187786=CARTESIAN_POINT('Ctrl Pts',(-6.74226255994324,0.578086994134694,
17.6700917325652));
#187787=CARTESIAN_POINT('Ctrl Pts',(-6.75870786789032,0.386284401820168,
17.6791210829802));
#187788=CARTESIAN_POINT('Ctrl Pts',(-6.76697523599835,0.193641289184741,
17.6881504333951));
#187789=CARTESIAN_POINT('Ctrl Pts',(-6.76699994441478,0.000867346750888167,
17.69717978381));
#187790=CARTESIAN_POINT('',(-6.76699928623195,0.00189866213851385,17.3028202161899));
#187791=CARTESIAN_POINT('Ctrl Pts',(3.09910619832134,6.0156321173694,16.6515631567322));
#187792=CARTESIAN_POINT('Ctrl Pts',(2.9290300129029,6.10325119881144,16.6605778338385));
#187793=CARTESIAN_POINT('Ctrl Pts',(2.75514883870212,6.18369867620815,16.6695925109447));
#187794=CARTESIAN_POINT('Ctrl Pts',(2.57805891666819,6.25666854022072,16.6786071880509));
#187795=CARTESIAN_POINT('Ctrl Pts',(2.40120466740917,6.32954129531744,16.6876098683482));
#187796=CARTESIAN_POINT('Ctrl Pts',(2.2211504107763,6.3949562038783,16.6966125486454));
#187797=CARTESIAN_POINT('Ctrl Pts',(2.03851437663987,6.45265434811385,16.7056152289427));
#187798=CARTESIAN_POINT('Ctrl Pts',(1.85627011947858,6.51022872266437,16.7145985973726));
#187799=CARTESIAN_POINT('Ctrl Pts',(1.6714553648832,6.5601192991368,16.7235819658025));
#187800=CARTESIAN_POINT('Ctrl Pts',(1.48470549405131,6.60211622102594,16.7325653342325));
#187801=CARTESIAN_POINT('Ctrl Pts',(1.41593201403153,6.61758222619944,16.7358735962756));
#187802=CARTESIAN_POINT('Ctrl Pts',(1.34689628536527,6.63197817138038,16.7391818583187));
#187803=CARTESIAN_POINT('Ctrl Pts',(1.27763067473933,6.64529524242265,16.7424901203618));
#187804=CARTESIAN_POINT('Ctrl Pts',(1.10759026829054,6.67798736990515,16.7506115852181));
#187805=CARTESIAN_POINT('Ctrl Pts',(0.936239495903021,6.70415924339922,
16.7587330500744));
#187806=CARTESIAN_POINT('Ctrl Pts',(0.764123403043425,6.72371953794337,
16.7668545149307));
#187807=CARTESIAN_POINT('Ctrl Pts',(0.592019584594924,6.74327843755057,
16.7749754006069));
#187808=CARTESIAN_POINT('Ctrl Pts',(0.419150918231919,6.75622665602547,
16.7830962862832));
#187809=CARTESIAN_POINT('Ctrl Pts',(0.246068696353916,6.76252461708456,
16.7912171719595));
#187810=CARTESIAN_POINT('Ctrl Pts',(0.0729657862011396,6.76882333093009,
16.7993390283139));
#187811=CARTESIAN_POINT('Ctrl Pts',(-0.100350364313188,6.76847019242484,
16.8074608846682));
#187812=CARTESIAN_POINT('Ctrl Pts',(-0.273327376901988,6.76147773382682,
16.8155827410226));
#187813=CARTESIAN_POINT('Ctrl Pts',(-0.446430591379407,6.7544801736175,
16.8237105229828));
#187814=CARTESIAN_POINT('Ctrl Pts',(-0.619193807480665,6.7408336334022,
16.8318383049431));
#187815=CARTESIAN_POINT('Ctrl Pts',(-0.791068043069388,6.72060267767961,
16.8399660869034));
#187816=CARTESIAN_POINT('Ctrl Pts',(-0.963012293833378,6.70036348061762,
16.8480971798199));
#187817=CARTESIAN_POINT('Ctrl Pts',(-1.13406648073328,6.67353457827942,
16.8562282727365));
#187818=CARTESIAN_POINT('Ctrl Pts',(-1.30369099925242,6.6402318316809,16.864359365653));
#187819=CARTESIAN_POINT('Ctrl Pts',(-1.47350065584488,6.60689273652619,
16.8724993333177));
#187820=CARTESIAN_POINT('Ctrl Pts',(-1.64187717144924,6.56706576828125,
16.8806393009823));
#187821=CARTESIAN_POINT('Ctrl Pts',(-1.80829457108359,6.52091709379821,
16.888779268647));
#187822=CARTESIAN_POINT('Ctrl Pts',(-1.89460582994727,6.49698239587435,
16.8930010078268));
#187823=CARTESIAN_POINT('Ctrl Pts',(-1.98039038954802,6.47134802511404,
16.8972227470067));
#187824=CARTESIAN_POINT('Ctrl Pts',(-2.06557696693827,6.44404227124979,
16.9014444861866));
#187825=CARTESIAN_POINT('Ctrl Pts',(-2.2358841615612,6.38945190642762,16.9098846956442));
#187826=CARTESIAN_POINT('Ctrl Pts',(-2.40415211785132,6.3280654831791,16.9183249051018));
#187827=CARTESIAN_POINT('Ctrl Pts',(-2.56982043884364,6.26005686173069,
16.9267651145594));
#187828=CARTESIAN_POINT('Ctrl Pts',(-2.73536324153929,6.1920997668884,16.935198929308));
#187829=CARTESIAN_POINT('Ctrl Pts',(-2.89831002782752,6.11753060167729,
16.9436327440565));
#187830=CARTESIAN_POINT('Ctrl Pts',(-3.05811755351506,6.03657237419408,
16.9520665588051));
#187831=CARTESIAN_POINT('Ctrl Pts',(-3.21782856803923,5.95566303910617,
16.9604952801935));
#187832=CARTESIAN_POINT('Ctrl Pts',(-3.37440380490131,5.8683724845296,16.968924001582));
#187833=CARTESIAN_POINT('Ctrl Pts',(-3.52732156913216,5.77497112961918,
16.9773527229705));
#187834=CARTESIAN_POINT('Ctrl Pts',(-3.6801704648151,5.68161183925057,16.9857776483722));
#187835=CARTESIAN_POINT('Ctrl Pts',(-3.82936488805848,5.58214740942622,
16.9942025737739));
#187836=CARTESIAN_POINT('Ctrl Pts',(-3.97440891114378,5.47689353621384,
17.0026274991757));
#187837=CARTESIAN_POINT('Ctrl Pts',(-4.11940986577368,5.37167091642127,
17.0110499229333));
#187838=CARTESIAN_POINT('Ctrl Pts',(-4.26026260829009,5.26066247711803,
17.019472346691));
#187839=CARTESIAN_POINT('Ctrl Pts',(-4.39650098195543,5.14422667809895,
17.0278947704486));
#187840=CARTESIAN_POINT('Ctrl Pts',(-4.53274149825916,5.02778904787912,
17.0363173266668));
#187841=CARTESIAN_POINT('Ctrl Pts',(-4.66436724294385,4.90592409895155,
17.044739882885));
#187842=CARTESIAN_POINT('Ctrl Pts',(-4.79094538165991,4.77903037759247,
17.0531624391032));
#187843=CARTESIAN_POINT('Ctrl Pts',(-4.91752779620949,4.65213236973942,
17.0615852798369));
#187844=CARTESIAN_POINT('Ctrl Pts',(-5.03906202911034,4.5202054867929,17.0700081205706));
#187845=CARTESIAN_POINT('Ctrl Pts',(-5.15515224362191,4.3836850189173,17.0784309613044));
#187846=CARTESIAN_POINT('Ctrl Pts',(-5.27126258716118,4.24714087958678,
17.086855262485));
#187847=CARTESIAN_POINT('Ctrl Pts',(-5.38192681428208,4.1060018214728,17.0952795636656));
#187848=CARTESIAN_POINT('Ctrl Pts',(-5.48678927499912,3.96073635221466,
17.1037038648463));
#187849=CARTESIAN_POINT('Ctrl Pts',(-5.59168456239499,3.81542540831408,
17.1121308032131));
#187850=CARTESIAN_POINT('Ctrl Pts',(-5.69077426719004,3.66598574821698,
17.1205577415798));
#187851=CARTESIAN_POINT('Ctrl Pts',(-5.78374577315878,3.51291528953772,
17.1289846799466));
#187852=CARTESIAN_POINT('Ctrl Pts',(-5.87680087219783,3.35970720127529,
17.1374191951903));
#187853=CARTESIAN_POINT('Ctrl Pts',(-5.96372660715476,3.20286207672421,
17.1458537104339));
#187854=CARTESIAN_POINT('Ctrl Pts',(-6.04425552838593,3.04290389391058,
17.1542882256775));
#187855=CARTESIAN_POINT('Ctrl Pts',(-6.12482334577584,2.8828684499245,17.1627268148643));
#187856=CARTESIAN_POINT('Ctrl Pts',(-6.19898804473388,2.71971725021237,
17.171165404051));
#187857=CARTESIAN_POINT('Ctrl Pts',(-6.26652993601944,2.55399521553432,
17.1796039932378));
#187858=CARTESIAN_POINT('Ctrl Pts',(-6.33414732385861,2.38808794111488,
17.1880520148581));
#187859=CARTESIAN_POINT('Ctrl Pts',(-6.39512699364902,2.21960440168293,
17.1965000364784));
#187860=CARTESIAN_POINT('Ctrl Pts',(-6.44929842583447,2.04910683336157,
17.2049480580986));
#187861=CARTESIAN_POINT('Ctrl Pts',(-6.48008859852863,1.9521987517259,17.2097497780111));
#187862=CARTESIAN_POINT('Ctrl Pts',(-6.50868021828342,1.85464027326941,
17.2145514979236));
#187863=CARTESIAN_POINT('Ctrl Pts',(-6.53504930254438,1.7565362544833,17.2193532178361));
#187864=CARTESIAN_POINT('Ctrl Pts',(-6.58542900941581,1.56910268036138,
17.2285271898738));
#187865=CARTESIAN_POINT('Ctrl Pts',(-6.62778878429327,1.37932214171602,
17.2377011619115));
#187866=CARTESIAN_POINT('Ctrl Pts',(-6.66192816455315,1.18785610674587,
17.2468751339492));
#187867=CARTESIAN_POINT('Ctrl Pts',(-6.69662651964657,0.993255138036172,
17.2561993143226));
#187868=CARTESIAN_POINT('Ctrl Pts',(-6.72283281816732,0.7969131662594,17.2655234946961));
#187869=CARTESIAN_POINT('Ctrl Pts',(-6.74038839512921,0.599544229233806,
17.2748476750695));
#187870=CARTESIAN_POINT('Ctrl Pts',(-6.75794397209109,0.402175292208195,
17.284171855443));
#187871=CARTESIAN_POINT('Ctrl Pts',(-6.7668486980841,0.203779598658603,
17.2934960358164));
#187872=CARTESIAN_POINT('Ctrl Pts',(-6.76699808730845,0.00508786436940122,
17.3028202161899));
#187873=CARTESIAN_POINT('Ctrl Pts',(-6.767,1.1633950350217E-12,17.3028202161899));
#187874=CARTESIAN_POINT('Ctrl Pts',(-6.76700000000003,-0.186007249525797,
17.3115697280011));
#187875=CARTESIAN_POINT('Ctrl Pts',(-6.75932637294526,-0.372014355748932,
17.3203192398123));
#187876=CARTESIAN_POINT('Ctrl Pts',(-6.74400518264188,-0.557389537486598,
17.3290687516235));
#187877=CARTESIAN_POINT('Ctrl Pts',(-6.72868405705094,-0.742763936251031,
17.3378182264791));
#187878=CARTESIAN_POINT('Ctrl Pts',(-6.70571545645734,-0.927506130241638,
17.3465677013348));
#187879=CARTESIAN_POINT('Ctrl Pts',(-6.67517739404809,-1.11098863990111,
17.3553171761905));
#187880=CARTESIAN_POINT('Ctrl Pts',(-6.64463945808678,-1.29447038982072,
17.3640666148175));
#187881=CARTESIAN_POINT('Ctrl Pts',(-6.60653217008321,-1.47669218313838,
17.3728160534445));
#187882=CARTESIAN_POINT('Ctrl Pts',(-6.56098496092631,-1.65703510599469,
17.3815654920716));
#187883=CARTESIAN_POINT('Ctrl Pts',(-6.51543793658245,-1.83737729708882,
17.3903148951967));
#187884=CARTESIAN_POINT('Ctrl Pts',(-6.46245112167364,-2.01584035511107,
17.3990642983219));
#187885=CARTESIAN_POINT('Ctrl Pts',(-6.40220448374192,-2.19181813760969,
17.4078137014471));
#187886=CARTESIAN_POINT('Ctrl Pts',(-6.34195808526437,-2.36779522067322,
17.4165630697972));
#187887=CARTESIAN_POINT('Ctrl Pts',(-6.27445201433031,-2.54128677684345,
17.4253124381473));
#187888=CARTESIAN_POINT('Ctrl Pts',(-6.19991555071823,-2.71170355384991,
17.4340618064974));
#187889=CARTESIAN_POINT('Ctrl Pts',(-6.12537937716609,-2.88211966767653,
17.4428111407991));
#187890=CARTESIAN_POINT('Ctrl Pts',(-6.04381298052433,-3.04946076371958,
17.4515604751009));
#187891=CARTESIAN_POINT('Ctrl Pts',(-5.9554933933574,-3.21315848374716,
17.4603098094027));
#187892=CARTESIAN_POINT('Ctrl Pts',(-5.86717414255315,-3.37685558033655,
17.4690591103829));
#187893=CARTESIAN_POINT('Ctrl Pts',(-5.77210188876502,-3.53690907646913,
17.4778084113631));
#187894=CARTESIAN_POINT('Ctrl Pts',(-5.67059953346898,-3.69277536969437,
17.4865577123433));
#187895=CARTESIAN_POINT('Ctrl Pts',(-5.56909755631284,-3.84864108225068,
17.4953069807285));
#187896=CARTESIAN_POINT('Ctrl Pts',(-5.46116568196749,-4.00031938297655,
17.5040562491138));
#187897=CARTESIAN_POINT('Ctrl Pts',(-5.347170485335,-4.14729511859987,17.5128055174991));
#187898=CARTESIAN_POINT('Ctrl Pts',(-5.23317570391736,-4.29427031888038,
17.5215547540161));
#187899=CARTESIAN_POINT('Ctrl Pts',(-5.11311782003418,-4.43654276189658,
17.5303039905332));
#187900=CARTESIAN_POINT('Ctrl Pts',(-4.98740458984661,-4.57362924351952,
17.5390532270502));
#187901=CARTESIAN_POINT('Ctrl Pts',(-4.86169180711658,-4.71071523720354,
17.5478024324256));
#187902=CARTESIAN_POINT('Ctrl Pts',(-4.73032391204094,-4.84261509523313,
17.5565516378011));
#187903=CARTESIAN_POINT('Ctrl Pts',(-4.5937470701353,-4.96888084538393,
17.5653008431765));
#187904=CARTESIAN_POINT('Ctrl Pts',(-4.45717070301363,-5.09514615659536,
17.574050018137));
#187905=CARTESIAN_POINT('Ctrl Pts',(-4.31538563570945,-5.21577720459607,
17.5827991930974));
#187906=CARTESIAN_POINT('Ctrl Pts',(-4.16887341029399,-5.33036429232972,
17.5915483680579));
#187907=CARTESIAN_POINT('Ctrl Pts',(-4.02236168203613,-5.44495099123684,
17.6002975133299));
#187908=CARTESIAN_POINT('Ctrl Pts',(-3.87112305348091,-5.55349359438653,
17.6090466586019));
#187909=CARTESIAN_POINT('Ctrl Pts',(-3.71567117017705,-5.6556234629893,
17.6177958038739));
#187910=CARTESIAN_POINT('Ctrl Pts',(-3.56021980145756,-5.75775299351683,
17.6265449201841));
#187911=CARTESIAN_POINT('Ctrl Pts',(-3.40055544538278,-5.85346967463914,
17.6352940364942));
#187912=CARTESIAN_POINT('Ctrl Pts',(-3.23722035986775,-5.94244842986944,
17.6440431528044));
#187913=CARTESIAN_POINT('Ctrl Pts',(-3.07388580147109,-6.03142689794565,
17.6527922408793));
#187914=CARTESIAN_POINT('Ctrl Pts',(-2.90688078896514,-6.11366734656812,
17.6615413289541));
#187915=CARTESIAN_POINT('Ctrl Pts',(-2.73677250721314,-6.18889046952379,
17.6702904170289));
#187916=CARTESIAN_POINT('Ctrl Pts',(-2.56666476031418,-6.26411335596354,
17.679039477595));
#187917=CARTESIAN_POINT('Ctrl Pts',(-2.39345402575093,-6.33231884500583,
17.687788538161));
#187918=CARTESIAN_POINT('Ctrl Pts',(-2.21772856065511,-6.39327529762755,
17.696537598727));
#187919=CARTESIAN_POINT('Ctrl Pts',(-2.04200363348415,-6.45423156365143,
17.7052866325107));
#187920=CARTESIAN_POINT('Ctrl Pts',(-1.86376426189162,-6.50793874375692,
17.7140356662944));
#187921=CARTESIAN_POINT('Ctrl Pts',(-1.6836157775302,-6.55421443909576,
17.7227847000781));
#187922=CARTESIAN_POINT('Ctrl Pts',(-1.50346782967657,-6.60048999661901,
17.731533707806));
#187923=CARTESIAN_POINT('Ctrl Pts',(-1.32141105794836,-6.63933404237743,
17.7402827155338));
#187924=CARTESIAN_POINT('Ctrl Pts',(-1.13806375486863,-6.67061465607588,
17.7490317232616));
#187925=CARTESIAN_POINT('Ctrl Pts',(-0.954716982601851,-6.70189517921312,
17.75778070566));
#187926=CARTESIAN_POINT('Ctrl Pts',(-0.770079968901402,-6.72561226592235,
17.7665296880584));
#187927=CARTESIAN_POINT('Ctrl Pts',(-0.584779765557945,-6.74168536983105,
17.7752786704568));
#187928=CARTESIAN_POINT('Ctrl Pts',(-0.391489830651026,-6.75845151013855,
17.7844048894666));
#187929=CARTESIAN_POINT('Ctrl Pts',(-0.197478578238093,-6.76689983031626,
17.7935311084765));
#187930=CARTESIAN_POINT('Ctrl Pts',(-0.00346287645113099,-6.76699911397118,
17.8026573274864));
#187931=CARTESIAN_POINT('Ctrl Pts',(0.184489834654988,-6.76709529501188,
17.8114983521522));
#187932=CARTESIAN_POINT('Ctrl Pts',(0.372446404250464,-6.75935639738162,
17.820339376818));
#187933=CARTESIAN_POINT('Ctrl Pts',(0.55975501948942,-6.74380925873178,
17.8291804014838));
#187934=CARTESIAN_POINT('Ctrl Pts',(0.745134705522872,-6.72842222659793,
17.8379303800935));
#187935=CARTESIAN_POINT('Ctrl Pts',(0.929879431229677,-6.70538706057508,
17.8466803587033));
#187936=CARTESIAN_POINT('Ctrl Pts',(1.11336163626937,-6.67478200894109,
17.855430337313));
#187937=CARTESIAN_POINT('Ctrl Pts',(1.29684196300853,-6.64417727060987,
17.8641802263496));
#187938=CARTESIAN_POINT('Ctrl Pts',(1.47905951217666,-6.60600284890556,
17.8729301153861));
#187939=CARTESIAN_POINT('Ctrl Pts',(1.65939532067261,-6.56038841607186,
17.8816800044226));
#187940=CARTESIAN_POINT('Ctrl Pts',(1.8397293430099,-6.51477443503204,17.8904298067948));
#187941=CARTESIAN_POINT('Ctrl Pts',(2.01818138406464,-6.46172066062079,
17.899179609167));
#187942=CARTESIAN_POINT('Ctrl Pts',(2.1941452835441,-6.40140730423406,17.9079294115391));
#187943=CARTESIAN_POINT('Ctrl Pts',(2.37010749864208,-6.34109452518564,
17.9166791301554));
#187944=CARTESIAN_POINT('Ctrl Pts',(2.54358134866666,-6.2735223961642,17.9254288487718));
#187945=CARTESIAN_POINT('Ctrl Pts',(2.7139775943576,-6.19892043966729,17.9341785673881));
#187946=CARTESIAN_POINT('Ctrl Pts',(2.88437226558316,-6.12431917249424,
17.9429282051568));
#187947=CARTESIAN_POINT('Ctrl Pts',(3.05168912681136,-6.04268832278707,
17.9516778429255));
#187948=CARTESIAN_POINT('Ctrl Pts',(3.21535986274024,-5.95430516123243,
17.9604274806942));
#187949=CARTESIAN_POINT('Ctrl Pts',(3.37902914073013,-5.86592278697342,
17.9691770405233));
#187950=CARTESIAN_POINT('Ctrl Pts',(3.53905210621745,-5.77078835741835,
17.9779266003523));
#187951=CARTESIAN_POINT('Ctrl Pts',(3.69488522831872,-5.66922500431515,
17.9866761601814));
#187952=CARTESIAN_POINT('Ctrl Pts',(3.85071701407118,-5.5676625221697,17.9954256449785));
#187953=CARTESIAN_POINT('Ctrl Pts',(4.00235878822585,-5.45967138329237,
18.0041751297756));
#187954=CARTESIAN_POINT('Ctrl Pts',(4.14929549611509,-5.34561838199464,
18.0129246145728));
#187955=CARTESIAN_POINT('Ctrl Pts',(4.2962309927627,-5.23156632086868,18.0216740272453));
#187956=CARTESIAN_POINT('Ctrl Pts',(4.43846127436203,-5.11145267304811,
18.0304234399179));
#187957=CARTESIAN_POINT('Ctrl Pts',(4.57550326054613,-4.98568540049728,
18.0391728525905));
#187958=CARTESIAN_POINT('Ctrl Pts',(4.71254416257948,-4.85991912290199,
18.0479221960458));
#187959=CARTESIAN_POINT('Ctrl Pts',(4.84439664018924,-4.72849950385252,
18.056671539501));
#187960=CARTESIAN_POINT('Ctrl Pts',(4.97061286794903,-4.59187289860897,
18.0654208829563));
#187961=CARTESIAN_POINT('Ctrl Pts',(5.09682813912833,-4.45524732884515,
18.0741701601011));
#187962=CARTESIAN_POINT('Ctrl Pts',(5.21740705147979,-4.31341506235618,
18.0829194372459));
#187963=CARTESIAN_POINT('Ctrl Pts',(5.33194007545827,-4.16685781275556,
18.0916687143907));
#187964=CARTESIAN_POINT('Ctrl Pts',(5.44647226944609,-4.02030162521673,
18.1004179281319));
#187965=CARTESIAN_POINT('Ctrl Pts',(5.5549584862823,-3.86902074887766,18.109167141873));
#187966=CARTESIAN_POINT('Ctrl Pts',(5.65703027291897,-3.71352898080495,
18.1179163556141));
#187967=CARTESIAN_POINT('Ctrl Pts',(5.75910135377104,-3.55803828789415,
18.126665508858));
#187968=CARTESIAN_POINT('Ctrl Pts',(5.85475793592856,-3.39833700106534,
18.1354146621019));
#187969=CARTESIAN_POINT('Ctrl Pts',(5.94367514427499,-3.23496750823369,
18.1441638153458));
#187970=CARTESIAN_POINT('Ctrl Pts',(6.03259176732734,-3.0715990907754,18.1529129109987));
#187971=CARTESIAN_POINT('Ctrl Pts',(6.11476896836012,-2.90456276731249,
18.1616620066516));
#187972=CARTESIAN_POINT('Ctrl Pts',(6.18992765547968,-2.73442583002864,
18.1704111023045));
#187973=CARTESIAN_POINT('Ctrl Pts',(6.26508587283129,-2.56428995615988,
18.1791601432726));
#187974=CARTESIAN_POINT('Ctrl Pts',(6.33322554827227,-2.39105376935023,
18.1879091842406));
#187975=CARTESIAN_POINT('Ctrl Pts',(6.39411526733091,-2.21530561053905,
18.1966582252086));
#187976=CARTESIAN_POINT('Ctrl Pts',(6.45500462602902,-2.03955849184926,
18.2054072143977));
#187977=CARTESIAN_POINT('Ctrl Pts',(6.50864402040789,-1.86129970164375,
18.2141562035867));
#187978=CARTESIAN_POINT('Ctrl Pts',(6.55485128368644,-1.68113463135892,
18.2229051927757));
#187979=CARTESIAN_POINT('Ctrl Pts',(6.6019980955436,-1.49730620116719,18.2318320782471));
#187980=CARTESIAN_POINT('Ctrl Pts',(6.64140720707899,-1.31149343245565,
18.2407589637186));
#187981=CARTESIAN_POINT('Ctrl Pts',(6.67293928722903,-1.12435326697408,
18.24968584919));
#187982=CARTESIAN_POINT('Ctrl Pts',(6.70384625876272,-0.940923067005458,
18.2584357633674));
#187983=CARTESIAN_POINT('Ctrl Pts',(6.72718554579808,-0.756217899520573,
18.2671856775449));
#187984=CARTESIAN_POINT('Ctrl Pts',(6.74287786815337,-0.570865181253446,
18.2759355917224));
#187985=CARTESIAN_POINT('Ctrl Pts',(6.75856988190852,-0.385516108072936,
18.2846853338269));
#187986=CARTESIAN_POINT('Ctrl Pts',(6.76661520773406,-0.199519795225378,
18.2934350759313));
#187987=CARTESIAN_POINT('Ctrl Pts',(6.76698651789579,-0.0135080204547203,
18.3021848180358));
#187988=CARTESIAN_POINT('Ctrl Pts',(6.767357821249,0.172500343513846,18.3109343997008));
#187989=CARTESIAN_POINT('Ctrl Pts',(6.76005538995179,0.358523882211763,
18.3196839813658));
#187990=CARTESIAN_POINT('Ctrl Pts',(6.74510402742355,0.543930748565174,
18.3284335630307));
#187991=CARTESIAN_POINT('Ctrl Pts',(6.73015291918022,0.729334461615976,
18.3371829958874));
#187992=CARTESIAN_POINT('Ctrl Pts',(6.70755316306585,0.914121237635365,
18.3459324287441));
#187993=CARTESIAN_POINT('Ctrl Pts',(6.67738151874564,1.09766345166185,18.3546818616008));
#187994=CARTESIAN_POINT('Ctrl Pts',(6.64721034747557,1.28120278799726,18.3634311572783));
#187995=CARTESIAN_POINT('Ctrl Pts',(6.60946757205128,1.4634973186039,18.3721804529558));
#187996=CARTESIAN_POINT('Ctrl Pts',(6.56428138111508,1.64392790278223,18.3809297486333));
#187997=CARTESIAN_POINT('Ctrl Pts',(6.51909583859835,1.8243558977911,18.3896789187589));
#187998=CARTESIAN_POINT('Ctrl Pts',(6.4664671639286,2.00291972192313,18.3984280888845));
#187999=CARTESIAN_POINT('Ctrl Pts',(6.40657409872869,2.17901292274706,18.4071772590101));
#188000=CARTESIAN_POINT('Ctrl Pts',(6.34668181342065,2.35510383059007,18.4159263152092));
#188001=CARTESIAN_POINT('Ctrl Pts',(6.27952541914042,2.52872390822599,18.4246753714083));
#188002=CARTESIAN_POINT('Ctrl Pts',(6.20533299175513,2.69928350890293,18.4334244276074));
#188003=CARTESIAN_POINT('Ctrl Pts',(6.12831602991544,2.87633637965634,18.4425065637656));
#188004=CARTESIAN_POINT('Ctrl Pts',(6.04371690605263,3.05009086601475,18.4515886999238));
#188005=CARTESIAN_POINT('Ctrl Pts',(5.95184520316622,3.2199111288275,18.460670836082));
#188006=CARTESIAN_POINT('Ctrl Pts',(5.86333549509262,3.3835169118304,18.4694206164256));
#188007=CARTESIAN_POINT('Ctrl Pts',(5.76807618099351,3.54347103712033,18.4781703967692));
#188008=CARTESIAN_POINT('Ctrl Pts',(5.66639083308993,3.6992301802773,18.4869201771127));
#188009=CARTESIAN_POINT('Ctrl Pts',(5.56470914082176,3.85498372382086,18.4956696428977));
#188010=CARTESIAN_POINT('Ctrl Pts',(5.4566020337204,4.00654234702035,18.5044191086826));
#188011=CARTESIAN_POINT('Ctrl Pts',(5.34243669839187,4.15339127986707,18.5131685744675));
#188012=CARTESIAN_POINT('Ctrl Pts',(5.2282748605056,4.30023571401317,18.5219177722135));
#188013=CARTESIAN_POINT('Ctrl Pts',(5.10805534167078,4.44237052028507,18.5306669699595));
#188014=CARTESIAN_POINT('Ctrl Pts',(4.98218644339917,4.57931296628758,18.5394161677055));
#188015=CARTESIAN_POINT('Ctrl Pts',(4.85632073219553,4.71625194483394,18.5481651439171));
#188016=CARTESIAN_POINT('Ctrl Pts',(4.72480612170287,4.84799861524539,18.5569141201288));
#188017=CARTESIAN_POINT('Ctrl Pts',(4.58808925235281,4.97410554898513,18.5656630963404));
#188018=CARTESIAN_POINT('Ctrl Pts',(4.4513634947402,5.10022068121231,18.5744126413421));
#188019=CARTESIAN_POINT('Ctrl Pts',(4.30943501210053,5.22069514871856,18.5831621863438));
#188020=CARTESIAN_POINT('Ctrl Pts',(4.16278587431757,5.33511975166276,18.5919117313455));
#188021=CARTESIAN_POINT('Ctrl Pts',(4.01614535740402,5.44953762807877,18.6006607619993));
#188022=CARTESIAN_POINT('Ctrl Pts',(3.86478496657856,5.55790617532831,18.609409792653));
#188023=CARTESIAN_POINT('Ctrl Pts',(3.70921874747106,5.65985735539415,18.6181588233067));
#188024=CARTESIAN_POINT('Ctrl Pts',(3.5536504160581,5.76180991977102,18.6269079727564));
#188025=CARTESIAN_POINT('Ctrl Pts',(3.39387638174431,5.85734478552866,18.635657122206));
#188026=CARTESIAN_POINT('Ctrl Pts',(3.23043927904447,5.94613749121282,18.6444062716556));
#188027=CARTESIAN_POINT('Ctrl Pts',(3.18691767070367,5.96978206944181,18.6467360795717));
#188028=CARTESIAN_POINT('Ctrl Pts',(3.14313645919597,5.99294880633443,18.6490658874879));
#188029=CARTESIAN_POINT('Ctrl Pts',(3.09910619832135,6.0156321173694,18.651395695404));
#188030=CARTESIAN_POINT('Origin',(0.,0.,4.30282021618968));
#188031=CARTESIAN_POINT('',(3.09910619832133,6.01563211736941,21.0459783413229));
#188032=CARTESIAN_POINT('',(3.09910619832131,6.01563211736942,20.6513174420499));
#188033=CARTESIAN_POINT('',(3.09910619832133,6.0156321173694,4.30282021618968));
#188034=CARTESIAN_POINT('',(-6.76699485396139,-0.00834544546909593,19.6971797837639));
#188035=CARTESIAN_POINT('Ctrl Pts',(-6.76699485396019,-0.00834544644487561,
19.69717978381));
#188036=CARTESIAN_POINT('Ctrl Pts',(-6.76663983601997,-0.296215555059323,
19.7107704646661));
#188037=CARTESIAN_POINT('Ctrl Pts',(-6.74791479279641,-0.583282457482189,
19.7243611455222));
#188038=CARTESIAN_POINT('Ctrl Pts',(-6.71113050647912,-0.867765132397808,
19.7379518263783));
#188039=CARTESIAN_POINT('Ctrl Pts',(-6.68857677325034,-1.04219141602641,
19.746284748425));
#188040=CARTESIAN_POINT('Ctrl Pts',(-6.65918964291552,-1.21596185562541,
19.7546176704717));
#188041=CARTESIAN_POINT('Ctrl Pts',(-6.62301540300872,-1.38850854210884,
19.7629505925184));
#188042=CARTESIAN_POINT('Ctrl Pts',(-6.58688391228112,-1.56085132025203,
19.771273667072));
#188043=CARTESIAN_POINT('Ctrl Pts',(-6.54398136066317,-1.73197288854462,
19.7795967416257));
#188044=CARTESIAN_POINT('Ctrl Pts',(-6.49440571141654,-1.9013109833797,
19.7879198161793));
#188045=CARTESIAN_POINT('Ctrl Pts',(-6.44487954867015,-2.07048004463076,
19.7962345826252));
#188046=CARTESIAN_POINT('Ctrl Pts',(-6.38869365649649,-2.23786884743151,
19.8045493490712));
#188047=CARTESIAN_POINT('Ctrl Pts',(-6.32599695399928,-2.40292562057002,
19.8128641155172));
#188048=CARTESIAN_POINT('Ctrl Pts',(-6.263351334775,-2.56784791071574,19.8211721073567));
#188049=CARTESIAN_POINT('Ctrl Pts',(-6.1942055985028,-2.73044163336407,
19.8294800991962));
#188050=CARTESIAN_POINT('Ctrl Pts',(-6.11875843919035,-2.89017026537138,
19.8377880910357));
#188051=CARTESIAN_POINT('Ctrl Pts',(-6.04335891981515,-3.04979803921418,
19.8460908369228));
#188052=CARTESIAN_POINT('Ctrl Pts',(-5.96166605513343,-3.20656401404263,
19.8543935828099));
#188053=CARTESIAN_POINT('Ctrl Pts',(-5.87392668322694,-3.35995153537586,
19.862696328697));
#188054=CARTESIAN_POINT('Ctrl Pts',(-5.78622316760571,-3.5132763721172,
19.8709956815165));
#188055=CARTESIAN_POINT('Ctrl Pts',(-5.69247824091975,-3.66322520490996,
19.8792950343359));
#188056=CARTESIAN_POINT('Ctrl Pts',(-5.59298485550267,-3.80930563306724,
19.8875943871553));
#188057=CARTESIAN_POINT('Ctrl Pts',(-5.49351263065923,-3.95535499236859,
19.8958919748417));
#188058=CARTESIAN_POINT('Ctrl Pts',(-5.38829457851184,-4.09753729874758,
19.904189562528));
#188059=CARTESIAN_POINT('Ctrl Pts',(-5.27766730990099,-4.23538862042227,
19.9124871502144));
#188060=CARTESIAN_POINT('Ctrl Pts',(-5.16704518633951,-4.37323353091222,
19.9207843519968));
#188061=CARTESIAN_POINT('Ctrl Pts',(-5.05101456549176,-4.50674758687055,
19.9290815537792));
#188062=CARTESIAN_POINT('Ctrl Pts',(-4.92995283800137,-4.63549932748159,
19.9373787555616));
#188063=CARTESIAN_POINT('Ctrl Pts',(-4.80887662427978,-4.76426647450985,
19.9456769501861));
#188064=CARTESIAN_POINT('Ctrl Pts',(-4.68276834305796,-4.88826991765115,
19.9539751448107));
#188065=CARTESIAN_POINT('Ctrl Pts',(-4.55204291185383,-5.00711437143604,
19.9622733394352));
#188066=CARTESIAN_POINT('Ctrl Pts',(-4.42122553992976,-5.12604240991092,
19.9705773702768));
#188067=CARTESIAN_POINT('Ctrl Pts',(-4.28578478702871,-5.23980397450223,
19.9788814011184));
#188068=CARTESIAN_POINT('Ctrl Pts',(-4.14617007011083,-5.34804288966694,
19.9871854319599));
#188069=CARTESIAN_POINT('Ctrl Pts',(-4.00650458543936,-5.4563211634802,
19.9954924823757));
#188070=CARTESIAN_POINT('Ctrl Pts',(-3.8626623910893,-5.55907257800273,
20.0037995327914));
#188071=CARTESIAN_POINT('Ctrl Pts',(-3.71512284945592,-5.6559836645318,
20.0121065832071));
#188072=CARTESIAN_POINT('Ctrl Pts',(-3.56742556315202,-5.75299836536822,
20.0204225152618));
#188073=CARTESIAN_POINT('Ctrl Pts',(-3.41602332625222,-5.84416007711451,
20.0287384473164));
#188074=CARTESIAN_POINT('Ctrl Pts',(-3.2614220687476,-5.92920020656126,
20.037054379371));
#188075=CARTESIAN_POINT('Ctrl Pts',(-3.14488035700249,-5.99330526244966,
20.04332310559));
#188076=CARTESIAN_POINT('Ctrl Pts',(-3.02652135922019,-6.05393268165057,
20.0495918318089));
#188077=CARTESIAN_POINT('Ctrl Pts',(-2.90656953784754,-6.1109853969435,
20.0558605580279));
#188078=CARTESIAN_POINT('Ctrl Pts',(-2.74487398933406,-6.18789269178828,
20.0643108267512));
#188079=CARTESIAN_POINT('Ctrl Pts',(-2.57998689571232,-6.25844371075106,
20.0727610954746));
#188080=CARTESIAN_POINT('Ctrl Pts',(-2.4124349855146,-6.32237664495443,
20.0812113641979));
#188081=CARTESIAN_POINT('Ctrl Pts',(-2.24503094556222,-6.38625315617428,
20.0896541752724));
#188082=CARTESIAN_POINT('Ctrl Pts',(-2.07496708493001,-6.44352310651362,
20.0980969863469));
#188083=CARTESIAN_POINT('Ctrl Pts',(-1.90279177887941,-6.49397200842666,
20.1065397974214));
#188084=CARTESIAN_POINT('Ctrl Pts',(-1.73074498126691,-6.54438325621996,
20.1149763069391));
#188085=CARTESIAN_POINT('Ctrl Pts',(-1.55659019695295,-6.5879835114835,
20.1234128164569));
#188086=CARTESIAN_POINT('Ctrl Pts',(-1.38089307407099,-6.62460740859281,
20.1318493259746));
#188087=CARTESIAN_POINT('Ctrl Pts',(-1.20532167193471,-6.66120509933301,
20.1402797987158));
#188088=CARTESIAN_POINT('Ctrl Pts',(-1.02821045640877,-6.69083632168633,
20.1487102714571));
#188089=CARTESIAN_POINT('Ctrl Pts',(-0.850137643089211,-6.71338625343446,
20.1571407441983));
#188090=CARTESIAN_POINT('Ctrl Pts',(-0.672141382789677,-6.73592649102801,
20.1655675927021));
#188091=CARTESIAN_POINT('Ctrl Pts',(-0.493184677152069,-6.75139146520927,
20.1739944412059));
#188092=CARTESIAN_POINT('Ctrl Pts',(-0.313853936722314,-6.75971779783771,
20.1824212897097));
#188093=CARTESIAN_POINT('Ctrl Pts',(-0.134578549287333,-6.76804156042465,
20.1908455371464));
#188094=CARTESIAN_POINT('Ctrl Pts',(0.0450703118637604,-6.76923106028667,
20.199269784583));
#188095=CARTESIAN_POINT('Ctrl Pts',(0.224502763877788,-6.76327491005735,
20.2076940320197));
#188096=CARTESIAN_POINT('Ctrl Pts',(0.275059963663833,-6.76159669480855,
20.2100676626307));
#188097=CARTESIAN_POINT('Ctrl Pts',(0.325599975128035,-6.75935150617513,
20.2124412932416));
#188098=CARTESIAN_POINT('Ctrl Pts',(0.376109601451067,-6.75653983690589,
20.2148149238526));
#188099=CARTESIAN_POINT('Ctrl Pts',(0.559512782420949,-6.74633051394407,
20.2234337047898));
#188100=CARTESIAN_POINT('Ctrl Pts',(0.742433063246356,-6.72865299871907,
20.232052485727));
#188101=CARTESIAN_POINT('Ctrl Pts',(0.92425870073124,-6.70358373216316,
20.2406712666643));
#188102=CARTESIAN_POINT('Ctrl Pts',(1.10619355977141,-6.67849940665122,
20.2492952248508));
#188103=CARTESIAN_POINT('Ctrl Pts',(1.28703216188696,-6.64601451010209,
20.2579191830374));
#188104=CARTESIAN_POINT('Ctrl Pts',(1.46617172243524,-6.60625684335171,
20.2665431412239));
#188105=CARTESIAN_POINT('Ctrl Pts',(1.65178298408685,-6.56506286775372,
20.2754786535951));
#188106=CARTESIAN_POINT('Ctrl Pts',(1.83556980291674,-6.51606092819704,
20.2844141659662));
#188107=CARTESIAN_POINT('Ctrl Pts',(2.01687810760223,-6.45944979847935,
20.2933496783373));
#188108=CARTESIAN_POINT('Ctrl Pts',(2.19219190446229,-6.40471037486297,
20.301989760232));
#188109=CARTESIAN_POINT('Ctrl Pts',(2.36518818459376,-6.34285701194278,
20.3106298421267));
#188110=CARTESIAN_POINT('Ctrl Pts',(2.53529492169012,-6.27411895488541,
20.3192699240214));
#188111=CARTESIAN_POINT('Ctrl Pts',(2.71412635289166,-6.20185535538658,
20.3283531516307));
#188112=CARTESIAN_POINT('Ctrl Pts',(2.88976369075558,-6.12198244898684,
20.3374363792401));
#188113=CARTESIAN_POINT('Ctrl Pts',(3.06156991882546,-6.03482217071415,
20.3465196068494));
#188114=CARTESIAN_POINT('Ctrl Pts',(3.23337614689534,-5.94766189244147,
20.3556028344587));
#188115=CARTESIAN_POINT('Ctrl Pts',(3.40135094365678,-5.85321446168417,
20.3646860620681));
#188116=CARTESIAN_POINT('Ctrl Pts',(3.56489050922797,-5.7518557576852,20.3737692896774));
#188117=CARTESIAN_POINT('Ctrl Pts',(3.72773450893392,-5.65092815214488,
20.3828138845372));
#188118=CARTESIAN_POINT('Ctrl Pts',(3.88633176894871,-5.54305547919057,
20.391858479397));
#188119=CARTESIAN_POINT('Ctrl Pts',(4.04011840715542,-5.42860315883966,
20.4009030742569));
#188120=CARTESIAN_POINT('Ctrl Pts',(4.19376392191441,-5.31425586650832,
20.4099393692772));
#188121=CARTESIAN_POINT('Ctrl Pts',(4.34260743776402,-5.19334112330998,
20.4189756642976));
#188122=CARTESIAN_POINT('Ctrl Pts',(4.48611524534255,-5.06626677204282,
20.4280119593179));
#188123=CARTESIAN_POINT('Ctrl Pts',(4.62936910460195,-4.93941728880516,
20.4370322639056));
#188124=CARTESIAN_POINT('Ctrl Pts',(4.76730593209654,-4.80643012073239,
20.4460525684933));
#188125=CARTESIAN_POINT('Ctrl Pts',(4.89942631473796,-4.66775221990769,
20.455072873081));
#188126=CARTESIAN_POINT('Ctrl Pts',(5.03138031742258,-4.52924895696012,
20.4640818183473));
#188127=CARTESIAN_POINT('Ctrl Pts',(5.15753232919754,-4.38506943460008,
20.4730907636137));
#188128=CARTESIAN_POINT('Ctrl Pts',(5.27741906373368,-4.23569793844419,
20.48209970888));
#188129=CARTESIAN_POINT('Ctrl Pts',(5.39703356087553,-4.08666563333435,
20.4910881967388));
#188130=CARTESIAN_POINT('Ctrl Pts',(5.51041103070356,-3.93246507321833,
20.5000766845976));
#188131=CARTESIAN_POINT('Ctrl Pts',(5.61712811593769,-3.77361374933131,
20.5090651724564));
#188132=CARTESIAN_POINT('Ctrl Pts',(5.71075767081434,-3.63424357524459,
20.5169513334716));
#188133=CARTESIAN_POINT('Ctrl Pts',(5.79926076377863,-3.49129401593223,
20.5248374944869));
#188134=CARTESIAN_POINT('Ctrl Pts',(5.88237643834799,-3.34513623602514,
20.5327236555021));
#188135=CARTESIAN_POINT('Ctrl Pts',(5.9679720822497,-3.19461746387762,20.5408451203583));
#188136=CARTESIAN_POINT('Ctrl Pts',(6.04781427862262,-3.04076273422171,
20.5489665852145));
#188137=CARTESIAN_POINT('Ctrl Pts',(6.12164141212632,-2.88405884498567,
20.5570880500707));
#188138=CARTESIAN_POINT('Ctrl Pts',(6.19546328066884,-2.72736613104327,
20.5652089357469));
#188139=CARTESIAN_POINT('Ctrl Pts',(6.26327078470796,-2.56782499350459,
20.5733298214231));
#188140=CARTESIAN_POINT('Ctrl Pts',(6.32484930615309,-2.40594477377492,
20.5814507070993));
#188141=CARTESIAN_POINT('Ctrl Pts',(6.38643518799235,-2.24404520473005,
20.5895725634535));
#188142=CARTESIAN_POINT('Ctrl Pts',(6.44179047561554,-2.07980633945318,
20.5976944198078));
#188143=CARTESIAN_POINT('Ctrl Pts',(6.49074954730195,-1.91375529109643,
20.605816276162));
#188144=CARTESIAN_POINT('Ctrl Pts',(6.53974433892135,-1.74758309394911,
20.6139440581222));
#188145=CARTESIAN_POINT('Ctrl Pts',(6.58233349046603,-1.57959642463423,
20.6220718400824));
#188146=CARTESIAN_POINT('Ctrl Pts',(6.61840174449271,-1.41033589917293,
20.6301996220426));
#188147=CARTESIAN_POINT('Ctrl Pts',(6.65448469138549,-1.24100642326463,
20.638330714959));
#188148=CARTESIAN_POINT('Ctrl Pts',(6.68404138340067,-1.07040241741154,
20.6464618078755));
#188149=CARTESIAN_POINT('Ctrl Pts',(6.70700815262058,-0.899072099823535,
20.6545929007919));
#188150=CARTESIAN_POINT('Ctrl Pts',(6.72999998910926,-0.727554782354139,
20.6627328684565));
#188151=CARTESIAN_POINT('Ctrl Pts',(6.74638750209217,-0.555309933885106,
20.670872836121));
#188152=CARTESIAN_POINT('Ctrl Pts',(6.75615904125024,-0.382889030049986,
20.6790128037856));
#188153=CARTESIAN_POINT('Ctrl Pts',(6.76122698395185,-0.293464094319782,
20.683234542966));
#188154=CARTESIAN_POINT('Ctrl Pts',(6.76451614724316,-0.203991791134683,
20.6874562821465));
#188155=CARTESIAN_POINT('Ctrl Pts',(6.76603041614926,-0.114548713406617,
20.6916780213269));
#188156=CARTESIAN_POINT('Ctrl Pts',(6.76905778145923,0.0642681860494812,
20.7001182307845));
#188157=CARTESIAN_POINT('Ctrl Pts',(6.76499423030045,0.243337685477338,
20.7085584402422));
#188158=CARTESIAN_POINT('Ctrl Pts',(6.75382433733469,0.422073240594176,
20.7169986496998));
#188159=CARTESIAN_POINT('Ctrl Pts',(6.74266290721768,0.600673377048167,
20.7254324644483));
#188160=CARTESIAN_POINT('Ctrl Pts',(6.72440588887434,0.77893974191567,20.7338662791969));
#188161=CARTESIAN_POINT('Ctrl Pts',(6.69908991008622,0.956286241969934,
20.7423000939454));
#188162=CARTESIAN_POINT('Ctrl Pts',(6.67378922015581,1.1335256387032,20.7507288153339));
#188163=CARTESIAN_POINT('Ctrl Pts',(6.64143811580303,1.30984594883357,20.7591575367225));
#188164=CARTESIAN_POINT('Ctrl Pts',(6.60212504588006,1.48466625157417,20.767586258111));
#188165=CARTESIAN_POINT('Ctrl Pts',(6.56282968112112,1.65940782166567,20.7760111835128));
#188166=CARTESIAN_POINT('Ctrl Pts',(6.51657867549774,1.83265040651704,20.7844361089145));
#188167=CARTESIAN_POINT('Ctrl Pts',(6.46351163328897,2.00382293787105,20.7928610343162));
#188168=CARTESIAN_POINT('Ctrl Pts',(6.41046034847175,2.1749446423373,20.8012834580739));
#188169=CARTESIAN_POINT('Ctrl Pts',(6.35059716183571,2.34399720090213,20.8097058818317));
#188170=CARTESIAN_POINT('Ctrl Pts',(6.2841117396454,2.51042399678836,20.8181283055894));
#188171=CARTESIAN_POINT('Ctrl Pts',(6.2176252718308,2.67685341008899,20.8265508618076));
#188172=CARTESIAN_POINT('Ctrl Pts',(6.14451647787865,2.84065666612478,20.8349734180258));
#188173=CARTESIAN_POINT('Ctrl Pts',(6.06502369189752,3.00129582292745,20.843395974244));
#188174=CARTESIAN_POINT('Ctrl Pts',(5.98552822063503,3.16194040615128,20.8518188149777));
#188175=CARTESIAN_POINT('Ctrl Pts',(5.89964847514893,3.31942037797676,20.8602416557115));
#188176=CARTESIAN_POINT('Ctrl Pts',(5.80766947296926,3.47322102561023,20.8686644964452));
#188177=CARTESIAN_POINT('Ctrl Pts',(5.71567452243535,3.62704834093037,20.8770887976259));
#188178=CARTESIAN_POINT('Ctrl Pts',(5.61757837795056,3.77719477387768,20.8855130988065));
#188179=CARTESIAN_POINT('Ctrl Pts',(5.51371042578661,3.92317299396446,20.8939373999871));
#188180=CARTESIAN_POINT('Ctrl Pts',(5.40980995826953,4.06919691181726,20.9023643383539));
#188181=CARTESIAN_POINT('Ctrl Pts',(5.30013427404017,4.21104974363724,20.9107912767208));
#188182=CARTESIAN_POINT('Ctrl Pts',(5.1850544373151,4.34827546069462,20.9192182150876));
#188183=CARTESIAN_POINT('Ctrl Pts',(5.0698711293515,4.48562456092064,20.9276527303312));
#188184=CARTESIAN_POINT('Ctrl Pts',(4.94927417435992,4.61833797749989,20.9360872455749));
#188185=CARTESIAN_POINT('Ctrl Pts',(4.82367382787709,4.74599407945834,20.9445217608185));
#188186=CARTESIAN_POINT('Ctrl Pts',(4.69801281535095,4.8737118404076,20.9529603500053));
#188187=CARTESIAN_POINT('Ctrl Pts',(4.56734383109422,4.99636718310635,20.9613989391921));
#188188=CARTESIAN_POINT('Ctrl Pts',(4.43211230911361,5.113576975015,20.9698375283789));
#188189=CARTESIAN_POINT('Ctrl Pts',(4.29672962888685,5.23091778095292,20.9782855499991));
#188190=CARTESIAN_POINT('Ctrl Pts',(4.15677447785778,5.34280066117938,20.9867335716194));
#188191=CARTESIAN_POINT('Ctrl Pts',(4.01272448631571,5.44888348167974,20.9951815932397));
#188192=CARTESIAN_POINT('Ctrl Pts',(3.93084878288709,5.50917925439849,20.999983313152));
#188193=CARTESIAN_POINT('Ctrl Pts',(3.84765073651829,5.56760204548384,21.0047850330642));
#188194=CARTESIAN_POINT('Ctrl Pts',(3.76322193724153,5.62409545180949,21.0095867529764));
#188195=CARTESIAN_POINT('Ctrl Pts',(3.61833740143535,5.72104129282245,21.0178267725729));
#188196=CARTESIAN_POINT('Ctrl Pts',(3.46950353234122,5.81251924285318,21.0260667921695));
#188197=CARTESIAN_POINT('Ctrl Pts',(3.3171691651141,5.89819275117525,21.034306811766));
#188198=CARTESIAN_POINT('Ctrl Pts',(3.24524477833348,5.93864333800981,21.0381973216183));
#188199=CARTESIAN_POINT('Ctrl Pts',(3.17254053868331,5.97780054540071,21.0420878314706));
#188200=CARTESIAN_POINT('Ctrl Pts',(3.09910619832133,6.01563211736941,21.0459783413229));
#188201=CARTESIAN_POINT('Ctrl Pts',(3.09910619832135,6.0156321173694,19.0455979788775));
#188202=CARTESIAN_POINT('Ctrl Pts',(2.93087086387512,6.10230283751758,19.0545209146099));
#188203=CARTESIAN_POINT('Ctrl Pts',(2.75912628990419,6.18184612462039,19.0634438503423));
#188204=CARTESIAN_POINT('Ctrl Pts',(2.58447961075416,6.25401903911365,19.0723667860748));
#188205=CARTESIAN_POINT('Ctrl Pts',(2.40953089484065,6.32631677060092,19.0813051532751));
#188206=CARTESIAN_POINT('Ctrl Pts',(2.23167027991639,6.39121854946046,19.0902435204755));
#188207=CARTESIAN_POINT('Ctrl Pts',(2.05152271824015,6.44853033927457,19.0991818876758));
#188208=CARTESIAN_POINT('Ctrl Pts',(2.03168758008735,6.45484065098886,19.1001660461436));
#188209=CARTESIAN_POINT('Ctrl Pts',(2.01182472940436,6.46105899903421,19.1011502046114));
#188210=CARTESIAN_POINT('Ctrl Pts',(1.99193500915975,6.4671851619761,19.1021343630793));
#188211=CARTESIAN_POINT('Ctrl Pts',(1.82575478240771,6.51836975051142,19.1103570869451));
#188212=CARTESIAN_POINT('Ctrl Pts',(1.65737931666312,6.56321309957973,19.118579810811));
#188213=CARTESIAN_POINT('Ctrl Pts',(1.48733340744237,6.60152469775778,19.1268025346769));
#188214=CARTESIAN_POINT('Ctrl Pts',(1.31746748605568,6.63979574440708,19.1350165550681));
#188215=CARTESIAN_POINT('Ctrl Pts',(1.14593498910629,6.67154872924817,19.1432305754594));
#188216=CARTESIAN_POINT('Ctrl Pts',(0.973277093441284,6.69664249451787,
19.1514445958506));
#188217=CARTESIAN_POINT('Ctrl Pts',(0.800767285486102,6.72171473700568,
19.1596515711225));
#188218=CARTESIAN_POINT('Ctrl Pts',(0.627134354172668,6.74013908371461,
19.1678585463945));
#188219=CARTESIAN_POINT('Ctrl Pts',(0.452931017569774,6.75182512312954,
19.1760655216665));
#188220=CARTESIAN_POINT('Ctrl Pts',(0.27884212908225,6.7635034850498,19.1842671051195));
#188221=CARTESIAN_POINT('Ctrl Pts',(0.104183938388189,6.76845233367149,
19.1924686885725));
#188222=CARTESIAN_POINT('Ctrl Pts',(-0.0704842496347184,6.76663291235408,
19.2006702720255));
#188223=CARTESIAN_POINT('Ctrl Pts',(-0.245072735382784,6.76481432125091,
19.2088681130405));
#188224=CARTESIAN_POINT('Ctrl Pts',(-0.419670851407023,6.75623361679936,
19.2170659540556));
#188225=CARTESIAN_POINT('Ctrl Pts',(-0.593717726144586,6.74090411307428,
19.2252637950706));
#188226=CARTESIAN_POINT('Ctrl Pts',(-0.767749241788536,6.72557596213007,
19.2334609126517));
#188227=CARTESIAN_POINT('Ctrl Pts',(-0.941229255217668,6.70350022109188,
19.2416580302329));
#188228=CARTESIAN_POINT('Ctrl Pts',(-1.11360008529399,6.6747422309804,19.249855147814));
#188229=CARTESIAN_POINT('Ctrl Pts',(-1.28596899755269,6.64598456083362,
19.2580521741931));
#188230=CARTESIAN_POINT('Ctrl Pts',(-1.45722839692184,6.61054484768785,
19.2662492005722));
#188231=CARTESIAN_POINT('Ctrl Pts',(-1.62682901058059,6.56853989637982,
19.2744462269513));
#188232=CARTESIAN_POINT('Ctrl Pts',(-1.79645857578088,6.52652777464907,
19.2826446525974));
#188233=CARTESIAN_POINT('Ctrl Pts',(-1.96442844280939,6.47794826822932,
19.2908430782435));
#188234=CARTESIAN_POINT('Ctrl Pts',(-2.13020270807044,6.42296858333663,
19.2990415038897));
#188235=CARTESIAN_POINT('Ctrl Pts',(-2.2960354148162,6.36796951609646,19.3072428197803));
#188236=CARTESIAN_POINT('Ctrl Pts',(-2.45967063753727,6.30656588870649,
19.315444135671));
#188237=CARTESIAN_POINT('Ctrl Pts',(-2.6205906716912,6.23897375627155,19.3236454515617));
#188238=CARTESIAN_POINT('Ctrl Pts',(-2.78169396682649,6.17130464771249,
19.3318561073783));
#188239=CARTESIAN_POINT('Ctrl Pts',(-2.94007556466262,6.09743309322177,
19.3400667631949));
#188240=CARTESIAN_POINT('Ctrl Pts',(-3.09523972006855,6.0176224603501,19.3482774190115));
#188241=CARTESIAN_POINT('Ctrl Pts',(-3.25049530995233,5.93776479700593,
19.3564929131687));
#188242=CARTESIAN_POINT('Ctrl Pts',(-3.40252936611668,5.85196125513129,
19.3647084073258));
#188243=CARTESIAN_POINT('Ctrl Pts',(-3.55087366035497,5.76051952936515,
19.372923901483));
#188244=CARTESIAN_POINT('Ctrl Pts',(-3.69944811349518,5.66893593007904,
19.3811521421305));
#188245=CARTESIAN_POINT('Ctrl Pts',(-3.84432106669312,5.57169686530648,
19.389380382778));
#188246=CARTESIAN_POINT('Ctrl Pts',(-3.98505493432114,5.46915223507654,
19.3976086234255));
#188247=CARTESIAN_POINT('Ctrl Pts',(-4.11295955168128,5.37595553755833,
19.4050867805266));
#188248=CARTESIAN_POINT('Ctrl Pts',(-4.23744558640654,5.27837712711518,
19.4125649376277));
#188249=CARTESIAN_POINT('Ctrl Pts',(-4.35821077628466,5.17670627228127,
19.4200430947288));
#188250=CARTESIAN_POINT('Ctrl Pts',(-4.48683218786717,5.06842135277147,
19.4280077335734));
#188251=CARTESIAN_POINT('Ctrl Pts',(-4.61167523612472,4.95512057304004,
19.435972372418));
#188252=CARTESIAN_POINT('Ctrl Pts',(-4.73230501151206,4.83710432779963,
19.4439370112626));
#188253=CARTESIAN_POINT('Ctrl Pts',(-4.85278451605925,4.7192350976744,19.4518917284028));
#188254=CARTESIAN_POINT('Ctrl Pts',(-4.96906091709185,4.59666234869501,
19.459846445543));
#188255=CARTESIAN_POINT('Ctrl Pts',(-5.08072985480975,4.46972853118005,
19.4678011626832));
#188256=CARTESIAN_POINT('Ctrl Pts',(-5.1922852483202,4.34292377909727,19.4757477915218));
#188257=CARTESIAN_POINT('Ctrl Pts',(-5.29924224750309,4.21176706368885,
19.4836944203604));
#188258=CARTESIAN_POINT('Ctrl Pts',(-5.40123123878462,4.07663956037043,
19.4916410491989));
#188259=CARTESIAN_POINT('Ctrl Pts',(-5.50313979131656,3.9416186321565,19.4995814105288));
#188260=CARTESIAN_POINT('Ctrl Pts',(-5.60008790270674,3.80263345049269,
19.5075217718587));
#188261=CARTESIAN_POINT('Ctrl Pts',(-5.69174453248446,3.66010015941276,
19.5154621331886));
#188262=CARTESIAN_POINT('Ctrl Pts',(-5.78335296646968,3.51764181659285,
19.5233983192394));
#188263=CARTESIAN_POINT('Ctrl Pts',(-5.86967524803693,3.37163939676288,
19.5313345052903));
#188264=CARTESIAN_POINT('Ctrl Pts',(-5.95042229290487,3.22253992001663,
19.5392706913411));
#188265=CARTESIAN_POINT('Ctrl Pts',(-6.03114767276121,3.07348044772997,
19.5472047480563));
#188266=CARTESIAN_POINT('Ctrl Pts',(-6.10630060867933,2.9213259069648,19.5551388047715));
#188267=CARTESIAN_POINT('Ctrl Pts',(-6.17563692211747,2.76654976571532,
19.5630728614866));
#188268=CARTESIAN_POINT('Ctrl Pts',(-6.24496888588621,2.61178333402511,
19.5710064204752));
#188269=CARTESIAN_POINT('Ctrl Pts',(-6.30848479697542,2.45439597819545,
19.5789399794639));
#188270=CARTESIAN_POINT('Ctrl Pts',(-6.36598788997289,2.29488282592349,
19.5868735384525));
#188271=CARTESIAN_POINT('Ctrl Pts',(-6.42349919835585,2.13534688423325,
19.5948082308975));
#188272=CARTESIAN_POINT('Ctrl Pts',(-6.47499585125896,1.9736849021302,19.6027429233424));
#188273=CARTESIAN_POINT('Ctrl Pts',(-6.52033047943041,1.81040863868101,
19.6106776157874));
#188274=CARTESIAN_POINT('Ctrl Pts',(-6.56570281025044,1.64699658614895,
19.6186189071377));
#188275=CARTESIAN_POINT('Ctrl Pts',(-6.60490278171912,1.48196794055604,
19.626560198488));
#188276=CARTESIAN_POINT('Ctrl Pts',(-6.63783372887719,1.31584664295669,
19.6345014898384));
#188277=CARTESIAN_POINT('Ctrl Pts',(-6.67077947895482,1.14965067151956,
19.6424463509098));
#188278=CARTESIAN_POINT('Ctrl Pts',(-6.69745053486376,0.982361447262679,
19.6503912119812));
#188279=CARTESIAN_POINT('Ctrl Pts',(-6.71780204686565,0.81450884533425,
19.6583360730526));
#188280=CARTESIAN_POINT('Ctrl Pts',(-6.7381790135413,0.646446301597885,
19.6662908711669));
#188281=CARTESIAN_POINT('Ctrl Pts',(-6.75222062424673,0.477819353365059,
19.6742456692812));
#188282=CARTESIAN_POINT('Ctrl Pts',(-6.75993413374877,0.309159355961101,
19.6822004673955));
#188283=CARTESIAN_POINT('Ctrl Pts',(-6.76477578602296,0.20329404785716,
19.6871935728516));
#188284=CARTESIAN_POINT('Ctrl Pts',(-6.76712528464591,0.0974156878556726,
19.6921866783078));
#188285=CARTESIAN_POINT('Ctrl Pts',(-6.76699485396139,-0.0083454454691123,
19.6971797837639));
#188286=CARTESIAN_POINT('',(-6.767,1.11697001474453E-12,19.3028202161899));
#188287=CARTESIAN_POINT('Ctrl Pts',(3.09910619832135,6.0156321173694,18.651395695404));
#188288=CARTESIAN_POINT('Ctrl Pts',(2.93375330764827,6.10081787314653,18.6601451433063));
#188289=CARTESIAN_POINT('Ctrl Pts',(2.76488627843071,6.17918207037039,18.6688945912086));
#188290=CARTESIAN_POINT('Ctrl Pts',(2.59307866646703,6.25045854553997,18.6776440391109));
#188291=CARTESIAN_POINT('Ctrl Pts',(2.42127244185377,6.32173444515037,18.6863934163612));
#188292=CARTESIAN_POINT('Ctrl Pts',(2.24652594672465,6.38592262741838,18.6951427936115));
#188293=CARTESIAN_POINT('Ctrl Pts',(2.06943269687121,6.44280508110562,18.7038921708618));
#188294=CARTESIAN_POINT('Ctrl Pts',(1.89234081822076,6.49968709436167,18.7126414803672));
#188295=CARTESIAN_POINT('Ctrl Pts',(1.71290249405587,6.54926340459545,18.7213907898725));
#188296=CARTESIAN_POINT('Ctrl Pts',(1.53172716625056,6.59136563150384,18.7301400993779));
#188297=CARTESIAN_POINT('Ctrl Pts',(1.35055318107333,6.6334675464071,18.7388893440451));
#188298=CARTESIAN_POINT('Ctrl Pts',(1.1676424971442,6.66809542395776,18.7476385887124));
#188299=CARTESIAN_POINT('Ctrl Pts',(0.983616340614383,6.69513165624668,
18.7563878333796));
#188300=CARTESIAN_POINT('Ctrl Pts',(0.799591486713904,6.7221676971596,18.7651370161153));
#188301=CARTESIAN_POINT('Ctrl Pts',(0.61445145952681,6.7416121586937,18.773886198851));
#188302=CARTESIAN_POINT('Ctrl Pts',(0.428825047910416,6.75339900185711,
18.7826353815867));
#188303=CARTESIAN_POINT('Ctrl Pts',(0.243199888597155,6.7651857655022,18.7913845052972));
#188304=CARTESIAN_POINT('Ctrl Pts',(0.0570886373920018,6.76931499599834,
18.8001336290078));
#188305=CARTESIAN_POINT('Ctrl Pts',(-0.128876626811089,6.76577266947847,
18.8088827527183));
#188306=CARTESIAN_POINT('Ctrl Pts',(-0.314840698188165,6.76223036567993,
18.8176318203099));
#188307=CARTESIAN_POINT('Ctrl Pts',(-0.500658497951326,6.75101660879223,
18.8263808879014));
#188308=CARTESIAN_POINT('Ctrl Pts',(-0.685698951926357,6.73216948296217,
18.8351299554929));
#188309=CARTESIAN_POINT('Ctrl Pts',(-0.870738280459992,6.71332247176291,
18.8438789698715));
#188310=CARTESIAN_POINT('Ctrl Pts',(-1.05499998761265,6.68684221356184,
18.85262798425));
#188311=CARTESIAN_POINT('Ctrl Pts',(-1.23785829161434,6.6528186394852,18.8613769986285));
#188312=CARTESIAN_POINT('Ctrl Pts',(-1.43007412917417,6.61705395368858,
18.8705737323277));
#188313=CARTESIAN_POINT('Ctrl Pts',(-1.62073882535804,6.57295372727787,
18.8797704660269));
#188314=CARTESIAN_POINT('Ctrl Pts',(-1.80913696091525,6.52068343478276,
18.8889671997261));
#188315=CARTESIAN_POINT('Ctrl Pts',(-1.98838356186127,6.47095219815194,
18.8977171974398));
#188316=CARTESIAN_POINT('Ctrl Pts',(-2.16557827572552,6.41382586850884,
18.9064671951534));
#188317=CARTESIAN_POINT('Ctrl Pts',(-2.34011918621723,6.34949849943269,
18.9152171928671));
#188318=CARTESIAN_POINT('Ctrl Pts',(-2.51465655691125,6.2851724349554,18.9239670131254));
#188319=CARTESIAN_POINT('Ctrl Pts',(-2.68653996295358,6.21364572242362,
18.9327168333837));
#188320=CARTESIAN_POINT('Ctrl Pts',(-2.85518555380022,6.13516132252206,
18.941466653642));
#188321=CARTESIAN_POINT('Ctrl Pts',(-3.02382794858724,6.05667841000489,
18.9502163080796));
#188322=CARTESIAN_POINT('Ctrl Pts',(-3.18923239109318,5.97123819492061,
18.9589659625171));
#188323=CARTESIAN_POINT('Ctrl Pts',(-3.35083705967737,5.87913088810691,
18.9677156169546));
#188324=CARTESIAN_POINT('Ctrl Pts',(-3.51243888042435,5.78702520443082,
18.9764651172035));
#188325=CARTESIAN_POINT('Ctrl Pts',(-3.67024081223721,5.68825280605763,
18.9852146174525));
#188326=CARTESIAN_POINT('Ctrl Pts',(-3.82370687544429,5.58314917682486,
18.9939641177014));
#188327=CARTESIAN_POINT('Ctrl Pts',(-3.97717043817844,5.47804726008001,
19.0027134753919));
#188328=CARTESIAN_POINT('Ctrl Pts',(-4.1262980372249,5.36661448084213,19.0114628330823));
#188329=CARTESIAN_POINT('Ctrl Pts',(-4.27058317206938,5.24922931204552,
19.0202121907728));
#188330=CARTESIAN_POINT('Ctrl Pts',(-4.41486614774846,5.1318458998678,19.0289614175329));
#188331=CARTESIAN_POINT('Ctrl Pts',(-4.55430658194406,5.0085104572304,19.0377106442929));
#188332=CARTESIAN_POINT('Ctrl Pts',(-4.68843089001821,4.87964187103142,
19.046459871053));
#188333=CARTESIAN_POINT('Ctrl Pts',(-4.82255336917803,4.75077504207994,
19.0552089785089));
#188334=CARTESIAN_POINT('Ctrl Pts',(-4.95135966065092,4.61637541908138,
19.0639580859648));
#188335=CARTESIAN_POINT('Ctrl Pts',(-5.07441230869194,4.47689945401902,
19.0727071934207));
#188336=CARTESIAN_POINT('Ctrl Pts',(-5.19746344226353,4.33742520555592,
19.0814561931971));
#188337=CARTESIAN_POINT('Ctrl Pts',(-5.31476088454691,4.19287495491432,
19.0902051929734));
#188338=CARTESIAN_POINT('Ctrl Pts',(-5.42590627628767,4.04373961586823,
19.0989541927498));
#188339=CARTESIAN_POINT('Ctrl Pts',(-5.53706380672587,3.89458798906849,
19.1077041480445));
#188340=CARTESIAN_POINT('Ctrl Pts',(-5.64206777071789,3.74085050155397,
19.1164541033392));
#188341=CARTESIAN_POINT('Ctrl Pts',(-5.74056148163939,3.58304938223271,
19.1252040586339));
#188342=CARTESIAN_POINT('Ctrl Pts',(-5.8390513895182,3.42525435593392,19.133953676075));
#188343=CARTESIAN_POINT('Ctrl Pts',(-5.93103139557593,3.26339625497292,
19.1427032935161));
#188344=CARTESIAN_POINT('Ctrl Pts',(-6.01618907820791,3.09802485065112,
19.1514529109572));
#188345=CARTESIAN_POINT('Ctrl Pts',(-6.10134392544933,2.93265895249744,
19.1602022370731));
#188346=CARTESIAN_POINT('Ctrl Pts',(-6.17967677261787,2.76378023986136,
19.168951563189));
#188347=CARTESIAN_POINT('Ctrl Pts',(-6.25092157009184,2.59196229227213,
19.1777008893048));
#188348=CARTESIAN_POINT('Ctrl Pts',(-6.3221643740772,2.42014915229179,19.1864499706073));
#188349=CARTESIAN_POINT('Ctrl Pts',(-6.38631941548894,2.24539720662929,
19.1951990519098));
#188350=CARTESIAN_POINT('Ctrl Pts',(-6.44316881037515,2.06829994947755,
19.2039481332122));
#188351=CARTESIAN_POINT('Ctrl Pts',(-6.50002334524552,1.89118668024518,
19.2126980055546));
#188352=CARTESIAN_POINT('Ctrl Pts',(-6.54957082411079,1.71172794807769,
19.2214478778969));
#188353=CARTESIAN_POINT('Ctrl Pts',(-6.59164294296068,1.53053334250405,
19.2301977502393));
#188354=CARTESIAN_POINT('Ctrl Pts',(-6.63371214082121,1.34935131693663,
19.2389470150942));
#188355=CARTESIAN_POINT('Ctrl Pts',(-6.66830695239679,1.16643393829825,
19.2476962799491));
#188356=CARTESIAN_POINT('Ctrl Pts',(-6.6953098815398,0.98240245834158,19.256445544804));
#188357=CARTESIAN_POINT('Ctrl Pts',(-6.72231419690476,0.798361530947684,
19.265195258811));
#188358=CARTESIAN_POINT('Ctrl Pts',(-6.74172580829272,0.613206671363136,
19.273944972818));
#188359=CARTESIAN_POINT('Ctrl Pts',(-6.75347878028175,0.427566795114092,
19.2826946868251));
#188360=CARTESIAN_POINT('Ctrl Pts',(-6.76248992368215,0.285234494205629,
19.2894031966133));
#188361=CARTESIAN_POINT('Ctrl Pts',(-6.76699999999998,0.142617266092147,
19.2961117064016));
#188362=CARTESIAN_POINT('Ctrl Pts',(-6.767,1.11697004507078E-12,19.3028202161899));
#188363=CARTESIAN_POINT('Ctrl Pts',(-6.7669994896834,-0.00262804578583102,
19.3028202161899));
#188364=CARTESIAN_POINT('Ctrl Pts',(-6.76692411827146,-0.196703167631038,
19.3119234788422));
#188365=CARTESIAN_POINT('Ctrl Pts',(-6.75849556223852,-0.390555835714825,
19.3210267414945));
#188366=CARTESIAN_POINT('Ctrl Pts',(-6.74179607552328,-0.583502078881353,
19.3301300041467));
#188367=CARTESIAN_POINT('Ctrl Pts',(-6.7242794658459,-0.785889379036061,
19.3396786987497));
#188368=CARTESIAN_POINT('Ctrl Pts',(-6.69766236172528,-0.987279027706483,
19.3492273933527));
#188369=CARTESIAN_POINT('Ctrl Pts',(-6.66209914580194,-1.18689678216142,
19.3587760879557));
#188370=CARTESIAN_POINT('Ctrl Pts',(-6.6279912981864,-1.37834549605109,
19.3679340173497));
#188371=CARTESIAN_POINT('Ctrl Pts',(-6.58565503867919,-1.56816428165398,
19.3770919467436));
#188372=CARTESIAN_POINT('Ctrl Pts',(-6.53527762040866,-1.75568659623117,
19.3862498761375));
#188373=CARTESIAN_POINT('Ctrl Pts',(-6.48482247995173,-1.94349821988346,
19.3954219343677));
#188374=CARTESIAN_POINT('Ctrl Pts',(-6.42630144353643,-2.1290060880081,
19.4045939925979));
#188375=CARTESIAN_POINT('Ctrl Pts',(-6.35995131213566,-2.31155971310799,
19.4137660508281));
#188376=CARTESIAN_POINT('Ctrl Pts',(-6.29348779166628,-2.49442531325727,
19.4229537836488));
#188377=CARTESIAN_POINT('Ctrl Pts',(-6.21916849175762,-2.67432637534773,
19.4321415164695));
#188378=CARTESIAN_POINT('Ctrl Pts',(-6.13727880330701,-2.8506311389723,
19.4413292492902));
#188379=CARTESIAN_POINT('Ctrl Pts',(-6.12722177115829,-2.87228347041101,
19.4424576126544));
#188380=CARTESIAN_POINT('Ctrl Pts',(-6.11705061400901,-2.89388158903475,
19.4435859760186));
#188381=CARTESIAN_POINT('Ctrl Pts',(-6.10676590851729,-2.91542434965667,
19.4447143393827));
#188382=CARTESIAN_POINT('Ctrl Pts',(-6.03166496039581,-3.07273383694952,
19.4529538712336));
#188383=CARTESIAN_POINT('Ctrl Pts',(-5.95037766933127,-3.22735753787452,
19.4611934030844));
#188384=CARTESIAN_POINT('Ctrl Pts',(-5.86311817374967,-3.37877703920314,
19.4694329349352));
#188385=CARTESIAN_POINT('Ctrl Pts',(-5.77595553010974,-3.53002847546775,
19.4776633214816));
#188386=CARTESIAN_POINT('Ctrl Pts',(-5.68283405700541,-3.67808248794971,
19.4858937080279));
#188387=CARTESIAN_POINT('Ctrl Pts',(-5.58401543055536,-3.82244171588261,
19.4941240945742));
#188388=CARTESIAN_POINT('Ctrl Pts',(-5.48528885753931,-3.96666646752155,
19.502346814192));
#188389=CARTESIAN_POINT('Ctrl Pts',(-5.38087590025924,-4.10720299712672,
19.5105695338098));
#188390=CARTESIAN_POINT('Ctrl Pts',(-5.27108355841995,-4.24357951735971,
19.5187922534277));
#188391=CARTESIAN_POINT('Ctrl Pts',(-5.16138850050598,-4.37983519816995,
19.5270076871234));
#188392=CARTESIAN_POINT('Ctrl Pts',(-5.04632378049846,-4.51193794011583,
19.5352231208192));
#188393=CARTESIAN_POINT('Ctrl Pts',(-4.92623892718506,-4.63944598333536,
19.543438554515));
#188394=CARTESIAN_POINT('Ctrl Pts',(-4.80621578816163,-4.76688849732172,
19.5516497661158));
#188395=CARTESIAN_POINT('Ctrl Pts',(-4.68117789746008,-4.88974075689622,
19.5598609777166));
#188396=CARTESIAN_POINT('Ctrl Pts',(-4.55151444305599,-5.0075947594282,
19.5680721893174));
#188397=CARTESIAN_POINT('Ctrl Pts',(-4.42189447061963,-5.12540924023094,
19.576280647331));
#188398=CARTESIAN_POINT('Ctrl Pts',(-4.28765228761291,-5.23822856387882,
19.5844891053445));
#188399=CARTESIAN_POINT('Ctrl Pts',(-4.14921331450017,-5.34568217075936,
19.592697563358));
#188400=CARTESIAN_POINT('Ctrl Pts',(-4.08753572905468,-5.39355509895859,
19.5963546106412));
#188401=CARTESIAN_POINT('Ctrl Pts',(-4.02502558672144,-5.44036350152121,
19.6000116579243));
#188402=CARTESIAN_POINT('Ctrl Pts',(-3.96172264090319,-5.48607717012394,
19.6036687052075));
#188403=CARTESIAN_POINT('Ctrl Pts',(-3.8083733814779,-5.59681699645,19.6125277793834));
#188404=CARTESIAN_POINT('Ctrl Pts',(-3.65052916837581,-5.70101476812618,
19.6213868535593));
#188405=CARTESIAN_POINT('Ctrl Pts',(-3.48875881748808,-5.79834898168429,
19.6302459277351));
#188406=CARTESIAN_POINT('Ctrl Pts',(-3.32668453265651,-5.89586606664766,
19.6391216463291));
#188407=CARTESIAN_POINT('Ctrl Pts',(-3.16066959080951,-5.98649368944297,
19.6479973649231));
#188408=CARTESIAN_POINT('Ctrl Pts',(-2.99130644250467,-6.06995673518602,
19.656873083517));
#188409=CARTESIAN_POINT('Ctrl Pts',(-2.82145997962814,-6.15365796087912,
19.665774130904));
#188410=CARTESIAN_POINT('Ctrl Pts',(-2.64824642373677,-6.23015357956474,
19.674675178291));
#188411=CARTESIAN_POINT('Ctrl Pts',(-2.4722800904021,-6.29921583648325,
19.683576225678));
#188412=CARTESIAN_POINT('Ctrl Pts',(-2.29607452842366,-6.36837198448732,
19.692489374161));
#188413=CARTESIAN_POINT('Ctrl Pts',(-2.11710895690211,-6.43007449522048,
19.701402522644));
#188414=CARTESIAN_POINT('Ctrl Pts',(-1.93601317239168,-6.4841454330024,
19.710315671127));
#188415=CARTESIAN_POINT('Ctrl Pts',(-1.75451530572022,-6.53833642305153,
19.7192486092369));
#188416=CARTESIAN_POINT('Ctrl Pts',(-1.57087801530508,-6.58486187421657,
19.7281815473467));
#188417=CARTESIAN_POINT('Ctrl Pts',(-1.38574443851102,-6.62359429246205,
19.7371144854566));
#188418=CARTESIAN_POINT('Ctrl Pts',(-1.20952411665315,-6.66046193866512,
19.7456173473152));
#188419=CARTESIAN_POINT('Ctrl Pts',(-1.03194837503492,-6.69026924440987,
19.7541202091737));
#188420=CARTESIAN_POINT('Ctrl Pts',(-0.853576295393243,-6.71294991102591,
19.7626230710323));
#188421=CARTESIAN_POINT('Ctrl Pts',(-0.681080919051054,-6.73488333318191,
19.7708457948981));
#188422=CARTESIAN_POINT('Ctrl Pts',(-0.507510078536465,-6.75019302760903,
19.779068518764));
#188423=CARTESIAN_POINT('Ctrl Pts',(-0.333413462753453,-6.75878128532465,
19.7872912426299));
#188424=CARTESIAN_POINT('Ctrl Pts',(-0.159501122340489,-6.76736045266042,
19.7955052630211));
#188425=CARTESIAN_POINT('Ctrl Pts',(0.0149355298302086,-6.76923233283801,
19.8037192834123));
#188426=CARTESIAN_POINT('Ctrl Pts',(0.189339128267373,-6.76435064839981,
19.8119333038036));
#188427=CARTESIAN_POINT('Ctrl Pts',(0.363593141715594,-6.759473150955,19.8201402790755));
#188428=CARTESIAN_POINT('Ctrl Pts',(0.537813801340364,-6.74785363512641,
19.8283472543475));
#188429=CARTESIAN_POINT('Ctrl Pts',(0.711441072268215,-6.72949779706405,
19.8365542296195));
#188430=CARTESIAN_POINT('Ctrl Pts',(0.884954273543917,-6.71115401842099,
19.8447558130725));
#188431=CARTESIAN_POINT('Ctrl Pts',(1.05787450718939,-6.68608277044488,
19.8529573965254));
#188432=CARTESIAN_POINT('Ctrl Pts',(1.22964410578536,-6.65434176858292,
19.8611589799784));
#188433=CARTESIAN_POINT('Ctrl Pts',(1.40133532475278,-6.62261525035461,
19.8693568209935));
#188434=CARTESIAN_POINT('Ctrl Pts',(1.57187660265974,-6.58422510659389,
19.8775546620085));
#188435=CARTESIAN_POINT('Ctrl Pts',(1.74071765662254,-6.53928062097985,
19.8857525030236));
#188436=CARTESIAN_POINT('Ctrl Pts',(1.90954381088925,-6.4943401015764,19.8939496206047));
#188437=CARTESIAN_POINT('Ctrl Pts',(2.07666969147306,-6.44284647633123,
19.9021467381859));
#188438=CARTESIAN_POINT('Ctrl Pts',(2.24155707918389,-6.38495973838211,
19.910343855767));
#188439=CARTESIAN_POINT('Ctrl Pts',(2.40644263233884,-6.32707364448745,
19.9185408821461));
#188440=CARTESIAN_POINT('Ctrl Pts',(2.56908940329754,-6.26279469741363,
19.9267379085252));
#188441=CARTESIAN_POINT('Ctrl Pts',(2.72897628063101,-6.19233215030923,
19.9349349349043));
#188442=CARTESIAN_POINT('Ctrl Pts',(2.88889045133025,-6.12185757495022,
19.9431333605504));
#188443=CARTESIAN_POINT('Ctrl Pts',(3.04604346141292,-6.04519744127166,
19.9513317861966));
#188444=CARTESIAN_POINT('Ctrl Pts',(3.199936012489,-5.96260836513485,19.9595302118427));
#188445=CARTESIAN_POINT('Ctrl Pts',(3.35388281631086,-5.8799901733318,19.9677315277334));
#188446=CARTESIAN_POINT('Ctrl Pts',(3.50456655546273,-5.79143904501214,
19.975932843624));
#188447=CARTESIAN_POINT('Ctrl Pts',(3.65151423670819,-5.69725660112983,
19.9841341595147));
#188448=CARTESIAN_POINT('Ctrl Pts',(3.7986292667642,-5.60296689920965,19.9923448153313));
#188449=CARTESIAN_POINT('Ctrl Pts',(3.94199943627073,-5.50303326327248,
20.0005554711479));
#188450=CARTESIAN_POINT('Ctrl Pts',(4.08118149837881,-5.3978001609258,20.0087661269645));
#188451=CARTESIAN_POINT('Ctrl Pts',(4.22044557710406,-5.29250504726142,
20.0169816211216));
#188452=CARTESIAN_POINT('Ctrl Pts',(4.35551635177849,-5.18190446923081,
20.0251971152787));
#188453=CARTESIAN_POINT('Ctrl Pts',(4.48598528528534,-5.06638184705846,
20.0334126094359));
#188454=CARTESIAN_POINT('Ctrl Pts',(4.61665664374337,-4.95067998941199,
20.0416408500834));
#188455=CARTESIAN_POINT('Ctrl Pts',(4.74271163374992,-4.83004107454375,
20.0498690907309));
#188456=CARTESIAN_POINT('Ctrl Pts',(4.86377914350231,-4.70488484909375,
20.0580973313784));
#188457=CARTESIAN_POINT('Ctrl Pts',(4.97381018130919,-4.59113782148561,
20.0655754884795));
#188458=CARTESIAN_POINT('Ctrl Pts',(5.07972197530185,-4.47366011755974,
20.0730536455807));
#188459=CARTESIAN_POINT('Ctrl Pts',(5.18126633726378,-4.35278854785495,
20.0805318026818));
#188460=CARTESIAN_POINT('Ctrl Pts',(5.29083783267295,-4.22236201910318,
20.0886011119043));
#188461=CARTESIAN_POINT('Ctrl Pts',(5.39568211999948,-4.08755634077539,
20.0966704211268));
#188462=CARTESIAN_POINT('Ctrl Pts',(5.49541878552054,-3.94875440762628,
20.1047397303493));
#188463=CARTESIAN_POINT('Ctrl Pts',(5.59503105231212,-3.81012559821299,
20.1127989749501));
#188464=CARTESIAN_POINT('Ctrl Pts',(5.68954815809697,-3.66751075082367,
20.1208582195509));
#188465=CARTESIAN_POINT('Ctrl Pts',(5.77862738107788,-3.52132852637425,
20.1289174641516));
#188466=CARTESIAN_POINT('Ctrl Pts',(5.86761504634572,-3.37529655144108,
20.1369684252719));
#188467=CARTESIAN_POINT('Ctrl Pts',(5.95117575886275,-3.22570481206129,
20.1450193863922));
#188468=CARTESIAN_POINT('Ctrl Pts',(6.02900793362165,-3.073003796992,20.1530703475124));
#188469=CARTESIAN_POINT('Ctrl Pts',(6.1067771652212,-2.92042627178219,20.1611147977915));
#188470=CARTESIAN_POINT('Ctrl Pts',(6.17882691105941,-2.76474480628899,
20.1691592480706));
#188471=CARTESIAN_POINT('Ctrl Pts',(6.24489974717524,-2.60643744366341,
20.1772036983497));
#188472=CARTESIAN_POINT('Ctrl Pts',(6.31093361267745,-2.44822345276856,
20.185243403908));
#188473=CARTESIAN_POINT('Ctrl Pts',(6.37099744283874,-2.28738699139377,
20.1932831094662));
#188474=CARTESIAN_POINT('Ctrl Pts',(6.42488054552516,-2.12442909407031,
20.2013228150244));
#188475=CARTESIAN_POINT('Ctrl Pts',(6.47992668617561,-1.95795383765508,
20.2095360533289));
#188476=CARTESIAN_POINT('Ctrl Pts',(6.52852206974812,-1.78926487949218,
20.2177492916333));
#188477=CARTESIAN_POINT('Ctrl Pts',(6.57049450686606,-1.618916593047,20.2259625299378));
#188478=CARTESIAN_POINT('Ctrl Pts',(6.61156690710525,-1.45222117382998,
20.233999647486));
#188479=CARTESIAN_POINT('Ctrl Pts',(6.64629743937475,-1.28393724887201,
20.2420367650341));
#188480=CARTESIAN_POINT('Ctrl Pts',(6.67457569905664,-1.11459779183461,
20.2500738825823));
#188481=CARTESIAN_POINT('Ctrl Pts',(6.70285695039861,-0.945240419759346,
20.2581118504064));
#188482=CARTESIAN_POINT('Ctrl Pts',(6.72468450832059,-0.774827661776648,
20.2661498182305));
#188483=CARTESIAN_POINT('Ctrl Pts',(6.73999949411888,-0.603900504451883,
20.2741877860546));
#188484=CARTESIAN_POINT('Ctrl Pts',(6.75531913460856,-0.432921397149721,
20.2822281968624));
#188485=CARTESIAN_POINT('Ctrl Pts',(6.76412222974144,-0.261427951225687,
20.2902686076701));
#188486=CARTESIAN_POINT('Ctrl Pts',(6.76640196070452,-0.0899639159557847,
20.2983090184778));
#188487=CARTESIAN_POINT('Ctrl Pts',(6.76876785264016,0.0879804927781306,
20.3066533114656));
#188488=CARTESIAN_POINT('Ctrl Pts',(6.76410764778107,0.265892778929249,
20.3149976044534));
#188489=CARTESIAN_POINT('Ctrl Pts',(6.75247289523313,0.443169041271924,
20.3233418974412));
#188490=CARTESIAN_POINT('Ctrl Pts',(6.74124205795728,0.614290932093335,
20.3313965076568));
#188491=CARTESIAN_POINT('Ctrl Pts',(6.72351292290034,0.78481986124143,20.3394511178723));
#188492=CARTESIAN_POINT('Ctrl Pts',(6.69938426918256,0.954221889200478,
20.3475057280878));
#188493=CARTESIAN_POINT('Ctrl Pts',(6.67523734973306,1.12375215688774,20.3555664357571));
#188494=CARTESIAN_POINT('Ctrl Pts',(6.64468133183714,1.29215345978572,20.3636271434263));
#188495=CARTESIAN_POINT('Ctrl Pts',(6.60786535590953,1.45890521904977,20.3716878510956));
#188496=CARTESIAN_POINT('Ctrl Pts',(6.5709974716616,1.62589208830386,20.3797599238797));
#188497=CARTESIAN_POINT('Ctrl Pts',(6.52785211311753,1.79122441563057,20.3878319966639));
#188498=CARTESIAN_POINT('Ctrl Pts',(6.47862735450224,1.95439929428337,20.395904069448));
#188499=CARTESIAN_POINT('Ctrl Pts',(6.47347143503538,1.97149062305806,20.3967495577424));
#188500=CARTESIAN_POINT('Ctrl Pts',(6.46824886099491,1.98855830321337,20.3975950460369));
#188501=CARTESIAN_POINT('Ctrl Pts',(6.46295988947777,2.00560177178859,20.3984405343313));
#188502=CARTESIAN_POINT('Ctrl Pts',(6.41082497459428,2.17360414816904,20.4067747558567));
#188503=CARTESIAN_POINT('Ctrl Pts',(6.35206824183237,2.33978817453824,20.4151089773821));
#188504=CARTESIAN_POINT('Ctrl Pts',(6.28683273756299,2.50360203105571,20.4234431989075));
#188505=CARTESIAN_POINT('Ctrl Pts',(6.22167602151371,2.66721804128795,20.4317673547717));
#188506=CARTESIAN_POINT('Ctrl Pts',(6.1500562503023,2.82846926380757,20.440091510636));
#188507=CARTESIAN_POINT('Ctrl Pts',(6.07216642814117,2.98681835218604,20.4484156665002));
#188508=CARTESIAN_POINT('Ctrl Pts',(5.99305939178687,3.14764202264083,20.4568699071481));
#188509=CARTESIAN_POINT('Ctrl Pts',(5.90748478019005,3.30547174461127,20.4653241477961));
#188510=CARTESIAN_POINT('Ctrl Pts',(5.81569669955021,3.45976312756247,20.473778388444));
#188511=CARTESIAN_POINT('Ctrl Pts',(5.72550545878816,3.61137029888859,20.4820855504242));
#188512=CARTESIAN_POINT('Ctrl Pts',(5.62931534185075,3.75956091274163,20.4903927124045));
#188513=CARTESIAN_POINT('Ctrl Pts',(5.52741478724101,3.90384102773019,20.4986998743848));
#188514=CARTESIAN_POINT('Ctrl Pts',(5.42557323608984,4.04803760023145,20.5070022262707));
#188515=CARTESIAN_POINT('Ctrl Pts',(5.3180280348611,4.18832790165481,20.5153045781566));
#188516=CARTESIAN_POINT('Ctrl Pts',(5.20511163705089,4.32424581237439,20.5236069300425));
#188517=CARTESIAN_POINT('Ctrl Pts',(5.09224185037621,4.46010761708739,20.5319058547729));
#188518=CARTESIAN_POINT('Ctrl Pts',(4.9740055072949,4.59160036058793,20.5402047795033));
#188519=CARTESIAN_POINT('Ctrl Pts',(4.85077626894283,4.71828979490038,20.5485037042337));
#188520=CARTESIAN_POINT('Ctrl Pts',(4.72355437961419,4.84908399120271,20.5570715157184));
#188521=CARTESIAN_POINT('Ctrl Pts',(4.59101084937444,4.97475808421853,20.5656393272031));
#188522=CARTESIAN_POINT('Ctrl Pts',(4.45359967091374,5.09487379345524,20.5742071386878));
#188523=CARTESIAN_POINT('Ctrl Pts',(4.32052411644,5.21119958868343,20.5825046169332));
#188524=CARTESIAN_POINT('Ctrl Pts',(4.18288370146673,5.32231219823381,20.5908020951786));
#188525=CARTESIAN_POINT('Ctrl Pts',(4.04112586324388,5.42785323654034,20.5990995734239));
#188526=CARTESIAN_POINT('Ctrl Pts',(3.89244028363945,5.53855209206316,20.6078025515283));
#188527=CARTESIAN_POINT('Ctrl Pts',(3.73922506593886,5.64312087543043,20.6165055296326));
#188528=CARTESIAN_POINT('Ctrl Pts',(3.58203235262422,5.74119614930142,20.6252085077369));
#188529=CARTESIAN_POINT('Ctrl Pts',(3.42483963930957,5.83927142317241,20.6339114858412));
#188530=CARTESIAN_POINT('Ctrl Pts',(3.2636698169091,5.93085297522223,20.6426144639456));
#188531=CARTESIAN_POINT('Ctrl Pts',(3.09910619832131,6.01563211736942,20.6513174420499));
#188532=CARTESIAN_POINT('Origin',(0.,0.,4.30282021618968));
#188533=CARTESIAN_POINT('',(3.09910619832132,6.01563211736941,23.0457234660332));
#188534=CARTESIAN_POINT('',(3.09910619832133,6.01563211736941,22.651395695404));
#188535=CARTESIAN_POINT('',(3.09910619832133,6.0156321173694,4.30282021618968));
#188536=CARTESIAN_POINT('',(-6.76699496442947,0.0082553852872212,21.6971797838552));
#188537=CARTESIAN_POINT('Ctrl Pts',(-6.76699496442947,0.0082553852872167,
21.6971797838552));
#188538=CARTESIAN_POINT('Ctrl Pts',(-6.76720014876307,-0.159935595989462,
21.7051103156268));
#188539=CARTESIAN_POINT('Ctrl Pts',(-6.76113088550322,-0.328408545218613,
21.7130408473984));
#188540=CARTESIAN_POINT('Ctrl Pts',(-6.74875105755394,-0.496636852402841,
21.7209713791701));
#188541=CARTESIAN_POINT('Ctrl Pts',(-6.73638286209287,-0.664707086808642,
21.7288944591566));
#188542=CARTESIAN_POINT('Ctrl Pts',(-6.71771592388165,-0.83253275655728,
21.7368175391432));
#188543=CARTESIAN_POINT('Ctrl Pts',(-6.69276612089855,-0.999585239463147,
21.7447406191297));
#188544=CARTESIAN_POINT('Ctrl Pts',(-6.66783403685853,-1.16651908442071,
21.7526580722741));
#188545=CARTESIAN_POINT('Ctrl Pts',(-6.63662802108039,-1.33268045684481,
21.7605755254185));
#188546=CARTESIAN_POINT('Ctrl Pts',(-6.59921591081262,-1.49754411036121,
21.7684929785628));
#188547=CARTESIAN_POINT('Ctrl Pts',(-6.56085853100868,-1.66657327574465,
21.7766104772863));
#188548=CARTESIAN_POINT('Ctrl Pts',(-6.51597730961295,-1.8342378645121,
21.7847279760097));
#188549=CARTESIAN_POINT('Ctrl Pts',(-6.46470159579191,-1.999980569247,21.7928454747331));
#188550=CARTESIAN_POINT('Ctrl Pts',(-6.41471783401116,-2.16154719120139,
21.8007584435094));
#188551=CARTESIAN_POINT('Ctrl Pts',(-6.35865807491377,-2.32128723103019,
21.8086714122856));
#188552=CARTESIAN_POINT('Ctrl Pts',(-6.29669306076058,-2.47869834763523,
21.8165843810619));
#188553=CARTESIAN_POINT('Ctrl Pts',(-6.23472660831995,-2.63611311795413,
21.8244975335083));
#188554=CARTESIAN_POINT('Ctrl Pts',(-6.16685476853288,-2.79119849962973,
21.8324106859548));
#188555=CARTESIAN_POINT('Ctrl Pts',(-6.09329676179189,-2.94347134736121,
21.8403238384012));
#188556=CARTESIAN_POINT('Ctrl Pts',(-6.01972182361219,-3.0957792449602,
21.8482388122816));
#188557=CARTESIAN_POINT('Ctrl Pts',(-5.94045828250411,-3.24527297503472,
21.8561537861621));
#188558=CARTESIAN_POINT('Ctrl Pts',(-5.85577156912129,-3.39149352502268,
21.8640687600425));
#188559=CARTESIAN_POINT('Ctrl Pts',(-5.76728249953132,-3.54427924437017,
21.8723391090327));
#188560=CARTESIAN_POINT('Ctrl Pts',(-5.6728722352669,-3.69349064921928,
21.8806094580229));
#188561=CARTESIAN_POINT('Ctrl Pts',(-5.57289370828325,-3.83863839351624,
21.8888798070131));
#188562=CARTESIAN_POINT('Ctrl Pts',(-5.47705412758578,-3.97777726035392,
21.8968077771819));
#188563=CARTESIAN_POINT('Ctrl Pts',(-5.37609834351553,-4.11318190804607,
21.9047357473506));
#188564=CARTESIAN_POINT('Ctrl Pts',(-5.27037764387939,-4.2444562067356,
21.9126637175194));
#188565=CARTESIAN_POINT('Ctrl Pts',(-5.16458109587965,-4.37582468698817,
21.9205973755389));
#188566=CARTESIAN_POINT('Ctrl Pts',(-5.05401308107522,-4.50305663475895,
21.9285310335585));
#188567=CARTESIAN_POINT('Ctrl Pts',(-4.93906107671895,-4.62579341091232,
21.936464691578));
#188568=CARTESIAN_POINT('Ctrl Pts',(-4.82394961633868,-4.74870044175967,
21.9444093547955));
#188569=CARTESIAN_POINT('Ctrl Pts',(-4.70444230869804,-4.86709959820524,
21.952354018013));
#188570=CARTESIAN_POINT('Ctrl Pts',(-4.58095924754832,-4.98067278309884,
21.9602986812305));
#188571=CARTESIAN_POINT('Ctrl Pts',(-4.56534243794244,-4.99503629812918,
21.9613034367953));
#188572=CARTESIAN_POINT('Ctrl Pts',(-4.54966207515606,-5.00932268186436,
21.9623081923601));
#188573=CARTESIAN_POINT('Ctrl Pts',(-4.53391904016846,-5.02353134131737,
21.9633129479249));
#188574=CARTESIAN_POINT('Ctrl Pts',(-4.4033544651371,-5.14137060069203,
21.9716458699717));
#188575=CARTESIAN_POINT('Ctrl Pts',(-4.26802527448159,-5.25426780731966,
21.9799787920184));
#188576=CARTESIAN_POINT('Ctrl Pts',(-4.12833594852465,-5.36182163971529,
21.9883117140651));
#188577=CARTESIAN_POINT('Ctrl Pts',(-3.98881170147592,-5.46924836956314,
21.9966347886187));
#188578=CARTESIAN_POINT('Ctrl Pts',(-3.84493785689512,-5.57134409384086,
22.0049578631723));
#188579=CARTESIAN_POINT('Ctrl Pts',(-3.69715448022344,-5.66774538501543,
22.0132809377259));
#188580=CARTESIAN_POINT('Ctrl Pts',(-3.54951862117828,-5.76405044825161,
22.0215957041719));
#188581=CARTESIAN_POINT('Ctrl Pts',(-3.39798129469385,-5.85467221420411,
22.0299104706178));
#188582=CARTESIAN_POINT('Ctrl Pts',(-3.24301445245601,-5.93928836319314,
22.0382252370638));
#188583=CARTESIAN_POINT('Ctrl Pts',(-3.08817387225721,-6.02383556964355,
22.0465332289033));
#188584=CARTESIAN_POINT('Ctrl Pts',(-2.9299096481701,-6.10238674317606,
22.0548412207429));
#188585=CARTESIAN_POINT('Ctrl Pts',(-2.7687216283401,-6.17466351672395,
22.0631492125824));
#188586=CARTESIAN_POINT('Ctrl Pts',(-2.60763538818261,-6.24689465222535,
22.0714519584695));
#188587=CARTESIAN_POINT('Ctrl Pts',(-2.4436293481048,-6.31285914132132,
22.0797547043565));
#188588=CARTESIAN_POINT('Ctrl Pts',(-2.27722700900109,-6.3723250191336,
22.0880574502436));
#188589=CARTESIAN_POINT('Ctrl Pts',(-2.1108926732303,-6.43176659513673,
22.096356803063));
#188590=CARTESIAN_POINT('Ctrl Pts',(-1.94216431686134,-6.4847147347854,
22.1046561558825));
#188591=CARTESIAN_POINT('Ctrl Pts',(-1.7715846998492,-6.53098588662234,
22.1129555087019));
#188592=CARTESIAN_POINT('Ctrl Pts',(-1.60104136225905,-6.57724719736178,
22.1212530963882));
#188593=CARTESIAN_POINT('Ctrl Pts',(-1.42864788400555,-6.61683425838779,
22.1295506840746));
#188594=CARTESIAN_POINT('Ctrl Pts',(-1.2549616774216,-6.64961353675559,
22.137848271761));
#188595=CARTESIAN_POINT('Ctrl Pts',(-1.08128354863033,-6.68239129062573,
22.1461454735434));
#188596=CARTESIAN_POINT('Ctrl Pts',(-0.906313153192367,-6.70836182841414,
22.1544426753258));
#188597=CARTESIAN_POINT('Ctrl Pts',(-0.730617766375759,-6.72744280387846,
22.1627398771082));
#188598=CARTESIAN_POINT('Ctrl Pts',(-0.55490135587092,-6.74652606256995,
22.1710380717327));
#188599=CARTESIAN_POINT('Ctrl Pts',(-0.378460127035671,-6.75871807925165,
22.1793362663573));
#188600=CARTESIAN_POINT('Ctrl Pts',(-0.201866337928561,-6.7639883930719,
22.1876344609818));
#188601=CARTESIAN_POINT('Ctrl Pts',(-0.025148348350608,-6.7692624135653,
22.1959384918234));
#188602=CARTESIAN_POINT('Ctrl Pts',(0.151722067725539,-6.76760499335631,
22.204242522665));
#188603=CARTESIAN_POINT('Ctrl Pts',(0.328171877683939,-6.75903781752236,
22.2125465535066));
#188604=CARTESIAN_POINT('Ctrl Pts',(0.504685849649502,-6.75046752642749,
22.2208536039223));
#188605=CARTESIAN_POINT('Ctrl Pts',(0.680778563572517,-6.7349824960736,
22.229160654338));
#188606=CARTESIAN_POINT('Ctrl Pts',(0.855882010926367,-6.71265632841222,
22.2374677047538));
#188607=CARTESIAN_POINT('Ctrl Pts',(1.0311726734178,-6.69030629030961,22.2457836368084));
#188608=CARTESIAN_POINT('Ctrl Pts',(1.20547161169683,-6.66110055214837,
22.254099568863));
#188609=CARTESIAN_POINT('Ctrl Pts',(1.37821981766227,-6.62516408356827,
22.2624155009176));
#188610=CARTESIAN_POINT('Ctrl Pts',(1.5084410846112,-6.59807441023697,22.2686842271366));
#188611=CARTESIAN_POINT('Ctrl Pts',(1.63778134385809,-6.56716108539172,
22.2749529533555));
#188612=CARTESIAN_POINT('Ctrl Pts',(1.76600695449821,-6.5324963403483,22.2812216795745));
#188613=CARTESIAN_POINT('Ctrl Pts',(1.93885560497011,-6.48576812147069,
22.2896719482978));
#188614=CARTESIAN_POINT('Ctrl Pts',(2.10999522057186,-6.43213574420275,
22.2981222170212));
#188615=CARTESIAN_POINT('Ctrl Pts',(2.278855405123,-6.37174285753448,22.3065724857445));
#188616=CARTESIAN_POINT('Ctrl Pts',(2.44756656483243,-6.31140326963762,
22.3150152968191));
#188617=CARTESIAN_POINT('Ctrl Pts',(2.61400199236264,-6.24431517555305,
22.3234581078936));
#188618=CARTESIAN_POINT('Ctrl Pts',(2.7776056207408,-6.1706722498954,22.3319009189681));
#188619=CARTESIAN_POINT('Ctrl Pts',(2.9410871384213,-6.09708428994431,22.3403374284858));
#188620=CARTESIAN_POINT('Ctrl Pts',(3.10174076892398,-6.01695138680906,
22.3487739380036));
#188621=CARTESIAN_POINT('Ctrl Pts',(3.25902926810792,-5.93051576421613,
22.3572104475213));
#188622=CARTESIAN_POINT('Ctrl Pts',(3.41620521890647,-5.84414199096255,
22.3656409202625));
#188623=CARTESIAN_POINT('Ctrl Pts',(3.57002055150506,-5.75147465334733,
22.3740713930037));
#188624=CARTESIAN_POINT('Ctrl Pts',(3.71996134355306,-5.65280254409005,
22.3825018657449));
#188625=CARTESIAN_POINT('Ctrl Pts',(3.86983767646135,-5.55417285370484,
22.3909287142488));
#188626=CARTESIAN_POINT('Ctrl Pts',(4.0158425128803,-5.44954371980091,22.3993555627526));
#188627=CARTESIAN_POINT('Ctrl Pts',(4.15748915962667,-5.33924834481285,
22.4077824112565));
#188628=CARTESIAN_POINT('Ctrl Pts',(4.29909208511144,-5.22898701406836,
22.4162066586931));
#188629=CARTESIAN_POINT('Ctrl Pts',(4.4363392422887,-5.11306313357175,22.4246309061297));
#188630=CARTESIAN_POINT('Ctrl Pts',(4.56877511030842,-4.9918516595975,22.4330551535663));
#188631=CARTESIAN_POINT('Ctrl Pts',(4.60609047084215,-4.95769890385387,
22.4354287841773));
#188632=CARTESIAN_POINT('Ctrl Pts',(4.64302406530954,-4.92312661393061,
22.4378024147883));
#188633=CARTESIAN_POINT('Ctrl Pts',(4.67956618893992,-4.88814374618119,
22.4401760453993));
#188634=CARTESIAN_POINT('Ctrl Pts',(4.81225261331216,-4.76111906412091,
22.4487948263365));
#188635=CARTESIAN_POINT('Ctrl Pts',(4.93971555115588,-4.62873506524635,
22.4574136072737));
#188636=CARTESIAN_POINT('Ctrl Pts',(5.06153999065129,-4.49144764224606,
22.466032388211));
#188637=CARTESIAN_POINT('Ctrl Pts',(5.18343760934638,-4.35407775152597,
22.4746563463975));
#188638=CARTESIAN_POINT('Ctrl Pts',(5.29968976835802,-4.21179878595593,
22.483280304584));
#188639=CARTESIAN_POINT('Ctrl Pts',(5.4099216612736,-4.06509982889507,22.4919042627705));
#188640=CARTESIAN_POINT('Ctrl Pts',(5.52413585637278,-3.91310113904741,
22.5008397751416));
#188641=CARTESIAN_POINT('Ctrl Pts',(5.63188647995301,-3.75635743750224,
22.5097752875127));
#188642=CARTESIAN_POINT('Ctrl Pts',(5.73280591916584,-3.59544507581149,
22.5187107998839));
#188643=CARTESIAN_POINT('Ctrl Pts',(5.83038870830528,-3.43985288085604,
22.5273508817785));
#188644=CARTESIAN_POINT('Ctrl Pts',(5.92158468450929,-3.28036355404071,
22.5359909636732));
#188645=CARTESIAN_POINT('Ctrl Pts',(6.00610837780384,-3.11752324034233,
22.5446310455679));
#188646=CARTESIAN_POINT('Ctrl Pts',(6.09496725135797,-2.94633092395816,
22.5537142731773));
#188647=CARTESIAN_POINT('Ctrl Pts',(6.17645126152661,-2.77143520727055,
22.5627975007866));
#188648=CARTESIAN_POINT('Ctrl Pts',(6.25028584452666,-2.59349491260532,
22.571880728396));
#188649=CARTESIAN_POINT('Ctrl Pts',(6.32412042752671,-2.41555461794009,
22.5809639560053));
#188650=CARTESIAN_POINT('Ctrl Pts',(6.39030548178426,-2.23457012104382,
22.5900471836147));
#188651=CARTESIAN_POINT('Ctrl Pts',(6.44862675758667,-2.05121962289202,
22.599130411224));
#188652=CARTESIAN_POINT('Ctrl Pts',(6.50669998155796,-1.86864895039006,
22.6081750060838));
#188653=CARTESIAN_POINT('Ctrl Pts',(6.5570306414638,-1.68356402629343,22.6172196009436));
#188654=CARTESIAN_POINT('Ctrl Pts',(6.59942801012511,-1.49660914709759,
22.6262641958035));
#188655=CARTESIAN_POINT('Ctrl Pts',(6.64178647252687,-1.30982582843211,
22.6353004908238));
#188656=CARTESIAN_POINT('Ctrl Pts',(6.67622612575914,-1.12117621242904,
22.6443367858441));
#188657=CARTESIAN_POINT('Ctrl Pts',(6.70260675191163,-0.931317201187977,
22.6533730808644));
#188658=CARTESIAN_POINT('Ctrl Pts',(6.72894069547753,-0.741794160354964,
22.6623933854521));
#188659=CARTESIAN_POINT('Ctrl Pts',(6.74724405682532,-0.551066233153369,
22.6714136900398));
#188660=CARTESIAN_POINT('Ctrl Pts',(6.75742810502057,-0.359797728561595,
22.6804339946275));
#188661=CARTESIAN_POINT('Ctrl Pts',(6.76759932838547,-0.168770089495615,
22.6894429398939));
#188662=CARTESIAN_POINT('Ctrl Pts',(6.76967163096781,0.0227965315663232,
22.6984518851602));
#188663=CARTESIAN_POINT('Ctrl Pts',(6.76360800458227,0.214232958133704,
22.7074608304266));
#188664=CARTESIAN_POINT('Ctrl Pts',(6.7575581474086,0.40523467310241,22.7164493182854));
#188665=CARTESIAN_POINT('Ctrl Pts',(6.74340924642376,0.596106546372357,
22.7254378061442));
#188666=CARTESIAN_POINT('Ctrl Pts',(6.72117622024647,0.786180142456833,
22.734426294003));
#188667=CARTESIAN_POINT('Ctrl Pts',(6.70166979969549,0.952943563292714,
22.7423124550182));
#188668=CARTESIAN_POINT('Ctrl Pts',(6.67594125548238,1.11909233995013,22.7501986160335));
#188669=CARTESIAN_POINT('Ctrl Pts',(6.64403371932614,1.28417480759331,22.7580847770488));
#188670=CARTESIAN_POINT('Ctrl Pts',(6.61117413998988,1.45418293407427,22.766206241905));
#188671=CARTESIAN_POINT('Ctrl Pts',(6.57177443920997,1.62298375675467,22.7743277067611));
#188672=CARTESIAN_POINT('Ctrl Pts',(6.52595244571703,1.79003733934237,22.7824491716173));
#188673=CARTESIAN_POINT('Ctrl Pts',(6.48013372000638,1.95707900855186,22.7905700572936));
#188674=CARTESIAN_POINT('Ctrl Pts',(6.42789371072715,2.12237333271924,22.7986909429698));
#188675=CARTESIAN_POINT('Ctrl Pts',(6.36940060920412,2.28539381277498,22.806811828646));
#188676=CARTESIAN_POINT('Ctrl Pts',(6.31090051608323,2.44843377843862,22.8149336850003));
#188677=CARTESIAN_POINT('Ctrl Pts',(6.24614596722672,2.60919901453646,22.8230555413545));
#188678=CARTESIAN_POINT('Ctrl Pts',(6.1753539321172,2.76718138420392,22.8311773977088));
#188679=CARTESIAN_POINT('Ctrl Pts',(6.10451024801452,2.9252790158541,22.839305179669));
#188680=CARTESIAN_POINT('Ctrl Pts',(6.02762042981907,3.08058939140805,22.8474329616291));
#188681=CARTESIAN_POINT('Ctrl Pts',(5.94494848823246,3.23262686870331,22.8555607435893));
#188682=CARTESIAN_POINT('Ctrl Pts',(5.86224286916956,3.38472628041598,22.8636918365058));
#188683=CARTESIAN_POINT('Ctrl Pts',(5.77375061871918,3.53354982178732,22.8718229294222));
#188684=CARTESIAN_POINT('Ctrl Pts',(5.67977988231148,3.67863962471044,22.8799540223387));
#188685=CARTESIAN_POINT('Ctrl Pts',(5.58570658077237,3.82388778708964,22.8880939900032));
#188686=CARTESIAN_POINT('Ctrl Pts',(5.48614306060679,3.96539377232738,22.8962339576678));
#188687=CARTESIAN_POINT('Ctrl Pts',(5.38143910172155,4.1027310653347,22.9043739253323));
#188688=CARTESIAN_POINT('Ctrl Pts',(5.3271351015356,4.17396012357099,22.9085956645127));
#188689=CARTESIAN_POINT('Ctrl Pts',(5.27144901479941,4.24406840679247,22.9128174036931));
#188690=CARTESIAN_POINT('Ctrl Pts',(5.21443360200505,4.3130002562347,22.9170391428736));
#188691=CARTESIAN_POINT('Ctrl Pts',(5.10043797033807,4.45082140553485,22.9254800152801));
#188692=CARTESIAN_POINT('Ctrl Pts',(4.98089045055199,4.58422245634782,22.9339208876866));
#188693=CARTESIAN_POINT('Ctrl Pts',(4.85616084904731,4.71274769197123,22.9423617600932));
#188694=CARTESIAN_POINT('Ctrl Pts',(4.72888071563014,4.84390107449051,22.9509752355882));
#188695=CARTESIAN_POINT('Ctrl Pts',(4.59620447748548,4.96997679336693,22.9595887110832));
#188696=CARTESIAN_POINT('Ctrl Pts',(4.45856823506176,5.09052632772863,22.9682021865782));
#188697=CARTESIAN_POINT('Ctrl Pts',(4.32388824965514,5.2084866065237,22.9766306552253));
#188698=CARTESIAN_POINT('Ctrl Pts',(4.18445941432856,5.32115543001297,22.9850591238723));
#188699=CARTESIAN_POINT('Ctrl Pts',(4.0407274065947,5.42814987132766,22.9934875925194));
#188700=CARTESIAN_POINT('Ctrl Pts',(3.89226297234072,5.53866714196594,23.0021935714383));
#188701=CARTESIAN_POINT('Ctrl Pts',(3.73920742249339,5.64312973429293,23.0108995503573));
#188702=CARTESIAN_POINT('Ctrl Pts',(3.58208886976396,5.74116088688631,23.0196055292763));
#188703=CARTESIAN_POINT('Ctrl Pts',(3.42497031703453,5.83919203947969,23.0283115081953));
#188704=CARTESIAN_POINT('Ctrl Pts',(3.26378908609646,5.9307915306607,23.0370174871142));
#188705=CARTESIAN_POINT('Ctrl Pts',(3.09910619832133,6.01563211736941,23.0457234660332));
#188706=CARTESIAN_POINT('Ctrl Pts',(3.09910619832133,6.01563211736941,21.0459783413229));
#188707=CARTESIAN_POINT('Ctrl Pts',(2.94382747564148,6.09562790875683,21.0542049202976));
#188708=CARTESIAN_POINT('Ctrl Pts',(2.78528255985401,6.16969361804676,21.0624314992722));
#188709=CARTESIAN_POINT('Ctrl Pts',(2.62396313098396,6.23755613098887,21.0706580782469));
#188710=CARTESIAN_POINT('Ctrl Pts',(2.46280817665563,6.30534945415147,21.0788762697457));
#188711=CARTESIAN_POINT('Ctrl Pts',(2.29888467345399,6.36695204846957,21.0870944612445));
#188712=CARTESIAN_POINT('Ctrl Pts',(2.13270787261217,6.42213719334133,21.0953126527434));
#188713=CARTESIAN_POINT('Ctrl Pts',(1.96663049601534,6.47728932072006,21.1035259272654));
#188714=CARTESIAN_POINT('Ctrl Pts',(1.79830284291209,6.52603153246958,21.1117392017873));
#188715=CARTESIAN_POINT('Ctrl Pts',(1.62825953586144,6.56818543312202,21.1199524763093));
#188716=CARTESIAN_POINT('Ctrl Pts',(1.45828312583814,6.61032274993653,21.128162519633));
#188717=CARTESIAN_POINT('Ctrl Pts',(1.28659275059701,6.64587683065302,21.1363725629566));
#188718=CARTESIAN_POINT('Ctrl Pts',(1.11373770206829,6.67471926982638,21.1445826062802));
#188719=CARTESIAN_POINT('Ctrl Pts',(0.945596086519667,6.7027752297781,21.1525687771206));
#188720=CARTESIAN_POINT('Ctrl Pts',(0.776352808330789,6.72448073582025,
21.1605549479609));
#188721=CARTESIAN_POINT('Ctrl Pts',(0.606522686664242,6.73976403374492,
21.1685411188012));
#188722=CARTESIAN_POINT('Ctrl Pts',(0.418129816635969,6.75671782457585,
21.1774001929771));
#188723=CARTESIAN_POINT('Ctrl Pts',(0.229210887468987,6.7657516186024,21.186259267153));
#188724=CARTESIAN_POINT('Ctrl Pts',(0.0404191399853253,6.76687928761278,
21.1951183413288));
#188725=CARTESIAN_POINT('Ctrl Pts',(-0.148727309209687,6.76800907528636,
21.2039940599228));
#188726=CARTESIAN_POINT('Ctrl Pts',(-0.337745839968023,6.7612030514985,
21.2128697785167));
#188727=CARTESIAN_POINT('Ctrl Pts',(-0.525986565538072,6.74652704232878,
21.2217454971107));
#188728=CARTESIAN_POINT('Ctrl Pts',(-0.714764476951838,6.73180915197556,
21.2306465444977));
#188729=CARTESIAN_POINT('Ctrl Pts',(-0.902759881300691,6.70917635351106,
21.2395475918846));
#188730=CARTESIAN_POINT('Ctrl Pts',(-1.08932826356542,6.67874635947478,
21.2484486392716));
#188731=CARTESIAN_POINT('Ctrl Pts',(-1.27615028810489,6.64827499544421,
21.2573617877546));
#188732=CARTESIAN_POINT('Ctrl Pts',(-1.4615411604175,6.60998530905217,21.2662749362377));
#188733=CARTESIAN_POINT('Ctrl Pts',(-1.64486848209565,6.56404575521898,
21.2751880847207));
#188734=CARTESIAN_POINT('Ctrl Pts',(-1.82860284055769,6.51800420301439,
21.2841210228305));
#188735=CARTESIAN_POINT('Ctrl Pts',(-2.01026423175698,6.46427887393469,
21.2930539609404));
#188736=CARTESIAN_POINT('Ctrl Pts',(-2.18923453205078,6.40308840823524,
21.3019868990503));
#188737=CARTESIAN_POINT('Ctrl Pts',(-2.3595883083182,6.34484395713719,21.3104897609089));
#188738=CARTESIAN_POINT('Ctrl Pts',(-2.52750384596131,6.27983632908412,
21.3189926227674));
#188739=CARTESIAN_POINT('Ctrl Pts',(-2.69246653831701,6.2082938831891,21.327495484626));
#188740=CARTESIAN_POINT('Ctrl Pts',(-2.85199431731393,6.13910849748365,
21.3357182084918));
#188741=CARTESIAN_POINT('Ctrl Pts',(-3.00906597722489,6.06367828421869,
21.3439409323577));
#188742=CARTESIAN_POINT('Ctrl Pts',(-3.16315895579046,5.98219979776692,
21.3521636562236));
#188743=CARTESIAN_POINT('Ctrl Pts',(-3.31708883215837,5.90080755353285,
21.3603776766148));
#188744=CARTESIAN_POINT('Ctrl Pts',(-3.46804599099936,5.81337995062288,
21.368591697006));
#188745=CARTESIAN_POINT('Ctrl Pts',(-3.61552752086404,5.72016168878772,
21.3768057173973));
#188746=CARTESIAN_POINT('Ctrl Pts',(-3.76288255664704,5.62702337973334,
21.3850126926692));
#188747=CARTESIAN_POINT('Ctrl Pts',(-3.90676759891499,5.5281044937726,21.3932196679412));
#188748=CARTESIAN_POINT('Ctrl Pts',(-4.04670396952207,5.42369578636693,
21.4014266432131));
#188749=CARTESIAN_POINT('Ctrl Pts',(-4.18654840472603,5.31935567339859,
21.4096282266661));
#188750=CARTESIAN_POINT('Ctrl Pts',(-4.32244904911747,5.20953313685444,
21.4178298101191));
#188751=CARTESIAN_POINT('Ctrl Pts',(-4.45395581245558,5.094562456256,21.4260313935721));
#188752=CARTESIAN_POINT('Ctrl Pts',(-4.58540256836945,4.97964423755557,
21.4342292345871));
#188753=CARTESIAN_POINT('Ctrl Pts',(-4.71245916808593,4.85958279046807,
21.4424270756022));
#188754=CARTESIAN_POINT('Ctrl Pts',(-4.83470819332551,4.73475296983815,
21.4506249166172));
#188755=CARTESIAN_POINT('Ctrl Pts',(-4.95694643046984,4.60993416505063,
21.4588220341984));
#188756=CARTESIAN_POINT('Ctrl Pts',(-5.07437768126029,4.48034807498078,
21.4670191517796));
#188757=CARTESIAN_POINT('Ctrl Pts',(-5.18662078474238,4.34640700294834,
21.4752162693607));
#188758=CARTESIAN_POINT('Ctrl Pts',(-5.29886263939499,4.21246742115944,
21.4834132957398));
#188759=CARTESIAN_POINT('Ctrl Pts',(-5.40591623041273,4.07417322825725,
21.4916103221189));
#188760=CARTESIAN_POINT('Ctrl Pts',(-5.5074402518264,3.93197035499537,21.499807348498));
#188761=CARTESIAN_POINT('Ctrl Pts',(-5.6089816038196,3.78974320710201,21.5080057741441));
#188762=CARTESIAN_POINT('Ctrl Pts',(-5.70499129713191,3.64360634158288,
21.5162041997903));
#188763=CARTESIAN_POINT('Ctrl Pts',(-5.79517095851232,3.49403528339589,
21.5244026254364));
#188764=CARTESIAN_POINT('Ctrl Pts',(-5.88538241151737,3.34441149594749,
21.5326039413271));
#188765=CARTESIAN_POINT('Ctrl Pts',(-5.96975955324907,3.19135141125988,
21.5408052572177));
#188766=CARTESIAN_POINT('Ctrl Pts',(-6.04804960264305,3.0353558282299,21.5490065731084));
#188767=CARTESIAN_POINT('Ctrl Pts',(-6.126428811298,2.87918259234359,21.557217228925));
#188768=CARTESIAN_POINT('Ctrl Pts',(-6.19870691723301,2.72006750035543,
21.5654278847415));
#188769=CARTESIAN_POINT('Ctrl Pts',(-6.26467858903202,2.55853301251396,
21.5736385405581));
#188770=CARTESIAN_POINT('Ctrl Pts',(-6.33068913633892,2.39690333631233,
21.5818540347153));
#188771=CARTESIAN_POINT('Ctrl Pts',(-6.39038571927823,2.23285175900436,
21.5900695288724));
#188772=CARTESIAN_POINT('Ctrl Pts',(-6.44361273654199,2.06691652019957,
21.5982850230296));
#188773=CARTESIAN_POINT('Ctrl Pts',(-6.49692233650246,1.90072382981839,
21.6065132636771));
#188774=CARTESIAN_POINT('Ctrl Pts',(-6.54374221538474,1.7326419830069,21.6147415043246));
#188775=CARTESIAN_POINT('Ctrl Pts',(-6.58396749668861,1.56322135430268,
21.6229697449721));
#188776=CARTESIAN_POINT('Ctrl Pts',(-6.62052585538449,1.40924505099579,
21.6304479020732));
#188777=CARTESIAN_POINT('Ctrl Pts',(-6.65163775084048,1.25416323714382,
21.6379260591743));
#188778=CARTESIAN_POINT('Ctrl Pts',(-6.67726167823053,1.09839222522469,
21.6454042162755));
#188779=CARTESIAN_POINT('Ctrl Pts',(-6.72073983845508,0.834083131951578,
21.6580930015533));
#188780=CARTESIAN_POINT('Ctrl Pts',(-6.74855195933655,0.56700790866886,
21.6707817868311));
#188781=CARTESIAN_POINT('Ctrl Pts',(-6.7604070780163,0.29863881111992,21.683470572109));
#188782=CARTESIAN_POINT('Ctrl Pts',(-6.76467657868595,0.201988404434906,
21.6880403093427));
#188783=CARTESIAN_POINT('Ctrl Pts',(-6.76687673293707,0.105170525308029,
21.6926100465764));
#188784=CARTESIAN_POINT('Ctrl Pts',(-6.7669949644283,0.00825538624319681,
21.6971797838101));
#188785=CARTESIAN_POINT('',(-6.767,9.7407047434505E-13,21.3028202161899));
#188786=CARTESIAN_POINT('Ctrl Pts',(3.09910619832131,6.01563211736942,20.6513174420499));
#188787=CARTESIAN_POINT('Ctrl Pts',(2.9420188085974,6.09655968967987,20.6596250383763));
#188788=CARTESIAN_POINT('Ctrl Pts',(2.78183949938961,6.17128913350124,20.6679326347026));
#188789=CARTESIAN_POINT('Ctrl Pts',(2.61909714245077,6.23960088133899,20.676240231029));
#188790=CARTESIAN_POINT('Ctrl Pts',(2.45618547297322,6.30798369878435,20.6845564703433));
#188791=CARTESIAN_POINT('Ctrl Pts',(2.29070575261917,6.36993535452906,20.6928727096575));
#188792=CARTESIAN_POINT('Ctrl Pts',(2.12320456495112,6.42528531470554,20.7011889489718));
#188793=CARTESIAN_POINT('Ctrl Pts',(2.02142093381408,6.45891922505858,20.7062423879748));
#188794=CARTESIAN_POINT('Ctrl Pts',(1.91889116698867,6.49011643561359,20.7112958269778));
#188795=CARTESIAN_POINT('Ctrl Pts',(1.81573999407531,6.51884784865511,20.7163492659808));
#188796=CARTESIAN_POINT('Ctrl Pts',(1.64325248018074,6.56689199460364,20.7247995347042));
#188797=CARTESIAN_POINT('Ctrl Pts',(1.46871052826714,6.60812677290956,20.7332498034276));
#188798=CARTESIAN_POINT('Ctrl Pts',(1.29267795625606,6.64238456440228,20.7417000721509));
#188799=CARTESIAN_POINT('Ctrl Pts',(1.11680073896188,6.67661212223178,20.7501428832254));
#188800=CARTESIAN_POINT('Ctrl Pts',(0.939435847604214,6.7038749030657,20.7585856942999));
#188801=CARTESIAN_POINT('Ctrl Pts',(0.761160312578012,6.72405561982916,
20.7670285053745));
#188802=CARTESIAN_POINT('Ctrl Pts',(0.583017839087675,6.74422127408185,
20.7754650148922));
#188803=CARTESIAN_POINT('Ctrl Pts',(0.40396640524696,6.7573153642745,20.7839015244099));
#188804=CARTESIAN_POINT('Ctrl Pts',(0.224591636110605,6.76327195941352,
20.7923380339276));
#188805=CARTESIAN_POINT('Ctrl Pts',(0.0453452192734122,6.7692242922882,
20.8007685066689));
#188806=CARTESIAN_POINT('Ctrl Pts',(-0.134223740770821,6.76804930638651,
20.8091989794101));
#188807=CARTESIAN_POINT('Ctrl Pts',(-0.313525903762525,6.75973302044318,
20.8176294521513));
#188808=CARTESIAN_POINT('Ctrl Pts',(-0.492750985240562,6.75142030964863,
20.8260563006551));
#188809=CARTESIAN_POINT('Ctrl Pts',(-0.671709167696662,6.73597243434907,
20.834483149159));
#188810=CARTESIAN_POINT('Ctrl Pts',(-0.84981185785603,6.71342750063239,
20.8429099976628));
#188811=CARTESIAN_POINT('Ctrl Pts',(-1.02785957407512,6.69088952573166,
20.8513342450994));
#188812=CARTESIAN_POINT('Ctrl Pts',(-1.20505199602207,6.66125890259825,
20.8597584925361));
#188813=CARTESIAN_POINT('Ctrl Pts',(-1.38080602384894,6.6246255535315,20.8681827399727));
#188814=CARTESIAN_POINT('Ctrl Pts',(-1.43032678443763,6.61430367737806,
20.8705563705837));
#188815=CARTESIAN_POINT('Ctrl Pts',(-1.47973339825789,6.60342617115657,
20.8729300011946));
#188816=CARTESIAN_POINT('Ctrl Pts',(-1.52901294840639,6.59199578303913,
20.8753036318056));
#188817=CARTESIAN_POINT('Ctrl Pts',(-1.70794965635648,6.55049142648222,
20.8839224127428));
#188818=CARTESIAN_POINT('Ctrl Pts',(-1.88513012267368,6.5017122707146,20.89254119368));
#188819=CARTESIAN_POINT('Ctrl Pts',(-2.05996476989152,6.44583851386348,
20.9011599746173));
#188820=CARTESIAN_POINT('Ctrl Pts',(-2.23490443921883,6.38993119398638,
20.9097839328038));
#188821=CARTESIAN_POINT('Ctrl Pts',(-2.40749518753538,6.32692086059346,
20.9184078909903));
#188822=CARTESIAN_POINT('Ctrl Pts',(-2.57716506940687,6.25703677510602,
20.9270318491768));
#188823=CARTESIAN_POINT('Ctrl Pts',(-2.75296454520189,6.18462801605229,
20.935967361548));
#188824=CARTESIAN_POINT('Ctrl Pts',(-2.92562784627793,6.10483973798158,
20.9449028739191));
#188825=CARTESIAN_POINT('Ctrl Pts',(-3.09454466900673,6.01797991783971,
20.9538383862902));
#188826=CARTESIAN_POINT('Ctrl Pts',(-3.25787667741909,5.93399190146027,
20.9624784681849));
#188827=CARTESIAN_POINT('Ctrl Pts',(-3.41770573619125,5.84339265523882,
20.9711185500796));
#188828=CARTESIAN_POINT('Ctrl Pts',(-3.5735075963264,5.7465061088454,20.9797586319743));
#188829=CARTESIAN_POINT('Ctrl Pts',(-3.73730046019193,5.6446502973034,20.9888418595836));
#188830=CARTESIAN_POINT('Ctrl Pts',(-3.89664184339482,5.53584552154564,
20.997925087193));
#188831=CARTESIAN_POINT('Ctrl Pts',(-4.05095936177605,5.42051817165472,
21.0070083148023));
#188832=CARTESIAN_POINT('Ctrl Pts',(-4.2052768801573,5.30519082176379,21.0160915424117));
#188833=CARTESIAN_POINT('Ctrl Pts',(-4.35457025457998,5.18334116900584,
21.025174770021));
#188834=CARTESIAN_POINT('Ctrl Pts',(-4.49830907481029,5.05544305352948,
21.0342579976303));
#188835=CARTESIAN_POINT('Ctrl Pts',(-4.64143654563083,4.92808891383698,
21.0433025924902));
#188836=CARTESIAN_POINT('Ctrl Pts',(-4.77918936808601,4.7946206990437,21.05234718735));
#188837=CARTESIAN_POINT('Ctrl Pts',(-4.91107466523752,4.65549510068072,
21.0613917822098));
#188838=CARTESIAN_POINT('Ctrl Pts',(-5.04283893686909,4.51649717195373,
21.0704280772301));
#188839=CARTESIAN_POINT('Ctrl Pts',(-5.16874626961175,4.37185239709217,
21.0794643722505));
#188840=CARTESIAN_POINT('Ctrl Pts',(-5.28834078624878,4.22205408876978,
21.0885006672708));
#188841=CARTESIAN_POINT('Ctrl Pts',(-5.40772367101038,4.0725208603007,21.0975209718586));
#188842=CARTESIAN_POINT('Ctrl Pts',(-5.52081589854251,3.9178524946821,21.1065412764463));
#188843=CARTESIAN_POINT('Ctrl Pts',(-5.62720208567325,3.75857495428715,
21.115561581034));
#188844=CARTESIAN_POINT('Ctrl Pts',(-5.73345430006742,3.59949799301376,
21.1245705263003));
#188845=CARTESIAN_POINT('Ctrl Pts',(-5.83301719554953,3.43582363770394,
21.1335794715666));
#188846=CARTESIAN_POINT('Ctrl Pts',(-5.92551738190147,3.26810843712132,
21.142588416833));
#188847=CARTESIAN_POINT('Ctrl Pts',(-6.01780751991234,3.1007740822542,21.1515769046918));
#188848=CARTESIAN_POINT('Ctrl Pts',(-6.10306684718191,2.92941740593767,
21.1605653925506));
#188849=CARTESIAN_POINT('Ctrl Pts',(-6.18096700465798,2.75462082460171,
21.1695538804094));
#188850=CARTESIAN_POINT('Ctrl Pts',(-6.24931367148559,2.60126088164081,
21.1774400414246));
#188851=CARTESIAN_POINT('Ctrl Pts',(-6.3119960736473,2.44525354068808,21.1853262024399));
#188852=CARTESIAN_POINT('Ctrl Pts',(-6.36882075883218,2.28700921333262,
21.1932123634551));
#188853=CARTESIAN_POINT('Ctrl Pts',(-6.42522204905894,2.12994394838879,
21.2010397654856));
#188854=CARTESIAN_POINT('Ctrl Pts',(-6.47584228433969,1.97069819679649,
21.208867167516));
#188855=CARTESIAN_POINT('Ctrl Pts',(-6.52050999703648,1.80976196737233,
21.2166945695465));
#188856=CARTESIAN_POINT('Ctrl Pts',(-6.56517995872835,1.6488176348964,21.2245223656824));
#188857=CARTESIAN_POINT('Ctrl Pts',(-6.60389668221933,1.48618302928765,
21.2323501618183));
#188858=CARTESIAN_POINT('Ctrl Pts',(-6.63653857191159,1.32236333264716,
21.2401779579542));
#188859=CARTESIAN_POINT('Ctrl Pts',(-6.66918049363267,1.15854347526379,
21.2480057617708));
#188860=CARTESIAN_POINT('Ctrl Pts',(-6.69574750043971,0.993538910979629,
21.2558335655875));
#188861=CARTESIAN_POINT('Ctrl Pts',(-6.71616928443157,0.827864205566292,
21.2636613694042));
#188862=CARTESIAN_POINT('Ctrl Pts',(-6.73660316178977,0.662091390952241,
21.2714938086875));
#188863=CARTESIAN_POINT('Ctrl Pts',(-6.75088450933278,0.495648033274671,
21.2793262479709));
#188864=CARTESIAN_POINT('Ctrl Pts',(-6.75899497096985,0.329053160453232,
21.2871586872542));
#188865=CARTESIAN_POINT('Ctrl Pts',(-6.76433416341804,0.21938220377068,
21.2923148549971));
#188866=CARTESIAN_POINT('Ctrl Pts',(-6.76700014338094,0.109645646085917,
21.2974710227399));
#188867=CARTESIAN_POINT('Ctrl Pts',(-6.76699999999422,-8.84868392606215E-6,
21.3026271904827));
#188868=CARTESIAN_POINT('Ctrl Pts',(-6.767,9.7407047898921E-13,21.3028202161899));
#188869=CARTESIAN_POINT('Ctrl Pts',(-6.76700000000003,-0.186007249526034,
21.3115697280011));
#188870=CARTESIAN_POINT('Ctrl Pts',(-6.75932637294525,-0.372014355749215,
21.3203192398123));
#188871=CARTESIAN_POINT('Ctrl Pts',(-6.74400518264185,-0.557389537486927,
21.3290687516235));
#188872=CARTESIAN_POINT('Ctrl Pts',(-6.7286840570509,-0.742763936251391,
21.3378182264791));
#188873=CARTESIAN_POINT('Ctrl Pts',(-6.70571545645729,-0.927506130242027,
21.3465677013348));
#188874=CARTESIAN_POINT('Ctrl Pts',(-6.67517739404803,-1.11098863990153,
21.3553171761905));
#188875=CARTESIAN_POINT('Ctrl Pts',(-6.64463945808673,-1.29447038982095,
21.3640666148175));
#188876=CARTESIAN_POINT('Ctrl Pts',(-6.6065321700832,-1.47669218313842,
21.3728160534445));
#188877=CARTESIAN_POINT('Ctrl Pts',(-6.56098496092634,-1.65703510599455,
21.3815654920715));
#188878=CARTESIAN_POINT('Ctrl Pts',(-6.51543793658252,-1.83737729708858,
21.3903148951967));
#188879=CARTESIAN_POINT('Ctrl Pts',(-6.46245112167374,-2.01584035511074,
21.3990642983219));
#188880=CARTESIAN_POINT('Ctrl Pts',(-6.40220448374207,-2.19181813760928,
21.407813701447));
#188881=CARTESIAN_POINT('Ctrl Pts',(-6.34195808526455,-2.36779522067275,
21.4165630697971));
#188882=CARTESIAN_POINT('Ctrl Pts',(-6.27445201433053,-2.54128677684292,
21.4253124381472));
#188883=CARTESIAN_POINT('Ctrl Pts',(-6.19991555071849,-2.71170355384933,
21.4340618064973));
#188884=CARTESIAN_POINT('Ctrl Pts',(-6.12537937716646,-2.88211966767575,
21.4428111407991));
#188885=CARTESIAN_POINT('Ctrl Pts',(-6.04381298052481,-3.04946076371861,
21.4515604751009));
#188886=CARTESIAN_POINT('Ctrl Pts',(-5.95549339335802,-3.21315848374601,
21.4603098094026));
#188887=CARTESIAN_POINT('Ctrl Pts',(-5.86717414255374,-3.37685558033555,
21.4690591103828));
#188888=CARTESIAN_POINT('Ctrl Pts',(-5.77210188876556,-3.53690907646826,
21.477808411363));
#188889=CARTESIAN_POINT('Ctrl Pts',(-5.67059953346946,-3.69277536969363,
21.4865577123432));
#188890=CARTESIAN_POINT('Ctrl Pts',(-5.56909755631333,-3.84864108224997,
21.4953069807285));
#188891=CARTESIAN_POINT('Ctrl Pts',(-5.46116568196798,-4.00031938297587,
21.5040562491138));
#188892=CARTESIAN_POINT('Ctrl Pts',(-5.34717048533551,-4.14729511859921,
21.512805517499));
#188893=CARTESIAN_POINT('Ctrl Pts',(-5.23317570391784,-4.2942703188798,
21.5215547540161));
#188894=CARTESIAN_POINT('Ctrl Pts',(-5.11311782003462,-4.43654276189607,
21.5303039905331));
#188895=CARTESIAN_POINT('Ctrl Pts',(-4.98740458984701,-4.57362924351909,
21.5390532270502));
#188896=CARTESIAN_POINT('Ctrl Pts',(-4.86169180711693,-4.71071523720318,
21.5478024324256));
#188897=CARTESIAN_POINT('Ctrl Pts',(-4.73032391204123,-4.84261509523285,
21.556551637801));
#188898=CARTESIAN_POINT('Ctrl Pts',(-4.59374707013553,-4.96888084538372,
21.5653008431765));
#188899=CARTESIAN_POINT('Ctrl Pts',(-4.45717070301427,-5.09514615659478,
21.5740500181369));
#188900=CARTESIAN_POINT('Ctrl Pts',(-4.31538563571052,-5.21577720459517,
21.5827991930973));
#188901=CARTESIAN_POINT('Ctrl Pts',(-4.16887341029552,-5.33036429232853,
21.5915483680578));
#188902=CARTESIAN_POINT('Ctrl Pts',(-4.02236168203746,-5.44495099123586,
21.6002975133298));
#188903=CARTESIAN_POINT('Ctrl Pts',(-3.87112305348203,-5.55349359438575,
21.6090466586018));
#188904=CARTESIAN_POINT('Ctrl Pts',(-3.71567117017795,-5.65562346298871,
21.6177958038738));
#188905=CARTESIAN_POINT('Ctrl Pts',(-3.5602198014585,-5.75775299351625,
21.626544920184));
#188906=CARTESIAN_POINT('Ctrl Pts',(-3.40055544538377,-5.85346967463857,
21.6352940364942));
#188907=CARTESIAN_POINT('Ctrl Pts',(-3.23722035986878,-5.94244842986888,
21.6440431528043));
#188908=CARTESIAN_POINT('Ctrl Pts',(-3.07388580147188,-6.03142689794526,
21.6527922408792));
#188909=CARTESIAN_POINT('Ctrl Pts',(-2.90688078896568,-6.11366734656787,
21.6615413289541));
#188910=CARTESIAN_POINT('Ctrl Pts',(-2.73677250721342,-6.18889046952366,
21.6702904170289));
#188911=CARTESIAN_POINT('Ctrl Pts',(-2.56666476031447,-6.26411335596342,
21.6790394775949));
#188912=CARTESIAN_POINT('Ctrl Pts',(-2.39345402575123,-6.33231884500572,
21.687788538161));
#188913=CARTESIAN_POINT('Ctrl Pts',(-2.2177285606554,-6.39327529762745,
21.696537598727));
#188914=CARTESIAN_POINT('Ctrl Pts',(-2.04200363348465,-6.45423156365126,
21.7052866325107));
#188915=CARTESIAN_POINT('Ctrl Pts',(-1.86376426189232,-6.50793874375671,
21.7140356662944));
#188916=CARTESIAN_POINT('Ctrl Pts',(-1.68361577753111,-6.55421443909553,
21.7227847000781));
#188917=CARTESIAN_POINT('Ctrl Pts',(-1.50346782967731,-6.60048999661884,
21.7315337078059));
#188918=CARTESIAN_POINT('Ctrl Pts',(-1.32141105794894,-6.63933404237732,
21.7402827155338));
#188919=CARTESIAN_POINT('Ctrl Pts',(-1.13806375486904,-6.67061465607581,
21.7490317232616));
#188920=CARTESIAN_POINT('Ctrl Pts',(-0.954716982601926,-6.70189517921312,
21.75778070566));
#188921=CARTESIAN_POINT('Ctrl Pts',(-0.770079968901146,-6.72561226592239,
21.7665296880584));
#188922=CARTESIAN_POINT('Ctrl Pts',(-0.584779765557352,-6.7416853698311,
21.7752786704568));
#188923=CARTESIAN_POINT('Ctrl Pts',(-0.391489830650432,-6.75845151013858,
21.7844048894667));
#188924=CARTESIAN_POINT('Ctrl Pts',(-0.197478578237495,-6.76689983031628,
21.7935311084765));
#188925=CARTESIAN_POINT('Ctrl Pts',(-0.00346287645053296,-6.76699911397118,
21.8026573274864));
#188926=CARTESIAN_POINT('Ctrl Pts',(0.184489834655586,-6.76709529501186,
21.8114983521522));
#188927=CARTESIAN_POINT('Ctrl Pts',(0.37244640425106,-6.75935639738159,
21.820339376818));
#188928=CARTESIAN_POINT('Ctrl Pts',(0.559755019490015,-6.74380925873173,
21.8291804014838));
#188929=CARTESIAN_POINT('Ctrl Pts',(0.745134705523545,-6.72842222659786,
21.8379303800936));
#188930=CARTESIAN_POINT('Ctrl Pts',(0.929879431230425,-6.70538706057498,
21.8466803587033));
#188931=CARTESIAN_POINT('Ctrl Pts',(1.1133616362702,-6.67478200894095,21.8554303373131));
#188932=CARTESIAN_POINT('Ctrl Pts',(1.2968419630093,-6.64417727060972,21.8641802263496));
#188933=CARTESIAN_POINT('Ctrl Pts',(1.47905951217738,-6.6060028489054,21.8729301153861));
#188934=CARTESIAN_POINT('Ctrl Pts',(1.65939532067327,-6.56038841607169,
21.8816800044227));
#188935=CARTESIAN_POINT('Ctrl Pts',(1.83972934301042,-6.51477443503189,
21.8904298067948));
#188936=CARTESIAN_POINT('Ctrl Pts',(2.01818138406502,-6.46172066062067,
21.899179609167));
#188937=CARTESIAN_POINT('Ctrl Pts',(2.19414528354434,-6.40140730423398,
21.9079294115391));
#188938=CARTESIAN_POINT('Ctrl Pts',(2.37010749864218,-6.3410945251856,21.9166791301554));
#188939=CARTESIAN_POINT('Ctrl Pts',(2.54358134866663,-6.27352239616421,
21.9254288487718));
#188940=CARTESIAN_POINT('Ctrl Pts',(2.71397759435744,-6.19892043966737,
21.9341785673881));
#188941=CARTESIAN_POINT('Ctrl Pts',(2.88437226558304,-6.1243191724943,21.9429282051568));
#188942=CARTESIAN_POINT('Ctrl Pts',(3.05168912681129,-6.04268832278711,
21.9516778429255));
#188943=CARTESIAN_POINT('Ctrl Pts',(3.21535986274021,-5.95430516123244,
21.9604274806942));
#188944=CARTESIAN_POINT('Ctrl Pts',(3.3790291407302,-5.86592278697338,21.9691770405233));
#188945=CARTESIAN_POINT('Ctrl Pts',(3.53905210621761,-5.77078835741826,
21.9779266003523));
#188946=CARTESIAN_POINT('Ctrl Pts',(3.69488522831897,-5.66922500431499,
21.9866761601814));
#188947=CARTESIAN_POINT('Ctrl Pts',(3.85071701407147,-5.56766252216951,
21.9954256449785));
#188948=CARTESIAN_POINT('Ctrl Pts',(4.00235878822617,-5.45967138329214,
22.0041751297757));
#188949=CARTESIAN_POINT('Ctrl Pts',(4.14929549611544,-5.34561838199437,
22.0129246145728));
#188950=CARTESIAN_POINT('Ctrl Pts',(4.29623099276303,-5.23156632086841,
22.0216740272454));
#188951=CARTESIAN_POINT('Ctrl Pts',(4.43846127436234,-5.11145267304785,
22.030423439918));
#188952=CARTESIAN_POINT('Ctrl Pts',(4.57550326054642,-4.98568540049701,
22.0391728525905));
#188953=CARTESIAN_POINT('Ctrl Pts',(4.71254416257969,-4.85991912290178,
22.0479221960458));
#188954=CARTESIAN_POINT('Ctrl Pts',(4.84439664018937,-4.72849950385238,
22.056671539501));
#188955=CARTESIAN_POINT('Ctrl Pts',(4.9706128679491,-4.5918728986089,22.0654208829563));
#188956=CARTESIAN_POINT('Ctrl Pts',(5.09682813912844,-4.45524732884502,
22.0741701601011));
#188957=CARTESIAN_POINT('Ctrl Pts',(5.21740705147993,-4.31341506235601,
22.0829194372459));
#188958=CARTESIAN_POINT('Ctrl Pts',(5.33194007545845,-4.16685781275533,
22.0916687143908));
#188959=CARTESIAN_POINT('Ctrl Pts',(5.44647226944631,-4.02030162521645,
22.1004179281319));
#188960=CARTESIAN_POINT('Ctrl Pts',(5.55495848628254,-3.86902074887732,
22.109167141873));
#188961=CARTESIAN_POINT('Ctrl Pts',(5.65703027291924,-3.71352898080455,
22.1179163556141));
#188962=CARTESIAN_POINT('Ctrl Pts',(5.75910135377131,-3.55803828789372,
22.126665508858));
#188963=CARTESIAN_POINT('Ctrl Pts',(5.85475793592884,-3.39833700106486,
22.1354146621019));
#188964=CARTESIAN_POINT('Ctrl Pts',(5.94367514427526,-3.23496750823319,
22.1441638153458));
#188965=CARTESIAN_POINT('Ctrl Pts',(6.0325917673276,-3.0715990907749,22.1529129109987));
#188966=CARTESIAN_POINT('Ctrl Pts',(6.11476896836036,-2.90456276731199,
22.1616620066516));
#188967=CARTESIAN_POINT('Ctrl Pts',(6.1899276554799,-2.73442583002816,22.1704111023046));
#188968=CARTESIAN_POINT('Ctrl Pts',(6.26508587283143,-2.56428995615952,
22.1791601432726));
#188969=CARTESIAN_POINT('Ctrl Pts',(6.33322554827235,-2.39105376935,22.1879091842406));
#188970=CARTESIAN_POINT('Ctrl Pts',(6.39411526733094,-2.21530561053896,
22.1966582252086));
#188971=CARTESIAN_POINT('Ctrl Pts',(6.45500462602905,-2.03955849184917,
22.2054072143977));
#188972=CARTESIAN_POINT('Ctrl Pts',(6.50864402040791,-1.86129970164366,
22.2141562035867));
#188973=CARTESIAN_POINT('Ctrl Pts',(6.55485128368646,-1.68113463135883,
22.2229051927757));
#188974=CARTESIAN_POINT('Ctrl Pts',(6.60199809554362,-1.49730620116709,
22.2318320782471));
#188975=CARTESIAN_POINT('Ctrl Pts',(6.64140720707901,-1.31149343245555,
22.2407589637186));
#188976=CARTESIAN_POINT('Ctrl Pts',(6.67293928722905,-1.12435326697399,
22.24968584919));
#188977=CARTESIAN_POINT('Ctrl Pts',(6.70384625876274,-0.940923067005333,
22.2584357633675));
#188978=CARTESIAN_POINT('Ctrl Pts',(6.7271855457981,-0.756217899520418,
22.2671856775449));
#188979=CARTESIAN_POINT('Ctrl Pts',(6.74287786815338,-0.570865181253259,
22.2759355917224));
#188980=CARTESIAN_POINT('Ctrl Pts',(6.75856988190853,-0.385516108072748,
22.2846853338269));
#188981=CARTESIAN_POINT('Ctrl Pts',(6.76661520773406,-0.199519795225191,
22.2934350759313));
#188982=CARTESIAN_POINT('Ctrl Pts',(6.76698651789579,-0.013508020454534,
22.3021848180358));
#188983=CARTESIAN_POINT('Ctrl Pts',(6.767357821249,0.172500343514016,22.3109343997008));
#188984=CARTESIAN_POINT('Ctrl Pts',(6.76005538995178,0.358523882211916,
22.3196839813658));
#188985=CARTESIAN_POINT('Ctrl Pts',(6.74510402742353,0.543930748565311,
22.3284335630307));
#188986=CARTESIAN_POINT('Ctrl Pts',(6.73015291918021,0.729334461616112,
22.3371829958874));
#188987=CARTESIAN_POINT('Ctrl Pts',(6.70755316306583,0.914121237635499,
22.3459324287441));
#188988=CARTESIAN_POINT('Ctrl Pts',(6.67738151874562,1.09766345166198,22.3546818616008));
#188989=CARTESIAN_POINT('Ctrl Pts',(6.64721034747555,1.28120278799735,22.3634311572783));
#188990=CARTESIAN_POINT('Ctrl Pts',(6.60946757205127,1.46349731860394,22.3721804529558));
#188991=CARTESIAN_POINT('Ctrl Pts',(6.56428138111508,1.64392790278222,22.3809297486333));
#188992=CARTESIAN_POINT('Ctrl Pts',(6.51909583859833,1.82435589779116,22.3896789187589));
#188993=CARTESIAN_POINT('Ctrl Pts',(6.46646716392857,2.00291972192325,22.3984280888845));
#188994=CARTESIAN_POINT('Ctrl Pts',(6.40657409872863,2.17901292274723,22.4071772590101));
#188995=CARTESIAN_POINT('Ctrl Pts',(6.34668181342056,2.35510383059032,22.4159263152092));
#188996=CARTESIAN_POINT('Ctrl Pts',(6.2795254191403,2.5287239082263,22.4246753714084));
#188997=CARTESIAN_POINT('Ctrl Pts',(6.20533299175497,2.69928350890331,22.4334244276075));
#188998=CARTESIAN_POINT('Ctrl Pts',(6.12831602991527,2.8763363796567,22.4425065637657));
#188999=CARTESIAN_POINT('Ctrl Pts',(6.04371690605246,3.0500908660151,22.4515886999238));
#189000=CARTESIAN_POINT('Ctrl Pts',(5.95184520316605,3.21991112882783,22.460670836082));
#189001=CARTESIAN_POINT('Ctrl Pts',(5.86333549509244,3.3835169118307,22.4694206164256));
#189002=CARTESIAN_POINT('Ctrl Pts',(5.76807618099333,3.54347103712061,22.4781703967692));
#189003=CARTESIAN_POINT('Ctrl Pts',(5.66639083308976,3.69923018027756,22.4869201771128));
#189004=CARTESIAN_POINT('Ctrl Pts',(5.56470914082156,3.85498372382113,22.4956696428977));
#189005=CARTESIAN_POINT('Ctrl Pts',(5.45660203372019,4.00654234702063,22.5044191086826));
#189006=CARTESIAN_POINT('Ctrl Pts',(5.34243669839164,4.15339127986736,22.5131685744675));
#189007=CARTESIAN_POINT('Ctrl Pts',(5.2282748605054,4.30023571401342,22.5219177722135));
#189008=CARTESIAN_POINT('Ctrl Pts',(5.1080553416706,4.44237052028527,22.5306669699595));
#189009=CARTESIAN_POINT('Ctrl Pts',(4.98218644339902,4.57931296628774,22.5394161677055));
#189010=CARTESIAN_POINT('Ctrl Pts',(4.85632073219533,4.71625194483416,22.5481651439172));
#189011=CARTESIAN_POINT('Ctrl Pts',(4.7248061217026,4.84799861524566,22.5569141201288));
#189012=CARTESIAN_POINT('Ctrl Pts',(4.58808925235248,4.97410554898544,22.5656630963404));
#189013=CARTESIAN_POINT('Ctrl Pts',(4.45136349473985,5.10022068121262,22.5744126413421));
#189014=CARTESIAN_POINT('Ctrl Pts',(4.30943501210018,5.22069514871886,22.5831621863438));
#189015=CARTESIAN_POINT('Ctrl Pts',(4.1627858743172,5.33511975166305,22.5919117313455));
#189016=CARTESIAN_POINT('Ctrl Pts',(4.01614535740374,5.44953762807897,22.6006607619993));
#189017=CARTESIAN_POINT('Ctrl Pts',(3.86478496657836,5.55790617532845,22.609409792653));
#189018=CARTESIAN_POINT('Ctrl Pts',(3.70921874747095,5.65985735539422,22.6181588233068));
#189019=CARTESIAN_POINT('Ctrl Pts',(3.55365041605811,5.76180991977101,22.6269079727564));
#189020=CARTESIAN_POINT('Ctrl Pts',(3.39387638174445,5.85734478552857,22.635657122206));
#189021=CARTESIAN_POINT('Ctrl Pts',(3.23043927904474,5.94613749121267,22.6444062716556));
#189022=CARTESIAN_POINT('Ctrl Pts',(3.18691767070385,5.96978206944171,22.6467360795717));
#189023=CARTESIAN_POINT('Ctrl Pts',(3.14313645919605,5.99294880633439,22.6490658874879));
#189024=CARTESIAN_POINT('Ctrl Pts',(3.09910619832133,6.01563211736941,22.651395695404));
#189025=CARTESIAN_POINT('Origin',(0.,0.,4.30282021618968));
#189026=CARTESIAN_POINT('',(3.09910619832135,6.0156321173694,25.0456877277983));
#189027=CARTESIAN_POINT('',(3.09910619832136,6.01563211736939,24.6515493092843));
#189028=CARTESIAN_POINT('',(3.09910619832133,6.0156321173694,4.30282021618968));
#189029=CARTESIAN_POINT('',(-6.76699999294629,0.000308974082675706,23.6971797837786));
#189030=CARTESIAN_POINT('Ctrl Pts',(-6.76699999294632,0.000308973411543368,
23.69717978381));
#189031=CARTESIAN_POINT('Ctrl Pts',(-6.76700839696929,-0.183752247735036,
23.7057925480764));
#189032=CARTESIAN_POINT('Ctrl Pts',(-6.75950283386235,-0.367668115774533,
23.7144053123428));
#189033=CARTESIAN_POINT('Ctrl Pts',(-6.7445446979283,-0.550822855051619,
23.7230180766092));
#189034=CARTESIAN_POINT('Ctrl Pts',(-6.72956763452131,-0.734209351573671,
23.7316417391495));
#189035=CARTESIAN_POINT('Ctrl Pts',(-6.70711919469231,-0.916832496864108,
23.7402654016899));
#189036=CARTESIAN_POINT('Ctrl Pts',(-6.67731230024053,-1.0980844434999,
23.7488890642302));
#189037=CARTESIAN_POINT('Ctrl Pts',(-6.64746597549211,-1.27957616077112,
23.7575241346538));
#189038=CARTESIAN_POINT('Ctrl Pts',(-6.61024180931559,-1.45969276150695,
23.7661592050773));
#189039=CARTESIAN_POINT('Ctrl Pts',(-6.56580334377247,-1.63783865228118,
23.7747942755009));
#189040=CARTESIAN_POINT('Ctrl Pts',(-6.52126396669316,-1.81638907942465,
23.7834489545723));
#189041=CARTESIAN_POINT('Ctrl Pts',(-6.46947760092728,-1.99295955446352,
23.7921036336437));
#189042=CARTESIAN_POINT('Ctrl Pts',(-6.41065772653007,-2.16696943062896,
23.8007583127152));
#189043=CARTESIAN_POINT('Ctrl Pts',(-6.35176769229646,-2.34118686426656,
23.8094233150128));
#189044=CARTESIAN_POINT('Ctrl Pts',(-6.28582750625708,-2.51283732057656,
23.8180883173104));
#189045=CARTESIAN_POINT('Ctrl Pts',(-6.21309833977904,-2.68136122524268,
23.826753319608));
#189046=CARTESIAN_POINT('Ctrl Pts',(-6.14021525281721,-2.85024178573469,
23.8354366600966));
#189047=CARTESIAN_POINT('Ctrl Pts',(-6.06051458184177,-3.01598229024215,
23.8441200005852));
#189048=CARTESIAN_POINT('Ctrl Pts',(-5.9743039486526,-3.17804677893734,
23.8528033410738));
#189049=CARTESIAN_POINT('Ctrl Pts',(-5.91486003936267,-3.28979339775612,
23.8587906733232));
#189050=CARTESIAN_POINT('Ctrl Pts',(-5.8523219878451,-3.39979286924712,
23.8647780055727));
#189051=CARTESIAN_POINT('Ctrl Pts',(-5.78680234959432,-3.50787792927999,
23.8707653378221));
#189052=CARTESIAN_POINT('Ctrl Pts',(-5.69849954641467,-3.65354744207876,
23.8788346470446));
#189053=CARTESIAN_POINT('Ctrl Pts',(-5.60453087510633,-3.79614752730647,
23.8869039562671));
#189054=CARTESIAN_POINT('Ctrl Pts',(-5.50513669195987,-3.93519491294106,
23.8949732654896));
#189055=CARTESIAN_POINT('Ctrl Pts',(-5.40586648037442,-4.07406886869366,
23.9030325100904));
#189056=CARTESIAN_POINT('Ctrl Pts',(-5.30118443589483,-4.20939864200793,
23.9110917546911));
#189057=CARTESIAN_POINT('Ctrl Pts',(-5.19137689545073,-4.34072516169595,
23.9191509992919));
#189058=CARTESIAN_POINT('Ctrl Pts',(-5.08168221776986,-4.47191670090961,
23.9272019604122));
#189059=CARTESIAN_POINT('Ctrl Pts',(-4.96687276507901,-4.59911289086791,
23.9352529215324));
#189060=CARTESIAN_POINT('Ctrl Pts',(-4.84727823237034,-4.72188338885965,
23.9433038826527));
#189061=CARTESIAN_POINT('Ctrl Pts',(-4.72778041619019,-4.84455460190833,
23.9513483329318));
#189062=CARTESIAN_POINT('Ctrl Pts',(-4.60350548104269,-4.9628069806052,
23.9593927832109));
#189063=CARTESIAN_POINT('Ctrl Pts',(-4.47482340490097,-5.07624314773736,
23.96743723349));
#189064=CARTESIAN_POINT('Ctrl Pts',(-4.34621722711222,-5.18961240875088,
23.9754769390482));
#189065=CARTESIAN_POINT('Ctrl Pts',(-4.21320936213674,-5.29817086699351,
23.9835166446065));
#189066=CARTESIAN_POINT('Ctrl Pts',(-4.07620657592594,-5.40155801138691,
23.9915563501647));
#189067=CARTESIAN_POINT('Ctrl Pts',(-3.93624665782077,-5.50717671201804,
23.9997695884692));
#189068=CARTESIAN_POINT('Ctrl Pts',(-3.79211767990105,-5.6073980352704,
24.0079828267737));
#189069=CARTESIAN_POINT('Ctrl Pts',(-3.64428929020167,-5.7018807922756,
24.0161960650781));
#189070=CARTESIAN_POINT('Ctrl Pts',(-3.499630861829,-5.79433750620236,24.0242331826263));
#189071=CARTESIAN_POINT('Ctrl Pts',(-3.35143040432046,-5.88129907050107,
24.0322703001745));
#189072=CARTESIAN_POINT('Ctrl Pts',(-3.20015715330492,-5.96248968084234,
24.0403074177227));
#189073=CARTESIAN_POINT('Ctrl Pts',(-3.04886789854126,-6.04368888063394,
24.0483453855468));
#189074=CARTESIAN_POINT('Ctrl Pts',(-2.89450553215143,-6.11911573401304,
24.0563833533709));
#189075=CARTESIAN_POINT('Ctrl Pts',(-2.73756343398679,-6.18854065550987,
24.064421321195));
#189076=CARTESIAN_POINT('Ctrl Pts',(-2.5805736363313,-6.25798667735801,
24.0724617320027));
#189077=CARTESIAN_POINT('Ctrl Pts',(-2.42100288772765,-6.32142698527623,
24.0805021428104));
#189078=CARTESIAN_POINT('Ctrl Pts',(-2.25936391204472,-6.37868040529936,
24.0885425536182));
#189079=CARTESIAN_POINT('Ctrl Pts',(-2.09161589473576,-6.43809768168619,
24.096886846606));
#189080=CARTESIAN_POINT('Ctrl Pts',(-1.92164068113192,-6.49085112549008,
24.1052311395937));
#189081=CARTESIAN_POINT('Ctrl Pts',(-1.75002671196019,-6.53679550754235,
24.1135754325815));
#189082=CARTESIAN_POINT('Ctrl Pts',(-1.58437054058157,-6.5811448717804,
24.1216300427971));
#189083=CARTESIAN_POINT('Ctrl Pts',(-1.41718786297993,-6.61915000585643,
24.1296846530126));
#189084=CARTESIAN_POINT('Ctrl Pts',(-1.24901604404221,-6.65073288606039,
24.1377392632281));
#189085=CARTESIAN_POINT('Ctrl Pts',(-1.08071691666178,-6.68233967495084,
24.1457999708974));
#189086=CARTESIAN_POINT('Ctrl Pts',(-0.91142752395205,-6.70751447511549,
24.1538606785666));
#189087=CARTESIAN_POINT('Ctrl Pts',(-0.741688760649546,-6.72623124656937,
24.1619213862359));
#189088=CARTESIAN_POINT('Ctrl Pts',(-0.571710675859674,-6.7449744075497,
24.1699934590201));
#189089=CARTESIAN_POINT('Ctrl Pts',(-0.401282325415514,-6.75724134637748,
24.1780655318042));
#189090=CARTESIAN_POINT('Ctrl Pts',(-0.230943592428832,-6.76305804034803,
24.1861376045884));
#189091=CARTESIAN_POINT('Ctrl Pts',(-0.213101904342152,-6.76366729484757,
24.1869830928828));
#189092=CARTESIAN_POINT('Ctrl Pts',(-0.195261193462865,-6.76420583064769,
24.1878285811772));
#189093=CARTESIAN_POINT('Ctrl Pts',(-0.177422075508533,-6.76467371032205,
24.1886740694716));
#189094=CARTESIAN_POINT('Ctrl Pts',(-0.00160417208491934,-6.76928501585913,
24.1970069915184));
#189095=CARTESIAN_POINT('Ctrl Pts',(0.174619392753329,-6.7670435200554,
24.2053399135651));
#189096=CARTESIAN_POINT('Ctrl Pts',(0.350680364474882,-6.75790738927161,
24.2136728356118));
#189097=CARTESIAN_POINT('Ctrl Pts',(0.526533274823219,-6.74878205517886,
24.2219959101654));
#189098=CARTESIAN_POINT('Ctrl Pts',(0.702223630309831,-6.73277833501112,
24.230318984719));
#189099=CARTESIAN_POINT('Ctrl Pts',(0.877180786330981,-6.70990632334698,
24.2386420592726));
#189100=CARTESIAN_POINT('Ctrl Pts',(1.05196329981107,-6.68705714256514,
24.2469568257185));
#189101=CARTESIAN_POINT('Ctrl Pts',(1.22601372910066,-6.65735337434626,
24.2552715921645));
#189102=CARTESIAN_POINT('Ctrl Pts',(1.39876393947533,-6.62085707757111,
24.2635863586104));
#189103=CARTESIAN_POINT('Ctrl Pts',(1.57137339849106,-6.58439051681398,
24.27189435045));
#189104=CARTESIAN_POINT('Ctrl Pts',(1.7426844105235,-6.54114252673414,24.2802023422896));
#189105=CARTESIAN_POINT('Ctrl Pts',(1.91213623161894,-6.49122669699111,
24.2885103341291));
#189106=CARTESIAN_POINT('Ctrl Pts',(2.08148105499195,-6.44134238582405,
24.2968130800162));
#189107=CARTESIAN_POINT('Ctrl Pts',(2.24896869415922,-6.38479872366975,
24.3051158259033));
#189108=CARTESIAN_POINT('Ctrl Pts',(2.41405061273598,-6.32175993210348,
24.3134185717903));
#189109=CARTESIAN_POINT('Ctrl Pts',(2.57906506759386,-6.25874690248225,
24.3217179246098));
#189110=CARTESIAN_POINT('Ctrl Pts',(2.74167543632087,-6.18924415636571,
24.3300172774292));
#189111=CARTESIAN_POINT('Ctrl Pts',(2.90135003577383,-6.11346521785437,
24.3383166302486));
#189112=CARTESIAN_POINT('Ctrl Pts',(3.06099067511859,-6.03770239625179,
24.346614217935));
#189113=CARTESIAN_POINT('Ctrl Pts',(3.21769647498928,-5.95566619063638,
24.3549118056213));
#189114=CARTESIAN_POINT('Ctrl Pts',(3.37095714884444,-5.86761765119836,
24.3632093933076));
#189115=CARTESIAN_POINT('Ctrl Pts',(3.52421069485756,-5.77957320671872,
24.3715065950901));
#189116=CARTESIAN_POINT('Ctrl Pts',(3.67401913257895,-5.68551715906454,
24.3798037968725));
#189117=CARTESIAN_POINT('Ctrl Pts',(3.81989797014447,-5.58575585732908,
24.3881009986549));
#189118=CARTESIAN_POINT('Ctrl Pts',(3.96579426355371,-5.48598261816857,
24.3963991932795));
#189119=CARTESIAN_POINT('Ctrl Pts',(4.1077597330308,-5.38050296145721,24.404697387904));
#189120=CARTESIAN_POINT('Ctrl Pts',(4.24533984304617,-5.26966589235453,
24.4129955825286));
#189121=CARTESIAN_POINT('Ctrl Pts',(4.38301671475655,-5.15875087024924,
24.4212996133702));
#189122=CARTESIAN_POINT('Ctrl Pts',(4.51630179276322,-5.04247112521428,
24.4296036442117));
#189123=CARTESIAN_POINT('Ctrl Pts',(4.6447738641648,-4.92121577974098,24.4379076750533));
#189124=CARTESIAN_POINT('Ctrl Pts',(4.77329265154732,-4.7999163424869,24.446214725469));
#189125=CARTESIAN_POINT('Ctrl Pts',(4.89699469616931,-4.67363794283716,
24.4545217758847));
#189126=CARTESIAN_POINT('Ctrl Pts',(5.01549636385109,-4.54280587568922,
24.4628288263005));
#189127=CARTESIAN_POINT('Ctrl Pts',(5.13412472981551,-4.41183392698056,
24.4711447583551));
#189128=CARTESIAN_POINT('Ctrl Pts',(5.24754138153794,-4.27629884613848,
24.4794606904097));
#189129=CARTESIAN_POINT('Ctrl Pts',(5.35540292711717,-4.13665909741483,
24.4877766224643));
#189130=CARTESIAN_POINT('Ctrl Pts',(5.43671125122884,-4.03139568878183,
24.4940453486833));
#189131=CARTESIAN_POINT('Ctrl Pts',(5.51486374138773,-3.92380050024206,
24.5003140749022));
#189132=CARTESIAN_POINT('Ctrl Pts',(5.58972988068549,-3.8140803427526,24.5065828011212));
#189133=CARTESIAN_POINT('Ctrl Pts',(5.69064974434689,-3.66617711923118,
24.5150330698445));
#189134=CARTESIAN_POINT('Ctrl Pts',(5.78578146237337,-3.51414042581447,
24.5234833385679));
#189135=CARTESIAN_POINT('Ctrl Pts',(5.87478513907061,-3.35845032265703,
24.5319336072912));
#189136=CARTESIAN_POINT('Ctrl Pts',(5.9637102670035,-3.2028976212978,24.5403764183657));
#189137=CARTESIAN_POINT('Ctrl Pts',(6.04651796933681,-3.04369822324832,
24.5488192294402));
#189138=CARTESIAN_POINT('Ctrl Pts',(6.12291176800583,-2.88136087313196,
24.5572620405147));
#189139=CARTESIAN_POINT('Ctrl Pts',(6.19924854776807,-2.71914468858655,
24.5656985500325));
#189140=CARTESIAN_POINT('Ctrl Pts',(6.26918082619156,-2.55379551987639,
24.5741350595503));
#189141=CARTESIAN_POINT('Ctrl Pts',(6.33245799631534,-2.38584675218295,
24.582571569068));
#189142=CARTESIAN_POINT('Ctrl Pts',(6.39568988821887,-2.21801816087034,
24.5910020418092));
#189143=CARTESIAN_POINT('Ctrl Pts',(6.45227605395097,-2.04759399048648,
24.5994325145504));
#189144=CARTESIAN_POINT('Ctrl Pts',(6.50201388768062,-1.87512783681763,
24.6078629872917));
#189145=CARTESIAN_POINT('Ctrl Pts',(6.55173033925025,-1.70273582588116,
24.6162898357955));
#189146=CARTESIAN_POINT('Ctrl Pts',(6.59460423622901,-1.52830389968372,
24.6247166842993));
#189147=CARTESIAN_POINT('Ctrl Pts',(6.63048253802696,-1.35240168327296,
24.6331435328031));
#189148=CARTESIAN_POINT('Ctrl Pts',(6.66634976547441,-1.17655376159469,
24.6415677802398));
#189149=CARTESIAN_POINT('Ctrl Pts',(6.69522563768748,-0.999236779253724,
24.6499920276764));
#189150=CARTESIAN_POINT('Ctrl Pts',(6.71700794767396,-0.821031808692466,
24.658416275113));
#189151=CARTESIAN_POINT('Ctrl Pts',(6.72314536922414,-0.770820466215451,
24.660789905724));
#189152=CARTESIAN_POINT('Ctrl Pts',(6.72871994764906,-0.720538683170418,
24.6631635363349));
#189153=CARTESIAN_POINT('Ctrl Pts',(6.73373013494738,-0.670199574531021,
24.6655371669459));
#189154=CARTESIAN_POINT('Ctrl Pts',(6.75192239560458,-0.487415552479185,
24.6741559478831));
#189155=CARTESIAN_POINT('Ctrl Pts',(6.76266131817743,-0.303957112434016,
24.6827747288204));
#189156=CARTESIAN_POINT('Ctrl Pts',(6.76592810289956,-0.120440468256793,
24.6913935097576));
#189157=CARTESIAN_POINT('Ctrl Pts',(6.76919684995943,0.0631864132535379,
24.7000174679442));
#189158=CARTESIAN_POINT('Ctrl Pts',(6.764984496136,0.246871264546113,24.7086414261308));
#189159=CARTESIAN_POINT('Ctrl Pts',(6.75332436868675,0.429998803837523,
24.7172653843173));
#189160=CARTESIAN_POINT('Ctrl Pts',(6.74124300061684,0.619742116296643,
24.7262008966885));
#189161=CARTESIAN_POINT('Ctrl Pts',(6.72116572968514,0.808886738339662,
24.7351364090596));
#189162=CARTESIAN_POINT('Ctrl Pts',(6.69318809927988,0.996755771319217,
24.7440719214307));
#189163=CARTESIAN_POINT('Ctrl Pts',(6.66613547958873,1.17841338232209,24.7527120033254));
#189164=CARTESIAN_POINT('Ctrl Pts',(6.63169665312615,1.35887811205017,24.7613520852201));
#189165=CARTESIAN_POINT('Ctrl Pts',(6.59000992100219,1.53754942720316,24.7699921671148));
#189166=CARTESIAN_POINT('Ctrl Pts',(6.54618509610065,1.72538470961921,24.7790753947241));
#189167=CARTESIAN_POINT('Ctrl Pts',(6.49434945907513,1.91123739957196,24.7881586223334));
#189168=CARTESIAN_POINT('Ctrl Pts',(6.43472287136891,2.09442845871658,24.7972418499427));
#189169=CARTESIAN_POINT('Ctrl Pts',(6.37509628366268,2.27761951786121,24.8063250775521));
#189170=CARTESIAN_POINT('Ctrl Pts',(6.30767891246507,2.45814859470026,24.8154083051614));
#189171=CARTESIAN_POINT('Ctrl Pts',(6.23274904006528,2.6353611523974,24.8244915327707));
#189172=CARTESIAN_POINT('Ctrl Pts',(6.15813785911683,2.81181999031096,24.8335361276305));
#189173=CARTESIAN_POINT('Ctrl Pts',(6.07600985101772,2.98515375718911,24.8425807224903));
#189174=CARTESIAN_POINT('Ctrl Pts',(5.98663911895625,3.1547489693132,24.8516253173502));
#189175=CARTESIAN_POINT('Ctrl Pts',(5.89735039860957,3.32418855113367,24.8606616123705));
#189176=CARTESIAN_POINT('Ctrl Pts',(5.8008323345595,3.48989621735583,24.8696979073908));
#189177=CARTESIAN_POINT('Ctrl Pts',(5.69740559785817,3.65128175487656,24.8787342024111));
#189178=CARTESIAN_POINT('Ctrl Pts',(5.59416188287733,3.81238170803407,24.8877545069988));
#189179=CARTESIAN_POINT('Ctrl Pts',(5.48403403607998,3.96917460523001,24.8967748115865));
#189180=CARTESIAN_POINT('Ctrl Pts',(5.36738665833089,4.12109808909854,24.9057951161742));
#189181=CARTESIAN_POINT('Ctrl Pts',(5.2508861752956,4.27283025484989,24.9148040614404));
#189182=CARTESIAN_POINT('Ctrl Pts',(5.1278826902548,4.41970505667135,24.9238130067067));
#189183=CARTESIAN_POINT('Ctrl Pts',(4.99878326161908,4.56119007533746,24.9328219519729));
#189184=CARTESIAN_POINT('Ctrl Pts',(4.86997699045438,4.70235381147973,24.9418104398317));
#189185=CARTESIAN_POINT('Ctrl Pts',(4.73510256676615,4.83815201927206,24.9507989276906));
#189186=CARTESIAN_POINT('Ctrl Pts',(4.59460601424922,4.96808661094238,24.9597874155494));
#189187=CARTESIAN_POINT('Ctrl Pts',(4.4713396258809,5.08208633230481,24.9676735765647));
#189188=CARTESIAN_POINT('Ctrl Pts',(4.34374619449053,5.19157281657845,24.9755597375801));
#189189=CARTESIAN_POINT('Ctrl Pts',(4.21215220819276,5.29623099713531,24.9834458985954));
#189190=CARTESIAN_POINT('Ctrl Pts',(4.0766388920244,5.40400626491476,24.9915669371101));
#189191=CARTESIAN_POINT('Ctrl Pts',(3.93694281200398,5.50661181659955,24.9996879756248));
#189192=CARTESIAN_POINT('Ctrl Pts',(3.79350453484897,5.60371415617181,25.0078090141395));
#189193=CARTESIAN_POINT('Ctrl Pts',(3.65006223752656,5.70081921724678,25.0159302802638));
#189194=CARTESIAN_POINT('Ctrl Pts',(3.50287783391915,5.79242054855094,25.0240515463882));
#189195=CARTESIAN_POINT('Ctrl Pts',(3.352421546756,5.87822751965642,25.0321728125125));
#189196=CARTESIAN_POINT('Ctrl Pts',(3.26896149081178,5.92582576060665,25.0366777842744));
#189197=CARTESIAN_POINT('Ctrl Pts',(3.18449515555498,5.97164181984657,25.0411827560364));
#189198=CARTESIAN_POINT('Ctrl Pts',(3.09910619832135,6.0156321173694,25.0456877277983));
#189199=CARTESIAN_POINT('Ctrl Pts',(3.09910619832133,6.01563211736941,23.0457234660332));
#189200=CARTESIAN_POINT('Ctrl Pts',(2.93978497401097,6.09771050649808,23.0541460000253));
#189201=CARTESIAN_POINT('Ctrl Pts',(2.77718683976508,6.17346302929853,23.0625685340173));
#189202=CARTESIAN_POINT('Ctrl Pts',(2.61184465515892,6.24264018643697,23.0709910680093));
#189203=CARTESIAN_POINT('Ctrl Pts',(2.44649484453277,6.31182053420933,23.0794139904709));
#189204=CARTESIAN_POINT('Ctrl Pts',(2.27840103887654,6.37442478275776,23.0878369129326));
#189205=CARTESIAN_POINT('Ctrl Pts',(2.10811606767989,6.43025160045778,23.0962598353942));
#189206=CARTESIAN_POINT('Ctrl Pts',(1.93779946839276,6.48608878722109,23.1046843222978));
#189207=CARTESIAN_POINT('Ctrl Pts',(1.76529120912389,6.53514592952525,23.1131088092014));
#189208=CARTESIAN_POINT('Ctrl Pts',(1.59115961664177,6.57727147640786,23.121533296105));
#189209=CARTESIAN_POINT('Ctrl Pts',(1.41697136254522,6.6194107307485,23.1299605242976));
#189210=CARTESIAN_POINT('Ctrl Pts',(1.24115904616213,6.65461381438227,23.1383877524902));
#189211=CARTESIAN_POINT('Ctrl Pts',(1.06430188866369,6.68278014674932,23.1468149806829));
#189212=CARTESIAN_POINT('Ctrl Pts',(0.887285161789312,6.71097189219064,
23.1552498123424));
#189213=CARTESIAN_POINT('Ctrl Pts',(0.709222039900094,6.73211414831943,
23.163684644002));
#189214=CARTESIAN_POINT('Ctrl Pts',(0.530698714041943,6.74615800844557,
23.1721194756615));
#189215=CARTESIAN_POINT('Ctrl Pts',(0.352087138154694,6.76020881091976,
23.1805584769394));
#189216=CARTESIAN_POINT('Ctrl Pts',(0.173015237454392,6.76715420118122,
23.1889974782174));
#189217=CARTESIAN_POINT('Ctrl Pts',(-0.00592953159499168,6.76699740214632,
23.1974364794953));
#189218=CARTESIAN_POINT('Ctrl Pts',(-0.185070786124451,6.76684043094247,
23.2058847469911));
#189219=CARTESIAN_POINT('Ctrl Pts',(-0.364084296715714,6.75956569786196,
23.2143330144869));
#189220=CARTESIAN_POINT('Ctrl Pts',(-0.542385286372779,6.74522847656967,
23.2227812819826));
#189221=CARTESIAN_POINT('Ctrl Pts',(-0.627977410903571,6.73834599525178,
23.2268368128295));
#189222=CARTESIAN_POINT('Ctrl Pts',(-0.713405440737646,6.72983679143008,
23.2308923436763));
#189223=CARTESIAN_POINT('Ctrl Pts',(-0.798605406967611,6.71971118456457,
23.2349478745231));
#189224=CARTESIAN_POINT('Ctrl Pts',(-0.971704284021721,6.69913921422855,
23.2431874063739));
#189225=CARTESIAN_POINT('Ctrl Pts',(-1.14424758579368,6.6718459625022,23.2514269382247));
#189226=CARTESIAN_POINT('Ctrl Pts',(-1.31567558325423,6.63786763649507,
23.2596664700755));
#189227=CARTESIAN_POINT('Ctrl Pts',(-1.48691330761874,6.60392702405506,
23.2678968566218));
#189228=CARTESIAN_POINT('Ctrl Pts',(-1.65703784651904,6.56331618031817,
23.2761272431681));
#189229=CARTESIAN_POINT('Ctrl Pts',(-1.82549413225624,6.51612309376504,
23.2843576297144));
#189230=CARTESIAN_POINT('Ctrl Pts',(-1.99379349434351,6.46897396942656,
23.2925803493322));
#189231=CARTESIAN_POINT('Ctrl Pts',(-2.16042735747433,6.41525490893963,
23.3008030689501));
#189232=CARTESIAN_POINT('Ctrl Pts',(-2.32485030793808,6.35510503813117,
23.3090257885679));
#189233=CARTESIAN_POINT('Ctrl Pts',(-2.48912756782124,6.29500846444199,
23.3172412222637));
#189234=CARTESIAN_POINT('Ctrl Pts',(-2.65119748659542,6.22849255921135,
23.3254566559595));
#189235=CARTESIAN_POINT('Ctrl Pts',(-2.81052942031948,6.15574637046708,
23.3336720896553));
#189236=CARTESIAN_POINT('Ctrl Pts',(-2.96977946980147,6.0830375676152,23.3418833012561));
#189237=CARTESIAN_POINT('Ctrl Pts',(-3.126294013654,6.00410500553679,23.3500945128569));
#189238=CARTESIAN_POINT('Ctrl Pts',(-3.27956163182627,5.91918613519232,
23.3583057244577));
#189239=CARTESIAN_POINT('Ctrl Pts',(-3.4327778524966,5.83429574195121,23.3665141824712));
#189240=CARTESIAN_POINT('Ctrl Pts',(-3.5827490055672,5.743423211815,23.3747226404847));
#189241=CARTESIAN_POINT('Ctrl Pts',(-3.72898748627362,5.64685233800342,
23.3829310984982));
#189242=CARTESIAN_POINT('Ctrl Pts',(-3.79413992266111,5.60382790501903,
23.3865881457814));
#189243=CARTESIAN_POINT('Ctrl Pts',(-3.85855179997451,5.55967301280929,
23.3902451930646));
#189244=CARTESIAN_POINT('Ctrl Pts',(-3.92218173829601,5.51441560020437,
23.3939022403478));
#189245=CARTESIAN_POINT('Ctrl Pts',(-4.07632312607218,5.40478103870544,
23.4027613145236));
#189246=CARTESIAN_POINT('Ctrl Pts',(-4.2257136889359,5.28878780201047,23.4116203886995));
#189247=CARTESIAN_POINT('Ctrl Pts',(-4.36986620126125,5.16687123732289,
23.4204794628753));
#189248=CARTESIAN_POINT('Ctrl Pts',(-4.51428954715842,5.04472561593595,
23.4293551814694));
#189249=CARTESIAN_POINT('Ctrl Pts',(-4.65345497742721,4.91663459381182,
23.4382309000634));
#189250=CARTESIAN_POINT('Ctrl Pts',(-4.78691160083519,4.78307080501527,
23.4471066186575));
#189251=CARTESIAN_POINT('Ctrl Pts',(-4.92074907173697,4.6491258629052,23.4560076660445));
#189252=CARTESIAN_POINT('Ctrl Pts',(-5.04884495019561,4.50967708541114,
23.4649087134315));
#189253=CARTESIAN_POINT('Ctrl Pts',(-5.17078616801533,4.36523302982342,
23.4738097608185));
#189254=CARTESIAN_POINT('Ctrl Pts',(-5.2928931665935,4.22059260056061,23.4827229093015));
#189255=CARTESIAN_POINT('Ctrl Pts',(-5.40882862802352,4.07094352971808,
23.4916360577845));
#189256=CARTESIAN_POINT('Ctrl Pts',(-5.51822168701323,3.91682504242619,
23.5005492062675));
#189257=CARTESIAN_POINT('Ctrl Pts',(-5.62785762850645,3.76236436995018,
23.5094821443774));
#189258=CARTESIAN_POINT('Ctrl Pts',(-5.73092196238738,3.60341464482035,
23.5184150824873));
#189259=CARTESIAN_POINT('Ctrl Pts',(-5.82708730349631,3.44054393336752,
23.5273480205972));
#189260=CARTESIAN_POINT('Ctrl Pts',(-5.91862276483766,3.28551463133511,
23.5358508824557));
#189261=CARTESIAN_POINT('Ctrl Pts',(-6.00390780897173,3.12693316730652,
23.5443537443141));
#189262=CARTESIAN_POINT('Ctrl Pts',(-6.08270000961948,2.96530767256539,
23.5528566061726));
#189263=CARTESIAN_POINT('Ctrl Pts',(-6.16234304813474,2.80193686432688,
23.561451286216));
#189264=CARTESIAN_POINT('Ctrl Pts',(-6.23549062257036,2.63517054773899,
23.5700459662594));
#189265=CARTESIAN_POINT('Ctrl Pts',(-6.30185609129933,2.4655422942131,23.5786406463028));
#189266=CARTESIAN_POINT('Ctrl Pts',(-6.36812013874254,2.29617327061358,
23.587222191752));
#189267=CARTESIAN_POINT('Ctrl Pts',(-6.42762262986473,2.12395131678241,
23.5958037372013));
#189268=CARTESIAN_POINT('Ctrl Pts',(-6.48012336589972,1.94943329270854,
23.6043852826505));
#189269=CARTESIAN_POINT('Ctrl Pts',(-6.53251894362134,1.77526482603999,
23.6129496393722));
#189270=CARTESIAN_POINT('Ctrl Pts',(-6.57794065302999,1.59880975946691,
23.6215139960939));
#189271=CARTESIAN_POINT('Ctrl Pts',(-6.61619694518648,1.42064315804677,
23.6300783528156));
#189272=CARTESIAN_POINT('Ctrl Pts',(-6.65440773370976,1.24268847543072,
23.6386325227334));
#189273=CARTESIAN_POINT('Ctrl Pts',(-6.68547002714938,1.06302661767811,
23.6471866926511));
#189274=CARTESIAN_POINT('Ctrl Pts',(-6.70924196611391,0.882247833738351,
23.6557408625689));
#189275=CARTESIAN_POINT('Ctrl Pts',(-6.73297736412048,0.701746933312983,
23.6642818834725));
#189276=CARTESIAN_POINT('Ctrl Pts',(-6.74944472068829,0.520132838360479,
23.672822904376));
#189277=CARTESIAN_POINT('Ctrl Pts',(-6.75855317738062,0.338005840952967,
23.6813639252796));
#189278=CARTESIAN_POINT('Ctrl Pts',(-6.76417538046449,0.225587788030584,
23.6866358781126));
#189279=CARTESIAN_POINT('Ctrl Pts',(-6.76699484875476,0.112974553477846,
23.6919078309456));
#189280=CARTESIAN_POINT('Ctrl Pts',(-6.76699999294629,0.000308974082697571,
23.6971797837786));
#189281=CARTESIAN_POINT('',(-6.76699999999747,5.85319020961543E-6,23.3029481390095));
#189282=CARTESIAN_POINT('Ctrl Pts',(3.09910619832133,6.01563211736941,22.651395695404));
#189283=CARTESIAN_POINT('Ctrl Pts',(2.93375330764819,6.10081787314657,22.6601451433063));
#189284=CARTESIAN_POINT('Ctrl Pts',(2.76488627843058,6.17918207037045,22.6688945912086));
#189285=CARTESIAN_POINT('Ctrl Pts',(2.59307866646683,6.25045854554005,22.6776440391109));
#189286=CARTESIAN_POINT('Ctrl Pts',(2.42127244185357,6.32173444515044,22.6863934163612));
#189287=CARTESIAN_POINT('Ctrl Pts',(2.24652594672445,6.38592262741845,22.6951427936115));
#189288=CARTESIAN_POINT('Ctrl Pts',(2.069432696871,6.44280508110568,22.7038921708618));
#189289=CARTESIAN_POINT('Ctrl Pts',(1.89234081822056,6.49968709436173,22.7126414803672));
#189290=CARTESIAN_POINT('Ctrl Pts',(1.71290249405566,6.54926340459551,22.7213907898726));
#189291=CARTESIAN_POINT('Ctrl Pts',(1.53172716625035,6.59136563150389,22.7301400993779));
#189292=CARTESIAN_POINT('Ctrl Pts',(1.35055318107313,6.63346754640714,22.7388893440451));
#189293=CARTESIAN_POINT('Ctrl Pts',(1.167642497144,6.66809542395779,22.7476385887124));
#189294=CARTESIAN_POINT('Ctrl Pts',(0.983616340614175,6.69513165624671,
22.7563878333796));
#189295=CARTESIAN_POINT('Ctrl Pts',(0.799591486713775,6.72216769715961,
22.7651370161153));
#189296=CARTESIAN_POINT('Ctrl Pts',(0.61445145952676,6.7416121586937,22.773886198851));
#189297=CARTESIAN_POINT('Ctrl Pts',(0.428825047910446,6.75339900185711,
22.7826353815867));
#189298=CARTESIAN_POINT('Ctrl Pts',(0.243199888597073,6.76518576550221,
22.7913845052972));
#189299=CARTESIAN_POINT('Ctrl Pts',(0.05708863739181,6.76931499599835,22.8001336290078));
#189300=CARTESIAN_POINT('Ctrl Pts',(-0.128876626811393,6.76577266947846,
22.8088827527183));
#189301=CARTESIAN_POINT('Ctrl Pts',(-0.314840698188196,6.76223036567992,
22.8176318203099));
#189302=CARTESIAN_POINT('Ctrl Pts',(-0.500658497951085,6.75101660879224,
22.8263808879014));
#189303=CARTESIAN_POINT('Ctrl Pts',(-0.685698951925846,6.73216948296222,
22.8351299554929));
#189304=CARTESIAN_POINT('Ctrl Pts',(-0.870738280459626,6.71332247176297,
22.8438789698714));
#189305=CARTESIAN_POINT('Ctrl Pts',(-1.05499998761242,6.68684221356188,
22.85262798425));
#189306=CARTESIAN_POINT('Ctrl Pts',(-1.23785829161425,6.65281863948521,
22.8613769986285));
#189307=CARTESIAN_POINT('Ctrl Pts',(-1.43007412917408,6.6170539536886,22.8705737323277));
#189308=CARTESIAN_POINT('Ctrl Pts',(-1.62073882535796,6.57295372727789,
22.8797704660269));
#189309=CARTESIAN_POINT('Ctrl Pts',(-1.80913696091517,6.52068343478279,
22.8889671997261));
#189310=CARTESIAN_POINT('Ctrl Pts',(-1.98838356186115,6.47095219815198,
22.8977171974398));
#189311=CARTESIAN_POINT('Ctrl Pts',(-2.16557827572535,6.4138258685089,22.9064671951534));
#189312=CARTESIAN_POINT('Ctrl Pts',(-2.34011918621702,6.34949849943277,
22.9152171928671));
#189313=CARTESIAN_POINT('Ctrl Pts',(-2.51465655691096,6.28517243495551,
22.9239670131254));
#189314=CARTESIAN_POINT('Ctrl Pts',(-2.68653996295322,6.21364572242377,
22.9327168333837));
#189315=CARTESIAN_POINT('Ctrl Pts',(-2.85518555379979,6.13516132252225,
22.941466653642));
#189316=CARTESIAN_POINT('Ctrl Pts',(-3.02382794858676,6.05667841000513,
22.9502163080795));
#189317=CARTESIAN_POINT('Ctrl Pts',(-3.18923239109266,5.97123819492089,
22.958965962517));
#189318=CARTESIAN_POINT('Ctrl Pts',(-3.3508370596768,5.87913088810723,22.9677156169545));
#189319=CARTESIAN_POINT('Ctrl Pts',(-3.51243888042388,5.7870252044311,22.9764651172035));
#189320=CARTESIAN_POINT('Ctrl Pts',(-3.67024081223685,5.68825280605787,
22.9852146174524));
#189321=CARTESIAN_POINT('Ctrl Pts',(-3.82370687544402,5.58314917682504,
22.9939641177014));
#189322=CARTESIAN_POINT('Ctrl Pts',(-3.97717043817833,5.47804726008009,
23.0027134753918));
#189323=CARTESIAN_POINT('Ctrl Pts',(-4.12629803722495,5.3666144808421,23.0114628330823));
#189324=CARTESIAN_POINT('Ctrl Pts',(-4.27058317206957,5.24922931204536,
23.0202121907728));
#189325=CARTESIAN_POINT('Ctrl Pts',(-4.4148661477489,5.13184589986744,23.0289614175329));
#189326=CARTESIAN_POINT('Ctrl Pts',(-4.55430658194473,5.00851045722981,
23.037710644293));
#189327=CARTESIAN_POINT('Ctrl Pts',(-4.68843089001908,4.87964187103059,
23.046459871053));
#189328=CARTESIAN_POINT('Ctrl Pts',(-4.8225533691789,4.75077504207906,23.055208978509));
#189329=CARTESIAN_POINT('Ctrl Pts',(-4.95135966065179,4.61637541908045,
23.0639580859649));
#189330=CARTESIAN_POINT('Ctrl Pts',(-5.0744123086928,4.47689945401804,23.0727071934208));
#189331=CARTESIAN_POINT('Ctrl Pts',(-5.1974634422646,4.33742520555465,23.0814561931972));
#189332=CARTESIAN_POINT('Ctrl Pts',(-5.31476088454816,4.19287495491275,
23.0902051929735));
#189333=CARTESIAN_POINT('Ctrl Pts',(-5.42590627628907,4.04373961586634,
23.0989541927499));
#189334=CARTESIAN_POINT('Ctrl Pts',(-5.53706380672721,3.89458798906659,
23.1077041480446));
#189335=CARTESIAN_POINT('Ctrl Pts',(-5.64206777071916,3.74085050155205,
23.1164541033393));
#189336=CARTESIAN_POINT('Ctrl Pts',(-5.74056148164059,3.58304938223079,
23.125204058634));
#189337=CARTESIAN_POINT('Ctrl Pts',(-5.83905138951931,3.42525435593201,
23.1339536760751));
#189338=CARTESIAN_POINT('Ctrl Pts',(-5.93103139557697,3.26339625497102,
23.1427032935162));
#189339=CARTESIAN_POINT('Ctrl Pts',(-6.01618907820888,3.09802485064924,
23.1514529109573));
#189340=CARTESIAN_POINT('Ctrl Pts',(-6.10134392545025,2.93265895249554,
23.1602022370732));
#189341=CARTESIAN_POINT('Ctrl Pts',(-6.17967677261873,2.76378023985943,
23.1689515631891));
#189342=CARTESIAN_POINT('Ctrl Pts',(-6.25092157009265,2.59196229227018,
23.1777008893049));
#189343=CARTESIAN_POINT('Ctrl Pts',(-6.32216437407788,2.42014915229001,
23.1864499706074));
#189344=CARTESIAN_POINT('Ctrl Pts',(-6.3863194154895,2.24539720662769,23.1951990519098));
#189345=CARTESIAN_POINT('Ctrl Pts',(-6.44316881037561,2.06829994947613,
23.2039481332123));
#189346=CARTESIAN_POINT('Ctrl Pts',(-6.50002334524594,1.89118668024373,
23.2126980055546));
#189347=CARTESIAN_POINT('Ctrl Pts',(-6.54957082411117,1.71172794807622,
23.221447877897));
#189348=CARTESIAN_POINT('Ctrl Pts',(-6.59164294296103,1.53053334250255,
23.2301977502393));
#189349=CARTESIAN_POINT('Ctrl Pts',(-6.63371214082149,1.34935131693523,
23.2389470150942));
#189350=CARTESIAN_POINT('Ctrl Pts',(-6.66830695239702,1.16643393829695,
23.2476962799491));
#189351=CARTESIAN_POINT('Ctrl Pts',(-6.69530988153997,0.982402458340393,
23.256445544804));
#189352=CARTESIAN_POINT('Ctrl Pts',(-6.7223141969049,0.798361530946461,
23.2651952588111));
#189353=CARTESIAN_POINT('Ctrl Pts',(-6.74172580829283,0.61320667136188,
23.2739449728181));
#189354=CARTESIAN_POINT('Ctrl Pts',(-6.75347878028183,0.427566795112802,
23.2826946868251));
#189355=CARTESIAN_POINT('Ctrl Pts',(-6.76248992368218,0.285234494204722,
23.2894031966134));
#189356=CARTESIAN_POINT('Ctrl Pts',(-6.76699999999998,0.142617266091624,
23.2961117064016));
#189357=CARTESIAN_POINT('Ctrl Pts',(-6.767,9.78733067650232E-13,23.3028202161899));
#189358=CARTESIAN_POINT('Ctrl Pts',(-6.76699999999747,5.85319020961541E-6,
23.3029481390095));
#189359=CARTESIAN_POINT('Ctrl Pts',(-6.76700016116128,-0.186319119314029,
23.3117377397451));
#189360=CARTESIAN_POINT('Ctrl Pts',(-6.75930048283915,-0.372762212440499,
23.3205273404807));
#189361=CARTESIAN_POINT('Ctrl Pts',(-6.74389773019003,-0.558688110431761,
23.3293169412162));
#189362=CARTESIAN_POINT('Ctrl Pts',(-6.72852054297525,-0.744305409275513,
23.3380919530036));
#189363=CARTESIAN_POINT('Ctrl Pts',(-6.70546582398969,-0.929406947033604,
23.346866964791));
#189364=CARTESIAN_POINT('Ctrl Pts',(-6.67478228873816,-1.11335995883966,
23.3556419765784));
#189365=CARTESIAN_POINT('Ctrl Pts',(-6.64413163720242,-1.29711582717739,
23.3644075841367));
#189366=CARTESIAN_POINT('Ctrl Pts',(-6.60586852253467,-1.47972534840579,
23.373173191695));
#189367=CARTESIAN_POINT('Ctrl Pts',(-6.56009335561501,-1.66056140073645,
23.3819387992533));
#189368=CARTESIAN_POINT('Ctrl Pts',(-6.51438605881939,-1.84112933028069,
23.3906914101824));
#189369=CARTESIAN_POINT('Ctrl Pts',(-6.46118900554621,-2.0199287666356,
23.3994440211115));
#189370=CARTESIAN_POINT('Ctrl Pts',(-6.4006535329081,-2.19634317711761,
23.4081966320406));
#189371=CARTESIAN_POINT('Ctrl Pts',(-6.37673047331703,-2.26606052251466,
23.4116555830276));
#189372=CARTESIAN_POINT('Ctrl Pts',(-6.35166189231806,-2.33540549336483,
23.4151145340147));
#189373=CARTESIAN_POINT('Ctrl Pts',(-6.32545932362219,-2.40434052188975,
23.4185734850018));
#189374=CARTESIAN_POINT('Ctrl Pts',(-6.26393684423442,-2.56619693836351,
23.4266949498579));
#189375=CARTESIAN_POINT('Ctrl Pts',(-6.19617809871287,-2.7257425637015,
23.4348164147141));
#189376=CARTESIAN_POINT('Ctrl Pts',(-6.12239174810059,-2.88246566029672,
23.4429378795703));
#189377=CARTESIAN_POINT('Ctrl Pts',(-6.04861065954114,-3.03917758022842,
23.4510587652465));
#189378=CARTESIAN_POINT('Ctrl Pts',(-5.96880297808581,-3.19306704104957,
23.4591796509227));
#189379=CARTESIAN_POINT('Ctrl Pts',(-5.88322467762074,-3.3436441785325,
23.4673005365989));
#189380=CARTESIAN_POINT('Ctrl Pts',(-5.79763614810189,-3.49423931428872,
23.4754223929531));
#189381=CARTESIAN_POINT('Ctrl Pts',(-5.70627580809272,-3.64152102058143,
23.4835442493073));
#189382=CARTESIAN_POINT('Ctrl Pts',(-5.6094445389146,-3.78502588694465,
23.4916661056616));
#189383=CARTESIAN_POINT('Ctrl Pts',(-5.51254262284014,-3.92863545268345,
23.4997938876217));
#189384=CARTESIAN_POINT('Ctrl Pts',(-5.41016201047141,-4.06846237107829,
23.5079216695819));
#189385=CARTESIAN_POINT('Ctrl Pts',(-5.30264607079231,-4.20407345890993,
23.5160494515421));
#189386=CARTESIAN_POINT('Ctrl Pts',(-5.19508633311552,-4.33973978965838,
23.5241805444585));
#189387=CARTESIAN_POINT('Ctrl Pts',(-5.08238733648211,-4.47118658883518,
23.532311637375));
#189388=CARTESIAN_POINT('Ctrl Pts',(-4.96493116889428,-4.59801560329476,
23.5404427302914));
#189389=CARTESIAN_POINT('Ctrl Pts',(-4.84734680280835,-4.72498304632309,
23.548582697956));
#189390=CARTESIAN_POINT('Ctrl Pts',(-4.72499515374034,-4.84732237923032,
23.5567226656205));
#189391=CARTESIAN_POINT('Ctrl Pts',(-4.59829395183759,-4.96467337621458,
23.5648626332851));
#189392=CARTESIAN_POINT('Ctrl Pts',(-4.53258123032184,-5.02553667718263,
23.5690843724656));
#189393=CARTESIAN_POINT('Ctrl Pts',(-4.46569905689552,-5.08505882860822,
23.573306111646));
#189394=CARTESIAN_POINT('Ctrl Pts',(-4.39770895395443,-5.14319404225712,
23.5775278508265));
#189395=CARTESIAN_POINT('Ctrl Pts',(-4.26178139298135,-5.25941945531155,
23.5859680602842));
#189396=CARTESIAN_POINT('Ctrl Pts',(-4.12114276942399,-5.37033913632986,
23.5944082697418));
#189397=CARTESIAN_POINT('Ctrl Pts',(-3.97623544461375,-5.47556761340752,
23.6028484791994));
#189398=CARTESIAN_POINT('Ctrl Pts',(-3.83143790857038,-5.58071636432397,
23.6112822939479));
#189399=CARTESIAN_POINT('Ctrl Pts',(-3.68237838725329,-5.6801823115947,
23.6197161086964));
#189400=CARTESIAN_POINT('Ctrl Pts',(-3.5295320477759,-5.77362040003695,
23.628149923445));
#189401=CARTESIAN_POINT('Ctrl Pts',(-3.37677801545152,-5.86700205923167,
23.6365786448335));
#189402=CARTESIAN_POINT('Ctrl Pts',(-3.22024200812601,-5.95436294365884,
23.645007366222));
#189403=CARTESIAN_POINT('Ctrl Pts',(-3.06042821103098,-6.03540124309277,
23.6534360876106));
#189404=CARTESIAN_POINT('Ctrl Pts',(-2.90068638820505,-6.1164030458507,
23.6618610130124));
#189405=CARTESIAN_POINT('Ctrl Pts',(-2.73767001591374,-6.1910877905604,
23.6702859384141));
#189406=CARTESIAN_POINT('Ctrl Pts',(-2.5719082655142,-6.25919937961556,
23.6787108638159));
#189407=CARTESIAN_POINT('Ctrl Pts',(-2.40619573535979,-6.32729074404651,
23.6871332875736));
#189408=CARTESIAN_POINT('Ctrl Pts',(-2.23773976090506,-6.38881271851174,
23.6955557113313));
#189409=CARTESIAN_POINT('Ctrl Pts',(-2.06709025772142,-6.44355700420452,
23.7039781350891));
#189410=CARTESIAN_POINT('Ctrl Pts',(-1.89643807071232,-6.49830215086734,
23.7124006913073));
#189411=CARTESIAN_POINT('Ctrl Pts',(-1.72359260147961,-6.54626928760543,
23.7208232475255));
#189412=CARTESIAN_POINT('Ctrl Pts',(-1.54912036595553,-6.58729952953271,
23.7292458037437));
#189413=CARTESIAN_POINT('Ctrl Pts',(-1.37464223672652,-6.62833115746927,
23.7376686444774));
#189414=CARTESIAN_POINT('Ctrl Pts',(-1.19853755631639,-6.66242534683531,
23.7460914852112));
#189415=CARTESIAN_POINT('Ctrl Pts',(-1.02138466599772,-6.68947399756249,
23.7545143259449));
#189416=CARTESIAN_POINT('Ctrl Pts',(-0.844201058918017,-6.71652733828903,
23.7629386271256));
#189417=CARTESIAN_POINT('Ctrl Pts',(-0.665969209309789,-6.73653265445048,
23.7713629283062));
#189418=CARTESIAN_POINT('Ctrl Pts',(-0.487274607743674,-6.74943349153455,
23.7797872294868));
#189419=CARTESIAN_POINT('Ctrl Pts',(-0.308524066708256,-6.76233836716245,
23.7882141678536));
#189420=CARTESIAN_POINT('Ctrl Pts',(-0.129310817465469,-6.76813430560661,
23.7966411062205));
#189421=CARTESIAN_POINT('Ctrl Pts',(0.0497772355627528,-6.76681691985381,
23.8050680445873));
#189422=CARTESIAN_POINT('Ctrl Pts',(0.229026311261498,-6.76549834960562,
23.8135025598309));
#189423=CARTESIAN_POINT('Ctrl Pts',(0.408149631944036,-6.75705367785012,
23.8219370750746));
#189424=CARTESIAN_POINT('Ctrl Pts',(0.586560849915647,-6.74153063994715,
23.8303715903183));
#189425=CARTESIAN_POINT('Ctrl Pts',(0.765058242033914,-6.7260001042839,
23.838810179505));
#189426=CARTESIAN_POINT('Ctrl Pts',(0.942842514119942,-6.70338442082986,
23.8472487686918));
#189427=CARTESIAN_POINT('Ctrl Pts',(1.1193345924047,-6.67378296547365,23.8556873578786));
#189428=CARTESIAN_POINT('Ctrl Pts',(1.29602394890242,-6.64414842238755,
23.8641353794989));
#189429=CARTESIAN_POINT('Ctrl Pts',(1.47141789791735,-6.60751256786978,
23.8725834011192));
#189430=CARTESIAN_POINT('Ctrl Pts',(1.64494846641265,-6.56402571162291,
23.8810314227395));
#189431=CARTESIAN_POINT('Ctrl Pts',(1.74358045666669,-6.53930848042433,
23.8858331426517));
#189432=CARTESIAN_POINT('Ctrl Pts',(1.84161072736434,-6.51237887841011,
23.8906348625639));
#189433=CARTESIAN_POINT('Ctrl Pts',(1.93893746026169,-6.48327159119483,
23.895436582476));
#189434=CARTESIAN_POINT('Ctrl Pts',(2.10594568446213,-6.43332481702085,
23.9036761143269));
#189435=CARTESIAN_POINT('Ctrl Pts',(2.27125413310745,-6.37685155447372,
23.9119156461777));
#189436=CARTESIAN_POINT('Ctrl Pts',(2.43431757415674,-6.31398344534982,
23.9201551780285));
#189437=CARTESIAN_POINT('Ctrl Pts',(2.59720002618313,-6.25118511543314,
23.9283855645748));
#189438=CARTESIAN_POINT('Ctrl Pts',(2.75784210305396,-6.18200619881975,
23.9366159511212));
#189439=CARTESIAN_POINT('Ctrl Pts',(2.91571204343896,-6.10662855262583,
23.9448463376675));
#189440=CARTESIAN_POINT('Ctrl Pts',(3.07343492177095,-6.03132112367132,
23.9530690572853));
#189441=CARTESIAN_POINT('Ctrl Pts',(3.22839048713255,-5.9498266173217,23.9612917769032));
#189442=CARTESIAN_POINT('Ctrl Pts',(3.38006525720238,-5.86237561548673,
23.969514496521));
#189443=CARTESIAN_POINT('Ctrl Pts',(3.53160563249717,-5.77500210154057,
23.9777299302168));
#189444=CARTESIAN_POINT('Ctrl Pts',(3.67987069931387,-5.68168278852421,
23.9859453639126));
#189445=CARTESIAN_POINT('Ctrl Pts',(3.82437008601423,-5.58269490884103,
23.9941607976084));
#189446=CARTESIAN_POINT('Ctrl Pts',(3.96879521125185,-5.48375790124047,
24.0023720092093));
#189447=CARTESIAN_POINT('Ctrl Pts',(4.10945821772749,-5.3791583295227,24.0105832208102));
#189448=CARTESIAN_POINT('Ctrl Pts',(4.24589597215357,-5.2692178161137,24.0187944324111));
#189449=CARTESIAN_POINT('Ctrl Pts',(4.38228797288418,-5.15931417068741,
24.0270028904246));
#189450=CARTESIAN_POINT('Ctrl Pts',(4.51445726735109,-5.04407337458221,
24.0352113484381));
#189451=CARTESIAN_POINT('Ctrl Pts',(4.64197213069801,-4.92385862285088,
24.0434198064517));
#189452=CARTESIAN_POINT('Ctrl Pts',(4.69878278670445,-4.87030032597276,
24.0470768537347));
#189453=CARTESIAN_POINT('Ctrl Pts',(4.75467002245515,-4.81575528655811,
24.0507339010178));
#189454=CARTESIAN_POINT('Ctrl Pts',(4.80959786119915,-4.7602581246765,24.0543909483008));
#189455=CARTESIAN_POINT('Ctrl Pts',(4.94265870512388,-4.62581811457868,
24.0632500224767));
#189456=CARTESIAN_POINT('Ctrl Pts',(5.06994882290606,-4.48592816802374,
24.0721090966526));
#189457=CARTESIAN_POINT('Ctrl Pts',(5.19106284858699,-4.34110072470334,
24.0809681708285));
#189458=CARTESIAN_POINT('Ctrl Pts',(5.31240442315599,-4.19600117975389,
24.0898438894224));
#189459=CARTESIAN_POINT('Ctrl Pts',(5.42754655013052,-4.04594579822502,
24.0987196080164));
#189460=CARTESIAN_POINT('Ctrl Pts',(5.53612605306277,-3.89147752461706,
24.1075953266103));
#189461=CARTESIAN_POINT('Ctrl Pts',(5.64501541121713,-3.73656844220137,
24.1164963739973));
#189462=CARTESIAN_POINT('Ctrl Pts',(5.74730451823662,-3.57722148048661,
24.1253974213843));
#189463=CARTESIAN_POINT('Ctrl Pts',(5.84267361997403,-3.41400849009776,
24.1342984687713));
#189464=CARTESIAN_POINT('Ctrl Pts',(5.93817237731328,-3.25057360940993,
24.1432116172543));
#189465=CARTESIAN_POINT('Ctrl Pts',(6.02673221148577,-3.08326242809785,
24.1521247657373));
#189466=CARTESIAN_POINT('Ctrl Pts',(6.10808020456531,-2.91266977438181,
24.1610379142203));
#189467=CARTESIAN_POINT('Ctrl Pts',(6.18960881243379,-2.74169835832662,
24.1699708523301));
#189468=CARTESIAN_POINT('Ctrl Pts',(6.2638934397176,-2.56743113195713,24.17890379044));
#189469=CARTESIAN_POINT('Ctrl Pts',(6.33070894983138,-2.39048388250683,
24.1878367285499));
#189470=CARTESIAN_POINT('Ctrl Pts',(6.39430762761436,-2.22205575731238,
24.1963395904085));
#189471=CARTESIAN_POINT('Ctrl Pts',(6.45113939758644,-2.05119976704901,
24.204842452267));
#189472=CARTESIAN_POINT('Ctrl Pts',(6.50105254746634,-1.87845808446219,
24.2133453141256));
#189473=CARTESIAN_POINT('Ctrl Pts',(6.5493212428263,-1.71140760432196,24.2215680379914));
#189474=CARTESIAN_POINT('Ctrl Pts',(6.59121125434896,-1.54227318927006,
24.2297907618573));
#189475=CARTESIAN_POINT('Ctrl Pts',(6.62654128339385,-1.37158288829985,
24.2380134857232));
#189476=CARTESIAN_POINT('Ctrl Pts',(6.66183391679992,-1.20107325723056,
24.2462275061144));
#189477=CARTESIAN_POINT('Ctrl Pts',(6.69058032240031,-1.02901136801331,
24.2544415265056));
#189478=CARTESIAN_POINT('Ctrl Pts',(6.71264883432086,-0.855940784803948,
24.2626555468968));
#189479=CARTESIAN_POINT('Ctrl Pts',(6.73469841820239,-0.683018643264092,
24.2708625221688));
#189480=CARTESIAN_POINT('Ctrl Pts',(6.75008147028002,-0.509089884581408,
24.2790694974408));
#189481=CARTESIAN_POINT('Ctrl Pts',(6.7587172651216,-0.334708724336901,
24.2872764727127));
#189482=CARTESIAN_POINT('Ctrl Pts',(6.7673473864183,-0.160442129034876,
24.2954780561657));
#189483=CARTESIAN_POINT('Ctrl Pts',(6.76923906243111,0.0142759188046485,
24.3036796396187));
#189484=CARTESIAN_POINT('Ctrl Pts',(6.76436332995802,0.188885521730087,
24.3118812230717));
#189485=CARTESIAN_POINT('Ctrl Pts',(6.75948982231459,0.363415449114437,
24.3200790640867));
#189486=CARTESIAN_POINT('Ctrl Pts',(6.74785506825636,0.537836672324922,
24.3282769051018));
#189487=CARTESIAN_POINT('Ctrl Pts',(6.72948219473935,0.7115886386713,24.3364747461168));
#189488=CARTESIAN_POINT('Ctrl Pts',(6.7111109425711,0.88532527194889,24.344671863698));
#189489=CARTESIAN_POINT('Ctrl Pts',(6.68600278450453,1.05839240863413,24.3528689812792));
#189490=CARTESIAN_POINT('Ctrl Pts',(6.65423281064427,1.23023359641381,24.3610660988603));
#189491=CARTESIAN_POINT('Ctrl Pts',(6.62246319026041,1.40207287226859,24.3692631252394));
#189492=CARTESIAN_POINT('Ctrl Pts',(6.58403196589232,1.57268587333772,24.3774601516185));
#189493=CARTESIAN_POINT('Ctrl Pts',(6.5390655364396,1.74152545492391,24.3856571779976));
#189494=CARTESIAN_POINT('Ctrl Pts',(6.49409143102741,1.91039385813992,24.3938556036437));
#189495=CARTESIAN_POINT('Ctrl Pts',(6.44257999030012,2.07748789198836,24.4020540292899));
#189496=CARTESIAN_POINT('Ctrl Pts',(6.38470777286537,2.24227466094422,24.410252454936));
#189497=CARTESIAN_POINT('Ctrl Pts',(6.32681515336021,2.40711952325493,24.4184537708266));
#189498=CARTESIAN_POINT('Ctrl Pts',(6.26255740908018,2.56965516202733,24.4266550867172));
#189499=CARTESIAN_POINT('Ctrl Pts',(6.19215962156899,2.72936773282945,24.4348564026078));
#189500=CARTESIAN_POINT('Ctrl Pts',(6.12168166276171,2.88926218951544,24.4430670584244));
#189501=CARTESIAN_POINT('Ctrl Pts',(6.04504983587016,3.04632682653853,24.451277714241));
#189502=CARTESIAN_POINT('Ctrl Pts',(5.96253614336249,3.2000705834553,24.4594883700576));
#189503=CARTESIAN_POINT('Ctrl Pts',(5.87997382753456,3.3539049378439,24.4677038642148));
#189504=CARTESIAN_POINT('Ctrl Pts',(5.79152291857737,3.50441420246484,24.4759193583719));
#189505=CARTESIAN_POINT('Ctrl Pts',(5.69749925772981,3.65113560528342,24.4841348525291));
#189506=CARTESIAN_POINT('Ctrl Pts',(5.60332971744261,3.79808464905782,24.4923630931766));
#189507=CARTESIAN_POINT('Ctrl Pts',(5.5035703517247,3.94123379239337,24.5005913338241));
#189508=CARTESIAN_POINT('Ctrl Pts',(5.39857866451535,4.0801516397114,24.5088195744716));
#189509=CARTESIAN_POINT('Ctrl Pts',(5.30315798287738,4.20640578454037,24.5162977315728));
#189510=CARTESIAN_POINT('Ctrl Pts',(5.20341608243987,4.32916519283054,24.5237758886739));
#189511=CARTESIAN_POINT('Ctrl Pts',(5.09964747685195,4.44813271068182,24.5312540457751));
#189512=CARTESIAN_POINT('Ctrl Pts',(4.98765384404185,4.57652996951629,24.5393249452127));
#189513=CARTESIAN_POINT('Ctrl Pts',(4.8706025363177,4.70093021253803,24.5473958446503));
#189514=CARTESIAN_POINT('Ctrl Pts',(4.74881340549579,4.82089828141846,24.555466744088));
#189515=CARTESIAN_POINT('Ctrl Pts',(4.62721738093441,4.94067613147553,24.5635248464788));
#189516=CARTESIAN_POINT('Ctrl Pts',(4.50089875728203,5.05603554475185,24.5715829488696));
#189517=CARTESIAN_POINT('Ctrl Pts',(4.37021819506817,5.16657351902546,24.5796410512604));
#189518=CARTESIAN_POINT('Ctrl Pts',(4.23965646947264,5.27701097368975,24.5876918258771));
#189519=CARTESIAN_POINT('Ctrl Pts',(4.10474097640636,5.38263547036333,24.5957426004938));
#189520=CARTESIAN_POINT('Ctrl Pts',(3.96587028875585,5.48307959569835,24.6037933751105));
#189521=CARTESIAN_POINT('Ctrl Pts',(3.82711688633064,5.58343888951083,24.6118373503304));
#189522=CARTESIAN_POINT('Ctrl Pts',(3.68441523993815,5.67862630420322,24.6198813255502));
#189523=CARTESIAN_POINT('Ctrl Pts',(3.53819790618462,5.76831384172799,24.6279253007701));
#189524=CARTESIAN_POINT('Ctrl Pts',(3.39505808443007,5.85611367917093,24.6357999702748));
#189525=CARTESIAN_POINT('Ctrl Pts',(3.24854938851748,5.93864264926404,24.6436746397796));
#189526=CARTESIAN_POINT('Ctrl Pts',(3.09910619832136,6.01563211736939,24.6515493092843));
#189527=CARTESIAN_POINT('Origin',(0.,0.,4.30282021618968));
#189528=CARTESIAN_POINT('',(3.09910619832137,6.01563211736939,27.0457199708935));
#189529=CARTESIAN_POINT('',(3.0991061983213,6.01563211736942,26.6512942524228));
#189530=CARTESIAN_POINT('',(3.09910619832133,6.0156321173694,4.30282021618968));
#189531=CARTESIAN_POINT('',(-6.76699810037806,-0.00507045163499823,25.6971797837853));
#189532=CARTESIAN_POINT('Ctrl Pts',(-6.76699810037766,-0.00507045216101548,
25.6971797838101));
#189533=CARTESIAN_POINT('Ctrl Pts',(-6.76683316558664,-0.225191534474847,
25.7075416747608));
#189534=CARTESIAN_POINT('Ctrl Pts',(-6.75592406321113,-0.444938118573672,
25.7179035657114));
#189535=CARTESIAN_POINT('Ctrl Pts',(-6.73440294215104,-0.663404863373404,
25.7282654566621));
#189536=CARTESIAN_POINT('Ctrl Pts',(-6.71261506930177,-0.884579478032097,
25.7387557820444));
#189537=CARTESIAN_POINT('Ctrl Pts',(-6.67995048580069,-1.10444249683336,
25.7492461074266));
#189538=CARTESIAN_POINT('Ctrl Pts',(-6.63659636700349,-1.32207324361249,
25.7597364328088));
#189539=CARTESIAN_POINT('Ctrl Pts',(-6.61113671010138,-1.44987665187149,
25.7658968644456));
#189540=CARTESIAN_POINT('Ctrl Pts',(-6.58199158231211,-1.576910575339,25.7720572960824));
#189541=CARTESIAN_POINT('Ctrl Pts',(-6.54920683200501,-1.70299115429851,
25.7782177277192));
#189542=CARTESIAN_POINT('Ctrl Pts',(-6.50544691960259,-1.87127900274119,
25.7864404515851));
#189543=CARTESIAN_POINT('Ctrl Pts',(-6.45513814673142,-2.03810301418025,
25.794663175451));
#189544=CARTESIAN_POINT('Ctrl Pts',(-6.39839414167517,-2.20291656850116,
25.8028858993169));
#189545=CARTESIAN_POINT('Ctrl Pts',(-6.34171019822605,-2.36755567325794,
25.8110999197081));
#189546=CARTESIAN_POINT('Ctrl Pts',(-6.27860470223396,-2.530188222065,25.8193139400993));
#189547=CARTESIAN_POINT('Ctrl Pts',(-6.20924188159528,-2.69027958692831,
25.8275279604905));
#189548=CARTESIAN_POINT('Ctrl Pts',(-6.13993855305911,-2.85023364232524,
25.8357349357625));
#189549=CARTESIAN_POINT('Ctrl Pts',(-6.06438873027047,-3.00765052726698,
25.8439419110344));
#189550=CARTESIAN_POINT('Ctrl Pts',(-5.98280588265044,-3.16201245578244,
25.8521488863064));
#189551=CARTESIAN_POINT('Ctrl Pts',(-5.90127663333316,-3.31627297159146,
25.8603504697594));
#189552=CARTESIAN_POINT('Ctrl Pts',(-5.81372242117327,-3.46748221275153,
25.8685520532124));
#189553=CARTESIAN_POINT('Ctrl Pts',(-5.72040412719173,-3.6151439282009,
25.8767536366654));
#189554=CARTESIAN_POINT('Ctrl Pts',(-5.6271284149782,-3.76273826461189,
25.8849514776804));
#189555=CARTESIAN_POINT('Ctrl Pts',(-5.52809405216928,-3.90678799766012,
25.8931493186955));
#189556=CARTESIAN_POINT('Ctrl Pts',(-5.42360704764637,-4.04682290108186,
25.9013471597106));
#189557=CARTESIAN_POINT('Ctrl Pts',(-5.31912926377572,-4.18684544686014,
25.9095442772917));
#189558=CARTESIAN_POINT('Ctrl Pts',(-5.20920000412085,-4.32285357629932,
25.9177413948729));
#189559=CARTESIAN_POINT('Ctrl Pts',(-5.09416786880838,-4.45440711255721,
25.925938512454));
#189560=CARTESIAN_POINT('Ctrl Pts',(-4.9791370133565,-4.58595918513554,
25.9341355388331));
#189561=CARTESIAN_POINT('Ctrl Pts',(-4.85900363072451,-4.71305649241487,
25.9423325652122));
#189562=CARTESIAN_POINT('Ctrl Pts',(-4.73415569167384,-4.83529305078732,
25.9505295915913));
#189563=CARTESIAN_POINT('Ctrl Pts',(-4.6092864405524,-4.95755047545683,
25.9587280172374));
#189564=CARTESIAN_POINT('Ctrl Pts',(-4.4797012860301,-5.07494524706564,
25.9669264428836));
#189565=CARTESIAN_POINT('Ctrl Pts',(-4.345824059073,-5.18710923806144,25.9751248685297));
#189566=CARTESIAN_POINT('Ctrl Pts',(-4.21189963550303,-5.29931277096127,
25.9833261844204));
#189567=CARTESIAN_POINT('Ctrl Pts',(-4.07368040025147,-5.40628161959457,
25.991527500311));
#189568=CARTESIAN_POINT('Ctrl Pts',(-3.93162218596216,-5.50768880628256,
25.9997288162017));
#189569=CARTESIAN_POINT('Ctrl Pts',(-3.78940219114661,-5.60921147878112,
26.0079394720183));
#189570=CARTESIAN_POINT('Ctrl Pts',(-3.64333477526494,-5.70515962682792,
26.0161501278349));
#189571=CARTESIAN_POINT('Ctrl Pts',(-3.49390448966299,-5.79524981490124,
26.0243607836515));
#189572=CARTESIAN_POINT('Ctrl Pts',(-3.34438614841412,-5.88539309093968,
26.0325762778086));
#189573=CARTESIAN_POINT('Ctrl Pts',(-3.19150130104384,-5.9696713531215,
26.0407917719657));
#189574=CARTESIAN_POINT('Ctrl Pts',(-3.03575775758443,-6.04784786823098,
26.0490072661229));
#189575=CARTESIAN_POINT('Ctrl Pts',(-2.87977257515131,-6.12614567564227,
26.0572355067704));
#189576=CARTESIAN_POINT('Ctrl Pts',(-2.72092015958877,-6.19832266890245,
26.0654637474179));
#189577=CARTESIAN_POINT('Ctrl Pts',(-2.55972813214299,-6.2641903618517,
26.0736919880654));
#189578=CARTESIAN_POINT('Ctrl Pts',(-2.41323031367543,-6.32405357889451,
26.0811701451665));
#189579=CARTESIAN_POINT('Ctrl Pts',(-2.26480039920582,-6.37870593032523,
26.0886483022676));
#189580=CARTESIAN_POINT('Ctrl Pts',(-2.1148433226718,-6.42804221521223,
26.0961264593687));
#189581=CARTESIAN_POINT('Ctrl Pts',(-1.95303206298607,-6.48127855850656,
26.1041957685913));
#189582=CARTESIAN_POINT('Ctrl Pts',(-1.78891270112995,-6.52849858136089,
26.1122650778138));
#189583=CARTESIAN_POINT('Ctrl Pts',(-1.62298210502701,-6.56949146332972,
26.1203343870363));
#189584=CARTESIAN_POINT('Ctrl Pts',(-1.45725846947591,-6.61043321603323,
26.1283936316371));
#189585=CARTESIAN_POINT('Ctrl Pts',(-1.28972845234976,-6.64516319362522,
26.1364528762378));
#189586=CARTESIAN_POINT('Ctrl Pts',(-1.12090811357158,-6.67351886195952,
26.1445121208386));
#189587=CARTESIAN_POINT('Ctrl Pts',(-0.952261292294172,-6.70184538567333,
26.1525630819588));
#189588=CARTESIAN_POINT('Ctrl Pts',(-0.782327153444256,-6.72381057677971,
26.1606140430791));
#189589=CARTESIAN_POINT('Ctrl Pts',(-0.611636012282423,-6.73930192145145,
26.1686650041994));
#189590=CARTESIAN_POINT('Ctrl Pts',(-0.441082909659608,-6.75478073821712,
26.1767094544785));
#189591=CARTESIAN_POINT('Ctrl Pts',(-0.269774392908001,-6.76379609521643,
26.1847539047576));
#189592=CARTESIAN_POINT('Ctrl Pts',(-0.0982499412038178,-6.76628671791652,
26.1927983550367));
#189593=CARTESIAN_POINT('Ctrl Pts',(0.0731733431595497,-6.76877587161511,
26.2008380605949));
#189594=CARTESIAN_POINT('Ctrl Pts',(0.24481193678314,-6.76474794657301,
26.2088777661531));
#189595=CARTESIAN_POINT('Ctrl Pts',(0.416122388243194,-6.75419359790662,
26.2169174717114));
#189596=CARTESIAN_POINT('Ctrl Pts',(0.591130484210459,-6.74341143926693,
26.2251307100158));
#189597=CARTESIAN_POINT('Ctrl Pts',(0.765795714195148,-6.72581787950676,
26.2333439483203));
#189598=CARTESIAN_POINT('Ctrl Pts',(0.939539422656506,-6.70145914508731,
26.2415571866247));
#189599=CARTESIAN_POINT('Ctrl Pts',(1.10955745408304,-6.67762274772528,
26.2495943041729));
#189600=CARTESIAN_POINT('Ctrl Pts',(1.27869270165765,-6.64730843924124,
26.2576314217211));
#189601=CARTESIAN_POINT('Ctrl Pts',(1.4464093433712,-6.61061184849092,26.2656685392693));
#189602=CARTESIAN_POINT('Ctrl Pts',(1.61414372843899,-6.57391137547463,
26.2737065070934));
#189603=CARTESIAN_POINT('Ctrl Pts',(1.78045884378302,-6.53082735551139,
26.2817444749175));
#189604=CARTESIAN_POINT('Ctrl Pts',(1.94483058238538,-6.48150622971378,
26.2897824427416));
#189605=CARTESIAN_POINT('Ctrl Pts',(2.10925227857359,-6.4321701137214,26.2978228535493));
#189606=CARTESIAN_POINT('Ctrl Pts',(2.27172906468335,-6.37659322595046,
26.3058632643571));
#189607=CARTESIAN_POINT('Ctrl Pts',(2.43175362115301,-6.31497136383129,
26.3139036751648));
#189608=CARTESIAN_POINT('Ctrl Pts',(2.59782620330735,-6.2510205428757,26.3222479681526));
#189609=CARTESIAN_POINT('Ctrl Pts',(2.76125715770875,-6.18055904831102,
26.3305922611404));
#189610=CARTESIAN_POINT('Ctrl Pts',(2.92150502034155,-6.10385922315703,
26.3389365541282));
#189611=CARTESIAN_POINT('Ctrl Pts',(3.0761896740647,-6.02982213024579,26.3469911643437));
#189612=CARTESIAN_POINT('Ctrl Pts',(3.22790824848203,-5.94997282165125,
26.3550457745593));
#189613=CARTESIAN_POINT('Ctrl Pts',(3.3762017846964,-5.86460147912992,26.3631003847748));
#189614=CARTESIAN_POINT('Ctrl Pts',(3.52460758121271,-5.77916550929621,
26.3711610924441));
#189615=CARTESIAN_POINT('Ctrl Pts',(3.6695828627128,-5.68819937932786,26.3792218001133));
#189616=CARTESIAN_POINT('Ctrl Pts',(3.81069979433565,-5.59203505688673,
26.3872825077826));
#189617=CARTESIAN_POINT('Ctrl Pts',(3.95201569237733,-5.49573514851249,
26.3953545805667));
#189618=CARTESIAN_POINT('Ctrl Pts',(4.08946208910927,-5.39422264460989,
26.4034266533509));
#189619=CARTESIAN_POINT('Ctrl Pts',(4.22264574554371,-5.28786837086946,
26.411498726135));
#189620=CARTESIAN_POINT('Ctrl Pts',(4.23659572165705,-5.27672856874997,
26.4123442144294));
#189621=CARTESIAN_POINT('Ctrl Pts',(4.25049896631731,-5.26553567933751,
26.4131897027239));
#189622=CARTESIAN_POINT('Ctrl Pts',(4.26435505247544,-5.25429015057478,
26.4140351910183));
#189623=CARTESIAN_POINT('Ctrl Pts',(4.40091718655803,-5.14345701997803,
26.422368113065));
#189624=CARTESIAN_POINT('Ctrl Pts',(4.53333104155898,-5.02715422503498,
26.4307010351117));
#189625=CARTESIAN_POINT('Ctrl Pts',(4.66113772746193,-4.90571952781965,
26.4390339571584));
#189626=CARTESIAN_POINT('Ctrl Pts',(4.78879337685559,-4.7844283369682,26.447357031712));
#189627=CARTESIAN_POINT('Ctrl Pts',(4.91185245304282,-4.65801756275112,
26.4556801062656));
#189628=CARTESIAN_POINT('Ctrl Pts',(5.02988801979945,-4.5268659697718,26.4640031808192));
#189629=CARTESIAN_POINT('Ctrl Pts',(5.14780576324589,-4.3958452925431,26.4723179472652));
#189630=CARTESIAN_POINT('Ctrl Pts',(5.26070975639224,-4.26009348182202,
26.4806327137112));
#189631=CARTESIAN_POINT('Ctrl Pts',(5.3682087626124,-4.12002714566439,26.4889474801571));
#189632=CARTESIAN_POINT('Ctrl Pts',(5.47562018207194,-3.98007493108879,
26.4972554719967));
#189633=CARTESIAN_POINT('Ctrl Pts',(5.57763517863231,-3.8358154705114,26.5055634638362));
#189634=CARTESIAN_POINT('Ctrl Pts',(5.67390164120109,-3.6876997120123,26.5138714556757));
#189635=CARTESIAN_POINT('Ctrl Pts',(5.77010731780679,-3.53967747890914,
26.5221742015628));
#189636=CARTESIAN_POINT('Ctrl Pts',(5.86057150514518,-3.38780409146745,
26.5304769474499));
#189637=CARTESIAN_POINT('Ctrl Pts',(5.94498429228834,-3.23256102254002,
26.538779693337));
#189638=CARTESIAN_POINT('Ctrl Pts',(6.02936258261544,-3.07738139650758,
26.5470790461564));
#189639=CARTESIAN_POINT('Ctrl Pts',(6.10769423447064,-2.91883513810672,
26.5553783989759));
#189640=CARTESIAN_POINT('Ctrl Pts',(6.17971420174618,-2.75743021393771,
26.5636777517953));
#189641=CARTESIAN_POINT('Ctrl Pts',(6.25171885158313,-2.59605961788781,
26.5719753394816));
#189642=CARTESIAN_POINT('Ctrl Pts',(6.31741434950007,-2.43183188485109,
26.580272927168));
#189643=CARTESIAN_POINT('Ctrl Pts',(6.37658281042349,-2.26527717107899,
26.5885705148543));
#189644=CARTESIAN_POINT('Ctrl Pts',(6.43574851954211,-2.09873020342796,
26.5968677166367));
#189645=CARTESIAN_POINT('Ctrl Pts',(6.48838768027942,-1.92985679856605,
26.6051649184192));
#189646=CARTESIAN_POINT('Ctrl Pts',(6.534331461314,-1.75920475035799,26.6134621202016));
#189647=CARTESIAN_POINT('Ctrl Pts',(6.58028073997568,-1.58853228194713,
26.6217603148261));
#189648=CARTESIAN_POINT('Ctrl Pts',(6.61953295265388,-1.41608108217307,
26.6300585094507));
#189649=CARTESIAN_POINT('Ctrl Pts',(6.65196976459586,-1.24241186846493,
26.6383567040752));
#189650=CARTESIAN_POINT('Ctrl Pts',(6.68442938972586,-1.06862051117402,
26.6466607349168));
#189651=CARTESIAN_POINT('Ctrl Pts',(6.71006397210905,-0.893609770615906,
26.6549647657583));
#189652=CARTESIAN_POINT('Ctrl Pts',(6.72880657986409,-0.717949170051566,
26.6632687965999));
#189653=CARTESIAN_POINT('Ctrl Pts',(6.74755600294716,-0.542224694458191,
26.6715758470157));
#189654=CARTESIAN_POINT('Ctrl Pts',(6.7594084268463,-0.365850234545319,
26.6798828974314));
#189655=CARTESIAN_POINT('Ctrl Pts',(6.76434899034665,-0.189398354787832,
26.6881899478471));
#189656=CARTESIAN_POINT('Ctrl Pts',(6.7692948361432,-0.012757818190803,
26.6965058799017));
#189657=CARTESIAN_POINT('Ctrl Pts',(6.76731405399805,0.16395995547355,26.7048218119564));
#189658=CARTESIAN_POINT('Ctrl Pts',(6.75844392386799,0.340183373979205,
26.713137744011));
#189659=CARTESIAN_POINT('Ctrl Pts',(6.75175743136825,0.47302432995617,26.7194064702299));
#189660=CARTESIAN_POINT('Ctrl Pts',(6.74115717014622,0.605584394745327,
26.7256751964489));
#189661=CARTESIAN_POINT('Ctrl Pts',(6.72667848189171,0.73762158404906,26.7319439226678));
#189662=CARTESIAN_POINT('Ctrl Pts',(6.70716115058081,0.915608258235449,
26.7403941913911));
#189663=CARTESIAN_POINT('Ctrl Pts',(6.6805587082356,1.09297090926716,26.7488444601145));
#189664=CARTESIAN_POINT('Ctrl Pts',(6.64692513480987,1.26912381280664,26.7572947288378));
#189665=CARTESIAN_POINT('Ctrl Pts',(6.61332124415374,1.44512125543255,26.7657375399124));
#189666=CARTESIAN_POINT('Ctrl Pts',(6.57269865242034,1.61991075439046,26.7741803509869));
#189667=CARTESIAN_POINT('Ctrl Pts',(6.52516297638257,1.79291302958236,26.7826231620614));
#189668=CARTESIAN_POINT('Ctrl Pts',(6.47766278008718,1.96578617910136,26.7910596715791));
#189669=CARTESIAN_POINT('Ctrl Pts',(6.4232598728177,2.13687444532391,26.7994961810969));
#189670=CARTESIAN_POINT('Ctrl Pts',(6.36211074219677,2.30560965994344,26.8079326906146));
#189671=CARTESIAN_POINT('Ctrl Pts',(6.30100536706913,2.47422413543755,26.8163631633558));
#189672=CARTESIAN_POINT('Ctrl Pts',(6.23316351008926,2.64048860682208,26.824793636097));
#189673=CARTESIAN_POINT('Ctrl Pts',(6.15879126699945,2.80385076805656,26.8332241088383));
#189674=CARTESIAN_POINT('Ctrl Pts',(6.08445099633536,2.96714270034071,26.8416509573421));
#189675=CARTESIAN_POINT('Ctrl Pts',(6.00358607333728,3.12753450857203,26.8500778058459));
#189676=CARTESIAN_POINT('Ctrl Pts',(5.91645067090267,3.28449394256945,26.8585046543498));
#189677=CARTESIAN_POINT('Ctrl Pts',(5.82934216405502,3.4414049287949,26.8669289017864));
#189678=CARTESIAN_POINT('Ctrl Pts',(5.73596719831479,3.59488536401621,26.875353149223));
#189679=CARTESIAN_POINT('Ctrl Pts',(5.63662600763035,3.74442735943764,26.8837773966597));
#189680=CARTESIAN_POINT('Ctrl Pts',(5.60863546094804,3.78656257218244,26.8861510272706));
#189681=CARTESIAN_POINT('Ctrl Pts',(5.58017153174439,3.82838527373419,26.8885246578816));
#189682=CARTESIAN_POINT('Ctrl Pts',(5.55124157285383,3.86988449437698,26.8908982884926));
#189683=CARTESIAN_POINT('Ctrl Pts',(5.44619741654609,4.02056741225946,26.8995168982133));
#189684=CARTESIAN_POINT('Ctrl Pts',(5.33505285427677,4.16691585411189,26.9081355079341));
#189685=CARTESIAN_POINT('Ctrl Pts',(5.21819431125555,4.30844950416971,26.9167541176549));
#189686=CARTESIAN_POINT('Ctrl Pts',(5.10126561269086,4.45006812336955,26.9253779015224));
#189687=CARTESIAN_POINT('Ctrl Pts',(4.97861628106307,4.58686594761258,26.9340016853899));
#189688=CARTESIAN_POINT('Ctrl Pts',(4.85067173123851,4.71839726557266,26.9426254692573));
#189689=CARTESIAN_POINT('Ctrl Pts',(4.72256918962313,4.85009100442916,26.9512599021682));
#189690=CARTESIAN_POINT('Ctrl Pts',(4.58915857053572,4.97650501759553,26.959894335079));
#189691=CARTESIAN_POINT('Ctrl Pts',(4.45090196717683,5.09723068720471,26.9685287679899));
#189692=CARTESIAN_POINT('Ctrl Pts',(4.31256466970492,5.21802681891546,26.9771682404278));
#189693=CARTESIAN_POINT('Ctrl Pts',(4.16937597702939,5.33312778630485,26.9858077128658));
#189694=CARTESIAN_POINT('Ctrl Pts',(4.02183034662315,5.44216589814948,26.9944471853038));
#189695=CARTESIAN_POINT('Ctrl Pts',(3.87409389252246,5.55134503114995,27.0030978313431));
#189696=CARTESIAN_POINT('Ctrl Pts',(3.72198948335512,5.65444545512441,27.0117484773824));
#189697=CARTESIAN_POINT('Ctrl Pts',(3.56604131887359,5.75114234844577,27.0203991234217));
#189698=CARTESIAN_POINT('Ctrl Pts',(3.4138854502671,5.8454877987034,27.0288394059123));
#189699=CARTESIAN_POINT('Ctrl Pts',(3.25807084116531,5.93373743027089,27.0372796884029));
#189700=CARTESIAN_POINT('Ctrl Pts',(3.09910619832137,6.01563211736939,27.0457199708935));
#189701=CARTESIAN_POINT('Ctrl Pts',(3.09910619832135,6.0156321173694,25.0456877277983));
#189702=CARTESIAN_POINT('Ctrl Pts',(2.9450685624596,6.09498853125241,25.0538144835559));
#189703=CARTESIAN_POINT('Ctrl Pts',(2.78802739907583,6.16840065421879,25.0619412393135));
#189704=CARTESIAN_POINT('Ctrl Pts',(2.62849061198312,6.23564961352998,25.070067995071));
#189705=CARTESIAN_POINT('Ctrl Pts',(2.46890098615892,6.30292084575872,25.0781974424176));
#189706=CARTESIAN_POINT('Ctrl Pts',(2.30681443123484,6.36402471473129,25.0863268897642));
#189707=CARTESIAN_POINT('Ctrl Pts',(2.14275652578268,6.41879143384608,25.0944563371108));
#189708=CARTESIAN_POINT('Ctrl Pts',(1.97850459579159,6.47362292330762,25.1025953988205));
#189709=CARTESIAN_POINT('Ctrl Pts',(1.81227700760014,6.52210218138668,25.1107344605303));
#189710=CARTESIAN_POINT('Ctrl Pts',(1.64461311299654,6.56410974226969,25.11887352224));
#189711=CARTESIAN_POINT('Ctrl Pts',(1.48306356498732,6.60458537651202,25.1267157696334));
#189712=CARTESIAN_POINT('Ctrl Pts',(1.3201809157762,6.63905298337215,25.1345580170268));
#189713=CARTESIAN_POINT('Ctrl Pts',(1.15645336321713,6.66745113358199,25.1424002644202));
#189714=CARTESIAN_POINT('Ctrl Pts',(0.980241778927664,6.6980146090701,25.1508404738778));
#189715=CARTESIAN_POINT('Ctrl Pts',(0.802687245849629,6.72161091930514,
25.1592806833354));
#189716=CARTESIAN_POINT('Ctrl Pts',(0.624366915154841,6.73813438239844,
25.167720892793));
#189717=CARTESIAN_POINT('Ctrl Pts',(0.446181688529219,6.75464532652046,
25.1761547075415));
#189718=CARTESIAN_POINT('Ctrl Pts',(0.267232151754892,6.76409407510952,
25.18458852229));
#189719=CARTESIAN_POINT('Ctrl Pts',(0.088103036568935,6.76642644643,25.1930223370385));
#189720=CARTESIAN_POINT('Ctrl Pts',(-0.0909178987375423,6.76875740918187,
25.2014510584271));
#189721=CARTESIAN_POINT('Ctrl Pts',(-0.270117863622306,6.76398055847807,
25.2098797798156));
#189722=CARTESIAN_POINT('Ctrl Pts',(-0.448909246482972,6.75209371146625,
25.2183085012042));
#189723=CARTESIAN_POINT('Ctrl Pts',(-0.62762010826532,6.74021221785416,
25.2267334266059));
#189724=CARTESIAN_POINT('Ctrl Pts',(-0.805922422723691,6.72122713460942,
25.2351583520076));
#189725=CARTESIAN_POINT('Ctrl Pts',(-0.983230425147443,6.69518834171709,
25.2435832774093));
#189726=CARTESIAN_POINT('Ctrl Pts',(-1.16048577885641,6.66915728061893,
25.2520057011671));
#189727=CARTESIAN_POINT('Ctrl Pts',(-1.33674707972042,6.6360767351359,25.2604281249248));
#189728=CARTESIAN_POINT('Ctrl Pts',(-1.51143512247197,6.59604827685169,
25.2688505486826));
#189729=CARTESIAN_POINT('Ctrl Pts',(-1.68612591256256,6.55601918903529,
25.2772731049008));
#189730=CARTESIAN_POINT('Ctrl Pts',(-1.8592430686407,6.50904203807539,25.2856956611189));
#189731=CARTESIAN_POINT('Ctrl Pts',(-2.03021833266987,6.45526936089356,
25.2941182173371));
#189732=CARTESIAN_POINT('Ctrl Pts',(-2.20119937227635,6.40149486726035,
25.3025410580709));
#189733=CARTESIAN_POINT('Ctrl Pts',(-2.37003805730619,6.34092448961307,
25.3109638988046));
#189734=CARTESIAN_POINT('Ctrl Pts',(-2.53618188283675,6.27376047177215,
25.3193867395384));
#189735=CARTESIAN_POINT('Ctrl Pts',(-2.70235451625344,6.20658480827799,
25.327811040719));
#189736=CARTESIAN_POINT('Ctrl Pts',(-2.86583104933623,6.13281335024041,
25.3362353418997));
#189737=CARTESIAN_POINT('Ctrl Pts',(-3.02607919064693,6.05269640176456,
25.3446596430804));
#189738=CARTESIAN_POINT('Ctrl Pts',(-3.18637749685227,5.97255437307095,
25.3530865814472));
#189739=CARTESIAN_POINT('Ctrl Pts',(-3.34344509812326,5.88606304265238,
25.361513519814));
#189740=CARTESIAN_POINT('Ctrl Pts',(-3.49677420398641,5.79351872063388,
25.3699404581808));
#189741=CARTESIAN_POINT('Ctrl Pts',(-3.65024117198855,5.70089118963746,
25.3783749734245));
#189742=CARTESIAN_POINT('Ctrl Pts',(-3.79996264216661,5.60219996479436,
25.3868094886681));
#189743=CARTESIAN_POINT('Ctrl Pts',(-3.94545876740386,5.49778538274422,
25.3952440039118));
#189744=CARTESIAN_POINT('Ctrl Pts',(-4.0910251685169,5.39332036755583,25.4036825930986));
#189745=CARTESIAN_POINT('Ctrl Pts',(-4.23236188833583,5.28312668275323,
25.4121211822854));
#189746=CARTESIAN_POINT('Ctrl Pts',(-4.36902169349185,5.16758535892709,
25.4205597714722));
#189747=CARTESIAN_POINT('Ctrl Pts',(-4.50583425339036,5.05191488604247,
25.4290077930925));
#189748=CARTESIAN_POINT('Ctrl Pts',(-4.63795920331072,4.93088505172183,
25.4374558147128));
#189749=CARTESIAN_POINT('Ctrl Pts',(-4.7649848536557,4.80491501948076,25.445903836333));
#189750=CARTESIAN_POINT('Ctrl Pts',(-4.83718419476079,4.73331567476501,
25.4507055562453));
#189751=CARTESIAN_POINT('Ctrl Pts',(-4.90773684972699,4.66012100067557,
25.4555072761575));
#189752=CARTESIAN_POINT('Ctrl Pts',(-4.97657296742492,4.58541279492867,
25.4603089960697));
#189753=CARTESIAN_POINT('Ctrl Pts',(-5.09469259843769,4.45721692927607,
25.4685485279206));
#189754=CARTESIAN_POINT('Ctrl Pts',(-5.20801925773606,4.32427641299698,
25.4767880597714));
#189755=CARTESIAN_POINT('Ctrl Pts',(-5.31615128256397,4.18698274905611,
25.4850275916222));
#189756=CARTESIAN_POINT('Ctrl Pts',(-5.42416328840127,4.04984147148727,
25.4932579781685));
#189757=CARTESIAN_POINT('Ctrl Pts',(-5.52699192193546,3.90835694409848,
25.5014883647148));
#189758=CARTESIAN_POINT('Ctrl Pts',(-5.62427273543654,3.76295697522908,
25.5097187512611));
#189759=CARTESIAN_POINT('Ctrl Pts',(-5.72146292803638,3.61769245214539,
25.5179414708788));
#189760=CARTESIAN_POINT('Ctrl Pts',(-5.81311539604065,3.46852004548224,
25.5261641904966));
#189761=CARTESIAN_POINT('Ctrl Pts',(-5.89890628069536,3.31590013293116,
25.5343869101143));
#189762=CARTESIAN_POINT('Ctrl Pts',(-5.98462114844598,3.16341545261717,
25.5426023438101));
#189763=CARTESIAN_POINT('Ctrl Pts',(-6.06448461081675,3.00748966386387,
25.5508177775059));
#189764=CARTESIAN_POINT('Ctrl Pts',(-6.13821649410676,2.8486114637619,25.5590332112018));
#189765=CARTESIAN_POINT('Ctrl Pts',(-6.21191048493394,2.68981491471812,
25.5672444228026));
#189766=CARTESIAN_POINT('Ctrl Pts',(-6.27947902302974,2.52806929822944,
25.5754556344034));
#189767=CARTESIAN_POINT('Ctrl Pts',(-6.34068801540674,2.36388758008441,
25.5836668460042));
#189768=CARTESIAN_POINT('Ctrl Pts',(-6.40187648166539,2.19976091942762,
25.5918753040177));
#189769=CARTESIAN_POINT('Ctrl Pts',(-6.4567095264163,2.03320011764541,25.6000837620313));
#189770=CARTESIAN_POINT('Ctrl Pts',(-6.5050012852481,1.86473785796304,25.6082922200448));
#189771=CARTESIAN_POINT('Ctrl Pts',(-6.5265163182963,1.78968424276826,25.611949267328));
#189772=CARTESIAN_POINT('Ctrl Pts',(-6.54673362252307,1.71425344630615,
25.6156063146112));
#189773=CARTESIAN_POINT('Ctrl Pts',(-6.56563993181014,1.63849360261803,
25.6192633618944));
#189774=CARTESIAN_POINT('Ctrl Pts',(-6.60796019411089,1.46891124743364,
25.6274493699577));
#189775=CARTESIAN_POINT('Ctrl Pts',(-6.64368652839661,1.29776665582351,
25.635635378021));
#189776=CARTESIAN_POINT('Ctrl Pts',(-6.67272679056475,1.12561368971754,
25.6438213860843));
#189777=CARTESIAN_POINT('Ctrl Pts',(-6.70178059404674,0.953380449634272,
25.6520112112379));
#189778=CARTESIAN_POINT('Ctrl Pts',(-6.72414206363312,0.780138252551122,
25.6602010363916));
#189779=CARTESIAN_POINT('Ctrl Pts',(-6.7397709151484,0.606446214696485,
25.6683908615452));
#189780=CARTESIAN_POINT('Ctrl Pts',(-6.75541550510242,0.432579266900768,
25.6765889339499));
#189781=CARTESIAN_POINT('Ctrl Pts',(-6.76431392100477,0.258261930867931,
25.6847870063546));
#189782=CARTESIAN_POINT('Ctrl Pts',(-6.766477954304,0.084054113034077,25.6929850787592));
#189783=CARTESIAN_POINT('Ctrl Pts',(-6.76684704437416,0.0543418273087019,
25.6943833137679));
#189784=CARTESIAN_POINT('Ctrl Pts',(-6.76702035669943,0.024632717883948,
25.6957815487766));
#189785=CARTESIAN_POINT('Ctrl Pts',(-6.76699810037806,-0.00507045163497854,
25.6971797837853));
#189786=CARTESIAN_POINT('',(-6.76699999946963,-8.47234480375662E-5,25.3028202161501));
#189787=CARTESIAN_POINT('Ctrl Pts',(3.09910619832136,6.01563211736939,24.6515493092843));
#189788=CARTESIAN_POINT('Ctrl Pts',(2.94284574041202,6.09613367468057,24.6597832037901));
#189789=CARTESIAN_POINT('Ctrl Pts',(2.78337708565397,6.17057824749298,24.668017098296));
#189790=CARTESIAN_POINT('Ctrl Pts',(2.62122488019941,6.23870732823905,24.6762509928018));
#189791=CARTESIAN_POINT('Ctrl Pts',(2.46294786818989,6.30520822658461,24.6842881096325));
#189792=CARTESIAN_POINT('Ctrl Pts',(2.3021144789861,6.36569192592313,24.6923252264631));
#189793=CARTESIAN_POINT('Ctrl Pts',(2.13923395749237,6.41996628301984,24.7003623432938));
#189794=CARTESIAN_POINT('Ctrl Pts',(1.97633678479312,6.47424618856069,24.7084002817554));
#189795=CARTESIAN_POINT('Ctrl Pts',(1.811392417538,6.52231536966561,24.7164382202171));
#189796=CARTESIAN_POINT('Ctrl Pts',(1.64492605312687,6.56403132836403,24.7244761586787));
#189797=CARTESIAN_POINT('Ctrl Pts',(1.47840968798621,6.60575981709142,24.7325165114587));
#189798=CARTESIAN_POINT('Ctrl Pts',(1.31037077793987,6.64113119421398,24.7405568642386));
#189799=CARTESIAN_POINT('Ctrl Pts',(1.14134537031516,6.67005395372932,24.7485972170185));
#189800=CARTESIAN_POINT('Ctrl Pts',(0.965170110909029,6.70020015915467,
24.7569776803857));
#189801=CARTESIAN_POINT('Ctrl Pts',(0.787923523518979,6.7233402141603,24.7653581437529));
#189802=CARTESIAN_POINT('Ctrl Pts',(0.610218097680674,6.73943045614858,
24.77373860712));
#189803=CARTESIAN_POINT('Ctrl Pts',(0.439423832667417,6.75489493080549,
24.7817931449852));
#189804=CARTESIAN_POINT('Ctrl Pts',(0.268206116151743,6.7638476589083,24.7898476828504));
#189805=CARTESIAN_POINT('Ctrl Pts',(0.0971077703182675,6.76630320640036,
24.7979022207156));
#189806=CARTESIAN_POINT('Ctrl Pts',(-0.0741196886831647,6.76876060688238,
24.805962836646));
#189807=CARTESIAN_POINT('Ctrl Pts',(-0.245227226744314,6.76471107333792,
24.8140234525764));
#189808=CARTESIAN_POINT('Ctrl Pts',(-0.415677386113846,6.75422099954344,
24.8220840685068));
#189809=CARTESIAN_POINT('Ctrl Pts',(-0.586368499081741,6.74371609665735,
24.8301560791723));
#189810=CARTESIAN_POINT('Ctrl Pts',(-0.756400011002734,6.72675252473188,
24.8382280898378));
#189811=CARTESIAN_POINT('Ctrl Pts',(-0.925244300123992,6.703447768506,24.8463001005033));
#189812=CARTESIAN_POINT('Ctrl Pts',(-0.945204079241676,6.70069281724836,
24.8472543261438));
#189813=CARTESIAN_POINT('Ctrl Pts',(-0.965147284995377,6.69784930783103,
24.8482085517842));
#189814=CARTESIAN_POINT('Ctrl Pts',(-0.985073060579621,6.69491748009789,
24.8491627774246));
#189815=CARTESIAN_POINT('Ctrl Pts',(-1.1590779579849,6.66931484386639,24.8574956994713));
#189816=CARTESIAN_POINT('Ctrl Pts',(-1.33230753138869,6.63689133378378,
24.865828621518));
#189817=CARTESIAN_POINT('Ctrl Pts',(-1.50419476867123,6.59770316836868,
24.8741615435647));
#189818=CARTESIAN_POINT('Ctrl Pts',(-1.6758788769231,6.55856131386171,24.8824846181184));
#189819=CARTESIAN_POINT('Ctrl Pts',(-1.84622347277167,6.51267080574074,
24.890807692672));
#189820=CARTESIAN_POINT('Ctrl Pts',(-2.01466809300645,6.46013943154649,
24.8991307672256));
#189821=CARTESIAN_POINT('Ctrl Pts',(-2.18294457152471,6.40766049426246,
24.9074455336716));
#189822=CARTESIAN_POINT('Ctrl Pts',(-2.34932452287968,6.34855400079885,
24.9157603001176));
#189823=CARTESIAN_POINT('Ctrl Pts',(-2.51325886634617,6.28297850312512,
24.9240750665635));
#189824=CARTESIAN_POINT('Ctrl Pts',(-2.67705964134008,6.21745643427464,
24.9323830584031));
#189825=CARTESIAN_POINT('Ctrl Pts',(-2.8384184572062,6.14547599226639,24.9406910502426));
#189826=CARTESIAN_POINT('Ctrl Pts',(-2.99680234998407,6.06724522951973,
24.9489990420822));
#189827=CARTESIAN_POINT('Ctrl Pts',(-3.15508623371199,5.98906386437357,
24.9573017879693));
#189828=CARTESIAN_POINT('Ctrl Pts',(-3.31039862682985,5.9046401973843,24.9656045338564));
#189829=CARTESIAN_POINT('Ctrl Pts',(-3.46222727349032,5.81423006998345,
24.9739072797435));
#189830=CARTESIAN_POINT('Ctrl Pts',(-3.61399387262131,5.72385689032053,
24.9822066325629));
#189831=CARTESIAN_POINT('Ctrl Pts',(-3.76227926364622,5.62750230276009,
24.9905059853824));
#189832=CARTESIAN_POINT('Ctrl Pts',(-3.9065962477699,5.52546783149718,24.9988053382018));
#189833=CARTESIAN_POINT('Ctrl Pts',(-4.05088253809232,5.42345506125443,
25.0071029258881));
#189834=CARTESIAN_POINT('Ctrl Pts',(-4.19120181906805,5.3157650146793,25.0154005135745));
#189835=CARTESIAN_POINT('Ctrl Pts',(-4.32709612044553,5.20274236959945,
25.0236981012608));
#189836=CARTESIAN_POINT('Ctrl Pts',(-4.46298410165557,5.08972498097284,
25.0319953030432));
#189837=CARTESIAN_POINT('Ctrl Pts',(-4.59444724600527,4.97137571063061,
25.0402925048257));
#189838=CARTESIAN_POINT('Ctrl Pts',(-4.72106076285954,4.8480794417365,25.0485897066081));
#189839=CARTESIAN_POINT('Ctrl Pts',(-4.84768943027238,4.72476841922532,
25.0568879012327));
#189840=CARTESIAN_POINT('Ctrl Pts',(-4.96946706504823,4.59650946175034,
25.0651860958573));
#189841=CARTESIAN_POINT('Ctrl Pts',(-5.08600570305688,4.46372434055609,
25.0734842904819));
#189842=CARTESIAN_POINT('Ctrl Pts',(-5.20262630404737,4.3308458300391,25.0817883213235));
#189843=CARTESIAN_POINT('Ctrl Pts',(-5.31400031585095,4.19343505673715,
25.0900923521651));
#189844=CARTESIAN_POINT('Ctrl Pts',(-5.41977948199487,4.05194760165374,
25.0983963830066));
#189845=CARTESIAN_POINT('Ctrl Pts',(-5.52559711235487,3.9104086978376,25.1067034334224));
#189846=CARTESIAN_POINT('Ctrl Pts',(-5.62581563978829,3.76479044066879,
25.1150104838381));
#189847=CARTESIAN_POINT('Ctrl Pts',(-5.72013003215047,3.61557760465604,
25.1233175342538));
#189848=CARTESIAN_POINT('Ctrl Pts',(-5.81454526251574,3.4662052349386,25.1316334663085));
#189849=CARTESIAN_POINT('Ctrl Pts',(-5.90304356559838,3.31323090579058,
25.1399493983631));
#189850=CARTESIAN_POINT('Ctrl Pts',(-5.98536524279265,3.15716516995384,
25.1482653304177));
#189851=CARTESIAN_POINT('Ctrl Pts',(-6.04742107162982,3.03951950333827,
25.1545340566365));
#189852=CARTESIAN_POINT('Ctrl Pts',(-6.10596799486901,2.92011768554067,
25.1608027828553));
#189853=CARTESIAN_POINT('Ctrl Pts',(-6.16091288811307,2.79918584325556,
25.1670715090741));
#189854=CARTESIAN_POINT('Ctrl Pts',(-6.2362297338961,2.63341602593716,25.1756644948459));
#189855=CARTESIAN_POINT('Ctrl Pts',(-6.30490854911061,2.46448051554261,
25.1842574806176));
#189856=CARTESIAN_POINT('Ctrl Pts',(-6.36669181460124,2.29292920472691,
25.1928504663894));
#189857=CARTESIAN_POINT('Ctrl Pts',(-6.42841383145778,2.12154796073075,
25.2014349335334));
#189858=CARTESIAN_POINT('Ctrl Pts',(-6.48325382472646,1.94755637993255,
25.2100194006774));
#189859=CARTESIAN_POINT('Ctrl Pts',(-6.53100212792579,1.77152482484124,
25.2186038678214));
#189860=CARTESIAN_POINT('Ctrl Pts',(-6.57869426496486,1.5957003350459,25.227178237087));
#189861=CARTESIAN_POINT('Ctrl Pts',(-6.61931127585403,1.41784095939495,
25.2357526063527));
#189862=CARTESIAN_POINT('Ctrl Pts',(-6.65269309676399,1.23853282567268,
25.2443269756183));
#189863=CARTESIAN_POINT('Ctrl Pts',(-6.68605066955921,1.05935493901554,
25.2528951165751));
#189864=CARTESIAN_POINT('Ctrl Pts',(-6.71218347386952,0.878730698365294,
25.2614632575319));
#189865=CARTESIAN_POINT('Ctrl Pts',(-6.73098208979044,0.697258278488218,
25.2700313984888));
#189866=CARTESIAN_POINT('Ctrl Pts',(-6.74976551552573,0.515932497052884,
25.2785926159757));
#189867=CARTESIAN_POINT('Ctrl Pts',(-6.76122654452264,0.333760213529871,
25.2871538334626));
#189868=CARTESIAN_POINT('Ctrl Pts',(-6.76530731846125,0.151346908705136,
25.2957150509495));
#189869=CARTESIAN_POINT('Ctrl Pts',(-6.76643623005296,0.100883810921509,
25.2980834393497));
#189870=CARTESIAN_POINT('Ctrl Pts',(-6.76700063157175,0.0504023040753878,
25.3004518277499));
#189871=CARTESIAN_POINT('Ctrl Pts',(-6.76699999946963,-8.47234480193804E-5,
25.3028202161501));
#189872=CARTESIAN_POINT('Ctrl Pts',(-6.76699999946962,-8.4724297419803E-5,
25.3028202161899));
#189873=CARTESIAN_POINT('Ctrl Pts',(-6.76699793498657,-0.164976700326648,
25.3105554357596));
#189874=CARTESIAN_POINT('Ctrl Pts',(-6.7609652682336,-0.329871544089191,
25.3182906553293));
#189875=CARTESIAN_POINT('Ctrl Pts',(-6.74892353752594,-0.494287451417036,
25.3260258748989));
#189876=CARTESIAN_POINT('Ctrl Pts',(-6.73550633092438,-0.677483891426879,
25.3346446558361));
#189877=CARTESIAN_POINT('Ctrl Pts',(-6.71463052610296,-0.860066816299092,
25.3432634367734));
#189878=CARTESIAN_POINT('Ctrl Pts',(-6.68638325743214,-1.04142591418264,
25.3518822177106));
#189879=CARTESIAN_POINT('Ctrl Pts',(-6.65811902079877,-1.22289395337372,
25.3605061758971));
#189880=CARTESIAN_POINT('Ctrl Pts',(-6.62247453019704,-1.40313639789951,
25.3691301340837));
#189881=CARTESIAN_POINT('Ctrl Pts',(-6.57958811526716,-1.58155279185841,
25.3777540922702));
#189882=CARTESIAN_POINT('Ctrl Pts',(-6.53515236049314,-1.76641476137923,
25.3866896046413));
#189883=CARTESIAN_POINT('Ctrl Pts',(-6.48294176403342,-1.94931593270744,
25.3956251170125));
#189884=CARTESIAN_POINT('Ctrl Pts',(-6.42316651510862,-2.12960581309954,
25.4045606293836));
#189885=CARTESIAN_POINT('Ctrl Pts',(-6.36536758601136,-2.30393485733067,
25.4132007112783));
#189886=CARTESIAN_POINT('Ctrl Pts',(-6.30049636211091,-2.47582224998501,
25.421840793173));
#189887=CARTESIAN_POINT('Ctrl Pts',(-6.22879206359173,-2.64470006400286,
25.4304808750677));
#189888=CARTESIAN_POINT('Ctrl Pts',(-6.15341008550919,-2.82223954124237,
25.439564102677));
#189889=CARTESIAN_POINT('Ctrl Pts',(-6.07047586045127,-2.99645225588371,
25.4486473302863));
#189890=CARTESIAN_POINT('Ctrl Pts',(-5.98032242155961,-3.16670692268664,
25.4577305578956));
#189891=CARTESIAN_POINT('Ctrl Pts',(-5.89016898266796,-3.33696158948953,
25.466813785505));
#189892=CARTESIAN_POINT('Ctrl Pts',(-5.7927965549236,-3.50325789082802,
25.4758970131143));
#189893=CARTESIAN_POINT('Ctrl Pts',(-5.68859152615251,-3.6649986969419,
25.4849802407236));
#189894=CARTESIAN_POINT('Ctrl Pts',(-5.58482970181796,-3.82605158766739,
25.4940248355834));
#189895=CARTESIAN_POINT('Ctrl Pts',(-5.47419818896963,-3.98273685442638,
25.5030694304433));
#189896=CARTESIAN_POINT('Ctrl Pts',(-5.35707221927229,-4.13449709608086,
25.5121140253031));
#189897=CARTESIAN_POINT('Ctrl Pts',(-5.2400537310889,-4.2861180738251,25.5211503203234));
#189898=CARTESIAN_POINT('Ctrl Pts',(-5.11655282982289,-4.43282286147519,
25.5301866153437));
#189899=CARTESIAN_POINT('Ctrl Pts',(-4.98698663541845,-4.57408496840164,
25.5392229103641));
#189900=CARTESIAN_POINT('Ctrl Pts',(-4.85764971855503,-4.7150971009527,
25.5482432149518));
#189901=CARTESIAN_POINT('Ctrl Pts',(-4.72226910160204,-4.8506856100701,
25.5572635195395));
#189902=CARTESIAN_POINT('Ctrl Pts',(-4.58130040763553,-4.9803589805353,
25.5662838241272));
#189903=CARTESIAN_POINT('Ctrl Pts',(-4.44050923635512,-5.10986905258016,
25.5752927693935));
#189904=CARTESIAN_POINT('Ctrl Pts',(-4.29414420624897,-5.23347869097792,
25.5843017146598));
#189905=CARTESIAN_POINT('Ctrl Pts',(-4.14269763601296,-5.35073315505199,
25.5933106599261));
#189906=CARTESIAN_POINT('Ctrl Pts',(-3.99159496887706,-5.46772135906066,
25.6022991477849));
#189907=CARTESIAN_POINT('Ctrl Pts',(-3.83543398241206,-5.57838304940959,
25.6112876356437));
#189908=CARTESIAN_POINT('Ctrl Pts',(-3.67473949711305,-5.68230398943574,
25.6202761235025));
#189909=CARTESIAN_POINT('Ctrl Pts',(-3.53375220255945,-5.77348031172516,
25.6281622845178));
#189910=CARTESIAN_POINT('Ctrl Pts',(-3.38927578092314,-5.85946831997876,
25.6360484455331));
#189911=CARTESIAN_POINT('Ctrl Pts',(-3.24168590658374,-5.94001359283431,
25.6439346065484));
#189912=CARTESIAN_POINT('Ctrl Pts',(-3.08969230979447,-6.02296214049372,
25.6520560714046));
#189913=CARTESIAN_POINT('Ctrl Pts',(-2.93446394824125,-6.10009974434972,
25.6601775362608));
#189914=CARTESIAN_POINT('Ctrl Pts',(-2.77649212342414,-6.1711733477973,
25.6682990011169));
#189915=CARTESIAN_POINT('Ctrl Pts',(-2.61853156432294,-6.242241882651,25.6764198867931));
#189916=CARTESIAN_POINT('Ctrl Pts',(-2.45782826560801,-6.30724712823443,
25.6845407724693));
#189917=CARTESIAN_POINT('Ctrl Pts',(-2.29489524638042,-6.36598341249336,
25.6926616581456));
#189918=CARTESIAN_POINT('Ctrl Pts',(-2.13194275199779,-6.42472671741788,
25.7007835144998));
#189919=CARTESIAN_POINT('Ctrl Pts',(-1.96676035129669,-6.47719944589699,
25.7089053708541));
#189920=CARTESIAN_POINT('Ctrl Pts',(-1.79987797499627,-6.52324522573875,
25.7170272272084));
#189921=CARTESIAN_POINT('Ctrl Pts',(-1.63287384337915,-6.56932460001169,
25.7251550091686));
#189922=CARTESIAN_POINT('Ctrl Pts',(-1.46416761234239,-6.60896756289479,
25.7332827911287));
#189923=CARTESIAN_POINT('Ctrl Pts',(-1.29430183206151,-6.64206833505364,
25.7414105730889));
#189924=CARTESIAN_POINT('Ctrl Pts',(-1.12436685477529,-6.67518259123678,
25.7495416660053));
#189925=CARTESIAN_POINT('Ctrl Pts',(-0.953271748300365,-6.70174928836536,
25.7576727589218));
#189926=CARTESIAN_POINT('Ctrl Pts',(-0.781565761050786,-6.72171436176465,
25.7658038518382));
#189927=CARTESIAN_POINT('Ctrl Pts',(-0.609672363892046,-6.74170122620717,
25.7739438195028));
#189928=CARTESIAN_POINT('Ctrl Pts',(-0.43716711888452,-6.75507204707863,
25.7820837871673));
#189929=CARTESIAN_POINT('Ctrl Pts',(-0.264601621089993,-6.76182482634063,
25.7902237548319));
#189930=CARTESIAN_POINT('Ctrl Pts',(-0.17510169268123,-6.76532710963732,
25.7944454940123));
#189931=CARTESIAN_POINT('Ctrl Pts',(-0.0855855316561024,-6.76705005699934,
25.7986672331927));
#189932=CARTESIAN_POINT('Ctrl Pts',(0.00387034878749698,-6.76699889318746,
25.8028889723731));
#189933=CARTESIAN_POINT('Ctrl Pts',(0.182712843762716,-6.76689660517995,
25.8113291818308));
#189934=CARTESIAN_POINT('Ctrl Pts',(0.361683813194869,-6.75970006616008,
25.8197693912884));
#189935=CARTESIAN_POINT('Ctrl Pts',(0.540196532682286,-6.74540411732893,
25.828209600746));
#189936=CARTESIAN_POINT('Ctrl Pts',(0.718574002337971,-6.73111899979696,
25.8366434154945));
#189937=CARTESIAN_POINT('Ctrl Pts',(0.896493582928289,-6.70974522136511,
25.8450772302431));
#189938=CARTESIAN_POINT('Ctrl Pts',(1.07336991193727,-6.68132966049033,
25.8535110449916));
#189939=CARTESIAN_POINT('Ctrl Pts',(1.25013942157147,-6.65293126037676,
25.8619397663802));
#189940=CARTESIAN_POINT('Ctrl Pts',(1.42586660726584,-6.61749960891584,
25.8703684877687));
#189941=CARTESIAN_POINT('Ctrl Pts',(1.59997218499026,-6.5751333071853,25.8787972091573));
#189942=CARTESIAN_POINT('Ctrl Pts',(1.77399935195162,-6.53278608568234,
25.887222134559));
#189943=CARTESIAN_POINT('Ctrl Pts',(1.94640604361477,-6.48351051976002,
25.8956470599607));
#189944=CARTESIAN_POINT('Ctrl Pts',(2.11662372216021,-6.42745618567631,
25.9040719853625));
#189945=CARTESIAN_POINT('Ctrl Pts',(2.28679085734594,-6.37141849601164,
25.9124944091202));
#189946=CARTESIAN_POINT('Ctrl Pts',(2.45476995922689,-6.30860615643662,
25.9209168328779));
#189947=CARTESIAN_POINT('Ctrl Pts',(2.62000781530578,-6.23921854463655,
25.9293392566357));
#189948=CARTESIAN_POINT('Ctrl Pts',(2.78524827010023,-6.16982984156919,
25.9377618128539));
#189949=CARTESIAN_POINT('Ctrl Pts',(2.94774708298164,-6.09386578261243,
25.9461843690721));
#189950=CARTESIAN_POINT('Ctrl Pts',(3.10697056506046,-6.01157407904518,
25.9546069252903));
#189951=CARTESIAN_POINT('Ctrl Pts',(3.26619942573861,-5.92927959564863,
25.963029766024));
#189952=CARTESIAN_POINT('Ctrl Pts',(3.42215243858913,-5.84065719445277,
25.9714526067578));
#189953=CARTESIAN_POINT('Ctrl Pts',(3.57431995727228,-5.74600085651274,
25.9798754474915));
#189954=CARTESIAN_POINT('Ctrl Pts',(3.72651386047188,-5.65132810599184,
25.9882997486721));
#189955=CARTESIAN_POINT('Ctrl Pts',(3.87492067766104,-5.55061950903333,
25.9967240498528));
#189956=CARTESIAN_POINT('Ctrl Pts',(4.0190589170397,-5.4442129294659,26.0051483510334));
#189957=CARTESIAN_POINT('Ctrl Pts',(4.16324227818725,-5.33777303984063,
26.0135752894002));
#189958=CARTESIAN_POINT('Ctrl Pts',(4.30315412913592,-5.22563180937416,
26.022002227767));
#189959=CARTESIAN_POINT('Ctrl Pts',(4.4383450043898,-5.10816822569579,26.0304291661338));
#189960=CARTESIAN_POINT('Ctrl Pts',(4.57365743323396,-4.99059902749059,
26.0388636813775));
#189961=CARTESIAN_POINT('Ctrl Pts',(4.70424015266259,-4.86769813294548,
26.0472981966211));
#189962=CARTESIAN_POINT('Ctrl Pts',(4.82967877549317,-4.73988311306838,
26.0557327118648));
#189963=CARTESIAN_POINT('Ctrl Pts',(4.9551779862531,-4.6120063574418,26.0641713010516));
#189964=CARTESIAN_POINT('Ctrl Pts',(5.07552791741531,-4.47921098625575,
26.0726098902383));
#189965=CARTESIAN_POINT('Ctrl Pts',(5.190353289939,-4.34194906990161,26.0810484794251));
#189966=CARTESIAN_POINT('Ctrl Pts',(5.30530701125062,-4.20453372577966,
26.0894965010454));
#189967=CARTESIAN_POINT('Ctrl Pts',(5.41472362707429,-4.06264212148597,
26.0979445226657));
#189968=CARTESIAN_POINT('Ctrl Pts',(5.51826941403206,-3.91675780131454,
26.106392544286));
#189969=CARTESIAN_POINT('Ctrl Pts',(5.57712317760059,-3.83383949493065,
26.1111942641982));
#189970=CARTESIAN_POINT('Ctrl Pts',(5.6340811061209,-3.7496318241605,26.1159959841105));
#189971=CARTESIAN_POINT('Ctrl Pts',(5.68908840787477,-3.66422735203274,
26.1207977040227));
#189972=CARTESIAN_POINT('Ctrl Pts',(5.78347842293469,-3.51767718226813,
26.1290372358735));
#189973=CARTESIAN_POINT('Ctrl Pts',(5.87233292907665,-3.36727442526352,
26.1372767677243));
#189974=CARTESIAN_POINT('Ctrl Pts',(5.95532333861317,-3.21347365518519,
26.1455162995752));
#189975=CARTESIAN_POINT('Ctrl Pts',(6.03822163459527,-3.05984359321258,
26.1537466861215));
#189976=CARTESIAN_POINT('Ctrl Pts',(6.1152686264389,-2.90282333842673,26.1619770726678));
#189977=CARTESIAN_POINT('Ctrl Pts',(6.1861786152737,-2.74289685185762,26.1702074592142));
#189978=CARTESIAN_POINT('Ctrl Pts',(6.257022548667,-2.58311934309613,26.178430178832));
#189979=CARTESIAN_POINT('Ctrl Pts',(6.32174072086143,-2.42044131756993,
26.1866528984498));
#189980=CARTESIAN_POINT('Ctrl Pts',(6.38009300521273,-2.25537186398067,
26.1948756180676));
#189981=CARTESIAN_POINT('Ctrl Pts',(6.43839358523597,-2.09044867382006,
26.2030910517634));
#189982=CARTESIAN_POINT('Ctrl Pts',(6.49033940156552,-1.92313861319645,
26.2113064854591));
#189983=CARTESIAN_POINT('Ctrl Pts',(6.53573822131611,-1.75397118061495,
26.2195219191549));
#189984=CARTESIAN_POINT('Ctrl Pts',(6.58111370959868,-1.58489068695753,
26.2277331307558));
#189985=CARTESIAN_POINT('Ctrl Pts',(6.61994881027167,-1.41395506530572,
26.2359443423566));
#189986=CARTESIAN_POINT('Ctrl Pts',(6.65210084986099,-1.24170982249427,
26.2441555539574));
#189987=CARTESIAN_POINT('Ctrl Pts',(6.68424210743033,-1.06952234123305,
26.2523640119709));
#189988=CARTESIAN_POINT('Ctrl Pts',(6.70970470320407,-0.896026463174697,
26.2605724699845));
#189989=CARTESIAN_POINT('Ctrl Pts',(6.72839685881742,-0.721778851349826,
26.268780927998));
#189990=CARTESIAN_POINT('Ctrl Pts',(6.73672462230109,-0.644147735448202,
26.2724379752812));
#189991=CARTESIAN_POINT('Ctrl Pts',(6.74370920349503,-0.566367531857892,
26.2760950225643));
#189992=CARTESIAN_POINT('Ctrl Pts',(6.74934578577647,-0.488487936413445,
26.2797520698475));
#189993=CARTESIAN_POINT('Ctrl Pts',(6.76300021697827,-0.299827233007562,
26.2886111440234));
#189994=CARTESIAN_POINT('Ctrl Pts',(6.76872665841279,-0.110779146266043,
26.2974702181993));
#189995=CARTESIAN_POINT('Ctrl Pts',(6.76655041107128,0.0780034257655365,
26.3063292923751));
#189996=CARTESIAN_POINT('Ctrl Pts',(6.76437007499884,0.267140682269253,
26.3152050109691));
#189997=CARTESIAN_POINT('Ctrl Pts',(6.75425738114367,0.456011167927298,
26.324080729563));
#189998=CARTESIAN_POINT('Ctrl Pts',(6.73628951813857,0.643966247420222,
26.3329564481569));
#189999=CARTESIAN_POINT('Ctrl Pts',(6.7182703799292,0.832457697604004,26.3418574955439));
#190000=CARTESIAN_POINT('Ctrl Pts',(6.69235123899935,1.02002825434488,26.3507585429309));
#190001=CARTESIAN_POINT('Ctrl Pts',(6.65866106849444,1.20603556121554,26.3596595903179));
#190002=CARTESIAN_POINT('Ctrl Pts',(6.62492509574062,1.39229574757126,26.3685727388009));
#190003=CARTESIAN_POINT('Ctrl Pts',(6.58339704213217,1.57698818484015,26.3774858872839));
#190004=CARTESIAN_POINT('Ctrl Pts',(6.53425640339181,1.75948351931275,26.3863990357669));
#190005=CARTESIAN_POINT('Ctrl Pts',(6.48500665899625,1.94238404333004,26.3953319738767));
#190006=CARTESIAN_POINT('Ctrl Pts',(6.42811059001266,2.1230774559697,26.4042649119866));
#190007=CARTESIAN_POINT('Ctrl Pts',(6.36379762001419,2.30094955431485,26.4131978500965));
#190008=CARTESIAN_POINT('Ctrl Pts',(6.30258099756759,2.47025800156024,26.4217007119551));
#190009=CARTESIAN_POINT('Ctrl Pts',(6.2346449015172,2.63701023195201,26.4302035738136));
#190010=CARTESIAN_POINT('Ctrl Pts',(6.16022666131992,2.800695713776,26.4387064356722));
#190011=CARTESIAN_POINT('Ctrl Pts',(6.08824396200822,2.95902413955698,26.4469310180707));
#190012=CARTESIAN_POINT('Ctrl Pts',(6.01005756673814,3.11478638128748,26.4551556004692));
#190013=CARTESIAN_POINT('Ctrl Pts',(5.92587328937933,3.26746304619051,26.4633801828677));
#190014=CARTESIAN_POINT('Ctrl Pts',(5.84180558029627,3.41992830278628,26.4715933768524));
#190015=CARTESIAN_POINT('Ctrl Pts',(5.75175671396695,3.5693161863398,26.479806570837));
#190016=CARTESIAN_POINT('Ctrl Pts',(5.65598008519765,3.7151282987062,26.4880197648217));
#190017=CARTESIAN_POINT('Ctrl Pts',(5.5602806087334,3.86082295297537,26.4962263427158));
#190018=CARTESIAN_POINT('Ctrl Pts',(5.45886275229027,4.00294727321016,26.50443292061));
#190019=CARTESIAN_POINT('Ctrl Pts',(5.35202556453078,4.1410278140347,26.5126394985041));
#190020=CARTESIAN_POINT('Ctrl Pts',(5.24525500932461,4.2790222363532,26.5208409580939));
#190021=CARTESIAN_POINT('Ctrl Pts',(5.13307207247803,4.41297761911667,26.5290424176837));
#190022=CARTESIAN_POINT('Ctrl Pts',(5.01581884608409,4.5424498129608,26.5372438772736));
#190023=CARTESIAN_POINT('Ctrl Pts',(4.8986174267608,4.6718648009156,26.5454417131371));
#190024=CARTESIAN_POINT('Ctrl Pts',(4.7763504207168,4.79680028042478,26.5536395490006));
#190025=CARTESIAN_POINT('Ctrl Pts',(4.64939993165243,4.91684545979945,26.5618373848642));
#190026=CARTESIAN_POINT('Ctrl Pts',(4.52246573338793,5.03687523449148,26.5700341687483));
#190027=CARTESIAN_POINT('Ctrl Pts',(4.39084950547198,5.15201570834916,26.5782309526324));
#190028=CARTESIAN_POINT('Ctrl Pts',(4.25497010847688,5.26189304109921,26.5864277365165));
#190029=CARTESIAN_POINT('Ctrl Pts',(4.11910289066643,5.37176052528977,26.594623785704));
#190030=CARTESIAN_POINT('Ctrl Pts',(3.97897354623155,5.47636558551816,26.6028198348914));
#190031=CARTESIAN_POINT('Ctrl Pts',(3.83503374755571,5.57537488919883,26.6110158840788));
#190032=CARTESIAN_POINT('Ctrl Pts',(3.69104291756391,5.67441929488119,26.6192148390308));
#190033=CARTESIAN_POINT('Ctrl Pts',(3.5432392309082,5.76786377837212,26.6274137939829));
#190034=CARTESIAN_POINT('Ctrl Pts',(3.39210345244099,5.85541827437955,26.6356127489349));
#190035=CARTESIAN_POINT('Ctrl Pts',(3.29574823599213,5.91123783278872,26.6408399167642));
#190036=CARTESIAN_POINT('Ctrl Pts',(3.19803922663916,5.96466424644638,26.6460670845935));
#190037=CARTESIAN_POINT('Ctrl Pts',(3.0991061983213,6.01563211736942,26.6512942524228));
#190038=CARTESIAN_POINT('Origin',(0.,0.,4.30282021618968));
#190039=CARTESIAN_POINT('',(3.09910619832132,6.01563211736941,29.0458282148631));
#190040=CARTESIAN_POINT('',(3.09910619832131,6.01563211736942,28.6513936431573));
#190041=CARTESIAN_POINT('',(3.09910619832133,6.0156321173694,4.30282021618968));
#190042=CARTESIAN_POINT('',(-6.76699906337236,0.00356038167509778,27.6971797838411));
#190043=CARTESIAN_POINT('Ctrl Pts',(-6.76699906337236,0.00356038167514286,
27.6971797838411));
#190044=CARTESIAN_POINT('Ctrl Pts',(-6.76708950334129,-0.168333319875732,
27.7052996038289));
#190045=CARTESIAN_POINT('Ctrl Pts',(-6.76062617083703,-0.340485372879538,
27.7134194238167));
#190046=CARTESIAN_POINT('Ctrl Pts',(-6.7475763930807,-0.512349313984179,
27.7215392438044));
#190047=CARTESIAN_POINT('Ctrl Pts',(-6.73453996609472,-0.684037427112826,
27.7296507566889));
#190048=CARTESIAN_POINT('Ctrl Pts',(-6.71493053232619,-0.85543765128416,
27.7377622695734));
#190049=CARTESIAN_POINT('Ctrl Pts',(-6.68876740218731,-1.02600177360295,
27.7458737824578));
#190050=CARTESIAN_POINT('Ctrl Pts',(-6.66222459940465,-1.19904107878064,
27.7541030075398));
#190051=CARTESIAN_POINT('Ctrl Pts',(-6.62893638057383,-1.3712194460363,
27.7623322326217));
#190052=CARTESIAN_POINT('Ctrl Pts',(-6.58897774974783,-1.54196667062814,
27.7705614577036));
#190053=CARTESIAN_POINT('Ctrl Pts',(-6.54965160517701,-1.71001121821551,
27.7786604262766));
#190054=CARTESIAN_POINT('Ctrl Pts',(-6.50386472768852,-1.87666921735391,
27.7867593948496));
#190055=CARTESIAN_POINT('Ctrl Pts',(-6.45174049729151,-2.04140479954581,
27.7948583634225));
#190056=CARTESIAN_POINT('Ctrl Pts',(-6.39835878820009,-2.21011456962003,
27.8031527167589));
#190057=CARTESIAN_POINT('Ctrl Pts',(-6.33833014407865,-2.37680760350063,
27.8114470700954));
#190058=CARTESIAN_POINT('Ctrl Pts',(-6.27184195620629,-2.54092256402482,
27.8197414234318));
#190059=CARTESIAN_POINT('Ctrl Pts',(-6.20535376833395,-2.70503752454898,
27.8280357767682));
#190060=CARTESIAN_POINT('Ctrl Pts',(-6.13240618107729,-2.86657402209651,
27.8363301301047));
#190061=CARTESIAN_POINT('Ctrl Pts',(-6.05324029813116,-3.02499105669438,
27.8446244834411));
#190062=CARTESIAN_POINT('Ctrl Pts',(-5.96868440802465,-3.19419391113072,
27.853483557617));
#190063=CARTESIAN_POINT('Ctrl Pts',(-5.87711334375679,-3.35968322021457,
27.8623426317929));
#190064=CARTESIAN_POINT('Ctrl Pts',(-5.77888211931975,-3.52091045768087,
27.8712017059688));
#190065=CARTESIAN_POINT('Ctrl Pts',(-5.68046633817515,-3.68244060868903,
27.8800774245627));
#190066=CARTESIAN_POINT('Ctrl Pts',(-5.57536552503268,-3.83969246402432,
27.8889531431566));
#190067=CARTESIAN_POINT('Ctrl Pts',(-5.4639771373322,-3.99214764790972,
27.8978288617505));
#190068=CARTESIAN_POINT('Ctrl Pts',(-5.35227087864533,-4.14503789581464,
27.9067299091375));
#190069=CARTESIAN_POINT('Ctrl Pts',(-5.23424129293976,-4.29310386935633,
27.9156309565245));
#190070=CARTESIAN_POINT('Ctrl Pts',(-5.11032716331366,-4.43585902434901,
27.9245320039115));
#190071=CARTESIAN_POINT('Ctrl Pts',(-4.98624457072872,-4.57880825693295,
27.9334451523945));
#190072=CARTESIAN_POINT('Ctrl Pts',(-4.85626162831484,-4.71643205684519,
27.9423583008775));
#190073=CARTESIAN_POINT('Ctrl Pts',(-4.72085392763827,-4.84828084932198,
27.9512714493605));
#190074=CARTESIAN_POINT('Ctrl Pts',(-4.58514558483985,-4.98042238217127,
27.9602043874704));
#190075=CARTESIAN_POINT('Ctrl Pts',(-4.44398857917533,-5.10676307945052,
27.9691373255803));
#190076=CARTESIAN_POINT('Ctrl Pts',(-4.29789370282457,-5.2268918794271,
27.9780702636902));
#190077=CARTESIAN_POINT('Ctrl Pts',(-4.15883256341283,-5.34123707905477,
27.9865731255487));
#190078=CARTESIAN_POINT('Ctrl Pts',(-4.01529797259374,-5.44995433033329,
27.9950759874073));
#190079=CARTESIAN_POINT('Ctrl Pts',(-3.86775460434358,-5.55272575593096,
28.0035788492659));
#190080=CARTESIAN_POINT('Ctrl Pts',(-3.72507224685697,-5.65211124143562,
28.0118015731317));
#190081=CARTESIAN_POINT('Ctrl Pts',(-3.57836687347787,-5.74612590434581,
28.0200242969976));
#190082=CARTESIAN_POINT('Ctrl Pts',(-3.42808027674972,-5.83442838812506,
28.0282470208635));
#190083=CARTESIAN_POINT('Ctrl Pts',(-3.27795275329339,-5.92263740671639,
28.0364610412547));
#190084=CARTESIAN_POINT('Ctrl Pts',(-3.12425186151364,-6.00514610578454,
28.0446750616459));
#190085=CARTESIAN_POINT('Ctrl Pts',(-2.96745003429532,-6.0816551442811,
28.0528890820371));
#190086=CARTESIAN_POINT('Ctrl Pts',(-2.8107826951253,-6.15809856140418,
28.0610960573091));
#190087=CARTESIAN_POINT('Ctrl Pts',(-2.65102003801491,-6.22855240999417,
28.069303032581));
#190088=CARTESIAN_POINT('Ctrl Pts',(-2.48866095055195,-6.29276216563107,
28.077510007853));
#190089=CARTESIAN_POINT('Ctrl Pts',(-2.32640852976953,-6.35692973673985,
28.085711591306));
#190090=CARTESIAN_POINT('Ctrl Pts',(-2.16156340877717,-6.41486125462091,
28.0939131747589));
#190091=CARTESIAN_POINT('Ctrl Pts',(-1.99464648789654,-6.46634938650256,
28.1021147582119));
#190092=CARTESIAN_POINT('Ctrl Pts',(-1.82780573233528,-6.51781402400156,
28.1103125992269));
#190093=CARTESIAN_POINT('Ctrl Pts',(-1.65889540238528,-6.56284102749984,
28.1185104402419));
#190094=CARTESIAN_POINT('Ctrl Pts',(-1.48845375639599,-6.60127218156248,
28.1267082812569));
#190095=CARTESIAN_POINT('Ctrl Pts',(-1.31802715134927,-6.63969994419589,
28.1349053988381));
#190096=CARTESIAN_POINT('Ctrl Pts',(-1.14606984721851,-6.67153292957121,
28.1431025164193));
#190097=CARTESIAN_POINT('Ctrl Pts',(-0.973132916139615,-6.69666344738375,
28.1512996340004));
#190098=CARTESIAN_POINT('Ctrl Pts',(-0.800197909176538,-6.72179368559131,
28.1594966603795));
#190099=CARTESIAN_POINT('Ctrl Pts',(-0.626283651922684,-6.74022155210216,
28.1676936867586));
#190100=CARTESIAN_POINT('Ctrl Pts',(-0.451948888939349,-6.75189093527039,
28.1758907131377));
#190101=CARTESIAN_POINT('Ctrl Pts',(-0.27758436627546,-6.76356231045164,
28.1840891387838));
#190102=CARTESIAN_POINT('Ctrl Pts',(-0.102799552912786,-6.76847287980788,
28.19228756443));
#190103=CARTESIAN_POINT('Ctrl Pts',(0.0718441828962487,-6.76661861001372,
28.2004859900761));
#190104=CARTESIAN_POINT('Ctrl Pts',(0.24654948700103,-6.76476368652173,
28.2086873059667));
#190105=CARTESIAN_POINT('Ctrl Pts',(0.421113255886029,-6.75613917703564,
28.2168886218574));
#190106=CARTESIAN_POINT('Ctrl Pts',(0.59497657081346,-6.74079311952111,
28.225089937748));
#190107=CARTESIAN_POINT('Ctrl Pts',(0.769037886953337,-6.72542958541586,
28.2333005935646));
#190108=CARTESIAN_POINT('Ctrl Pts',(0.942396797659656,-6.70332924210075,
28.2415112493812));
#190109=CARTESIAN_POINT('Ctrl Pts',(1.11450088340976,-6.67459188122232,
28.2497219051978));
#190110=CARTESIAN_POINT('Ctrl Pts',(1.28670638592829,-6.6458375861133,28.2579373993549));
#190111=CARTESIAN_POINT('Ctrl Pts',(1.45765523873773,-6.6104385500377,28.2661528935121));
#190112=CARTESIAN_POINT('Ctrl Pts',(1.62680772441081,-6.56854516828478,
28.2743683876692));
#190113=CARTESIAN_POINT('Ctrl Pts',(1.79622265327796,-6.5265867881792,28.2825966283167));
#190114=CARTESIAN_POINT('Ctrl Pts',(1.96383530081299,-6.47811402600845,
28.2908248689642));
#190115=CARTESIAN_POINT('Ctrl Pts',(2.12912227518776,-6.42332681227565,
28.2990531096118));
#190116=CARTESIAN_POINT('Ctrl Pts',(2.27934174665302,-6.37353398182954,
28.306531266713));
#190117=CARTESIAN_POINT('Ctrl Pts',(2.42764029131424,-6.31852615803697,
28.3140094238142));
#190118=CARTESIAN_POINT('Ctrl Pts',(2.57364188029135,-6.25848675575897,
28.3214875809154));
#190119=CARTESIAN_POINT('Ctrl Pts',(2.73118496911533,-6.19370120820232,
28.3295568901379));
#190120=CARTESIAN_POINT('Ctrl Pts',(2.88656897566729,-6.12284426780645,
28.3376261993604));
#190121=CARTESIAN_POINT('Ctrl Pts',(3.03927934623883,-6.04607889921444,
28.3456955085829));
#190122=CARTESIAN_POINT('Ctrl Pts',(3.19179924547299,-5.96940927790119,
28.3537547531837));
#190123=CARTESIAN_POINT('Ctrl Pts',(3.34165181482521,-5.8868460570315,28.3618139977845));
#190124=CARTESIAN_POINT('Ctrl Pts',(3.4883393221044,-5.79860136359279,28.3698732423852));
#190125=CARTESIAN_POINT('Ctrl Pts',(3.634876060526,-5.71044737011802,28.3779242035055));
#190126=CARTESIAN_POINT('Ctrl Pts',(3.77825389361887,-5.61662371561286,
28.3859751646258));
#190127=CARTESIAN_POINT('Ctrl Pts',(3.91799678858754,-5.5173897963274,28.3940261257461));
#190128=CARTESIAN_POINT('Ctrl Pts',(4.05762667297448,-5.41823612786935,
28.4020705760252));
#190129=CARTESIAN_POINT('Ctrl Pts',(4.19362716730172,-5.31368111786948,
28.4101150263042));
#190130=CARTESIAN_POINT('Ctrl Pts',(4.32554859867539,-5.20402904685373,
28.4181594765833));
#190131=CARTESIAN_POINT('Ctrl Pts',(4.45739222108193,-5.09444165004824,
28.4261991821415));
#190132=CARTESIAN_POINT('Ctrl Pts',(4.58516128370464,-4.97976341480909,
28.4342388876997));
#190133=CARTESIAN_POINT('Ctrl Pts',(4.70843686644385,-4.86034065418386,
28.4422785932579));
#190134=CARTESIAN_POINT('Ctrl Pts',(4.83437328673022,-4.73834021711699,
28.4504918315624));
#190135=CARTESIAN_POINT('Ctrl Pts',(4.95561971810547,-4.61138834123703,
28.4587050698669));
#190136=CARTESIAN_POINT('Ctrl Pts',(5.07176663562319,-4.47989644900185,
28.4669183081713));
#190137=CARTESIAN_POINT('Ctrl Pts',(5.18542295415974,-4.35122420605082,
28.4749554257195));
#190138=CARTESIAN_POINT('Ctrl Pts',(5.29419599707397,-4.21820498034962,
28.4829925432677));
#190139=CARTESIAN_POINT('Ctrl Pts',(5.3977409055983,-4.08125986872079,28.4910296608158));
#190140=CARTESIAN_POINT('Ctrl Pts',(5.50129676851557,-3.94430026916991,
28.4990676286399));
#190141=CARTESIAN_POINT('Ctrl Pts',(5.59962317029237,-3.80341425466986,
28.5071055964641));
#190142=CARTESIAN_POINT('Ctrl Pts',(5.69241719540748,-3.6590539041437,28.5151435642882));
#190143=CARTESIAN_POINT('Ctrl Pts',(5.78523942345759,-3.51464967810317,
28.5231839750959));
#190144=CARTESIAN_POINT('Ctrl Pts',(5.87252572601679,-3.36676932827826,
28.5312243859036));
#190145=CARTESIAN_POINT('Ctrl Pts',(5.95401803739081,-3.21589151098493,
28.5392647967114));
#190146=CARTESIAN_POINT('Ctrl Pts',(6.03859029851253,-3.05931136315917,
28.5476090896992));
#190147=CARTESIAN_POINT('Ctrl Pts',(6.11692183960478,-2.89950313826752,
28.555953382687));
#190148=CARTESIAN_POINT('Ctrl Pts',(6.18877843488688,-2.73702584640319,
28.5642976756748));
#190149=CARTESIAN_POINT('Ctrl Pts',(6.25814043682762,-2.58018916092742,
28.5723522858903));
#190150=CARTESIAN_POINT('Ctrl Pts',(6.32146945744517,-2.42086598918543,
28.5804068961058));
#190151=CARTESIAN_POINT('Ctrl Pts',(6.37860554822771,-2.25957523887096,
28.5884615063214));
#190152=CARTESIAN_POINT('Ctrl Pts',(6.43578489183809,-2.09816238918004,
28.5965222139907));
#190153=CARTESIAN_POINT('Ctrl Pts',(6.4867618604932,-1.93477934931919,28.6045829216599));
#190154=CARTESIAN_POINT('Ctrl Pts',(6.53142732344164,-1.76995653014417,
28.6126436293292));
#190155=CARTESIAN_POINT('Ctrl Pts',(6.57615576201672,-1.6049013206694,28.6207157021133));
#190156=CARTESIAN_POINT('Ctrl Pts',(6.61455485703562,-1.43840264222174,
28.6287877748974));
#190157=CARTESIAN_POINT('Ctrl Pts',(6.64656702892482,-1.27099792683131,
28.6368598476815));
#190158=CARTESIAN_POINT('Ctrl Pts',(6.64992006070939,-1.25346355479516,
28.637705335976));
#190159=CARTESIAN_POINT('Ctrl Pts',(6.65320306885883,-1.23591924395092,
28.6385508242705));
#190160=CARTESIAN_POINT('Ctrl Pts',(6.65641602025913,-1.21836561230103,
28.6393963125649));
#190161=CARTESIAN_POINT('Ctrl Pts',(6.68808206901938,-1.04536139079481,
28.6477292346116));
#190162=CARTESIAN_POINT('Ctrl Pts',(6.71303982097927,-0.870899705245018,
28.6560621566584));
#190163=CARTESIAN_POINT('Ctrl Pts',(6.73116032192443,-0.695535563828484,
28.6643950787051));
#190164=CARTESIAN_POINT('Ctrl Pts',(6.74925940883177,-0.520378660300522,
28.6727181532587));
#190165=CARTESIAN_POINT('Ctrl Pts',(6.7605373052033,-0.344321768575867,
28.6810412278123));
#190166=CARTESIAN_POINT('Ctrl Pts',(6.76491599548732,-0.167930265288237,
28.6893643023659));
#190167=CARTESIAN_POINT('Ctrl Pts',(6.76929031495499,0.00828516369006133,
28.6976790688119));
#190168=CARTESIAN_POINT('Ctrl Pts',(6.76677914047182,0.184834193098326,
28.7059938352578));
#190169=CARTESIAN_POINT('Ctrl Pts',(6.75735618633986,0.361145913633897,
28.7143086017038));
#190170=CARTESIAN_POINT('Ctrl Pts',(6.74794090973028,0.537313981005039,
28.7226165935433));
#190171=CARTESIAN_POINT('Ctrl Pts',(6.73162509318644,0.713244778819943,
28.7309245853828));
#190172=CARTESIAN_POINT('Ctrl Pts',(6.70843450512467,0.888366754472935,
28.7392325772224));
#190173=CARTESIAN_POINT('Ctrl Pts',(6.68525856039957,1.06337815207409,28.7475353231095));
#190174=CARTESIAN_POINT('Ctrl Pts',(6.65521654073805,1.23758140135111,28.7558380689966));
#190175=CARTESIAN_POINT('Ctrl Pts',(6.61838612327401,1.41040920418651,28.7641408148837));
#190176=CARTESIAN_POINT('Ctrl Pts',(6.58157075722798,1.58316637780612,28.7724401677032));
#190177=CARTESIAN_POINT('Ctrl Pts',(6.53797259358396,1.75454888526294,28.7807395205226));
#190178=CARTESIAN_POINT('Ctrl Pts',(6.48772062103169,1.9239984780244,28.789038873342));
#190179=CARTESIAN_POINT('Ctrl Pts',(6.43747933623078,2.09341203170075,28.7973364610284));
#190180=CARTESIAN_POINT('Ctrl Pts',(6.38058716068607,2.26089315632913,28.8056340487147));
#190181=CARTESIAN_POINT('Ctrl Pts',(6.3172233400068,2.42589741590062,28.8139316364011));
#190182=CARTESIAN_POINT('Ctrl Pts',(6.25386246625003,2.59089400145942,28.8222288381835));
#190183=CARTESIAN_POINT('Ctrl Pts',(6.18403067200167,2.75341362681236,28.8305260399659));
#190184=CARTESIAN_POINT('Ctrl Pts',(6.10795593739177,2.91293035736879,28.8388232417483));
#190185=CARTESIAN_POINT('Ctrl Pts',(6.03187209968865,3.07246617567722,28.8471214363729));
#190186=CARTESIAN_POINT('Ctrl Pts',(5.94954398337093,3.2289980694472,28.8554196309974));
#190187=CARTESIAN_POINT('Ctrl Pts',(5.86124633355747,3.38202312490012,28.863717825622));
#190188=CARTESIAN_POINT('Ctrl Pts',(5.77288658297748,3.53515580465857,28.8720218564635));
#190189=CARTESIAN_POINT('Ctrl Pts',(5.67854908367685,3.68477641604058,28.8803258873051));
#190190=CARTESIAN_POINT('Ctrl Pts',(5.57855335644909,3.83040878357006,28.8886299181467));
#190191=CARTESIAN_POINT('Ctrl Pts',(5.47852126802292,3.97609410703631,28.8969369685624));
#190192=CARTESIAN_POINT('Ctrl Pts',(5.3728270538298,4.11778801356652,28.9052440189781));
#190193=CARTESIAN_POINT('Ctrl Pts',(5.26183176885043,4.25504587946081,28.9135510693938));
#190194=CARTESIAN_POINT('Ctrl Pts',(5.15071781117833,4.39245049717925,28.9218670014484));
#190195=CARTESIAN_POINT('Ctrl Pts',(5.0342916831421,4.52540933192618,28.9301829335031));
#190196=CARTESIAN_POINT('Ctrl Pts',(4.91295341747405,4.65351240653015,28.9384988655577));
#190197=CARTESIAN_POINT('Ctrl Pts',(4.82148605550475,4.75007922516458,28.9447675917766));
#190198=CARTESIAN_POINT('Ctrl Pts',(4.72722819245259,4.84388749541669,28.9510363179955));
#190199=CARTESIAN_POINT('Ctrl Pts',(4.63036404117561,4.93477637245984,28.9573050442145));
#190200=CARTESIAN_POINT('Ctrl Pts',(4.49979797673741,5.05728818741187,28.965754846341));
#190201=CARTESIAN_POINT('Ctrl Pts',(4.36425593395156,5.1747189922691,28.9742046484675));
#190202=CARTESIAN_POINT('Ctrl Pts',(4.22415975134858,5.28665900121114,28.9826544505941));
#190203=CARTESIAN_POINT('Ctrl Pts',(4.08417659437682,5.39850870012521,28.9910974356596));
#190204=CARTESIAN_POINT('Ctrl Pts',(3.93964687644033,5.50487622392519,28.9995404207252));
#190205=CARTESIAN_POINT('Ctrl Pts',(3.79102756981362,5.60539017062265,29.0079834057908));
#190206=CARTESIAN_POINT('Ctrl Pts',(3.6425351055428,5.70581833152224,29.0164191850084));
#190207=CARTESIAN_POINT('Ctrl Pts',(3.48996028683844,5.8004026930279,29.0248549642261));
#190208=CARTESIAN_POINT('Ctrl Pts',(3.33379134897792,5.88881348333261,29.0332907434438));
#190209=CARTESIAN_POINT('Ctrl Pts',(3.25642392211295,5.93261294465112,29.0374699005836));
#190210=CARTESIAN_POINT('Ctrl Pts',(3.17817486874918,5.974897876672,29.0416490577234));
#190211=CARTESIAN_POINT('Ctrl Pts',(3.09910619832131,6.01563211736941,29.0458282148631));
#190212=CARTESIAN_POINT('Ctrl Pts',(3.09910619832137,6.01563211736939,27.0457199708935));
#190213=CARTESIAN_POINT('Ctrl Pts',(3.07316115263563,6.02899836888404,27.0470975320348));
#190214=CARTESIAN_POINT('Ctrl Pts',(3.04713223696845,6.04219542789079,27.048475093176));
#190215=CARTESIAN_POINT('Ctrl Pts',(3.0210217104256,6.05522227710405,27.0498526543173));
#190216=CARTESIAN_POINT('Ctrl Pts',(2.84958893181414,6.14075210943112,27.0588972491771));
#190217=CARTESIAN_POINT('Ctrl Pts',(2.67447812095438,6.21901965298881,27.067941844037));
#190218=CARTESIAN_POINT('Ctrl Pts',(2.49629646023971,6.28973711553946,27.0769864388968));
#190219=CARTESIAN_POINT('Ctrl Pts',(2.31827830924617,6.36038968368666,27.0860227339171));
#190220=CARTESIAN_POINT('Ctrl Pts',(2.13719515544994,6.42350591570578,27.0950590289375));
#190221=CARTESIAN_POINT('Ctrl Pts',(1.95367442427087,6.47884598087884,27.1040953239578));
#190222=CARTESIAN_POINT('Ctrl Pts',(1.77047844741676,6.53408811746698,27.1131156285455));
#190223=CARTESIAN_POINT('Ctrl Pts',(1.58485373412527,6.58158149665532,27.1221359331332));
#190224=CARTESIAN_POINT('Ctrl Pts',(1.39744296704592,6.62113601686704,27.1311562377209));
#190225=CARTESIAN_POINT('Ctrl Pts',(1.2102682074221,6.66064072584424,27.1401651829873));
#190226=CARTESIAN_POINT('Ctrl Pts',(1.02131211468574,6.69222647833871,27.1491741282536));
#190227=CARTESIAN_POINT('Ctrl Pts',(0.831230156072832,6.71575352642093,
27.1581830735199));
#190228=CARTESIAN_POINT('Ctrl Pts',(0.641579833347911,6.73922714955759,
27.1671715613787));
#190229=CARTESIAN_POINT('Ctrl Pts',(0.450808983602992,6.75467856671836,
27.1761600492375));
#190230=CARTESIAN_POINT('Ctrl Pts',(0.259580348682078,6.76201945002956,
27.1851485370963));
#190231=CARTESIAN_POINT('Ctrl Pts',(0.0918035402349528,6.76846006481325,
27.1930346981116));
#190232=CARTESIAN_POINT('Ctrl Pts',(-0.0763253826688315,6.76865819405494,
27.2009208591268));
#190233=CARTESIAN_POINT('Ctrl Pts',(-0.244353506158314,6.76258681009184,
27.2088070201421));
#190234=CARTESIAN_POINT('Ctrl Pts',(-0.417395179683282,6.75633427081586,
27.2169284849983));
#190235=CARTESIAN_POINT('Ctrl Pts',(-0.590252428843142,6.74343366726387,
27.2250499498544));
#190236=CARTESIAN_POINT('Ctrl Pts',(-0.762373606214561,6.72391816462302,
27.2331714147106));
#190237=CARTESIAN_POINT('Ctrl Pts',(-0.934482508813035,6.70440405372471,
27.2412923003868));
#190238=CARTESIAN_POINT('Ctrl Pts',(-1.10585508032576,6.67827602463097,
27.249413186063));
#190239=CARTESIAN_POINT('Ctrl Pts',(-1.27594518429308,6.64561907474987,
27.2575340717392));
#190240=CARTESIAN_POINT('Ctrl Pts',(-1.44605561889158,6.61295822142942,
27.2656559280935));
#190241=CARTESIAN_POINT('Ctrl Pts',(-1.61488292132075,6.57376696360522,
27.2737777844478));
#190242=CARTESIAN_POINT('Ctrl Pts',(-1.78189157647687,6.52818132481634,
27.281899640802));
#190243=CARTESIAN_POINT('Ctrl Pts',(-1.94902207908151,6.48256242730939,
27.2900274227622));
#190244=CARTESIAN_POINT('Ctrl Pts',(-2.11433093068078,6.43053992756398,
27.2981552047224));
#190245=CARTESIAN_POINT('Ctrl Pts',(-2.27729758842626,6.37229979628611,
27.3062829866826));
#190246=CARTESIAN_POINT('Ctrl Pts',(-2.44033063273094,6.31403594014343,
27.314414079599));
#190247=CARTESIAN_POINT('Ctrl Pts',(-2.60101924174457,6.24954954010989,
27.3225451725155));
#190248=CARTESIAN_POINT('Ctrl Pts',(-2.75886350925092,6.17907445636672,
27.3306762654319));
#190249=CARTESIAN_POINT('Ctrl Pts',(-2.91688005717841,6.10852245201504,
27.3388162330965));
#190250=CARTESIAN_POINT('Ctrl Pts',(-3.07204573492137,6.03196887041107,
27.346956200761));
#190251=CARTESIAN_POINT('Ctrl Pts',(-3.22388519457764,5.94969354271152,
27.3550961684256));
#190252=CARTESIAN_POINT('Ctrl Pts',(-3.30263570347203,5.9070220004098,27.359317907606));
#190253=CARTESIAN_POINT('Ctrl Pts',(-3.38049194906336,5.86281208461277,
27.3635396467864));
#190254=CARTESIAN_POINT('Ctrl Pts',(-3.45739080292563,5.81710734264422,
27.3677613859669));
#190255=CARTESIAN_POINT('Ctrl Pts',(-3.61112896767471,5.72573324800347,
27.3762015954245));
#190256=CARTESIAN_POINT('Ctrl Pts',(-3.76135650917294,5.62819308269307,
27.3846418048821));
#190257=CARTESIAN_POINT('Ctrl Pts',(-3.90756625773005,5.52478189084869,
27.3930820143397));
#190258=CARTESIAN_POINT('Ctrl Pts',(-4.05366523074137,5.42144904830269,
27.4015158290883));
#190259=CARTESIAN_POINT('Ctrl Pts',(-4.19575220767966,5.31225423823208,
27.4099496438368));
#190260=CARTESIAN_POINT('Ctrl Pts',(-4.33334775121705,5.19753655754552,
27.4183834585853));
#190261=CARTESIAN_POINT('Ctrl Pts',(-4.47086019788112,5.08288815730464,
27.4268121799739));
#190262=CARTESIAN_POINT('Ctrl Pts',(-4.60388636334862,4.96272374902026,
27.4352409013624));
#190263=CARTESIAN_POINT('Ctrl Pts',(-4.73197843795805,4.83742380433016,
27.443669622751));
#190264=CARTESIAN_POINT('Ctrl Pts',(-4.86001282459775,4.71218029013694,
27.4520945481527));
#190265=CARTESIAN_POINT('Ctrl Pts',(-4.98311731306697,4.58180608392272,
27.4605194735544));
#190266=CARTESIAN_POINT('Ctrl Pts',(-5.1008793537298,4.44672000677949,27.4689443989562));
#190267=CARTESIAN_POINT('Ctrl Pts',(-5.21860642687796,4.31167404124064,
27.4773668227139));
#190268=CARTESIAN_POINT('Ctrl Pts',(-5.33099399684997,4.17191924601885,
27.4857892464717));
#190269=CARTESIAN_POINT('Ctrl Pts',(-5.4376681125929,4.02790944502112,27.4942116702294));
#190270=CARTESIAN_POINT('Ctrl Pts',(-5.54434390601232,3.88389737916414,
27.5026342264476));
#190271=CARTESIAN_POINT('Ctrl Pts',(-5.64530586187403,3.73563043777246,
27.5110567826658));
#190272=CARTESIAN_POINT('Ctrl Pts',(-5.74022148867819,3.58359404242684,
27.519479338884));
#190273=CARTESIAN_POINT('Ctrl Pts',(-5.83514032175027,3.43155251126289,
27.5279021796178));
#190274=CARTESIAN_POINT('Ctrl Pts',(-5.92401224172111,3.27574155512807,
27.5363250203515));
#190275=CARTESIAN_POINT('Ctrl Pts',(-6.00654904914689,3.11667411196497,
27.5447478610853));
#190276=CARTESIAN_POINT('Ctrl Pts',(-6.08910016773277,2.95757908789926,
27.5531721622659));
#190277=CARTESIAN_POINT('Ctrl Pts',(-6.16531383015456,2.79522674714078,
27.5615964634465));
#190278=CARTESIAN_POINT('Ctrl Pts',(-6.234948446618,2.63015339248795,27.5700207646271));
#190279=CARTESIAN_POINT('Ctrl Pts',(-6.30460486185674,2.46502836243069,
27.5784477029939));
#190280=CARTESIAN_POINT('Ctrl Pts',(-6.36767799538117,2.29718092743717,
27.5868746413607));
#190281=CARTESIAN_POINT('Ctrl Pts',(-6.42397478820149,2.12716640640822,
27.5953015797276));
#190282=CARTESIAN_POINT('Ctrl Pts',(-6.48032219891496,1.95699902095436,
27.6037360949712));
#190283=CARTESIAN_POINT('Ctrl Pts',(-6.52988098962663,1.78466097304688,
27.6121706102149));
#190284=CARTESIAN_POINT('Ctrl Pts',(-6.57250795993592,1.61072285529788,
27.6206051254585));
#190285=CARTESIAN_POINT('Ctrl Pts',(-6.61515551943702,1.43670072394806,
27.6290437146453));
#190286=CARTESIAN_POINT('Ctrl Pts',(-6.65086450963091,1.26107730706265,
27.637482303832));
#190287=CARTESIAN_POINT('Ctrl Pts',(-6.67954296945572,1.08443290211735,
27.6459208930188));
#190288=CARTESIAN_POINT('Ctrl Pts',(-6.70825348531028,0.907591048692114,
27.6543689146391));
#190289=CARTESIAN_POINT('Ctrl Pts',(-6.72991772269395,0.729726257331115,
27.6628169362594));
#190290=CARTESIAN_POINT('Ctrl Pts',(-6.74449552026904,0.551424679417716,
27.6712649578797));
#190291=CARTESIAN_POINT('Ctrl Pts',(-6.75278130646117,0.450080923977191,
27.6760666777919));
#190292=CARTESIAN_POINT('Ctrl Pts',(-6.75877869763147,0.348596103748422,
27.6808683977041));
#190293=CARTESIAN_POINT('Ctrl Pts',(-6.76248782396277,0.247077782803984,
27.6856701176163));
#190294=CARTESIAN_POINT('Ctrl Pts',(-6.76545140137005,0.165965042092728,
27.6895066730142));
#190295=CARTESIAN_POINT('Ctrl Pts',(-6.76695633114201,0.0847788957426476,
27.6933432284121));
#190296=CARTESIAN_POINT('Ctrl Pts',(-6.76699906337201,0.00356038233445201,
27.69717978381));
#190297=CARTESIAN_POINT('',(-6.76699961187957,-0.00229190351974674,27.3028202162279));
#190298=CARTESIAN_POINT('Ctrl Pts',(3.0991061983213,6.01563211736942,26.6512942524228));
#190299=CARTESIAN_POINT('Ctrl Pts',(2.94383276466504,6.09562518398154,26.6594981890752));
#190300=CARTESIAN_POINT('Ctrl Pts',(2.78554342077026,6.16955974932361,26.6677021257276));
#190301=CARTESIAN_POINT('Ctrl Pts',(2.62475652218203,6.23722231440109,26.6759060623801));
#190302=CARTESIAN_POINT('Ctrl Pts',(2.46378057777883,6.30496443399993,26.6841196448426));
#190303=CARTESIAN_POINT('Ctrl Pts',(2.30030154507449,6.36641968763182,26.6923332273051));
#190304=CARTESIAN_POINT('Ctrl Pts',(2.1348554629473,6.4214236079178,26.7005468097676));
#190305=CARTESIAN_POINT('Ctrl Pts',(1.96929468394184,6.47646566013093,26.7087660863648));
#190306=CARTESIAN_POINT('Ctrl Pts',(1.80176448095945,6.52504736574828,26.7169853629619));
#190307=CARTESIAN_POINT('Ctrl Pts',(1.63281263736181,6.56705503945807,26.7252046395591));
#190308=CARTESIAN_POINT('Ctrl Pts',(1.46362873059184,6.60912041265084,26.7334352057129));
#190309=CARTESIAN_POINT('Ctrl Pts',(1.29301963370594,6.64459365085365,26.7416657718666));
#190310=CARTESIAN_POINT('Ctrl Pts',(1.12154069219706,6.67341258096232,26.7498963380204));
#190311=CARTESIAN_POINT('Ctrl Pts',(1.07487975720384,6.68125446645883,26.7521359477875));
#190312=CARTESIAN_POINT('Ctrl Pts',(1.02815442916004,6.68860394334448,26.7543755575546));
#190313=CARTESIAN_POINT('Ctrl Pts',(0.981375910960085,6.69546042639244,
26.7566151673218));
#190314=CARTESIAN_POINT('Ctrl Pts',(0.812833009482774,6.72016432021596,
26.7646844765443));
#190315=CARTESIAN_POINT('Ctrl Pts',(0.643047741566264,6.73854524219892,
26.7727537857668));
#190316=CARTESIAN_POINT('Ctrl Pts',(0.472545764272061,6.7504806866377,26.7808230949893));
#190317=CARTESIAN_POINT('Ctrl Pts',(0.302256449284434,6.76240124433331,
26.7888823395901));
#190318=CARTESIAN_POINT('Ctrl Pts',(0.131252571120187,6.76789229474629,
26.7969415841908));
#190319=CARTESIAN_POINT('Ctrl Pts',(-0.0399295845166925,6.76688219405956,
26.8050008287916));
#190320=CARTESIAN_POINT('Ctrl Pts',(-0.210935795122136,6.76587313157799,
26.8130517899119));
#190321=CARTESIAN_POINT('Ctrl Pts',(-0.382119548577863,6.75837621755593,
26.8211027510321));
#190322=CARTESIAN_POINT('Ctrl Pts',(-0.552939091407244,6.74437153196603,
26.8291537121524));
#190323=CARTESIAN_POINT('Ctrl Pts',(-0.723620491858464,6.73037817201569,
26.8371981624315));
#190324=CARTESIAN_POINT('Ctrl Pts',(-0.893937897912533,6.70988754566047,
26.8452426127106));
#190325=CARTESIAN_POINT('Ctrl Pts',(-1.06334931334904,6.68293178461371,
26.8532870629897));
#190326=CARTESIAN_POINT('Ctrl Pts',(-1.23266080774108,6.65599192242353,
26.8613267685479));
#190327=CARTESIAN_POINT('Ctrl Pts',(-1.40106700770738,6.6225945750113,26.8693664741062));
#190328=CARTESIAN_POINT('Ctrl Pts',(-1.56803090743718,6.58282371580173,
26.8774061796644));
#190329=CARTESIAN_POINT('Ctrl Pts',(-1.7385986336788,6.54219442385881,26.8856194179688));
#190330=CARTESIAN_POINT('Ctrl Pts',(-1.90766069180216,6.49491338734593,
26.8938326562733));
#190331=CARTESIAN_POINT('Ctrl Pts',(-2.07465492144769,6.4411253641668,26.9020458945777));
#190332=CARTESIAN_POINT('Ctrl Pts',(-2.23806820665575,6.38849074564611,
26.9100830121259));
#190333=CARTESIAN_POINT('Ctrl Pts',(-2.39950108146646,6.32962550801559,
26.9181201296741));
#190334=CARTESIAN_POINT('Ctrl Pts',(-2.55844205524812,6.2647157357647,26.9261572472223));
#190335=CARTESIAN_POINT('Ctrl Pts',(-2.71739984397433,6.19979909647256,
26.9341952150464));
#190336=CARTESIAN_POINT('Ctrl Pts',(-2.87386486079827,6.12883679043341,
26.9422331828705));
#190337=CARTESIAN_POINT('Ctrl Pts',(-3.02734586883941,6.05206295327643,
26.9502711506946));
#190338=CARTESIAN_POINT('Ctrl Pts',(-3.18087352444107,5.97526578220823,
26.9583115615023));
#190339=CARTESIAN_POINT('Ctrl Pts',(-3.33141503206904,5.89265373127158,
26.9663519723101));
#190340=CARTESIAN_POINT('Ctrl Pts',(-3.47850415630701,5.80450668313466,
26.9743923831178));
#190341=CARTESIAN_POINT('Ctrl Pts',(-3.63115241984803,5.71302817373379,
26.9827366761056));
#190342=CARTESIAN_POINT('Ctrl Pts',(-3.78008185807882,5.61558833844509,
26.9910809690934));
#190343=CARTESIAN_POINT('Ctrl Pts',(-3.92480572123883,5.51254832636694,
26.9994252620812));
#190344=CARTESIAN_POINT('Ctrl Pts',(-4.06450531092812,5.4130854797113,27.0074798722967));
#190345=CARTESIAN_POINT('Ctrl Pts',(-4.20028618576589,5.30840505205388,
27.0155344825122));
#190346=CARTESIAN_POINT('Ctrl Pts',(-4.33174593792675,5.19887162077071,
27.0235890927278));
#190347=CARTESIAN_POINT('Ctrl Pts',(-4.46330520697713,5.08925527113269,
27.031649800397));
#190348=CARTESIAN_POINT('Ctrl Pts',(-4.59053656432683,4.97477885105254,
27.0397105080663));
#190349=CARTESIAN_POINT('Ctrl Pts',(-4.71307542986726,4.85584276849875,
27.0477712157355));
#190350=CARTESIAN_POINT('Ctrl Pts',(-4.83578706786635,4.73673899319445,
27.0558432885197));
#190351=CARTESIAN_POINT('Ctrl Pts',(-4.95379275822236,4.61316327767268,
27.0639153613038));
#190352=CARTESIAN_POINT('Ctrl Pts',(-5.06676866695437,4.48554838069656,
27.0719874340879));
#190353=CARTESIAN_POINT('Ctrl Pts',(-5.07860203502974,4.47218168982619,
27.0728329223824));
#190354=CARTESIAN_POINT('Ctrl Pts',(-5.09038026136851,4.45877071037642,
27.0736784106768));
#190355=CARTESIAN_POINT('Ctrl Pts',(-5.10210300204977,4.44531595687806,
27.0745238989712));
#190356=CARTESIAN_POINT('Ctrl Pts',(-5.21798439699456,4.3123133044761,27.0828817024604));
#190357=CARTESIAN_POINT('Ctrl Pts',(-5.32881037871687,4.17460609882494,
27.0912395059495));
#190358=CARTESIAN_POINT('Ctrl Pts',(-5.43418447660398,4.03260809827045,
27.0995973094387));
#190359=CARTESIAN_POINT('Ctrl Pts',(-5.54094314081068,3.88874431045931,
27.1080649305533));
#190360=CARTESIAN_POINT('Ctrl Pts',(-5.64210535689717,3.74047639141668,
27.116532551668));
#190361=CARTESIAN_POINT('Ctrl Pts',(-5.7372978182351,3.58827294737661,27.1250001727826));
#190362=CARTESIAN_POINT('Ctrl Pts',(-5.83100808026938,3.43843939519139,
27.1333359483504));
#190363=CARTESIAN_POINT('Ctrl Pts',(-5.91893291945275,3.28479227163124,
27.1416717239182));
#190364=CARTESIAN_POINT('Ctrl Pts',(-6.00075701597266,3.1278114129939,27.150007499486));
#190365=CARTESIAN_POINT('Ctrl Pts',(-6.08251488675048,2.97095760951879,
27.1583365283502));
#190366=CARTESIAN_POINT('Ctrl Pts',(-6.15818169342941,2.81077575102921,
27.1666655572145));
#190367=CARTESIAN_POINT('Ctrl Pts',(-6.2274864770947,2.64777287122643,27.1749945860787));
#190368=CARTESIAN_POINT('Ctrl Pts',(-6.29674637522643,2.48487556092182,
27.1833182206125));
#190369=CARTESIAN_POINT('Ctrl Pts',(-6.35965232603162,2.31916118643877,
27.1916418551463));
#190370=CARTESIAN_POINT('Ctrl Pts',(-6.41598012033015,2.15115970944242,
27.1999654896801));
#190371=CARTESIAN_POINT('Ctrl Pts',(-6.47398342659767,1.97816090405742,
27.2085367168893));
#190372=CARTESIAN_POINT('Ctrl Pts',(-6.52501100444624,1.80273715993301,
27.2171079440984));
#190373=CARTESIAN_POINT('Ctrl Pts',(-6.56887177036432,1.62548843875023,
27.2256791713076));
#190374=CARTESIAN_POINT('Ctrl Pts',(-6.61143244030448,1.45349362375625,
27.2339963350551));
#190375=CARTESIAN_POINT('Ctrl Pts',(-6.64724502646991,1.279780837463,27.2423134988025));
#190376=CARTESIAN_POINT('Ctrl Pts',(-6.67618580650384,1.10491270109302,
27.25063066255));
#190377=CARTESIAN_POINT('Ctrl Pts',(-6.70645266264653,0.922032048904484,
27.25932892149));
#190378=CARTESIAN_POINT('Ctrl Pts',(-6.72920303762109,0.737888063829979,
27.26802718043));
#190379=CARTESIAN_POINT('Ctrl Pts',(-6.74435547311584,0.553134931325414,
27.27672543937));
#190380=CARTESIAN_POINT('Ctrl Pts',(-6.7595079086106,0.368381798820848,
27.2854236983099));
#190381=CARTESIAN_POINT('Ctrl Pts',(-6.76706237481184,0.183019949639337,
27.2941219572499));
#190382=CARTESIAN_POINT('Ctrl Pts',(-6.76699961187985,-0.00229190270927458,
27.3028202161899));
#190383=CARTESIAN_POINT('Ctrl Pts',(-6.76699961187957,-0.00229190351973855,
27.3028202162279));
#190384=CARTESIAN_POINT('Ctrl Pts',(-6.76692935620143,-0.209726528320418,
27.3125568847506));
#190385=CARTESIAN_POINT('Ctrl Pts',(-6.75731700521489,-0.416851375284489,
27.3222935532733));
#190386=CARTESIAN_POINT('Ctrl Pts',(-6.7382722925091,-0.622876803231719,
27.332030221796));
#190387=CARTESIAN_POINT('Ctrl Pts',(-6.7185813253142,-0.835893402940784,
27.3420972899335));
#190388=CARTESIAN_POINT('Ctrl Pts',(-6.68880680709447,-1.04773457373278,
27.3521643580709));
#190389=CARTESIAN_POINT('Ctrl Pts',(-6.64912538009576,-1.25754549808999,
27.3622314262084));
#190390=CARTESIAN_POINT('Ctrl Pts',(-6.60944395309706,-1.4673564224472,
27.3722984943459));
#190391=CARTESIAN_POINT('Ctrl Pts',(-6.55985570281287,-1.67513707154593,
27.3823655624833));
#190392=CARTESIAN_POINT('Ctrl Pts',(-6.50059196810456,-1.88005134616439,
27.3924326306208));
#190393=CARTESIAN_POINT('Ctrl Pts',(-6.45084615562013,-2.05205581282049,
27.4008828993441));
#190394=CARTESIAN_POINT('Ctrl Pts',(-6.39422714905118,-2.22223068762529,
27.4093331680675));
#190395=CARTESIAN_POINT('Ctrl Pts',(-6.33088855698631,-2.39000817551317,
27.4177834367908));
#190396=CARTESIAN_POINT('Ctrl Pts',(-6.26760586337782,-2.55763759407583,
27.4262262478653));
#190397=CARTESIAN_POINT('Ctrl Pts',(-6.19761552091997,-2.72287353407569,
27.4346690589398));
#190398=CARTESIAN_POINT('Ctrl Pts',(-6.12112090541313,-2.88516340287936,
27.4431118700143));
#190399=CARTESIAN_POINT('Ctrl Pts',(-6.04468338406107,-3.04733214155083,
27.4515483795321));
#190400=CARTESIAN_POINT('Ctrl Pts',(-5.96175140807754,-3.20655889344229,
27.4599848890498));
#190401=CARTESIAN_POINT('Ctrl Pts',(-5.87257656555222,-3.36231073545068,
27.4684213985675));
#190402=CARTESIAN_POINT('Ctrl Pts',(-5.78346553242522,-3.5179511286351,
27.4768518713087));
#190403=CARTESIAN_POINT('Ctrl Pts',(-5.68812070747364,-3.67012128457289,
27.4852823440499));
#190404=CARTESIAN_POINT('Ctrl Pts',(-5.58683983253178,-3.81831241330988,
27.4937128167911));
#190405=CARTESIAN_POINT('Ctrl Pts',(-5.4856024979637,-3.96643983508205,
27.502139665295));
#190406=CARTESIAN_POINT('Ctrl Pts',(-5.37843438744359,-4.1105913664876,
27.5105665137988));
#190407=CARTESIAN_POINT('Ctrl Pts',(-5.26567716922619,-4.25028621971392,
27.5189933623026));
#190408=CARTESIAN_POINT('Ctrl Pts',(-5.15295475513509,-4.38993795412807,
27.5274176097392));
#190409=CARTESIAN_POINT('Ctrl Pts',(-5.03464688174096,-4.52513549595337,
27.5358418571758));
#190410=CARTESIAN_POINT('Ctrl Pts',(-4.9111364192475,-4.65542995560462,
27.5442661046125));
#190411=CARTESIAN_POINT('Ctrl Pts',(-4.8763358964991,-4.6921419491924,27.5466397352235));
#190412=CARTESIAN_POINT('Ctrl Pts',(-4.84112258449267,-4.72846489357281,
27.5490133658345));
#190413=CARTESIAN_POINT('Ctrl Pts',(-4.80550560803795,-4.7643892421921,
27.5513869964455));
#190414=CARTESIAN_POINT('Ctrl Pts',(-4.67617844302602,-4.89483249213332,
27.5600057773828));
#190415=CARTESIAN_POINT('Ctrl Pts',(-4.5415841897705,-5.0199592705319,27.56862455832));
#190416=CARTESIAN_POINT('Ctrl Pts',(-4.4021859336116,-5.1393626069691,27.5772433392572));
#190417=CARTESIAN_POINT('Ctrl Pts',(-4.26270394176749,-5.25883766826476,
27.5858672974438));
#190418=CARTESIAN_POINT('Ctrl Pts',(-4.11841241898026,-5.37258222844547,
27.5944912556303));
#190419=CARTESIAN_POINT('Ctrl Pts',(-3.96980693260753,-5.48023009716026,
27.6031152138169));
#190420=CARTESIAN_POINT('Ctrl Pts',(-3.8158328370502,-5.59176691608001,
27.612050726188));
#190421=CARTESIAN_POINT('Ctrl Pts',(-3.65722756505202,-5.69675811833182,
27.6209862385591));
#190422=CARTESIAN_POINT('Ctrl Pts',(-3.49457381291732,-5.79484623316896,
27.6299217509302));
#190423=CARTESIAN_POINT('Ctrl Pts',(-3.33729780225805,-5.88969130862654,
27.6385618328249));
#190424=CARTESIAN_POINT('Ctrl Pts',(-3.17623702193311,-5.97808235164047,
27.6472019147197));
#190425=CARTESIAN_POINT('Ctrl Pts',(-3.01194252884547,-6.05974349316306,
27.6558419966144));
#190426=CARTESIAN_POINT('Ctrl Pts',(-2.8392214488999,-6.14559299601794,
27.6649252242237));
#190427=CARTESIAN_POINT('Ctrl Pts',(-2.66292659147694,-6.22400395746316,
27.674008451833));
#190428=CARTESIAN_POINT('Ctrl Pts',(-2.48372148272282,-6.29471338475877,
27.6830916794423));
#190429=CARTESIAN_POINT('Ctrl Pts',(-2.3045163739687,-6.36542281205437,
27.6921749070516));
#190430=CARTESIAN_POINT('Ctrl Pts',(-2.12240139134993,-6.42843061021735,
27.701258134661));
#190431=CARTESIAN_POINT('Ctrl Pts',(-1.93805838123456,-6.48353443045739,
27.7103413622703));
#190432=CARTESIAN_POINT('Ctrl Pts',(-1.75449941811638,-6.53840388333648,
27.7193859571301));
#190433=CARTESIAN_POINT('Ctrl Pts',(-1.56856207868349,-6.58548795982809,
27.7284305519899));
#190434=CARTESIAN_POINT('Ctrl Pts',(-1.38089389838517,-6.62460723676526,
27.7374751468497));
#190435=CARTESIAN_POINT('Ctrl Pts',(-1.19339793318271,-6.66369061560816,
27.7465114418701));
#190436=CARTESIAN_POINT('Ctrl Pts',(-1.00417453088861,-6.6948237387627,
27.7555477368904));
#190437=CARTESIAN_POINT('Ctrl Pts',(-0.813882946743737,-6.71787790518701,
27.7645840319108));
#190438=CARTESIAN_POINT('Ctrl Pts',(-0.623928098479182,-6.74089127545598,
27.7736043364985));
#190439=CARTESIAN_POINT('Ctrl Pts',(-0.432909078774653,-6.75585420840333,
27.7826246410862));
#190440=CARTESIAN_POINT('Ctrl Pts',(-0.241491647624095,-6.76268961169503,
27.7916449456739));
#190441=CARTESIAN_POINT('Ctrl Pts',(-0.0503152695442017,-6.76951640712409,
27.8006538909402));
#190442=CARTESIAN_POINT('Ctrl Pts',(0.141258281686187,-6.76823609006339,
27.8096628362065));
#190443=CARTESIAN_POINT('Ctrl Pts',(0.332559284423795,-6.75882336818647,
27.8186717814728));
#190444=CARTESIAN_POINT('Ctrl Pts',(0.52342588308228,-6.74943202060828,
27.8276602693316));
#190445=CARTESIAN_POINT('Ctrl Pts',(0.714020931458135,-6.7319451415487,
27.8366487571904));
#190446=CARTESIAN_POINT('Ctrl Pts',(0.903676357486737,-6.70638934456683,
27.8456372450492));
#190447=CARTESIAN_POINT('Ctrl Pts',(1.07007289165117,-6.68396764994602,
27.8535234060645));
#190448=CARTESIAN_POINT('Ctrl Pts',(1.2357459922794,-6.65533554034296,27.8614095670797));
#190449=CARTESIAN_POINT('Ctrl Pts',(1.40024481847694,-6.62054404473896,
27.869295728095));
#190450=CARTESIAN_POINT('Ctrl Pts',(1.56965188907279,-6.58471445562782,
27.8774171929512));
#190451=CARTESIAN_POINT('Ctrl Pts',(1.73773739248944,-6.54236687363886,
27.8855386578074));
#190452=CARTESIAN_POINT('Ctrl Pts',(1.90396353704619,-6.49362855802506,
27.8936601226635));
#190453=CARTESIAN_POINT('Ctrl Pts',(2.07017782723239,-6.44489371817047,
27.9017810083397));
#190454=CARTESIAN_POINT('Ctrl Pts',(2.23453267128481,-6.38976915551758,
27.9099018940159));
#190455=CARTESIAN_POINT('Ctrl Pts',(2.39650459400326,-6.32843224905832,
27.9180227796922));
#190456=CARTESIAN_POINT('Ctrl Pts',(2.55849587699832,-6.2670880110847,27.9261446360464));
#190457=CARTESIAN_POINT('Ctrl Pts',(2.71810332948052,-6.19953008151649,
27.9342664924007));
#190458=CARTESIAN_POINT('Ctrl Pts',(2.87482268923173,-6.12598428870646,
27.942388348755));
#190459=CARTESIAN_POINT('Ctrl Pts',(3.03165638948868,-6.05238483779601,
27.9505161307152));
#190460=CARTESIAN_POINT('Ctrl Pts',(3.18559745668893,-5.9727889539448,27.9586439126753));
#190461=CARTESIAN_POINT('Ctrl Pts',(3.33616494306543,-5.88746910587744,
27.9667716946355));
#190462=CARTESIAN_POINT('Ctrl Pts',(3.48679376503956,-5.80211450167516,
27.974902787552));
#190463=CARTESIAN_POINT('Ctrl Pts',(3.63404595567512,-5.7110314779604,27.9830338804684));
#190464=CARTESIAN_POINT('Ctrl Pts',(3.77746910933932,-5.61453614539859,
27.9911649733849));
#190465=CARTESIAN_POINT('Ctrl Pts',(3.92104880338185,-5.51793549221399,
27.9993049410494));
#190466=CARTESIAN_POINT('Ctrl Pts',(4.06079081773718,-5.41591094698189,
28.007444908714));
#190467=CARTESIAN_POINT('Ctrl Pts',(4.19627482356807,-5.30881969980982,
28.0155848763785));
#190468=CARTESIAN_POINT('Ctrl Pts',(4.26654268694401,-5.25327754869835,
28.019806615559));
#190469=CARTESIAN_POINT('Ctrl Pts',(4.33566576122989,-5.19637313556894,
28.0240283547394));
#190470=CARTESIAN_POINT('Ctrl Pts',(4.40358931946146,-5.13816018683,28.0282500939198));
#190471=CARTESIAN_POINT('Ctrl Pts',(4.53938384254327,-5.02177936378421,
28.0366903033774));
#190472=CARTESIAN_POINT('Ctrl Pts',(4.6706624990829,-4.89992571217488,28.0451305128351));
#190473=CARTESIAN_POINT('Ctrl Pts',(4.79697621810871,-4.77297686595059,
28.0535707222927));
#190474=CARTESIAN_POINT('Ctrl Pts',(4.92319423577882,-4.64612420228494,
28.0620045370412));
#190475=CARTESIAN_POINT('Ctrl Pts',(5.04445458021174,-4.51418427493211,
28.0704383517898));
#190476=CARTESIAN_POINT('Ctrl Pts',(5.16034305538164,-4.37757336326583,
28.0788721665383));
#190477=CARTESIAN_POINT('Ctrl Pts',(5.27616154303811,-4.24104495383284,
28.0873008879268));
#190478=CARTESIAN_POINT('Ctrl Pts',(5.38661441399116,-4.09985143763769,
28.0957296093154));
#190479=CARTESIAN_POINT('Ctrl Pts',(5.49132572560371,-3.95444443320714,
28.1041583307039));
#190480=CARTESIAN_POINT('Ctrl Pts',(5.59598987908404,-3.80910291475547,
28.1125832561057));
#190481=CARTESIAN_POINT('Ctrl Pts',(5.69491743443856,-3.65955196183723,
28.1210081815074));
#190482=CARTESIAN_POINT('Ctrl Pts',(5.78777376227501,-3.50627492885555,
28.1294331069091));
#190483=CARTESIAN_POINT('Ctrl Pts',(5.88060251794135,-3.35304340898564,
28.1378555306669));
#190484=CARTESIAN_POINT('Ctrl Pts',(5.96736346856393,-3.19608830037617,
28.1462779544246));
#190485=CARTESIAN_POINT('Ctrl Pts',(6.04776601329938,-3.03592082379975,
28.1547003781823));
#190486=CARTESIAN_POINT('Ctrl Pts',(6.12816982253537,-2.87575082825006,
28.1631229344005));
#190487=CARTESIAN_POINT('Ctrl Pts',(6.20221487056331,-2.71236865877128,
28.1715454906187));
#190488=CARTESIAN_POINT('Ctrl Pts',(6.2696568198473,-2.54630955724993,28.1799680468369));
#190489=CARTESIAN_POINT('Ctrl Pts',(6.33710104733314,-2.38024484622059,
28.1883908875706));
#190490=CARTESIAN_POINT('Ctrl Pts',(6.39794160564978,-2.21150333184239,
28.1968137283044));
#190491=CARTESIAN_POINT('Ctrl Pts',(6.45198251134582,-2.04063977058366,
28.2052365690381));
#190492=CARTESIAN_POINT('Ctrl Pts',(6.50603278726208,-1.86974658307837,
28.2136608702188));
#190493=CARTESIAN_POINT('Ctrl Pts',(6.55328095939107,-1.69673093315023,
28.2220851713994));
#190494=CARTESIAN_POINT('Ctrl Pts',(6.59358096982342,-1.52216260444884,
28.2305094725801));
#190495=CARTESIAN_POINT('Ctrl Pts',(6.63389359597634,-1.34753962798846,
28.2389364109468));
#190496=CARTESIAN_POINT('Ctrl Pts',(6.66725364889593,-1.17136332857334,
28.2473633493137));
#190497=CARTESIAN_POINT('Ctrl Pts',(6.69356614328442,-0.994213903280681,
28.2557902876804));
#190498=CARTESIAN_POINT('Ctrl Pts',(6.71990229591283,-0.816905198387038,
28.2642248029241));
#190499=CARTESIAN_POINT('Ctrl Pts',(6.73917817934357,-0.638621949562761,
28.2726593181678));
#190500=CARTESIAN_POINT('Ctrl Pts',(6.75135054734373,-0.459950852680545,
28.2810938334114));
#190501=CARTESIAN_POINT('Ctrl Pts',(6.76352879470191,-0.281193456127886,
28.2895324225982));
#190502=CARTESIAN_POINT('Ctrl Pts',(6.76859666922576,-0.102048170990221,
28.297971011785));
#190503=CARTESIAN_POINT('Ctrl Pts',(6.76656306921745,0.0768975311863861,
28.3064096009717));
#190504=CARTESIAN_POINT('Ctrl Pts',(6.76452719610442,0.256043254172507,
28.314857622592));
#190505=CARTESIAN_POINT('Ctrl Pts',(6.75537399924369,0.434988615036042,
28.3233056442123));
#190506=CARTESIAN_POINT('Ctrl Pts',(6.73916441327626,0.613149256568786,
28.3317536658326));
#190507=CARTESIAN_POINT('Ctrl Pts',(6.72995114474939,0.714412906032747,
28.3365553857449));
#190508=CARTESIAN_POINT('Ctrl Pts',(6.71845918276298,0.815423164162881,
28.3413571056571));
#190509=CARTESIAN_POINT('Ctrl Pts',(6.70470709845652,0.916074082106259,
28.3461588255693));
#190510=CARTESIAN_POINT('Ctrl Pts',(6.68110915048584,1.08878645587435,28.3543983574201));
#190511=CARTESIAN_POINT('Ctrl Pts',(6.65080067256821,1.26082572099317,28.362637889271));
#190512=CARTESIAN_POINT('Ctrl Pts',(6.61382766119517,1.43163286774565,28.3708774211218));
#190513=CARTESIAN_POINT('Ctrl Pts',(6.5768956872807,1.60225043050297,28.3791078076681));
#190514=CARTESIAN_POINT('Ctrl Pts',(6.53331398354332,1.77163825316013,28.3873381942145));
#190515=CARTESIAN_POINT('Ctrl Pts',(6.48318023834598,1.93924289276001,28.3955685807608));
#190516=CARTESIAN_POINT('Ctrl Pts',(6.43309319470263,2.10669140205094,28.4037913003786));
#190517=CARTESIAN_POINT('Ctrl Pts',(6.37646636618576,2.27235969742888,28.4120140199964));
#190518=CARTESIAN_POINT('Ctrl Pts',(6.31344840173509,2.43570488331995,28.4202367396142));
#190519=CARTESIAN_POINT('Ctrl Pts',(6.25048627574123,2.59890533360766,28.42845217331));
#190520=CARTESIAN_POINT('Ctrl Pts',(6.18114442833579,2.75978644629152,28.4366676070058));
#190521=CARTESIAN_POINT('Ctrl Pts',(6.10562116455277,2.9178209669144,28.4448830407015));
#190522=CARTESIAN_POINT('Ctrl Pts',(6.03013671386276,3.07577427006547,28.4530942523024));
#190523=CARTESIAN_POINT('Ctrl Pts',(5.9484773266948,3.23088357436767,28.4613054639032));
#190524=CARTESIAN_POINT('Ctrl Pts',(5.86088936719711,3.38264169333317,28.469516675504));
#190525=CARTESIAN_POINT('Ctrl Pts',(5.77333077986805,3.53434892099937,28.4777251335175));
#190526=CARTESIAN_POINT('Ctrl Pts',(5.67984775842618,3.68270689412139,28.4859335915311));
#190527=CARTESIAN_POINT('Ctrl Pts',(5.58073258542937,3.82723304881305,28.4941420495446));
#190528=CARTESIAN_POINT('Ctrl Pts',(5.53657461160154,3.89162260657044,28.4977990968278));
#190529=CARTESIAN_POINT('Ctrl Pts',(5.49129931099631,3.95525193628647,28.5014561441109));
#190530=CARTESIAN_POINT('Ctrl Pts',(5.44493534228971,4.01808015329268,28.5051131913941));
#190531=CARTESIAN_POINT('Ctrl Pts',(5.33263634492837,4.17025750075933,28.5139709909885));
#190532=CARTESIAN_POINT('Ctrl Pts',(5.21406458886683,4.31757487740604,28.5228287905828));
#190533=CARTESIAN_POINT('Ctrl Pts',(5.08966368674469,4.45955295470661,28.5316865901772));
#190534=CARTESIAN_POINT('Ctrl Pts',(4.96502798744218,4.60179900476024,28.5405611081902));
#190535=CARTESIAN_POINT('Ctrl Pts',(4.83454132547222,4.73868542096927,28.5494356262033));
#190536=CARTESIAN_POINT('Ctrl Pts',(4.69868395107327,4.86976982288963,28.5583101442164));
#190537=CARTESIAN_POINT('Ctrl Pts',(4.56245570530148,5.00121206664459,28.5672088884055));
#190538=CARTESIAN_POINT('Ctrl Pts',(4.42082759892887,5.126820423822,28.5761076325947));
#190539=CARTESIAN_POINT('Ctrl Pts',(4.27431492765299,5.24619108489606,28.5850063767839));
#190540=CARTESIAN_POINT('Ctrl Pts',(4.12760021857274,5.36572635552953,28.5939173921488));
#190541=CARTESIAN_POINT('Ctrl Pts',(3.97598769379786,5.47900658847,28.6028284075138));
#190542=CARTESIAN_POINT('Ctrl Pts',(3.82002257712792,5.58567064104508,28.6117394228787));
#190543=CARTESIAN_POINT('Ctrl Pts',(3.66374397081258,5.69254908820232,28.6206683493708));
#190544=CARTESIAN_POINT('Ctrl Pts',(3.50309549256772,5.79278461607391,28.629597275863));
#190545=CARTESIAN_POINT('Ctrl Pts',(3.33865005573199,5.88606021081681,28.6385262023551));
#190546=CARTESIAN_POINT('Ctrl Pts',(3.25965616527438,5.93086657489275,28.6428153492892));
#190547=CARTESIAN_POINT('Ctrl Pts',(3.1797864617139,5.97406762348353,28.6471044962232));
#190548=CARTESIAN_POINT('Ctrl Pts',(3.09910619832131,6.01563211736942,28.6513936431573));
#190549=CARTESIAN_POINT('Origin',(0.,0.,4.30282021618968));
#190550=CARTESIAN_POINT('',(3.09910619832132,6.01563211736941,31.0457552630242));
#190551=CARTESIAN_POINT('',(3.09910619832131,6.01563211736941,30.6515994289918));
#190552=CARTESIAN_POINT('',(3.09910619832133,6.0156321173694,4.30282021618968));
#190553=CARTESIAN_POINT('',(-6.767,7.81740666123965E-13,29.6971797838101));
#190554=CARTESIAN_POINT('Ctrl Pts',(-6.767,7.81740771273666E-13,29.6971797838101));
#190555=CARTESIAN_POINT('Ctrl Pts',(-6.76700000000002,-0.186007249526226,
29.7059292956213));
#190556=CARTESIAN_POINT('Ctrl Pts',(-6.75932637294523,-0.37201435574941,
29.7146788074325));
#190557=CARTESIAN_POINT('Ctrl Pts',(-6.74400518264183,-0.557389537487122,
29.7234283192437));
#190558=CARTESIAN_POINT('Ctrl Pts',(-6.72868405705087,-0.742763936251697,
29.7321777940994));
#190559=CARTESIAN_POINT('Ctrl Pts',(-6.70571545645723,-0.927506130242437,
29.740927268955));
#190560=CARTESIAN_POINT('Ctrl Pts',(-6.67517739404794,-1.11098863990204,
29.7496767438107));
#190561=CARTESIAN_POINT('Ctrl Pts',(-6.64463945808665,-1.29447038982134,
29.7584261824377));
#190562=CARTESIAN_POINT('Ctrl Pts',(-6.60653217008313,-1.47669218313869,
29.7671756210647));
#190563=CARTESIAN_POINT('Ctrl Pts',(-6.56098496092631,-1.65703510599469,
29.7759250596917));
#190564=CARTESIAN_POINT('Ctrl Pts',(-6.51543793658245,-1.83737729708884,
29.7846744628169));
#190565=CARTESIAN_POINT('Ctrl Pts',(-6.46245112167363,-2.01584035511112,
29.7934238659421));
#190566=CARTESIAN_POINT('Ctrl Pts',(-6.4022044837419,-2.19181813760978,
29.8021732690673));
#190567=CARTESIAN_POINT('Ctrl Pts',(-6.34195808526437,-2.36779522067323,
29.8109226374173));
#190568=CARTESIAN_POINT('Ctrl Pts',(-6.27445201433034,-2.54128677684338,
29.8196720057674));
#190569=CARTESIAN_POINT('Ctrl Pts',(-6.1999155507183,-2.71170355384977,
29.8284213741175));
#190570=CARTESIAN_POINT('Ctrl Pts',(-6.12537937716614,-2.88211966767644,
29.8371707084193));
#190571=CARTESIAN_POINT('Ctrl Pts',(-6.04381298052436,-3.04946076371953,
29.8459200427211));
#190572=CARTESIAN_POINT('Ctrl Pts',(-5.95549339335741,-3.21315848374715,
29.8546693770229));
#190573=CARTESIAN_POINT('Ctrl Pts',(-5.86717414255318,-3.3768555803365,
29.8634186780031));
#190574=CARTESIAN_POINT('Ctrl Pts',(-5.77210188876508,-3.53690907646903,
29.8721679789833));
#190575=CARTESIAN_POINT('Ctrl Pts',(-5.67059953346907,-3.69277536969424,
29.8809172799634));
#190576=CARTESIAN_POINT('Ctrl Pts',(-5.56909755631295,-3.84864108225051,
29.8896665483487));
#190577=CARTESIAN_POINT('Ctrl Pts',(-5.46116568196763,-4.00031938297635,
29.898415816734));
#190578=CARTESIAN_POINT('Ctrl Pts',(-5.34717048533519,-4.14729511859963,
29.9071650851193));
#190579=CARTESIAN_POINT('Ctrl Pts',(-5.23317570391761,-4.29427031888008,
29.9159143216363));
#190580=CARTESIAN_POINT('Ctrl Pts',(-5.11311782003448,-4.43654276189623,
29.9246635581533));
#190581=CARTESIAN_POINT('Ctrl Pts',(-4.98740458984698,-4.57362924351912,
29.9334127946704));
#190582=CARTESIAN_POINT('Ctrl Pts',(-4.86169180711681,-4.71071523720332,
29.9421620000458));
#190583=CARTESIAN_POINT('Ctrl Pts',(-4.73032391204102,-4.84261509523306,
29.9509112054213));
#190584=CARTESIAN_POINT('Ctrl Pts',(-4.59374707013521,-4.96888084538402,
29.9596604107967));
#190585=CARTESIAN_POINT('Ctrl Pts',(-4.45717070301378,-5.09514615659522,
29.9684095857571));
#190586=CARTESIAN_POINT('Ctrl Pts',(-4.31538563570984,-5.21577720459574,
29.9771587607176));
#190587=CARTESIAN_POINT('Ctrl Pts',(-4.16887341029465,-5.33036429232921,
29.985907935678));
#190588=CARTESIAN_POINT('Ctrl Pts',(-4.02236168203633,-5.44495099123671,
29.99465708095));
#190589=CARTESIAN_POINT('Ctrl Pts',(-3.87112305348063,-5.55349359438674,
30.0034062262221));
#190590=CARTESIAN_POINT('Ctrl Pts',(-3.71567117017626,-5.65562346298982,
30.0121553714941));
#190591=CARTESIAN_POINT('Ctrl Pts',(-3.56021980145682,-5.75775299351728,
30.0209044878043));
#190592=CARTESIAN_POINT('Ctrl Pts',(-3.40055544538211,-5.85346967463953,
30.0296536041145));
#190593=CARTESIAN_POINT('Ctrl Pts',(-3.23722035986713,-5.94244842986977,
30.0384027204246));
#190594=CARTESIAN_POINT('Ctrl Pts',(-3.07388580147008,-6.03142689794618,
30.0471518084995));
#190595=CARTESIAN_POINT('Ctrl Pts',(-2.90688078896373,-6.1136673465688,
30.0559008965743));
#190596=CARTESIAN_POINT('Ctrl Pts',(-2.73677250721131,-6.18889046952459,
30.0646499846492));
#190597=CARTESIAN_POINT('Ctrl Pts',(-2.56666476031231,-6.2641133559643,
30.0733990452152));
#190598=CARTESIAN_POINT('Ctrl Pts',(-2.39345402574903,-6.33231884500655,
30.0821481057813));
#190599=CARTESIAN_POINT('Ctrl Pts',(-2.21772856065317,-6.39327529762822,
30.0908971663473));
#190600=CARTESIAN_POINT('Ctrl Pts',(-2.04200363348209,-6.45423156365208,
30.099646200131));
#190601=CARTESIAN_POINT('Ctrl Pts',(-1.86376426188944,-6.50793874375755,
30.1083952339147));
#190602=CARTESIAN_POINT('Ctrl Pts',(-1.6836157775279,-6.55421443909636,
30.1171442676984));
#190603=CARTESIAN_POINT('Ctrl Pts',(-1.50346782967444,-6.60048999661949,
30.1258932754262));
#190604=CARTESIAN_POINT('Ctrl Pts',(-1.3214110579464,-6.63933404237781,
30.1346422831541));
#190605=CARTESIAN_POINT('Ctrl Pts',(-1.13806375486686,-6.67061465607618,
30.1433912908819));
#190606=CARTESIAN_POINT('Ctrl Pts',(-0.95471698259975,-6.70189517921342,
30.1521402732803));
#190607=CARTESIAN_POINT('Ctrl Pts',(-0.770079968898975,-6.72561226592264,
30.1608892556787));
#190608=CARTESIAN_POINT('Ctrl Pts',(-0.584779765555192,-6.74168536983129,
30.1696382380771));
#190609=CARTESIAN_POINT('Ctrl Pts',(-0.391489830648283,-6.7584515101387,
30.178764457087));
#190610=CARTESIAN_POINT('Ctrl Pts',(-0.197478578235363,-6.76689983031634,
30.1878906760968));
#190611=CARTESIAN_POINT('Ctrl Pts',(-0.00346287644841733,-6.76699911397118,
30.1970168951067));
#190612=CARTESIAN_POINT('Ctrl Pts',(0.184489834657685,-6.76709529501181,
30.2058579197725));
#190613=CARTESIAN_POINT('Ctrl Pts',(0.37244640425314,-6.75935639738147,
30.2146989444383));
#190614=CARTESIAN_POINT('Ctrl Pts',(0.559755019492074,-6.74380925873156,
30.2235399691041));
#190615=CARTESIAN_POINT('Ctrl Pts',(0.745134705525503,-6.72842222659764,
30.2322899477139));
#190616=CARTESIAN_POINT('Ctrl Pts',(0.929879431232284,-6.70538706057472,
30.2410399263236));
#190617=CARTESIAN_POINT('Ctrl Pts',(1.11336163627195,-6.67478200894066,
30.2497899049333));
#190618=CARTESIAN_POINT('Ctrl Pts',(1.29684196301104,-6.64417727060938,
30.2585397939699));
#190619=CARTESIAN_POINT('Ctrl Pts',(1.47905951217911,-6.60600284890501,
30.2672896830064));
#190620=CARTESIAN_POINT('Ctrl Pts',(1.659395320675,-6.56038841607126,30.2760395720429));
#190621=CARTESIAN_POINT('Ctrl Pts',(1.83972934301221,-6.51477443503138,
30.2847893744151));
#190622=CARTESIAN_POINT('Ctrl Pts',(2.01818138406688,-6.46172066062009,
30.2935391767873));
#190623=CARTESIAN_POINT('Ctrl Pts',(2.19414528354625,-6.40140730423332,
30.3022889791594));
#190624=CARTESIAN_POINT('Ctrl Pts',(2.37010749864422,-6.34109452518484,
30.3110386977757));
#190625=CARTESIAN_POINT('Ctrl Pts',(2.54358134866877,-6.27352239616335,
30.3197884163921));
#190626=CARTESIAN_POINT('Ctrl Pts',(2.71397759435968,-6.19892043966638,
30.3285381350084));
#190627=CARTESIAN_POINT('Ctrl Pts',(2.88437226558535,-6.12431917249321,
30.3372877727771));
#190628=CARTESIAN_POINT('Ctrl Pts',(3.05168912681365,-6.04268832278592,
30.3460374105458));
#190629=CARTESIAN_POINT('Ctrl Pts',(3.21535986274262,-5.95430516123114,
30.3547870483145));
#190630=CARTESIAN_POINT('Ctrl Pts',(3.37902914073255,-5.86592278697203,
30.3635366081436));
#190631=CARTESIAN_POINT('Ctrl Pts',(3.5390521062199,-5.77078835741686,30.3722861679727));
#190632=CARTESIAN_POINT('Ctrl Pts',(3.69488522832119,-5.66922500431355,
30.3810357278017));
#190633=CARTESIAN_POINT('Ctrl Pts',(3.85071701407367,-5.56766252216798,
30.3897852125989));
#190634=CARTESIAN_POINT('Ctrl Pts',(4.00235878822836,-5.45967138329054,
30.398534697396));
#190635=CARTESIAN_POINT('Ctrl Pts',(4.14929549611761,-5.34561838199269,
30.4072841821931));
#190636=CARTESIAN_POINT('Ctrl Pts',(4.29623099276522,-5.23156632086661,
30.4160335948657));
#190637=CARTESIAN_POINT('Ctrl Pts',(4.43846127436456,-5.11145267304592,
30.4247830075383));
#190638=CARTESIAN_POINT('Ctrl Pts',(4.57550326054866,-4.98568540049496,
30.4335324202109));
#190639=CARTESIAN_POINT('Ctrl Pts',(4.71254416258193,-4.8599191228996,30.4422817636661));
#190640=CARTESIAN_POINT('Ctrl Pts',(4.84439664019163,-4.72849950385007,
30.4510311071214));
#190641=CARTESIAN_POINT('Ctrl Pts',(4.97061286795135,-4.59187289860646,
30.4597804505766));
#190642=CARTESIAN_POINT('Ctrl Pts',(5.09682813913057,-4.45524732884258,
30.4685297277214));
#190643=CARTESIAN_POINT('Ctrl Pts',(5.21740705148194,-4.31341506235357,
30.4772790048663));
#190644=CARTESIAN_POINT('Ctrl Pts',(5.33194007546035,-4.16685781275291,
30.4860282820111));
#190645=CARTESIAN_POINT('Ctrl Pts',(5.44647226944804,-4.0203016252141,30.4947774957522));
#190646=CARTESIAN_POINT('Ctrl Pts',(5.55495848628411,-3.86902074887505,
30.5035267094933));
#190647=CARTESIAN_POINT('Ctrl Pts',(5.65703027292067,-3.71352898080238,
30.5122759232344));
#190648=CARTESIAN_POINT('Ctrl Pts',(5.75910135377258,-3.55803828789165,
30.5210250764783));
#190649=CARTESIAN_POINT('Ctrl Pts',(5.85475793592996,-3.39833700106292,
30.5297742297222));
#190650=CARTESIAN_POINT('Ctrl Pts',(5.94367514427625,-3.23496750823137,
30.5385233829661));
#190651=CARTESIAN_POINT('Ctrl Pts',(6.03259176732859,-3.07159909077295,
30.547272478619));
#190652=CARTESIAN_POINT('Ctrl Pts',(6.11476896836134,-2.90456276730992,
30.5560215742719));
#190653=CARTESIAN_POINT('Ctrl Pts',(6.18992765548087,-2.73442583002596,
30.5647706699249));
#190654=CARTESIAN_POINT('Ctrl Pts',(6.26508587283246,-2.56428995615703,
30.5735197108929));
#190655=CARTESIAN_POINT('Ctrl Pts',(6.33322554827342,-2.39105376934722,
30.5822687518609));
#190656=CARTESIAN_POINT('Ctrl Pts',(6.39411526733201,-2.21530561053587,
30.591017792829));
#190657=CARTESIAN_POINT('Ctrl Pts',(6.45500462603,-2.03955849184614,30.599766782018));
#190658=CARTESIAN_POINT('Ctrl Pts',(6.50864402040876,-1.8612997016407,30.608515771207));
#190659=CARTESIAN_POINT('Ctrl Pts',(6.5548512836872,-1.68113463135594,30.617264760396));
#190660=CARTESIAN_POINT('Ctrl Pts',(6.60199809554427,-1.49730620116425,
30.6261916458675));
#190661=CARTESIAN_POINT('Ctrl Pts',(6.64140720707956,-1.31149343245275,
30.6351185313389));
#190662=CARTESIAN_POINT('Ctrl Pts',(6.67293928722951,-1.12435326697124,
30.6440454168103));
#190663=CARTESIAN_POINT('Ctrl Pts',(6.70384625876313,-0.940923067002602,
30.6527953309878));
#190664=CARTESIAN_POINT('Ctrl Pts',(6.7271855457984,-0.756217899517709,
30.6615452451652));
#190665=CARTESIAN_POINT('Ctrl Pts',(6.74287786815361,-0.570865181250576,
30.6702951593427));
#190666=CARTESIAN_POINT('Ctrl Pts',(6.75856988190868,-0.385516108070075,
30.6790449014472));
#190667=CARTESIAN_POINT('Ctrl Pts',(6.76661520773414,-0.19951979522253,
30.6877946435517));
#190668=CARTESIAN_POINT('Ctrl Pts',(6.7669865178958,-0.0135080204518887,
30.6965443856561));
#190669=CARTESIAN_POINT('Ctrl Pts',(6.76735782124893,0.172500343516661,
30.7052939673211));
#190670=CARTESIAN_POINT('Ctrl Pts',(6.76005538995164,0.358523882214559,
30.7140435489861));
#190671=CARTESIAN_POINT('Ctrl Pts',(6.74510402742332,0.543930748567948,
30.722793130651));
#190672=CARTESIAN_POINT('Ctrl Pts',(6.73015291917992,0.729334461618776,
30.7315425635077));
#190673=CARTESIAN_POINT('Ctrl Pts',(6.70755316306547,0.914121237638186,
30.7402919963644));
#190674=CARTESIAN_POINT('Ctrl Pts',(6.67738151874517,1.09766345166468,30.7490414292211));
#190675=CARTESIAN_POINT('Ctrl Pts',(6.64721034747502,1.28120278800011,30.7577907248986));
#190676=CARTESIAN_POINT('Ctrl Pts',(6.60946757205065,1.46349731860674,30.7665400205761));
#190677=CARTESIAN_POINT('Ctrl Pts',(6.56428138111437,1.64392790278506,30.7752893162537));
#190678=CARTESIAN_POINT('Ctrl Pts',(6.51909583859753,1.82435589779401,30.7840384863793));
#190679=CARTESIAN_POINT('Ctrl Pts',(6.46646716392768,2.00291972192611,30.7927876565049));
#190680=CARTESIAN_POINT('Ctrl Pts',(6.40657409872766,2.1790129227501,30.8015368266305));
#190681=CARTESIAN_POINT('Ctrl Pts',(6.34668181341948,2.35510383059322,30.8102858828296));
#190682=CARTESIAN_POINT('Ctrl Pts',(6.27952541913912,2.52872390822924,30.8190349390287));
#190683=CARTESIAN_POINT('Ctrl Pts',(6.20533299175368,2.69928350890627,30.8277839952278));
#190684=CARTESIAN_POINT('Ctrl Pts',(6.12831602991395,2.8763363796595,30.836866131386));
#190685=CARTESIAN_POINT('Ctrl Pts',(6.04371690605112,3.05009086601774,30.8459482675442));
#190686=CARTESIAN_POINT('Ctrl Pts',(5.9518452031647,3.21991112883033,30.8550304037024));
#190687=CARTESIAN_POINT('Ctrl Pts',(5.86333549509103,3.38351691183315,30.8637801840459));
#190688=CARTESIAN_POINT('Ctrl Pts',(5.76807618099186,3.54347103712301,30.8725299643895));
#190689=CARTESIAN_POINT('Ctrl Pts',(5.66639083308823,3.6992301802799,30.8812797447331));
#190690=CARTESIAN_POINT('Ctrl Pts',(5.56470914081996,3.85498372382346,30.890029210518));
#190691=CARTESIAN_POINT('Ctrl Pts',(5.4566020337185,4.00654234702293,30.8987786763029));
#190692=CARTESIAN_POINT('Ctrl Pts',(5.34243669838987,4.15339127986964,30.9075281420878));
#190693=CARTESIAN_POINT('Ctrl Pts',(5.22827486050352,4.30023571401571,30.9162773398338));
#190694=CARTESIAN_POINT('Ctrl Pts',(5.10805534166861,4.44237052028758,30.9250265375798));
#190695=CARTESIAN_POINT('Ctrl Pts',(4.9821864433969,4.57931296629005,30.9337757353259));
#190696=CARTESIAN_POINT('Ctrl Pts',(4.85632073219319,4.71625194483636,30.9425247115375));
#190697=CARTESIAN_POINT('Ctrl Pts',(4.72480612170045,4.84799861524775,30.9512736877491));
#190698=CARTESIAN_POINT('Ctrl Pts',(4.58808925235032,4.97410554898743,30.9600226639608));
#190699=CARTESIAN_POINT('Ctrl Pts',(4.45136349473761,5.10022068121457,30.9687722089625));
#190700=CARTESIAN_POINT('Ctrl Pts',(4.30943501209786,5.22069514872076,30.9775217539642));
#190701=CARTESIAN_POINT('Ctrl Pts',(4.16278587431482,5.33511975166491,30.9862712989659));
#190702=CARTESIAN_POINT('Ctrl Pts',(4.01614535740143,5.44953762808067,30.9950203296196));
#190703=CARTESIAN_POINT('Ctrl Pts',(3.86478496657614,5.55790617532999,31.0037693602733));
#190704=CARTESIAN_POINT('Ctrl Pts',(3.70921874746882,5.65985735539561,31.0125183909271));
#190705=CARTESIAN_POINT('Ctrl Pts',(3.55365041605579,5.76180991977244,31.0212675403767));
#190706=CARTESIAN_POINT('Ctrl Pts',(3.39387638174194,5.85734478553003,31.0300166898263));
#190707=CARTESIAN_POINT('Ctrl Pts',(3.23043927904203,5.94613749121414,31.0387658392759));
#190708=CARTESIAN_POINT('Ctrl Pts',(3.18691767070203,5.96978206944267,31.041095647192));
#190709=CARTESIAN_POINT('Ctrl Pts',(3.14313645919513,5.99294880633486,31.0434254551081));
#190710=CARTESIAN_POINT('Ctrl Pts',(3.09910619832133,6.01563211736941,31.0457552630242));
#190711=CARTESIAN_POINT('Ctrl Pts',(3.09910619832131,6.01563211736941,29.0458282148631));
#190712=CARTESIAN_POINT('Ctrl Pts',(2.93964010377536,6.09778514009208,29.054256760126));
#190713=CARTESIAN_POINT('Ctrl Pts',(2.77683871929303,6.17362780397065,29.0626853053889));
#190714=CARTESIAN_POINT('Ctrl Pts',(2.6112299438694,6.24289733859526,29.0711138506517));
#190715=CARTESIAN_POINT('Ctrl Pts',(2.44567997482292,6.31214227615147,29.0795394030043));
#190716=CARTESIAN_POINT('Ctrl Pts',(2.27732490764698,6.37481860978555,29.0879649553568));
#190717=CARTESIAN_POINT('Ctrl Pts',(2.10671402246393,6.43071108257507,29.0963905077094));
#190718=CARTESIAN_POINT('Ctrl Pts',(1.97260408037893,6.47464577220961,29.1030134751527));
#190719=CARTESIAN_POINT('Ctrl Pts',(1.83710078387265,6.51438972229086,29.1096364425959));
#190720=CARTESIAN_POINT('Ctrl Pts',(1.70047857745579,6.54985966319996,29.1162594100392));
#190721=CARTESIAN_POINT('Ctrl Pts',(1.52268563519071,6.59601837576647,29.1248781909764));
#190722=CARTESIAN_POINT('Ctrl Pts',(1.34307708786584,6.63491687714489,29.1334969719136));
#190723=CARTESIAN_POINT('Ctrl Pts',(1.16225888109226,6.66644157653258,29.1421157528508));
#190724=CARTESIAN_POINT('Ctrl Pts',(0.981332057920183,6.6979852126157,29.1507397110374));
#190725=CARTESIAN_POINT('Ctrl Pts',(0.799194424809612,6.72214615473156,
29.1593636692239));
#190726=CARTESIAN_POINT('Ctrl Pts',(0.61645904406323,6.73886245942093,29.1679876274105));
#190727=CARTESIAN_POINT('Ctrl Pts',(0.427122057498962,6.75618266716312,
29.1769231397816));
#190728=CARTESIAN_POINT('Ctrl Pts',(0.237143689164434,6.76551028319707,
29.1858586521527));
#190729=CARTESIAN_POINT('Ctrl Pts',(0.0472074746267504,6.76683533524641,
29.1947941645239));
#190730=CARTESIAN_POINT('Ctrl Pts',(-0.136448971720794,6.76811657774773,
29.2034342464186));
#190731=CARTESIAN_POINT('Ctrl Pts',(-0.320065704186172,6.7619160130467,
29.2120743283132));
#190732=CARTESIAN_POINT('Ctrl Pts',(-0.503028046335158,6.74827769024069,
29.2207144102079));
#190733=CARTESIAN_POINT('Ctrl Pts',(-0.695374440493255,6.73393986430729,
29.2297976378173));
#190734=CARTESIAN_POINT('Ctrl Pts',(-0.886997163713638,6.71138132769076,
29.2388808654266));
#190735=CARTESIAN_POINT('Ctrl Pts',(-1.07719139734627,6.68071460949225,
29.2479640930359));
#190736=CARTESIAN_POINT('Ctrl Pts',(-1.26738563097888,6.65004789129375,
29.2570473206453));
#190737=CARTESIAN_POINT('Ctrl Pts',(-1.4561510019505,6.6112731025047,29.2661305482546));
#190738=CARTESIAN_POINT('Ctrl Pts',(-1.6427978920141,6.56456427236371,29.2752137758639));
#190739=CARTESIAN_POINT('Ctrl Pts',(-1.8286509362264,6.51805410404351,29.2842583707237));
#190740=CARTESIAN_POINT('Ctrl Pts',(-2.01257532509177,6.46363514011707,
29.2933029655835));
#190741=CARTESIAN_POINT('Ctrl Pts',(-2.19392264690429,6.40148361080464,
29.3023475604433));
#190742=CARTESIAN_POINT('Ctrl Pts',(-2.37510355400318,6.33938911530363,
29.3113838554636));
#190743=CARTESIAN_POINT('Ctrl Pts',(-2.55371189066327,6.26957629836902,
29.320420150484));
#190744=CARTESIAN_POINT('Ctrl Pts',(-2.7291150570561,6.19227098933418,29.3294564455043));
#190745=CARTESIAN_POINT('Ctrl Pts',(-2.90420783379178,6.11510247810556,
29.338476750092));
#190746=CARTESIAN_POINT('Ctrl Pts',(-3.07610654871627,6.0304680462325,29.3474970546796));
#190747=CARTESIAN_POINT('Ctrl Pts',(-3.24419935093474,5.93864122265309,
29.3565173592673));
#190748=CARTESIAN_POINT('Ctrl Pts',(-3.4120804729224,5.84693003711977,29.3655263045337));
#190749=CARTESIAN_POINT('Ctrl Pts',(-3.57616503885175,5.74804464908513,
29.3745352498));
#190750=CARTESIAN_POINT('Ctrl Pts',(-3.73586423127392,5.64230515352441,
29.3835441950664));
#190751=CARTESIAN_POINT('Ctrl Pts',(-3.89520078063752,5.53680576997366,
29.3925326829251));
#190752=CARTESIAN_POINT('Ctrl Pts',(-4.05017163604127,5.42448347752928,
29.4015211707839));
#190753=CARTESIAN_POINT('Ctrl Pts',(-4.20021589273682,5.30570216412503,
29.4105096586427));
#190754=CARTESIAN_POINT('Ctrl Pts',(-4.33185907747665,5.20148790942121,
29.418395819658));
#190755=CARTESIAN_POINT('Ctrl Pts',(-4.45971019984325,5.09230245030685,
29.4262819806734));
#190756=CARTESIAN_POINT('Ctrl Pts',(-4.5834076189865,4.97841978927214,29.4341681416887));
#190757=CARTESIAN_POINT('Ctrl Pts',(-4.71079586789761,4.86113914695132,
29.4422896065449));
#190758=CARTESIAN_POINT('Ctrl Pts',(-4.83372071066561,4.73892811148528,
29.4504110714011));
#190759=CARTESIAN_POINT('Ctrl Pts',(-4.95178464568388,4.61217061943391,
29.4585325362572));
#190760=CARTESIAN_POINT('Ctrl Pts',(-5.06984016100606,4.48542216705718,
29.4666534219335));
#190761=CARTESIAN_POINT('Ctrl Pts',(-5.18303520948358,4.35412817187285,
29.4747743076097));
#190762=CARTESIAN_POINT('Ctrl Pts',(-5.29101018304382,4.21870836191915,
29.4828951932859));
#190763=CARTESIAN_POINT('Ctrl Pts',(-5.39899806270143,4.08327236542524,
29.4910170496402));
#190764=CARTESIAN_POINT('Ctrl Pts',(-5.5017643976717,3.94370985924083,29.4991389059945));
#190765=CARTESIAN_POINT('Ctrl Pts',(-5.59899083141245,3.80047242718051,
29.5072607623488));
#190766=CARTESIAN_POINT('Ctrl Pts',(-5.69628820035554,3.65713049086313,
29.515388544309));
#190767=CARTESIAN_POINT('Ctrl Pts',(-5.78803738953845,3.51010857691508,
29.5235163262691));
#190768=CARTESIAN_POINT('Ctrl Pts',(-5.87396389752997,3.35988647583733,
29.5316441082293));
#190769=CARTESIAN_POINT('Ctrl Pts',(-5.95992540878718,3.20960317985896,
29.5397752011457));
#190770=CARTESIAN_POINT('Ctrl Pts',(-6.040059341546,3.05611742261582,29.5479062940622));
#190771=CARTESIAN_POINT('Ctrl Pts',(-6.11413801439777,2.8999319545286,29.5560373869786));
#190772=CARTESIAN_POINT('Ctrl Pts',(-6.18829754102527,2.74357601652982,
29.5641773546432));
#190773=CARTESIAN_POINT('Ctrl Pts',(-6.25638846331034,2.58451481853252,
29.5723173223077));
#190774=CARTESIAN_POINT('Ctrl Pts',(-6.31823165142553,2.4232700631429,29.5804572899723));
#190775=CARTESIAN_POINT('Ctrl Pts',(-6.35030620270938,2.33964156122346,
29.5846790291527));
#190776=CARTESIAN_POINT('Ctrl Pts',(-6.38070099002848,2.25542595378637,
29.5889007683331));
#190777=CARTESIAN_POINT('Ctrl Pts',(-6.40939637596837,2.17069737543572,
29.5931225075134));
#190778=CARTESIAN_POINT('Ctrl Pts',(-6.47710331149741,1.9707797857622,29.6030837264741));
#190779=CARTESIAN_POINT('Ctrl Pts',(-6.53544742714254,1.7677082918809,29.6130449454347));
#190780=CARTESIAN_POINT('Ctrl Pts',(-6.58419091130636,1.56228007843368,
29.6230061643953));
#190781=CARTESIAN_POINT('Ctrl Pts',(-6.63281384523588,1.35735992097974,
29.6329427477087));
#190782=CARTESIAN_POINT('Ctrl Pts',(-6.67188356067146,1.15009468543861,
29.6428793310221));
#190783=CARTESIAN_POINT('Ctrl Pts',(-6.70121328168156,0.941291428525053,
29.6528159143355));
#190784=CARTESIAN_POINT('Ctrl Pts',(-6.73033525608324,0.733967154941493,
29.6626821154083));
#190785=CARTESIAN_POINT('Ctrl Pts',(-6.74985470567611,0.525126579051215,
29.672548316481));
#190786=CARTESIAN_POINT('Ctrl Pts',(-6.75963765824527,0.315575235454933,
29.6824145175538));
#190787=CARTESIAN_POINT('Ctrl Pts',(-6.76451788513943,0.211040526173875,
29.6873362729725));
#190788=CARTESIAN_POINT('Ctrl Pts',(-6.76697593628995,0.106329183087804,
29.6922580283913));
#190789=CARTESIAN_POINT('Ctrl Pts',(-6.76699982416302,0.00154265278611927,
29.69717978381));
#190790=CARTESIAN_POINT('',(-6.76699936525298,-0.00293098375184019,29.3028202162149));
#190791=CARTESIAN_POINT('Ctrl Pts',(3.09910619832131,6.01563211736942,28.6513936431573));
#190792=CARTESIAN_POINT('Ctrl Pts',(3.01963936879232,6.05657147987517,28.6556182811778));
#190793=CARTESIAN_POINT('Ctrl Pts',(2.93938618624693,6.09592314957077,28.6598429191983));
#190794=CARTESIAN_POINT('Ctrl Pts',(2.85840996112926,6.13365971456821,28.6640675572189));
#190795=CARTESIAN_POINT('Ctrl Pts',(2.70079997522997,6.20710916801571,28.6722902810847));
#190796=CARTESIAN_POINT('Ctrl Pts',(2.54014742829101,6.27457755010999,28.6805130049506));
#190797=CARTESIAN_POINT('Ctrl Pts',(2.37694609925172,6.33580430894548,28.6887357288165));
#190798=CARTESIAN_POINT('Ctrl Pts',(2.2139175132905,6.39696626133089,28.6969497492077));
#190799=CARTESIAN_POINT('Ctrl Pts',(2.04834585048812,6.45189962125721,28.7051637695989));
#190800=CARTESIAN_POINT('Ctrl Pts',(1.88074787242205,6.5003904836848,28.7133777899902));
#190801=CARTESIAN_POINT('Ctrl Pts',(1.71329364220257,6.54883975577143,28.7215847652621));
#190802=CARTESIAN_POINT('Ctrl Pts',(1.54381690065292,6.59085743612007,28.7297917405341));
#190803=CARTESIAN_POINT('Ctrl Pts',(1.37285278805253,6.6262783085482,28.7379987158061));
#190804=CARTESIAN_POINT('Ctrl Pts',(1.20200099546234,6.66167591017001,28.7462002992591));
#190805=CARTESIAN_POINT('Ctrl Pts',(1.02966412823749,6.69048526410618,28.754401882712));
#190806=CARTESIAN_POINT('Ctrl Pts',(0.856390921950913,6.71259142126199,
28.762603466165));
#190807=CARTESIAN_POINT('Ctrl Pts',(0.683196781399244,6.73468749122891,
28.7708013071801));
#190808=CARTESIAN_POINT('Ctrl Pts',(0.509067508093343,6.75008641281681,
28.7789991481951));
#190809=CARTESIAN_POINT('Ctrl Pts',(0.334560516946642,6.75872460309639,
28.7871969892101));
#190810=CARTESIAN_POINT('Ctrl Pts',(0.160068925497279,6.76736203108264,
28.7953941067913));
#190811=CARTESIAN_POINT('Ctrl Pts',(-0.0147999598090707,6.76923988984333,
28.8035912243725));
#190812=CARTESIAN_POINT('Ctrl Pts',(-0.189484763044477,6.76434657040678,
28.8117883419536));
#190813=CARTESIAN_POINT('Ctrl Pts',(-0.364167622716883,6.75945330541386,
28.8199853683327));
#190814=CARTESIAN_POINT('Ctrl Pts',(-0.538666045676,6.74778902125161,28.8281823947118));
#190815=CARTESIAN_POINT('Ctrl Pts',(-0.712419940840349,6.7293942392977,
28.8363794210909));
#190816=CARTESIAN_POINT('Ctrl Pts',(-0.886203496528949,6.71099631727677,
28.844577846737));
#190817=CARTESIAN_POINT('Ctrl Pts',(-1.05924191436472,6.68586564624408,
28.8527762723832));
#190818=CARTESIAN_POINT('Ctrl Pts',(-1.23098144775283,6.65409450453541,
28.8609746980293));
#190819=CARTESIAN_POINT('Ctrl Pts',(-1.40278152559977,6.62231216233875,
28.86917601392));
#190820=CARTESIAN_POINT('Ctrl Pts',(-1.57328145421884,6.58388475138881,
28.8773773298106));
#190821=CARTESIAN_POINT('Ctrl Pts',(-1.74193882837407,6.53895543020464,
28.8855786457013));
#190822=CARTESIAN_POINT('Ctrl Pts',(-1.91078827504614,6.49397494204457,
28.8937893015179));
#190823=CARTESIAN_POINT('Ctrl Pts',(-2.07779062800259,6.44247784306836,
28.9019999573344));
#190824=CARTESIAN_POINT('Ctrl Pts',(-2.24241875863819,6.38465716471195,
28.910210613151));
#190825=CARTESIAN_POINT('Ctrl Pts',(-2.40714390064255,6.32680241403065,
28.9184261073082));
#190826=CARTESIAN_POINT('Ctrl Pts',(-2.56949169834462,6.26261678781179,
28.9266416014653));
#190827=CARTESIAN_POINT('Ctrl Pts',(-2.72895621360771,6.1923409938578,28.9348570956225));
#190828=CARTESIAN_POINT('Ctrl Pts',(-2.88866814100077,6.12195616571626,
28.94308533627));
#190829=CARTESIAN_POINT('Ctrl Pts',(-3.04548752391195,6.04546244421245,
28.9513135769175));
#190830=CARTESIAN_POINT('Ctrl Pts',(-3.19893300132467,5.96314653962452,
28.959541817565));
#190831=CARTESIAN_POINT('Ctrl Pts',(-3.33839044255761,5.88833452417665,
28.9670199746661));
#190832=CARTESIAN_POINT('Ctrl Pts',(-3.47506124340677,5.80871410454857,
28.9744981317673));
#190833=CARTESIAN_POINT('Ctrl Pts',(-3.60860639176604,5.72453045317302,
28.9819762888684));
#190834=CARTESIAN_POINT('Ctrl Pts',(-3.75270835200911,5.63369204134993,
28.9900455980909));
#190835=CARTESIAN_POINT('Ctrl Pts',(-3.8936422053575,5.53724234215498,28.9981149073134));
#190836=CARTESIAN_POINT('Ctrl Pts',(-4.03092895988346,5.43543013204777,
29.006184216536));
#190837=CARTESIAN_POINT('Ctrl Pts',(-4.16804448051318,5.33374490943824,
29.0142434611367));
#190838=CARTESIAN_POINT('Ctrl Pts',(-4.30152165754444,5.22671070372065,
29.0223027057375));
#190839=CARTESIAN_POINT('Ctrl Pts',(-4.43090650081178,5.11462184145259,
29.0303619503382));
#190840=CARTESIAN_POINT('Ctrl Pts',(-4.56015835930497,5.00264818674407,
29.0384129114585));
#190841=CARTESIAN_POINT('Ctrl Pts',(-4.68532597480511,4.88563045647616,
29.0464638725788));
#190842=CARTESIAN_POINT('Ctrl Pts',(-4.80598483996478,4.7639058258984,29.054514833699));
#190843=CARTESIAN_POINT('Ctrl Pts',(-4.9265461278667,4.64227963446672,29.0625592839781));
#190844=CARTESIAN_POINT('Ctrl Pts',(-5.04260566130644,4.51595438255239,
29.0706037342572));
#190845=CARTESIAN_POINT('Ctrl Pts',(-5.15377259831527,4.38530694534085,
29.0786481845363));
#190846=CARTESIAN_POINT('Ctrl Pts',(-5.26487396762636,4.25473656567811,
29.0866878900946));
#190847=CARTESIAN_POINT('Ctrl Pts',(-5.37108824391054,4.11984935903987,
29.0947275956528));
#190848=CARTESIAN_POINT('Ctrl Pts',(-5.47206208945628,3.98105833782116,
29.102767301211));
#190849=CARTESIAN_POINT('Ctrl Pts',(-5.57521540147456,3.83927158661118,
29.1109805395155));
#190850=CARTESIAN_POINT('Ctrl Pts',(-5.67289920651918,3.69341086488444,
29.1191937778199));
#190851=CARTESIAN_POINT('Ctrl Pts',(-5.76478058652902,3.5439517193633,29.1274070161244));
#190852=CARTESIAN_POINT('Ctrl Pts',(-5.85469170614516,3.39769750431736,
29.1354441336726));
#190853=CARTESIAN_POINT('Ctrl Pts',(-5.93904653417511,3.24799796437482,
29.1434812512207));
#190854=CARTESIAN_POINT('Ctrl Pts',(-6.01757751986774,3.09532708972451,
29.1515183687689));
#190855=CARTESIAN_POINT('Ctrl Pts',(-6.09611681363938,2.94264006346631,
29.159556336593));
#190856=CARTESIAN_POINT('Ctrl Pts',(-6.16883086726497,2.786981408797,29.1675943044171));
#190857=CARTESIAN_POINT('Ctrl Pts',(-6.23549876428527,2.62884844762814,
29.1756322722413));
#190858=CARTESIAN_POINT('Ctrl Pts',(-6.30218692371324,2.4706674250284,29.183672683049));
#190859=CARTESIAN_POINT('Ctrl Pts',(-6.36282512373256,2.31001094312603,
29.1917130938567));
#190860=CARTESIAN_POINT('Ctrl Pts',(-6.41724119048436,2.14739481771537,
29.1997535046645));
#190861=CARTESIAN_POINT('Ctrl Pts',(-6.47371387764892,1.97863271993062,
29.2080977976523));
#190862=CARTESIAN_POINT('Ctrl Pts',(-6.52348477802392,1.80776038001368,
29.21644209064));
#190863=CARTESIAN_POINT('Ctrl Pts',(-6.56641898204299,1.63536869001015,
29.2247863836278));
#190864=CARTESIAN_POINT('Ctrl Pts',(-6.60786267041708,1.46896179737004,
29.2328409938434));
#190865=CARTESIAN_POINT('Ctrl Pts',(-6.64293638714389,1.30113965252255,
29.2408956040589));
#190866=CARTESIAN_POINT('Ctrl Pts',(-6.67157152402784,1.13244090343861,
29.2489502142744));
#190867=CARTESIAN_POINT('Ctrl Pts',(-6.70022833811489,0.963614447018662,
29.2570109219437));
#190868=CARTESIAN_POINT('Ctrl Pts',(-6.72243681932683,0.793910432895307,
29.2650716296129));
#190869=CARTESIAN_POINT('Ctrl Pts',(-6.73818039700338,0.623870128664149,
29.2731323372822));
#190870=CARTESIAN_POINT('Ctrl Pts',(-6.75394617218128,0.453590077790773,
29.2812044100664));
#190871=CARTESIAN_POINT('Ctrl Pts',(-6.76322883750484,0.282973160259584,
29.2892764828505));
#190872=CARTESIAN_POINT('Ctrl Pts',(-6.76606381392599,0.112558721924744,
29.2973485556347));
#190873=CARTESIAN_POINT('Ctrl Pts',(-6.76636075616661,0.0947091042783638,
29.2981940439291));
#190874=CARTESIAN_POINT('Ctrl Pts',(-6.76658700763728,0.0768617012250634,
29.2990395322235));
#190875=CARTESIAN_POINT('Ctrl Pts',(-6.76674264167672,0.0590171272931185,
29.2998850205179));
#190876=CARTESIAN_POINT('Ctrl Pts',(-6.7669227412957,0.0383673968275339,
29.3008634190753));
#190877=CARTESIAN_POINT('Ctrl Pts',(-6.76700830886146,0.0177178525793984,
29.3018418176326));
#190878=CARTESIAN_POINT('Ctrl Pts',(-6.76699936525321,-0.00293098322481845,
29.3028202161899));
#190879=CARTESIAN_POINT('Ctrl Pts',(-6.76699936525298,-0.00293098375180045,
29.3028202162149));
#190880=CARTESIAN_POINT('Ctrl Pts',(-6.76692334343068,-0.17844871664729,
29.3111367285007));
#190881=CARTESIAN_POINT('Ctrl Pts',(-6.76001423110666,-0.35419545525724,
29.3194532407865));
#190882=CARTESIAN_POINT('Ctrl Pts',(-6.74624402573338,-0.52960414014304,
29.3277697530723));
#190883=CARTESIAN_POINT('Ctrl Pts',(-6.73249024537216,-0.704803598682164,
29.3360763454759));
#190884=CARTESIAN_POINT('Ctrl Pts',(-6.71189170086085,-0.879665461091391,
29.3443829378796));
#190885=CARTESIAN_POINT('Ctrl Pts',(-6.6844723585507,-1.05362151068196,
29.3526895302832));
#190886=CARTESIAN_POINT('Ctrl Pts',(-6.65708060167097,-1.22740255051303,
29.3609877657787));
#190887=CARTESIAN_POINT('Ctrl Pts',(-6.62288177172376,-1.40027924971875,
29.3692860012741));
#190888=CARTESIAN_POINT('Ctrl Pts',(-6.58195172285144,-1.57168715654644,
29.3775842367696));
#190889=CARTESIAN_POINT('Ctrl Pts',(-6.54105521325882,-1.74295460671968,
29.385875672448));
#190890=CARTESIAN_POINT('Ctrl Pts',(-6.49343855552541,-1.91275532387974,
29.3941671081265));
#190891=CARTESIAN_POINT('Ctrl Pts',(-6.43922893693435,-2.08053351276717,
29.4024585438049));
#190892=CARTESIAN_POINT('Ctrl Pts',(-6.38505362700411,-2.2482055167169,
29.4107447319266));
#190893=CARTESIAN_POINT('Ctrl Pts',(-6.32429377847391,-2.41385721133037,
29.4190309200482));
#190894=CARTESIAN_POINT('Ctrl Pts',(-6.25712688900796,-2.57694627317947,
29.4273171081698));
#190895=CARTESIAN_POINT('Ctrl Pts',(-6.18998725095775,-2.73996916540451,
29.4355999343618));
#190896=CARTESIAN_POINT('Ctrl Pts',(-6.11644588430375,-2.90043117357467,
29.4438827605538));
#190897=CARTESIAN_POINT('Ctrl Pts',(-6.03672914460988,-3.05780807681216,
29.4521655867458));
#190898=CARTESIAN_POINT('Ctrl Pts',(-5.95702895048088,-3.21515231577145,
29.4604466938002));
#190899=CARTESIAN_POINT('Ctrl Pts',(-5.87115609458469,-3.36941241358713,
29.4687278008547));
#190900=CARTESIAN_POINT('Ctrl Pts',(-5.77938388808665,-3.52008677082319,
29.4770089079091));
#190901=CARTESIAN_POINT('Ctrl Pts',(-5.68761521411714,-3.67075532824812,
29.4852896962043));
#190902=CARTESIAN_POINT('Ctrl Pts',(-5.58994782412242,-3.81783812156665,
29.4935704844994));
#190903=CARTESIAN_POINT('Ctrl Pts',(-5.48669963192837,-3.9608605313741,
29.5018512727945));
#190904=CARTESIAN_POINT('Ctrl Pts',(-5.38343795931271,-4.10390161465509,
29.5101331422564));
#190905=CARTESIAN_POINT('Ctrl Pts',(-5.27459423789114,-4.24288097498686,
29.5184150117184));
#190906=CARTESIAN_POINT('Ctrl Pts',(-5.16052821794216,-4.37735508176144,
29.5266968811803));
#190907=CARTESIAN_POINT('Ctrl Pts',(-5.04638099100757,-4.51192492464446,
29.5349846467509));
#190908=CARTESIAN_POINT('Ctrl Pts',(-4.92700426361538,-4.64198283850877,
29.5432724123216));
#190909=CARTESIAN_POINT('Ctrl Pts',(-4.80279697001287,-4.76711970322072,
29.5515601778922));
#190910=CARTESIAN_POINT('Ctrl Pts',(-4.67854263339442,-4.89230396301996,
29.559851082421));
#190911=CARTESIAN_POINT('Ctrl Pts',(-4.54945433598132,-5.01256321634397,
29.5681419869497));
#190912=CARTESIAN_POINT('Ctrl Pts',(-4.4159661242158,-5.12752690775763,
29.5764328914784));
#190913=CARTESIAN_POINT('Ctrl Pts',(-4.28233650304424,-5.24261238481141,
29.5847325788942));
#190914=CARTESIAN_POINT('Ctrl Pts',(-4.14429792605753,-5.3523908706024,
29.5930322663099));
#190915=CARTESIAN_POINT('Ctrl Pts',(-4.00231641433118,-5.45653299445493,
29.6013319537257));
#190916=CARTESIAN_POINT('Ctrl Pts',(-3.90844657275726,-5.52538565384941,
29.6068192198729));
#190917=CARTESIAN_POINT('Ctrl Pts',(-3.81285386559171,-5.59177549299337,
29.6123064860202));
#190918=CARTESIAN_POINT('Ctrl Pts',(-3.71567934690656,-5.65561809097573,
29.6177937521674));
#190919=CARTESIAN_POINT('Ctrl Pts',(-3.56603273347159,-5.75393428240353,
29.6262440208908));
#190920=CARTESIAN_POINT('Ctrl Pts',(-3.41235457220222,-5.84639088124095,
29.6346942896141));
#190921=CARTESIAN_POINT('Ctrl Pts',(-3.25513079771634,-5.93265644460882,
29.6431445583375));
#190922=CARTESIAN_POINT('Ctrl Pts',(-3.09804577854547,-6.01884587569035,
29.651587369412));
#190923=CARTESIAN_POINT('Ctrl Pts',(-2.93742167241164,-6.09885500288081,
29.6600301804865));
#190924=CARTESIAN_POINT('Ctrl Pts',(-2.7737723342264,-6.17239629624348,
29.668472991561));
#190925=CARTESIAN_POINT('Ctrl Pts',(-2.6102451408566,-6.24588269975566,
29.6769095010787));
#190926=CARTESIAN_POINT('Ctrl Pts',(-2.44369751804175,-6.31291075726125,
29.6853460105964));
#190927=CARTESIAN_POINT('Ctrl Pts',(-2.27466715476121,-6.37323923409835,
29.6937825201141));
#190928=CARTESIAN_POINT('Ctrl Pts',(-2.10575774180036,-6.43352454266427,
29.7022129928554));
#190929=CARTESIAN_POINT('Ctrl Pts',(-1.93436944348861,-6.48711972159933,
29.7106434655966));
#190930=CARTESIAN_POINT('Ctrl Pts',(-1.76105931632406,-6.53383188369492,
29.7190739383378));
#190931=CARTESIAN_POINT('Ctrl Pts',(-1.58782369471363,-6.58052396435857,
29.7275007868416));
#190932=CARTESIAN_POINT('Ctrl Pts',(-1.41266821085646,-6.62033884089884,
29.7359276353455));
#190933=CARTESIAN_POINT('Ctrl Pts',(-1.23616508069522,-6.65313346426102,
29.7443544838493));
#190934=CARTESIAN_POINT('Ctrl Pts',(-1.05971643074671,-6.68591796509417,
29.7527787312859));
#190935=CARTESIAN_POINT('Ctrl Pts',(-0.881921289659919,-6.7116864735628,
29.7612029787226));
#190936=CARTESIAN_POINT('Ctrl Pts',(-0.703362429461534,-6.73034696674859,
29.7696272261592));
#190937=CARTESIAN_POINT('Ctrl Pts',(-0.653051374424555,-6.73560477976691,
29.7720008567702));
#190938=CARTESIAN_POINT('Ctrl Pts',(-0.602679739026944,-6.74029860317789,
29.7743744873812));
#190939=CARTESIAN_POINT('Ctrl Pts',(-0.552260663323196,-6.74442711872149,
29.7767481179922));
#190940=CARTESIAN_POINT('Ctrl Pts',(-0.36918627654349,-6.75941798162218,
29.7853668989294));
#190941=CARTESIAN_POINT('Ctrl Pts',(-0.185568004040187,-6.76694484582585,
29.7939856798667));
#190942=CARTESIAN_POINT('Ctrl Pts',(-0.00202229430074478,-6.7669996978222,
29.8026044608039));
#190943=CARTESIAN_POINT('Ctrl Pts',(0.181633670230526,-6.76705458276781,
29.8112284189904));
#190944=CARTESIAN_POINT('Ctrl Pts',(0.365216680836257,-6.75962849794704,
29.819852377177));
#190945=CARTESIAN_POINT('Ctrl Pts',(0.548112133156137,-6.74476553258058,
29.8284763353635));
#190946=CARTESIAN_POINT('Ctrl Pts',(0.73761497413429,-6.72936561898745,
29.8374118477346));
#190947=CARTESIAN_POINT('Ctrl Pts',(0.926379292811044,-6.70598150364335,
29.8463473601057));
#190948=CARTESIAN_POINT('Ctrl Pts',(1.11372996614274,-6.67472056063141,
29.8552828724768));
#190949=CARTESIAN_POINT('Ctrl Pts',(1.29488635576899,-6.64449318289294,
29.8639229543715));
#190950=CARTESIAN_POINT('Ctrl Pts',(1.47472079254162,-6.60690160412118,
29.8725630362662));
#190951=CARTESIAN_POINT('Ctrl Pts',(1.65263525530527,-6.56209461322542,
29.8812031181609));
#190952=CARTESIAN_POINT('Ctrl Pts',(1.83967486673138,-6.51498949295507,
29.8902863457703));
#190953=CARTESIAN_POINT('Ctrl Pts',(2.02459200481753,-6.45990948142009,
29.8993695733796));
#190954=CARTESIAN_POINT('Ctrl Pts',(2.20671158264246,-6.39708628916569,
29.9084528009889));
#190955=CARTESIAN_POINT('Ctrl Pts',(2.3888311604674,-6.33426309691129,29.9175360285983));
#190956=CARTESIAN_POINT('Ctrl Pts',(2.56815282951321,-6.2636968972522,29.9266192562076));
#190957=CARTESIAN_POINT('Ctrl Pts',(2.74402702294552,-6.18567738387194,
29.9357024838169));
#190958=CARTESIAN_POINT('Ctrl Pts',(2.91915318891973,-6.10798970279257,
29.9447470786767));
#190959=CARTESIAN_POINT('Ctrl Pts',(3.09102322236968,-6.02284103247761,
29.9537916735366));
#190960=CARTESIAN_POINT('Ctrl Pts',(3.25902853016055,-5.93051616974438,
29.9628362683964));
#190961=CARTESIAN_POINT('Ctrl Pts',(3.42687966663643,-5.83827602960522,
29.9718725634168));
#190962=CARTESIAN_POINT('Ctrl Pts',(3.5908729497389,-5.7388729590765,29.9809088584371));
#190963=CARTESIAN_POINT('Ctrl Pts',(3.75042386829534,-5.63263790848663,
29.9899451534575));
#190964=CARTESIAN_POINT('Ctrl Pts',(3.90969244898952,-5.52659084914966,
29.9989654580452));
#190965=CARTESIAN_POINT('Ctrl Pts',(4.06453416501961,-5.41373608306452,
30.0079857626329));
#190966=CARTESIAN_POINT('Ctrl Pts',(4.21439312543053,-5.29444799618656,
30.0170060672206));
#190967=CARTESIAN_POINT('Ctrl Pts',(4.36406336759178,-5.17531012948162,
30.0260150124869));
#190968=CARTESIAN_POINT('Ctrl Pts',(4.50876319093296,-5.04975525754166,
30.0350239577532));
#190969=CARTESIAN_POINT('Ctrl Pts',(4.64796738103697,-4.91819969346674,
30.0440329030196));
#190970=CARTESIAN_POINT('Ctrl Pts',(4.78685546789453,-4.78694286422776,
30.0530213908784));
#190971=CARTESIAN_POINT('Ctrl Pts',(4.92027265893366,-4.64971270522507,
30.0620098787372));
#190972=CARTESIAN_POINT('Ctrl Pts',(5.0477287478029,-4.50696388809631,30.070998366596));
#190973=CARTESIAN_POINT('Ctrl Pts',(5.15955392407119,-4.38172144751043,
30.0788845276112));
#190974=CARTESIAN_POINT('Ctrl Pts',(5.26679083365828,-4.25223160546079,
30.0867706886265));
#190975=CARTESIAN_POINT('Ctrl Pts',(5.36913017152967,-4.11882631354732,
30.0946568496417));
#190976=CARTESIAN_POINT('Ctrl Pts',(5.47452306603439,-3.98144053258129,
30.1027783144979));
#190977=CARTESIAN_POINT('Ctrl Pts',(5.5746732893869,-3.83996266533143,30.110899779354));
#190978=CARTESIAN_POINT('Ctrl Pts',(5.66925505609524,-3.69483911814013,
30.1190212442102));
#190979=CARTESIAN_POINT('Ctrl Pts',(5.76383007773165,-3.54972592039354,
30.1271421298864));
#190980=CARTESIAN_POINT('Ctrl Pts',(5.85283723377556,-3.40096786735389,
30.1352630155626));
#190981=CARTESIAN_POINT('Ctrl Pts',(5.93599420789973,-3.24904012960457,
30.1433839012388));
#190982=CARTESIAN_POINT('Ctrl Pts',(6.01916112166023,-3.09709423214613,
30.1515057575931));
#190983=CARTESIAN_POINT('Ctrl Pts',(6.09647628634571,-2.94197821735398,
30.1596276139474));
#190984=CARTESIAN_POINT('Ctrl Pts',(6.16770348824845,-2.78419156687322,
30.1677494703016));
#190985=CARTESIAN_POINT('Ctrl Pts',(6.23898265663644,-2.62628979720448,
30.1758772522618));
#190986=CARTESIAN_POINT('Ctrl Pts',(6.30416484013487,-2.46571383433586,
30.184005034222));
#190987=CARTESIAN_POINT('Ctrl Pts',(6.36306186700887,-2.30298342951433,
30.1921328161821));
#190988=CARTESIAN_POINT('Ctrl Pts',(6.42198288634252,-2.14018673437428,
30.2002639090986));
#190989=CARTESIAN_POINT('Ctrl Pts',(6.47461353434605,-1.97523419651346,
30.208395002015));
#190990=CARTESIAN_POINT('Ctrl Pts',(6.52081570265401,-1.80866015935027,
30.2165260949315));
#190991=CARTESIAN_POINT('Ctrl Pts',(6.56706829869779,-1.64190431358699,
30.224666062596));
#190992=CARTESIAN_POINT('Ctrl Pts',(6.60687831677082,-1.47352378957396,
30.2328060302606));
#190993=CARTESIAN_POINT('Ctrl Pts',(6.64015873062925,-1.30406327762429,
30.2409459979251));
#190994=CARTESIAN_POINT('Ctrl Pts',(6.65741939220892,-1.21617372912516,
30.2451677371056));
#190995=CARTESIAN_POINT('Ctrl Pts',(6.67292450033912,-1.12799378098362,
30.249389476286));
#190996=CARTESIAN_POINT('Ctrl Pts',(6.68666741949639,-1.0395998369784,30.2536112154665));
#190997=CARTESIAN_POINT('Ctrl Pts',(6.71414261663411,-0.862880392620828,
30.2620514249241));
#190998=CARTESIAN_POINT('Ctrl Pts',(6.73462821456756,-0.684940126377725,
30.2704916343817));
#190999=CARTESIAN_POINT('Ctrl Pts',(6.74802864739416,-0.506357950414263,
30.2789318438393));
#191000=CARTESIAN_POINT('Ctrl Pts',(6.76141892740761,-0.327911076906168,
30.2873656585879));
#191001=CARTESIAN_POINT('Ctrl Pts',(6.76773471832173,-0.148823594521152,
30.2957994733364));
#191002=CARTESIAN_POINT('Ctrl Pts',(6.76693207915634,0.0303189063932844,
30.3042332880849));
#191003=CARTESIAN_POINT('Ctrl Pts',(6.7661299247218,0.209353219343611,30.3126620094735));
#191004=CARTESIAN_POINT('Ctrl Pts',(6.75821791231362,0.3884421519357,30.321090730862));
#191005=CARTESIAN_POINT('Ctrl Pts',(6.74320414226847,0.566998144347376,
30.3295194522506));
#191006=CARTESIAN_POINT('Ctrl Pts',(6.7281971338744,0.745473721692369,30.3379443776523));
#191007=CARTESIAN_POINT('Ctrl Pts',(6.70609477293042,0.923416505664779,
30.346369303054));
#191008=CARTESIAN_POINT('Ctrl Pts',(6.67695718231888,1.10024169412013,30.3547942284558));
#191009=CARTESIAN_POINT('Ctrl Pts',(6.64782824363899,1.27701437722366,30.3632166522135));
#191010=CARTESIAN_POINT('Ctrl Pts',(6.61166829537166,1.45266979789972,30.3716390759712));
#191011=CARTESIAN_POINT('Ctrl Pts',(6.56858902929615,1.62663061701489,30.3800614997289));
#191012=CARTESIAN_POINT('Ctrl Pts',(6.52550908570783,1.80059417203284,30.3884840559471));
#191013=CARTESIAN_POINT('Ctrl Pts',(6.47550968056998,1.97286274701657,30.3969066121654));
#191014=CARTESIAN_POINT('Ctrl Pts',(6.41875327162557,2.14287084025054,30.4053291683836));
#191015=CARTESIAN_POINT('Ctrl Pts',(6.36199494543892,2.31288467639009,30.4137520091173));
#191016=CARTESIAN_POINT('Ctrl Pts',(6.29847926580235,2.48063756206188,30.4221748498511));
#191017=CARTESIAN_POINT('Ctrl Pts',(6.22841811407609,2.64558061609335,30.4305976905848));
#191018=CARTESIAN_POINT('Ctrl Pts',(6.15834481435909,2.81055226980729,30.4390219917654));
#191019=CARTESIAN_POINT('Ctrl Pts',(6.08172391024639,2.97271281353646,30.4474462929461));
#191020=CARTESIAN_POINT('Ctrl Pts',(5.99881498229965,3.13153441752397,30.4558705941267));
#191021=CARTESIAN_POINT('Ctrl Pts',(5.91588010011969,3.2904057398356,30.4642975324935));
#191022=CARTESIAN_POINT('Ctrl Pts',(5.82665342388158,3.4459357429023,30.4727244708603));
#191023=CARTESIAN_POINT('Ctrl Pts',(5.73144010436975,3.59762189925819,30.4811514092271));
#191024=CARTESIAN_POINT('Ctrl Pts',(5.63614117611542,3.74944444053551,30.4895859244708));
#191025=CARTESIAN_POINT('Ctrl Pts',(5.53484502651753,3.89741594647505,30.4980204397144));
#191026=CARTESIAN_POINT('Ctrl Pts',(5.4279003371413,4.04106259912679,30.5064549549581));
#191027=CARTESIAN_POINT('Ctrl Pts',(5.32090399256389,4.1847786343424,30.5148935441448));
#191028=CARTESIAN_POINT('Ctrl Pts',(5.20825387249812,4.324165387617,30.5233321333316));
#191029=CARTESIAN_POINT('Ctrl Pts',(5.09033877550769,4.45878236187447,30.5317707225184));
#191030=CARTESIAN_POINT('Ctrl Pts',(4.97229187611655,4.59354980745272,30.5402187441387));
#191031=CARTESIAN_POINT('Ctrl Pts',(4.84896846634489,4.72353657520099,30.548666765759));
#191032=CARTESIAN_POINT('Ctrl Pts',(4.72079484984724,4.84833837367564,30.5571147873793));
#191033=CARTESIAN_POINT('Ctrl Pts',(4.64794302320433,4.91927371306638,30.5619165072915));
#191034=CARTESIAN_POINT('Ctrl Pts',(4.57352492750606,4.98853470115086,30.5667182272037));
#191035=CARTESIAN_POINT('Ctrl Pts',(4.49762357029666,5.05605292890728,30.571519947116));
#191036=CARTESIAN_POINT('Ctrl Pts',(4.36738098180202,5.17191052456671,30.5797594365478));
#191037=CARTESIAN_POINT('Ctrl Pts',(4.23247839139077,5.28289290409624,30.5879989259797));
#191038=CARTESIAN_POINT('Ctrl Pts',(4.09331426468497,5.38860532332129,30.5962384154116));
#191039=CARTESIAN_POINT('Ctrl Pts',(3.95429111441627,5.49421065345253,30.6044695580527));
#191040=CARTESIAN_POINT('Ctrl Pts',(3.81101530141311,5.59455643582094,30.6127007006937));
#191041=CARTESIAN_POINT('Ctrl Pts',(3.66392106719515,5.68928566811015,30.6209318433347));
#191042=CARTESIAN_POINT('Ctrl Pts',(3.5169829921805,5.78391433329337,30.6291542475728));
#191043=CARTESIAN_POINT('Ctrl Pts',(3.36623487045386,5.87293813722831,30.637376651811));
#191044=CARTESIAN_POINT('Ctrl Pts',(3.21214262503794,5.95604136624439,30.6455990560492));
#191045=CARTESIAN_POINT('Ctrl Pts',(3.17465922751093,5.97625647415317,30.6475991803634));
#191046=CARTESIAN_POINT('Ctrl Pts',(3.13697809406508,5.99612144508233,30.6495993046776));
#191047=CARTESIAN_POINT('Ctrl Pts',(3.09910619832131,6.01563211736941,30.6515994289918));
#191048=CARTESIAN_POINT('Origin',(0.,0.,4.30282021618968));
#191049=CARTESIAN_POINT('',(3.09910619832137,6.01563211736938,33.0454119479742));
#191050=CARTESIAN_POINT('',(3.09910619832135,6.0156321173694,32.6513224177368));
#191051=CARTESIAN_POINT('',(3.09910619832133,6.0156321173694,4.30282021618968));
#191052=CARTESIAN_POINT('',(-6.7669999994793,-8.39470370789987E-5,31.6971797838101));
#191053=CARTESIAN_POINT('Ctrl Pts',(-6.7669999994793,-8.39470370789987E-5,
31.6971797838101));
#191054=CARTESIAN_POINT('Ctrl Pts',(-6.76699779048473,-0.178151771749838,
31.7055231531321));
#191055=CARTESIAN_POINT('Ctrl Pts',(-6.75996269808484,-0.356151551338823,
31.7138665224542));
#191056=CARTESIAN_POINT('Ctrl Pts',(-6.745936741221,-0.533503967599661,
31.7222098917762));
#191057=CARTESIAN_POINT('Ctrl Pts',(-6.73189495467664,-0.711056543615564,
31.7305626774163));
#191058=CARTESIAN_POINT('Ctrl Pts',(-6.71084656433386,-0.887959956551547,
31.7389154630564));
#191059=CARTESIAN_POINT('Ctrl Pts',(-6.68288543867111,-1.06364054717637,
31.7472682486965));
#191060=CARTESIAN_POINT('Ctrl Pts',(-6.65490792499826,-1.23942410415982,
31.7556259299026));
#191061=CARTESIAN_POINT('Ctrl Pts',(-6.62000965983928,-1.4139830754286,
31.7639836111087));
#191062=CARTESIAN_POINT('Ctrl Pts',(-6.57833536682154,-1.58675543220273,
31.7723412923148));
#191063=CARTESIAN_POINT('Ctrl Pts',(-6.53660132810523,-1.75977548136477,
31.7807109553798));
#191064=CARTESIAN_POINT('Ctrl Pts',(-6.48807193581272,-1.93100346826878,
31.7890806184449));
#191065=CARTESIAN_POINT('Ctrl Pts',(-6.43294181850615,-2.09989251146692,
31.7974502815099));
#191066=CARTESIAN_POINT('Ctrl Pts',(-6.38676031319846,-2.24136781799481,
31.80446139736));
#191067=CARTESIAN_POINT('Ctrl Pts',(-6.33594791712753,-2.38120208121305,
31.81147251321));
#191068=CARTESIAN_POINT('Ctrl Pts',(-6.28064456195365,-2.51908572430596,
31.8184836290601));
#191069=CARTESIAN_POINT('Ctrl Pts',(-6.21406858298535,-2.68507454168897,
31.8269238385177));
#191070=CARTESIAN_POINT('Ctrl Pts',(-6.1408589613978,-2.84854548522437,
31.8353640479753));
#191071=CARTESIAN_POINT('Ctrl Pts',(-6.06122901080011,-3.00895195685062,
31.8438042574329));
#191072=CARTESIAN_POINT('Ctrl Pts',(-5.98165939168721,-3.16923689681031,
31.8522380721815));
#191073=CARTESIAN_POINT('Ctrl Pts',(-5.89567928807107,-3.32646169556683,
31.86067188693));
#191074=CARTESIAN_POINT('Ctrl Pts',(-5.80354981563181,-3.48010036313322,
31.8691057016786));
#191075=CARTESIAN_POINT('Ctrl Pts',(-5.71147598213936,-3.63364624504236,
31.8775344230671));
#191076=CARTESIAN_POINT('Ctrl Pts',(-5.61326035475892,-3.78361002818852,
31.8859631444556));
#191077=CARTESIAN_POINT('Ctrl Pts',(-5.50920980585384,-3.92949059231397,
31.8943918658442));
#191078=CARTESIAN_POINT('Ctrl Pts',(-5.40520611749779,-4.07530545718649,
31.9028167912459));
#191079=CARTESIAN_POINT('Ctrl Pts',(-5.29537294054972,-4.21704049861424,
31.9112417166476));
#191080=CARTESIAN_POINT('Ctrl Pts',(-5.18006047504566,-4.35422352146393,
31.9196666420493));
#191081=CARTESIAN_POINT('Ctrl Pts',(-5.06478224969517,-4.49136581005519,
31.928089065807));
#191082=CARTESIAN_POINT('Ctrl Pts',(-4.94402819470515,-4.62395852054418,
31.9365114895647));
#191083=CARTESIAN_POINT('Ctrl Pts',(-4.81818904595063,-4.75156219758106,
31.9449339133224));
#191084=CARTESIAN_POINT('Ctrl Pts',(-4.69234791810826,-4.87916788145675,
31.9533564695406));
#191085=CARTESIAN_POINT('Ctrl Pts',(-4.56142176607839,-5.00178413305368,
31.9617790257588));
#191086=CARTESIAN_POINT('Ctrl Pts',(-4.42583893829837,-5.11900758860953,
31.970201581977));
#191087=CARTESIAN_POINT('Ctrl Pts',(-4.29025153050468,-5.23623500399597,
31.9786244227108));
#191088=CARTESIAN_POINT('Ctrl Pts',(-4.15000738554183,-5.34806904181338,
31.9870472634445));
#191089=CARTESIAN_POINT('Ctrl Pts',(-4.00556886865909,-5.45414585782496,
31.9954701041783));
#191090=CARTESIAN_POINT('Ctrl Pts',(-3.86110530740117,-5.56024106662839,
32.0038944053589));
#191091=CARTESIAN_POINT('Ctrl Pts',(-3.71244619311137,-5.66057686596334,
32.0123187065395));
#191092=CARTESIAN_POINT('Ctrl Pts',(-3.56008416335048,-5.75483186112862,
32.0207430077202));
#191093=CARTESIAN_POINT('Ctrl Pts',(-3.40767443740344,-5.84911636235786,
32.029169946087));
#191094=CARTESIAN_POINT('Ctrl Pts',(-3.25155976845531,-5.93731608880691,
32.0375968844538));
#191095=CARTESIAN_POINT('Ctrl Pts',(-3.09225906586156,-6.01915466403689,
32.0460238228206));
#191096=CARTESIAN_POINT('Ctrl Pts',(-2.93281513191226,-6.10106682243301,
32.0544583380643));
#191097=CARTESIAN_POINT('Ctrl Pts',(-2.77017973728863,-6.17660624862224,
32.0628928533079));
#191098=CARTESIAN_POINT('Ctrl Pts',(-2.60489457024093,-6.24554347338399,
32.0713273685516));
#191099=CARTESIAN_POINT('Ctrl Pts',(-2.43952956904178,-6.31451399541578,
32.0797659577384));
#191100=CARTESIAN_POINT('Ctrl Pts',(-2.27151255362936,-6.37687583527864,
32.0882045469251));
#191101=CARTESIAN_POINT('Ctrl Pts',(-2.1014027018023,-6.43244865388431,
32.0966431361119));
#191102=CARTESIAN_POINT('Ctrl Pts',(-1.93110270564717,-6.48808359032818,
32.1050911577322));
#191103=CARTESIAN_POINT('Ctrl Pts',(-1.75870551827341,-6.53691424640581,
32.1135391793525));
#191104=CARTESIAN_POINT('Ctrl Pts',(-1.58478408853412,-6.57881056063549,
32.1219872009728));
#191105=CARTESIAN_POINT('Ctrl Pts',(-1.48592993902001,-6.60262375327748,
32.1267889208851));
#191106=CARTESIAN_POINT('Ctrl Pts',(-1.38658355724041,-6.62419766959716,
32.1315906407974));
#191107=CARTESIAN_POINT('Ctrl Pts',(-1.28685124095519,-6.64351585259282,
32.1363923607096));
#191108=CARTESIAN_POINT('Ctrl Pts',(-1.1157151456392,-6.67666497145037,
32.1446318925605));
#191109=CARTESIAN_POINT('Ctrl Pts',(-0.943060246836166,-6.70324312969394,
32.1528714244113));
#191110=CARTESIAN_POINT('Ctrl Pts',(-0.769430690151189,-6.72311426446505,
32.1611109562621));
#191111=CARTESIAN_POINT('Ctrl Pts',(-0.595993850139201,-6.74296334366536,
32.1693413428085));
#191112=CARTESIAN_POINT('Ctrl Pts',(-0.42158485677799,-6.75612018218729,
32.1775717293548));
#191113=CARTESIAN_POINT('Ctrl Pts',(-0.246759193670351,-6.76249945658698,
32.1858021159011));
#191114=CARTESIAN_POINT('Ctrl Pts',(-0.0720963875388228,-6.76887278844185,
32.1940248355189));
#191115=CARTESIAN_POINT('Ctrl Pts',(0.102981961764185,-6.76848111684952,
32.2022475551367));
#191116=CARTESIAN_POINT('Ctrl Pts',(0.277913984123325,-6.7612907656326,
32.2104702747545));
#191117=CARTESIAN_POINT('Ctrl Pts',(0.45269100410728,-6.75410678558491,
32.2186857084503));
#191118=CARTESIAN_POINT('Ctrl Pts',(0.627321601313725,-6.74013614711203,
32.2269011421461));
#191119=CARTESIAN_POINT('Ctrl Pts',(0.801242761887947,-6.71939722270697,
32.2351165758419));
#191120=CARTESIAN_POINT('Ctrl Pts',(0.975074540490718,-6.69866895649867,
32.2433277874427));
#191121=CARTESIAN_POINT('Ctrl Pts',(1.1481972560462,-6.67117937388351,32.2515389990435));
#191122=CARTESIAN_POINT('Ctrl Pts',(1.32005145620136,-6.63699880616086,
32.2597502106443));
#191123=CARTESIAN_POINT('Ctrl Pts',(1.49184802594091,-6.6028297007145,32.2679586686578));
#191124=CARTESIAN_POINT('Ctrl Pts',(1.66237657899897,-6.56197414933219,
32.2761671266713));
#191125=CARTESIAN_POINT('Ctrl Pts',(1.83108622547783,-6.51455387842217,
32.2843755846849));
#191126=CARTESIAN_POINT('Ctrl Pts',(1.90625005689209,-6.49342711227282,
32.2880326319681));
#191127=CARTESIAN_POINT('Ctrl Pts',(1.98105299213458,-6.4709979944983,32.2916896792512));
#191128=CARTESIAN_POINT('Ctrl Pts',(2.05544710603844,-6.4472805270345,32.2953467265344));
#191129=CARTESIAN_POINT('Ctrl Pts',(2.23566434751522,-6.38982575895074,
32.3042058007103));
#191130=CARTESIAN_POINT('Ctrl Pts',(2.41329414565916,-6.32486711023106,
32.3130648748862));
#191131=CARTESIAN_POINT('Ctrl Pts',(2.58773979349527,-6.25267077025179,
32.3219239490621));
#191132=CARTESIAN_POINT('Ctrl Pts',(2.76251318960721,-6.18033878787476,
32.330799667656));
#191133=CARTESIAN_POINT('Ctrl Pts',(2.93409024044558,-6.10074203822208,
32.3396753862499));
#191134=CARTESIAN_POINT('Ctrl Pts',(3.10189748446334,-6.01419329552019,
32.3485511048438));
#191135=CARTESIAN_POINT('Ctrl Pts',(3.27018360294229,-5.92739756716062,
32.3574521522308));
#191136=CARTESIAN_POINT('Ctrl Pts',(3.4346781545769,-5.83361026468774,32.3663531996178));
#191137=CARTESIAN_POINT('Ctrl Pts',(3.59483275660182,-5.73318990197103,
32.3752542470048));
#191138=CARTESIAN_POINT('Ctrl Pts',(3.75520509100505,-5.63263301639373,
32.3841673954878));
#191139=CARTESIAN_POINT('Ctrl Pts',(3.91122547361042,-5.52542520029555,
32.3930805439708));
#191140=CARTESIAN_POINT('Ctrl Pts',(4.06237637333955,-5.41196703623855,
32.4019936924538));
#191141=CARTESIAN_POINT('Ctrl Pts',(4.21386286939723,-5.298256964033,32.4109266305637));
#191142=CARTESIAN_POINT('Ctrl Pts',(4.36045804925197,-5.17826894262874,
32.4198595686736));
#191143=CARTESIAN_POINT('Ctrl Pts',(4.50167700658102,-5.05244427266841,
32.4287925067834));
#191144=CARTESIAN_POINT('Ctrl Pts',(4.63609697806302,-4.93267743068279,
32.437295368642));
#191145=CARTESIAN_POINT('Ctrl Pts',(4.7656460821748,-4.80762284615651,32.4457982305006));
#191146=CARTESIAN_POINT('Ctrl Pts',(4.8899385936831,-4.67769062145077,32.4543010923592));
#191147=CARTESIAN_POINT('Ctrl Pts',(5.01013612455314,-4.55203918516906,
32.462523816225));
#191148=CARTESIAN_POINT('Ctrl Pts',(5.12564738476965,-4.42158470198206,
32.4707465400909));
#191149=CARTESIAN_POINT('Ctrl Pts',(5.23606697884529,-4.28671104613385,
32.4789692639568));
#191150=CARTESIAN_POINT('Ctrl Pts',(5.34636969752114,-4.15198014948142,
32.487183284348));
#191151=CARTESIAN_POINT('Ctrl Pts',(5.4515912566418,-4.01283966992172,32.4953973047392));
#191152=CARTESIAN_POINT('Ctrl Pts',(5.55136304920776,-3.86971023409902,
32.5036113251304));
#191153=CARTESIAN_POINT('Ctrl Pts',(5.65104926806641,-3.72670355959127,
32.5118183004024));
#191154=CARTESIAN_POINT('Ctrl Pts',(5.74529482553669,-3.5797150352594,32.5200252756744));
#191155=CARTESIAN_POINT('Ctrl Pts',(5.83377131614394,-3.42919833648277,
32.5282322509463));
#191156=CARTESIAN_POINT('Ctrl Pts',(5.92218967946257,-3.27878052417342,
32.5364338343993));
#191157=CARTESIAN_POINT('Ctrl Pts',(6.00484634433252,-3.12483946262162,
32.5446354178523));
#191158=CARTESIAN_POINT('Ctrl Pts',(6.08145613834093,-2.9678578533069,32.5528370013053));
#191159=CARTESIAN_POINT('Ctrl Pts',(6.15803097478276,-2.81094787576107,
32.5610348423204));
#191160=CARTESIAN_POINT('Ctrl Pts',(6.22856428041561,-2.65100043625445,
32.5692326833354));
#191161=CARTESIAN_POINT('Ctrl Pts',(6.29281673627029,-2.48852296025505,
32.5774305243505));
#191162=CARTESIAN_POINT('Ctrl Pts',(6.35706352204614,-2.32605982238614,
32.5856276419316));
#191163=CARTESIAN_POINT('Ctrl Pts',(6.41503042226882,-2.1610674229237,32.5938247595128));
#191164=CARTESIAN_POINT('Ctrl Pts',(6.46652606306023,-1.99407363850053,
32.6020218770939));
#191165=CARTESIAN_POINT('Ctrl Pts',(6.5180211309053,-1.82708171206919,32.610218903473));
#191166=CARTESIAN_POINT('Ctrl Pts',(6.56304497596077,-1.65808878761181,
32.6184159298521));
#191167=CARTESIAN_POINT('Ctrl Pts',(6.60145600313079,-1.48763827549859,
32.6266129562312));
#191168=CARTESIAN_POINT('Ctrl Pts',(6.63987358722549,-1.31715866676256,
32.6348113818773));
#191169=CARTESIAN_POINT('Ctrl Pts',(6.67167602557125,-1.14522132471924,
32.6430098075235));
#191170=CARTESIAN_POINT('Ctrl Pts',(6.69677277402005,-0.972380282165284,
32.6512082331696));
#191171=CARTESIAN_POINT('Ctrl Pts',(6.72187836998941,-0.799478306830294,
32.6594095490603));
#191172=CARTESIAN_POINT('Ctrl Pts',(6.74027351541787,-0.625672351247381,
32.6676108649509));
#191173=CARTESIAN_POINT('Ctrl Pts',(6.75191949241272,-0.451522057021841,
32.6758121808416));
#191174=CARTESIAN_POINT('Ctrl Pts',(6.76357873222588,-0.277173434762984,
32.6840228366582));
#191175=CARTESIAN_POINT('Ctrl Pts',(6.76847342403245,-0.102480048831869,
32.6922334924748));
#191176=CARTESIAN_POINT('Ctrl Pts',(6.76661698681875,0.0719969005999661,
32.7004441482914));
#191177=CARTESIAN_POINT('Ctrl Pts',(6.76475945565157,0.246576665070998,
32.7086596424485));
#191178=CARTESIAN_POINT('Ctrl Pts',(6.75614288306288,0.420939381007314,
32.7168751366057));
#191179=CARTESIAN_POINT('Ctrl Pts',(6.7408326450742,0.594528595697426,32.7250906307628));
#191180=CARTESIAN_POINT('Ctrl Pts',(6.72549865296955,0.768387137248436,
32.7333188714103));
#191181=CARTESIAN_POINT('Ctrl Pts',(6.70345028676967,0.941469423557725,
32.7415471120578));
#191182=CARTESIAN_POINT('Ctrl Pts',(6.67480438259898,1.1132274942874,32.7497753527053));
#191183=CARTESIAN_POINT('Ctrl Pts',(6.64876982905722,1.26932815922007,32.7572535098064));
#191184=CARTESIAN_POINT('Ctrl Pts',(6.6172864561182,1.42433498569818,32.7647316669076));
#191185=CARTESIAN_POINT('Ctrl Pts',(6.58047750411487,1.57784816057762,32.7722098240087));
#191186=CARTESIAN_POINT('Ctrl Pts',(6.54075442868357,1.74351480126009,32.7802800184165));
#191187=CARTESIAN_POINT('Ctrl Pts',(6.49469826418184,1.9079840842533,32.7883502128243));
#191188=CARTESIAN_POINT('Ctrl Pts',(6.4423907154619,2.07072230618457,32.7964204072321));
#191189=CARTESIAN_POINT('Ctrl Pts',(6.39014957552271,2.23325391841677,32.8044803558574));
#191190=CARTESIAN_POINT('Ctrl Pts',(6.33167295723089,2.39405849188848,32.8125403044826));
#191191=CARTESIAN_POINT('Ctrl Pts',(6.26709374653857,2.55261140248516,32.8206002531079));
#191192=CARTESIAN_POINT('Ctrl Pts',(6.20258234835552,2.71099782187504,32.8286517382456));
#191193=CARTESIAN_POINT('Ctrl Pts',(6.13198125093969,2.86713694125061,32.8367032233834));
#191194=CARTESIAN_POINT('Ctrl Pts',(6.05547339459548,3.02051832759649,32.8447547085212));
#191195=CARTESIAN_POINT('Ctrl Pts',(5.97602710307384,3.17979062871556,32.8531154268317));
#191196=CARTESIAN_POINT('Ctrl Pts',(5.89021140791942,3.33608876421771,32.8614761451422));
#191197=CARTESIAN_POINT('Ctrl Pts',(5.79828704848706,3.48886174895871,32.8698368634528));
#191198=CARTESIAN_POINT('Ctrl Pts',(5.70989303947358,3.63576749487417,32.8778764887955));
#191199=CARTESIAN_POINT('Ctrl Pts',(5.61585104634007,3.77941345614814,32.8859161141381));
#191200=CARTESIAN_POINT('Ctrl Pts',(5.51644043469078,3.91933335281763,32.8939557394808));
#191201=CARTESIAN_POINT('Ctrl Pts',(5.4170614940298,4.05920867274284,32.9019928034985));
#191202=CARTESIAN_POINT('Ctrl Pts',(5.31231755445393,4.19535998632222,32.9100298675162));
#191203=CARTESIAN_POINT('Ctrl Pts',(5.20253156485098,4.32734957181983,32.918066931534));
#191204=CARTESIAN_POINT('Ctrl Pts',(5.09275880476625,4.45932325220392,32.926103027063));
#191205=CARTESIAN_POINT('Ctrl Pts',(4.97794544321802,4.58713591610239,32.9341391225921));
#191206=CARTESIAN_POINT('Ctrl Pts',(4.85845491233771,4.71038266649129,32.9421752181211));
#191207=CARTESIAN_POINT('Ctrl Pts',(4.73895511116022,4.83363897859186,32.9502119371054));
#191208=CARTESIAN_POINT('Ctrl Pts',(4.61477767949704,4.95232840523451,32.9582486560897));
#191209=CARTESIAN_POINT('Ctrl Pts',(4.48632300569103,5.06608279527757,32.966285375074));
#191210=CARTESIAN_POINT('Ctrl Pts',(4.35778545910317,5.17991057418591,32.9743272789631));
#191211=CARTESIAN_POINT('Ctrl Pts',(4.22496544038581,5.28879671172445,32.9823691828522));
#191212=CARTESIAN_POINT('Ctrl Pts',(4.08829686519804,5.39241297954931,32.9904110867413));
#191213=CARTESIAN_POINT('Ctrl Pts',(3.9515756999819,5.49606911888419,32.9984560851527));
#191214=CARTESIAN_POINT('Ctrl Pts',(3.81100333320647,5.59445113434709,33.0065010835641));
#191215=CARTESIAN_POINT('Ctrl Pts',(3.66704237855232,5.6872743202611,33.0145460819755));
#191216=CARTESIAN_POINT('Ctrl Pts',(3.52294177556791,5.78018754866583,33.0225988843821));
#191217=CARTESIAN_POINT('Ctrl Pts',(3.37544634346979,5.86753099361946,33.0306516867887));
#191218=CARTESIAN_POINT('Ctrl Pts',(3.22504338389341,5.94906582347223,33.0387044891953));
#191219=CARTESIAN_POINT('Ctrl Pts',(3.18328476783862,5.97170355390324,33.0409403087882));
#191220=CARTESIAN_POINT('Ctrl Pts',(3.14130214153681,5.99389380182556,33.0431761283812));
#191221=CARTESIAN_POINT('Ctrl Pts',(3.09910619832137,6.01563211736938,33.0454119479742));
#191222=CARTESIAN_POINT('Ctrl Pts',(3.09910619832133,6.01563211736941,31.0457552630242));
#191223=CARTESIAN_POINT('Ctrl Pts',(2.93375330764826,6.10081787314653,31.0545047109265));
#191224=CARTESIAN_POINT('Ctrl Pts',(2.76488627843072,6.17918207037038,31.0632541588288));
#191225=CARTESIAN_POINT('Ctrl Pts',(2.59307866646706,6.25045854553996,31.0720036067311));
#191226=CARTESIAN_POINT('Ctrl Pts',(2.42127244185383,6.32173444515035,31.0807529839814));
#191227=CARTESIAN_POINT('Ctrl Pts',(2.24652594672473,6.38592262741835,31.0895023612317));
#191228=CARTESIAN_POINT('Ctrl Pts',(2.06943269687132,6.44280508110558,31.098251738482));
#191229=CARTESIAN_POINT('Ctrl Pts',(1.89234081822088,6.49968709436163,31.1070010479874));
#191230=CARTESIAN_POINT('Ctrl Pts',(1.71290249405599,6.54926340459542,31.1157503574927));
#191231=CARTESIAN_POINT('Ctrl Pts',(1.53172716625068,6.59136563150381,31.1244996669981));
#191232=CARTESIAN_POINT('Ctrl Pts',(1.35055318107347,6.63346754640707,31.1332489116653));
#191233=CARTESIAN_POINT('Ctrl Pts',(1.16764249714436,6.66809542395773,31.1419981563326));
#191234=CARTESIAN_POINT('Ctrl Pts',(0.983616340614552,6.69513165624665,
31.1507474009998));
#191235=CARTESIAN_POINT('Ctrl Pts',(0.799591486713964,6.7221676971596,31.1594965837355));
#191236=CARTESIAN_POINT('Ctrl Pts',(0.61445145952676,6.74161215869371,31.1682457664712));
#191237=CARTESIAN_POINT('Ctrl Pts',(0.428825047910254,6.75339900185712,
31.1769949492069));
#191238=CARTESIAN_POINT('Ctrl Pts',(0.243199888597137,6.7651857655022,31.1857440729174));
#191239=CARTESIAN_POINT('Ctrl Pts',(0.0570886373921277,6.76931499599834,
31.194493196628));
#191240=CARTESIAN_POINT('Ctrl Pts',(-0.128876626810819,6.76577266947847,
31.2032423203385));
#191241=CARTESIAN_POINT('Ctrl Pts',(-0.314840698187879,6.76223036567994,
31.21199138793));
#191242=CARTESIAN_POINT('Ctrl Pts',(-0.500658497951023,6.75101660879225,
31.2207404555216));
#191243=CARTESIAN_POINT('Ctrl Pts',(-0.685698951926038,6.7321694829622,
31.2294895231131));
#191244=CARTESIAN_POINT('Ctrl Pts',(-0.870738280459658,6.71332247176296,
31.2382385374916));
#191245=CARTESIAN_POINT('Ctrl Pts',(-1.0549999876123,6.6868422135619,31.2469875518702));
#191246=CARTESIAN_POINT('Ctrl Pts',(-1.23785829161397,6.65281863948526,
31.2557365662487));
#191247=CARTESIAN_POINT('Ctrl Pts',(-1.43007412917382,6.61705395368866,
31.2649332999479));
#191248=CARTESIAN_POINT('Ctrl Pts',(-1.62073882535771,6.57295372727795,
31.2741300336471));
#191249=CARTESIAN_POINT('Ctrl Pts',(-1.80913696091494,6.52068343478285,
31.2833267673463));
#191250=CARTESIAN_POINT('Ctrl Pts',(-1.9883835618609,6.47095219815205,31.2920767650599));
#191251=CARTESIAN_POINT('Ctrl Pts',(-2.16557827572509,6.41382586850899,
31.3008267627736));
#191252=CARTESIAN_POINT('Ctrl Pts',(-2.34011918621675,6.34949849943287,
31.3095767604873));
#191253=CARTESIAN_POINT('Ctrl Pts',(-2.51465655691071,6.28517243495561,
31.3183265807456));
#191254=CARTESIAN_POINT('Ctrl Pts',(-2.68653996295299,6.21364572242387,
31.3270764010039));
#191255=CARTESIAN_POINT('Ctrl Pts',(-2.85518555379957,6.13516132252236,
31.3358262212622));
#191256=CARTESIAN_POINT('Ctrl Pts',(-3.02382794858655,6.05667841000524,
31.3445758756997));
#191257=CARTESIAN_POINT('Ctrl Pts',(-3.18923239109244,5.971238194921,31.3533255301372));
#191258=CARTESIAN_POINT('Ctrl Pts',(-3.35083705967659,5.87913088810735,
31.3620751845747));
#191259=CARTESIAN_POINT('Ctrl Pts',(-3.51243888042352,5.78702520443132,
31.3708246848236));
#191260=CARTESIAN_POINT('Ctrl Pts',(-3.67024081223635,5.68825280605819,
31.3795741850726));
#191261=CARTESIAN_POINT('Ctrl Pts',(-3.82370687544338,5.58314917682548,
31.3883236853215));
#191262=CARTESIAN_POINT('Ctrl Pts',(-3.97717043817748,5.4780472600807,31.397073043012));
#191263=CARTESIAN_POINT('Ctrl Pts',(-4.1262980372239,5.3666144808429,31.4058224007024));
#191264=CARTESIAN_POINT('Ctrl Pts',(-4.27058317206834,5.24922931204636,
31.4145717583929));
#191265=CARTESIAN_POINT('Ctrl Pts',(-4.41486614774763,5.13184589986852,
31.423320985153));
#191266=CARTESIAN_POINT('Ctrl Pts',(-4.55430658194344,5.00851045723098,
31.4320702119131));
#191267=CARTESIAN_POINT('Ctrl Pts',(-4.68843089001777,4.87964187103185,
31.4408194386731));
#191268=CARTESIAN_POINT('Ctrl Pts',(-4.82255336917799,4.75077504208,31.4495685461291));
#191269=CARTESIAN_POINT('Ctrl Pts',(-4.95135966065125,4.61637541908105,
31.458317653585));
#191270=CARTESIAN_POINT('Ctrl Pts',(-5.07441230869261,4.47689945401826,
31.467066761041));
#191271=CARTESIAN_POINT('Ctrl Pts',(-5.19746344226432,4.33742520555498,
31.4758157608173));
#191272=CARTESIAN_POINT('Ctrl Pts',(-5.3147608845478,4.19287495491321,31.4845647605937));
#191273=CARTESIAN_POINT('Ctrl Pts',(-5.42590627628864,4.04373961586692,
31.4933137603701));
#191274=CARTESIAN_POINT('Ctrl Pts',(-5.53706380672678,3.89458798906719,
31.5020637156647));
#191275=CARTESIAN_POINT('Ctrl Pts',(-5.64206777071874,3.74085050155268,
31.5108136709595));
#191276=CARTESIAN_POINT('Ctrl Pts',(-5.74056148164018,3.58304938223145,
31.5195636262542));
#191277=CARTESIAN_POINT('Ctrl Pts',(-5.83905138951893,3.42525435593267,
31.5283132436953));
#191278=CARTESIAN_POINT('Ctrl Pts',(-5.9310313955766,3.26339625497169,31.5370628611364));
#191279=CARTESIAN_POINT('Ctrl Pts',(-6.01618907820853,3.09802485064992,
31.5458124785775));
#191280=CARTESIAN_POINT('Ctrl Pts',(-6.10134392544993,2.9326589524962,31.5545618046934));
#191281=CARTESIAN_POINT('Ctrl Pts',(-6.17967677261844,2.76378023986007,
31.5633111308092));
#191282=CARTESIAN_POINT('Ctrl Pts',(-6.25092157009239,2.5919622922708,31.5720604569251));
#191283=CARTESIAN_POINT('Ctrl Pts',(-6.32216437407773,2.4201491522904,31.5808095382276));
#191284=CARTESIAN_POINT('Ctrl Pts',(-6.38631941548945,2.24539720662784,
31.58955861953));
#191285=CARTESIAN_POINT('Ctrl Pts',(-6.44316881037564,2.06829994947604,
31.5983077008325));
#191286=CARTESIAN_POINT('Ctrl Pts',(-6.50002334524598,1.89118668024359,
31.6070575731748));
#191287=CARTESIAN_POINT('Ctrl Pts',(-6.54957082411122,1.71172794807603,
31.6158074455172));
#191288=CARTESIAN_POINT('Ctrl Pts',(-6.59164294296109,1.53053334250232,
31.6245573178595));
#191289=CARTESIAN_POINT('Ctrl Pts',(-6.63371214082158,1.34935131693482,
31.6333065827144));
#191290=CARTESIAN_POINT('Ctrl Pts',(-6.66830695239712,1.16643393829637,
31.6420558475694));
#191291=CARTESIAN_POINT('Ctrl Pts',(-6.69530988154008,0.982402458339632,
31.6508051124243));
#191292=CARTESIAN_POINT('Ctrl Pts',(-6.72231419690499,0.798361530945697,
31.6595548264313));
#191293=CARTESIAN_POINT('Ctrl Pts',(-6.7417258082929,0.613206671361114,
31.6683045404383));
#191294=CARTESIAN_POINT('Ctrl Pts',(-6.75347878028188,0.427566795112034,
31.6770542544453));
#191295=CARTESIAN_POINT('Ctrl Pts',(-6.7624899236822,0.285234494204129,
31.6837627642336));
#191296=CARTESIAN_POINT('Ctrl Pts',(-6.76699999999999,0.142617266091207,
31.6904712740219));
#191297=CARTESIAN_POINT('Ctrl Pts',(-6.767,7.38320933005802E-13,31.6971797838101));
#191298=CARTESIAN_POINT('',(-6.76699549529041,0.00780811880521902,31.3028202161435));
#191299=CARTESIAN_POINT('Ctrl Pts',(3.09910619832131,6.01563211736941,30.6515994289918));
#191300=CARTESIAN_POINT('Ctrl Pts',(2.94357060213463,6.0957602436905,30.6598137135304));
#191301=CARTESIAN_POINT('Ctrl Pts',(2.78481548965909,6.1699090339229,30.6680279980691));
#191302=CARTESIAN_POINT('Ctrl Pts',(2.62334051058967,6.23781801317569,30.6762422826077));
#191303=CARTESIAN_POINT('Ctrl Pts',(2.46194222829986,6.30569473727635,30.6844526655563));
#191304=CARTESIAN_POINT('Ctrl Pts',(2.2978269799286,6.36733741584077,30.6926630485049));
#191305=CARTESIAN_POINT('Ctrl Pts',(2.13151676911067,6.42253262062561,30.7008734314535));
#191306=CARTESIAN_POINT('Ctrl Pts',(1.96525728650907,6.47771098967754,30.7090813100575));
#191307=CARTESIAN_POINT('Ctrl Pts',(1.79680451303939,6.52644569168536,30.7172891886614));
#191308=CARTESIAN_POINT('Ctrl Pts',(1.62669815475407,6.56857230403379,30.7254970672654));
#191309=CARTESIAN_POINT('Ctrl Pts',(1.59231407181106,6.57708747623368,30.7271561491572));
#191310=CARTESIAN_POINT('Ctrl Pts',(1.55786247707645,6.58533281996979,30.7288152310489));
#191311=CARTESIAN_POINT('Ctrl Pts',(1.52334789899919,6.59330722616615,30.7304743129407));
#191312=CARTESIAN_POINT('Ctrl Pts',(1.33904885453736,6.63588852149155,30.7393333871166));
#191313=CARTESIAN_POINT('Ctrl Pts',(1.15314461898355,6.670696371689,30.7481924612925));
#191314=CARTESIAN_POINT('Ctrl Pts',(0.966284183446046,6.69765510285667,
30.7570515354684));
#191315=CARTESIAN_POINT('Ctrl Pts',(0.779072674744174,6.72466448405645,
30.7659272540623));
#191316=CARTESIAN_POINT('Ctrl Pts',(0.590901632418583,6.74379523835157,
30.7748029726563));
#191317=CARTESIAN_POINT('Ctrl Pts',(0.402423836541893,6.75502361622688,
30.7836786912502));
#191318=CARTESIAN_POINT('Ctrl Pts',(0.213408178289638,6.76628403672011,
30.7925797386372));
#191319=CARTESIAN_POINT('Ctrl Pts',(0.0240842751173204,6.76959693729915,
30.8014807860242));
#191320=CARTESIAN_POINT('Ctrl Pts',(-0.164893311894069,6.76499070181864,
30.8103818334112));
#191321=CARTESIAN_POINT('Ctrl Pts',(-0.35412781652711,6.76037820409781,
30.8192949818942));
#191322=CARTESIAN_POINT('Ctrl Pts',(-0.543014805549959,6.74782507704769,
30.8282081303772));
#191323=CARTESIAN_POINT('Ctrl Pts',(-0.730904774868618,6.72741162781603,
30.8371212788602));
#191324=CARTESIAN_POINT('Ctrl Pts',(-0.919211911296424,6.70695285514515,
30.8460542169701));
#191325=CARTESIAN_POINT('Ctrl Pts',(-1.10651734152201,6.67859888108208,
30.85498715508));
#191326=CARTESIAN_POINT('Ctrl Pts',(-1.29217883252649,6.64248167967142,
30.8639200931899));
#191327=CARTESIAN_POINT('Ctrl Pts',(-1.46890165216808,6.60810334070451,
30.8724229550484));
#191328=CARTESIAN_POINT('Ctrl Pts',(-1.64413492123316,6.56669173726127,
30.880925816907));
#191329=CARTESIAN_POINT('Ctrl Pts',(-1.81733761904343,6.51840264009593,
30.8894286787655));
#191330=CARTESIAN_POINT('Ctrl Pts',(-1.98483392565318,6.47170449089288,
30.8976514026314));
#191331=CARTESIAN_POINT('Ctrl Pts',(-2.15075201823491,6.41848410030407,
30.9058741264973));
#191332=CARTESIAN_POINT('Ctrl Pts',(-2.31454734880366,6.3588646447417,30.9140968503632));
#191333=CARTESIAN_POINT('Ctrl Pts',(-2.47816930756371,6.29930829435338,
30.9223108707544));
#191334=CARTESIAN_POINT('Ctrl Pts',(-2.63967264426746,6.23336648827075,
30.9305248911456));
#191335=CARTESIAN_POINT('Ctrl Pts',(-2.79852568667736,6.16121278491556,
30.9387389115368));
#191336=CARTESIAN_POINT('Ctrl Pts',(-2.95724248172313,6.08912096738734,
30.9469458868088));
#191337=CARTESIAN_POINT('Ctrl Pts',(-3.11331318487453,6.01082801108859,
30.9551528620807));
#191338=CARTESIAN_POINT('Ctrl Pts',(-3.26622382503544,5.92655641370019,
30.9633598373527));
#191339=CARTESIAN_POINT('Ctrl Pts',(-3.41903400595708,5.84234018106964,
30.9715614208057));
#191340=CARTESIAN_POINT('Ctrl Pts',(-3.56868794618186,5.75215330367483,
30.9797630042587));
#191341=CARTESIAN_POINT('Ctrl Pts',(-3.71469403590035,5.65626530668836,
30.9879645877116));
#191342=CARTESIAN_POINT('Ctrl Pts',(-3.86063350205369,5.56042106404273,
30.9961624287267));
#191343=CARTESIAN_POINT('Ctrl Pts',(-4.00292813464445,5.45888108106069,
31.0043602697417));
#191344=CARTESIAN_POINT('Ctrl Pts',(-4.14111313438697,5.35195954844651,
31.0125581107568));
#191345=CARTESIAN_POINT('Ctrl Pts',(-4.27928593973443,5.24504745132396,
31.0207552283379));
#191346=CARTESIAN_POINT('Ctrl Pts',(-4.41334954586082,5.13275496308821,
31.0289523459191));
#191347=CARTESIAN_POINT('Ctrl Pts',(-4.54286994362221,5.01543833331983,
31.0371494635002));
#191348=CARTESIAN_POINT('Ctrl Pts',(-4.67238890032491,4.89812300882963,
31.0453464898793));
#191349=CARTESIAN_POINT('Ctrl Pts',(-4.79736448266942,4.7757838942429,31.0535435162584));
#191350=CARTESIAN_POINT('Ctrl Pts',(-4.91739755847299,4.64881600538501,
31.0617405426375));
#191351=CARTESIAN_POINT('Ctrl Pts',(-5.03745112442993,4.52182644257186,
31.0699389682836));
#191352=CARTESIAN_POINT('Ctrl Pts',(-5.15256025641228,4.3902067920332,31.0781373939298));
#191353=CARTESIAN_POINT('Ctrl Pts',(-5.26236430002846,4.25438726184934,
31.0863358195759));
#191354=CARTESIAN_POINT('Ctrl Pts',(-5.37220705358104,4.11851985031975,
31.0945371354666));
#191355=CARTESIAN_POINT('Ctrl Pts',(-5.47674076777648,3.97844988862926,
31.1027384513572));
#191356=CARTESIAN_POINT('Ctrl Pts',(-5.57564649180597,3.83463886153726,
31.1109397672479));
#191357=CARTESIAN_POINT('Ctrl Pts',(-5.67466485289878,3.69066405775869,
31.1191504230644));
#191358=CARTESIAN_POINT('Ctrl Pts',(-5.7680422155583,3.5429399729292,31.1273610788811));
#191359=CARTESIAN_POINT('Ctrl Pts',(-5.85550366702557,3.39195604415065,
31.1355717346976));
#191360=CARTESIAN_POINT('Ctrl Pts',(-5.94301665740724,3.2408831442008,31.1437872288548));
#191361=CARTESIAN_POINT('Ctrl Pts',(-6.02460662015879,3.08654688789638,
31.1520027230119));
#191362=CARTESIAN_POINT('Ctrl Pts',(-6.10004574468918,2.92945915020152,
31.1602182171691));
#191363=CARTESIAN_POINT('Ctrl Pts',(-6.17560191440945,2.77212768799103,
31.1684464578166));
#191364=CARTESIAN_POINT('Ctrl Pts',(-6.2449880323563,2.61203654231964,31.1766746984641));
#191365=CARTESIAN_POINT('Ctrl Pts',(-6.3080248742912,2.4497165520369,31.1849029391116));
#191366=CARTESIAN_POINT('Ctrl Pts',(-6.36531529971067,2.30219359543024,
31.1923810962127));
#191367=CARTESIAN_POINT('Ctrl Pts',(-6.41736184690403,2.15283002573584,
31.1998592533139));
#191368=CARTESIAN_POINT('Ctrl Pts',(-6.46406641715259,2.00203255583923,
31.207337410415));
#191369=CARTESIAN_POINT('Ctrl Pts',(-6.52558928020088,1.80339049492085,
31.2171882158659));
#191370=CARTESIAN_POINT('Ctrl Pts',(-6.57800965699778,1.60172401471904,
31.2270390213168));
#191371=CARTESIAN_POINT('Ctrl Pts',(-6.62106237412575,1.3977918435648,31.2368898267678));
#191372=CARTESIAN_POINT('Ctrl Pts',(-6.66381959841371,1.19525936331145,
31.2466730210974));
#191373=CARTESIAN_POINT('Ctrl Pts',(-6.69733723382138,0.990492200673051,
31.2564562154271));
#191374=CARTESIAN_POINT('Ctrl Pts',(-6.72140083822521,0.784257465316973,
31.2662394097567));
#191375=CARTESIAN_POINT('Ctrl Pts',(-6.7451831335258,0.580433661735232,
31.275908236281));
#191376=CARTESIAN_POINT('Ctrl Pts',(-6.75973107202396,0.375176437153415,
31.2855770628053));
#191377=CARTESIAN_POINT('Ctrl Pts',(-6.76488312322251,0.1692493106021,31.2952458893297));
#191378=CARTESIAN_POINT('Ctrl Pts',(-6.76622845433865,0.115476519857375,
31.2977706649343));
#191379=CARTESIAN_POINT('Ctrl Pts',(-6.76693336023889,0.0616581720950804,
31.3002954405389));
#191380=CARTESIAN_POINT('Ctrl Pts',(-6.76699549529041,0.00780811880521902,
31.3028202161435));
#191381=CARTESIAN_POINT('Ctrl Pts',(-6.76699549529156,0.00780811781447526,
31.3028202161899));
#191382=CARTESIAN_POINT('Ctrl Pts',(-6.76719184327957,-0.162359134009222,
31.3107985578972));
#191383=CARTESIAN_POINT('Ctrl Pts',(-6.76096531296404,-0.332675349828753,
31.3187768996044));
#191384=CARTESIAN_POINT('Ctrl Pts',(-6.74830930116178,-0.502603796099331,
31.3267552413117));
#191385=CARTESIAN_POINT('Ctrl Pts',(-6.73518991247414,-0.678753863793646,
31.3350256955097));
#191386=CARTESIAN_POINT('Ctrl Pts',(-6.71516126771013,-0.854486811391087,
31.3432961497078));
#191387=CARTESIAN_POINT('Ctrl Pts',(-6.68827515678769,-1.02920572632327,
31.3515666039058));
#191388=CARTESIAN_POINT('Ctrl Pts',(-6.66235021874996,-1.19767847631315,
31.3595413910829));
#191389=CARTESIAN_POINT('Ctrl Pts',(-6.63004972960425,-1.36520804468051,
31.3675161782601));
#191390=CARTESIAN_POINT('Ctrl Pts',(-6.59147278417489,-1.5312659910942,
31.3754909654373));
#191391=CARTESIAN_POINT('Ctrl Pts',(-6.55289330849773,-1.69733482918813,
31.3834662756778));
#191392=CARTESIAN_POINT('Ctrl Pts',(-6.50803664249827,-1.86193148395629,
31.3914415859184));
#191393=CARTESIAN_POINT('Ctrl Pts',(-6.45705259235887,-2.02453965619635,
31.3994168961589));
#191394=CARTESIAN_POINT('Ctrl Pts',(-6.4060548599749,-2.18719146649134,
31.4073943466795));
#191395=CARTESIAN_POINT('Ctrl Pts',(-6.34892658479085,-2.3478533709865,
31.4153717972001));
#191396=CARTESIAN_POINT('Ctrl Pts',(-6.28586676284999,-2.50602634457378,
31.4233492477207));
#191397=CARTESIAN_POINT('Ctrl Pts',(-6.22277722222699,-2.66427386154194,
31.4313304578351));
#191398=CARTESIAN_POINT('Ctrl Pts',(-6.15375071269929,-2.82002976236166,
31.4393116679495));
#191399=CARTESIAN_POINT('Ctrl Pts',(-6.07903336624391,-2.97281723825957,
31.4472928780639));
#191400=CARTESIAN_POINT('Ctrl Pts',(-6.00422403241851,-3.12579281663631,
31.4552839141499));
#191401=CARTESIAN_POINT('Ctrl Pts',(-5.92371004415084,-3.27579233613148,
31.463274950236));
#191402=CARTESIAN_POINT('Ctrl Pts',(-5.8377826042711,-3.42236515662338,
31.471265986322));
#191403=CARTESIAN_POINT('Ctrl Pts',(-5.75179237700291,-3.56904507823024,
31.4792628614775));
#191404=CARTESIAN_POINT('Ctrl Pts',(-5.66038102722886,-3.71229299987543,
31.487259736633));
#191405=CARTESIAN_POINT('Ctrl Pts',(-5.56388123139021,-3.85168984252156,
31.4952566117885));
#191406=CARTESIAN_POINT('Ctrl Pts',(-5.46724056855824,-3.99129017175469,
31.5032651604998));
#191407=CARTESIAN_POINT('Ctrl Pts',(-5.36549686450026,-4.1270279052731,
31.5112737092112));
#191408=CARTESIAN_POINT('Ctrl Pts',(-5.25902133096911,-4.25851894916671,
31.5192822579225));
#191409=CARTESIAN_POINT('Ctrl Pts',(-5.23259091813481,-4.29115896005807,
31.5212702193032));
#191410=CARTESIAN_POINT('Ctrl Pts',(-5.20586910604315,-4.32353748584664,
31.5232581806838));
#191411=CARTESIAN_POINT('Ctrl Pts',(-5.17886189454373,-4.35564903053987,
31.5252461420645));
#191412=CARTESIAN_POINT('Ctrl Pts',(-5.06565597901967,-4.49025073927117,
31.5335790641112));
#191413=CARTESIAN_POINT('Ctrl Pts',(-4.94705382912415,-4.62060908824771,
31.5419119861579));
#191414=CARTESIAN_POINT('Ctrl Pts',(-4.82340118551416,-4.74627116835739,
31.5502449082046));
#191415=CARTESIAN_POINT('Ctrl Pts',(-4.69989466934291,-4.87178474636167,
31.5585679827582));
#191416=CARTESIAN_POINT('Ctrl Pts',(-4.57134979105569,-4.99261286534171,
31.5668910573118));
#191417=CARTESIAN_POINT('Ctrl Pts',(-4.43815272838792,-5.10833528260458,
31.5752141318654));
#191418=CARTESIAN_POINT('Ctrl Pts',(-4.30508862326199,-5.22394218554734,
31.5835288983114));
#191419=CARTESIAN_POINT('Ctrl Pts',(-4.16738184676328,-5.33445331389551,
31.5918436647574));
#191420=CARTESIAN_POINT('Ctrl Pts',(-4.02545578956299,-5.4394847813257,
31.6001584312033));
#191421=CARTESIAN_POINT('Ctrl Pts',(-3.88364536918663,-5.54443067246674,
31.6084664230428));
#191422=CARTESIAN_POINT('Ctrl Pts',(-3.73762279656343,-5.64390559279126,
31.6167744148823));
#191423=CARTESIAN_POINT('Ctrl Pts',(-3.58784511245682,-5.73756537644842,
31.6250824067218));
#191424=CARTESIAN_POINT('Ctrl Pts',(-3.4381620031427,-5.83116602008979,
31.6333851526089));
#191425=CARTESIAN_POINT('Ctrl Pts',(-3.28472880186222,-5.91895866071897,
31.641687898496));
#191426=CARTESIAN_POINT('Ctrl Pts',(-3.12803233099951,-6.00064186035309,
31.6499906443831));
#191427=CARTESIAN_POINT('Ctrl Pts',(-2.97139989699096,-6.08229167866654,
31.6582899972025));
#191428=CARTESIAN_POINT('Ctrl Pts',(-2.81150715872327,-6.15783687033687,
31.666589350022));
#191429=CARTESIAN_POINT('Ctrl Pts',(-2.64886664316344,-6.22702131895629,
31.6748887028414));
#191430=CARTESIAN_POINT('Ctrl Pts',(-2.48626071851213,-6.29619105320441,
31.6831862905278));
#191431=CARTESIAN_POINT('Ctrl Pts',(-2.32090850079585,-6.35900260342622,
31.6914838782141));
#191432=CARTESIAN_POINT('Ctrl Pts',(-2.15334387794478,-6.41524739533229,
31.6997814659004));
#191433=CARTESIAN_POINT('Ctrl Pts',(-1.98578704818373,-6.47148957140742,
31.7080786676829));
#191434=CARTESIAN_POINT('Ctrl Pts',(-1.81601834817873,-6.52116548721558,
31.7163758694653));
#191435=CARTESIAN_POINT('Ctrl Pts',(-1.64458844236092,-6.56411592335578,
31.7246730712477));
#191436=CARTESIAN_POINT('Ctrl Pts',(-1.47313802326137,-6.60707149893996,
31.7329712658723));
#191437=CARTESIAN_POINT('Ctrl Pts',(-1.30002633985434,-6.64329990729337,
31.7412694604968));
#191438=CARTESIAN_POINT('Ctrl Pts',(-1.12581609449634,-6.67269264400609,
31.7495676551214));
#191439=CARTESIAN_POINT('Ctrl Pts',(-0.951483325042399,-6.70210605297311,
31.757871685963));
#191440=CARTESIAN_POINT('Ctrl Pts',(-0.776050793243537,-6.72467412580284,
31.7661757168045));
#191441=CARTESIAN_POINT('Ctrl Pts',(-0.600089106419969,-6.74033990718243,
31.7744797476461));
#191442=CARTESIAN_POINT('Ctrl Pts',(-0.424063435083924,-6.75601138507133,
31.7827867980618));
#191443=CARTESIAN_POINT('Ctrl Pts',(-0.247508572355687,-6.76477554554829,
31.7910938484776));
#191444=CARTESIAN_POINT('Ctrl Pts',(-0.0709972550978696,-6.76662754921302,
31.7994008988933));
#191445=CARTESIAN_POINT('Ctrl Pts',(0.10570278254808,-6.76848153298223,
31.8077168309479));
#191446=CARTESIAN_POINT('Ctrl Pts',(0.282358833551052,-6.76340859785611,
31.8160327630025));
#191447=CARTESIAN_POINT('Ctrl Pts',(0.458400045588006,-6.75145602060807,
31.8243486950572));
#191448=CARTESIAN_POINT('Ctrl Pts',(0.59110365045948,-6.74244591399742,
31.8306174212761));
#191449=CARTESIAN_POINT('Ctrl Pts',(0.723457918522209,-6.72952755339485,
31.8368861474951));
#191450=CARTESIAN_POINT('Ctrl Pts',(0.855221520991356,-6.71274050966021,
31.843154873714));
#191451=CARTESIAN_POINT('Ctrl Pts',(1.03283939899858,-6.69011150566907,
31.8516051424374));
#191452=CARTESIAN_POINT('Ctrl Pts',(1.20970936416206,-6.66040939559615,
31.8600554111607));
#191453=CARTESIAN_POINT('Ctrl Pts',(1.38524672645127,-6.62369840095819,
31.8685056798841));
#191454=CARTESIAN_POINT('Ctrl Pts',(1.56062917106292,-6.58701980501847,
31.8769484909586));
#191455=CARTESIAN_POINT('Ctrl Pts',(1.73468103386601,-6.54334472104775,
31.8853913020331));
#191456=CARTESIAN_POINT('Ctrl Pts',(1.9068249716965,-6.49278888670459,31.8938341131076));
#191457=CARTESIAN_POINT('Ctrl Pts',(2.07884042450166,-6.4422707862935,31.9022706226254));
#191458=CARTESIAN_POINT('Ctrl Pts',(2.24895047397252,-6.38488226629492,
31.9107071321431));
#191459=CARTESIAN_POINT('Ctrl Pts',(2.41658977724467,-6.32078973297772,
31.9191436416609));
#191460=CARTESIAN_POINT('Ctrl Pts',(2.58410912557434,-6.25674306131705,
31.9275741144021));
#191461=CARTESIAN_POINT('Ctrl Pts',(2.74916094520258,-6.186002063016,31.9360045871433));
#191462=CARTESIAN_POINT('Ctrl Pts',(2.91119662121485,-6.10878246728653,
31.9444350598845));
#191463=CARTESIAN_POINT('Ctrl Pts',(3.07316263853026,-6.03159606805145,
31.9528619083884));
#191464=CARTESIAN_POINT('Ctrl Pts',(3.23211479832979,-5.9479367660304,31.9612887568923));
#191465=CARTESIAN_POINT('Ctrl Pts',(3.38752537980897,-5.85806800926296,
31.9697156053962));
#191466=CARTESIAN_POINT('Ctrl Pts',(3.54288799159001,-5.7682269917723,31.9781398528328));
#191467=CARTESIAN_POINT('Ctrl Pts',(3.69471091835848,-5.67218050755823,
31.9865641002694));
#191468=CARTESIAN_POINT('Ctrl Pts',(3.84249160300592,-5.57023763234829,
31.994988347706));
#191469=CARTESIAN_POINT('Ctrl Pts',(3.88413054576305,-5.5415140305089,31.9973619783169));
#191470=CARTESIAN_POINT('Ctrl Pts',(3.92544874126732,-5.51232258739618,
31.9997356089279));
#191471=CARTESIAN_POINT('Ctrl Pts',(3.96643535015279,-5.48267084668214,
32.0021092395388));
#191472=CARTESIAN_POINT('Ctrl Pts',(4.11525994051487,-5.37500377479484,
32.010728020476));
#191473=CARTESIAN_POINT('Ctrl Pts',(4.25964378853244,-5.26131284237969,
32.0193468014133));
#191474=CARTESIAN_POINT('Ctrl Pts',(4.39911338632861,-5.14199284462984,
32.0279655823505));
#191475=CARTESIAN_POINT('Ctrl Pts',(4.53866676266386,-5.02260117208309,
32.036589540537));
#191476=CARTESIAN_POINT('Ctrl Pts',(4.67329976643146,-4.89757388380107,
32.0452134987235));
#191477=CARTESIAN_POINT('Ctrl Pts',(4.80257417362319,-4.76734415653491,
32.05383745691));
#191478=CARTESIAN_POINT('Ctrl Pts',(4.93651882406666,-4.63240967356224,
32.0627729692812));
#191479=CARTESIAN_POINT('Ctrl Pts',(5.06471023354607,-4.49189011125268,
32.0717084816523));
#191480=CARTESIAN_POINT('Ctrl Pts',(5.18670535870331,-4.34630607780888,
32.0806439940234));
#191481=CARTESIAN_POINT('Ctrl Pts',(5.30466701868792,-4.2055354180784,32.0892840759181));
#191482=CARTESIAN_POINT('Ctrl Pts',(5.41683541664909,-4.06003008503996,
32.0979241578128));
#191483=CARTESIAN_POINT('Ctrl Pts',(5.52285301360676,-3.91029200828976,
32.1065642397075));
#191484=CARTESIAN_POINT('Ctrl Pts',(5.63430820297883,-3.75287393639111,
32.1156474673169));
#191485=CARTESIAN_POINT('Ctrl Pts',(5.73896486183385,-3.59077785566703,
32.1247306949262));
#191486=CARTESIAN_POINT('Ctrl Pts',(5.83646083153779,-3.42461880534538,
32.1338139225356));
#191487=CARTESIAN_POINT('Ctrl Pts',(5.93395680124173,-3.25845975502374,
32.1428971501449));
#191488=CARTESIAN_POINT('Ctrl Pts',(6.0242919297448,-3.0882380934111,32.1519803777542));
#191489=CARTESIAN_POINT('Ctrl Pts',(6.10716115225622,-2.91459631173385,
32.1610636053636));
#191490=CARTESIAN_POINT('Ctrl Pts',(6.18967791570172,-2.74169306263019,
32.1701082002234));
#191491=CARTESIAN_POINT('Ctrl Pts',(6.26486913904146,-2.56523943023071,
32.1791527950832));
#191492=CARTESIAN_POINT('Ctrl Pts',(6.33245769943833,-2.38584754014675,
32.188197389943));
#191493=CARTESIAN_POINT('Ctrl Pts',(6.3999842366925,-2.20662027035845,32.1972336849634));
#191494=CARTESIAN_POINT('Ctrl Pts',(6.4599219560979,-2.02446034851526,32.2062699799837));
#191495=CARTESIAN_POINT('Ctrl Pts',(6.51204204323386,-1.83999930085709,
32.2153062750041));
#191496=CARTESIAN_POINT('Ctrl Pts',(6.56406989978825,-1.65586467148865,
32.2243265795918));
#191497=CARTESIAN_POINT('Ctrl Pts',(6.60830768403376,-1.46943727624787,
32.2333468841795));
#191498=CARTESIAN_POINT('Ctrl Pts',(6.64457657006855,-1.28136302603753,
32.2423671887672));
#191499=CARTESIAN_POINT('Ctrl Pts',(6.6807997824869,-1.09352561881039,32.2513761340335));
#191500=CARTESIAN_POINT('Ctrl Pts',(6.70907407874981,-0.904045728284308,
32.2603850792999));
#191501=CARTESIAN_POINT('Ctrl Pts',(6.72927120261495,-0.713581166831877,
32.2693940245662));
#191502=CARTESIAN_POINT('Ctrl Pts',(6.74942246308742,-0.52354911007812,
32.278382512425));
#191503=CARTESIAN_POINT('Ctrl Pts',(6.7615331374365,-0.332537081736051,
32.2873710002838));
#191504=CARTESIAN_POINT('Ctrl Pts',(6.76552650890326,-0.141209267851879,
32.2963594881426));
#191505=CARTESIAN_POINT('Ctrl Pts',(6.76903014275974,0.0266545564857062,
32.3042456491578));
#191506=CARTESIAN_POINT('Ctrl Pts',(6.76628608516899,0.194761201565154,
32.3121318101731));
#191507=CARTESIAN_POINT('Ctrl Pts',(6.75727523833114,0.362657349900467,
32.3200179711883));
#191508=CARTESIAN_POINT('Ctrl Pts',(6.74799552976617,0.535563110454366,
32.3281394360445));
#191509=CARTESIAN_POINT('Ctrl Pts',(6.73207200223608,0.708168137699135,
32.3362609009007));
#191510=CARTESIAN_POINT('Ctrl Pts',(6.70954746935247,0.879921449054339,
32.3443823657569));
#191511=CARTESIAN_POINT('Ctrl Pts',(6.68702454279963,1.05166251187013,32.352503251433));
#191512=CARTESIAN_POINT('Ctrl Pts',(6.65790159617412,1.22255161670381,32.3606241371092));
#191513=CARTESIAN_POINT('Ctrl Pts',(6.62227317093297,1.39204419812784,32.3687450227854));
#191514=CARTESIAN_POINT('Ctrl Pts',(6.58664048707617,1.56155703876218,32.3768668791397));
#191515=CARTESIAN_POINT('Ctrl Pts',(6.54450085274506,1.72967266550059,32.3849887354939));
#191516=CARTESIAN_POINT('Ctrl Pts',(6.49599964184681,1.89585802557211,32.3931105918482));
#191517=CARTESIAN_POINT('Ctrl Pts',(6.44746304506513,2.06216463242634,32.4012383738083));
#191518=CARTESIAN_POINT('Ctrl Pts',(6.39255570441807,2.2265378079745,32.4093661557685));
#191519=CARTESIAN_POINT('Ctrl Pts',(6.33147267132592,2.38846034345412,32.4174939377287));
#191520=CARTESIAN_POINT('Ctrl Pts',(6.27036475527627,2.55044884015679,32.4256250306451));
#191521=CARTESIAN_POINT('Ctrl Pts',(6.20307627439913,2.7099843697335,32.4337561235616));
#191522=CARTESIAN_POINT('Ctrl Pts',(6.12984980112805,2.8665711949314,32.441887216478));
#191523=CARTESIAN_POINT('Ctrl Pts',(6.05654340422177,3.02332892810471,32.4500271841426));
#191524=CARTESIAN_POINT('Ctrl Pts',(5.97728623760122,3.1771312035923,32.4581671518071));
#191525=CARTESIAN_POINT('Ctrl Pts',(5.8923664078801,3.3275076431597,32.4663071194717));
#191526=CARTESIAN_POINT('Ctrl Pts',(5.84832331248869,3.40549936657975,32.4705288586522));
#191527=CARTESIAN_POINT('Ctrl Pts',(5.80275772824519,3.48257004300769,32.4747505978326));
#191528=CARTESIAN_POINT('Ctrl Pts',(5.75571430051519,3.55865731573651,32.4789723370131));
#191529=CARTESIAN_POINT('Ctrl Pts',(5.6616666918867,3.71076838400895,32.4874122933117));
#191530=CARTESIAN_POINT('Ctrl Pts',(5.56151575697688,3.85926168118158,32.4958522496103));
#191531=CARTESIAN_POINT('Ctrl Pts',(5.45556534188854,4.00363532310132,32.5042922059089));
#191532=CARTESIAN_POINT('Ctrl Pts',(5.34969215428111,4.14790373076912,32.5127260103055));
#191533=CARTESIAN_POINT('Ctrl Pts',(5.2380281087655,4.28805820050605,32.5211598147022));
#191534=CARTESIAN_POINT('Ctrl Pts',(5.12092063759979,4.42362530323315,32.5295936190988));
#191535=CARTESIAN_POINT('Ctrl Pts',(5.00388213697058,4.55911256360934,32.5380224563998));
#191536=CARTESIAN_POINT('Ctrl Pts',(4.88140681907092,4.69001759109137,32.5464512937007));
#191537=CARTESIAN_POINT('Ctrl Pts',(4.75388294872376,4.81589928360566,32.5548801310017));
#191538=CARTESIAN_POINT('Ctrl Pts',(4.62641663704579,4.94172415865764,32.563305163896));
#191539=CARTESIAN_POINT('Ctrl Pts',(4.49390655336497,5.06252998563764,32.5717301967904));
#191540=CARTESIAN_POINT('Ctrl Pts',(4.35677868991053,5.17791159128287,32.5801552296847));
#191541=CARTESIAN_POINT('Ctrl Pts',(4.21969089840114,5.29325947974441,32.5885778005888));
#191542=CARTESIAN_POINT('Ctrl Pts',(4.07798827294214,5.40318609321708,32.597000371493));
#191543=CARTESIAN_POINT('Ctrl Pts',(3.93213113612272,5.50732546054201,32.6054229423971));
#191544=CARTESIAN_POINT('Ctrl Pts',(3.78627698404962,5.61146269681186,32.613845340946));
#191545=CARTESIAN_POINT('Ctrl Pts',(3.63626875842448,5.70981272508494,32.622267739495));
#191546=CARTESIAN_POINT('Ctrl Pts',(3.48259759741858,5.80205161769993,32.6306901380439));
#191547=CARTESIAN_POINT('Ctrl Pts',(3.35711527563958,5.87737056712343,32.6375675646082));
#191548=CARTESIAN_POINT('Ctrl Pts',(3.2291912354976,5.94861549514981,32.6444449911725));
#191549=CARTESIAN_POINT('Ctrl Pts',(3.09910619832134,6.0156321173694,32.6513224177368));
#191550=CARTESIAN_POINT('Origin',(0.,0.,4.30282021618968));
#191551=CARTESIAN_POINT('',(3.09910619832134,6.0156321173694,35.0460577214445));
#191552=CARTESIAN_POINT('',(3.09910619832129,6.01563211736943,34.6512344137135));
#191553=CARTESIAN_POINT('',(3.09910619832133,6.0156321173694,4.30282021618968));
#191554=CARTESIAN_POINT('',(-6.76699957039783,-0.0024112725963184,33.6971797837815));
#191555=CARTESIAN_POINT('Ctrl Pts',(-6.76699957039762,-0.00241127320226596,
33.6971797838101));
#191556=CARTESIAN_POINT('Ctrl Pts',(-6.7669271526358,-0.205644553729062,
33.7067651955258));
#191557=CARTESIAN_POINT('Ctrl Pts',(-6.75769587893337,-0.408730533938623,
33.7163506072415));
#191558=CARTESIAN_POINT('Ctrl Pts',(-6.73936492970196,-0.610941359136269,
33.7259360189573));
#191559=CARTESIAN_POINT('Ctrl Pts',(-6.72206822778545,-0.801743282352738,
33.7349806138171));
#191560=CARTESIAN_POINT('Ctrl Pts',(-6.69665992838825,-0.991859096466692,
33.7440252086769));
#191561=CARTESIAN_POINT('Ctrl Pts',(-6.66321417359887,-1.18062097082473,
33.7530698035367));
#191562=CARTESIAN_POINT('Ctrl Pts',(-6.62979911055412,-1.36920962645055,
33.7621060985571));
#191563=CARTESIAN_POINT('Ctrl Pts',(-6.58836135906894,-1.5564465888405,
33.7711423935774));
#191564=CARTESIAN_POINT('Ctrl Pts',(-6.53902650525747,-1.74167200228408,
33.7801786885978));
#191565=CARTESIAN_POINT('Ctrl Pts',(-6.48977895333856,-1.92656964483361,
33.7891989931855));
#191566=CARTESIAN_POINT('Ctrl Pts',(-6.43266226562066,-2.10946261691137,
33.7982192977732));
#191567=CARTESIAN_POINT('Ctrl Pts',(-6.36785235671145,-2.28970420865327,
33.8072396023609));
#191568=CARTESIAN_POINT('Ctrl Pts',(-6.30312406329269,-2.46971882112366,
33.8162485476272));
#191569=CARTESIAN_POINT('Ctrl Pts',(-6.230721963088,-2.64708849335919,33.8252574928936));
#191570=CARTESIAN_POINT('Ctrl Pts',(-6.1508715314434,-2.82118209332171,
33.8342664381599));
#191571=CARTESIAN_POINT('Ctrl Pts',(-6.07120242322513,-2.99488036357349,
33.8432549260187));
#191572=CARTESIAN_POINT('Ctrl Pts',(-5.98411884353561,-3.16531719513597,
33.8522434138775));
#191573=CARTESIAN_POINT('Ctrl Pts',(-5.8898938408915,-3.33188228228855,
33.8612319017363));
#191574=CARTESIAN_POINT('Ctrl Pts',(-5.80722436920872,-3.47802022199983,
33.8691180627515));
#191575=CARTESIAN_POINT('Ctrl Pts',(-5.71905843551334,-3.62117797452296,
33.8770042237668));
#191576=CARTESIAN_POINT('Ctrl Pts',(-5.62561100294064,-3.76095597469489,
33.884890384782));
#191577=CARTESIAN_POINT('Ctrl Pts',(-5.52937532653589,-3.90490461001544,
33.8930118496382));
#191578=CARTESIAN_POINT('Ctrl Pts',(-5.42757999479772,-4.04520345033654,
33.9011333144944));
#191579=CARTESIAN_POINT('Ctrl Pts',(-5.3205430607239,-4.18140054754178,
33.9092547793505));
#191580=CARTESIAN_POINT('Ctrl Pts',(-5.21351375995882,-4.31758793188949,
33.9173756650267));
#191581=CARTESIAN_POINT('Ctrl Pts',(-5.10124382769221,-4.4496738678554,
33.9254965507029));
#191582=CARTESIAN_POINT('Ctrl Pts',(-4.98409252327873,-4.57723832888316,
33.9336174363792));
#191583=CARTESIAN_POINT('Ctrl Pts',(-4.86692721593431,-4.70481803751185,
33.9417392927334));
#191584=CARTESIAN_POINT('Ctrl Pts',(-4.7448796232044,-4.82787492616167,
33.9498611490877));
#191585=CARTESIAN_POINT('Ctrl Pts',(-4.61834683994616,-4.9460248145313,
33.957983005442));
#191586=CARTESIAN_POINT('Ctrl Pts',(-4.4917217399348,-5.06426090359765,
33.9661107874021));
#191587=CARTESIAN_POINT('Ctrl Pts',(-4.360605181564,-5.17758259180336,33.9742385693623));
#191588=CARTESIAN_POINT('Ctrl Pts',(-4.22542889119776,-5.28564468020991,
33.9823663513225));
#191589=CARTESIAN_POINT('Ctrl Pts',(-4.09019753503495,-5.3937507890949,
33.9904974442389));
#191590=CARTESIAN_POINT('Ctrl Pts',(-3.95090344480812,-5.4965928100976,
33.9986285371554));
#191591=CARTESIAN_POINT('Ctrl Pts',(-3.80800825153753,-5.59386826411045,
34.0067596300718));
#191592=CARTESIAN_POINT('Ctrl Pts',(-3.66495709413552,-5.69124989021592,
34.0148995977364));
#191593=CARTESIAN_POINT('Ctrl Pts',(-3.5182972932805,-5.7830526201265,34.0230395654009));
#191594=CARTESIAN_POINT('Ctrl Pts',(-3.36851669183846,-5.8690190233808,
34.0311795330655));
#191595=CARTESIAN_POINT('Ctrl Pts',(-3.29083399583325,-5.91360491705708,
34.0354012722459));
#191596=CARTESIAN_POINT('Ctrl Pts',(-3.21231220779933,-5.95662166305593,
34.0396230114264));
#191597=CARTESIAN_POINT('Ctrl Pts',(-3.13302154779433,-5.99803842777424,
34.0438447506068));
#191598=CARTESIAN_POINT('Ctrl Pts',(-2.97450162274143,-6.08083988810595,
34.0522849600644));
#191599=CARTESIAN_POINT('Ctrl Pts',(-2.81257972647671,-6.15741467235917,
34.0607251695221));
#191600=CARTESIAN_POINT('Ctrl Pts',(-2.64777336502189,-6.22748626714509,
34.0691653789797));
#191601=CARTESIAN_POINT('Ctrl Pts',(-2.48309186880216,-6.29750477231675,
34.0775991937282));
#191602=CARTESIAN_POINT('Ctrl Pts',(-2.31553056965315,-6.36102977990712,
34.0860330084768));
#191603=CARTESIAN_POINT('Ctrl Pts',(-2.14562988568944,-6.41783151801575,
34.0944668232253));
#191604=CARTESIAN_POINT('Ctrl Pts',(-1.97583180836011,-6.47459895234738,
34.1028955446139));
#191605=CARTESIAN_POINT('Ctrl Pts',(-1.80369747832809,-6.52465110656424,
34.1113242660024));
#191606=CARTESIAN_POINT('Ctrl Pts',(-1.62978590058578,-6.56780685756302,
34.1197529873909));
#191607=CARTESIAN_POINT('Ctrl Pts',(-1.45595264623619,-6.6109431727952,
34.1281779127927));
#191608=CARTESIAN_POINT('Ctrl Pts',(-1.28034406322702,-6.64718919741407,
34.1366028381944));
#191609=CARTESIAN_POINT('Ctrl Pts',(-1.10353326092001,-6.67641395825957,
34.1450277635961));
#191610=CARTESIAN_POINT('Ctrl Pts',(-0.926774959693113,-6.70563004128964,
34.1534501873539));
#191611=CARTESIAN_POINT('Ctrl Pts',(-0.7488154797323,-6.72782896386837,
34.1618726111116));
#191612=CARTESIAN_POINT('Ctrl Pts',(-0.570237433187901,-6.74293098509775,
34.1702950348693));
#191613=CARTESIAN_POINT('Ctrl Pts',(-0.391656578125033,-6.75803324383844,
34.1787175910875));
#191614=CARTESIAN_POINT('Ctrl Pts',(-0.212457468695141,-6.76603834350035,
34.1871401473057));
#191615=CARTESIAN_POINT('Ctrl Pts',(-0.0332278194027092,-6.76691842067109,
34.1955627035239));
#191616=CARTESIAN_POINT('Ctrl Pts',(0.146007884301281,-6.76779852757101,
34.2039855442577));
#191617=CARTESIAN_POINT('Ctrl Pts',(0.325273796352285,-6.76155313026978,
34.2124083849914));
#191618=CARTESIAN_POINT('Ctrl Pts',(0.503982060694046,-6.74820650858423,
34.2208312257252));
#191619=CARTESIAN_POINT('Ctrl Pts',(0.682721311485282,-6.73485757271126,
34.2292555269058));
#191620=CARTESIAN_POINT('Ctrl Pts',(0.860902389161484,-6.71440498246587,
34.2376798280864));
#191621=CARTESIAN_POINT('Ctrl Pts',(1.03794204611007,-6.68692495164383,
34.2461041292671));
#191622=CARTESIAN_POINT('Ctrl Pts',(1.21503712445465,-6.65943631833297,
34.2545310676339));
#191623=CARTESIAN_POINT('Ctrl Pts',(1.3909897401937,-6.62491590957336,34.2629580060007));
#191624=CARTESIAN_POINT('Ctrl Pts',(1.5652259636951,-6.58349122294355,34.2713849443675));
#191625=CARTESIAN_POINT('Ctrl Pts',(1.739618847463,-6.54202929031335,34.2798194596111));
#191626=CARTESIAN_POINT('Ctrl Pts',(1.91229193050123,-6.49365075284648,
34.2882539748548));
#191627=CARTESIAN_POINT('Ctrl Pts',(2.08268448301231,-6.43853355541615,
34.2966884900984));
#191628=CARTESIAN_POINT('Ctrl Pts',(2.25315933658591,-6.3833897359073,34.3051270792852));
#191629=CARTESIAN_POINT('Ctrl Pts',(2.42135114815643,-6.32150087536006,
34.313565668472));
#191630=CARTESIAN_POINT('Ctrl Pts',(2.58671785149581,-6.25309361490398,
34.3220042576587));
#191631=CARTESIAN_POINT('Ctrl Pts',(2.75226939739626,-6.18460989060746,
34.330452279279));
#191632=CARTESIAN_POINT('Ctrl Pts',(2.91498922011784,-6.10959334256098,
34.3389003008993));
#191633=CARTESIAN_POINT('Ctrl Pts',(3.07435748803953,-6.02831776167575,
34.3473483225196));
#191634=CARTESIAN_POINT('Ctrl Pts',(3.16493985392956,-5.982122025839,34.3521500424319));
#191635=CARTESIAN_POINT('Ctrl Pts',(3.25443992877924,-5.93390507819876,
34.3569517623441));
#191636=CARTESIAN_POINT('Ctrl Pts',(3.34276625935181,-5.88372354341527,
34.3617534822563));
#191637=CARTESIAN_POINT('Ctrl Pts',(3.49433020463023,-5.79761432385856,
34.3699930141071));
#191638=CARTESIAN_POINT('Ctrl Pts',(3.64277477392542,-5.70552565776409,
34.3782325459579));
#191639=CARTESIAN_POINT('Ctrl Pts',(3.78759811378457,-5.60770804593602,
34.3864720778088));
#191640=CARTESIAN_POINT('Ctrl Pts',(3.93226070985816,-5.50999900482062,
34.3947024643551));
#191641=CARTESIAN_POINT('Ctrl Pts',(4.07330978728402,-5.40657387672074,
34.4029328509015));
#191642=CARTESIAN_POINT('Ctrl Pts',(4.21026787585194,-5.29772908080143,
34.4111632374478));
#191643=CARTESIAN_POINT('Ctrl Pts',(4.34709838257771,-5.18898567808728,
34.4193859570656));
#191644=CARTESIAN_POINT('Ctrl Pts',(4.47984521295829,-5.07483288212843,
34.4276086766834));
#191645=CARTESIAN_POINT('Ctrl Pts',(4.60805963189971,-4.95561050011563,
34.4358313963012));
#191646=CARTESIAN_POINT('Ctrl Pts',(4.73616044362843,-4.83649375772296,
34.444046829997));
#191647=CARTESIAN_POINT('Ctrl Pts',(4.85973658862605,-4.71231662372661,
34.4522622636928));
#191648=CARTESIAN_POINT('Ctrl Pts',(4.97837231072254,-4.58345918884756,
34.4604776973885));
#191649=CARTESIAN_POINT('Ctrl Pts',(5.09694706327011,-4.45466797668406,
34.4686889089894));
#191650=CARTESIAN_POINT('Ctrl Pts',(5.21058620907145,-4.32120151522181,
34.4769001205902));
#191651=CARTESIAN_POINT('Ctrl Pts',(5.31891048686519,-4.18347705057832,
34.485111332191));
#191652=CARTESIAN_POINT('Ctrl Pts',(5.4271984386734,-4.04579877112076,34.4933197902045));
#191653=CARTESIAN_POINT('Ctrl Pts',(5.53017485320515,-3.90386561242643,
34.501528248218));
#191654=CARTESIAN_POINT('Ctrl Pts',(5.62750039659726,-3.75812829561442,
34.5097367062316));
#191655=CARTESIAN_POINT('Ctrl Pts',(5.67086105135836,-3.69319913868554,
34.5133937535147));
#191656=CARTESIAN_POINT('Ctrl Pts',(5.71310061191423,-3.62751532051784,
34.5170508007979));
#191657=CARTESIAN_POINT('Ctrl Pts',(5.75419177661988,-3.56111864417351,
34.5207078480811));
#191658=CARTESIAN_POINT('Ctrl Pts',(5.8537337425594,-3.40027492649089,34.529566922257));
#191659=CARTESIAN_POINT('Ctrl Pts',(5.94643025790849,-3.23541338678471,
34.5384259964329));
#191660=CARTESIAN_POINT('Ctrl Pts',(6.03200112876272,-3.06712428548393,
34.5472850706088));
#191661=CARTESIAN_POINT('Ctrl Pts',(6.11773277006746,-2.89851900281952,
34.5561607892027));
#191662=CARTESIAN_POINT('Ctrl Pts',(6.19631189493145,-2.72647352027105,
34.5650365077966));
#191663=CARTESIAN_POINT('Ctrl Pts',(6.26750626288204,-2.55159837057764,
34.5739122263905));
#191664=CARTESIAN_POINT('Ctrl Pts',(6.33890379944304,-2.37622417661734,
34.5828132737775));
#191665=CARTESIAN_POINT('Ctrl Pts',(6.40287430870817,-2.19800439778514,
34.5917143211645));
#191666=CARTESIAN_POINT('Ctrl Pts',(6.45923434673109,-2.01756800480415,
34.6006153685515));
#191667=CARTESIAN_POINT('Ctrl Pts',(6.51567100699877,-1.83688630607194,
34.6095285170345));
#191668=CARTESIAN_POINT('Ctrl Pts',(6.56447645711243,-1.65398222284785,
34.6184416655175));
#191669=CARTESIAN_POINT('Ctrl Pts',(6.60551804789054,-1.46949662095304,
34.6273548140005));
#191670=CARTESIAN_POINT('Ctrl Pts',(6.64665076222272,-1.28460141057566,
34.6362877521104));
#191671=CARTESIAN_POINT('Ctrl Pts',(6.67998508175404,-1.09811791216753,
34.6452206902203));
#191672=CARTESIAN_POINT('Ctrl Pts',(6.7054396206955,-0.910696707585425,
34.6541536283302));
#191673=CARTESIAN_POINT('Ctrl Pts',(6.72966865101346,-0.732298895765291,
34.6626564901887));
#191674=CARTESIAN_POINT('Ctrl Pts',(6.74675876246543,-0.553051726812206,
34.6711593520473));
#191675=CARTESIAN_POINT('Ctrl Pts',(6.75668362546571,-0.373517583740801,
34.6796622139058));
#191676=CARTESIAN_POINT('Ctrl Pts',(6.76628150077116,-0.199898429680771,
34.6878849377717));
#191677=CARTESIAN_POINT('Ctrl Pts',(6.76919589212276,-0.0256780814334027,
34.6961076616376));
#191678=CARTESIAN_POINT('Ctrl Pts',(6.7653684706439,0.148588210896766,34.7043303855035));
#191679=CARTESIAN_POINT('Ctrl Pts',(6.76154510036101,0.32267004825996,34.7125444058947));
#191680=CARTESIAN_POINT('Ctrl Pts',(6.75099413508758,0.496797377211207,
34.7207584262859));
#191681=CARTESIAN_POINT('Ctrl Pts',(6.73370909347369,0.670410951931526,
34.7289724466771));
#191682=CARTESIAN_POINT('Ctrl Pts',(6.71643887714313,0.843875619261818,
34.7371794219491));
#191683=CARTESIAN_POINT('Ctrl Pts',(6.69244612277225,1.01682705500566,34.7453863972211));
#191684=CARTESIAN_POINT('Ctrl Pts',(6.66177638078357,1.18870705072113,34.753593372493));
#191685=CARTESIAN_POINT('Ctrl Pts',(6.63112678820333,1.36047412470952,34.761794955946));
#191686=CARTESIAN_POINT('Ctrl Pts',(6.59380900846871,1.5311708089034,34.769996539399));
#191687=CARTESIAN_POINT('Ctrl Pts',(6.54992031077734,1.70024495954743,34.778198122852));
#191688=CARTESIAN_POINT('Ctrl Pts',(6.50605163979526,1.86924196051419,34.786395963867));
#191689=CARTESIAN_POINT('Ctrl Pts',(6.45561811425605,2.03661755643509,34.7945938048821));
#191690=CARTESIAN_POINT('Ctrl Pts',(6.39876791504692,2.20183064048216,34.8027916458971));
#191691=CARTESIAN_POINT('Ctrl Pts',(6.34192273269053,2.36702914498994,34.8109887634783));
#191692=CARTESIAN_POINT('Ctrl Pts',(6.27866211308071,2.53006517600267,34.8191858810594));
#191693=CARTESIAN_POINT('Ctrl Pts',(6.20918395909201,2.69041326976999,34.8273829986406));
#191694=CARTESIAN_POINT('Ctrl Pts',(6.13970657812516,2.85075957948618,34.8355800250197));
#191695=CARTESIAN_POINT('Ctrl Pts',(6.0640119422426,3.00841768184325,34.8437770513988));
#191696=CARTESIAN_POINT('Ctrl Pts',(5.98234587145017,3.16288268425231,34.8519740777779));
#191697=CARTESIAN_POINT('Ctrl Pts',(5.9006658599143,3.31737405449014,34.860172503424));
#191698=CARTESIAN_POINT('Ctrl Pts',(5.81301255034493,3.4686709215932,34.8683709290701));
#191699=CARTESIAN_POINT('Ctrl Pts',(5.71967745242754,3.61629352240551,34.8765693547163));
#191700=CARTESIAN_POINT('Ctrl Pts',(5.62630945047878,3.76396816557697,34.8847706706069));
#191701=CARTESIAN_POINT('Ctrl Pts',(5.52725586175385,3.90796565906952,34.8929719864976));
#191702=CARTESIAN_POINT('Ctrl Pts',(5.4228512141872,4.04783568203903,34.9011733023882));
#191703=CARTESIAN_POINT('Ctrl Pts',(5.31832766720378,4.18786499355118,34.9093839582048));
#191704=CARTESIAN_POINT('Ctrl Pts',(5.20844110159758,4.32375715592714,34.9175946140214));
#191705=CARTESIAN_POINT('Ctrl Pts',(5.09356666560883,4.4550945694787,34.925805269838));
#191706=CARTESIAN_POINT('Ctrl Pts',(4.97862453689802,4.58650937698614,34.9340207639951));
#191707=CARTESIAN_POINT('Ctrl Pts',(4.85868892501422,4.71336382520894,34.9422362581523));
#191708=CARTESIAN_POINT('Ctrl Pts',(4.73417136100773,4.83527770915117,34.9504517523094));
#191709=CARTESIAN_POINT('Ctrl Pts',(4.60946060570938,4.95738074472775,34.9586799929569));
#191710=CARTESIAN_POINT('Ctrl Pts',(4.48015395749285,5.07452765682164,34.9669082336044));
#191711=CARTESIAN_POINT('Ctrl Pts',(4.34669651735882,5.18637815686253,34.9751364742519));
#191712=CARTESIAN_POINT('Ctrl Pts',(4.22540501090053,5.28803240434733,34.9826146313531));
#191713=CARTESIAN_POINT('Ctrl Pts',(4.10068554142758,5.38531227359529,34.9900927884542));
#191714=CARTESIAN_POINT('Ctrl Pts',(3.97289173337,5.47799418354203,34.9975709455553));
#191715=CARTESIAN_POINT('Ctrl Pts',(3.83479376690758,5.57814914007742,35.0056520748702));
#191716=CARTESIAN_POINT('Ctrl Pts',(3.69265246187375,5.67326238485263,35.0137332041851));
#191717=CARTESIAN_POINT('Ctrl Pts',(3.54687864974605,5.7629802050654,35.0218143334999));
#191718=CARTESIAN_POINT('Ctrl Pts',(3.40110483761835,5.85269802527818,35.0298954628148));
#191719=CARTESIAN_POINT('Ctrl Pts',(3.25169878737696,5.93702015617671,35.0379765921297));
#191720=CARTESIAN_POINT('Ctrl Pts',(3.09910619832134,6.0156321173694,35.0460577214446));
#191721=CARTESIAN_POINT('Ctrl Pts',(3.09910619832137,6.01563211736938,33.0454119479742));
#191722=CARTESIAN_POINT('Ctrl Pts',(2.94681999133791,6.09408623802922,33.0534810764109));
#191723=CARTESIAN_POINT('Ctrl Pts',(2.79175421223906,6.16665004262685,33.0615502048476));
#191724=CARTESIAN_POINT('Ctrl Pts',(2.63442150037846,6.23314626479627,33.0696193332843));
#191725=CARTESIAN_POINT('Ctrl Pts',(2.50118950502637,6.28945638783577,33.0764524074089));
#191726=CARTESIAN_POINT('Ctrl Pts',(2.36633229850053,6.34141627804308,33.0832854815335));
#191727=CARTESIAN_POINT('Ctrl Pts',(2.23016766295296,6.38894679858261,33.0901185556582));
#191728=CARTESIAN_POINT('Ctrl Pts',(2.06411512600675,6.44691018596453,33.0984514777049));
#191729=CARTESIAN_POINT('Ctrl Pts',(1.89558818275161,6.49847023352894,33.1067843997516));
#191730=CARTESIAN_POINT('Ctrl Pts',(1.72511532004303,6.54341395087861,33.1151173217983));
#191731=CARTESIAN_POINT('Ctrl Pts',(1.55484391491809,6.58830455565333,33.1234403963519));
#191732=CARTESIAN_POINT('Ctrl Pts',(1.38263150491179,6.62659431812345,33.1317634709055));
#191733=CARTESIAN_POINT('Ctrl Pts',(1.20902467572304,6.65811897862248,33.1400865454592));
#191734=CARTESIAN_POINT('Ctrl Pts',(1.03559114117627,6.68961217115,33.1484013119051));
#191735=CARTESIAN_POINT('Ctrl Pts',(0.860766300803221,6.71435365394648,
33.1567160783511));
#191736=CARTESIAN_POINT('Ctrl Pts',(0.685110183186748,6.73222942544993,
33.1650308447971));
#191737=CARTESIAN_POINT('Ctrl Pts',(0.509597184570617,6.75009063234507,
33.1733388366366));
#191738=CARTESIAN_POINT('Ctrl Pts',(0.333254602950186,6.76109723930545,
33.1816468284761));
#191739=CARTESIAN_POINT('Ctrl Pts',(0.156651128898255,6.76518657716215,
33.1899548203157));
#191740=CARTESIAN_POINT('Ctrl Pts',(-0.0198408316317251,6.76927333286994,
33.1982575662028));
#191741=CARTESIAN_POINT('Ctrl Pts',(-0.196593009420326,6.76645151595209,
33.2065603120898));
#191742=CARTESIAN_POINT('Ctrl Pts',(-0.373032913541262,6.75671040118007,
33.2148630579769));
#191743=CARTESIAN_POINT('Ctrl Pts',(-0.549400712296347,6.74697326729122,
33.2231624107964));
#191744=CARTESIAN_POINT('Ctrl Pts',(-0.725456144818687,6.73032248909197,
33.2314617636158));
#191745=CARTESIAN_POINT('Ctrl Pts',(-0.900627749657548,6.70679943464443,
33.2397611164352));
#191746=CARTESIAN_POINT('Ctrl Pts',(-1.07576209843538,6.68328138315585,
33.2480587041216));
#191747=CARTESIAN_POINT('Ctrl Pts',(-1.2500126494086,6.6528940135678,33.2563562918079));
#191748=CARTESIAN_POINT('Ctrl Pts',(-1.42281383919723,6.61573047962119,
33.2646538794943));
#191749=CARTESIAN_POINT('Ctrl Pts',(-1.59560699235385,6.57856867407499,
33.2729510812767));
#191750=CARTESIAN_POINT('Ctrl Pts',(-1.76695057857995,6.5346314054757,33.2812482830591));
#191751=CARTESIAN_POINT('Ctrl Pts',(-1.9362898001284,6.48406283204587,33.2895454848415));
#191752=CARTESIAN_POINT('Ctrl Pts',(-2.1056492847869,6.43348820758688,33.2978436794661));
#191753=CARTESIAN_POINT('Ctrl Pts',(-2.27300359369002,6.37628079726977,
33.3061418740906));
#191754=CARTESIAN_POINT('Ctrl Pts',(-2.43781346375676,6.31263451467977,
33.3144400687152));
#191755=CARTESIAN_POINT('Ctrl Pts',(-2.60273924652664,6.24894346891717,
33.3227440995567));
#191756=CARTESIAN_POINT('Ctrl Pts',(-2.76511668967857,6.17880462746615,
33.3310481303983));
#191757=CARTESIAN_POINT('Ctrl Pts',(-2.92442604456808,6.10246026696216,
33.3393521612399));
#191758=CARTESIAN_POINT('Ctrl Pts',(-3.08379332872378,6.02608814554743,
33.3476592116556));
#191759=CARTESIAN_POINT('Ctrl Pts',(-3.24008999050089,5.94350616458784,
33.3559662620714));
#191760=CARTESIAN_POINT('Ctrl Pts',(-3.39282105141429,5.85500250325139,
33.3642733124871));
#191761=CARTESIAN_POINT('Ctrl Pts',(-3.54571540760837,5.76640421656413,
33.3725892445417));
#191762=CARTESIAN_POINT('Ctrl Pts',(-3.69503624859151,5.67187178046481,
33.3809051765964));
#191763=CARTESIAN_POINT('Ctrl Pts',(-3.84031681796374,5.57173722798059,
33.389221108651));
#191764=CARTESIAN_POINT('Ctrl Pts',(-3.94983239701644,5.49625367539074,
33.3954898348699));
#191765=CARTESIAN_POINT('Ctrl Pts',(-4.05705269361544,5.41758764516095,
33.4017585610888));
#191766=CARTESIAN_POINT('Ctrl Pts',(-4.16179038218382,5.33589634595372,
33.4080272873078));
#191767=CARTESIAN_POINT('Ctrl Pts',(-4.30297721710928,5.22577613866572,
33.4164775560311));
#191768=CARTESIAN_POINT('Ctrl Pts',(-4.43991059809946,5.10995537588841,
33.4249278247545));
#191769=CARTESIAN_POINT('Ctrl Pts',(-4.57212051848605,4.98878772493267,
33.4333780934778));
#191770=CARTESIAN_POINT('Ctrl Pts',(-4.70421375913251,4.86772700853966,
33.4418209045523));
#191771=CARTESIAN_POINT('Ctrl Pts',(-4.83159160466415,4.74132903239765,
33.4502637156268));
#191772=CARTESIAN_POINT('Ctrl Pts',(-4.95381666139334,4.60998801357463,
33.4587065267013));
#191773=CARTESIAN_POINT('Ctrl Pts',(-5.07595049161931,4.47874502523895,
33.4671430362191));
#191774=CARTESIAN_POINT('Ctrl Pts',(-5.19293897456915,4.34256659076512,
33.4755795457368));
#191775=CARTESIAN_POINT('Ctrl Pts',(-5.30438089851626,4.20188437292792,
33.4840160552546));
#191776=CARTESIAN_POINT('Ctrl Pts',(-5.41574307976984,4.06130282078801,
33.4924465279958));
#191777=CARTESIAN_POINT('Ctrl Pts',(-5.52156641316081,3.9162241727613,33.500877000737));
#191778=CARTESIAN_POINT('Ctrl Pts',(-5.62148924746264,3.76711396703922,
33.5093074734782));
#191779=CARTESIAN_POINT('Ctrl Pts',(-5.7213691252086,3.61806786339078,33.517734321982));
#191780=CARTESIAN_POINT('Ctrl Pts',(-5.81535337643285,3.46499393209991,
33.5261611704858));
#191781=CARTESIAN_POINT('Ctrl Pts',(-5.90312267419187,3.30838808083965,
33.5345880189896));
#191782=CARTESIAN_POINT('Ctrl Pts',(-5.99086488070321,3.15183056821275,
33.5430122664263));
#191783=CARTESIAN_POINT('Ctrl Pts',(-6.07239579744064,2.99174359860373,
33.5514365138629));
#191784=CARTESIAN_POINT('Ctrl Pts',(-6.14744102587402,2.82864947163853,
33.5598607612995));
#191785=CARTESIAN_POINT('Ctrl Pts',(-6.16858589997194,2.78269578673703,
33.5622343919105));
#191786=CARTESIAN_POINT('Ctrl Pts',(-6.18921615777526,2.73650351364091,
33.5646080225215));
#191787=CARTESIAN_POINT('Ctrl Pts',(-6.20932632878607,2.69008467202133,
33.5669816531325));
#191788=CARTESIAN_POINT('Ctrl Pts',(-6.28108308539527,2.52445378214046,
33.5754511999076));
#191789=CARTESIAN_POINT('Ctrl Pts',(-6.34619125863235,2.35599024723317,
33.5839207466827));
#191790=CARTESIAN_POINT('Ctrl Pts',(-6.40444782480402,2.18525446100975,
33.5923902934579));
#191791=CARTESIAN_POINT('Ctrl Pts',(-6.46451278498047,2.0092187130396,33.6011227509848));
#191792=CARTESIAN_POINT('Ctrl Pts',(-6.51729378950696,1.83076772316103,
33.6098552085118));
#191793=CARTESIAN_POINT('Ctrl Pts',(-6.56262398702231,1.65053185517863,
33.6185876660388));
#191794=CARTESIAN_POINT('Ctrl Pts',(-6.60664942458908,1.47548379917879,
33.6270687732196));
#191795=CARTESIAN_POINT('Ctrl Pts',(-6.64364700528507,1.298752522188,33.6355498804005));
#191796=CARTESIAN_POINT('Ctrl Pts',(-6.67351596073093,1.12092538639715,
33.6440309875814));
#191797=CARTESIAN_POINT('Ctrl Pts',(-6.70471273319322,0.935192989328691,
33.6528891202814));
#191798=CARTESIAN_POINT('Ctrl Pts',(-6.72813253998287,0.748265475079885,
33.6617472529814));
#191799=CARTESIAN_POINT('Ctrl Pts',(-6.74372097542174,0.560817622455764,
33.6706053856814));
#191800=CARTESIAN_POINT('Ctrl Pts',(-6.7593094108606,0.373369769831643,
33.6794635183815));
#191801=CARTESIAN_POINT('Ctrl Pts',(-6.76706649355167,0.185401981686163,
33.6883216510815));
#191802=CARTESIAN_POINT('Ctrl Pts',(-6.76699957039783,-0.00241127259631757,
33.6971797837815));
#191803=CARTESIAN_POINT('',(-6.76699870538252,-0.00418585132867157,33.3028202162336));
#191804=CARTESIAN_POINT('Ctrl Pts',(3.09910619832134,6.0156321173694,32.6513224177368));
#191805=CARTESIAN_POINT('Ctrl Pts',(2.93976909702956,6.09771868592969,32.659746362849));
#191806=CARTESIAN_POINT('Ctrl Pts',(2.77718943464024,6.1734601017708,32.6681703079613));
#191807=CARTESIAN_POINT('Ctrl Pts',(2.61190384602355,6.24261542137007,32.6765942530736));
#191808=CARTESIAN_POINT('Ctrl Pts',(2.44657075146376,6.31179061740688,32.6850206193737));
#191809=CARTESIAN_POINT('Ctrl Pts',(2.27853048772618,6.37437581447125,32.6934469856739));
#191810=CARTESIAN_POINT('Ctrl Pts',(2.10833867007918,6.43017861744514,32.701873351974));
#191811=CARTESIAN_POINT('Ctrl Pts',(1.93799498176463,6.48603121604997,32.710307237542));
#191812=CARTESIAN_POINT('Ctrl Pts',(1.76549622016069,6.53508922196037,32.71874112311));
#191813=CARTESIAN_POINT('Ctrl Pts',(1.5914132705117,6.57721010782226,32.7271750086781));
#191814=CARTESIAN_POINT('Ctrl Pts',(1.41725032812322,6.61935034862417,32.7356127696952));
#191815=CARTESIAN_POINT('Ctrl Pts',(1.2415020718237,6.65454704126416,32.7440505307124));
#191816=CARTESIAN_POINT('Ctrl Pts',(1.06474905880451,6.68270891493674,32.7524882917295));
#191817=CARTESIAN_POINT('Ctrl Pts',(0.887791059201659,6.71090344890842,
32.76093583831));
#191818=CARTESIAN_POINT('Ctrl Pts',(0.709826304952664,6.73204681432255,
32.7693833848905));
#191819=CARTESIAN_POINT('Ctrl Pts',(0.531441288722675,6.74609955134378,
32.777830931471));
#191820=CARTESIAN_POINT('Ctrl Pts',(0.397348744821141,6.75666303529429,
32.7841809772015));
#191821=CARTESIAN_POINT('Ctrl Pts',(0.263018840592247,6.76322098232725,
32.7905310229321));
#191822=CARTESIAN_POINT('Ctrl Pts',(0.128700420179844,6.76577602362401,
32.7968810686626));
#191823=CARTESIAN_POINT('Ctrl Pts',(-0.0455850810752542,6.76909132953489,
32.8051206005134));
#191824=CARTESIAN_POINT('Ctrl Pts',(-0.220240240340706,6.76567256978095,
32.8133601323642));
#191825=CARTESIAN_POINT('Ctrl Pts',(-0.394705640901005,6.75547899538152,
32.8215996642151));
#191826=CARTESIAN_POINT('Ctrl Pts',(-0.568977397060637,6.74529673513721,
32.8298300507614));
#191827=CARTESIAN_POINT('Ctrl Pts',(-0.743059461722417,6.72835465355148,
32.8380604373078));
#191828=CARTESIAN_POINT('Ctrl Pts',(-0.916389947831463,6.70466393367434,
32.8462908238541));
#191829=CARTESIAN_POINT('Ctrl Pts',(-1.08955896978082,6.6809952826338,32.854513543472));
#191830=CARTESIAN_POINT('Ctrl Pts',(-1.26197745693309,6.65059056112991,
32.8627362630898));
#191831=CARTESIAN_POINT('Ctrl Pts',(-1.43308608571328,6.61351292967172,
32.8709589827077));
#191832=CARTESIAN_POINT('Ctrl Pts',(-1.60404309991955,6.57646815166654,
32.8791744164035));
#191833=CARTESIAN_POINT('Ctrl Pts',(-1.77369222248841,6.53276232331814,
32.8873898500992));
#191834=CARTESIAN_POINT('Ctrl Pts',(-1.94148192728308,6.48251007913086,
32.895605283795));
#191835=CARTESIAN_POINT('Ctrl Pts',(-2.10918540119871,6.4322836606949,32.9038164953959));
#191836=CARTESIAN_POINT('Ctrl Pts',(-2.27503102038421,6.37551762868008,
32.9120277069967));
#191837=CARTESIAN_POINT('Ctrl Pts',(-2.43847967629493,6.31237719629432,
32.9202389185975));
#191838=CARTESIAN_POINT('Ctrl Pts',(-2.60187352054539,6.24925793772556,
32.928447376611));
#191839=CARTESIAN_POINT('Ctrl Pts',(-2.76287167113866,6.17976866522749,
32.9366558346245));
#191840=CARTESIAN_POINT('Ctrl Pts',(-2.92095226736622,6.10412375790073,
32.9448642926381));
#191841=CARTESIAN_POINT('Ctrl Pts',(-2.99138062479868,6.07042229992112,
32.9485213399212));
#191842=CARTESIAN_POINT('Ctrl Pts',(-3.0612301299238,6.03549965571144,32.9521783872043));
#191843=CARTESIAN_POINT('Ctrl Pts',(-3.13045596805582,5.99937783708142,
32.9558354344874));
#191844=CARTESIAN_POINT('Ctrl Pts',(-3.2981532351189,5.91187394505123,32.9646945086632));
#191845=CARTESIAN_POINT('Ctrl Pts',(-3.46201476408152,5.81742093791027,
32.9735535828391));
#191846=CARTESIAN_POINT('Ctrl Pts',(-3.62149832520691,5.71638337417318,
32.982412657015));
#191847=CARTESIAN_POINT('Ctrl Pts',(-3.78128152385848,5.61515598118074,
32.9912883756089));
#191848=CARTESIAN_POINT('Ctrl Pts',(-3.93667009785948,5.50731944748327,
33.0001640942028));
#191849=CARTESIAN_POINT('Ctrl Pts',(-4.08715270607949,5.39328024092825,
33.0090398127968));
#191850=CARTESIAN_POINT('Ctrl Pts',(-4.23806474914441,5.27891559869957,
33.0179408601838));
#191851=CARTESIAN_POINT('Ctrl Pts',(-4.38404260209493,5.15831301966201,
33.0268419075708));
#191852=CARTESIAN_POINT('Ctrl Pts',(-4.52460747369214,5.03191973395933,
33.0357429549577));
#191853=CARTESIAN_POINT('Ctrl Pts',(-4.6653634451595,4.90535461485181,33.0446561034407));
#191854=CARTESIAN_POINT('Ctrl Pts',(-4.80069154679471,4.77298324132962,
33.0535692519236));
#191855=CARTESIAN_POINT('Ctrl Pts',(-4.93015059524625,4.63528899942529,
33.0624824004066));
#191856=CARTESIAN_POINT('Ctrl Pts',(-5.05989707818596,4.4972890386514,33.0714153385164));
#191857=CARTESIAN_POINT('Ctrl Pts',(-5.18374826544594,4.35394276052935,
33.0803482766263));
#191858=CARTESIAN_POINT('Ctrl Pts',(-5.30130209679829,4.20576807235992,
33.0892812147362));
#191859=CARTESIAN_POINT('Ctrl Pts',(-5.4131962996516,4.06472725365568,33.0977840765948));
#191860=CARTESIAN_POINT('Ctrl Pts',(-5.51938513319482,3.91931215430751,
33.1062869384535));
#191861=CARTESIAN_POINT('Ctrl Pts',(-5.61955890029082,3.7699929398027,33.1147898003121));
#191862=CARTESIAN_POINT('Ctrl Pts',(-5.71636857825428,3.62568824318374,
33.1230071145069));
#191863=CARTESIAN_POINT('Ctrl Pts',(-5.80775482896632,3.47744567269272,
33.1312244287017));
#191864=CARTESIAN_POINT('Ctrl Pts',(-5.89338115962983,3.32571007565604,
33.1394417428965));
#191865=CARTESIAN_POINT('Ctrl Pts',(-5.97891380324206,3.17414049835361,
33.1476500662127));
#191866=CARTESIAN_POINT('Ctrl Pts',(-6.05869889872921,3.01908581222887,
33.155858389529));
#191867=CARTESIAN_POINT('Ctrl Pts',(-6.13244214595523,2.86102120343629,
33.1640667128453));
#191868=CARTESIAN_POINT('Ctrl Pts',(-6.20611811168363,2.70310080884637,
33.1722675470923));
#191869=CARTESIAN_POINT('Ctrl Pts',(-6.2737630546176,2.54217628233276,33.1804683813393));
#191870=CARTESIAN_POINT('Ctrl Pts',(-6.33512766578461,2.37874892710653,
33.1886692155863));
#191871=CARTESIAN_POINT('Ctrl Pts',(-6.39644744104012,2.21544097970014,
33.1968640579127));
#191872=CARTESIAN_POINT('Ctrl Pts',(-6.45149589761738,2.04963417970298,
33.2050589002391));
#191873=CARTESIAN_POINT('Ctrl Pts',(-6.50007108122949,1.88185146570183,
33.2132537425655));
#191874=CARTESIAN_POINT('Ctrl Pts',(-6.54861871409412,1.71416391426809,
33.2214439369624));
#191875=CARTESIAN_POINT('Ctrl Pts',(-6.59070028934588,1.54450302516549,
33.2296341313592));
#191876=CARTESIAN_POINT('Ctrl Pts',(-6.6261631197505,1.37340864656457,33.237824325756));
#191877=CARTESIAN_POINT('Ctrl Pts',(-6.66161398315837,1.20237200407354,
33.2460117563569));
#191878=CARTESIAN_POINT('Ctrl Pts',(-6.690450478747,1.02990318643661,33.2541991869577));
#191879=CARTESIAN_POINT('Ctrl Pts',(-6.7125705924874,0.856554166923097,
33.2623866175585));
#191880=CARTESIAN_POINT('Ctrl Pts',(-6.73469010246755,0.683209878906435,
33.2705738246865));
#191881=CARTESIAN_POINT('Ctrl Pts',(-6.75009354462253,0.508985791705292,
33.2787610318144));
#191882=CARTESIAN_POINT('Ctrl Pts',(-6.75873050626867,0.334441240927599,
33.2869482389424));
#191883=CARTESIAN_POINT('Ctrl Pts',(-6.76431180143616,0.221648722252779,
33.2922388980249));
#191884=CARTESIAN_POINT('Ctrl Pts',(-6.76706854691273,0.108722518485693,
33.2975295571074));
#191885=CARTESIAN_POINT('Ctrl Pts',(-6.7669987053831,-0.00418585039646904,
33.3028202161899));
#191886=CARTESIAN_POINT('Ctrl Pts',(-6.76699870538252,-0.00418585132862214,
33.3028202162336));
#191887=CARTESIAN_POINT('Ctrl Pts',(-6.76687598560987,-0.202579075886211,
33.3121165237244));
#191888=CARTESIAN_POINT('Ctrl Pts',(-6.75802467330528,-0.400624589624038,
33.3214128312153));
#191889=CARTESIAN_POINT('Ctrl Pts',(-6.74056009748527,-0.597610719607133,
33.3307091387062));
#191890=CARTESIAN_POINT('Ctrl Pts',(-6.72296064155559,-0.796118186901281,
33.3400772422135));
#191891=CARTESIAN_POINT('Ctrl Pts',(-6.69661444238275,-0.993549688353143,
33.3494453457209));
#191892=CARTESIAN_POINT('Ctrl Pts',(-6.66168924145868,-1.18919529524538,
33.3588134492283));
#191893=CARTESIAN_POINT('Ctrl Pts',(-6.62663418857151,-1.38556831287409,
33.3682163833622));
#191894=CARTESIAN_POINT('Ctrl Pts',(-6.58293632376023,-1.58014199450794,
33.3776193174961));
#191895=CARTESIAN_POINT('Ctrl Pts',(-6.53081377367392,-1.77221907607129,
33.38702225163));
#191896=CARTESIAN_POINT('Ctrl Pts',(-6.47844794047052,-1.96519268152013,
33.3964690741601));
#191897=CARTESIAN_POINT('Ctrl Pts',(-6.41757868048744,-2.15564619035235,
33.4059158966902));
#191898=CARTESIAN_POINT('Ctrl Pts',(-6.34847464685296,-2.3428953579418,
33.4153627192203));
#191899=CARTESIAN_POINT('Ctrl Pts',(-6.30620383452604,-2.45743533491929,
33.4211413234674));
#191900=CARTESIAN_POINT('Ctrl Pts',(-6.26085269822801,-2.57077678281479,
33.4269199277145));
#191901=CARTESIAN_POINT('Ctrl Pts',(-6.21249120912136,-2.68276759645517,
33.4326985319617));
#191902=CARTESIAN_POINT('Ctrl Pts',(-6.14495867126726,-2.83915285259983,
33.4407678411842));
#191903=CARTESIAN_POINT('Ctrl Pts',(-6.07139345292414,-2.99327311130894,
33.4488371504067));
#191904=CARTESIAN_POINT('Ctrl Pts',(-5.99196749816581,-3.1446167494505,
33.4569064596292));
#191905=CARTESIAN_POINT('Ctrl Pts',(-5.91264060916037,-3.29577162094135,
33.46496570423));
#191906=CARTESIAN_POINT('Ctrl Pts',(-5.8274676997558,-3.4441564364899,33.4730249488308));
#191907=CARTESIAN_POINT('Ctrl Pts',(-5.73666957447558,-3.58927725221752,
33.4810841934315));
#191908=CARTESIAN_POINT('Ctrl Pts',(-5.64596477363654,-3.7342489093696,
33.4891351545518));
#191909=CARTESIAN_POINT('Ctrl Pts',(-5.54964645891247,-3.87596292919723,
33.497186115672));
#191910=CARTESIAN_POINT('Ctrl Pts',(-5.44798231712482,-4.01394789107872,
33.5052370767923));
#191911=CARTESIAN_POINT('Ctrl Pts',(-5.34640039149385,-4.15182126402584,
33.5132815270714));
#191912=CARTESIAN_POINT('Ctrl Pts',(-5.23948146358352,-4.28597128239312,
33.5213259773505));
#191913=CARTESIAN_POINT('Ctrl Pts',(-5.12753763633549,-4.41595366687232,
33.5293704276296));
#191914=CARTESIAN_POINT('Ctrl Pts',(-5.01565983500512,-4.54585938605942,
33.5374101331878));
#191915=CARTESIAN_POINT('Ctrl Pts',(-4.89876327716363,-4.67160208273011,
33.5454498387461));
#191916=CARTESIAN_POINT('Ctrl Pts',(-4.77720155368238,-4.79276896120548,
33.5534895443043));
#191917=CARTESIAN_POINT('Ctrl Pts',(-4.65301598539016,-4.91655116197347,
33.5617027826087));
#191918=CARTESIAN_POINT('Ctrl Pts',(-4.52396180850659,-5.03555744474693,
33.5699160209132));
#191919=CARTESIAN_POINT('Ctrl Pts',(-4.39045754893377,-5.14938554693766,
33.5781292592176));
#191920=CARTESIAN_POINT('Ctrl Pts',(-4.25981609088834,-5.26077277371472,
33.5861663767658));
#191921=CARTESIAN_POINT('Ctrl Pts',(-4.12491377015921,-5.36720140300616,
33.594203494314));
#191922=CARTESIAN_POINT('Ctrl Pts',(-3.98617765391193,-5.46833399779615,
33.6022406118622));
#191923=CARTESIAN_POINT('Ctrl Pts',(-3.84742686026559,-5.56947729177169,
33.6102785796863));
#191924=CARTESIAN_POINT('Ctrl Pts',(-3.70484176537793,-5.6653232154408,
33.6183165475104));
#191925=CARTESIAN_POINT('Ctrl Pts',(-3.55887967978884,-5.7555768107798,
33.6263545153345));
#191926=CARTESIAN_POINT('Ctrl Pts',(-3.41287323186925,-5.84585783693967,
33.6343949261422));
#191927=CARTESIAN_POINT('Ctrl Pts',(-3.26348806786615,-5.93054295519892,
33.6424353369499));
#191928=CARTESIAN_POINT('Ctrl Pts',(-3.11120728679728,-6.00938251558174,
33.6504757477577));
#191929=CARTESIAN_POINT('Ctrl Pts',(-2.95317115107825,-6.0912017666864,
33.6588200407455));
#191930=CARTESIAN_POINT('Ctrl Pts',(-2.79201664149837,-6.16672476394506,
33.6671643337333));
#191931=CARTESIAN_POINT('Ctrl Pts',(-2.62830678136401,-6.23572709978844,
33.6755086267211));
#191932=CARTESIAN_POINT('Ctrl Pts',(-2.47028031779755,-6.30233393154681,
33.6835632369366));
#191933=CARTESIAN_POINT('Ctrl Pts',(-2.3098733223086,-6.36286519375461,
33.6916178471521));
#191934=CARTESIAN_POINT('Ctrl Pts',(-2.1476074221366,-6.41717004296939,
33.6996724573677));
#191935=CARTESIAN_POINT('Ctrl Pts',(-1.98521868438587,-6.47151600172218,
33.7077331650369));
#191936=CARTESIAN_POINT('Ctrl Pts',(-1.82096859603854,-6.5196260581066,
33.7157938727062));
#191937=CARTESIAN_POINT('Ctrl Pts',(-1.65538939645397,-6.5614003799576,
33.7238545803754));
#191938=CARTESIAN_POINT('Ctrl Pts',(-1.48957674011847,-6.60323360109956,
33.7319266531596));
#191939=CARTESIAN_POINT('Ctrl Pts',(-1.32243159560379,-6.63871318802318,
33.7399987259437));
#191940=CARTESIAN_POINT('Ctrl Pts',(-1.15449232025342,-6.66779097471388,
33.7480707987278));
#191941=CARTESIAN_POINT('Ctrl Pts',(-1.13690195712319,-6.67083665194362,
33.7489162870223));
#191942=CARTESIAN_POINT('Ctrl Pts',(-1.11930288207885,-6.67381214233745,
33.7497617753167));
#191943=CARTESIAN_POINT('Ctrl Pts',(-1.10169571360772,-6.67671742360109,
33.7506072636112));
#191944=CARTESIAN_POINT('Ctrl Pts',(-0.928163846523169,-6.70535115212547,
33.7589401856579));
#191945=CARTESIAN_POINT('Ctrl Pts',(-0.753292129788909,-6.72725210630963,
33.7672731077046));
#191946=CARTESIAN_POINT('Ctrl Pts',(-0.577637743217702,-6.74230106399962,
33.7756060297513));
#191947=CARTESIAN_POINT('Ctrl Pts',(-0.402190937534932,-6.75733223747101,
33.7839291043049));
#191948=CARTESIAN_POINT('Ctrl Pts',(-0.225963648258534,-6.76552751565066,
33.7922521788585));
#191949=CARTESIAN_POINT('Ctrl Pts',(-0.0495225306741007,-6.76681878868909,
33.8005752534121));
#191950=CARTESIAN_POINT('Ctrl Pts',(0.126742463076882,-6.7681087727765,
33.8088900198581));
#191951=CARTESIAN_POINT('Ctrl Pts',(0.303220514111993,-6.76250847945381,
33.817204786304));
#191952=CARTESIAN_POINT('Ctrl Pts',(0.479340340565712,-6.7500016176225,
33.82551955275));
#191953=CARTESIAN_POINT('Ctrl Pts',(0.655316670203667,-6.7375049459832,
33.8338275445895));
#191954=CARTESIAN_POINT('Ctrl Pts',(0.830935011259,-6.71811294314075,33.8421355364291));
#191955=CARTESIAN_POINT('Ctrl Pts',(1.00562434957782,-6.69186137539745,
33.8504435282686));
#191956=CARTESIAN_POINT('Ctrl Pts',(1.18020338302623,-6.66562638379901,
33.8587462741557));
#191957=CARTESIAN_POINT('Ctrl Pts',(1.35385423965773,-6.63254051075785,
33.8670490200428));
#191958=CARTESIAN_POINT('Ctrl Pts',(1.52601106752696,-6.59269134889426,
33.8753517659298));
#191959=CARTESIAN_POINT('Ctrl Pts',(1.69809754038708,-6.55285847211318,
33.8836511187493));
#191960=CARTESIAN_POINT('Ctrl Pts',(1.86869086264453,-6.5062678922022,33.8919504715687));
#191961=CARTESIAN_POINT('Ctrl Pts',(2.03723512847489,-6.45305834711789,
33.9002498243881));
#191962=CARTESIAN_POINT('Ctrl Pts',(2.20574354776793,-6.39986011881102,
33.9085474120745));
#191963=CARTESIAN_POINT('Ctrl Pts',(2.37220344727305,-6.34004583454991,
33.9168449997608));
#191964=CARTESIAN_POINT('Ctrl Pts',(2.53607361104077,-6.273804239804,33.9251425874472));
#191965=CARTESIAN_POINT('Ctrl Pts',(2.6999361535403,-6.20756572582001,33.9334397892296));
#191966=CARTESIAN_POINT('Ctrl Pts',(2.86120887784884,-6.13490062754828,
33.941736991012));
#191967=CARTESIAN_POINT('Ctrl Pts',(3.01936991942733,-6.0560460937527,33.9500341927944));
#191968=CARTESIAN_POINT('Ctrl Pts',(3.17754988653657,-5.97718212423333,
33.958332387419));
#191969=CARTESIAN_POINT('Ctrl Pts',(3.33261711791284,-5.89212739916181,
33.9666305820435));
#191970=CARTESIAN_POINT('Ctrl Pts',(3.48407358466363,-5.80116542227931,
33.9749287766681));
#191971=CARTESIAN_POINT('Ctrl Pts',(3.63563657251316,-5.71013947077805,
33.9832328075096));
#191972=CARTESIAN_POINT('Ctrl Pts',(3.78358342271712,-5.61319814502181,
33.9915368383512));
#191973=CARTESIAN_POINT('Ctrl Pts',(3.92744362413891,-5.51066924966566,
33.9998408691928));
#191974=CARTESIAN_POINT('Ctrl Pts',(4.07135613708945,-5.40810307198121,
34.0081479196085));
#191975=CARTESIAN_POINT('Ctrl Pts',(4.2111787604503,-5.29994548298093,34.0164549700243));
#191976=CARTESIAN_POINT('Ctrl Pts',(4.34647325685333,-5.1865652630097,34.02476202044));
#191977=CARTESIAN_POINT('Ctrl Pts',(4.48191240590684,-5.07306382044798,
34.0330779524946));
#191978=CARTESIAN_POINT('Ctrl Pts',(4.61281349292275,-4.9543288195222,34.0413938845493));
#191979=CARTESIAN_POINT('Ctrl Pts',(4.73877360384359,-4.83076740606658,
34.0497098166039));
#191980=CARTESIAN_POINT('Ctrl Pts',(4.83372501093598,-4.73762418807348,
34.0559785428228));
#191981=CARTESIAN_POINT('Ctrl Pts',(4.92586945993759,-4.64173916925834,
34.0622472690418));
#191982=CARTESIAN_POINT('Ctrl Pts',(5.01504935426716,-4.54329934896046,
34.0685159952607));
#191983=CARTESIAN_POINT('Ctrl Pts',(5.13526421857672,-4.41060206636408,
34.0769662639841));
#191984=CARTESIAN_POINT('Ctrl Pts',(5.25031120312685,-4.27301794204137,
34.0854165327074));
#191985=CARTESIAN_POINT('Ctrl Pts',(5.35978790112841,-4.1309759930212,34.0938668014307));
#191986=CARTESIAN_POINT('Ctrl Pts',(5.46916798222985,-3.98905940084,34.1023096125053));
#191987=CARTESIAN_POINT('Ctrl Pts',(5.57298737371688,-3.84269308690014,
34.1107524235798));
#191988=CARTESIAN_POINT('Ctrl Pts',(5.67088275146282,-3.69234042568687,
34.1191952346543));
#191989=CARTESIAN_POINT('Ctrl Pts',(5.76870506192389,-3.54209998489687,
34.127631744172));
#191990=CARTESIAN_POINT('Ctrl Pts',(5.86061199246948,-3.38787940495988,
34.1360682536897));
#191991=CARTESIAN_POINT('Ctrl Pts',(5.94628228554423,-3.23017274779894,
34.1445047632075));
#191992=CARTESIAN_POINT('Ctrl Pts',(6.03189127691449,-3.07257893823715,
34.1529352359487));
#191993=CARTESIAN_POINT('Ctrl Pts',(6.1112723743925,-2.91150431774581,34.1613657086899));
#191994=CARTESIAN_POINT('Ctrl Pts',(6.18414910334081,-2.74746953898474,
34.1697961814311));
#191995=CARTESIAN_POINT('Ctrl Pts',(6.25699450278089,-2.58350527833043,
34.1782230299349));
#191996=CARTESIAN_POINT('Ctrl Pts',(6.32334097365471,-2.41658369877348,
34.1866498784388));
#191997=CARTESIAN_POINT('Ctrl Pts',(6.38295894597132,-2.24724811581737,
34.1950767269426));
#191998=CARTESIAN_POINT('Ctrl Pts',(6.44255851634897,-2.07796480070834,
34.2035009743792));
#191999=CARTESIAN_POINT('Ctrl Pts',(6.49543361990836,-1.90626928053868,
34.2119252218159));
#192000=CARTESIAN_POINT('Ctrl Pts',(6.5414034748861,-1.73272316852638,34.2203494692525));
#192001=CARTESIAN_POINT('Ctrl Pts',(6.55435602118504,-1.683824514138,34.2227230998635));
#192002=CARTESIAN_POINT('Ctrl Pts',(6.56676066383916,-1.6347790406321,34.2250967304745));
#192003=CARTESIAN_POINT('Ctrl Pts',(6.57861407424934,-1.58559952765146,
34.2274703610854));
#192004=CARTESIAN_POINT('Ctrl Pts',(6.62165444759655,-1.40702606006075,
34.2360891420226));
#192005=CARTESIAN_POINT('Ctrl Pts',(6.65740394947293,-1.22676431481958,
34.2447079229599));
#192006=CARTESIAN_POINT('Ctrl Pts',(6.68575961015859,-1.04542213252451,
34.2533267038971));
#192007=CARTESIAN_POINT('Ctrl Pts',(6.71413230391721,-0.863971019083175,
34.2619506620836));
#192008=CARTESIAN_POINT('Ctrl Pts',(6.73510224573738,-0.681438473878653,
34.2705746202702));
#192009=CARTESIAN_POINT('Ctrl Pts',(6.74861822987197,-0.498438549311445,
34.2791985784567));
#192010=CARTESIAN_POINT('Ctrl Pts',(6.76262250039721,-0.308827461859928,
34.2881340908278));
#192011=CARTESIAN_POINT('Ctrl Pts',(6.76862417928981,-0.118714956467937,
34.2970696031989));
#192012=CARTESIAN_POINT('Ctrl Pts',(6.76662525726767,0.071215361455789,
34.3060051155701));
#192013=CARTESIAN_POINT('Ctrl Pts',(6.76469242462695,0.254866106146177,
34.3146451974648));
#192014=CARTESIAN_POINT('Ctrl Pts',(6.75527962541511,0.438346215844395,
34.3232852793595));
#192015=CARTESIAN_POINT('Ctrl Pts',(6.7384416584577,0.621041879072454,34.3319253612542));
#192016=CARTESIAN_POINT('Ctrl Pts',(6.72074008013742,0.813107916473974,
34.3410085888635));
#192017=CARTESIAN_POINT('Ctrl Pts',(6.6948317137539,1.00430653618667,34.3500918164728));
#192018=CARTESIAN_POINT('Ctrl Pts',(6.66084140508571,1.1939349966794,34.3591750440822));
#192019=CARTESIAN_POINT('Ctrl Pts',(6.62685109641752,1.38356345717214,34.3682582716915));
#192020=CARTESIAN_POINT('Ctrl Pts',(6.58477896296765,1.57162138737109,34.3773414993009));
#192021=CARTESIAN_POINT('Ctrl Pts',(6.53481107523681,1.75742232003644,34.3864247269102));
#192022=CARTESIAN_POINT('Ctrl Pts',(6.48505571073819,1.9424330048736,34.39546932177));
#192023=CARTESIAN_POINT('Ctrl Pts',(6.42742651200367,2.12537693045655,34.4045139166298));
#192024=CARTESIAN_POINT('Ctrl Pts',(6.36211102908855,2.30560886829267,34.4135585114896));
#192025=CARTESIAN_POINT('Ctrl Pts',(6.29685548341016,2.48567541495596,34.42259480651));
#192026=CARTESIAN_POINT('Ctrl Pts',(6.2239278166343,2.66303471905864,34.4316311015303));
#192027=CARTESIAN_POINT('Ctrl Pts',(6.14356489363596,2.83705822951941,34.4406673965507));
#192028=CARTESIAN_POINT('Ctrl Pts',(6.06334417913174,3.0107737917319,34.4496877011384));
#192029=CARTESIAN_POINT('Ctrl Pts',(5.97571458140068,3.18116513204231,34.4587080057261));
#192030=CARTESIAN_POINT('Ctrl Pts',(5.88096029452438,3.34762527984059,34.4677283103138));
#192031=CARTESIAN_POINT('Ctrl Pts',(5.78632533226585,3.51387580341852,34.4767372555801));
#192032=CARTESIAN_POINT('Ctrl Pts',(5.68458370354612,3.67620480799962,34.4857462008464));
#192033=CARTESIAN_POINT('Ctrl Pts',(5.57606575828179,3.83402916777082,34.4947551461128));
#192034=CARTESIAN_POINT('Ctrl Pts',(5.46779423429805,3.99149514183217,34.5037436339716));
#192035=CARTESIAN_POINT('Ctrl Pts',(5.35277724324437,4.14447669357504,34.5127321218304));
#192036=CARTESIAN_POINT('Ctrl Pts',(5.23138843283429,4.29241937196351,34.5217206096892));
#192037=CARTESIAN_POINT('Ctrl Pts',(5.12488645837745,4.42221871097652,34.5296067707044));
#192038=CARTESIAN_POINT('Ctrl Pts',(5.01348039957638,4.54813957515049,34.5374929317197));
#192039=CARTESIAN_POINT('Ctrl Pts',(4.89745054546475,4.66982517389324,34.5453790927349));
#192040=CARTESIAN_POINT('Ctrl Pts',(4.77796699932706,4.79513281099226,34.5534999896431));
#192041=CARTESIAN_POINT('Ctrl Pts',(4.65363260093625,4.91589208310284,34.5616208865514));
#192042=CARTESIAN_POINT('Ctrl Pts',(4.5248381008275,5.03171234882319,34.5697417834596));
#192043=CARTESIAN_POINT('Ctrl Pts',(4.39603319210573,5.1475419746352,34.5778633366634));
#192044=CARTESIAN_POINT('Ctrl Pts',(4.26276772961882,5.25843154700934,34.5859848898673));
#192045=CARTESIAN_POINT('Ctrl Pts',(4.12546777413614,5.36402876992324,34.5941064430712));
#192046=CARTESIAN_POINT('Ctrl Pts',(3.98816086652181,5.46963133971283,34.6022284075069));
#192047=CARTESIAN_POINT('Ctrl Pts',(3.84681935301713,5.56994080785572,34.6103503719426));
#192048=CARTESIAN_POINT('Ctrl Pts',(3.70190033812664,5.66464675744021,34.6184723363782));
#192049=CARTESIAN_POINT('Ctrl Pts',(3.55690923914435,5.75939981466181,34.626598340756));
#192050=CARTESIAN_POINT('Ctrl Pts',(3.40833739558179,5.84854359293189,34.6347243451338));
#192051=CARTESIAN_POINT('Ctrl Pts',(3.25666900829462,5.93181219952329,34.6428503495116));
#192052=CARTESIAN_POINT('Ctrl Pts',(3.20450735387843,5.96044986330035,34.6456450375789));
#192053=CARTESIAN_POINT('Ctrl Pts',(3.15197964667623,5.98839301292847,34.6484397256462));
#192054=CARTESIAN_POINT('Ctrl Pts',(3.09910619832129,6.01563211736943,34.6512344137135));
#192055=CARTESIAN_POINT('Origin',(0.,0.,4.30282021618968));
#192056=CARTESIAN_POINT('',(3.09910619832131,6.01563211736941,37.0458284616795));
#192057=CARTESIAN_POINT('',(3.0991061983213,6.01563211736942,36.6515010185242));
#192058=CARTESIAN_POINT('',(3.09910619832133,6.0156321173694,4.30282021618968));
#192059=CARTESIAN_POINT('',(-6.76699950557411,0.00258680493565955,35.6971797838413));
#192060=CARTESIAN_POINT('Ctrl Pts',(-6.76699950557411,0.00258680493565955,
35.6971797838413));
#192061=CARTESIAN_POINT('Ctrl Pts',(-6.76706491533245,-0.168523044232433,
35.7052286768605));
#192062=CARTESIAN_POINT('Ctrl Pts',(-6.76063604028297,-0.339784646345535,
35.7132775698797));
#192063=CARTESIAN_POINT('Ctrl Pts',(-6.74770474594979,-0.510656108831311,
35.7213264628988));
#192064=CARTESIAN_POINT('Ctrl Pts',(-6.7347794102295,-0.681448835432342,
35.7293716470675));
#192065=CARTESIAN_POINT('Ctrl Pts',(-6.71535764621149,-0.851851407750275,
35.7374168312361));
#192066=CARTESIAN_POINT('Ctrl Pts',(-6.68948339477062,-1.02132311786633,
35.7454620154047));
#192067=CARTESIAN_POINT('Ctrl Pts',(-6.66361188957647,-1.19077684055841,
35.7535063456719));
#192068=CARTESIAN_POINT('Ctrl Pts',(-6.63128930707785,-1.35929952639152,
35.7615506759391));
#192069=CARTESIAN_POINT('Ctrl Pts',(-6.59261134108946,-1.52635667697255,
35.7695950062063));
#192070=CARTESIAN_POINT('Ctrl Pts',(-6.55615347216897,-1.6838248256322,
35.7771775956973));
#192071=CARTESIAN_POINT('Ctrl Pts',(-6.51404935939128,-1.83999064974016,
35.7847601851882));
#192072=CARTESIAN_POINT('Ctrl Pts',(-6.46642052635441,-1.99441584839831,
35.7923427746792));
#192073=CARTESIAN_POINT('Ctrl Pts',(-6.41228302112202,-2.16994387348973,
35.8009615556164));
#192074=CARTESIAN_POINT('Ctrl Pts',(-6.35101420069501,-2.34320222199084,
35.8095803365536));
#192075=CARTESIAN_POINT('Ctrl Pts',(-6.2828357778544,-2.51361564056893,
35.8181991174909));
#192076=CARTESIAN_POINT('Ctrl Pts',(-6.2146164006499,-2.68413142545095,
35.8268230756774));
#192077=CARTESIAN_POINT('Ctrl Pts',(-6.13947925076779,-2.85179858749008,
35.8354470338639));
#192078=CARTESIAN_POINT('Ctrl Pts',(-6.05769372457999,-3.01606295345178,
35.8440709920504));
#192079=CARTESIAN_POINT('Ctrl Pts',(-5.97295356638063,-3.18626163049089,
35.8530065044216));
#192080=CARTESIAN_POINT('Ctrl Pts',(-5.88107587592368,-3.35280674405556,
35.8619420167927));
#192081=CARTESIAN_POINT('Ctrl Pts',(-5.78241129609706,-3.51511146377596,
35.8708775291638));
#192082=CARTESIAN_POINT('Ctrl Pts',(-5.68700881503044,-3.67204998190839,
35.8795176110585));
#192083=CARTESIAN_POINT('Ctrl Pts',(-5.58526125217604,-3.82502378651878,
35.8881576929532));
#192084=CARTESIAN_POINT('Ctrl Pts',(-5.4775290364657,-3.97353301920031,
35.8967977748479));
#192085=CARTESIAN_POINT('Ctrl Pts',(-5.36427128635596,-4.12965922019907,
35.9058810024572));
#192086=CARTESIAN_POINT('Ctrl Pts',(-5.24439910264273,-4.28085054005772,
35.9149642300665));
#192087=CARTESIAN_POINT('Ctrl Pts',(-5.11837854143579,-4.42656640146397,
35.9240474576759));
#192088=CARTESIAN_POINT('Ctrl Pts',(-4.99235798022887,-4.57228226287019,
35.9331306852852));
#192089=CARTESIAN_POINT('Ctrl Pts',(-4.86018933197781,-4.71252240670671,
35.9422139128946));
#192090=CARTESIAN_POINT('Ctrl Pts',(-4.72238299435586,-4.84679150104671,
35.9512971405039));
#192091=CARTESIAN_POINT('Ctrl Pts',(-4.58516277413118,-4.98048952257928,
35.9603417353637));
#192092=CARTESIAN_POINT('Ctrl Pts',(-4.44222661118032,-5.1083912730571,
35.9693863302235));
#192093=CARTESIAN_POINT('Ctrl Pts',(-4.29406512608389,-5.23003763781392,
35.9784309250834));
#192094=CARTESIAN_POINT('Ctrl Pts',(-4.146039602472,-5.35157237288282,35.9874672201037));
#192095=CARTESIAN_POINT('Ctrl Pts',(-3.99279851377013,-5.46686303194261,
35.996503515124));
#192096=CARTESIAN_POINT('Ctrl Pts',(-3.83486637478639,-5.5754900132215,
36.0055398101443));
#192097=CARTESIAN_POINT('Ctrl Pts',(-3.67721370910681,-5.68392477053905,
36.014560114732));
#192098=CARTESIAN_POINT('Ctrl Pts',(-3.51488676529724,-5.78571926235838,
36.0235804193198));
#192099=CARTESIAN_POINT('Ctrl Pts',(-3.34843974226654,-5.88049660253367,
36.0326007239075));
#192100=CARTESIAN_POINT('Ctrl Pts',(-3.18220232692764,-5.97515458906028,
36.0416096691738));
#192101=CARTESIAN_POINT('Ctrl Pts',(-3.01185539281924,-6.06281294167381,
36.0506186144402));
#192102=CARTESIAN_POINT('Ctrl Pts',(-2.83798065817008,-6.14313883807395,
36.0596275597065));
#192103=CARTESIAN_POINT('Ctrl Pts',(-2.66450075623476,-6.22328233136801,
36.0686160475653));
#192104=CARTESIAN_POINT('Ctrl Pts',(-2.48750925974602,-6.29612650461054,
36.0776045354241));
#192105=CARTESIAN_POINT('Ctrl Pts',(-2.30761048321135,-6.36138529392561,
36.0865930232829));
#192106=CARTESIAN_POINT('Ctrl Pts',(-2.14977406617603,-6.4186409000168,
36.0944791842982));
#192107=CARTESIAN_POINT('Ctrl Pts',(-1.98970020554991,-6.47005814533542,
36.1023653453134));
#192108=CARTESIAN_POINT('Ctrl Pts',(-1.82781204343855,-6.51547328548441,
36.1102515063287));
#192109=CARTESIAN_POINT('Ctrl Pts',(-1.66109353278753,-6.56224350282395,
36.1183729711848));
#192110=CARTESIAN_POINT('Ctrl Pts',(-1.49252502542138,-6.60262558404109,
36.126494436041));
#192111=CARTESIAN_POINT('Ctrl Pts',(-1.32264204275989,-6.63648303145001,
36.1346159008972));
#192112=CARTESIAN_POINT('Ctrl Pts',(-1.15277117525538,-6.67033806432463,
36.1427367865734));
#192113=CARTESIAN_POINT('Ctrl Pts',(-0.981586378299208,-6.69766931863469,
36.1508576722496));
#192114=CARTESIAN_POINT('Ctrl Pts',(-0.809633717570386,-6.71839134342241,
36.1589785579257));
#192115=CARTESIAN_POINT('Ctrl Pts',(-0.637660503579715,-6.73911584508487,
36.1671004142801));
#192116=CARTESIAN_POINT('Ctrl Pts',(-0.464919606751438,-6.75322950155105,
36.1752222706344));
#192117=CARTESIAN_POINT('Ctrl Pts',(-0.29196252402161,-6.7606986979577,
36.1833441269888));
#192118=CARTESIAN_POINT('Ctrl Pts',(-0.118879253945957,-6.76817334379755,
36.1914719089489));
#192119=CARTESIAN_POINT('Ctrl Pts',(0.0544201508324774,-6.76899383155364,
36.1995996909091));
#192120=CARTESIAN_POINT('Ctrl Pts',(0.227383234888612,-6.76317868050901,
36.2077274728692));
#192121=CARTESIAN_POINT('Ctrl Pts',(0.400416777676826,-6.75736116058797,
36.2158585657857));
#192122=CARTESIAN_POINT('Ctrl Pts',(0.573113361673498,-6.74490264013385,
36.2239896587021));
#192123=CARTESIAN_POINT('Ctrl Pts',(0.744925594969273,-6.72587353865352,
36.2321207516186));
#192124=CARTESIAN_POINT('Ctrl Pts',(0.916925354137106,-6.70682366770422,
36.2402607192831));
#192125=CARTESIAN_POINT('Ctrl Pts',(1.08803847300764,-6.68118894601193,
36.2484006869477));
#192126=CARTESIAN_POINT('Ctrl Pts',(1.25772694295228,-6.64909106096254,
36.2565406546122));
#192127=CARTESIAN_POINT('Ctrl Pts',(1.34573472032298,-6.63244370995266,
36.2607623937926));
#192128=CARTESIAN_POINT('Ctrl Pts',(1.43335949671735,-6.61405865640257,
36.264984132973));
#192129=CARTESIAN_POINT('Ctrl Pts',(1.52052787674695,-6.59395814181705,
36.2692058721534));
#192130=CARTESIAN_POINT('Ctrl Pts',(1.69479714211257,-6.55377267652449,
36.277646081611));
#192131=CARTESIAN_POINT('Ctrl Pts',(1.86760150681647,-6.50664466348891,
36.2860862910686));
#192132=CARTESIAN_POINT('Ctrl Pts',(2.03836801823528,-6.45270058364989,
36.2945265005263));
#192133=CARTESIAN_POINT('Ctrl Pts',(2.20900514872209,-6.39879737444333,
36.3029603152748));
#192134=CARTESIAN_POINT('Ctrl Pts',(2.37760718688367,-6.33808849297188,
36.3113941300233));
#192135=CARTESIAN_POINT('Ctrl Pts',(2.54361417096903,-6.27075082819,36.3198279447718));
#192136=CARTESIAN_POINT('Ctrl Pts',(2.70952089990792,-6.20345383005527,
36.3282566661604));
#192137=CARTESIAN_POINT('Ctrl Pts',(2.87283539097089,-6.12953615472672,
36.3366853875489));
#192138=CARTESIAN_POINT('Ctrl Pts',(3.03301519935228,-6.04922373536457,
36.3451141089374));
#192139=CARTESIAN_POINT('Ctrl Pts',(3.19312286862617,-5.96894748576883,
36.3535390343391));
#192140=CARTESIAN_POINT('Ctrl Pts',(3.35009837246566,-5.88228238367233,
36.3619639597408));
#192141=CARTESIAN_POINT('Ctrl Pts',(3.50342116444249,-5.78950163179323,
36.3703888851426));
#192142=CARTESIAN_POINT('Ctrl Pts',(3.65669842971953,-5.69674842964357,
36.3788113089002));
#192143=CARTESIAN_POINT('Ctrl Pts',(3.80632486108276,-5.59788337156605,
36.3872337326579));
#192144=CARTESIAN_POINT('Ctrl Pts',(3.95180601000119,-5.49322475958508,
36.3956561564156));
#192145=CARTESIAN_POINT('Ctrl Pts',(4.09728944692012,-5.38856450162481,
36.4040787126338));
#192146=CARTESIAN_POINT('Ctrl Pts',(4.23862719660897,-5.27811069700969,
36.412501268852));
#192147=CARTESIAN_POINT('Ctrl Pts',(4.37535467090177,-5.16222437557862,
36.4209238250702));
#192148=CARTESIAN_POINT('Ctrl Pts',(4.51208676387452,-5.04633413948569,
36.4293466658039));
#192149=CARTESIAN_POINT('Ctrl Pts',(4.64420801634832,-4.92501123622479,
36.4377695065377));
#192150=CARTESIAN_POINT('Ctrl Pts',(4.77128764190422,-4.79865639926554,
36.4461923472714));
#192151=CARTESIAN_POINT('Ctrl Pts',(4.89838930195545,-4.67227965348295,
36.4546166484521));
#192152=CARTESIAN_POINT('Ctrl Pts',(5.02044735570816,-4.54086946969294,
36.4630409496327));
#192153=CARTESIAN_POINT('Ctrl Pts',(5.13706829083558,-4.40486303706388,
36.4714652508134));
#192154=CARTESIAN_POINT('Ctrl Pts',(5.25372573357491,-4.26881402828797,
36.4798921891802));
#192155=CARTESIAN_POINT('Ctrl Pts',(5.36494244719491,-4.12816615515036,
36.488319127547));
#192156=CARTESIAN_POINT('Ctrl Pts',(5.47036534831931,-3.98338950592424,
36.4967460659138));
#192157=CARTESIAN_POINT('Ctrl Pts',(5.57588303788324,-3.83848268429237,
36.5051805811575));
#192158=CARTESIAN_POINT('Ctrl Pts',(5.67559630927362,-3.68943993873915,
36.5136150964012));
#192159=CARTESIAN_POINT('Ctrl Pts',(5.76919491301089,-3.53676109677899,
36.5220496116448));
#192160=CARTESIAN_POINT('Ctrl Pts',(5.86283872567579,-3.38400850962989,
36.5304882008316));
#192161=CARTESIAN_POINT('Ctrl Pts',(5.95036181311914,-3.22761661180973,
36.5389267900184));
#192162=CARTESIAN_POINT('Ctrl Pts',(6.03149977166802,-3.06811008674209,
36.5473653792052));
#192163=CARTESIAN_POINT('Ctrl Pts',(6.11272842409734,-2.90842526946731,
36.5558134008255));
#192164=CARTESIAN_POINT('Ctrl Pts',(6.18755754249105,-2.7456191693734,36.5642614224458));
#192165=CARTESIAN_POINT('Ctrl Pts',(6.25577027609986,-2.58023782870215,
36.5727094440661));
#192166=CARTESIAN_POINT('Ctrl Pts',(6.29454129918217,-2.48623772876007,
36.5775111639784));
#192167=CARTESIAN_POINT('Ctrl Pts',(6.33117572478765,-2.39140600253605,
36.5823128838907));
#192168=CARTESIAN_POINT('Ctrl Pts',(6.36564090235695,-2.29584513899352,
36.587114603803));
#192169=CARTESIAN_POINT('Ctrl Pts',(6.42478157143281,-2.13186706587876,
36.5953541356538));
#192170=CARTESIAN_POINT('Ctrl Pts',(6.47766405255244,-1.96537515686491,
36.6035936675047));
#192171=CARTESIAN_POINT('Ctrl Pts',(6.52407000662113,-1.79688607004079,
36.6118331993555));
#192172=CARTESIAN_POINT('Ctrl Pts',(6.57042445332396,-1.62858399432788,
36.6200635859018));
#192173=CARTESIAN_POINT('Ctrl Pts',(6.61031659279737,-1.45828949478854,
36.6282939724482));
#192174=CARTESIAN_POINT('Ctrl Pts',(6.64357647031582,-1.28653825557814,
36.6365243589945));
#192175=CARTESIAN_POINT('Ctrl Pts',(6.67680536495121,-1.11494700939706,
36.6447470786123));
#192176=CARTESIAN_POINT('Ctrl Pts',(6.70341423438039,-0.941902073415117,
36.6529697982301));
#192177=CARTESIAN_POINT('Ctrl Pts',(6.72328316872599,-0.767953405569558,
36.6611925178479));
#192178=CARTESIAN_POINT('Ctrl Pts',(6.74313449776428,-0.594158868776013,
36.6694079515437));
#192179=CARTESIAN_POINT('Ctrl Pts',(6.75625775437691,-0.419462548391257,
36.6776233852395));
#192180=CARTESIAN_POINT('Ctrl Pts',(6.76258427853708,-0.244423557954591,
36.6858388189353));
#192181=CARTESIAN_POINT('Ctrl Pts',(6.76890755135511,-0.069474523966355,
36.6940500305361));
#192182=CARTESIAN_POINT('Ctrl Pts',(6.76844103549978,0.10581647453887,36.702261242137));
#192183=CARTESIAN_POINT('Ctrl Pts',(6.76116795752074,0.280885831246064,
36.7104724537378));
#192184=CARTESIAN_POINT('Ctrl Pts',(6.75389731853075,0.455896479350804,
36.7186809117514));
#192185=CARTESIAN_POINT('Ctrl Pts',(6.73982467920251,0.630685278503534,
36.7268893697649));
#192186=CARTESIAN_POINT('Ctrl Pts',(6.71898536681812,0.804689157677629,
36.7350978277784));
#192187=CARTESIAN_POINT('Ctrl Pts',(6.70970099810832,0.882211685359438,
36.7387548750615));
#192188=CARTESIAN_POINT('Ctrl Pts',(6.69907420526101,0.959578446429873,
36.7424119223446));
#192189=CARTESIAN_POINT('Ctrl Pts',(6.68711143303382,1.03673992987072,36.7460689696277));
#192190=CARTESIAN_POINT('Ctrl Pts',(6.65813201923183,1.22366103107891,36.7549280438036));
#192191=CARTESIAN_POINT('Ctrl Pts',(6.62133949993905,1.40918267875476,36.7637871179795));
#192192=CARTESIAN_POINT('Ctrl Pts',(6.57690487306358,1.59267425755317,36.7726461921554));
#192193=CARTESIAN_POINT('Ctrl Pts',(6.53238676246426,1.77651058011047,36.7815219107493));
#192194=CARTESIAN_POINT('Ctrl Pts',(6.48019791169681,1.9583089595996,36.7903976293432));
#192195=CARTESIAN_POINT('Ctrl Pts',(6.42055893068183,2.13745456504736,36.799273347937));
#192196=CARTESIAN_POINT('Ctrl Pts',(6.36074975686555,2.3171114014369,36.808174395324));
#192197=CARTESIAN_POINT('Ctrl Pts',(6.29344798985411,2.49410006711822,36.817075442711));
#192198=CARTESIAN_POINT('Ctrl Pts',(6.21892329917187,2.66782345724325,36.825976490098));
#192199=CARTESIAN_POINT('Ctrl Pts',(6.14429729115033,2.84178302670024,36.834889638581));
#192200=CARTESIAN_POINT('Ctrl Pts',(6.06242885224265,3.01246821742171,36.843802787064));
#192201=CARTESIAN_POINT('Ctrl Pts',(5.97363397466996,3.17930592058531,36.852715935547));
#192202=CARTESIAN_POINT('Ctrl Pts',(5.8846419481887,3.34651404907056,36.8616488736568));
#192203=CARTESIAN_POINT('Ctrl Pts',(5.78869284534651,3.50985737369966,36.8705818117667));
#192204=CARTESIAN_POINT('Ctrl Pts',(5.68614791999638,3.66878874179488,36.8795147498766));
#192205=CARTESIAN_POINT('Ctrl Pts',(5.58854001945675,3.82006836013483,36.8880176117352));
#192206=CARTESIAN_POINT('Ctrl Pts',(5.4849565601488,3.96735069595758,36.8965204735938));
#192207=CARTESIAN_POINT('Ctrl Pts',(5.37574326378257,4.11019140209995,36.9050233354524));
#192208=CARTESIAN_POINT('Ctrl Pts',(5.27012059960917,4.24833589949314,36.913246646647));
#192209=CARTESIAN_POINT('Ctrl Pts',(5.15902895751334,4.38259021076979,36.9214699578416));
#192210=CARTESIAN_POINT('Ctrl Pts',(5.0427851812063,4.5124945004073,36.9296932690362));
#192211=CARTESIAN_POINT('Ctrl Pts',(4.92666151119018,4.64226456933298,36.9379080836778));
#192212=CARTESIAN_POINT('Ctrl Pts',(4.80539654369622,4.7676933006627,36.9461228983194));
#192213=CARTESIAN_POINT('Ctrl Pts',(4.67934914740928,4.88835151729498,36.954337712961));
#192214=CARTESIAN_POINT('Ctrl Pts',(4.55343102504504,5.00888598713493,36.9625441025074));
#192215=CARTESIAN_POINT('Ctrl Pts',(4.42274050632266,5.12465944592435,36.9707504920537));
#192216=CARTESIAN_POINT('Ctrl Pts',(4.2876751231104,5.23527755125363,36.9789568816001));
#192217=CARTESIAN_POINT('Ctrl Pts',(4.15269036318479,5.3458296263759,36.9871583725849));
#192218=CARTESIAN_POINT('Ctrl Pts',(4.01333621478219,5.45123224877674,36.9953598635698));
#192219=CARTESIAN_POINT('Ctrl Pts',(3.87004562352525,5.55112924294085,37.0035613545546));
#192220=CARTESIAN_POINT('Ctrl Pts',(3.72681512970077,5.65098433935852,37.0117594057563));
#192221=CARTESIAN_POINT('Ctrl Pts',(3.57965177466728,5.74533820145981,37.019957456958));
#192222=CARTESIAN_POINT('Ctrl Pts',(3.42902005282767,5.83387611089795,37.0281555081598));
#192223=CARTESIAN_POINT('Ctrl Pts',(3.32077857961416,5.89749799369786,37.0340464926663));
#192224=CARTESIAN_POINT('Ctrl Pts',(3.21074685607432,5.95811758727905,37.0399374771729));
#192225=CARTESIAN_POINT('Ctrl Pts',(3.09910619832131,6.01563211736941,37.0458284616795));
#192226=CARTESIAN_POINT('Ctrl Pts',(3.09910619832134,6.0156321173694,35.0460577214446));
#192227=CARTESIAN_POINT('Ctrl Pts',(2.94708384676306,6.09395030618239,35.0541086516326));
#192228=CARTESIAN_POINT('Ctrl Pts',(2.79189904270229,6.16660071990929,35.0621595818206));
#192229=CARTESIAN_POINT('Ctrl Pts',(2.63402271304241,6.23331479609178,35.0702105120086));
#192230=CARTESIAN_POINT('Ctrl Pts',(2.47627391386713,6.2999749814948,35.0782549387579));
#192231=CARTESIAN_POINT('Ctrl Pts',(2.31583825840021,6.3607082290828,35.0862993655072));
#192232=CARTESIAN_POINT('Ctrl Pts',(2.15321099490439,6.41529199736246,35.0943437922565));
#192233=CARTESIAN_POINT('Ctrl Pts',(1.9906795021762,6.46984362140459,35.1023834816641));
#192234=CARTESIAN_POINT('Ctrl Pts',(1.82595932353737,6.51825285686615,35.1104231710717));
#192235=CARTESIAN_POINT('Ctrl Pts',(1.65956529319152,6.56034542060357,35.1184628604792));
#192236=CARTESIAN_POINT('Ctrl Pts',(1.48966640925584,6.60332460432857,35.1266718945095));
#192237=CARTESIAN_POINT('Ctrl Pts',(1.31802274300623,6.63971790327552,35.1348809285397));
#192238=CARTESIAN_POINT('Ctrl Pts',(1.14519870426525,6.66939344526541,35.1430899625699));
#192239=CARTESIAN_POINT('Ctrl Pts',(0.975994003012665,6.69844751235866,
35.1511270803273));
#192240=CARTESIAN_POINT('Ctrl Pts',(0.805658264584453,6.72106235791392,
35.1591641980846));
#192241=CARTESIAN_POINT('Ctrl Pts',(0.634730995471674,6.73716598900365,
35.1672013158419));
#192242=CARTESIAN_POINT('Ctrl Pts',(0.463785519346714,6.75327133543704,
35.1752392897055));
#192243=CARTESIAN_POINT('Ctrl Pts',(0.29224875906145,6.76286405125259,35.183277263569));
#192244=CARTESIAN_POINT('Ctrl Pts',(0.120664526296393,6.76592411072528,
35.1913152374326));
#192245=CARTESIAN_POINT('Ctrl Pts',(-0.0509719806591898,6.76898510246389,
35.1993556601143));
#192246=CARTESIAN_POINT('Ctrl Pts',(-0.222655615537248,6.76550946970699,
35.2073960827959));
#192247=CARTESIAN_POINT('Ctrl Pts',(-0.393843536411067,6.75552931078145,
35.2154365054776));
#192248=CARTESIAN_POINT('Ctrl Pts',(-0.571344388912239,6.745181111514,35.2237734364549));
#192249=CARTESIAN_POINT('Ctrl Pts',(-0.74831182610218,6.7278395231367,35.2321103674321));
#192250=CARTESIAN_POINT('Ctrl Pts',(-0.924148767020826,6.70359888838927,
35.2404472984094));
#192251=CARTESIAN_POINT('Ctrl Pts',(-1.09403149957942,6.68017909247874,
35.2485019233828));
#192252=CARTESIAN_POINT('Ctrl Pts',(-1.26285869709422,6.65031998160127,
35.2565565483562));
#192253=CARTESIAN_POINT('Ctrl Pts',(-1.43010484633272,6.61415823279846,
35.2646111733296));
#192254=CARTESIAN_POINT('Ctrl Pts',(-1.60614369396661,6.57609533797752,
35.2730892573088));
#192255=CARTESIAN_POINT('Ctrl Pts',(-1.78043028805679,6.531049369789,35.281567341288));
#192256=CARTESIAN_POINT('Ctrl Pts',(-1.95237352217877,6.47923812109844,
35.2900454252672));
#192257=CARTESIAN_POINT('Ctrl Pts',(-2.12431675630074,6.42742687240789,
35.2985235092464));
#192258=CARTESIAN_POINT('Ctrl Pts',(-2.29391621380858,6.36885058085278,
35.3070015932256));
#192259=CARTESIAN_POINT('Ctrl Pts',(-2.46060943853249,6.30378379951318,
35.3154796772048));
#192260=CARTESIAN_POINT('Ctrl Pts',(-2.6244485383512,6.23983109297434,35.3238125992515));
#192261=CARTESIAN_POINT('Ctrl Pts',(-2.78600320925251,6.16940483780113,
35.3321455212982));
#192262=CARTESIAN_POINT('Ctrl Pts',(-2.9447334664738,6.09268691230964,35.3404784433449));
#192263=CARTESIAN_POINT('Ctrl Pts',(-3.10327614302356,6.01605964880179,
35.3488015178985));
#192264=CARTESIAN_POINT('Ctrl Pts',(-3.25900074439442,5.93315567665279,
35.3571245924521));
#192265=CARTESIAN_POINT('Ctrl Pts',(-3.41138522679582,5.84420566325307,
35.3654476670058));
#192266=CARTESIAN_POINT('Ctrl Pts',(-3.56361759873903,5.75534443991308,
35.3737624334517));
#192267=CARTESIAN_POINT('Ctrl Pts',(-3.71251619570537,5.6604493736353,35.3820771998977));
#192268=CARTESIAN_POINT('Ctrl Pts',(-3.85758144512978,5.55979805336403,
35.3903919663436));
#192269=CARTESIAN_POINT('Ctrl Pts',(-4.00252850001729,5.45922874057722,
35.3986999581832));
#192270=CARTESIAN_POINT('Ctrl Pts',(-4.14364814613331,5.35291271652895,
35.4070079500227));
#192271=CARTESIAN_POINT('Ctrl Pts',(-4.28046761265466,5.24117219875617,
35.4153159418623));
#192272=CARTESIAN_POINT('Ctrl Pts',(-4.41720068664815,5.12950223779844,
35.4236186877493));
#192273=CARTESIAN_POINT('Ctrl Pts',(-4.5496387235486,5.01241482863005,35.4319214336364));
#192274=CARTESIAN_POINT('Ctrl Pts',(-4.67733984520325,4.8902741203816,35.4402241795235));
#192275=CARTESIAN_POINT('Ctrl Pts',(-4.804988779479,4.7681833271483,35.4485235323429));
#192276=CARTESIAN_POINT('Ctrl Pts',(-4.92790440474795,4.64104358985111,
35.4568228851624));
#192277=CARTESIAN_POINT('Ctrl Pts',(-5.04567950172157,4.50925796178338,
35.4651222379818));
#192278=CARTESIAN_POINT('Ctrl Pts',(-5.16342954990833,4.37750036230737,
35.4734198256682));
#192279=CARTESIAN_POINT('Ctrl Pts',(-5.27604101621247,4.24109909984328,
35.4817174133545));
#192280=CARTESIAN_POINT('Ctrl Pts',(-5.38314483868581,4.10049273206652,
35.4900150010409));
#192281=CARTESIAN_POINT('Ctrl Pts',(-5.4902436799781,3.95989290360609,35.4983122028233));
#192282=CARTESIAN_POINT('Ctrl Pts',(-5.59183517720703,3.81508863639148,
35.5066094046057));
#192283=CARTESIAN_POINT('Ctrl Pts',(-5.68759161547871,3.66655023360328,
35.5149066063881));
#192284=CARTESIAN_POINT('Ctrl Pts',(-5.78335951195384,3.51799405672836,
35.5232048010126));
#192285=CARTESIAN_POINT('Ctrl Pts',(-5.87329077019387,3.3657031466418,35.5315029956372));
#192286=CARTESIAN_POINT('Ctrl Pts',(-5.95710183292946,3.21017550176131,
35.5398011902617));
#192287=CARTESIAN_POINT('Ctrl Pts',(-6.0409718409626,3.05453847247494,35.5481052211033));
#192288=CARTESIAN_POINT('Ctrl Pts',(-6.11871288720063,2.89566046627381,
35.5564092519449));
#192289=CARTESIAN_POINT('Ctrl Pts',(-6.19008768987053,2.73406353103095,
35.5647132827864));
#192290=CARTESIAN_POINT('Ctrl Pts',(-6.26148844638324,2.57240783469454,
35.5730203332022));
#192291=CARTESIAN_POINT('Ctrl Pts',(-6.3265182115725,2.40803155994252,35.5813273836179));
#192292=CARTESIAN_POINT('Ctrl Pts',(-6.38498837166966,2.24147551707423,
35.5896344340337));
#192293=CARTESIAN_POINT('Ctrl Pts',(-6.443521046236,2.07474139768638,35.5979503660883));
#192294=CARTESIAN_POINT('Ctrl Pts',(-6.49547999468642,1.90582318462834,
35.6062662981429));
#192295=CARTESIAN_POINT('Ctrl Pts',(-6.54072656130306,1.73527664948983,
35.6145822301976));
#192296=CARTESIAN_POINT('Ctrl Pts',(-6.5748343842871,1.60671504877589,35.6208509564165));
#192297=CARTESIAN_POINT('Ctrl Pts',(-6.60512895506477,1.47722846531531,
35.6271196826355));
#192298=CARTESIAN_POINT('Ctrl Pts',(-6.63157020267617,1.34705814535883,
35.6333884088544));
#192299=CARTESIAN_POINT('Ctrl Pts',(-6.67246149404957,1.14575022828408,
35.6430829707043));
#192300=CARTESIAN_POINT('Ctrl Pts',(-6.70419740181038,0.942504625848324,
35.6527775325543));
#192301=CARTESIAN_POINT('Ctrl Pts',(-6.72662719127631,0.738089174546172,
35.6624720944042));
#192302=CARTESIAN_POINT('Ctrl Pts',(-6.74895889811254,0.534567606133308,
35.6721242631626));
#192303=CARTESIAN_POINT('Ctrl Pts',(-6.7620656592192,0.329886476403177,
35.6817764319209));
#192304=CARTESIAN_POINT('Ctrl Pts',(-6.76584879210263,0.124816354711093,
35.6914286006792));
#192305=CARTESIAN_POINT('Ctrl Pts',(-6.76660017729443,0.0840864471273353,
35.6933456617228));
#192306=CARTESIAN_POINT('Ctrl Pts',(-6.76698392647106,0.0433412329773021,
35.6952627227665));
#192307=CARTESIAN_POINT('Ctrl Pts',(-6.76699950557385,0.00258680559947647,
35.6971797838101));
#192308=CARTESIAN_POINT('',(-6.76699947070562,-0.00267646592832112,35.302820216152));
#192309=CARTESIAN_POINT('Ctrl Pts',(3.09910619832129,6.01563211736943,34.6512344137135));
#192310=CARTESIAN_POINT('Ctrl Pts',(2.94524428385927,6.09489800389497,34.6593669654902));
#192311=CARTESIAN_POINT('Ctrl Pts',(2.78845331533177,6.16819833692683,34.6674995172669));
#192312=CARTESIAN_POINT('Ctrl Pts',(2.62924644675822,6.23533095530697,34.6756320690436));
#192313=CARTESIAN_POINT('Ctrl Pts',(2.46987617618944,6.30253247526081,34.6837729676661));
#192314=CARTESIAN_POINT('Ctrl Pts',(2.30808539730431,6.36355351502733,34.6919138662887));
#192315=CARTESIAN_POINT('Ctrl Pts',(2.14440346720432,6.4182414078813,34.7000547649112));
#192316=CARTESIAN_POINT('Ctrl Pts',(2.11572748325503,6.42782236246036,34.7014809961274));
#192317=CARTESIAN_POINT('Ctrl Pts',(2.08699348323649,6.43720906171219,34.7029072273436));
#192318=CARTESIAN_POINT('Ctrl Pts',(2.05820434701039,6.44640084589436,34.7043334585597));
#192319=CARTESIAN_POINT('Ctrl Pts',(1.88783481849595,6.50079636248869,34.7127736680173));
#192320=CARTESIAN_POINT('Ctrl Pts',(1.71518132090391,6.5484741124627,34.721213877475));
#192321=CARTESIAN_POINT('Ctrl Pts',(1.5408011074484,6.58925040860383,34.7296540869326));
#192322=CARTESIAN_POINT('Ctrl Pts',(1.36655301283911,6.62999581065961,34.7380879016811));
#192323=CARTESIAN_POINT('Ctrl Pts',(1.19058113381837,6.663850106632,34.7465217164297));
#192324=CARTESIAN_POINT('Ctrl Pts',(1.01345728211852,6.6906795871063,34.7549555311782));
#192325=CARTESIAN_POINT('Ctrl Pts',(0.836440399277796,6.71749286468704,
34.7633842525668));
#192326=CARTESIAN_POINT('Ctrl Pts',(0.658273259633997,6.73728973485391,
34.7718129739553));
#192327=CARTESIAN_POINT('Ctrl Pts',(0.479537645247769,6.74998760345456,
34.7802416953438));
#192328=CARTESIAN_POINT('Ctrl Pts',(0.30088252682305,6.76267975340118,34.7886666207456));
#192329=CARTESIAN_POINT('Ctrl Pts',(0.121659776223405,6.76827925290529,
34.7970915461473));
#192330=CARTESIAN_POINT('Ctrl Pts',(-0.0575435276757699,6.76675533342404,
34.8055164715491));
#192331=CARTESIAN_POINT('Ctrl Pts',(-0.236693620080711,6.76523186644578,
34.8139388953068));
#192332=CARTESIAN_POINT('Ctrl Pts',(-0.41582394418443,6.75658920145334,
34.8223613190645));
#192333=CARTESIAN_POINT('Ctrl Pts',(-0.59434684330733,6.74084867281937,
34.8307837428223));
#192334=CARTESIAN_POINT('Ctrl Pts',(-0.772872550081101,6.72510789663223,
34.8392062990405));
#192335=CARTESIAN_POINT('Ctrl Pts',(-0.950790480090896,6.70226905642334,
34.8476288552587));
#192336=CARTESIAN_POINT('Ctrl Pts',(-1.12751684475177,6.67240547065307,
34.8560514114769));
#192337=CARTESIAN_POINT('Ctrl Pts',(-1.30424917926287,6.64254087608519,
34.8644742522106));
#192338=CARTESIAN_POINT('Ctrl Pts',(-1.47978953922511,6.60565111822101,
34.8728970929444));
#192339=CARTESIAN_POINT('Ctrl Pts',(-1.65356293705119,6.56186091084005,
34.8813199336781));
#192340=CARTESIAN_POINT('Ctrl Pts',(-1.82736646566389,6.51806311062032,
34.8897442348588));
#192341=CARTESIAN_POINT('Ctrl Pts',(-1.99940209787068,6.46736255696685,
34.8981685360394));
#192342=CARTESIAN_POINT('Ctrl Pts',(-2.16910829085744,6.40993433839486,
34.90659283722));
#192343=CARTESIAN_POINT('Ctrl Pts',(-2.33886760953542,6.35248814220076,
34.9150197755868));
#192344=CARTESIAN_POINT('Ctrl Pts',(-2.50629571928938,6.28831018905033,
34.9234467139536));
#192345=CARTESIAN_POINT('Ctrl Pts',(-2.67084905039007,6.21762449413202,
34.9318736523204));
#192346=CARTESIAN_POINT('Ctrl Pts',(-2.83555033561984,6.14687524388876,
34.9403081675641));
#192347=CARTESIAN_POINT('Ctrl Pts',(-2.99737137060435,6.06960669187759,
34.9487426828077));
#192348=CARTESIAN_POINT('Ctrl Pts',(-3.15579023964393,5.98609029027863,
34.9571771980514));
#192349=CARTESIAN_POINT('Ctrl Pts',(-3.3142856263542,5.90253354954234,34.9656157872381));
#192350=CARTESIAN_POINT('Ctrl Pts',(-3.46937527873959,5.81272310325608,
34.9740543764249));
#192351=CARTESIAN_POINT('Ctrl Pts',(-3.62056401772094,5.71697517867486,
34.9824929656117));
#192352=CARTESIAN_POINT('Ctrl Pts',(-3.77192175150706,5.62112022957626,
34.990940987232));
#192353=CARTESIAN_POINT('Ctrl Pts',(-3.91936958179618,5.51931472613761,
34.9993890088523));
#192354=CARTESIAN_POINT('Ctrl Pts',(-4.06244231912662,5.41191753482711,
35.0078370304726));
#192355=CARTESIAN_POINT('Ctrl Pts',(-4.14376256694475,5.35087469483328,
35.0126387503848));
#192356=CARTESIAN_POINT('Ctrl Pts',(-4.2236699951816,5.28802614393199,35.017440470297));
#192357=CARTESIAN_POINT('Ctrl Pts',(-4.30208421375348,5.22344334876652,
35.0222421902092));
#192358=CARTESIAN_POINT('Ctrl Pts',(-4.43663942798737,5.11262222477164,
35.0304817220601));
#192359=CARTESIAN_POINT('Ctrl Pts',(-4.56709622751511,4.99644504958966,
35.0387212539109));
#192360=CARTESIAN_POINT('Ctrl Pts',(-4.69300314149685,4.87524466195295,
35.0469607857617));
#192361=CARTESIAN_POINT('Ctrl Pts',(-4.81877030760365,4.75417879827588,
35.055191172308));
#192362=CARTESIAN_POINT('Ctrl Pts',(-4.93999738951996,4.62810106838202,
35.0634215588544));
#192363=CARTESIAN_POINT('Ctrl Pts',(-5.05626481170138,4.49738536862814,
35.0716519454007));
#192364=CARTESIAN_POINT('Ctrl Pts',(-5.1724239262096,4.36679143568583,35.0798746650185));
#192365=CARTESIAN_POINT('Ctrl Pts',(-5.28363234687956,4.23156840150379,
35.0880973846363));
#192366=CARTESIAN_POINT('Ctrl Pts',(-5.38950624703963,4.09212798102904,
35.0963201042541));
#192367=CARTESIAN_POINT('Ctrl Pts',(-5.49528633529622,3.95281111481315,
35.1045355379499));
#192368=CARTESIAN_POINT('Ctrl Pts',(-5.59574110953696,3.80928459269179,
35.1127509716456));
#192369=CARTESIAN_POINT('Ctrl Pts',(-5.69052614062956,3.66199416203954,
35.1209664053414));
#192370=CARTESIAN_POINT('Ctrl Pts',(-5.78526245957638,3.51477942723131,
35.1291776169422));
#192371=CARTESIAN_POINT('Ctrl Pts',(-5.87433464635052,3.36380493489245,
35.1373888285431));
#192372=CARTESIAN_POINT('Ctrl Pts',(-5.95744059692783,3.20954678016635,
35.1456000401439));
#192373=CARTESIAN_POINT('Ctrl Pts',(-6.04051867835514,3.05534035511332,
35.1538084981574));
#192374=CARTESIAN_POINT('Ctrl Pts',(-6.11763434062253,2.89785277426996,
35.1620169561709));
#192375=CARTESIAN_POINT('Ctrl Pts',(-6.18853055543361,2.73758626612288,
35.1702254141845));
#192376=CARTESIAN_POINT('Ctrl Pts',(-6.22011636720662,2.66618403719796,
35.1738824614677));
#192377=CARTESIAN_POINT('Ctrl Pts',(-6.25046829301772,2.59423054496445,
35.1775395087508));
#192378=CARTESIAN_POINT('Ctrl Pts',(-6.27956660306054,2.52177165455691,
35.181196556034));
#192379=CARTESIAN_POINT('Ctrl Pts',(-6.34676898490522,2.35442825853,35.1896424859724));
#192380=CARTESIAN_POINT('Ctrl Pts',(-6.40723500136563,2.18450425283061,
35.1980884159108));
#192381=CARTESIAN_POINT('Ctrl Pts',(-6.46079362546452,2.01256918617895,
35.2065343458492));
#192382=CARTESIAN_POINT('Ctrl Pts',(-6.51443996200314,1.84035254313462,
35.2149941076053));
#192383=CARTESIAN_POINT('Ctrl Pts',(-6.56115619788299,1.66611856781043,
35.2234538693613));
#192384=CARTESIAN_POINT('Ctrl Pts',(-6.60082171080229,1.49045018105308,
35.2319136311174));
#192385=CARTESIAN_POINT('Ctrl Pts',(-6.64052142330933,1.31463033309016,
35.2403806868763));
#192386=CARTESIAN_POINT('Ctrl Pts',(-6.67315822316374,1.13737392599471,
35.2488477426351));
#192387=CARTESIAN_POINT('Ctrl Pts',(-6.69866314743055,0.959271096852089,
35.257314798394));
#192388=CARTESIAN_POINT('Ctrl Pts',(-6.72421360004147,0.780850339814223,
35.2657969685294));
#192389=CARTESIAN_POINT('Ctrl Pts',(-6.74260669113894,0.601580464528102,
35.2742791386648));
#192390=CARTESIAN_POINT('Ctrl Pts',(-6.75382544137001,0.42205557395115,
35.2827613088002));
#192391=CARTESIAN_POINT('Ctrl Pts',(-6.7626689278794,0.280540172037556,
35.2894476112508));
#192392=CARTESIAN_POINT('Ctrl Pts',(-6.7670554533611,0.138866378318778,
35.2961339137014));
#192393=CARTESIAN_POINT('Ctrl Pts',(-6.76699947070562,-0.00267646592831579,
35.302820216152));
#192394=CARTESIAN_POINT('Ctrl Pts',(-6.7669994707053,-0.002676466730765,
35.3028202161899));
#192395=CARTESIAN_POINT('Ctrl Pts',(-6.76689528394057,-0.266095314299261,
35.3152637847462));
#192396=CARTESIAN_POINT('Ctrl Pts',(-6.75140799360082,-0.529171608800042,
35.3277073533025));
#192397=CARTESIAN_POINT('Ctrl Pts',(-6.72066816122544,-0.790511522174531,
35.3401509218588));
#192398=CARTESIAN_POINT('Ctrl Pts',(-6.7003552459903,-0.963205226001814,
35.3483736457246));
#192399=CARTESIAN_POINT('Ctrl Pts',(-6.67335474094204,-1.13534527406606,
35.3565963695905));
#192400=CARTESIAN_POINT('Ctrl Pts',(-6.63970438390436,-1.3063746378284,
35.3648190934564));
#192401=CARTESIAN_POINT('Ctrl Pts',(-6.60608964462966,-1.47722297280297,
35.3730331138476));
#192402=CARTESIAN_POINT('Ctrl Pts',(-6.56583913824034,-1.64696261546586,
35.3812471342388));
#192403=CARTESIAN_POINT('Ctrl Pts',(-6.51904236738862,-1.81504149048779,
35.3894611546301));
#192404=CARTESIAN_POINT('Ctrl Pts',(-6.47228573386492,-1.98297620520089,
35.397668129902));
#192405=CARTESIAN_POINT('Ctrl Pts',(-6.41899411369779,-2.14925264552916,
35.405875105174));
#192406=CARTESIAN_POINT('Ctrl Pts',(-6.35930809291377,-2.31332867950091,
35.414082080446));
#192407=CARTESIAN_POINT('Ctrl Pts',(-6.29966128465423,-2.47729691879288,
35.422283663899));
#192408=CARTESIAN_POINT('Ctrl Pts',(-6.23362856584403,-2.63906729533269,
35.4304852473521));
#192409=CARTESIAN_POINT('Ctrl Pts',(-6.16140043554176,-2.7981125197007,
35.4386868308051));
#192410=CARTESIAN_POINT('Ctrl Pts',(-6.0892052634236,-2.95708517065772,
35.4468846718201));
#192411=CARTESIAN_POINT('Ctrl Pts',(-6.01082045992842,-3.11333482086274,
35.4550825128352));
#192412=CARTESIAN_POINT('Ctrl Pts',(-5.92648478947531,-3.26635378367344,
35.4632803538502));
#192413=CARTESIAN_POINT('Ctrl Pts',(-5.84215656138202,-3.41935924303805,
35.4714774714314));
#192414=CARTESIAN_POINT('Ctrl Pts',(-5.75187867785699,-3.56913426481417,
35.4796745890125));
#192415=CARTESIAN_POINT('Ctrl Pts',(-5.6559362068274,-3.71519509908953,
35.4878717065937));
#192416=CARTESIAN_POINT('Ctrl Pts',(-5.55999480326459,-3.86125430827554,
35.4960687329728));
#192417=CARTESIAN_POINT('Ctrl Pts',(-5.45838913383538,-4.00359911176378,
35.5042657593519));
#192418=CARTESIAN_POINT('Ctrl Pts',(-5.35144794687987,-4.14177424201697,
35.5124627857309));
#192419=CARTESIAN_POINT('Ctrl Pts',(-5.24448850461171,-4.27997295934895,
35.5206612113771));
#192420=CARTESIAN_POINT('Ctrl Pts',(-5.13219194987402,-4.41400030158837,
35.5288596370232));
#192421=CARTESIAN_POINT('Ctrl Pts',(-5.014927735395,-4.54343359242391,35.5370580626694));
#192422=CARTESIAN_POINT('Ctrl Pts',(-4.89762218099701,-4.67291251322233,
35.54525937856));
#192423=CARTESIAN_POINT('Ctrl Pts',(-4.7753457190642,-4.79779389065165,
35.5534606944507));
#192424=CARTESIAN_POINT('Ctrl Pts',(-4.6485051353589,-4.91769143059443,
35.5616620103414));
#192425=CARTESIAN_POINT('Ctrl Pts',(-4.52152010146121,-5.037725513765,35.5698726661579));
#192426=CARTESIAN_POINT('Ctrl Pts',(-4.38996082261079,-5.15276417354653,
35.5780833219745));
#192427=CARTESIAN_POINT('Ctrl Pts',(-4.25426849298258,-5.26246031715354,
35.5862939777911));
#192428=CARTESIAN_POINT('Ctrl Pts',(-4.11849620315205,-5.37222110204029,
35.5945094719483));
#192429=CARTESIAN_POINT('Ctrl Pts',(-3.97858629483901,-5.4766328810103,
35.6027249661054));
#192430=CARTESIAN_POINT('Ctrl Pts',(-3.83500939456544,-5.57539164037782,
35.6109404602626));
#192431=CARTESIAN_POINT('Ctrl Pts',(-3.691209732089,-5.67430362577785,35.6191687009101));
#192432=CARTESIAN_POINT('Ctrl Pts',(-3.54373201107681,-5.76754487250477,
35.6273969415576));
#192433=CARTESIAN_POINT('Ctrl Pts',(-3.39307308681808,-5.85485644807034,
35.6356251822051));
#192434=CARTESIAN_POINT('Ctrl Pts',(-3.25614817752705,-5.934208730872,35.6431033393062));
#192435=CARTESIAN_POINT('Ctrl Pts',(-3.11659609816114,-6.0086636579805,
35.6505814964072));
#192436=CARTESIAN_POINT('Ctrl Pts',(-2.9748035714871,-6.07806159158227,
35.6580596535083));
#192437=CARTESIAN_POINT('Ctrl Pts',(-2.82180227347862,-6.1529454671238,
35.6661289627308));
#192438=CARTESIAN_POINT('Ctrl Pts',(-2.66569108822884,-6.22218558074512,
35.6741982719533));
#192439=CARTESIAN_POINT('Ctrl Pts',(-2.506933350062,-6.28550508538072,35.6822675811759));
#192440=CARTESIAN_POINT('Ctrl Pts',(-2.34837362594366,-6.34874561338434,
35.6903268257766));
#192441=CARTESIAN_POINT('Ctrl Pts',(-2.18717425916129,-6.40608008931937,
35.6983860703774));
#192442=CARTESIAN_POINT('Ctrl Pts',(-2.02382420479174,-6.45727687094948,
35.7064453149781));
#192443=CARTESIAN_POINT('Ctrl Pts',(-1.86064204543636,-6.50842103132757,
35.7144962760984));
#192444=CARTESIAN_POINT('Ctrl Pts',(-1.69531395053249,-6.55343994071516,
35.7225472372186));
#192445=CARTESIAN_POINT('Ctrl Pts',(-1.52834984306422,-6.59214955513037,
35.7305981983389));
#192446=CARTESIAN_POINT('Ctrl Pts',(-1.36152076006945,-6.63082786494135,
35.738642648618));
#192447=CARTESIAN_POINT('Ctrl Pts',(-1.19305865946455,-6.66320695129684,
35.7466870988971));
#192448=CARTESIAN_POINT('Ctrl Pts',(-1.02348955549306,-6.68915227288157,
35.7547315491762));
#192449=CARTESIAN_POINT('Ctrl Pts',(-0.854020465573154,-6.71508229157992,
35.7627712547344));
#192450=CARTESIAN_POINT('Ctrl Pts',(-0.683446039977079,-6.73458604336561,
35.7708109602926));
#192451=CARTESIAN_POINT('Ctrl Pts',(-0.512303335900461,-6.74757988407883,
35.7788506658509));
#192452=CARTESIAN_POINT('Ctrl Pts',(-0.337466608053861,-6.76085418989699,
35.7870639041553));
#192453=CARTESIAN_POINT('Ctrl Pts',(-0.162037179450421,-6.76733427404382,
35.7952771424598));
#192454=CARTESIAN_POINT('Ctrl Pts',(0.01340541338267,-6.76698672193851,
35.8034903807642));
#192455=CARTESIAN_POINT('Ctrl Pts',(0.185085899116309,-6.76664662257441,
35.8115274983124));
#192456=CARTESIAN_POINT('Ctrl Pts',(0.356778601719374,-6.75976874907977,
35.8195646158606));
#192457=CARTESIAN_POINT('Ctrl Pts',(0.527939652872292,-6.74637448730243,
35.8276017334087));
#192458=CARTESIAN_POINT('Ctrl Pts',(0.699118811776092,-6.73297880849736,
35.8356397012329));
#192459=CARTESIAN_POINT('Ctrl Pts',(0.869765834724054,-6.71306539776337,
35.843677669057));
#192460=CARTESIAN_POINT('Ctrl Pts',(1.03934150297878,-6.68670757848628,
35.8517156368811));
#192461=CARTESIAN_POINT('Ctrl Pts',(1.20896871045226,-6.66034174826382,
35.8597560476888));
#192462=CARTESIAN_POINT('Ctrl Pts',(1.37752354611965,-6.62752766817689,
35.8677964584965));
#192463=CARTESIAN_POINT('Ctrl Pts',(1.54447666483523,-6.58838985122916,
35.8758368693043));
#192464=CARTESIAN_POINT('Ctrl Pts',(1.7177396698112,-6.54777284554079,35.8841811622921));
#192465=CARTESIAN_POINT('Ctrl Pts',(1.88927708696084,-6.50034486233937,
35.8925254552799));
#192466=CARTESIAN_POINT('Ctrl Pts',(2.05851527055682,-6.44630156608302,
35.9008697482677));
#192467=CARTESIAN_POINT('Ctrl Pts',(2.22187813478561,-6.39413445177577,
35.9089243584832));
#192468=CARTESIAN_POINT('Ctrl Pts',(2.38309840904916,-6.33580383312127,
35.9169789686987));
#192469=CARTESIAN_POINT('Ctrl Pts',(2.54168173442563,-6.27153433865168,
35.9250335789143));
#192470=CARTESIAN_POINT('Ctrl Pts',(2.70038510961958,-6.20721619126689,
35.9330942865835));
#192471=CARTESIAN_POINT('Ctrl Pts',(2.85644722297175,-6.13695036868298,
35.9411549942527));
#192472=CARTESIAN_POINT('Ctrl Pts',(3.00939882702473,-6.06100715227281,
35.949215701922));
#192473=CARTESIAN_POINT('Ctrl Pts',(3.16256608367581,-5.98495686047742,
35.9572877747061));
#192474=CARTESIAN_POINT('Ctrl Pts',(3.31261375603508,-5.90321338096559,
35.9653598474903));
#192475=CARTESIAN_POINT('Ctrl Pts',(3.45910154803444,-5.81609022285467,
35.9734319202744));
#192476=CARTESIAN_POINT('Ctrl Pts',(3.47444503126758,-5.80696473398323,
35.9742774085689));
#192477=CARTESIAN_POINT('Ctrl Pts',(3.4897494894461,-5.79778026092327,35.9751228968634));
#192478=CARTESIAN_POINT('Ctrl Pts',(3.50501443822637,-5.7885371889472,35.9759683851578));
#192479=CARTESIAN_POINT('Ctrl Pts',(3.65546197140124,-5.69743977370033,
35.9843013072045));
#192480=CARTESIAN_POINT('Ctrl Pts',(3.80254895383336,-5.60035636262105,
35.9926342292513));
#192481=CARTESIAN_POINT('Ctrl Pts',(3.94577458207431,-5.49755872614894,
36.000967151298));
#192482=CARTESIAN_POINT('Ctrl Pts',(4.08883095235525,-5.39488257155445,
36.0092902258516));
#192483=CARTESIAN_POINT('Ctrl Pts',(4.22803477840236,-5.28650584488286,
36.0176133004052));
#192484=CARTESIAN_POINT('Ctrl Pts',(4.36291129740579,-5.17274530698825,
36.0259363749588));
#192485=CARTESIAN_POINT('Ctrl Pts',(4.49765318243103,-5.05909832506239,
36.0342511414048));
#192486=CARTESIAN_POINT('Ctrl Pts',(4.62807610197493,-4.94007846184567,
36.0425659078507));
#192487=CARTESIAN_POINT('Ctrl Pts',(4.75373547682771,-4.81604485198692,
36.0508806742967));
#192488=CARTESIAN_POINT('Ctrl Pts',(4.87929246843091,-4.69211230075628,
36.0591886661362));
#192489=CARTESIAN_POINT('Ctrl Pts',(5.00009340235943,-4.56317438604016,
36.0674966579758));
#192490=CARTESIAN_POINT('Ctrl Pts',(5.11572775623998,-4.4296296147687,36.0758046498153));
#192491=CARTESIAN_POINT('Ctrl Pts',(5.23128909460308,-4.29616916826967,
36.0841073957024));
#192492=CARTESIAN_POINT('Ctrl Pts',(5.34169012728582,-4.15810792466243,
36.0924101415895));
#192493=CARTESIAN_POINT('Ctrl Pts',(5.44655795667186,-4.01588040467025,
36.1007128874766));
#192494=CARTESIAN_POINT('Ctrl Pts',(5.55138292991797,-3.87371100853297,
36.109012240296));
#192495=CARTESIAN_POINT('Ctrl Pts',(5.65067899941118,-3.72737900821017,
36.1173115931154));
#192496=CARTESIAN_POINT('Ctrl Pts',(5.74411408363114,-3.57735130987025,
36.1256109459349));
#192497=CARTESIAN_POINT('Ctrl Pts',(5.83752929577646,-3.42735551990441,
36.1339085336212));
#192498=CARTESIAN_POINT('Ctrl Pts',(5.92508582221167,-3.27366589298205,
36.1422061213076));
#192499=CARTESIAN_POINT('Ctrl Pts',(6.00649526125543,-3.11677777143576,
36.1505037089939));
#192500=CARTESIAN_POINT('Ctrl Pts',(6.08790091411175,-2.95989694643693,
36.1588009107763));
#192501=CARTESIAN_POINT('Ctrl Pts',(6.16315988919264,-2.79981823210372,
36.1670981125587));
#192502=CARTESIAN_POINT('Ctrl Pts',(6.2320299626385,-2.63706115681378,36.1753953143411));
#192503=CARTESIAN_POINT('Ctrl Pts',(6.30090827706874,-2.47428460603254,
36.1836935089657));
#192504=CARTESIAN_POINT('Ctrl Pts',(6.36339603150264,-2.30882937628908,
36.1919917035902));
#192505=CARTESIAN_POINT('Ctrl Pts',(6.41929925439431,-2.14123470981878,
36.2002898982148));
#192506=CARTESIAN_POINT('Ctrl Pts',(6.47524179467439,-1.97352217206561,
36.2085939290563));
#192507=CARTESIAN_POINT('Ctrl Pts',(6.52459043958811,-1.80366752134964,
36.2168979598979));
#192508=CARTESIAN_POINT('Ctrl Pts',(6.56720093130783,-1.63222575884269,
36.2252019907395));
#192509=CARTESIAN_POINT('Ctrl Pts',(6.6098269173751,-1.46072165539234,36.2335090411552));
#192510=CARTESIAN_POINT('Ctrl Pts',(6.64570979000095,-1.28762962925029,
36.241816091571));
#192511=CARTESIAN_POINT('Ctrl Pts',(6.67475645564233,-1.11351482157222,
36.2501231419867));
#192512=CARTESIAN_POINT('Ctrl Pts',(6.70383417707155,-0.939213855779091,
36.2584390740413));
#192513=CARTESIAN_POINT('Ctrl Pts',(6.72606103795095,-0.76388826813644,
36.2667550060959));
#192514=CARTESIAN_POINT('Ctrl Pts',(6.74139572822352,-0.588109373747527,
36.2750709381506));
#192515=CARTESIAN_POINT('Ctrl Pts',(6.75295534347028,-0.455603509493314,
36.2813396643694));
#192516=CARTESIAN_POINT('Ctrl Pts',(6.76059957923247,-0.322840178810183,
36.2876083905883));
#192517=CARTESIAN_POINT('Ctrl Pts',(6.76433032192128,-0.190063925920677,
36.2938771168071));
#192518=CARTESIAN_POINT('Ctrl Pts',(6.76935937840859,-0.0110809909792215,
36.3023273855305));
#192519=CARTESIAN_POINT('Ctrl Pts',(6.76728459495253,0.168253599084478,
36.3107776542538));
#192520=CARTESIAN_POINT('Ctrl Pts',(6.75807926991523,0.347352244187413,
36.3192279229772));
#192521=CARTESIAN_POINT('Ctrl Pts',(6.74888206888957,0.526292828659922,
36.3276707340517));
#192522=CARTESIAN_POINT('Ctrl Pts',(6.73256688619761,0.704997553608084,
36.3361135451262));
#192523=CARTESIAN_POINT('Ctrl Pts',(6.70915905308408,0.88287813452362,36.3445563562007));
#192524=CARTESIAN_POINT('Ctrl Pts',(6.68576869114079,1.06062594868987,36.3529928657185));
#192525=CARTESIAN_POINT('Ctrl Pts',(6.65529627483146,1.23755051737008,36.3614293752362));
#192526=CARTESIAN_POINT('Ctrl Pts',(6.61781904841466,1.41306760009566,36.3698658847539));
#192527=CARTESIAN_POINT('Ctrl Pts',(6.58036863896995,1.58845909090426,36.3782963574951));
#192528=CARTESIAN_POINT('Ctrl Pts',(6.53592348636612,1.76244478115858,36.3867268302363));
#192529=CARTESIAN_POINT('Ctrl Pts',(6.48461214727213,1.93444935303325,36.3951573029776));
#192530=CARTESIAN_POINT('Ctrl Pts',(6.43332286678374,2.10637998060868,36.4035841514814));
#192531=CARTESIAN_POINT('Ctrl Pts',(6.37517337884471,2.2763308704905,36.4120109999852));
#192532=CARTESIAN_POINT('Ctrl Pts',(6.31034260999571,2.44373999117594,36.4204378484891));
#192533=CARTESIAN_POINT('Ctrl Pts',(6.2455318520898,2.61109743864438,36.4288620959257));
#192534=CARTESIAN_POINT('Ctrl Pts',(6.17404404553782,2.77591437265637,36.4372863433624));
#192535=CARTESIAN_POINT('Ctrl Pts',(6.09610707896122,2.93764658899585,36.445710590799));
#192536=CARTESIAN_POINT('Ctrl Pts',(6.07414742369342,2.98321653959202,36.4480842214101));
#192537=CARTESIAN_POINT('Ctrl Pts',(6.05167606520156,3.02854171668513,36.4504578520211));
#192538=CARTESIAN_POINT('Ctrl Pts',(6.02869878558656,3.07361024735849,36.4528314826322));
#192539=CARTESIAN_POINT('Ctrl Pts',(5.94526704241081,3.23725651617065,36.4614502635694));
#192540=CARTESIAN_POINT('Ctrl Pts',(5.85519874817166,3.39744398776223,36.4700690445067));
#192541=CARTESIAN_POINT('Ctrl Pts',(5.75881096500374,3.5536439423995,36.478687825444));
#192542=CARTESIAN_POINT('Ctrl Pts',(5.66236528228048,3.70993772539988,36.4873117836305));
#192543=CARTESIAN_POINT('Ctrl Pts',(5.55959269454276,3.86223895234433,36.4959357418171));
#192544=CARTESIAN_POINT('Ctrl Pts',(5.45085362699419,4.01004784723129,36.5045597000037));
#192545=CARTESIAN_POINT('Ctrl Pts',(5.33818618795038,4.16319657316984,36.5134952123748));
#192546=CARTESIAN_POINT('Ctrl Pts',(5.21911335343159,4.31152204278115,36.5224307247459));
#192547=CARTESIAN_POINT('Ctrl Pts',(5.094081191368,4.4545062370313,36.531366237117));
#192548=CARTESIAN_POINT('Ctrl Pts',(4.9731829065423,4.59276301478131,36.5400063190117));
#192549=CARTESIAN_POINT('Ctrl Pts',(4.84671329108184,4.72602586710489,36.5486464009064));
#192550=CARTESIAN_POINT('Ctrl Pts',(4.71511314186959,4.85386413688813,36.5572864828012));
#192551=CARTESIAN_POINT('Ctrl Pts',(4.57676328323695,4.9882591710748,36.5663697104104));
#192552=CARTESIAN_POINT('Ctrl Pts',(4.43274307541669,5.11665829633533,36.5754529380197));
#192553=CARTESIAN_POINT('Ctrl Pts',(4.28360435989835,5.23860885043537,36.584536165629));
#192554=CARTESIAN_POINT('Ctrl Pts',(4.13446564438004,5.3605594045354,36.5936193932383));
#192555=CARTESIAN_POINT('Ctrl Pts',(3.98020875174013,5.47606118199518,36.6027026208476));
#192556=CARTESIAN_POINT('Ctrl Pts',(3.82142145063258,5.5847136987177,36.6117858484568));
#192557=CARTESIAN_POINT('Ctrl Pts',(3.6633094499645,5.69290413130769,36.6208304463549));
#192558=CARTESIAN_POINT('Ctrl Pts',(3.5005599757691,5.79440407155689,36.6298750442529));
#192559=CARTESIAN_POINT('Ctrl Pts',(3.33373510326058,5.88884532495872,36.6389196421509));
#192560=CARTESIAN_POINT('Ctrl Pts',(3.25638187602201,5.93263577194207,36.6431134342753));
#192561=CARTESIAN_POINT('Ctrl Pts',(3.17815286472116,5.97490921260783,36.6473072263997));
#192562=CARTESIAN_POINT('Ctrl Pts',(3.0991061983213,6.01563211736942,36.6515010185242));
#192563=CARTESIAN_POINT('Origin',(0.,0.,4.30282021618968));
#192564=CARTESIAN_POINT('',(3.09910619832132,6.01563211736941,39.0457552630242));
#192565=CARTESIAN_POINT('',(3.0991061983213,6.01563211736942,38.6513937037315));
#192566=CARTESIAN_POINT('',(3.09910619832133,6.0156321173694,4.30282021618968));
#192567=CARTESIAN_POINT('',(-6.767,4.99256668992643E-13,37.6971797838101));
#192568=CARTESIAN_POINT('Ctrl Pts',(-6.767,4.9925651306646E-13,37.6971797838101));
#192569=CARTESIAN_POINT('Ctrl Pts',(-6.76700000000001,-0.186007249526497,
37.7059292956213));
#192570=CARTESIAN_POINT('Ctrl Pts',(-6.75932637294522,-0.372014355749668,
37.7146788074325));
#192571=CARTESIAN_POINT('Ctrl Pts',(-6.74400518264181,-0.557389537487367,
37.7234283192437));
#192572=CARTESIAN_POINT('Ctrl Pts',(-6.72868405705086,-0.74276393625177,
37.7321777940993));
#192573=CARTESIAN_POINT('Ctrl Pts',(-6.70571545645724,-0.927506130242345,
37.740927268955));
#192574=CARTESIAN_POINT('Ctrl Pts',(-6.67517739404798,-1.11098863990178,
37.7496767438107));
#192575=CARTESIAN_POINT('Ctrl Pts',(-6.64463945808664,-1.29447038982144,
37.7584261824377));
#192576=CARTESIAN_POINT('Ctrl Pts',(-6.60653217008304,-1.47669218313915,
37.7671756210647));
#192577=CARTESIAN_POINT('Ctrl Pts',(-6.5609849609261,-1.65703510599551,
37.7759250596918));
#192578=CARTESIAN_POINT('Ctrl Pts',(-6.51543793658224,-1.83737729708959,
37.7846744628169));
#192579=CARTESIAN_POINT('Ctrl Pts',(-6.46245112167342,-2.01584035511179,
37.7934238659421));
#192580=CARTESIAN_POINT('Ctrl Pts',(-6.40220448374169,-2.19181813761036,
37.8021732690673));
#192581=CARTESIAN_POINT('Ctrl Pts',(-6.34195808526415,-2.3677952206738,
37.8109226374174));
#192582=CARTESIAN_POINT('Ctrl Pts',(-6.27445201433011,-2.54128677684393,
37.8196720057675));
#192583=CARTESIAN_POINT('Ctrl Pts',(-6.19991555071806,-2.71170355385031,
37.8284213741175));
#192584=CARTESIAN_POINT('Ctrl Pts',(-6.12537937716588,-2.88211966767699,
37.8371707084193));
#192585=CARTESIAN_POINT('Ctrl Pts',(-6.04381298052407,-3.04946076372009,
37.8459200427211));
#192586=CARTESIAN_POINT('Ctrl Pts',(-5.9554933933571,-3.21315848374772,
37.8546693770229));
#192587=CARTESIAN_POINT('Ctrl Pts',(-5.86717414255279,-3.37685558033719,
37.8634186780031));
#192588=CARTESIAN_POINT('Ctrl Pts',(-5.77210188876459,-3.53690907646984,
37.8721679789833));
#192589=CARTESIAN_POINT('Ctrl Pts',(-5.67059953346847,-3.69277536969515,
37.8809172799635));
#192590=CARTESIAN_POINT('Ctrl Pts',(-5.5690975563123,-3.84864108225145,
37.8896665483487));
#192591=CARTESIAN_POINT('Ctrl Pts',(-5.46116568196693,-4.00031938297732,
37.898415816734));
#192592=CARTESIAN_POINT('Ctrl Pts',(-5.34717048533442,-4.14729511860062,
37.9071650851193));
#192593=CARTESIAN_POINT('Ctrl Pts',(-5.23317570391682,-4.29427031888104,
37.9159143216363));
#192594=CARTESIAN_POINT('Ctrl Pts',(-5.11311782003368,-4.43654276189715,
37.9246635581534));
#192595=CARTESIAN_POINT('Ctrl Pts',(-4.98740458984616,-4.57362924352002,
37.9334127946704));
#192596=CARTESIAN_POINT('Ctrl Pts',(-4.86169180711615,-4.71071523720399,
37.9421620000458));
#192597=CARTESIAN_POINT('Ctrl Pts',(-4.73032391204053,-4.84261509523353,
37.9509112054213));
#192598=CARTESIAN_POINT('Ctrl Pts',(-4.59374707013491,-4.9688808453843,
37.9596604107967));
#192599=CARTESIAN_POINT('Ctrl Pts',(-4.45717070301345,-5.09514615659551,
37.9684095857571));
#192600=CARTESIAN_POINT('Ctrl Pts',(-4.3153856357095,-5.21577720459602,
37.9771587607176));
#192601=CARTESIAN_POINT('Ctrl Pts',(-4.16887341029428,-5.3303642923295,
37.985907935678));
#192602=CARTESIAN_POINT('Ctrl Pts',(-4.02236168203632,-5.4449509912367,
37.99465708095));
#192603=CARTESIAN_POINT('Ctrl Pts',(-3.87112305348099,-5.55349359438647,
38.0034062262221));
#192604=CARTESIAN_POINT('Ctrl Pts',(-3.71567117017703,-5.65562346298932,
38.0121553714941));
#192605=CARTESIAN_POINT('Ctrl Pts',(-3.56021980145756,-5.75775299351683,
38.0209044878042));
#192606=CARTESIAN_POINT('Ctrl Pts',(-3.40055544538281,-5.85346967463913,
38.0296536041144));
#192607=CARTESIAN_POINT('Ctrl Pts',(-3.2372203598678,-5.94244842986941,
38.0384027204246));
#192608=CARTESIAN_POINT('Ctrl Pts',(-3.0738858014711,-6.03142689794564,
38.0471518084994));
#192609=CARTESIAN_POINT('Ctrl Pts',(-2.90688078896512,-6.11366734656813,
38.0559008965743));
#192610=CARTESIAN_POINT('Ctrl Pts',(-2.73677250721309,-6.18889046952381,
38.0646499846491));
#192611=CARTESIAN_POINT('Ctrl Pts',(-2.56666476031374,-6.26411335596373,
38.0733990452151));
#192612=CARTESIAN_POINT('Ctrl Pts',(-2.3934540257501,-6.33231884500616,
38.0821481057812));
#192613=CARTESIAN_POINT('Ctrl Pts',(-2.21772856065386,-6.39327529762798,
38.0908971663473));
#192614=CARTESIAN_POINT('Ctrl Pts',(-2.04200363348265,-6.45423156365191,
38.099646200131));
#192615=CARTESIAN_POINT('Ctrl Pts',(-1.86376426188986,-6.50793874375743,
38.1083952339147));
#192616=CARTESIAN_POINT('Ctrl Pts',(-1.68361577752817,-6.55421443909629,
38.1171442676984));
#192617=CARTESIAN_POINT('Ctrl Pts',(-1.50346782967488,-6.60048999661938,
38.1258932754262));
#192618=CARTESIAN_POINT('Ctrl Pts',(-1.32141105794702,-6.63933404237768,
38.134642283154));
#192619=CARTESIAN_POINT('Ctrl Pts',(-1.13806375486765,-6.67061465607605,
38.1433912908818));
#192620=CARTESIAN_POINT('Ctrl Pts',(-0.954716982601093,-6.70189517921322,
38.1521402732802));
#192621=CARTESIAN_POINT('Ctrl Pts',(-0.770079968900879,-6.72561226592241,
38.1608892556786));
#192622=CARTESIAN_POINT('Ctrl Pts',(-0.584779765557656,-6.74168536983107,
38.169638238077));
#192623=CARTESIAN_POINT('Ctrl Pts',(-0.391489830650733,-6.75845151013856,
38.1787644570868));
#192624=CARTESIAN_POINT('Ctrl Pts',(-0.197478578237794,-6.76689983031627,
38.1878906760967));
#192625=CARTESIAN_POINT('Ctrl Pts',(-0.00346287645082897,-6.76699911397118,
38.1970168951066));
#192626=CARTESIAN_POINT('Ctrl Pts',(0.184489834655294,-6.76709529501187,
38.2058579197724));
#192627=CARTESIAN_POINT('Ctrl Pts',(0.372446404250773,-6.7593563973816,
38.2146989444382));
#192628=CARTESIAN_POINT('Ctrl Pts',(0.559755019489732,-6.74380925873175,
38.223539969104));
#192629=CARTESIAN_POINT('Ctrl Pts',(0.745134705523219,-6.7284222265979,
38.2322899477137));
#192630=CARTESIAN_POINT('Ctrl Pts',(0.92987943123006,-6.70538706057503,
38.2410399263235));
#192631=CARTESIAN_POINT('Ctrl Pts',(1.11336163626979,-6.67478200894102,
38.2497899049332));
#192632=CARTESIAN_POINT('Ctrl Pts',(1.29684196300894,-6.64417727060979,
38.2585397939698));
#192633=CARTESIAN_POINT('Ctrl Pts',(1.47905951217707,-6.60600284890547,
38.2672896830063));
#192634=CARTESIAN_POINT('Ctrl Pts',(1.65939532067302,-6.56038841607176,
38.2760395720428));
#192635=CARTESIAN_POINT('Ctrl Pts',(1.83972934301021,-6.51477443503195,
38.284789374415));
#192636=CARTESIAN_POINT('Ctrl Pts',(2.01818138406485,-6.46172066062072,
38.2935391767871));
#192637=CARTESIAN_POINT('Ctrl Pts',(2.1941452835442,-6.40140730423403,38.3022889791593));
#192638=CARTESIAN_POINT('Ctrl Pts',(2.3701074986422,-6.3410945251856,38.3110386977756));
#192639=CARTESIAN_POINT('Ctrl Pts',(2.5435813486668,-6.27352239616415,38.3197884163919));
#192640=CARTESIAN_POINT('Ctrl Pts',(2.71397759435775,-6.19892043966723,
38.3285381350083));
#192641=CARTESIAN_POINT('Ctrl Pts',(2.88437226558332,-6.12431917249417,
38.337287772777));
#192642=CARTESIAN_POINT('Ctrl Pts',(3.05168912681152,-6.04268832278699,
38.3460374105457));
#192643=CARTESIAN_POINT('Ctrl Pts',(3.21535986274039,-5.95430516123234,
38.3547870483144));
#192644=CARTESIAN_POINT('Ctrl Pts',(3.37902914073035,-5.8659227869733,38.3635366081435));
#192645=CARTESIAN_POINT('Ctrl Pts',(3.53905210621772,-5.77078835741819,
38.3722861679725));
#192646=CARTESIAN_POINT('Ctrl Pts',(3.69488522831904,-5.66922500431494,
38.3810357278016));
#192647=CARTESIAN_POINT('Ctrl Pts',(3.85071701407155,-5.56766252216945,
38.3897852125987));
#192648=CARTESIAN_POINT('Ctrl Pts',(4.00235878822627,-5.45967138329207,
38.3985346973958));
#192649=CARTESIAN_POINT('Ctrl Pts',(4.14929549611555,-5.34561838199428,
38.407284182193));
#192650=CARTESIAN_POINT('Ctrl Pts',(4.29623099276313,-5.23156632086832,
38.4160335948656));
#192651=CARTESIAN_POINT('Ctrl Pts',(4.43846127436243,-5.11145267304777,
38.4247830075381));
#192652=CARTESIAN_POINT('Ctrl Pts',(4.5755032605465,-4.98568540049694,38.4335324202107));
#192653=CARTESIAN_POINT('Ctrl Pts',(4.7125441625798,-4.85991912290167,38.442281763666));
#192654=CARTESIAN_POINT('Ctrl Pts',(4.84439664018952,-4.72849950385223,
38.4510311071212));
#192655=CARTESIAN_POINT('Ctrl Pts',(4.97061286794928,-4.5918728986087,38.4597804505765));
#192656=CARTESIAN_POINT('Ctrl Pts',(5.09682813912862,-4.45524732884482,
38.4685297277213));
#192657=CARTESIAN_POINT('Ctrl Pts',(5.21740705148011,-4.3134150623558,38.4772790048661));
#192658=CARTESIAN_POINT('Ctrl Pts',(5.33194007545862,-4.16685781275511,
38.4860282820109));
#192659=CARTESIAN_POINT('Ctrl Pts',(5.44647226944641,-4.02030162521631,
38.4947774957521));
#192660=CARTESIAN_POINT('Ctrl Pts',(5.55495848628257,-3.86902074887726,
38.5035267094932));
#192661=CARTESIAN_POINT('Ctrl Pts',(5.65703027291922,-3.71352898080459,
38.5122759232343));
#192662=CARTESIAN_POINT('Ctrl Pts',(5.75910135377133,-3.5580382878937,38.5210250764782));
#192663=CARTESIAN_POINT('Ctrl Pts',(5.85475793592888,-3.39833700106479,
38.5297742297221));
#192664=CARTESIAN_POINT('Ctrl Pts',(5.94367514427534,-3.23496750823305,
38.538523382966));
#192665=CARTESIAN_POINT('Ctrl Pts',(6.03259176732766,-3.07159909077478,
38.5472724786189));
#192666=CARTESIAN_POINT('Ctrl Pts',(6.1147689683604,-2.9045627673119,38.5560215742718));
#192667=CARTESIAN_POINT('Ctrl Pts',(6.18992765547993,-2.73442583002809,
38.5647706699247));
#192668=CARTESIAN_POINT('Ctrl Pts',(6.26508587283156,-2.56428995615922,
38.5735197108928));
#192669=CARTESIAN_POINT('Ctrl Pts',(6.33322554827256,-2.39105376934948,
38.5822687518608));
#192670=CARTESIAN_POINT('Ctrl Pts',(6.39411526733121,-2.21530561053819,
38.5910177928289));
#192671=CARTESIAN_POINT('Ctrl Pts',(6.45500462602929,-2.03955849184841,
38.5997667820179));
#192672=CARTESIAN_POINT('Ctrl Pts',(6.50864402040813,-1.86129970164291,
38.6085157712069));
#192673=CARTESIAN_POINT('Ctrl Pts',(6.55485128368665,-1.68113463135808,
38.6172647603959));
#192674=CARTESIAN_POINT('Ctrl Pts',(6.60199809554379,-1.49730620116635,
38.6261916458674));
#192675=CARTESIAN_POINT('Ctrl Pts',(6.64140720707916,-1.31149343245482,
38.6351185313388));
#192676=CARTESIAN_POINT('Ctrl Pts',(6.67293928722917,-1.12435326697326,
38.6440454168102));
#192677=CARTESIAN_POINT('Ctrl Pts',(6.70384625876285,-0.940923067004551,
38.6527953309877));
#192678=CARTESIAN_POINT('Ctrl Pts',(6.72718554579819,-0.75621789951958,
38.6615452451651));
#192679=CARTESIAN_POINT('Ctrl Pts',(6.74287786815346,-0.570865181252368,
38.6702951593426));
#192680=CARTESIAN_POINT('Ctrl Pts',(6.75856988190857,-0.385516108071883,
38.6790449014471));
#192681=CARTESIAN_POINT('Ctrl Pts',(6.76661520773408,-0.199519795224353,
38.6877946435516));
#192682=CARTESIAN_POINT('Ctrl Pts',(6.76698651789579,-0.0135080204537233,
38.696544385656));
#192683=CARTESIAN_POINT('Ctrl Pts',(6.76735782124898,0.172500343514815,
38.705293967321));
#192684=CARTESIAN_POINT('Ctrl Pts',(6.76005538995174,0.358523882212703,
38.714043548986));
#192685=CARTESIAN_POINT('Ctrl Pts',(6.74510402742347,0.543930748566084,
38.7227931306509));
#192686=CARTESIAN_POINT('Ctrl Pts',(6.73015291918012,0.729334461616904,
38.7315425635076));
#192687=CARTESIAN_POINT('Ctrl Pts',(6.70755316306572,0.914121237636309,
38.7402919963643));
#192688=CARTESIAN_POINT('Ctrl Pts',(6.67738151874548,1.0976634516628,38.749041429221));
#192689=CARTESIAN_POINT('Ctrl Pts',(6.64721034747539,1.28120278799822,38.7577907248985));
#192690=CARTESIAN_POINT('Ctrl Pts',(6.60946757205107,1.46349731860486,38.766540020576));
#192691=CARTESIAN_POINT('Ctrl Pts',(6.56428138111484,1.64392790278318,38.7752893162536));
#192692=CARTESIAN_POINT('Ctrl Pts',(6.51909583859811,1.82435589779195,38.7840384863792));
#192693=CARTESIAN_POINT('Ctrl Pts',(6.46646716392837,2.00291972192387,38.7927876565047));
#192694=CARTESIAN_POINT('Ctrl Pts',(6.40657409872848,2.17901292274768,38.8015368266303));
#192695=CARTESIAN_POINT('Ctrl Pts',(6.34668181342035,2.35510383059088,38.8102858828294));
#192696=CARTESIAN_POINT('Ctrl Pts',(6.27952541914004,2.52872390822696,38.8190349390286));
#192697=CARTESIAN_POINT('Ctrl Pts',(6.20533299175464,2.69928350890407,38.8277839952277));
#192698=CARTESIAN_POINT('Ctrl Pts',(6.12831602991493,2.87633637965741,38.8368661313859));
#192699=CARTESIAN_POINT('Ctrl Pts',(6.04371690605213,3.05009086601576,38.8459482675441));
#192700=CARTESIAN_POINT('Ctrl Pts',(5.95184520316572,3.21991112882844,38.8550304037022));
#192701=CARTESIAN_POINT('Ctrl Pts',(5.86333549509209,3.38351691183131,38.8637801840458));
#192702=CARTESIAN_POINT('Ctrl Pts',(5.76807618099297,3.54347103712121,38.8725299643894));
#192703=CARTESIAN_POINT('Ctrl Pts',(5.66639083308937,3.69923018027816,38.881279744733));
#192704=CARTESIAN_POINT('Ctrl Pts',(5.56470914082117,3.85498372382171,38.8900292105179));
#192705=CARTESIAN_POINT('Ctrl Pts',(5.45660203371979,4.00654234702118,38.8987786763028));
#192706=CARTESIAN_POINT('Ctrl Pts',(5.34243669839123,4.15339127986789,38.9075281420877));
#192707=CARTESIAN_POINT('Ctrl Pts',(5.22827486050489,4.30023571401404,38.9162773398337));
#192708=CARTESIAN_POINT('Ctrl Pts',(5.10805534166999,4.44237052028598,38.9250265375797));
#192709=CARTESIAN_POINT('Ctrl Pts',(4.9821864433983,4.57931296628853,38.9337757353257));
#192710=CARTESIAN_POINT('Ctrl Pts',(4.85632073219463,4.71625194483487,38.9425247115374));
#192711=CARTESIAN_POINT('Ctrl Pts',(4.72480612170194,4.8479986152463,38.951273687749));
#192712=CARTESIAN_POINT('Ctrl Pts',(4.58808925235186,4.97410554898601,38.9600226639607));
#192713=CARTESIAN_POINT('Ctrl Pts',(4.4513634947392,5.10022068121318,38.9687722089624));
#192714=CARTESIAN_POINT('Ctrl Pts',(4.3094350120995,5.22069514871942,38.9775217539641));
#192715=CARTESIAN_POINT('Ctrl Pts',(4.16278587431649,5.3351197516636,38.9862712989658));
#192716=CARTESIAN_POINT('Ctrl Pts',(4.01614535740297,5.44953762807954,38.9950203296195));
#192717=CARTESIAN_POINT('Ctrl Pts',(3.86478496657754,5.55790617532902,39.0037693602732));
#192718=CARTESIAN_POINT('Ctrl Pts',(3.70921874747007,5.6598573553948,39.012518390927));
#192719=CARTESIAN_POINT('Ctrl Pts',(3.55365041605713,5.76180991977162,39.0212675403766));
#192720=CARTESIAN_POINT('Ctrl Pts',(3.39387638174336,5.85734478552921,39.0300166898262));
#192721=CARTESIAN_POINT('Ctrl Pts',(3.23043927904355,5.94613749121332,39.0387658392758));
#192722=CARTESIAN_POINT('Ctrl Pts',(3.18691767070304,5.96978206944214,39.041095647192));
#192723=CARTESIAN_POINT('Ctrl Pts',(3.14313645919564,5.9929488063346,39.0434254551081));
#192724=CARTESIAN_POINT('Ctrl Pts',(3.09910619832132,6.01563211736941,39.0457552630242));
#192725=CARTESIAN_POINT('Ctrl Pts',(3.09910619832131,6.01563211736941,37.0458284616795));
#192726=CARTESIAN_POINT('Ctrl Pts',(2.9437658708396,6.09565964604056,37.054025363067));
#192727=CARTESIAN_POINT('Ctrl Pts',(2.78530975093572,6.16967354755004,37.0622222644545));
#192728=CARTESIAN_POINT('Ctrl Pts',(2.62424690404949,6.23743674810308,37.0704191658421));
#192729=CARTESIAN_POINT('Ctrl Pts',(2.46316479927292,6.30520805093613,37.0786170473131));
#192730=CARTESIAN_POINT('Ctrl Pts',(2.29947567723226,6.36672702439135,37.086814928784));
#192731=CARTESIAN_POINT('Ctrl Pts',(2.13370830002611,6.42180487794512,37.095012810255));
#192732=CARTESIAN_POINT('Ctrl Pts',(1.96789096067751,6.47689933191575,37.1032131625603));
#192733=CARTESIAN_POINT('Ctrl Pts',(1.7999944587886,6.52554868564942,37.1114135148655));
#192734=CARTESIAN_POINT('Ctrl Pts',(1.63056246409196,6.56761410640838,37.1196138671708));
#192735=CARTESIAN_POINT('Ctrl Pts',(1.45266961214355,6.61178013113482,37.128223717165));
#192736=CARTESIAN_POINT('Ctrl Pts',(1.2730844187967,6.64868769951069,37.1368335671593));
#192737=CARTESIAN_POINT('Ctrl Pts',(1.09244692275168,6.678236947052,37.1454434171536));
#192738=CARTESIAN_POINT('Ctrl Pts',(0.920109234862118,6.70642848597189,
37.1536576676474));
#192739=CARTESIAN_POINT('Ctrl Pts',(0.746814140581132,6.72792277328595,
37.1618719181412));
#192740=CARTESIAN_POINT('Ctrl Pts',(0.573121202973082,6.74268648883386,
37.170086168635));
#192741=CARTESIAN_POINT('Ctrl Pts',(0.399304144714054,6.75746075450551,
37.1783062890169));
#192742=CARTESIAN_POINT('Ctrl Pts',(0.225089033396702,6.76549484641998,
37.1865264093989));
#192743=CARTESIAN_POINT('Ctrl Pts',(0.051034827200337,6.76680755204496,
37.1947465297809));
#192744=CARTESIAN_POINT('Ctrl Pts',(-0.123252425226701,6.76812201528961,
37.2029776563207));
#192745=CARTESIAN_POINT('Ctrl Pts',(-0.297377985862902,6.76269713672645,
37.2112087828605));
#192746=CARTESIAN_POINT('Ctrl Pts',(-0.470787829535581,6.75060351520967,
37.2194399094004));
#192747=CARTESIAN_POINT('Ctrl Pts',(-0.495311589767621,6.7488932254814,
37.2206039619676));
#192748=CARTESIAN_POINT('Ctrl Pts',(-0.519821052605789,6.74704964539409,
37.2217680145347));
#192749=CARTESIAN_POINT('Ctrl Pts',(-0.544314668960146,6.74507305676928,
37.2229320671019));
#192750=CARTESIAN_POINT('Ctrl Pts',(-0.714106454926598,6.73137118000788,
37.2310013763244));
#192751=CARTESIAN_POINT('Ctrl Pts',(-0.883691765990604,6.7112287430705,
37.239070685547));
#192752=CARTESIAN_POINT('Ctrl Pts',(-1.05253086097781,6.68464417801646,
37.2471399947695));
#192753=CARTESIAN_POINT('Ctrl Pts',(-1.22115936772438,6.65809277114052,
37.2551992393702));
#192754=CARTESIAN_POINT('Ctrl Pts',(-1.38904314637551,6.62511528112674,
37.263258483971));
#192755=CARTESIAN_POINT('Ctrl Pts',(-1.55564349772948,6.58576209014355,
37.2713177285718));
#192756=CARTESIAN_POINT('Ctrl Pts',(-1.72207261333684,6.54644934729259,
37.279368689692));
#192757=CARTESIAN_POINT('Ctrl Pts',(-1.88722056668069,6.5007740293082,37.2874196508122));
#192758=CARTESIAN_POINT('Ctrl Pts',(-2.05055492328046,6.44883815168363,
37.2954706119324));
#192759=CARTESIAN_POINT('Ctrl Pts',(-2.21375719080067,6.39694427478943,
37.3035150622115));
#192760=CARTESIAN_POINT('Ctrl Pts',(-2.375148426933,6.33880002766862,37.3115595124906));
#192761=CARTESIAN_POINT('Ctrl Pts',(-2.53420762751316,6.27455820760746,
37.3196039627697));
#192762=CARTESIAN_POINT('Ctrl Pts',(-2.69317301291823,6.21035427820321,
37.327643668328));
#192763=CARTESIAN_POINT('Ctrl Pts',(-2.8498087558028,6.14006007465764,37.3356833738862));
#192764=CARTESIAN_POINT('Ctrl Pts',(-3.00361033524864,6.06387779840487,
37.3437230794444));
#192765=CARTESIAN_POINT('Ctrl Pts',(-3.1607316395605,5.98605116844822,37.3519363177489));
#192766=CARTESIAN_POINT('Ctrl Pts',(-3.31489466169615,5.90207951539378,
37.3601495560533));
#192767=CARTESIAN_POINT('Ctrl Pts',(-3.46558399043854,5.81222991675451,
37.3683627943578));
#192768=CARTESIAN_POINT('Ctrl Pts',(-3.61304200924495,5.72430700996031,
37.376399911906));
#192769=CARTESIAN_POINT('Ctrl Pts',(-3.75717347361353,5.63075589959779,
37.3844370294542));
#192770=CARTESIAN_POINT('Ctrl Pts',(-3.89752161580777,5.53187258117098,
37.3924741470024));
#192771=CARTESIAN_POINT('Ctrl Pts',(-4.03788460594328,5.43297880151766,
37.4005121148265));
#192772=CARTESIAN_POINT('Ctrl Pts',(-4.17446317143389,5.3287519056758,37.4085500826506));
#192773=CARTESIAN_POINT('Ctrl Pts',(-4.30683105316518,5.21953017804209,
37.4165880504748));
#192774=CARTESIAN_POINT('Ctrl Pts',(-4.43923916553369,5.11027525459348,
37.4246284612825));
#192775=CARTESIAN_POINT('Ctrl Pts',(-4.5674337587902,4.99602271528344,37.4326688720903));
#192776=CARTESIAN_POINT('Ctrl Pts',(-4.69102319291762,4.87714982377094,
37.4407092828981));
#192777=CARTESIAN_POINT('Ctrl Pts',(-4.81928361060147,4.75378420741122,
37.4490535758858));
#192778=CARTESIAN_POINT('Ctrl Pts',(-4.94258364897058,4.62544247759992,
37.4573978688736));
#192779=CARTESIAN_POINT('Ctrl Pts',(-5.06052989067974,4.49258569484623,
37.4657421618614));
#192780=CARTESIAN_POINT('Ctrl Pts',(-5.1743814781955,4.36434120473315,37.4737967720769));
#192781=CARTESIAN_POINT('Ctrl Pts',(-5.28324458573389,4.23189022616613,
37.4818513822925));
#192782=CARTESIAN_POINT('Ctrl Pts',(-5.38680876038135,4.09567825629391,
37.489905992508));
#192783=CARTESIAN_POINT('Ctrl Pts',(-5.49045133457159,3.95936317203687,
37.4979667001772));
#192784=CARTESIAN_POINT('Ctrl Pts',(-5.58878677562368,3.81928173115245,
37.5060274078465));
#192785=CARTESIAN_POINT('Ctrl Pts',(-5.68154952696108,3.67590587103212,
37.5140881155157));
#192786=CARTESIAN_POINT('Ctrl Pts',(-5.77444306822101,3.5323278595378,37.5221601882999));
#192787=CARTESIAN_POINT('Ctrl Pts',(-5.86174805435501,3.38544647943955,
37.530232261084));
#192788=CARTESIAN_POINT('Ctrl Pts',(-5.94324588931876,3.23575606297751,
37.5383043338682));
#192789=CARTESIAN_POINT('Ctrl Pts',(-5.95178216832952,3.22007712916626,
37.5391498221626));
#192790=CARTESIAN_POINT('Ctrl Pts',(-5.96025478173107,3.2043673930891,37.539995310457));
#192791=CARTESIAN_POINT('Ctrl Pts',(-5.96866350967991,3.18862743327212,
37.5408407987514));
#192792=CARTESIAN_POINT('Ctrl Pts',(-6.05851105501668,3.02044542502301,
37.5498748700551));
#192793=CARTESIAN_POINT('Ctrl Pts',(-6.1413108520305,2.84834316167856,37.5589089413587));
#192794=CARTESIAN_POINT('Ctrl Pts',(-6.21674145466605,2.67290379285088,
37.5679430126624));
#192795=CARTESIAN_POINT('Ctrl Pts',(-6.29202726850127,2.49780117933015,
37.5769597430951));
#192796=CARTESIAN_POINT('Ctrl Pts',(-6.35997201579616,2.31937446278634,
37.5859764735278));
#192797=CARTESIAN_POINT('Ctrl Pts',(-6.42030078831588,2.13822982570877,
37.5949932039605));
#192798=CARTESIAN_POINT('Ctrl Pts',(-6.48043547153938,1.95766796586426,
37.6039809258325));
#192799=CARTESIAN_POINT('Ctrl Pts',(-6.53300299195141,1.7744058617648,37.6129686477044));
#192800=CARTESIAN_POINT('Ctrl Pts',(-6.57777737586843,1.58906695690065,
37.6219563695763));
#192801=CARTESIAN_POINT('Ctrl Pts',(-6.62246057309719,1.40410550984739,
37.6309257872189));
#192802=CARTESIAN_POINT('Ctrl Pts',(-6.65938223385962,1.21707593198739,
37.6398952048615));
#192803=CARTESIAN_POINT('Ctrl Pts',(-6.68836562468187,1.02861765033172,
37.6488646225041));
#192804=CARTESIAN_POINT('Ctrl Pts',(-6.71725025336708,0.840801548286838,
37.6578034764745));
#192805=CARTESIAN_POINT('Ctrl Pts',(-6.73825053371445,0.651566692490344,
37.666742330445));
#192806=CARTESIAN_POINT('Ctrl Pts',(-6.75124057061721,0.461562300943391,
37.6756811844155));
#192807=CARTESIAN_POINT('Ctrl Pts',(-6.76165456777378,0.309237468603303,
37.6828473842137));
#192808=CARTESIAN_POINT('Ctrl Pts',(-6.7669212299791,0.156418407734503,
37.6900135840119));
#192809=CARTESIAN_POINT('Ctrl Pts',(-6.76699912273183,0.00344571424731888,
37.6971797838101));
#192810=CARTESIAN_POINT('',(-6.76699756085807,0.00574554966943631,37.3028202162268));
#192811=CARTESIAN_POINT('Ctrl Pts',(3.0991061983213,6.01563211736942,36.6515010185242));
#192812=CARTESIAN_POINT('Ctrl Pts',(2.92887035067861,6.1033334528754,36.6605328194799));
#192813=CARTESIAN_POINT('Ctrl Pts',(2.75484054269377,6.18384034560604,36.6695646204357));
#192814=CARTESIAN_POINT('Ctrl Pts',(2.57761663267981,6.25685076495616,36.6785964213915));
#192815=CARTESIAN_POINT('Ctrl Pts',(2.40071872169563,6.32972688343304,36.6876116085712));
#192816=CARTESIAN_POINT('Ctrl Pts',(2.22063865975616,6.3951339710474,36.6966267957509));
#192817=CARTESIAN_POINT('Ctrl Pts',(2.03799658225956,6.45281790620953,36.7056419829307));
#192818=CARTESIAN_POINT('Ctrl Pts',(1.85559641772055,6.51042543788594,36.714645229321));
#192819=CARTESIAN_POINT('Ctrl Pts',(1.6706412354187,6.56033015820393,36.7236484757112));
#192820=CARTESIAN_POINT('Ctrl Pts',(1.48376906171766,6.60232673922531,36.7326517221015));
#192821=CARTESIAN_POINT('Ctrl Pts',(1.2973000589344,6.64423271392592,36.741635544267));
#192822=CARTESIAN_POINT('Ctrl Pts',(1.1089225512334,6.67826454966805,36.7506193664325));
#192823=CARTESIAN_POINT('Ctrl Pts',(0.919287431701544,6.70426726927825,
36.7596031885979));
#192824=CARTESIAN_POINT('Ctrl Pts',(0.840925417633422,6.71501224882072,
36.7633155304925));
#192825=CARTESIAN_POINT('Ctrl Pts',(0.762348841543449,6.72438680262534,
36.767027872387));
#192826=CARTESIAN_POINT('Ctrl Pts',(0.683604340953227,6.73238249841985,
36.7707402142816));
#192827=CARTESIAN_POINT('Ctrl Pts',(0.511335538045042,6.74987462717316,
36.7788616791378));
#192828=CARTESIAN_POINT('Ctrl Pts',(0.338339441484207,6.76075602110291,
36.786983143994));
#192829=CARTESIAN_POINT('Ctrl Pts',(0.165167046070349,6.7649840241417,36.7951046088501));
#192830=CARTESIAN_POINT('Ctrl Pts',(-0.00799299960279759,6.76921172566164,
36.8032254945263));
#192831=CARTESIAN_POINT('Ctrl Pts',(-0.181328953008264,6.76678697245923,
36.8113463802025));
#192832=CARTESIAN_POINT('Ctrl Pts',(-0.354288183683026,6.75771920716617,
36.8194672658787));
#192833=CARTESIAN_POINT('Ctrl Pts',(-0.527268087931676,6.74865035801587,
36.827589122233));
#192834=CARTESIAN_POINT('Ctrl Pts',(-0.699870814171343,6.73293693605041,
36.8357109785872));
#192835=CARTESIAN_POINT('Ctrl Pts',(-0.871547268904518,6.71064038360461,
36.8438328349414));
#192836=CARTESIAN_POINT('Ctrl Pts',(-1.04334897665523,6.68832756386999,
36.8519606169016));
#192837=CARTESIAN_POINT('Ctrl Pts',(-1.21422269964026,6.65942206802559,
36.8600883988618));
#192838=CARTESIAN_POINT('Ctrl Pts',(-1.383627338963,6.62403686484867,36.868216180822));
#192839=CARTESIAN_POINT('Ctrl Pts',(-1.55310098743957,6.58863724705513,
36.8763472737384));
#192840=CARTESIAN_POINT('Ctrl Pts',(-1.7211040043136,6.54675274900076,36.8844783666548));
#192841=CARTESIAN_POINT('Ctrl Pts',(-1.887109178007,6.49854660291682,36.8926094595713));
#192842=CARTESIAN_POINT('Ctrl Pts',(-2.0532955394097,6.4502878418391,36.9007494272359));
#192843=CARTESIAN_POINT('Ctrl Pts',(-2.21747935526281,6.39569376690599,
36.9088893949004));
#192844=CARTESIAN_POINT('Ctrl Pts',(-2.3791514486796,6.33497651015738,36.917029362565));
#192845=CARTESIAN_POINT('Ctrl Pts',(-2.46300158657844,6.30348591556178,
36.9212511017454));
#192846=CARTESIAN_POINT('Ctrl Pts',(-2.54617644965186,6.27034902093991,
36.9254728409259));
#192847=CARTESIAN_POINT('Ctrl Pts',(-2.62860754292939,6.23560032276402,
36.9296945801064));
#192848=CARTESIAN_POINT('Ctrl Pts',(-2.79340590288101,6.16612983241687,
36.938134789564));
#192849=CARTESIAN_POINT('Ctrl Pts',(-2.95557068972406,6.09007077653584,
36.9465749990216));
#192850=CARTESIAN_POINT('Ctrl Pts',(-3.1145591219573,6.00764600120818,36.9550152084792));
#192851=CARTESIAN_POINT('Ctrl Pts',(-3.27342709689875,5.92528367485918,
36.9634490232278));
#192852=CARTESIAN_POINT('Ctrl Pts',(-3.42912321954626,5.83656539627821,
36.9718828379763));
#192853=CARTESIAN_POINT('Ctrl Pts',(-3.5811261498254,5.74176144567472,36.9803166527248));
#192854=CARTESIAN_POINT('Ctrl Pts',(-3.73303728230423,5.647014749192,36.9887453741134));
#192855=CARTESIAN_POINT('Ctrl Pts',(-3.88125938678123,5.54618988389685,
36.9971740955019));
#192856=CARTESIAN_POINT('Ctrl Pts',(-4.02529678981785,5.43960244446983,
37.0056028168905));
#192857=CARTESIAN_POINT('Ctrl Pts',(-4.16926932369352,5.33306300811436,
37.0140277422922));
#192858=CARTESIAN_POINT('Ctrl Pts',(-4.30906064625791,5.22076637030717,
37.0224526676939));
#192859=CARTESIAN_POINT('Ctrl Pts',(-4.44420476297629,5.10307094059438,
37.0308775930957));
#192860=CARTESIAN_POINT('Ctrl Pts',(-4.57930875085604,4.98541045861756,
37.0393000168534));
#192861=CARTESIAN_POINT('Ctrl Pts',(-4.70976803352087,4.86235460041507,
37.0477224406111));
#192862=CARTESIAN_POINT('Ctrl Pts',(-4.83515006055934,4.73430173223814,
37.0561448643688));
#192863=CARTESIAN_POINT('Ctrl Pts',(-4.96053405949648,4.60624685015789,
37.064567420587));
#192864=CARTESIAN_POINT('Ctrl Pts',(-5.08084040525924,4.47319503464877,
37.0729899768052));
#192865=CARTESIAN_POINT('Ctrl Pts',(-5.19567329169468,4.33558162718344,
37.0814125330234));
#192866=CARTESIAN_POINT('Ctrl Pts',(-5.3105100572068,4.1979635711111,37.0898353737571));
#192867=CARTESIAN_POINT('Ctrl Pts',(-5.41987278087791,4.05578387184934,
37.0982582144909));
#192868=CARTESIAN_POINT('Ctrl Pts',(-5.52340576530313,3.90951119090561,
37.1066810552246));
#192869=CARTESIAN_POINT('Ctrl Pts',(-5.62695670144184,3.76321314755901,
37.1151053564052));
#192870=CARTESIAN_POINT('Ctrl Pts',(-5.72467569033827,3.61282097988212,
37.1235296575859));
#192871=CARTESIAN_POINT('Ctrl Pts',(-5.81625000737054,3.45883287421671,
37.1319539587665));
#192872=CARTESIAN_POINT('Ctrl Pts',(-5.90785299129355,3.30479656333018,
37.1403808971333));
#192873=CARTESIAN_POINT('Ctrl Pts',(-5.99330729786934,3.14716235671892,
37.1488078355001));
#192874=CARTESIAN_POINT('Ctrl Pts',(-6.07234567358564,2.98645392070358,
37.1572347738669));
#192875=CARTESIAN_POINT('Ctrl Pts',(-6.15145511473691,2.82560098760307,
37.1656692891105));
#192876=CARTESIAN_POINT('Ctrl Pts',(-6.22413695084444,2.66166860156118,
37.1741038043542));
#192877=CARTESIAN_POINT('Ctrl Pts',(-6.29017122704871,2.4952023834568,37.1825383195978));
#192878=CARTESIAN_POINT('Ctrl Pts',(-6.35623739837415,2.32865576074286,
37.1909769087846));
#192879=CARTESIAN_POINT('Ctrl Pts',(-6.41564949081724,2.15957317792961,
37.1994154979714));
#192880=CARTESIAN_POINT('Ctrl Pts',(-6.46823697818444,1.98851688301797,
37.2078540871582));
#192881=CARTESIAN_POINT('Ctrl Pts',(-6.52088324646486,1.81726938586923,
37.2163021087785));
#192882=CARTESIAN_POINT('Ctrl Pts',(-6.56668957669043,1.64404408951035,
37.2247501303988));
#192883=CARTESIAN_POINT('Ctrl Pts',(-6.6055359535606,1.46941613105964,37.2331981520191));
#192884=CARTESIAN_POINT('Ctrl Pts',(-6.6276156107538,1.37016040196483,37.2379998719313));
#192885=CARTESIAN_POINT('Ctrl Pts',(-6.64744772074405,1.27045170198658,
37.2428015918436));
#192886=CARTESIAN_POINT('Ctrl Pts',(-6.66501768919741,1.17039660059555,
37.2476033117559));
#192887=CARTESIAN_POINT('Ctrl Pts',(-6.70147283283432,0.962796734807662,
37.2575661861669));
#192888=CARTESIAN_POINT('Ctrl Pts',(-6.72825461317304,0.753321225376306,
37.2675290605779));
#192889=CARTESIAN_POINT('Ctrl Pts',(-6.74519660546739,0.542781497097296,
37.2774919349889));
#192890=CARTESIAN_POINT('Ctrl Pts',(-6.75955362491231,0.364365469022645,
37.2859346953892));
#192891=CARTESIAN_POINT('Ctrl Pts',(-6.76684520655625,0.18518548270118,
37.2943774557896));
#192892=CARTESIAN_POINT('Ctrl Pts',(-6.7669975608574,0.00574555045427647,
37.3028202161899));
#192893=CARTESIAN_POINT('Ctrl Pts',(-6.76699756085807,0.00574554966948139,
37.3028202162268));
#192894=CARTESIAN_POINT('Ctrl Pts',(-6.76713851673575,-0.160269563827458,
37.3106313305565));
#192895=CARTESIAN_POINT('Ctrl Pts',(-6.76116605585226,-0.326516156793914,
37.3184424448862));
#192896=CARTESIAN_POINT('Ctrl Pts',(-6.749055763498,-0.492478731717873,
37.3262535592158));
#192897=CARTESIAN_POINT('Ctrl Pts',(-6.73695361445242,-0.658329708635924,
37.3340594211277));
#192898=CARTESIAN_POINT('Ctrl Pts',(-6.71872187055446,-0.823896656406961,
37.3418652830396));
#192899=CARTESIAN_POINT('Ctrl Pts',(-6.69438819322006,-0.988663602281313,
37.3496711449514));
#192900=CARTESIAN_POINT('Ctrl Pts',(-6.6700641320408,-1.15336543574001,
37.3574739221516));
#192901=CARTESIAN_POINT('Ctrl Pts',(-6.63964298988069,-1.31726750716917,
37.3652766993517));
#192902=CARTESIAN_POINT('Ctrl Pts',(-6.60320428531312,-1.47985883327513,
37.3730794765519));
#192903=CARTESIAN_POINT('Ctrl Pts',(-6.56676827782901,-1.64243812485955,
37.3808816762139));
#192904=CARTESIAN_POINT('Ctrl Pts',(-6.524315674495,-1.80370647872397,37.3886838758759));
#192905=CARTESIAN_POINT('Ctrl Pts',(-6.47597707366099,-1.96316324879446,
37.3964860755379));
#192906=CARTESIAN_POINT('Ctrl Pts',(-6.45517750550536,-2.03177574273791,
37.3998432762189));
#192907=CARTESIAN_POINT('Ctrl Pts',(-6.43328878854922,-2.10005298722402,
37.4032004768998));
#192908=CARTESIAN_POINT('Ctrl Pts',(-6.410324172489,-2.16795595056801,37.4065576775807));
#192909=CARTESIAN_POINT('Ctrl Pts',(-6.34972450734084,-2.34714017165063,
37.4154167517565));
#192910=CARTESIAN_POINT('Ctrl Pts',(-6.28166738932326,-2.52360603214291,
37.4242758259324));
#192911=CARTESIAN_POINT('Ctrl Pts',(-6.20642940907034,-2.69676157459772,
37.4331349001083));
#192912=CARTESIAN_POINT('Ctrl Pts',(-6.13105007179007,-2.8702424414787,
37.4420106187021));
#192913=CARTESIAN_POINT('Ctrl Pts',(-6.04846301380922,-3.04040032340966,
37.450886337296));
#192914=CARTESIAN_POINT('Ctrl Pts',(-5.95899099669742,-3.2066673200192,
37.4597620558899));
#192915=CARTESIAN_POINT('Ctrl Pts',(-5.86926365172822,-3.37340879565996,
37.4686631032768));
#192916=CARTESIAN_POINT('Ctrl Pts',(-5.77261215341232,-3.53623693664242,
37.4775641506638));
#192917=CARTESIAN_POINT('Ctrl Pts',(-5.66940455709463,-3.69460971795327,
37.4864651980508));
#192918=CARTESIAN_POINT('Ctrl Pts',(-5.56605664863431,-3.85319780923227,
37.4953783465337));
#192919=CARTESIAN_POINT('Ctrl Pts',(-5.45613498466277,-4.00731822777013,
37.5042914950167));
#192920=CARTESIAN_POINT('Ctrl Pts',(-5.34004914288942,-4.15646053169352,
37.5132046434997));
#192921=CARTESIAN_POINT('Ctrl Pts',(-5.22370555880406,-4.30593397231406,
37.5221375816095));
#192922=CARTESIAN_POINT('Ctrl Pts',(-5.10117058197372,-4.45040698533129,
37.5310705197194));
#192923=CARTESIAN_POINT('Ctrl Pts',(-4.97289393103948,-4.58940246117408,
37.5400034578293));
#192924=CARTESIAN_POINT('Ctrl Pts',(-4.85079315868725,-4.72170600067458,
37.548506319688));
#192925=CARTESIAN_POINT('Ctrl Pts',(-4.72349069077873,-4.84904688630267,
37.5570091815467));
#192926=CARTESIAN_POINT('Ctrl Pts',(-4.59140331684061,-4.97104662843802,
37.5655120434054));
#192927=CARTESIAN_POINT('Ctrl Pts',(-4.46366773556069,-5.08902692824291,
37.5737347672712));
#192928=CARTESIAN_POINT('Ctrl Pts',(-4.33121184980721,-5.20223762451192,
37.5819574911371));
#192929=CARTESIAN_POINT('Ctrl Pts',(-4.19442656922371,-5.31028010140616,
37.590180215003));
#192930=CARTESIAN_POINT('Ctrl Pts',(-4.05778607122618,-5.41820821899849,
37.5983942353942));
#192931=CARTESIAN_POINT('Ctrl Pts',(-3.91682558282514,-5.52097879000792,
37.6066082557854));
#192932=CARTESIAN_POINT('Ctrl Pts',(-3.77197211665981,-5.61823062459534,
37.6148222761767));
#192933=CARTESIAN_POINT('Ctrl Pts',(-3.62724289050052,-5.71539904682933,
37.6230292514486));
#192934=CARTESIAN_POINT('Ctrl Pts',(-3.47862763259262,-5.80705796077186,
37.6312362267206));
#192935=CARTESIAN_POINT('Ctrl Pts',(-3.32658569574698,-5.89288695028605,
37.6394432019925));
#192936=CARTESIAN_POINT('Ctrl Pts',(-3.17464364741953,-5.97865955186702,
37.6476447854455));
#192937=CARTESIAN_POINT('Ctrl Pts',(-3.01927971565959,-6.0586096824938,
37.6558463688985));
#192938=CARTESIAN_POINT('Ctrl Pts',(-2.86098151838054,-6.13246066041071,
37.6640479523515));
#192939=CARTESIAN_POINT('Ctrl Pts',(-2.70275555363839,-6.20627793962745,
37.6722457933666));
#192940=CARTESIAN_POINT('Ctrl Pts',(-2.541598315259,-6.2740014593689,37.6804436343817));
#192941=CARTESIAN_POINT('Ctrl Pts',(-2.37802133895028,-6.33540081695682,
37.6886414753967));
#192942=CARTESIAN_POINT('Ctrl Pts',(-2.21445879779948,-6.39679475624295,
37.6968385929779));
#192943=CARTESIAN_POINT('Ctrl Pts',(-2.04847727662655,-6.45186551101317,
37.705035710559));
#192944=CARTESIAN_POINT('Ctrl Pts',(-1.88060792016194,-6.50043097422196,
37.7132328281402));
#192945=CARTESIAN_POINT('Ctrl Pts',(-1.71274043143095,-6.54899589708585,
37.7214298545193));
#192946=CARTESIAN_POINT('Ctrl Pts',(-1.54298549364252,-6.59105557179551,
37.7296268808984));
#192947=CARTESIAN_POINT('Ctrl Pts',(-1.37188891178661,-6.62647793429639,
37.7378239072775));
#192948=CARTESIAN_POINT('Ctrl Pts',(-1.20076312302135,-6.6619063435442,
37.7460223329236));
#192949=CARTESIAN_POINT('Ctrl Pts',(-1.02829558529569,-6.69069511052739,
37.7542207585697));
#192950=CARTESIAN_POINT('Ctrl Pts',(-0.855041831038226,-6.71276340020821,
37.7624191842158));
#192951=CARTESIAN_POINT('Ctrl Pts',(-0.681726998503361,-6.73483946976729,
37.7706205001065));
#192952=CARTESIAN_POINT('Ctrl Pts',(-0.507625753050677,-6.75019029721376,
37.7788218159972));
#192953=CARTESIAN_POINT('Ctrl Pts',(-0.333298328129745,-6.75878696398,37.7870231318878));
#192954=CARTESIAN_POINT('Ctrl Pts',(-0.158772373453413,-6.76739342091064,
37.7952337877044));
#192955=CARTESIAN_POINT('Ctrl Pts',(0.0159799165223041,-6.76923033250532,
37.803444443521));
#192956=CARTESIAN_POINT('Ctrl Pts',(0.190397662384689,-6.76432093636593,
37.8116550993376));
#192957=CARTESIAN_POINT('Ctrl Pts',(0.364918188399296,-6.75940864723833,
37.8198705934948));
#192958=CARTESIAN_POINT('Ctrl Pts',(0.539103419896524,-6.74774214989725,
37.8280860876519));
#192959=CARTESIAN_POINT('Ctrl Pts',(0.712398133414095,-6.72939654794604,
37.8363015818091));
#192960=CARTESIAN_POINT('Ctrl Pts',(0.885961716868385,-6.71102248245584,
37.8445298224566));
#192961=CARTESIAN_POINT('Ctrl Pts',(1.05863166637931,-6.68594865502462,
37.8527580631041));
#192962=CARTESIAN_POINT('Ctrl Pts',(1.22986215007908,-6.65430147286722,
37.8609863037516));
#192963=CARTESIAN_POINT('Ctrl Pts',(1.38548332263012,-6.62553923679303,
37.8684644608527));
#192964=CARTESIAN_POINT('Ctrl Pts',(1.5399154731124,-6.59134815720409,37.8759426179537));
#192965=CARTESIAN_POINT('Ctrl Pts',(1.69276100623654,-6.55185845205504,
37.8834207750548));
#192966=CARTESIAN_POINT('Ctrl Pts',(1.85768905647565,-6.50924706563356,
37.8914900842773));
#192967=CARTESIAN_POINT('Ctrl Pts',(2.02130939409484,-6.46032589831497,
37.8995593934999));
#192968=CARTESIAN_POINT('Ctrl Pts',(2.18309000201918,-6.40518594914183,
37.9076287027224));
#192969=CARTESIAN_POINT('Ctrl Pts',(2.34466882555505,-6.3501147744718,37.9156879473232));
#192970=CARTESIAN_POINT('Ctrl Pts',(2.50441213640657,-6.28884037018999,
37.9237471919239));
#192971=CARTESIAN_POINT('Ctrl Pts',(2.66179785138195,-6.22150473747135,
37.9318064365247));
#192972=CARTESIAN_POINT('Ctrl Pts',(2.81902180163089,-6.15423831389414,
37.939857397645));
#192973=CARTESIAN_POINT('Ctrl Pts',(2.97389263804433,-6.08092320497609,
37.9479083587652));
#192974=CARTESIAN_POINT('Ctrl Pts',(3.12590330240368,-6.00175120644148,
37.9559593198855));
#192975=CARTESIAN_POINT('Ctrl Pts',(3.27779103519237,-5.92264323458667,
37.9640037701646));
#192976=CARTESIAN_POINT('Ctrl Pts',(3.42682287036525,-5.8376879717809,37.9720482204437));
#192977=CARTESIAN_POINT('Ctrl Pts',(3.57251171777222,-5.74712528368576,
37.9800926707228));
#192978=CARTESIAN_POINT('Ctrl Pts',(3.71811463601211,-5.65661601063574,
37.988132376281));
#192979=CARTESIAN_POINT('Ctrl Pts',(3.86037817552832,-5.56050609270054,
37.9961720818393));
#192980=CARTESIAN_POINT('Ctrl Pts',(3.99883995613077,-5.45908124186223,
38.0042117873975));
#192981=CARTESIAN_POINT('Ctrl Pts',(4.14029036024209,-5.35546718984306,
38.012425025702));
#192982=CARTESIAN_POINT('Ctrl Pts',(4.27777266816484,-5.24630634100549,
38.0206382640064));
#192983=CARTESIAN_POINT('Ctrl Pts',(4.41082489430424,-5.1319501899167,38.0288515023109));
#192984=CARTESIAN_POINT('Ctrl Pts',(4.54102401210514,-5.02004623746973,
38.0368886198591));
#192985=CARTESIAN_POINT('Ctrl Pts',(4.66698082876847,-4.90316779802486,
38.0449257374072));
#192986=CARTESIAN_POINT('Ctrl Pts',(4.78829609200327,-4.78168480091549,
38.0529628549554));
#192987=CARTESIAN_POINT('Ctrl Pts',(4.90962418962153,-4.66018895167748,
38.0610008227795));
#192988=CARTESIAN_POINT('Ctrl Pts',(5.02630949196048,-4.53408783912808,
38.0690387906036));
#192989=CARTESIAN_POINT('Ctrl Pts',(5.13799005438748,-4.40378782425032,
38.0770767584278));
#192990=CARTESIAN_POINT('Ctrl Pts',(5.24970455994399,-4.2734482072235,38.0851171692355));
#192991=CARTESIAN_POINT('Ctrl Pts',(5.3564110548689,-4.13890743117581,38.0931575800432));
#192992=CARTESIAN_POINT('Ctrl Pts',(5.4577883843241,-4.00060432334128,38.1011979908509));
#192993=CARTESIAN_POINT('Ctrl Pts',(5.56299720505791,-3.85707413806921,
38.1095422838387));
#192994=CARTESIAN_POINT('Ctrl Pts',(5.66246590187949,-3.70949203405389,
38.1178865768265));
#192995=CARTESIAN_POINT('Ctrl Pts',(5.75588593671061,-3.55837969918572,
38.1262308698143));
#192996=CARTESIAN_POINT('Ctrl Pts',(5.84606277589728,-3.41251342173075,
38.1342854800299));
#192997=CARTESIAN_POINT('Ctrl Pts',(5.93060376618149,-3.26335827140706,
38.1423400902454));
#192998=CARTESIAN_POINT('Ctrl Pts',(6.00927943682381,-3.11140637817796,
38.150394700461));
#192999=CARTESIAN_POINT('Ctrl Pts',(6.08801466606033,-2.95933945521893,
38.1584554081303));
#193000=CARTESIAN_POINT('Ctrl Pts',(6.1608755769082,-2.80447190949692,38.1665161157995));
#193001=CARTESIAN_POINT('Ctrl Pts',(6.22768146353394,-2.64731422176435,
38.1745768234688));
#193002=CARTESIAN_POINT('Ctrl Pts',(6.29458154245726,-2.4899349511079,38.182648896253));
#193003=CARTESIAN_POINT('Ctrl Pts',(6.35540943224122,-2.33025944187843,
38.1907209690371));
#193004=CARTESIAN_POINT('Ctrl Pts',(6.41003453196383,-2.16881218620499,
38.1987930418213));
#193005=CARTESIAN_POINT('Ctrl Pts',(6.4157560961312,-2.15190181281123,38.1996385301157));
#193006=CARTESIAN_POINT('Ctrl Pts',(6.42140965616103,-2.13497200937217,
38.2004840184101));
#193007=CARTESIAN_POINT('Ctrl Pts',(6.42699509465927,-2.11802338354082,
38.2013295067046));
#193008=CARTESIAN_POINT('Ctrl Pts',(6.48204378534905,-1.9509819486917,38.2096624287513));
#193009=CARTESIAN_POINT('Ctrl Pts',(6.53064681609766,-1.78157854108172,
38.217995350798));
#193010=CARTESIAN_POINT('Ctrl Pts',(6.572600477329,-1.61034529384682,38.2263282728447));
#193011=CARTESIAN_POINT('Ctrl Pts',(6.61450455950663,-1.43931440278568,
38.2346513473984));
#193012=CARTESIAN_POINT('Ctrl Pts',(6.64977484370763,-1.26645831488991,
38.242974421952));
#193013=CARTESIAN_POINT('Ctrl Pts',(6.67825666034375,-1.09232640660853,
38.2512974965056));
#193014=CARTESIAN_POINT('Ctrl Pts',(6.70671004638049,-0.918368317103827,
38.2596122629516));
#193015=CARTESIAN_POINT('Ctrl Pts',(6.72838840952356,-0.743137285736674,
38.2679270293975));
#193016=CARTESIAN_POINT('Ctrl Pts',(6.74318756583585,-0.567195250294588,
38.2762417958435));
#193017=CARTESIAN_POINT('Ctrl Pts',(6.75797466426776,-0.391396566809408,
38.2845497876831));
#193018=CARTESIAN_POINT('Ctrl Pts',(6.7658936951739,-0.214888378786781,
38.2928577795226));
#193019=CARTESIAN_POINT('Ctrl Pts',(6.76689195072957,-0.038240386391329,
38.3011657713622));
#193020=CARTESIAN_POINT('Ctrl Pts',(6.76788957595228,0.138296064372749,
38.3094685172494));
#193021=CARTESIAN_POINT('Ctrl Pts',(6.76197513278595,0.314971796623375,
38.3177712631365));
#193022=CARTESIAN_POINT('Ctrl Pts',(6.74914791589627,0.49121421941257,38.3260740090236));
#193023=CARTESIAN_POINT('Ctrl Pts',(6.73632594108143,0.667384617538833,
38.3343733618431));
#193024=CARTESIAN_POINT('Ctrl Pts',(6.71659684684124,0.843121712586421,
38.3426727146625));
#193025=CARTESIAN_POINT('Ctrl Pts',(6.69001199513991,1.01785485452697,38.350972067482));
#193026=CARTESIAN_POINT('Ctrl Pts',(6.66343279759041,1.19255083366045,38.3592696551683));
#193027=CARTESIAN_POINT('Ctrl Pts',(6.63000079975274,1.36624294132703,38.3675672428547));
#193028=CARTESIAN_POINT('Ctrl Pts',(6.58981903812744,1.53836733088464,38.375864830541));
#193029=CARTESIAN_POINT('Ctrl Pts',(6.54963914527426,1.71048371528651,38.3841620323235));
#193030=CARTESIAN_POINT('Ctrl Pts',(6.50271019343199,1.88103218813741,38.3924592341059));
#193031=CARTESIAN_POINT('Ctrl Pts',(6.44918602738049,2.04946055932782,38.4007564358883));
#193032=CARTESIAN_POINT('Ctrl Pts',(6.3956554566342,2.21790908463531,38.4090546305128));
#193033=CARTESIAN_POINT('Ctrl Pts',(6.33552820507133,2.38423667141169,38.4173528251373));
#193034=CARTESIAN_POINT('Ctrl Pts',(6.26900759336808,2.54790753252417,38.4256510197618));
#193035=CARTESIAN_POINT('Ctrl Pts',(6.20244019694276,2.71169350526221,38.4339550506034));
#193036=CARTESIAN_POINT('Ctrl Pts',(6.12947058658925,2.8728186959976,38.4422590814449));
#193037=CARTESIAN_POINT('Ctrl Pts',(6.05035009713727,3.03076767537056,38.4505631122865));
#193038=CARTESIAN_POINT('Ctrl Pts',(5.97120083729755,3.18877408933993,38.4588701627023));
#193039=CARTESIAN_POINT('Ctrl Pts',(5.88589640287763,3.3436016822627,38.467177213118));
#193040=CARTESIAN_POINT('Ctrl Pts',(5.79473359074778,3.49476059441263,38.4754842635338));
#193041=CARTESIAN_POINT('Ctrl Pts',(5.70347331018626,3.64608112095067,38.4838001955884));
#193042=CARTESIAN_POINT('Ctrl Pts',(5.60634232328536,3.79372483537982,38.492116127643));
#193043=CARTESIAN_POINT('Ctrl Pts',(5.50368078018955,3.93723086315397,38.5004320596976));
#193044=CARTESIAN_POINT('Ctrl Pts',(5.42629232840349,4.04540875505498,38.5067007859164));
#193045=CARTESIAN_POINT('Ctrl Pts',(5.34576205238126,4.15123602449831,38.5129695121352));
#193046=CARTESIAN_POINT('Ctrl Pts',(5.26225041479912,4.25452812564995,38.519238238354));
#193047=CARTESIAN_POINT('Ctrl Pts',(5.1496660934682,4.39377903059797,38.5276892795189));
#193048=CARTESIAN_POINT('Ctrl Pts',(5.03145549337433,4.52867658034508,38.5361403206837));
#193049=CARTESIAN_POINT('Ctrl Pts',(4.90798055367651,4.65875690337382,38.5445913618486));
#193050=CARTESIAN_POINT('Ctrl Pts',(4.78461598664243,4.78872094927146,38.5530348487362));
#193051=CARTESIAN_POINT('Ctrl Pts',(4.6559966870466,4.91387611205978,38.5614783356238));
#193052=CARTESIAN_POINT('Ctrl Pts',(4.52252456739381,5.03379186471982,38.5699218225115));
#193053=CARTESIAN_POINT('Ctrl Pts',(4.38917673031639,5.15359595781675,38.5783574472456));
#193054=CARTESIAN_POINT('Ctrl Pts',(4.25098533229574,5.26817015116777,38.5867930719797));
#193055=CARTESIAN_POINT('Ctrl Pts',(4.10838885729898,5.37712097662137,38.5952286967138));
#193056=CARTESIAN_POINT('Ctrl Pts',(3.96587158772197,5.48601128518028,38.6036596358678));
#193057=CARTESIAN_POINT('Ctrl Pts',(3.81895438078495,5.58928425063585,38.6120905750219));
#193058=CARTESIAN_POINT('Ctrl Pts',(3.66810911342265,5.68658636899377,38.620521514176));
#193059=CARTESIAN_POINT('Ctrl Pts',(3.51733768316777,5.78384085902969,38.6289483264776));
#193060=CARTESIAN_POINT('Ctrl Pts',(3.36264230529054,5.8751301513764,38.6373751387792));
#193061=CARTESIAN_POINT('Ctrl Pts',(3.20452439648501,5.96014365534358,38.6458019510809));
#193062=CARTESIAN_POINT('Ctrl Pts',(3.16955046628708,5.97894770085678,38.6476658686311));
#193063=CARTESIAN_POINT('Ctrl Pts',(3.13440919851847,5.99744487709346,38.6495297861813));
#193064=CARTESIAN_POINT('Ctrl Pts',(3.0991061983213,6.01563211736942,38.6513937037315));
#193065=CARTESIAN_POINT('Origin',(0.,0.,4.30282021618968));
#193066=CARTESIAN_POINT('',(3.09910619832129,6.01563211736942,41.0459058825584));
#193067=CARTESIAN_POINT('',(3.09910619832134,6.0156321173694,40.651395695404));
#193068=CARTESIAN_POINT('',(3.09910619832133,6.0156321173694,4.30282021618968));
#193069=CARTESIAN_POINT('',(-6.76699683428592,-0.00454281799175943,39.69717978381));
#193070=CARTESIAN_POINT('Ctrl Pts',(-6.76699342768056,-0.00943131635262364,
39.69717978381));
#193071=CARTESIAN_POINT('Ctrl Pts',(-6.76668020929751,-0.234166301401713,
39.7077500331228));
#193072=CARTESIAN_POINT('Ctrl Pts',(-6.7551688358066,-0.458328916408552,
39.7183202824357));
#193073=CARTESIAN_POINT('Ctrl Pts',(-6.73264806908026,-0.680983830872519,
39.7288905317485));
#193074=CARTESIAN_POINT('Ctrl Pts',(-6.70948849224833,-0.909954436589295,
39.7397606101995));
#193075=CARTESIAN_POINT('Ctrl Pts',(-6.67468607867271,-1.1373308841783,
39.7506306886506));
#193076=CARTESIAN_POINT('Ctrl Pts',(-6.62849165631605,-1.36212604488297,
39.7615007671016));
#193077=CARTESIAN_POINT('Ctrl Pts',(-6.62183218103256,-1.39453294035194,
39.7630678181671));
#193078=CARTESIAN_POINT('Ctrl Pts',(-6.61493602539058,-1.42688623496732,
39.7646348692326));
#193079=CARTESIAN_POINT('Ctrl Pts',(-6.60780401710258,-1.45918301510227,
39.7662019202981));
#193080=CARTESIAN_POINT('Ctrl Pts',(-6.56987898044705,-1.63092378165966,
39.7745348423448));
#193081=CARTESIAN_POINT('Ctrl Pts',(-6.52520557100435,-1.80140561528577,
39.7828677643916));
#193082=CARTESIAN_POINT('Ctrl Pts',(-6.47388023008809,-1.97006694466829,
39.7912006864383));
#193083=CARTESIAN_POINT('Ctrl Pts',(-6.42261554327828,-2.13852895726023,
39.7995237609919));
#193084=CARTESIAN_POINT('Ctrl Pts',(-6.36471468509409,-2.30517442132003,
39.8078468355455));
#193085=CARTESIAN_POINT('Ctrl Pts',(-6.300325068815,-2.46945196901282,39.8161699100991));
#193086=CARTESIAN_POINT('Ctrl Pts',(-6.23599972636393,-2.63356553456907,
39.8244846765451));
#193087=CARTESIAN_POINT('Ctrl Pts',(-6.16519865644741,-2.79531557098695,
39.832799442991));
#193088=CARTESIAN_POINT('Ctrl Pts',(-6.08811909765784,-2.95416567794258,
39.841114209437));
#193089=CARTESIAN_POINT('Ctrl Pts',(-6.01110234083374,-3.11288635889876,
39.8494222012766));
#193090=CARTESIAN_POINT('Ctrl Pts',(-5.92781743946158,-3.26871150671735,
39.8577301931161));
#193091=CARTESIAN_POINT('Ctrl Pts',(-5.83850985964285,-3.42112432087073,
39.8660381849556));
#193092=CARTESIAN_POINT('Ctrl Pts',(-5.74925867170873,-3.57344089631911,
39.8743409308427));
#193093=CARTESIAN_POINT('Ctrl Pts',(-5.65399255952059,-3.72234913273447,
39.8826436767298));
#193094=CARTESIAN_POINT('Ctrl Pts',(-5.55300318273677,-3.86735628724784,
39.8909464226169));
#193095=CARTESIAN_POINT('Ctrl Pts',(-5.45205507709289,-4.01230418195826,
39.8992457754363));
#193096=CARTESIAN_POINT('Ctrl Pts',(-5.34538856584358,-4.15335388636473,
39.9075451282557));
#193097=CARTESIAN_POINT('Ctrl Pts',(-5.23333909169961,-4.2900409032186,
39.9158444810752));
#193098=CARTESIAN_POINT('Ctrl Pts',(-5.12131344859866,-4.42669884903752,
39.9241420687615));
#193099=CARTESIAN_POINT('Ctrl Pts',(-5.00390734386614,-4.55899568693043,
39.9324396564479));
#193100=CARTESIAN_POINT('Ctrl Pts',(-4.88149718358398,-4.68649914612835,
39.9407372441342));
#193101=CARTESIAN_POINT('Ctrl Pts',(-4.75909271634931,-4.8139966753998,
39.9490344459166));
#193102=CARTESIAN_POINT('Ctrl Pts',(-4.63168489837398,-4.93670101938003,
39.9573316476991));
#193103=CARTESIAN_POINT('Ctrl Pts',(-4.49968787701916,-5.05421586493956,
39.9656288494815));
#193104=CARTESIAN_POINT('Ctrl Pts',(-4.36767506091743,-5.17174477231069,
39.973927044106));
#193105=CARTESIAN_POINT('Ctrl Pts',(-4.23107220743187,-5.28408271302187,
39.9822252387306));
#193106=CARTESIAN_POINT('Ctrl Pts',(-4.09032763674328,-5.39087273306412,
39.9905234333551));
#193107=CARTESIAN_POINT('Ctrl Pts',(-3.94948407875723,-5.49773785977248,
39.9988274641967));
#193108=CARTESIAN_POINT('Ctrl Pts',(-3.80449326047922,-5.59904705846489,
40.0071314950383));
#193109=CARTESIAN_POINT('Ctrl Pts',(-3.65583439928966,-5.69448538895047,
40.0154355258798));
#193110=CARTESIAN_POINT('Ctrl Pts',(-3.50712148164643,-5.78995842343991,
40.0237425762956));
#193111=CARTESIAN_POINT('Ctrl Pts',(-3.35473815937241,-5.87955615306873,
40.0320496267113));
#193112=CARTESIAN_POINT('Ctrl Pts',(-3.19918969215561,-5.96300883058254,
40.040356677127));
#193113=CARTESIAN_POINT('Ctrl Pts',(-3.04347491737529,-6.046550733093,40.0486726091817));
#193114=CARTESIAN_POINT('Ctrl Pts',(-2.88458854646557,-6.12393429831167,
40.0569885412363));
#193115=CARTESIAN_POINT('Ctrl Pts',(-2.72305832466099,-6.19493683264765,
40.0653044732909));
#193116=CARTESIAN_POINT('Ctrl Pts',(-2.60129341245105,-6.24846005117306,
40.0715731995099));
#193117=CARTESIAN_POINT('Ctrl Pts',(-2.47802660277811,-6.29835824701142,
40.0778419257288));
#193118=CARTESIAN_POINT('Ctrl Pts',(-2.35349007810612,-6.34455462993708,
40.0841106519477));
#193119=CARTESIAN_POINT('Ctrl Pts',(-2.18561433068993,-6.4068275441042,
40.0925609206711));
#193120=CARTESIAN_POINT('Ctrl Pts',(-2.01512298024384,-6.46248632007681,
40.1010111893944));
#193121=CARTESIAN_POINT('Ctrl Pts',(-1.84256388736499,-6.51131686534901,
40.1094614581177));
#193122=CARTESIAN_POINT('Ctrl Pts',(-1.67015708373984,-6.56010431600838,
40.1179042691923));
#193123=CARTESIAN_POINT('Ctrl Pts',(-1.49568649251017,-6.60207545729679,
40.1263470802668));
#193124=CARTESIAN_POINT('Ctrl Pts',(-1.31971734153615,-6.63706525042874,
40.1347898913413));
#193125=CARTESIAN_POINT('Ctrl Pts',(-1.14387953065585,-6.67202892783142,
40.143226400859));
#193126=CARTESIAN_POINT('Ctrl Pts',(-0.96654571384302,-6.7000215799563,
40.1516629103767));
#193127=CARTESIAN_POINT('Ctrl Pts',(-0.788293969984889,-6.72092862756967,
40.1600994198945));
#193128=CARTESIAN_POINT('Ctrl Pts',(-0.610169774840731,-6.74182071506552,
40.1685298926357));
#193129=CARTESIAN_POINT('Ctrl Pts',(-0.431129291323293,-6.75563727271,40.1769603653769));
#193130=CARTESIAN_POINT('Ctrl Pts',(-0.251758636464925,-6.762315179653,
40.1853908381181));
#193131=CARTESIAN_POINT('Ctrl Pts',(-0.0724650925651713,-6.76899021578189,
40.1938176866219));
#193132=CARTESIAN_POINT('Ctrl Pts',(0.107158008968874,-6.76853270682738,
40.2022445351258));
#193133=CARTESIAN_POINT('Ctrl Pts',(0.286520948093409,-6.76093149989731,
40.2106713836296));
#193134=CARTESIAN_POINT('Ctrl Pts',(0.465828524284084,-6.75333263918836,
40.2190956310662));
#193135=CARTESIAN_POINT('Ctrl Pts',(0.644875767309722,-6.73859449182824,
40.2275198785029));
#193136=CARTESIAN_POINT('Ctrl Pts',(0.823074106626459,-6.71675799884149,
40.2359441259395));
#193137=CARTESIAN_POINT('Ctrl Pts',(0.873283580672546,-6.71060531059489,
40.2383177565505));
#193138=CARTESIAN_POINT('Ctrl Pts',(0.923425681025626,-6.70388940388024,
40.2406913871614));
#193139=CARTESIAN_POINT('Ctrl Pts',(0.973487306479602,-6.69661193919157,
40.2430650177724));
#193140=CARTESIAN_POINT('Ctrl Pts',(1.15526377209883,-6.67018707188496,
40.2516837987096));
#193141=CARTESIAN_POINT('Ctrl Pts',(1.33589730369004,-6.63636620633356,
40.2603025796469));
#193142=CARTESIAN_POINT('Ctrl Pts',(1.51478534096077,-6.59527970375862,
40.2689213605841));
#193143=CARTESIAN_POINT('Ctrl Pts',(1.69378083518798,-6.55416852077135,
40.2775453187706));
#193144=CARTESIAN_POINT('Ctrl Pts',(1.87102844613696,-6.50578305878432,
40.2861692769572));
#193145=CARTESIAN_POINT('Ctrl Pts',(2.04593908903496,-6.45030404275324,
40.2947932351437));
#193146=CARTESIAN_POINT('Ctrl Pts',(2.22716865667085,-6.39282075916574,
40.3037287475148));
#193147=CARTESIAN_POINT('Ctrl Pts',(2.40588891227613,-6.32772194894361,
40.312664259886));
#193148=CARTESIAN_POINT('Ctrl Pts',(2.5814659768532,-6.25526357640902,40.3215997722571));
#193149=CARTESIAN_POINT('Ctrl Pts',(2.75123802279417,-6.18520085961636,
40.3302398541518));
#193150=CARTESIAN_POINT('Ctrl Pts',(2.91807113745933,-6.10825761238182,
40.3388799360465));
#193151=CARTESIAN_POINT('Ctrl Pts',(3.08141586475482,-6.02471287850611,
40.3475200179412));
#193152=CARTESIAN_POINT('Ctrl Pts',(3.2531384658705,-5.93688317473671,40.3566032455505));
#193153=CARTESIAN_POINT('Ctrl Pts',(3.42100510273873,-5.84175721689526,
40.3656864731598));
#193154=CARTESIAN_POINT('Ctrl Pts',(3.58440980035587,-5.73971213416778,
40.3747697007692));
#193155=CARTESIAN_POINT('Ctrl Pts',(3.74781449797301,-5.6376670514403,40.3838529283785));
#193156=CARTESIAN_POINT('Ctrl Pts',(3.90675695553529,-5.52870309084873,
40.3929361559879));
#193157=CARTESIAN_POINT('Ctrl Pts',(4.06066906516457,-5.41324816937257,
40.4020193835972));
#193158=CARTESIAN_POINT('Ctrl Pts',(4.21392655638789,-5.29828430033433,
40.411063978457));
#193159=CARTESIAN_POINT('Ctrl Pts',(4.36233845402035,-5.17677910252117,
40.4201085733168));
#193160=CARTESIAN_POINT('Ctrl Pts',(4.5053754838023,-5.0491465367875,40.4291531681767));
#193161=CARTESIAN_POINT('Ctrl Pts',(4.64828125459441,-4.92163109402313,
40.438189463197));
#193162=CARTESIAN_POINT('Ctrl Pts',(4.78582182752243,-4.78799966758519,
40.4472257582174));
#193163=CARTESIAN_POINT('Ctrl Pts',(4.91750174242367,-4.64870579981786,
40.4562620532377));
#193164=CARTESIAN_POINT('Ctrl Pts',(5.04894863938934,-4.50965842347277,
40.4652823578255));
#193165=CARTESIAN_POINT('Ctrl Pts',(5.17455542446903,-4.36496878737805,
40.4743026624132));
#193166=CARTESIAN_POINT('Ctrl Pts',(5.29386426519827,-4.21512634942973,
40.4833229670009));
#193167=CARTESIAN_POINT('Ctrl Pts',(5.41302285961901,-4.06547260892428,
40.4923319122672));
#193168=CARTESIAN_POINT('Ctrl Pts',(5.52589918957355,-3.91067920183336,
40.5013408575335));
#193169=CARTESIAN_POINT('Ctrl Pts',(5.63207471618558,-3.75126957059914,
40.5103498027998));
#193170=CARTESIAN_POINT('Ctrl Pts',(5.73800914065386,-3.59222192489072,
40.5193382906586));
#193171=CARTESIAN_POINT('Ctrl Pts',(5.83727300280782,-3.42857917657921,
40.5283267785174));
#193172=CARTESIAN_POINT('Ctrl Pts',(5.92949047881157,-3.26089430397291,
40.5373152663762));
#193173=CARTESIAN_POINT('Ctrl Pts',(6.01039862216227,-3.11377390664147,
40.5452014273915));
#193174=CARTESIAN_POINT('Ctrl Pts',(6.08588322532871,-2.96354258947786,
40.5530875884067));
#193175=CARTESIAN_POINT('Ctrl Pts',(6.15571725662143,-2.81059318588322,
40.560973749422));
#193176=CARTESIAN_POINT('Ctrl Pts',(6.22763496535337,-2.65308014453613,
40.5690952142782));
#193177=CARTESIAN_POINT('Ctrl Pts',(6.29352619185559,-2.49275422514349,
40.5772166791343));
#193178=CARTESIAN_POINT('Ctrl Pts',(6.35317349719531,-2.3301234977003,40.5853381439905));
#193179=CARTESIAN_POINT('Ctrl Pts',(6.4128165488043,-2.16750436822152,40.5934590296667));
#193180=CARTESIAN_POINT('Ctrl Pts',(6.4662164401011,-2.00258110188059,40.6015799153428));
#193181=CARTESIAN_POINT('Ctrl Pts',(6.5132045425492,-1.83588005787863,40.609700801019));
#193182=CARTESIAN_POINT('Ctrl Pts',(6.56019826141917,-1.66915908833511,
40.6178226573733));
#193183=CARTESIAN_POINT('Ctrl Pts',(6.60077856718998,-1.50066027077619,
40.6259445137275));
#193184=CARTESIAN_POINT('Ctrl Pts',(6.63482721003681,-1.33092332346952,
40.6340663700818));
#193185=CARTESIAN_POINT('Ctrl Pts',(6.66890069435223,-1.161062538186,40.6421941520419));
#193186=CARTESIAN_POINT('Ctrl Pts',(6.69643292580591,-0.989962178373673,
40.6503219340021));
#193187=CARTESIAN_POINT('Ctrl Pts',(6.71735701744158,-0.818170948047107,
40.6584497159622));
#193188=CARTESIAN_POINT('Ctrl Pts',(6.73828963277449,-0.646309736358405,
40.6665808088787));
#193189=CARTESIAN_POINT('Ctrl Pts',(6.75260871229353,-0.473757457852254,
40.6747119017951));
#193190=CARTESIAN_POINT('Ctrl Pts',(6.76029942933705,-0.3010658162349,40.6828429947116));
#193191=CARTESIAN_POINT('Ctrl Pts',(6.7679985404768,-0.128185688907929,
40.6909829623761));
#193192=CARTESIAN_POINT('Ctrl Pts',(6.76905483703964,0.0448337396062329,
40.6991229300406));
#193193=CARTESIAN_POINT('Ctrl Pts',(6.76350559395359,0.217442131516707,
40.7072628977052));
#193194=CARTESIAN_POINT('Ctrl Pts',(6.76062751655525,0.30696430667064,40.7114846368857));
#193195=CARTESIAN_POINT('Ctrl Pts',(6.75597346216984,0.39637600283174,40.7157063760662));
#193196=CARTESIAN_POINT('Ctrl Pts',(6.7495540892548,0.485601272881148,40.7199281152467));
#193197=CARTESIAN_POINT('Ctrl Pts',(6.73672031396149,0.66398272562659,40.7283683247043));
#193198=CARTESIAN_POINT('Ctrl Pts',(6.71680114117658,0.841987289132607,
40.7368085341619));
#193199=CARTESIAN_POINT('Ctrl Pts',(6.68983319393488,1.01902936038517,40.7452487436196));
#193200=CARTESIAN_POINT('Ctrl Pts',(6.66288567890855,1.19593729603986,40.7536825583681));
#193201=CARTESIAN_POINT('Ctrl Pts',(6.62890008537371,1.3718838646168,40.7621163731167));
#193202=CARTESIAN_POINT('Ctrl Pts',(6.58796484463954,1.54628852604988,40.7705501878652));
#193203=CARTESIAN_POINT('Ctrl Pts',(6.54705432556735,1.72058786080084,40.7789789092538));
#193204=CARTESIAN_POINT('Ctrl Pts',(6.4992026027077,1.89334682102212,40.7874076306423));
#193205=CARTESIAN_POINT('Ctrl Pts',(6.44454926603385,2.06399461182983,40.7958363520309));
#193206=CARTESIAN_POINT('Ctrl Pts',(6.38992054321726,2.23456554913469,40.8042612774326));
#193207=CARTESIAN_POINT('Ctrl Pts',(6.32849641580291,2.40302689573561,40.8126862028343));
#193208=CARTESIAN_POINT('Ctrl Pts',(6.26046655459002,2.56882220460269,40.8211111282361));
#193209=CARTESIAN_POINT('Ctrl Pts',(6.19245689373339,2.73456828326046,40.8295335519938));
#193210=CARTESIAN_POINT('Ctrl Pts',(6.11784553712781,2.89764959468847,40.8379559757516));
#193211=CARTESIAN_POINT('Ctrl Pts',(6.03687073963793,3.05752852364511,40.8463783995093));
#193212=CARTESIAN_POINT('Ctrl Pts',(5.95589466864763,3.21740996703697,40.8548009557275));
#193213=CARTESIAN_POINT('Ctrl Pts',(5.86855510151997,3.37408862689546,40.8632235119457));
#193214=CARTESIAN_POINT('Ctrl Pts',(5.7751371142008,3.52704980290618,40.8716460681639));
#193215=CARTESIAN_POINT('Ctrl Pts',(5.6817159712043,3.68001614597441,40.8800689088977));
#193216=CARTESIAN_POINT('Ctrl Pts',(5.58221617232746,3.8292644700334,40.8884917496314));
#193217=CARTESIAN_POINT('Ctrl Pts',(5.47696723431399,3.97430735024997,40.8969145903652));
#193218=CARTESIAN_POINT('Ctrl Pts',(5.37170004705555,4.1193753796329,40.9053388915458));
#193219=CARTESIAN_POINT('Ctrl Pts',(5.2606819291352,4.26023624141864,40.9137631927264));
#193220=CARTESIAN_POINT('Ctrl Pts',(5.14428416441681,4.39643371788208,40.9221874939071));
#193221=CARTESIAN_POINT('Ctrl Pts',(5.02784996194912,4.53267383029747,40.9306144322739));
#193222=CARTESIAN_POINT('Ctrl Pts',(4.90603297172752,4.66424739337065,40.9390413706407));
#193223=CARTESIAN_POINT('Ctrl Pts',(4.77924321713337,4.79073306201511,40.9474683090075));
#193224=CARTESIAN_POINT('Ctrl Pts',(4.65233946261239,4.9173324571749,40.9559028242512));
#193225=CARTESIAN_POINT('Ctrl Pts',(4.5204542460474,5.03883458120982,40.9643373394948));
#193226=CARTESIAN_POINT('Ctrl Pts',(4.38403357908909,5.15485582508563,40.9727718547385));
#193227=CARTESIAN_POINT('Ctrl Pts',(4.24754701977988,5.27093310821624,40.9812104439253));
#193228=CARTESIAN_POINT('Ctrl Pts',(4.10652090021877,5.38152402168038,40.989649033112));
#193229=CARTESIAN_POINT('Ctrl Pts',(3.96143285981027,5.48628642136149,40.9980876222988));
#193230=CARTESIAN_POINT('Ctrl Pts',(3.81618264379811,5.59116592170342,41.0065356439191));
#193231=CARTESIAN_POINT('Ctrl Pts',(3.66686170979056,5.6902037016385,41.0149836655394));
#193232=CARTESIAN_POINT('Ctrl Pts',(3.51397613290303,5.78310130789595,41.0234316871597));
#193233=CARTESIAN_POINT('Ctrl Pts',(3.42707842456215,5.83590281643894,41.0282334070719));
#193234=CARTESIAN_POINT('Ctrl Pts',(3.33902958718176,5.88672151057191,41.033035126984));
#193235=CARTESIAN_POINT('Ctrl Pts',(3.24992584954597,5.93550932713048,41.0378368468961));
#193236=CARTESIAN_POINT('Ctrl Pts',(3.20001448099601,5.96283777324972,41.0405265254502));
#193237=CARTESIAN_POINT('Ctrl Pts',(3.14973585451903,5.98954895964303,41.0432162040043));
#193238=CARTESIAN_POINT('Ctrl Pts',(3.09910619832129,6.01563211736942,41.0459058825584));
#193239=CARTESIAN_POINT('Ctrl Pts',(3.09910619832132,6.01563211736941,39.0457552630242));
#193240=CARTESIAN_POINT('Ctrl Pts',(2.93375330764821,6.10081787314655,39.0545047109265));
#193241=CARTESIAN_POINT('Ctrl Pts',(2.76488627843062,6.17918207037043,39.0632541588288));
#193242=CARTESIAN_POINT('Ctrl Pts',(2.59307866646691,6.25045854554002,39.0720036067311));
#193243=CARTESIAN_POINT('Ctrl Pts',(2.42127244185369,6.3217344451504,39.0807529839814));
#193244=CARTESIAN_POINT('Ctrl Pts',(2.24652594672461,6.38592262741839,39.0895023612317));
#193245=CARTESIAN_POINT('Ctrl Pts',(2.06943269687121,6.44280508110562,39.098251738482));
#193246=CARTESIAN_POINT('Ctrl Pts',(1.89234081822083,6.49968709436164,39.1070010479874));
#193247=CARTESIAN_POINT('Ctrl Pts',(1.71290249405601,6.54926340459541,39.1157503574927));
#193248=CARTESIAN_POINT('Ctrl Pts',(1.53172716625078,6.59136563150379,39.1244996669981));
#193249=CARTESIAN_POINT('Ctrl Pts',(1.35055318107349,6.63346754640707,39.1332489116653));
#193250=CARTESIAN_POINT('Ctrl Pts',(1.16764249714429,6.66809542395774,39.1419981563325));
#193251=CARTESIAN_POINT('Ctrl Pts',(0.983616340614404,6.69513165624667,
39.1507474009998));
#193252=CARTESIAN_POINT('Ctrl Pts',(0.799591486713889,6.7221676971596,39.1594965837355));
#193253=CARTESIAN_POINT('Ctrl Pts',(0.614451459526761,6.74161215869371,
39.1682457664712));
#193254=CARTESIAN_POINT('Ctrl Pts',(0.428825047910331,6.75339900185712,
39.1769949492069));
#193255=CARTESIAN_POINT('Ctrl Pts',(0.243199888597193,6.7651857655022,39.1857440729174));
#193256=CARTESIAN_POINT('Ctrl Pts',(0.0570886373921646,6.76931499599834,
39.1944931966279));
#193257=CARTESIAN_POINT('Ctrl Pts',(-0.128876626810802,6.76577266947848,
39.2032423203385));
#193258=CARTESIAN_POINT('Ctrl Pts',(-0.314840698187818,6.76223036567995,
39.21199138793));
#193259=CARTESIAN_POINT('Ctrl Pts',(-0.500658497950919,6.75101660879225,
39.2207404555216));
#193260=CARTESIAN_POINT('Ctrl Pts',(-0.68569895192589,6.73216948296222,
39.2294895231131));
#193261=CARTESIAN_POINT('Ctrl Pts',(-0.870738280459308,6.713322471763,39.2382385374916));
#193262=CARTESIAN_POINT('Ctrl Pts',(-1.05499998761175,6.68684221356198,
39.2469875518701));
#193263=CARTESIAN_POINT('Ctrl Pts',(-1.23785829161323,6.6528186394854,39.2557365662486));
#193264=CARTESIAN_POINT('Ctrl Pts',(-1.4300741291731,6.61705395368882,39.2649332999478));
#193265=CARTESIAN_POINT('Ctrl Pts',(-1.62073882535701,6.57295372727812,
39.274130033647));
#193266=CARTESIAN_POINT('Ctrl Pts',(-1.80913696091426,6.52068343478304,
39.2833267673462));
#193267=CARTESIAN_POINT('Ctrl Pts',(-1.98838356186025,6.47095219815225,
39.2920767650599));
#193268=CARTESIAN_POINT('Ctrl Pts',(-2.16557827572447,6.4138258685092,39.3008267627736));
#193269=CARTESIAN_POINT('Ctrl Pts',(-2.34011918621615,6.34949849943309,
39.3095767604872));
#193270=CARTESIAN_POINT('Ctrl Pts',(-2.51465655691014,6.28517243495584,
39.3183265807455));
#193271=CARTESIAN_POINT('Ctrl Pts',(-2.68653996295244,6.21364572242411,
39.3270764010039));
#193272=CARTESIAN_POINT('Ctrl Pts',(-2.85518555379905,6.1351613225226,39.3358262212622));
#193273=CARTESIAN_POINT('Ctrl Pts',(-3.02382794858611,6.05667841000546,
39.3445758756997));
#193274=CARTESIAN_POINT('Ctrl Pts',(-3.18923239109208,5.9712381949212,39.3533255301372));
#193275=CARTESIAN_POINT('Ctrl Pts',(-3.35083705967631,5.87913088810751,
39.3620751845747));
#193276=CARTESIAN_POINT('Ctrl Pts',(-3.51243888042335,5.78702520443143,
39.3708246848236));
#193277=CARTESIAN_POINT('Ctrl Pts',(-3.67024081223627,5.68825280605824,
39.3795741850726));
#193278=CARTESIAN_POINT('Ctrl Pts',(-3.8237068754434,5.58314917682547,39.3883236853215));
#193279=CARTESIAN_POINT('Ctrl Pts',(-3.97717043817747,5.47804726008071,
39.397073043012));
#193280=CARTESIAN_POINT('Ctrl Pts',(-4.12629803722385,5.36661448084293,
39.4058224007024));
#193281=CARTESIAN_POINT('Ctrl Pts',(-4.27058317206826,5.24922931204643,
39.4145717583929));
#193282=CARTESIAN_POINT('Ctrl Pts',(-4.41486614774757,5.13184589986858,
39.423320985153));
#193283=CARTESIAN_POINT('Ctrl Pts',(-4.55430658194339,5.00851045723103,
39.4320702119131));
#193284=CARTESIAN_POINT('Ctrl Pts',(-4.68843089001774,4.87964187103188,
39.4408194386731));
#193285=CARTESIAN_POINT('Ctrl Pts',(-4.82255336917779,4.7507750420802,39.4495685461291));
#193286=CARTESIAN_POINT('Ctrl Pts',(-4.95135966065089,4.61637541908142,
39.458317653585));
#193287=CARTESIAN_POINT('Ctrl Pts',(-5.07441230869211,4.47689945401882,
39.4670667610409));
#193288=CARTESIAN_POINT('Ctrl Pts',(-5.19746344226393,4.33742520555545,
39.4758157608173));
#193289=CARTESIAN_POINT('Ctrl Pts',(-5.31476088454752,4.19287495491357,
39.4845647605937));
#193290=CARTESIAN_POINT('Ctrl Pts',(-5.42590627628846,4.04373961586716,
39.49331376037));
#193291=CARTESIAN_POINT('Ctrl Pts',(-5.53706380672662,3.89458798906743,
39.5020637156647));
#193292=CARTESIAN_POINT('Ctrl Pts',(-5.6420677707186,3.74085050155291,39.5108136709594));
#193293=CARTESIAN_POINT('Ctrl Pts',(-5.74056148164005,3.58304938223166,
39.5195636262541));
#193294=CARTESIAN_POINT('Ctrl Pts',(-5.83905138951876,3.42525435593295,
39.5283132436952));
#193295=CARTESIAN_POINT('Ctrl Pts',(-5.93103139557641,3.26339625497204,
39.5370628611363));
#193296=CARTESIAN_POINT('Ctrl Pts',(-6.01618907820831,3.09802485065034,
39.5458124785775));
#193297=CARTESIAN_POINT('Ctrl Pts',(-6.10134392544966,2.93265895249676,
39.5545618046933));
#193298=CARTESIAN_POINT('Ctrl Pts',(-6.17967677261813,2.76378023986076,
39.5633111308092));
#193299=CARTESIAN_POINT('Ctrl Pts',(-6.25092157009205,2.59196229227162,
39.572060456925));
#193300=CARTESIAN_POINT('Ctrl Pts',(-6.32216437407752,2.42014915229098,
39.5808095382275));
#193301=CARTESIAN_POINT('Ctrl Pts',(-6.38631941548934,2.24539720662817,
39.58955861953));
#193302=CARTESIAN_POINT('Ctrl Pts',(-6.44316881037562,2.0682999494761,39.5983077008325));
#193303=CARTESIAN_POINT('Ctrl Pts',(-6.50002334524594,1.89118668024373,
39.6070575731748));
#193304=CARTESIAN_POINT('Ctrl Pts',(-6.54957082411117,1.71172794807624,
39.6158074455172));
#193305=CARTESIAN_POINT('Ctrl Pts',(-6.59164294296102,1.5305333425026,39.6245573178595));
#193306=CARTESIAN_POINT('Ctrl Pts',(-6.63371214082151,1.34935131693515,
39.6333065827144));
#193307=CARTESIAN_POINT('Ctrl Pts',(-6.66830695239706,1.16643393829675,
39.6420558475693));
#193308=CARTESIAN_POINT('Ctrl Pts',(-6.69530988154002,0.982402458340054,
39.6508051124242));
#193309=CARTESIAN_POINT('Ctrl Pts',(-6.72231419690493,0.798361530946196,
39.6595548264312));
#193310=CARTESIAN_POINT('Ctrl Pts',(-6.74172580829285,0.613206671361688,
39.6683045404383));
#193311=CARTESIAN_POINT('Ctrl Pts',(-6.75347878028184,0.427566795112685,
39.6770542544453));
#193312=CARTESIAN_POINT('Ctrl Pts',(-6.76248992368219,0.285234494204469,
39.6837627642336));
#193313=CARTESIAN_POINT('Ctrl Pts',(-6.76699999999999,0.142617266091236,
39.6904712740218));
#193314=CARTESIAN_POINT('Ctrl Pts',(-6.767,4.55836674798597E-13,39.6971797838101));
#193315=CARTESIAN_POINT('',(-6.76699999743973,-0.000186146809638267,39.3028289722665));
#193316=CARTESIAN_POINT('Ctrl Pts',(3.0991061983213,6.01563211736942,38.6513937037315));
#193317=CARTESIAN_POINT('Ctrl Pts',(2.93955787853499,6.09782750052023,38.6598174895769));
#193318=CARTESIAN_POINT('Ctrl Pts',(2.77670433697083,6.173688756113,38.6682412754222));
#193319=CARTESIAN_POINT('Ctrl Pts',(2.61107769107173,6.2429610195153,38.6766650612676));
#193320=CARTESIAN_POINT('Ctrl Pts',(2.60106628553135,6.24714822452604,38.677174242238));
#193321=CARTESIAN_POINT('Ctrl Pts',(2.59104475479507,6.25131136978227,38.6776834232084));
#193322=CARTESIAN_POINT('Ctrl Pts',(2.58101321895029,6.25545040453554,38.6781926041788));
#193323=CARTESIAN_POINT('Ctrl Pts',(2.41121188124054,6.32551082686845,38.6868113851161));
#193324=CARTESIAN_POINT('Ctrl Pts',(2.23861825503386,6.38862789171524,38.6954301660533));
#193325=CARTESIAN_POINT('Ctrl Pts',(2.06381703439645,6.44460613602841,38.7040489469906));
#193326=CARTESIAN_POINT('Ctrl Pts',(1.88891081173156,6.50061800613165,38.712672905177));
#193327=CARTESIAN_POINT('Ctrl Pts',(1.71179463784775,6.54948240489686,38.7212968633634));
#193328=CARTESIAN_POINT('Ctrl Pts',(1.53306732596922,6.59105405637411,38.7299208215498));
#193329=CARTESIAN_POINT('Ctrl Pts',(1.34788320612202,6.63412754977864,38.738856333921));
#193330=CARTESIAN_POINT('Ctrl Pts',(1.16096972126086,6.66937147171092,38.7477918462921));
#193331=CARTESIAN_POINT('Ctrl Pts',(0.97300260833897,6.69668238190864,38.7567273586633));
#193332=CARTESIAN_POINT('Ctrl Pts',(0.791250160164018,6.72309032483632,
38.7653674405579));
#193333=CARTESIAN_POINT('Ctrl Pts',(0.608512947785567,6.74208144528608,
38.7740075224526));
#193334=CARTESIAN_POINT('Ctrl Pts',(0.425405891550251,6.75361524129369,
38.7826476043473));
#193335=CARTESIAN_POINT('Ctrl Pts',(0.232907360987668,6.76574060024446,
38.7917308319567));
#193336=CARTESIAN_POINT('Ctrl Pts',(0.0400004451269104,6.76962356844915,
38.800814059566));
#193337=CARTESIAN_POINT('Ctrl Pts',(-0.152601268419071,6.76527914079507,
38.8098972871754));
#193338=CARTESIAN_POINT('Ctrl Pts',(-0.345202981965021,6.760934713141,38.8189805147848));
#193339=CARTESIAN_POINT('Ctrl Pts',(-0.537499108441993,6.74836294850892,
38.8280637423941));
#193340=CARTESIAN_POINT('Ctrl Pts',(-0.728782699476038,6.72764184368821,
38.8371469700035));
#193341=CARTESIAN_POINT('Ctrl Pts',(-0.919252723859074,6.7070088697927,
38.8461915648633));
#193342=CARTESIAN_POINT('Ctrl Pts',(-1.10889479605317,6.67827754701845,
38.8552361597231));
#193343=CARTESIAN_POINT('Ctrl Pts',(-1.29704248510996,6.64153369274144,
38.8642807545829));
#193344=CARTESIAN_POINT('Ctrl Pts',(-1.48501751904548,6.60482355673463,
38.8733170496033));
#193345=CARTESIAN_POINT('Ctrl Pts',(-1.67150067443269,6.56011561460289,
38.8823533446236));
#193346=CARTESIAN_POINT('Ctrl Pts',(-1.85583439428491,6.50754698031364,
38.8913896396439));
#193347=CARTESIAN_POINT('Ctrl Pts',(-2.03984192116548,6.45507137034489,
38.9004099442316));
#193348=CARTESIAN_POINT('Ctrl Pts',(-2.22170737933003,6.39476291009423,
38.9094302488193));
#193349=CARTESIAN_POINT('Ctrl Pts',(-2.40078723634419,6.32680880427146,
38.918450553407));
#193350=CARTESIAN_POINT('Ctrl Pts',(-2.57964157706582,6.25894027344446,
38.9274594986733));
#193351=CARTESIAN_POINT('Ctrl Pts',(-2.7557170954925,6.18344539577992,38.9364684439396));
#193352=CARTESIAN_POINT('Ctrl Pts',(-2.92838670191392,6.10056065653426,
38.9454773892059));
#193353=CARTESIAN_POINT('Ctrl Pts',(-3.10066421221319,6.01786413098478,
38.9544658770647));
#193354=CARTESIAN_POINT('Ctrl Pts',(-3.26955103437948,5.92781134255887,
38.9634543649236));
#193355=CARTESIAN_POINT('Ctrl Pts',(-3.43444173433328,5.8306859779506,38.9724428527824));
#193356=CARTESIAN_POINT('Ctrl Pts',(-3.57911062972357,5.74547183781903,
38.9803290137977));
#193357=CARTESIAN_POINT('Ctrl Pts',(-3.72070360944361,5.65481422883725,
38.988215174813));
#193358=CARTESIAN_POINT('Ctrl Pts',(-3.85882493124176,5.55893507337755,
38.9961013358283));
#193359=CARTESIAN_POINT('Ctrl Pts',(-4.00106745693917,5.46019511739701,
39.0042228006845));
#193360=CARTESIAN_POINT('Ctrl Pts',(-4.13956345584402,5.35596022666187,
39.0123442655406));
#193361=CARTESIAN_POINT('Ctrl Pts',(-4.27386661478399,5.24655631429177,
39.0204657303968));
#193362=CARTESIAN_POINT('Ctrl Pts',(-4.40816019593243,5.13716020403053,
39.028586616073));
#193363=CARTESIAN_POINT('Ctrl Pts',(-4.5382612487939,5.02259603766209,39.0367075017493));
#193364=CARTESIAN_POINT('Ctrl Pts',(-4.66375609795499,4.90323036974479,
39.0448283874255));
#193365=CARTESIAN_POINT('Ctrl Pts',(-4.78926594733842,4.78385043421754,
39.0529502437797));
#193366=CARTESIAN_POINT('Ctrl Pts',(-4.91016823220562,4.65966810758013,
39.061072100134));
#193367=CARTESIAN_POINT('Ctrl Pts',(-5.026085780008,4.53108714681162,39.0691939564882));
#193368=CARTESIAN_POINT('Ctrl Pts',(-5.14208789981946,4.40241237496455,
39.0773217384484));
#193369=CARTESIAN_POINT('Ctrl Pts',(-5.25309777343552,4.26933283162074,
39.0854495204086));
#193370=CARTESIAN_POINT('Ctrl Pts',(-5.35877780973219,4.13228621781235,
39.0935773023688));
#193371=CARTESIAN_POINT('Ctrl Pts',(-5.46450089614862,3.99518377630609,
39.1017083952853));
#193372=CARTESIAN_POINT('Ctrl Pts',(-5.56488960531525,3.85411134126507,
39.1098394882018));
#193373=CARTESIAN_POINT('Ctrl Pts',(-5.6596495827113,3.7095357662268,39.1179705811183));
#193374=CARTESIAN_POINT('Ctrl Pts',(-5.75451298666182,3.56480239299146,
39.1261105487829));
#193375=CARTESIAN_POINT('Ctrl Pts',(-5.84373519957199,3.41655855625808,
39.1342505164475));
#193376=CARTESIAN_POINT('Ctrl Pts',(-5.92706736736082,3.26529652907152,
39.142390484112));
#193377=CARTESIAN_POINT('Ctrl Pts',(-5.97028703262615,3.18684550162526,
39.1466122232923));
#193378=CARTESIAN_POINT('Ctrl Pts',(-6.01192310687886,3.10758296979167,
39.1508339624726));
#193379=CARTESIAN_POINT('Ctrl Pts',(-6.05194599004669,3.02757968244566,
39.1550557016529));
#193380=CARTESIAN_POINT('Ctrl Pts',(-6.13730252520239,2.85695720679128,
39.1640593765569));
#193381=CARTESIAN_POINT('Ctrl Pts',(-6.21546903201688,2.68266435945838,
39.1730630514608));
#193382=CARTESIAN_POINT('Ctrl Pts',(-6.2861558532949,2.50530109729075,39.1820667263648));
#193383=CARTESIAN_POINT('Ctrl Pts',(-6.3567693877612,2.32812172213015,39.1910610664222));
#193384=CARTESIAN_POINT('Ctrl Pts',(-6.419918626014,2.14787851373907,39.2000554064796));
#193385=CARTESIAN_POINT('Ctrl Pts',(-6.47536170120775,1.9651920614871,39.209049746537));
#193386=CARTESIAN_POINT('Ctrl Pts',(-6.53070441239066,1.78283631140145,
39.218027804885));
#193387=CARTESIAN_POINT('Ctrl Pts',(-6.57836874168706,1.59804638192057,
39.2270058632329));
#193388=CARTESIAN_POINT('Ctrl Pts',(-6.61816240750102,1.41145858881525,
39.2359839215808));
#193389=CARTESIAN_POINT('Ctrl Pts',(-6.65790533220295,1.2251087147837,39.2449505319595));
#193390=CARTESIAN_POINT('Ctrl Pts',(-6.68979756797501,1.03696579016012,
39.2539171423381));
#193391=CARTESIAN_POINT('Ctrl Pts',(-6.71369709982694,0.847679333106166,
39.2628837527167));
#193392=CARTESIAN_POINT('Ctrl Pts',(-6.73754730394719,0.658783556155203,
39.27183185635));
#193393=CARTESIAN_POINT('Ctrl Pts',(-6.7534376990638,0.468749199963441,
39.2807799599832));
#193394=CARTESIAN_POINT('Ctrl Pts',(-6.76127761090634,0.278233837368261,
39.2897280636165));
#193395=CARTESIAN_POINT('Ctrl Pts',(-6.76509309690497,0.185514848544821,
39.294082878417));
#193396=CARTESIAN_POINT('Ctrl Pts',(-6.76700257553491,0.0926820920658435,
39.2984376932176));
#193397=CARTESIAN_POINT('Ctrl Pts',(-6.76699999739247,-0.000187857213484029,
39.3027925080181));
#193398=CARTESIAN_POINT('Ctrl Pts',(-6.76699999743974,-0.000186146809638268,
39.3028289722665));
#193399=CARTESIAN_POINT('Ctrl Pts',(-6.76699488074755,-0.186193396001483,
39.3115784840652));
#193400=CARTESIAN_POINT('Ctrl Pts',(-6.75931613702926,-0.372200290803175,
39.3203279958639));
#193401=CARTESIAN_POINT('Ctrl Pts',(-6.74398984746996,-0.557575050752965,
39.3290775076626));
#193402=CARTESIAN_POINT('Ctrl Pts',(-6.7286636226442,-0.742949027736605,
39.3378269825061));
#193403=CARTESIAN_POINT('Ctrl Pts',(-6.70568994023064,-0.927690589582378,
39.3465764573496));
#193404=CARTESIAN_POINT('Ctrl Pts',(-6.67514683067657,-1.11117225888182,
39.3553259321931));
#193405=CARTESIAN_POINT('Ctrl Pts',(-6.64460384759053,-1.29465316844967,
39.3640753708081));
#193406=CARTESIAN_POINT('Ctrl Pts',(-6.60649154714446,-1.47687391320333,
39.3728248094232));
#193407=CARTESIAN_POINT('Ctrl Pts',(-6.56093937725161,-1.65721558284652,
39.3815742480382));
#193408=CARTESIAN_POINT('Ctrl Pts',(-6.51538739219062,-1.83755652073779,
39.3903236511517));
#193409=CARTESIAN_POINT('Ctrl Pts',(-6.46239566827804,-2.01601812091156,
39.3990730542651));
#193410=CARTESIAN_POINT('Ctrl Pts',(-6.40214418972864,-2.19199424586922,
39.4078224573786));
#193411=CARTESIAN_POINT('Ctrl Pts',(-6.34189295065092,-2.36796967140345,
39.4165718257172));
#193412=CARTESIAN_POINT('Ctrl Pts',(-6.27438210750929,-2.54145937035588,
39.4253211940558));
#193413=CARTESIAN_POINT('Ctrl Pts',(-6.1998409562901,-2.71187409676552,
39.4340705623944));
#193414=CARTESIAN_POINT('Ctrl Pts',(-6.12530009514714,-2.8822881600078,
39.442819896685));
#193415=CARTESIAN_POINT('Ctrl Pts',(-6.04372909552121,-3.04962701209198,
39.4515692309755));
#193416=CARTESIAN_POINT('Ctrl Pts',(-5.95540500560968,-3.21332230240901,
39.4603185652661));
#193417=CARTESIAN_POINT('Ctrl Pts',(-5.86708125207551,-3.37701696930168,
39.4690678662352));
#193418=CARTESIAN_POINT('Ctrl Pts',(-5.77200459580281,-3.53706784999082,
39.4778171672044));
#193419=CARTESIAN_POINT('Ctrl Pts',(-5.67049795321926,-3.69293135091031,
39.4865664681736));
#193420=CARTESIAN_POINT('Ctrl Pts',(-5.5689916887887,-3.84879427117568,
39.4953157365482));
#193421=CARTESIAN_POINT('Ctrl Pts',(-5.46105564237136,-4.00046960275369,
39.5040650049227));
#193422=CARTESIAN_POINT('Ctrl Pts',(-5.34705640303826,-4.14744220245775,
39.5128142732972));
#193423=CARTESIAN_POINT('Ctrl Pts',(-5.23305757893143,-4.29441426683468,
39.5215635098038));
#193424=CARTESIAN_POINT('Ctrl Pts',(-5.11299578173536,-4.43668340718169,
39.5303127463103));
#193425=CARTESIAN_POINT('Ctrl Pts',(-4.98727878090113,-4.57376643058796,
39.5390619828169));
#193426=CARTESIAN_POINT('Ctrl Pts',(-4.86156222753462,-4.71084896607114,
39.547811188182));
#193427=CARTESIAN_POINT('Ctrl Pts',(-4.73019070449323,-4.84274521035855,
39.5565603935472));
#193428=CARTESIAN_POINT('Ctrl Pts',(-4.5936103896132,-4.96900720350028,
39.5653095989123));
#193429=CARTESIAN_POINT('Ctrl Pts',(-4.45703054952563,-5.09526875771901,
39.5740587738628));
#193430=CARTESIAN_POINT('Ctrl Pts',(-4.3152421642509,-5.2158959054666,39.5828079488132));
#193431=CARTESIAN_POINT('Ctrl Pts',(-4.16872678712792,-5.33047896293402,
39.5915571237636));
#193432=CARTESIAN_POINT('Ctrl Pts',(-4.02221190716869,-5.44506163159212,
39.6003062690258));
#193433=CARTESIAN_POINT('Ctrl Pts',(-3.87097029317856,-5.5536000744864,
39.6090554142881));
#193434=CARTESIAN_POINT('Ctrl Pts',(-3.71551560084441,-5.6557256669575,
39.6178045595503));
#193435=CARTESIAN_POINT('Ctrl Pts',(-3.5600614230999,-5.75785092137014,
39.626553675851));
#193436=CARTESIAN_POINT('Ctrl Pts',(-3.40039443440767,-5.85356321050832,
39.6353027921516));
#193437=CARTESIAN_POINT('Ctrl Pts',(-3.23705690162253,-5.94253747280217,
39.6440519084522));
#193438=CARTESIAN_POINT('Ctrl Pts',(-3.07371989595894,-6.031511447959,39.6528009965178));
#193439=CARTESIAN_POINT('Ctrl Pts',(-2.90671262153579,-6.11374730271696,
39.6615500845833));
#193440=CARTESIAN_POINT('Ctrl Pts',(-2.73660227089706,-6.18896574646532,
39.6702991726489));
#193441=CARTESIAN_POINT('Ctrl Pts',(-2.56649245511316,-6.26418395371457,
39.6790482332058));
#193442=CARTESIAN_POINT('Ctrl Pts',(-2.39327984469725,-6.33238467823092,
39.6877972937628));
#193443=CARTESIAN_POINT('Ctrl Pts',(-2.21755270315058,-6.39333629717299,
39.6965463543198));
#193444=CARTESIAN_POINT('Ctrl Pts',(-2.04182609952928,-6.45428772953361,
39.7052953880947));
#193445=CARTESIAN_POINT('Ctrl Pts',(-1.86358525088945,-6.50799000682964,
39.7140444218696));
#193446=CARTESIAN_POINT('Ctrl Pts',(-1.68343549389886,-6.55426074686395,
39.7227934556445));
#193447=CARTESIAN_POINT('Ctrl Pts',(-1.50328627341453,-6.60053134909878,
39.7315424633637));
#193448=CARTESIAN_POINT('Ctrl Pts',(-1.32122843347438,-6.63937038708123,
39.740291471083));
#193449=CARTESIAN_POINT('Ctrl Pts',(-1.13788027022808,-6.67064595752358,
39.7490404788023));
#193450=CARTESIAN_POINT('Ctrl Pts',(-0.954532637792132,-6.70192143742018,
39.7577894611924));
#193451=CARTESIAN_POINT('Ctrl Pts',(-0.769894971967928,-6.72563344541621,
39.7665384435824));
#193452=CARTESIAN_POINT('Ctrl Pts',(-0.584594326759636,-6.74170145238726,
39.7752874259725));
#193453=CARTESIAN_POINT('Ctrl Pts',(-0.391305862408406,-6.75846210850439,
39.7844135537791));
#193454=CARTESIAN_POINT('Ctrl Pts',(-0.197296323759575,-6.76690509100547,
39.7935396815856));
#193455=CARTESIAN_POINT('Ctrl Pts',(-0.00328255830076272,-6.76699920384294,
39.8026658093922));
#193456=CARTESIAN_POINT('Ctrl Pts',(0.184668276987458,-6.76709037565425,
39.8115067457049));
#193457=CARTESIAN_POINT('Ctrl Pts',(0.372622761917631,-6.75934662538464,
39.8203476820175));
#193458=CARTESIAN_POINT('Ctrl Pts',(0.559929103887351,-6.74379480697774,
39.8291886183301));
#193459=CARTESIAN_POINT('Ctrl Pts',(0.745308392054773,-6.72840298951089,
39.8379385969113));
#193460=CARTESIAN_POINT('Ctrl Pts',(0.930052522471095,-6.70536305459828,
39.8466885754926));
#193461=CARTESIAN_POINT('Ctrl Pts',(1.11353393682208,-6.67475326671672,
39.8554385540738));
#193462=CARTESIAN_POINT('Ctrl Pts',(1.29701347289961,-6.64414379218326,
39.8641884430828));
#193463=CARTESIAN_POINT('Ctrl Pts',(1.47923003601286,-6.60596466692396,
39.8729383320917));
#193464=CARTESIAN_POINT('Ctrl Pts',(1.65956466641403,-6.56034557915893,
39.8816882211007));
#193465=CARTESIAN_POINT('Ctrl Pts',(1.83989751068703,-6.51472694322911,
39.8904380234462));
#193466=CARTESIAN_POINT('Ctrl Pts',(2.01834818164281,-6.46166856255618,
39.8991878257917));
#193467=CARTESIAN_POINT('Ctrl Pts',(2.19431052364624,-6.40135066418138,
39.9079376281372));
#193468=CARTESIAN_POINT('Ctrl Pts',(2.37027118130145,-6.34103334318208,
39.9166873467277));
#193469=CARTESIAN_POINT('Ctrl Pts',(2.54374328651165,-6.27345673648762,
39.9254370653183));
#193470=CARTESIAN_POINT('Ctrl Pts',(2.71413760594672,-6.19885038180354,
39.9341867839088));
#193471=CARTESIAN_POINT('Ctrl Pts',(2.88453035095198,-6.12424471647617,
39.9429364216527));
#193472=CARTESIAN_POINT('Ctrl Pts',(3.05184510452406,-6.04260954810436,
39.9516860593966));
#193473=CARTESIAN_POINT('Ctrl Pts',(3.21551355852316,-5.95422216204214,
39.9604356971404));
#193474=CARTESIAN_POINT('Ctrl Pts',(3.37918055462056,-5.86583556330403,
39.9691852569455));
#193475=CARTESIAN_POINT('Ctrl Pts',(3.53920106394761,-5.77069700343036,
39.9779348167507));
#193476=CARTESIAN_POINT('Ctrl Pts',(3.69503156396635,-5.66912962819624,
39.9866843765558));
#193477=CARTESIAN_POINT('Ctrl Pts',(3.85086072767506,-5.56756312394374,
39.9954338613299));
#193478=CARTESIAN_POINT('Ctrl Pts',(4.00249971386974,-5.45956807115004,
40.004183346104));
#193479=CARTESIAN_POINT('Ctrl Pts',(4.14943347735481,-5.34551127741839,
40.0129328308781));
#193480=CARTESIAN_POINT('Ctrl Pts',(4.29636602963781,-5.2314554238779,40.0216822435285));
#193481=CARTESIAN_POINT('Ctrl Pts',(4.43859321043452,-5.11133810512784,
40.030431656179));
#193482=CARTESIAN_POINT('Ctrl Pts',(4.57563194991217,-4.98556729559867,
40.0391810688295));
#193483=CARTESIAN_POINT('Ctrl Pts',(4.71266960527883,-4.85979748104009,
40.0479304122635));
#193484=CARTESIAN_POINT('Ctrl Pts',(4.84451869032434,-4.72837445898066,
40.0566797556975));
#193485=CARTESIAN_POINT('Ctrl Pts',(4.97073139114703,-4.59174459623633,
40.0654290991316));
#193486=CARTESIAN_POINT('Ctrl Pts',(5.09694313542921,-4.45511576898207,
40.0741783762561));
#193487=CARTESIAN_POINT('Ctrl Pts',(5.21751838651698,-4.31328039051357,
40.0829276533806));
#193488=CARTESIAN_POINT('Ctrl Pts',(5.33204762730209,-4.16672018501149,
40.0916769305051));
#193489=CARTESIAN_POINT('Ctrl Pts',(5.44657603813579,-4.02016104157748,
40.1004261442269));
#193490=CARTESIAN_POINT('Ctrl Pts',(5.55505834989452,-3.86887736542261,
40.1091753579486));
#193491=CARTESIAN_POINT('Ctrl Pts',(5.65712612279487,-3.71338296312027,
40.1179245716703));
#193492=CARTESIAN_POINT('Ctrl Pts',(5.75919318994895,-3.55788963598193,
40.1266737248957));
#193493=CARTESIAN_POINT('Ctrl Pts',(5.85484564975599,-3.39818588051262,
40.1354228781211));
#193494=CARTESIAN_POINT('Ctrl Pts',(5.94375864110141,-3.23481409300941,
40.1441720313465));
#193495=CARTESIAN_POINT('Ctrl Pts',(6.03267104718983,-3.07144338087755,
40.1529211269819));
#193496=CARTESIAN_POINT('Ctrl Pts',(6.11484393661448,-2.90440493671046,
40.1616702226172));
#193497=CARTESIAN_POINT('Ctrl Pts',(6.189998232126,-2.73426605989194,40.1704193182526));
#193498=CARTESIAN_POINT('Ctrl Pts',(6.26515205790492,-2.56412824648274,
40.179168359204));
#193499=CARTESIAN_POINT('Ctrl Pts',(6.3332872617796,-2.39089030130223,40.1879174001553));
#193500=CARTESIAN_POINT('Ctrl Pts',(6.39417244446545,-2.21514057125925,
40.1966664411067));
#193501=CARTESIAN_POINT('Ctrl Pts',(6.45505726682384,-2.03939188132899,
40.20541543028));
#193502=CARTESIAN_POINT('Ctrl Pts',(6.50869206006277,-1.86113170702176,
40.2141644194533));
#193503=CARTESIAN_POINT('Ctrl Pts',(6.55489467302792,-1.68096544447239,
40.2229134086265));
#193504=CARTESIAN_POINT('Ctrl Pts',(6.60203583620101,-1.49713932218074,
40.2318401229344));
#193505=CARTESIAN_POINT('Ctrl Pts',(6.64143954473786,-1.31132913720938,
40.2407668372423));
#193506=CARTESIAN_POINT('Ctrl Pts',(6.67296649201383,-1.12419179700824,
40.2496935515501));
#193507=CARTESIAN_POINT('Ctrl Pts',(6.70386902476921,-0.94076085031058,
40.2584434656754));
#193508=CARTESIAN_POINT('Ctrl Pts',(6.72720384226755,-0.75605511923264,
40.2671933798007));
#193509=CARTESIAN_POINT('Ctrl Pts',(6.74289167951043,-0.570702022415406,
40.2759432939259));
#193510=CARTESIAN_POINT('Ctrl Pts',(6.7585792082475,-0.385352570619957,
40.2846930359816));
#193511=CARTESIAN_POINT('Ctrl Pts',(6.76662003348113,-0.199356064193198,
40.2934427780373));
#193512=CARTESIAN_POINT('Ctrl Pts',(6.76698684276469,-0.0133442815295733,
40.302192520093));
#193513=CARTESIAN_POINT('Ctrl Pts',(6.76735364532241,0.172664090404337,
40.3109421017126));
#193514=CARTESIAN_POINT('Ctrl Pts',(6.76004671294439,0.358687451388182,
40.3196916833322));
#193515=CARTESIAN_POINT('Ctrl Pts',(6.74509086433814,0.544093954958275,
40.3284412649518));
#193516=CARTESIAN_POINT('Ctrl Pts',(6.73013527008728,0.729497305304266,
40.3371906977665));
#193517=CARTESIAN_POINT('Ctrl Pts',(6.70753104296859,0.91428353355598,40.3459401305813));
#193518=CARTESIAN_POINT('Ctrl Pts',(6.67735495783224,1.09782501661842,40.354689563396));
#193519=CARTESIAN_POINT('Ctrl Pts',(6.6471793458039,1.2813636220728,40.363438859035));
#193520=CARTESIAN_POINT('Ctrl Pts',(6.60943215980949,1.46365723860794,40.372188154674));
#193521=CARTESIAN_POINT('Ctrl Pts',(6.56424160347017,1.64408672863429,40.3809374503129));
#193522=CARTESIAN_POINT('Ctrl Pts',(6.51905169559535,1.82451362957721,40.3896866204034));
#193523=CARTESIAN_POINT('Ctrl Pts',(6.46641870073413,2.0030761795682,40.3984357904939));
#193524=CARTESIAN_POINT('Ctrl Pts',(6.40652137518049,2.17916793050821,40.4071849605843));
#193525=CARTESIAN_POINT('Ctrl Pts',(6.34662482955081,2.35525738855497,40.4159340167517));
#193526=CARTESIAN_POINT('Ctrl Pts',(6.27946423478602,2.52887584065665,40.4246830729191));
#193527=CARTESIAN_POINT('Ctrl Pts',(6.20526768101723,2.69943364558626,40.4334321290865));
#193528=CARTESIAN_POINT('Ctrl Pts',(6.12824915677822,2.87647839720717,40.4425139443497));
#193529=CARTESIAN_POINT('Ctrl Pts',(6.04364908642058,3.05022481423258,40.4515957596129));
#193530=CARTESIAN_POINT('Ctrl Pts',(5.95177703455489,3.22003713192023,40.4606775748762));
#193531=CARTESIAN_POINT('Ctrl Pts',(5.86326386375463,3.38364103946599,40.469427355133));
#193532=CARTESIAN_POINT('Ctrl Pts',(5.76800116437186,3.54359314647918,40.4781771353899));
#193533=CARTESIAN_POINT('Ctrl Pts',(5.66631252012015,3.69935013540617,40.4869269156467));
#193534=CARTESIAN_POINT('Ctrl Pts',(5.56462753148356,3.85510152500977,40.4956763813569));
#193535=CARTESIAN_POINT('Ctrl Pts',(5.45651721693046,4.00665785831769,40.504425847067));
#193536=CARTESIAN_POINT('Ctrl Pts',(5.34234877395471,4.15350437310768,40.5131753127771));
#193537=CARTESIAN_POINT('Ctrl Pts',(5.22818382836054,4.30034638947163,40.5219245104603));
#193538=CARTESIAN_POINT('Ctrl Pts',(5.10796130160446,4.44247864979492,40.5306737081435));
#193539=CARTESIAN_POINT('Ctrl Pts',(4.98208950540816,4.5794184303361,40.5394229058267));
#193540=CARTESIAN_POINT('Ctrl Pts',(4.85622089618151,4.71635474367543,40.5481718819874));
#193541=CARTESIAN_POINT('Ctrl Pts',(4.72470349764587,4.84809862936311,40.5569208581481));
#193542=CARTESIAN_POINT('Ctrl Pts',(4.58798395969625,4.97420266832484,40.5656698343089));
#193543=CARTESIAN_POINT('Ctrl Pts',(4.45125553495138,5.10031490407241,40.5744193791547));
#193544=CARTESIAN_POINT('Ctrl Pts',(4.30932450476746,5.2207863651704,40.5831689240005));
#193545=CARTESIAN_POINT('Ctrl Pts',(4.16267294766396,5.33520786200375,40.5919184688463));
#193546=CARTESIAN_POINT('Ctrl Pts',(4.01603001077209,5.44962263311569,40.6006674993919));
#193547=CARTESIAN_POINT('Ctrl Pts',(3.86466732812914,5.55798797530905,40.6094165299374));
#193548=CARTESIAN_POINT('Ctrl Pts',(3.70909895313569,5.6599358614606,40.618165560483));
#193549=CARTESIAN_POINT('Ctrl Pts',(3.55352846818182,5.76188513032251,40.626914709691));
#193550=CARTESIAN_POINT('Ctrl Pts',(3.39375241639409,5.85741661190576,40.6356638588989));
#193551=CARTESIAN_POINT('Ctrl Pts',(3.23031343910922,5.94620585626754,40.6444130081068));
#193552=CARTESIAN_POINT('Ctrl Pts',(3.18683327726978,5.96982672552765,40.6467405705392));
#193553=CARTESIAN_POINT('Ctrl Pts',(3.14309402254946,5.99297066865441,40.6490681329716));
#193554=CARTESIAN_POINT('Ctrl Pts',(3.09910619832134,6.0156321173694,40.651395695404));
#193555=CARTESIAN_POINT('Origin',(0.,0.,4.30282021618968));
#193556=CARTESIAN_POINT('',(3.09910619832137,6.01563211736938,43.0457451347211));
#193557=CARTESIAN_POINT('',(3.09910619832134,6.0156321173694,42.651395695404));
#193558=CARTESIAN_POINT('',(3.09910619832133,6.0156321173694,4.30282021618968));
#193559=CARTESIAN_POINT('',(-6.76699752108395,0.00579220542896902,41.6971797838367));
#193560=CARTESIAN_POINT('Ctrl Pts',(-6.76699752108395,0.00579220542897352,
41.6971797838367));
#193561=CARTESIAN_POINT('Ctrl Pts',(-6.7671419157541,-0.162903188225639,
41.7051597747815));
#193562=CARTESIAN_POINT('Ctrl Pts',(-6.76097415360396,-0.331919362032048,
41.7131397657264));
#193563=CARTESIAN_POINT('Ctrl Pts',(-6.74844880523453,-0.500727194317024,
41.7211197566712));
#193564=CARTESIAN_POINT('Ctrl Pts',(-6.73593791874819,-0.669340119517491,
41.7290905338447));
#193565=CARTESIAN_POINT('Ctrl Pts',(-6.71708407476151,-0.837744806685119,
41.7370613110182));
#193566=CARTESIAN_POINT('Ctrl Pts',(-6.69189373650032,-1.00540898115535,
41.7450320881916));
#193567=CARTESIAN_POINT('Ctrl Pts',(-6.66672676650753,-1.1729176189516,
41.7529954711309));
#193568=CARTESIAN_POINT('Ctrl Pts',(-6.63523505233561,-1.3396867371706,
41.7609588540702));
#193569=CARTESIAN_POINT('Ctrl Pts',(-6.59747704608564,-1.50518624308525,
41.7689222370095));
#193570=CARTESIAN_POINT('Ctrl Pts',(-6.5597455214126,-1.67056967592472,
41.7768800348303));
#193571=CARTESIAN_POINT('Ctrl Pts',(-6.51575653367953,-1.83468489874086,
41.7848378326512));
#193572=CARTESIAN_POINT('Ctrl Pts',(-6.46562006098974,-1.99700932069108,
41.792795630472));
#193573=CARTESIAN_POINT('Ctrl Pts',(-6.41344117349947,-2.16594636981835,
41.8010776059459));
#193574=CARTESIAN_POINT('Ctrl Pts',(-6.35460345110363,-2.33294322299446,
41.8093595814197));
#193575=CARTESIAN_POINT('Ctrl Pts',(-6.28928922096292,-2.49742469257426,
41.8176415568936));
#193576=CARTESIAN_POINT('Ctrl Pts',(-6.22656637487845,-2.65538025414138,
41.825594939668));
#193577=CARTESIAN_POINT('Ctrl Pts',(-6.15787122358108,-2.81101581324948,
41.8335483224424));
#193578=CARTESIAN_POINT('Ctrl Pts',(-6.08341529326123,-2.96383997032825,
41.8415017052167));
#193579=CARTESIAN_POINT('Ctrl Pts',(-6.00895734476367,-3.11666826980785,
41.8494553035729));
#193580=CARTESIAN_POINT('Ctrl Pts',(-5.92873847287648,-3.26668467282175,
41.857408901929));
#193581=CARTESIAN_POINT('Ctrl Pts',(-5.84301703124469,-3.41342071426662,
41.8653625002851));
#193582=CARTESIAN_POINT('Ctrl Pts',(-5.75727574448061,-3.56019072616391,
41.8733179399567));
#193583=CARTESIAN_POINT('Ctrl Pts',(-5.66602954574324,-3.7036785367616,
41.8812733796282));
#193584=CARTESIAN_POINT('Ctrl Pts',(-5.56958099527458,-3.84344331779151,
41.8892288192998));
#193585=CARTESIAN_POINT('Ctrl Pts',(-5.47309038661119,-3.98326904586883,
41.8971877280896));
#193586=CARTESIAN_POINT('Ctrl Pts',(-5.37139312906561,-4.11936820155264,
41.9051466368794));
#193587=CARTESIAN_POINT('Ctrl Pts',(-5.26483288548004,-4.25133198985541,
41.9131055456693));
#193588=CARTESIAN_POINT('Ctrl Pts',(-5.15814568872913,-4.38345299646091,
41.9210739365007));
#193589=CARTESIAN_POINT('Ctrl Pts',(-5.04658418186476,-4.51142850673486,
41.9290423273321));
#193590=CARTESIAN_POINT('Ctrl Pts',(-4.93053021868755,-4.63488519411311,
41.9370107181636));
#193591=CARTESIAN_POINT('Ctrl Pts',(-4.81439468646419,-4.75842865357526,
41.9449847096141));
#193592=CARTESIAN_POINT('Ctrl Pts',(-4.6937606833546,-4.87744670354447,
41.9529587010646));
#193593=CARTESIAN_POINT('Ctrl Pts',(-4.5690435503665,-4.99160595749046,
41.9609326925151));
#193594=CARTESIAN_POINT('Ctrl Pts',(-4.44414673822428,-5.10592967992361,
41.9689181720427));
#193595=CARTESIAN_POINT('Ctrl Pts',(-4.31515534748906,-5.21538039602099,
41.9769036515704));
#193596=CARTESIAN_POINT('Ctrl Pts',(-4.18251456892623,-5.31966736560848,
41.984889131098));
#193597=CARTESIAN_POINT('Ctrl Pts',(-4.14556280272493,-5.34872017847487,
41.9871137680136));
#193598=CARTESIAN_POINT('Ctrl Pts',(-4.10832795919166,-5.3773725065816,
41.9893384049292));
#193599=CARTESIAN_POINT('Ctrl Pts',(-4.07081999675313,-5.40561870224259,
41.9915630418449));
#193600=CARTESIAN_POINT('Ctrl Pts',(-3.93032474337721,-5.51142174133862,
41.9998959638916));
#193601=CARTESIAN_POINT('Ctrl Pts',(-3.78552165961881,-5.61187987212897,
42.0082288859383));
#193602=CARTESIAN_POINT('Ctrl Pts',(-3.63684920453656,-5.70662920325667,
42.016561807985));
#193603=CARTESIAN_POINT('Ctrl Pts',(-3.48835244424243,-5.80126656365214,
42.0248848825387));
#193604=CARTESIAN_POINT('Ctrl Pts',(-3.33599571263826,-5.89020837836998,
42.0332079570923));
#193605=CARTESIAN_POINT('Ctrl Pts',(-3.18024955516211,-5.97313165491028,
42.0415310316459));
#193606=CARTESIAN_POINT('Ctrl Pts',(-3.02465886377403,-6.05597215729022,
42.0498457980919));
#193607=CARTESIAN_POINT('Ctrl Pts',(-2.86568579241507,-6.13280592828548,
42.0581605645379));
#193608=CARTESIAN_POINT('Ctrl Pts',(-2.70382900372628,-6.20335374766009,
42.0664753309839));
#193609=CARTESIAN_POINT('Ctrl Pts',(-2.54210409078569,-6.27384408692196,
42.0747833228234));
#193610=CARTESIAN_POINT('Ctrl Pts',(-2.37750045979973,-6.33805854133451,
42.083091314663));
#193611=CARTESIAN_POINT('Ctrl Pts',(-2.21054066438813,-6.39576414285944,
42.0913993065025));
#193612=CARTESIAN_POINT('Ctrl Pts',(-2.04368629314711,-6.45343330707822,
42.0997020523896));
#193613=CARTESIAN_POINT('Ctrl Pts',(-1.87447905034718,-6.50460169563769,
42.1080047982766));
#193614=CARTESIAN_POINT('Ctrl Pts',(-1.70346093646292,-6.54908465649551,
42.1163075441637));
#193615=CARTESIAN_POINT('Ctrl Pts',(-1.53251271223167,-6.59354943858484,
42.1246068969831));
#193616=CARTESIAN_POINT('Ctrl Pts',(-1.35975542770278,-6.63133414948042,
42.1329062498026));
#193617=CARTESIAN_POINT('Ctrl Pts',(-1.18574597554647,-6.66230406702331,
42.141205602622));
#193618=CARTESIAN_POINT('Ctrl Pts',(-1.01177353228092,-6.69326739778439,
42.1495031903083));
#193619=CARTESIAN_POINT('Ctrl Pts',(-0.836549794271697,-6.71741876178281,
42.1578007779947));
#193620=CARTESIAN_POINT('Ctrl Pts',(-0.66064181556716,-6.73467455720944,
42.166098365681));
#193621=CARTESIAN_POINT('Ctrl Pts',(-0.484742017984839,-6.75192955010413,
42.1743955674634));
#193622=CARTESIAN_POINT('Ctrl Pts',(-0.308158389356044,-6.76228957969436,
42.1826927692459));
#193623=CARTESIAN_POINT('Ctrl Pts',(-0.131463270973249,-6.76572290360646,
42.1909899710283));
#193624=CARTESIAN_POINT('Ctrl Pts',(0.0452529907255948,-6.76915663834968,
42.1992881656528));
#193625=CARTESIAN_POINT('Ctrl Pts',(0.222080420934282,-6.76566200967775,
42.2075863602774));
#193626=CARTESIAN_POINT('Ctrl Pts',(0.398446313981372,-6.75525939804495,
42.2158845549019));
#193627=CARTESIAN_POINT('Ctrl Pts',(0.5749362472169,-6.74484947013414,42.2241885857435));
#193628=CARTESIAN_POINT('Ctrl Pts',(0.750963646941569,-6.72752187160386,
42.2324926165851));
#193629=CARTESIAN_POINT('Ctrl Pts',(0.92595965786807,-6.70334899225759,
42.2407966474267));
#193630=CARTESIAN_POINT('Ctrl Pts',(1.10101930216068,-6.67916732298706,
42.2491036978424));
#193631=CARTESIAN_POINT('Ctrl Pts',(1.27504646657759,-6.64813546666324,
42.2574107482581));
#193632=CARTESIAN_POINT('Ctrl Pts',(1.44748190173852,-6.61037708032904,
42.2657177986739));
#193633=CARTESIAN_POINT('Ctrl Pts',(1.62010169948183,-6.5725783239073,42.2740337307285));
#193634=CARTESIAN_POINT('Ctrl Pts',(1.79112602924616,-6.52803874986931,
42.2823496627831));
#193635=CARTESIAN_POINT('Ctrl Pts',(1.96000915956826,-6.47693238303509,
42.2906655948378));
#193636=CARTESIAN_POINT('Ctrl Pts',(2.08731685039777,-6.4384073181814,42.2969343210566));
#193637=CARTESIAN_POINT('Ctrl Pts',(2.21340809606874,-6.39615173772712,
42.3032030472755));
#193638=CARTESIAN_POINT('Ctrl Pts',(2.33805657735998,-6.35025829719262,
42.3094717734943));
#193639=CARTESIAN_POINT('Ctrl Pts',(2.50608324276164,-6.2883937506138,42.3179220422176));
#193640=CARTESIAN_POINT('Ctrl Pts',(2.67179565761498,-6.21980369679273,
42.326372310941));
#193641=CARTESIAN_POINT('Ctrl Pts',(2.83463840281996,-6.14468177575197,
42.3348225796643));
#193642=CARTESIAN_POINT('Ctrl Pts',(2.99733743377775,-6.06962615235508,
42.3432653907389));
#193643=CARTESIAN_POINT('Ctrl Pts',(3.15717154329149,-5.98805028986467,
42.3517082018134));
#193644=CARTESIAN_POINT('Ctrl Pts',(3.31360401903543,-5.90019638698851,
42.3601510128879));
#193645=CARTESIAN_POINT('Ctrl Pts',(3.46991973649539,-5.81240805662785,
42.3685875224056));
#193646=CARTESIAN_POINT('Ctrl Pts',(3.6228385932091,-5.71835118861923,42.3770240319233));
#193647=CARTESIAN_POINT('Ctrl Pts',(3.7718469286948,-5.61831467136681,42.385460541441));
#193648=CARTESIAN_POINT('Ctrl Pts',(3.92074864069892,-5.51834973562506,
42.3938910141822));
#193649=CARTESIAN_POINT('Ctrl Pts',(4.06574513828252,-5.41241386968859,
42.4023214869235));
#193650=CARTESIAN_POINT('Ctrl Pts',(4.20635011855401,-5.30084028057257,
42.4107519596647));
#193651=CARTESIAN_POINT('Ctrl Pts',(4.34689465312561,-5.18931465664007,
42.4191788081685));
#193652=CARTESIAN_POINT('Ctrl Pts',(4.48305117471774,-5.07215634687458,
42.4276056566723));
#193653=CARTESIAN_POINT('Ctrl Pts',(4.61436443864262,-4.94974037979674,
42.4360325051761));
#193654=CARTESIAN_POINT('Ctrl Pts',(4.74563717085251,-4.8273621981561,42.4444567526128));
#193655=CARTESIAN_POINT('Ctrl Pts',(4.87206938440724,-4.69972982139218,
42.4528810000495));
#193656=CARTESIAN_POINT('Ctrl Pts',(4.99324058506915,-4.56725710461086,
42.4613052474861));
#193657=CARTESIAN_POINT('Ctrl Pts',(5.0273819933344,-4.52993136150579,42.4636788780971));
#193658=CARTESIAN_POINT('Ctrl Pts',(5.06110595313962,-4.49222157277779,
42.4660525087081));
#193659=CARTESIAN_POINT('Ctrl Pts',(5.09440359174525,-4.45413751970156,
42.4684261393191));
#193660=CARTESIAN_POINT('Ctrl Pts',(5.21530911577234,-4.3158522662398,42.4770449202563));
#193661=CARTESIAN_POINT('Ctrl Pts',(5.33053669471643,-4.17269176633671,
42.4856637011936));
#193662=CARTESIAN_POINT('Ctrl Pts',(5.43971335764167,-4.02514690249869,
42.4942824821308));
#193663=CARTESIAN_POINT('Ctrl Pts',(5.54895560232493,-3.8775134093575,42.5029064403173));
#193664=CARTESIAN_POINT('Ctrl Pts',(5.65213949620672,-3.72549054080655,
42.5115303985039));
#193665=CARTESIAN_POINT('Ctrl Pts',(5.74893505733717,-3.56959867583454,
42.5201543566905));
#193666=CARTESIAN_POINT('Ctrl Pts',(5.84922751182715,-3.40807496968036,
42.5290898690616));
#193667=CARTESIAN_POINT('Ctrl Pts',(5.94266126508607,-3.24239781794299,
42.5380253814327));
#193668=CARTESIAN_POINT('Ctrl Pts',(6.02892123533005,-3.07317388674744,
42.5469608938038));
#193669=CARTESIAN_POINT('Ctrl Pts',(6.11232923435509,-2.90954492364616,
42.5556009756985));
#193670=CARTESIAN_POINT('Ctrl Pts',(6.1890301394651,-2.74260025437282,42.5642410575931));
#193671=CARTESIAN_POINT('Ctrl Pts',(6.25878801113481,-2.57290917672489,
42.5728811394877));
#193672=CARTESIAN_POINT('Ctrl Pts',(6.33212373105573,-2.39451472394703,
42.5819643670971));
#193673=CARTESIAN_POINT('Ctrl Pts',(6.39778536647262,-2.21308510877036,
42.5910475947064));
#193674=CARTESIAN_POINT('Ctrl Pts',(6.45555782815182,-2.02930089621716,
42.6001308223158));
#193675=CARTESIAN_POINT('Ctrl Pts',(6.51333028983101,-1.84551668366399,
42.6092140499251));
#193676=CARTESIAN_POINT('Ctrl Pts',(6.56321350990222,-1.65937825700491,
42.6182972775345));
#193677=CARTESIAN_POINT('Ctrl Pts',(6.60505419342663,-1.47158013777615,
42.6273805051438));
#193678=CARTESIAN_POINT('Ctrl Pts',(6.64671692031331,-1.2845807608015,42.6364251000036));
#193679=CARTESIAN_POINT('Ctrl Pts',(6.68044470798201,-1.09576328069521,
42.6454696948635));
#193680=CARTESIAN_POINT('Ctrl Pts',(6.70610468636559,-0.905786363059985,
42.6545142897234));
#193681=CARTESIAN_POINT('Ctrl Pts',(6.73174111768006,-0.715983779149547,
42.6635505847438));
#193682=CARTESIAN_POINT('Ctrl Pts',(6.74932448898829,-0.525024117474134,
42.6725868797642));
#193683=CARTESIAN_POINT('Ctrl Pts',(6.75877335798435,-0.333574122798727,
42.6816231747846));
#193684=CARTESIAN_POINT('Ctrl Pts',(6.76820550646572,-0.142462913902861,
42.6906434793724));
#193685=CARTESIAN_POINT('Ctrl Pts',(6.769531885184,0.0491366580460953,42.6996637839601));
#193686=CARTESIAN_POINT('Ctrl Pts',(6.76272299267066,0.240555034043397,
42.7086840885478));
#193687=CARTESIAN_POINT('Ctrl Pts',(6.75592267463481,0.431732355779322,
42.7176930338142));
#193688=CARTESIAN_POINT('Ctrl Pts',(6.74100753888465,0.622728699902162,
42.7267019790805));
#193689=CARTESIAN_POINT('Ctrl Pts',(6.71800003456061,0.812874243437263,
42.7357109243468));
#193690=CARTESIAN_POINT('Ctrl Pts',(6.69504477540808,1.00258800669779,42.7446994122056));
#193691=CARTESIAN_POINT('Ctrl Pts',(6.66403385639883,1.19145459005036,42.7536879000645));
#193692=CARTESIAN_POINT('Ctrl Pts',(6.62504138342984,1.37880951107905,42.7626763879233));
#193693=CARTESIAN_POINT('Ctrl Pts',(6.59083085491407,1.54318766871784,42.7705625489384));
#193694=CARTESIAN_POINT('Ctrl Pts',(6.5504771695524,1.70640211062867,42.7784487099534));
#193695=CARTESIAN_POINT('Ctrl Pts',(6.50406332209127,1.86800677253244,42.7863348709685));
#193696=CARTESIAN_POINT('Ctrl Pts',(6.45626459844424,2.03443332402401,42.7944563358247));
#193697=CARTESIAN_POINT('Ctrl Pts',(6.40205850140957,2.19907764734956,42.8025778006808));
#193698=CARTESIAN_POINT('Ctrl Pts',(6.3416102525954,2.36141237486741,42.810699265537));
#193699=CARTESIAN_POINT('Ctrl Pts',(6.28116631463095,2.5237355255302,42.8188201512132));
#193700=CARTESIAN_POINT('Ctrl Pts',(6.21448123936187,2.68374906529327,42.8269410368894));
#193701=CARTESIAN_POINT('Ctrl Pts',(6.14176922178484,2.84094347468169,42.8350619225656));
#193702=CARTESIAN_POINT('Ctrl Pts',(6.06904851304248,2.99815667329708,42.8431837789199));
#193703=CARTESIAN_POINT('Ctrl Pts',(5.99029958234779,3.15254973871702,42.8513056352741));
#193704=CARTESIAN_POINT('Ctrl Pts',(5.90578358336553,3.30363576479767,42.8594274916284));
#193705=CARTESIAN_POINT('Ctrl Pts',(5.82120592255594,3.45483202137389,42.8675552735886));
#193706=CARTESIAN_POINT('Ctrl Pts',(5.73085296872741,3.60271609973036,42.8756830555488));
#193707=CARTESIAN_POINT('Ctrl Pts',(5.63503073783105,3.74682766933565,42.8838108375089));
#193708=CARTESIAN_POINT('Ctrl Pts',(5.53916947251942,3.89099794463796,42.8919419304254));
#193709=CARTESIAN_POINT('Ctrl Pts',(5.43783470331295,4.03139235124276,42.9000730233418));
#193710=CARTESIAN_POINT('Ctrl Pts',(5.33137394546845,4.16758213519304,42.9082041162583));
#193711=CARTESIAN_POINT('Ctrl Pts',(5.22479699015606,4.30392056460075,42.9163440839229));
#193712=CARTESIAN_POINT('Ctrl Pts',(5.11308310766669,4.43604492596168,42.9244840515874));
#193713=CARTESIAN_POINT('Ctrl Pts',(4.99661850493419,4.56356138516283,42.932624019252));
#193714=CARTESIAN_POINT('Ctrl Pts',(4.93621492634999,4.62969693436335,42.9368457584325));
#193715=CARTESIAN_POINT('Ctrl Pts',(4.87453403930079,4.69459361999119,42.941067497613));
#193716=CARTESIAN_POINT('Ctrl Pts',(4.81163332987714,4.7582006787036,42.9452892367935));
#193717=CARTESIAN_POINT('Ctrl Pts',(4.68589120127583,4.88535484007718,42.9537287357407));
#193718=CARTESIAN_POINT('Ctrl Pts',(4.55501247853667,5.00761580790413,42.9621682346878));
#193719=CARTESIAN_POINT('Ctrl Pts',(4.4194057018988,5.12456263909657,42.970607733635));
#193720=CARTESIAN_POINT('Ctrl Pts',(4.28389115220958,5.24142993407657,42.9790414928304));
#193721=CARTESIAN_POINT('Ctrl Pts',(4.14365520789653,5.35299007747284,42.9874752520258));
#193722=CARTESIAN_POINT('Ctrl Pts',(3.99914256677247,5.45885956318978,42.9959090112212));
#193723=CARTESIAN_POINT('Ctrl Pts',(3.85472117236771,5.56466220186019,43.0043374452571));
#193724=CARTESIAN_POINT('Ctrl Pts',(3.70602873374957,5.66478115071055,43.0127658792931));
#193725=CARTESIAN_POINT('Ctrl Pts',(3.55354243465342,5.7588736021133,43.021194313329));
#193726=CARTESIAN_POINT('Ctrl Pts',(3.40548551692778,5.8502328810683,43.0293779204597));
#193727=CARTESIAN_POINT('Ctrl Pts',(3.25385232116557,5.93591070836102,43.0375615275904));
#193728=CARTESIAN_POINT('Ctrl Pts',(3.09910619832137,6.01563211736938,43.0457451347211));
#193729=CARTESIAN_POINT('Ctrl Pts',(3.09910619832129,6.01563211736942,41.0459058825584));
#193730=CARTESIAN_POINT('Ctrl Pts',(2.94406710095791,6.09550445966803,41.054142267447));
#193731=CARTESIAN_POINT('Ctrl Pts',(2.78573418535561,6.16948443241409,41.0623786523356));
#193732=CARTESIAN_POINT('Ctrl Pts',(2.62459330575604,6.23729099684956,41.0706150372242));
#193733=CARTESIAN_POINT('Ctrl Pts',(2.4636219004224,6.30502624811012,41.0788427597841));
#193734=CARTESIAN_POINT('Ctrl Pts',(2.29984873717746,6.3666008827864,41.0870704823439));
#193735=CARTESIAN_POINT('Ctrl Pts',(2.13378450708244,6.42177955689348,41.0952982049037));
#193736=CARTESIAN_POINT('Ctrl Pts',(1.96307750522898,6.47850089909751,41.1037559555552));
#193737=CARTESIAN_POINT('Ctrl Pts',(1.78994978312948,6.52846323509716,41.1122137062066));
#193738=CARTESIAN_POINT('Ctrl Pts',(1.61497995666406,6.57146321146009,41.1206714568581));
#193739=CARTESIAN_POINT('Ctrl Pts',(1.44505721225939,6.61322283447926,41.1288852399498));
#193740=CARTESIAN_POINT('Ctrl Pts',(1.27339753524235,6.6484160883722,41.1370990230415));
#193741=CARTESIAN_POINT('Ctrl Pts',(1.10054774648411,6.6769067432239,41.1453128061333));
#193742=CARTESIAN_POINT('Ctrl Pts',(0.919996925079205,6.70666675145296,
41.1538925405646));
#193743=CARTESIAN_POINT('Ctrl Pts',(0.738147891892085,6.72911308957362,
41.1624722749959));
#193744=CARTESIAN_POINT('Ctrl Pts',(0.555637124469811,6.74414978970003,
41.1710520094272));
#193745=CARTESIAN_POINT('Ctrl Pts',(0.373126357047538,6.75918648982644,
41.1796317438585));
#193746=CARTESIAN_POINT('Ctrl Pts',(0.189954295794854,6.76681349632012,
41.1882114782898));
#193747=CARTESIAN_POINT('Ctrl Pts',(0.00676451732140437,6.76699661898138,
41.1967912127211));
#193748=CARTESIAN_POINT('Ctrl Pts',(-0.182389569994082,6.76718570376627,
41.205650286897));
#193749=CARTESIAN_POINT('Ctrl Pts',(-0.371365666416525,6.75943933602207,
41.2145093610729));
#193750=CARTESIAN_POINT('Ctrl Pts',(-0.559514331608083,6.74382923217405,
41.2233684352488));
#193751=CARTESIAN_POINT('Ctrl Pts',(-0.74801649028807,6.72818980008147,
41.2322441538427));
#193752=CARTESIAN_POINT('Ctrl Pts',(-0.93568785266029,6.70465712757872,
41.2411198724367));
#193753=CARTESIAN_POINT('Ctrl Pts',(-1.12188692416418,6.67335438362069,
41.2499955910306));
#193754=CARTESIAN_POINT('Ctrl Pts',(-1.30861735520857,6.64196231047582,
41.2588966384176));
#193755=CARTESIAN_POINT('Ctrl Pts',(-1.49386683033995,6.60275583669487,
41.2677976858046));
#193756=CARTESIAN_POINT('Ctrl Pts',(-1.67700380448391,6.55590933736477,
41.2766987331917));
#193757=CARTESIAN_POINT('Ctrl Pts',(-1.86038975585627,6.50899914957624,
41.2856118816747));
#193758=CARTESIAN_POINT('Ctrl Pts',(-2.04165721980538,6.45442825866837,
41.2945250301577));
#193759=CARTESIAN_POINT('Ctrl Pts',(-2.22019121767212,6.39242050845934,
41.3034381786407));
#193760=CARTESIAN_POINT('Ctrl Pts',(-2.39912160983302,6.33027508408925,
41.3123711167506));
#193761=CARTESIAN_POINT('Ctrl Pts',(-2.57530615082169,6.26065985907395,
41.3213040548605));
#193762=CARTESIAN_POINT('Ctrl Pts',(-2.7481485286805,6.18384739982409,41.3302369929704));
#193763=CARTESIAN_POINT('Ctrl Pts',(-2.91266941129938,6.11073307596171,
41.3387398548289));
#193764=CARTESIAN_POINT('Ctrl Pts',(-3.0741622052832,6.0310983035465,41.3472427166873));
#193765=CARTESIAN_POINT('Ctrl Pts',(-3.23213456965948,5.94521615449027,
41.3557455785458));
#193766=CARTESIAN_POINT('Ctrl Pts',(-3.38490232624872,5.86216350604646,
41.3639683024117));
#193767=CARTESIAN_POINT('Ctrl Pts',(-3.53467012740325,5.77310830317956,
41.3721910262775));
#193768=CARTESIAN_POINT('Ctrl Pts',(-3.68093488888944,5.67829264337058,
41.3804137501434));
#193769=CARTESIAN_POINT('Ctrl Pts',(-3.82704483408053,5.5835773427255,41.3886277705346));
#193770=CARTESIAN_POINT('Ctrl Pts',(-3.96965882461234,5.48311392022527,
41.3968417909258));
#193771=CARTESIAN_POINT('Ctrl Pts',(-4.10829761703015,5.3771906875156,41.405055811317));
#193772=CARTESIAN_POINT('Ctrl Pts',(-4.24681749973279,5.2713583045689,41.413262786589));
#193773=CARTESIAN_POINT('Ctrl Pts',(-4.38136869121096,5.16007565425907,
41.421469761861));
#193774=CARTESIAN_POINT('Ctrl Pts',(-4.51150016803177,5.04367477478964,
41.4296767371329));
#193775=CARTESIAN_POINT('Ctrl Pts',(-4.64154615106915,4.92735036837518,
41.4378783205859));
#193776=CARTESIAN_POINT('Ctrl Pts',(-4.76717793678927,4.80591466894603,
41.4460799040389));
#193777=CARTESIAN_POINT('Ctrl Pts',(-4.88797683485411,4.67974053361184,
41.4542814874919));
#193778=CARTESIAN_POINT('Ctrl Pts',(-5.00872061156571,4.55362397238796,
41.462479328507));
#193779=CARTESIAN_POINT('Ctrl Pts',(-5.12463564651238,4.42277354143135,
41.470677169522));
#193780=CARTESIAN_POINT('Ctrl Pts',(-5.2353393890757,4.28759961764068,41.4788750105371));
#193781=CARTESIAN_POINT('Ctrl Pts',(-5.34603336237893,4.15243762252729,
41.4870721281182));
#193782=CARTESIAN_POINT('Ctrl Pts',(-5.4515167255638,4.01295316642926,41.4952692456993));
#193783=CARTESIAN_POINT('Ctrl Pts',(-5.55144636183972,3.86959071370818,
41.5034663632805));
#193784=CARTESIAN_POINT('Ctrl Pts',(-5.65137488628714,3.72622985605405,
41.5116633896596));
#193785=CARTESIAN_POINT('Ctrl Pts',(-5.74574960082674,3.57899138147709,
41.5198604160387));
#193786=CARTESIAN_POINT('Ctrl Pts',(-5.83427006732313,3.42834971692466,
41.5280574424177));
#193787=CARTESIAN_POINT('Ctrl Pts',(-5.92280564463728,3.27768233720341,
41.5362558680639));
#193788=CARTESIAN_POINT('Ctrl Pts',(-6.00548480111659,3.12361091948588,
41.54445429371));
#193789=CARTESIAN_POINT('Ctrl Pts',(-6.08205248542011,2.96663556315822,
41.5526527193561));
#193790=CARTESIAN_POINT('Ctrl Pts',(-6.15864716262927,2.80960486728333,
41.5608540352468));
#193791=CARTESIAN_POINT('Ctrl Pts',(-6.22912591862728,2.64966851580437,
41.5690553511374));
#193792=CARTESIAN_POINT('Ctrl Pts',(-6.29328135494752,2.48734774156529,
41.5772566670281));
#193793=CARTESIAN_POINT('Ctrl Pts',(-6.35750985357043,2.32484211113605,
41.5854673228447));
#193794=CARTESIAN_POINT('Ctrl Pts',(-6.4154005137618,2.15994696700335,41.5936779786613));
#193795=CARTESIAN_POINT('Ctrl Pts',(-6.46679511988317,1.993200912466,41.6018886344779));
#193796=CARTESIAN_POINT('Ctrl Pts',(-6.51822001160071,1.82635659851869,
41.610104128635));
#193797=CARTESIAN_POINT('Ctrl Pts',(-6.56314112660341,1.6576595462069,41.6183196227921));
#193798=CARTESIAN_POINT('Ctrl Pts',(-6.60145118222209,1.48765966831751,
41.6265351169493));
#193799=CARTESIAN_POINT('Ctrl Pts',(-6.63982067659705,1.31739603248923,
41.6347633575968));
#193800=CARTESIAN_POINT('Ctrl Pts',(-6.67155854847443,1.14582588422684,
41.6429915982443));
#193801=CARTESIAN_POINT('Ctrl Pts',(-6.69660911591914,0.97350672755184,
41.6512198388918));
#193802=CARTESIAN_POINT('Ctrl Pts',(-6.7193760823766,0.816896125071227,
41.658697995993));
#193803=CARTESIAN_POINT('Ctrl Pts',(-6.73662003573352,0.659667103896605,
41.6661761530942));
#193804=CARTESIAN_POINT('Ctrl Pts',(-6.74833653388256,0.502238016747035,
41.6736543101954));
#193805=CARTESIAN_POINT('Ctrl Pts',(-6.7606228126333,0.337153055046718,
41.6814961347336));
#193806=CARTESIAN_POINT('Ctrl Pts',(-6.76685562646407,0.171566789773337,
41.6893379592718));
#193807=CARTESIAN_POINT('Ctrl Pts',(-6.76699752108346,0.00579220599325065,
41.69717978381));
#193808=CARTESIAN_POINT('',(-6.767,9.39225326770929E-10,41.3028202161458));
#193809=CARTESIAN_POINT('Ctrl Pts',(3.09910619832134,6.0156321173694,40.651395695404));
#193810=CARTESIAN_POINT('Ctrl Pts',(2.93375330764826,6.10081787314653,40.6601451433063));
#193811=CARTESIAN_POINT('Ctrl Pts',(2.7648862784307,6.17918207037039,40.6688945912086));
#193812=CARTESIAN_POINT('Ctrl Pts',(2.59307866646702,6.25045854553997,40.6776440391109));
#193813=CARTESIAN_POINT('Ctrl Pts',(2.4212724418538,6.32173444515035,40.6863934163612));
#193814=CARTESIAN_POINT('Ctrl Pts',(2.24652594672472,6.38592262741835,40.6951427936115));
#193815=CARTESIAN_POINT('Ctrl Pts',(2.06943269687133,6.44280508110558,40.7038921708618));
#193816=CARTESIAN_POINT('Ctrl Pts',(1.89234081822086,6.49968709436164,40.7126414803672));
#193817=CARTESIAN_POINT('Ctrl Pts',(1.71290249405596,6.54926340459543,40.7213907898725));
#193818=CARTESIAN_POINT('Ctrl Pts',(1.53172716625063,6.59136563150382,40.7301400993779));
#193819=CARTESIAN_POINT('Ctrl Pts',(1.35055318107334,6.6334675464071,40.7388893440451));
#193820=CARTESIAN_POINT('Ctrl Pts',(1.16764249714415,6.66809542395777,40.7476385887124));
#193821=CARTESIAN_POINT('Ctrl Pts',(0.983616340614261,6.6951316562467,40.7563878333796));
#193822=CARTESIAN_POINT('Ctrl Pts',(0.79959148671378,6.72216769715962,40.7651370161153));
#193823=CARTESIAN_POINT('Ctrl Pts',(0.614451459526685,6.74161215869371,
40.773886198851));
#193824=CARTESIAN_POINT('Ctrl Pts',(0.428825047910289,6.75339900185712,
40.7826353815867));
#193825=CARTESIAN_POINT('Ctrl Pts',(0.24319988859693,6.76518576550222,40.7913845052972));
#193826=CARTESIAN_POINT('Ctrl Pts',(0.0570886373916788,6.76931499599835,
40.8001336290078));
#193827=CARTESIAN_POINT('Ctrl Pts',(-0.12887662681151,6.76577266947846,
40.8088827527183));
#193828=CARTESIAN_POINT('Ctrl Pts',(-0.314840698188363,6.76223036567992,
40.8176318203098));
#193829=CARTESIAN_POINT('Ctrl Pts',(-0.500658497951302,6.75101660879222,
40.8263808879014));
#193830=CARTESIAN_POINT('Ctrl Pts',(-0.685698951926112,6.73216948296219,
40.8351299554929));
#193831=CARTESIAN_POINT('Ctrl Pts',(-0.870738280459781,6.71332247176294,
40.8438789698714));
#193832=CARTESIAN_POINT('Ctrl Pts',(-1.05499998761247,6.68684221356187,
40.85262798425));
#193833=CARTESIAN_POINT('Ctrl Pts',(-1.2378582916142,6.65281863948522,40.8613769986285));
#193834=CARTESIAN_POINT('Ctrl Pts',(-1.4300741291548,6.61705395369219,40.8705737323268));
#193835=CARTESIAN_POINT('Ctrl Pts',(-1.62073882531976,6.57295372728672,
40.879770466025));
#193836=CARTESIAN_POINT('Ctrl Pts',(-1.80913696085859,6.52068343479848,
40.8889671997233));
#193837=CARTESIAN_POINT('Ctrl Pts',(-1.98838356180497,6.47095219816924,
40.897717197437));
#193838=CARTESIAN_POINT('Ctrl Pts',(-2.16557827566964,6.41382586852771,
40.9064671951507));
#193839=CARTESIAN_POINT('Ctrl Pts',(-2.34011918616184,6.34949849945311,
40.9152171928643));
#193840=CARTESIAN_POINT('Ctrl Pts',(-2.51465655685641,6.28517243497734,
40.9239670131226));
#193841=CARTESIAN_POINT('Ctrl Pts',(-2.68653996289935,6.21364572244706,
40.9327168333809));
#193842=CARTESIAN_POINT('Ctrl Pts',(-2.85518555374665,6.13516132254698,
40.9414666536392));
#193843=CARTESIAN_POINT('Ctrl Pts',(-3.02382794853427,6.05667841003134,
40.9502163080767));
#193844=CARTESIAN_POINT('Ctrl Pts',(-3.18923239104086,5.97123819494855,
40.9589659625142));
#193845=CARTESIAN_POINT('Ctrl Pts',(-3.35083705962576,5.87913088813632,
40.9677156169518));
#193846=CARTESIAN_POINT('Ctrl Pts',(-3.51243888037353,5.78702520446166,
40.9764651172007));
#193847=CARTESIAN_POINT('Ctrl Pts',(-3.67024081218725,5.68825280608986,
40.9852146174496));
#193848=CARTESIAN_POINT('Ctrl Pts',(-3.82370687539524,5.58314917685845,
40.9939641176986));
#193849=CARTESIAN_POINT('Ctrl Pts',(-3.97717043813042,5.47804726011487,
41.0027134753891));
#193850=CARTESIAN_POINT('Ctrl Pts',(-4.12629803717796,5.36661448087823,
41.0114628330795));
#193851=CARTESIAN_POINT('Ctrl Pts',(-4.27058317202357,5.24922931208279,
41.02021219077));
#193852=CARTESIAN_POINT('Ctrl Pts',(-4.41486614770382,5.13184589990621,
41.0289614175301));
#193853=CARTESIAN_POINT('Ctrl Pts',(-4.55430658190064,5.00851045726989,
41.0377106442901));
#193854=CARTESIAN_POINT('Ctrl Pts',(-4.68843088997604,4.87964187107194,
41.0464598710502));
#193855=CARTESIAN_POINT('Ctrl Pts',(-4.82255336913684,4.75077504212174,
41.0552089785061));
#193856=CARTESIAN_POINT('Ctrl Pts',(-4.95135966061078,4.61637541912442,
41.063958085962));
#193857=CARTESIAN_POINT('Ctrl Pts',(-5.0744123086529,4.47689945406326,41.0727071934179));
#193858=CARTESIAN_POINT('Ctrl Pts',(-5.19746344222582,4.33742520560111,
41.0814561931943));
#193859=CARTESIAN_POINT('Ctrl Pts',(-5.31476088451055,4.19287495496041,
41.0902051929707));
#193860=CARTESIAN_POINT('Ctrl Pts',(-5.4259062762527,4.04373961591515,41.098954192747));
#193861=CARTESIAN_POINT('Ctrl Pts',(-5.53706380669211,3.89458798911648,
41.1077041480417));
#193862=CARTESIAN_POINT('Ctrl Pts',(-5.6420677706854,3.74085050160297,41.1164541033364));
#193863=CARTESIAN_POINT('Ctrl Pts',(-5.7405614816082,3.58304938228267,41.1252040586311));
#193864=CARTESIAN_POINT('Ctrl Pts',(-5.83905138948832,3.42525435598484,
41.1339536760722));
#193865=CARTESIAN_POINT('Ctrl Pts',(-5.9310313955474,3.26339625502476,41.1427032935133));
#193866=CARTESIAN_POINT('Ctrl Pts',(-6.01618907818077,3.09802485070382,
41.1514529109544));
#193867=CARTESIAN_POINT('Ctrl Pts',(-6.10134392542359,2.93265895255099,
41.1602022370703));
#193868=CARTESIAN_POINT('Ctrl Pts',(-6.17967677259356,2.76378023991569,
41.1689515631862));
#193869=CARTESIAN_POINT('Ctrl Pts',(-6.25092157006901,2.59196229232719,
41.177700889302));
#193870=CARTESIAN_POINT('Ctrl Pts',(-6.32216437405586,2.42014915234754,
41.1864499706045));
#193871=CARTESIAN_POINT('Ctrl Pts',(-6.38631941546912,2.24539720668566,
41.1951990519069));
#193872=CARTESIAN_POINT('Ctrl Pts',(-6.44316881035688,2.06829994953448,
41.2039481332094));
#193873=CARTESIAN_POINT('Ctrl Pts',(-6.50002334522881,1.89118668030262,
41.2126980055517));
#193874=CARTESIAN_POINT('Ctrl Pts',(-6.54957082409566,1.71172794813559,
41.2214478778941));
#193875=CARTESIAN_POINT('Ctrl Pts',(-6.59164294294715,1.53053334256234,
41.2301977502364));
#193876=CARTESIAN_POINT('Ctrl Pts',(-6.63371214080929,1.34935131699523,
41.2389470150913));
#193877=CARTESIAN_POINT('Ctrl Pts',(-6.6683069523865,1.16643393835711,41.2476962799462));
#193878=CARTESIAN_POINT('Ctrl Pts',(-6.69530988153113,0.982402458400636,
41.2564455448012));
#193879=CARTESIAN_POINT('Ctrl Pts',(-6.72231419689771,0.798361531006992,
41.2651952588082));
#193880=CARTESIAN_POINT('Ctrl Pts',(-6.74172580828731,0.613206671422632,
41.2739449728152));
#193881=CARTESIAN_POINT('Ctrl Pts',(-6.75347878027798,0.427566795173706,
41.2826946868222));
#193882=CARTESIAN_POINT('Ctrl Pts',(-6.76248992366113,0.28523449455753,
41.2894031965967));
#193883=CARTESIAN_POINT('Ctrl Pts',(-6.76699999998021,0.142617266737464,
41.2961117063712));
#193884=CARTESIAN_POINT('Ctrl Pts',(-6.767,9.39226155489418E-10,41.3028202161458));
#193885=CARTESIAN_POINT('Ctrl Pts',(-6.767,5.59359546727568E-13,41.3028202161899));
#193886=CARTESIAN_POINT('Ctrl Pts',(-6.76700000000002,-0.186007249526374,
41.3115697280011));
#193887=CARTESIAN_POINT('Ctrl Pts',(-6.75932637294523,-0.372014355749482,
41.3203192398123));
#193888=CARTESIAN_POINT('Ctrl Pts',(-6.74400518264183,-0.557389537487119,
41.3290687516235));
#193889=CARTESIAN_POINT('Ctrl Pts',(-6.72868405705088,-0.742763936251683,
41.3378182264791));
#193890=CARTESIAN_POINT('Ctrl Pts',(-6.70571545645723,-0.927506130242415,
41.3465677013348));
#193891=CARTESIAN_POINT('Ctrl Pts',(-6.67517739404794,-1.11098863990201,
41.3553171761905));
#193892=CARTESIAN_POINT('Ctrl Pts',(-6.64463945808663,-1.29447038982145,
41.3640666148175));
#193893=CARTESIAN_POINT('Ctrl Pts',(-6.60653217008308,-1.47669218313894,
41.3728160534445));
#193894=CARTESIAN_POINT('Ctrl Pts',(-6.56098496092621,-1.65703510599509,
41.3815654920716));
#193895=CARTESIAN_POINT('Ctrl Pts',(-6.51543793658235,-1.8373772970892,
41.3903148951967));
#193896=CARTESIAN_POINT('Ctrl Pts',(-6.46245112167353,-2.01584035511143,
41.3990642983219));
#193897=CARTESIAN_POINT('Ctrl Pts',(-6.4022044837418,-2.19181813761005,
41.4078137014471));
#193898=CARTESIAN_POINT('Ctrl Pts',(-6.34195808526423,-2.36779522067361,
41.4165630697972));
#193899=CARTESIAN_POINT('Ctrl Pts',(-6.27445201433015,-2.54128677684386,
41.4253124381473));
#193900=CARTESIAN_POINT('Ctrl Pts',(-6.19991555071804,-2.71170355385035,
41.4340618064974));
#193901=CARTESIAN_POINT('Ctrl Pts',(-6.12537937716586,-2.88211966767704,
41.4428111407991));
#193902=CARTESIAN_POINT('Ctrl Pts',(-6.04381298052405,-3.04946076372014,
41.4515604751009));
#193903=CARTESIAN_POINT('Ctrl Pts',(-5.95549339335707,-3.21315848374777,
41.4603098094027));
#193904=CARTESIAN_POINT('Ctrl Pts',(-5.86717414255276,-3.37685558033724,
41.4690591103829));
#193905=CARTESIAN_POINT('Ctrl Pts',(-5.77210188876456,-3.53690907646989,
41.4778084113631));
#193906=CARTESIAN_POINT('Ctrl Pts',(-5.67059953346844,-3.6927753696952,
41.4865577123433));
#193907=CARTESIAN_POINT('Ctrl Pts',(-5.56909755631226,-3.84864108225152,
41.4953069807286));
#193908=CARTESIAN_POINT('Ctrl Pts',(-5.46116568196686,-4.00031938297741,
41.5040562491138));
#193909=CARTESIAN_POINT('Ctrl Pts',(-5.34717048533433,-4.14729511860074,
41.5128055174991));
#193910=CARTESIAN_POINT('Ctrl Pts',(-5.2331757039167,-4.29427031888118,
41.5215547540162));
#193911=CARTESIAN_POINT('Ctrl Pts',(-5.11311782003353,-4.43654276189732,
41.5303039905332));
#193912=CARTESIAN_POINT('Ctrl Pts',(-4.98740458984599,-4.5736292435202,
41.5390532270502));
#193913=CARTESIAN_POINT('Ctrl Pts',(-4.86169180711571,-4.71071523720445,
41.5478024324257));
#193914=CARTESIAN_POINT('Ctrl Pts',(-4.7303239120398,-4.84261509523426,
41.5565516378011));
#193915=CARTESIAN_POINT('Ctrl Pts',(-4.59374707013388,-4.96888084538525,
41.5653008431766));
#193916=CARTESIAN_POINT('Ctrl Pts',(-4.45717070301225,-5.09514615659657,
41.574050018137));
#193917=CARTESIAN_POINT('Ctrl Pts',(-4.31538563570812,-5.21577720459717,
41.5827991930975));
#193918=CARTESIAN_POINT('Ctrl Pts',(-4.16887341029271,-5.33036429233073,
41.5915483680579));
#193919=CARTESIAN_POINT('Ctrl Pts',(-4.02236168203444,-5.4449509912381,
41.6002975133299));
#193920=CARTESIAN_POINT('Ctrl Pts',(-3.87112305347878,-5.55349359438802,
41.609046658602));
#193921=CARTESIAN_POINT('Ctrl Pts',(-3.71567117017448,-5.65562346299099,
41.617795803874));
#193922=CARTESIAN_POINT('Ctrl Pts',(-3.56021980145488,-5.75775299351849,
41.6265449201842));
#193923=CARTESIAN_POINT('Ctrl Pts',(-3.40055544538,-5.85346967464076,41.6352940364944));
#193924=CARTESIAN_POINT('Ctrl Pts',(-3.23722035986486,-5.94244842987101,
41.6440431528045));
#193925=CARTESIAN_POINT('Ctrl Pts',(-3.07388580146793,-6.03142689794727,
41.6527922408794));
#193926=CARTESIAN_POINT('Ctrl Pts',(-2.9068807889617,-6.11366734656976,
41.6615413289542));
#193927=CARTESIAN_POINT('Ctrl Pts',(-2.73677250720942,-6.18889046952543,
41.6702904170291));
#193928=CARTESIAN_POINT('Ctrl Pts',(-2.56666476031041,-6.26411335596508,
41.6790394775951));
#193929=CARTESIAN_POINT('Ctrl Pts',(-2.39345402574712,-6.33231884500728,
41.6877885381612));
#193930=CARTESIAN_POINT('Ctrl Pts',(-2.21772856065125,-6.39327529762889,
41.6965375987272));
#193931=CARTESIAN_POINT('Ctrl Pts',(-2.04200363348049,-6.45423156365258,
41.7052866325109));
#193932=CARTESIAN_POINT('Ctrl Pts',(-1.86376426188818,-6.5079387437579,
41.7140356662946));
#193933=CARTESIAN_POINT('Ctrl Pts',(-1.68361577752698,-6.55421443909659,
41.7227847000783));
#193934=CARTESIAN_POINT('Ctrl Pts',(-1.50346782967368,-6.60048999661966,
41.7315337078061));
#193935=CARTESIAN_POINT('Ctrl Pts',(-1.32141105794581,-6.63933404237792,
41.7402827155339));
#193936=CARTESIAN_POINT('Ctrl Pts',(-1.13806375486643,-6.67061465607626,
41.7490317232617));
#193937=CARTESIAN_POINT('Ctrl Pts',(-0.95471698259936,-6.70189517921348,
41.7577807056601));
#193938=CARTESIAN_POINT('Ctrl Pts',(-0.770079968898631,-6.72561226592268,
41.7665296880585));
#193939=CARTESIAN_POINT('Ctrl Pts',(-0.58477976555489,-6.74168536983132,
41.7752786704569));
#193940=CARTESIAN_POINT('Ctrl Pts',(-0.391489830647991,-6.75845151013872,
41.7844048894668));
#193941=CARTESIAN_POINT('Ctrl Pts',(-0.19747857823508,-6.76689983031635,
41.7935311084766));
#193942=CARTESIAN_POINT('Ctrl Pts',(-0.00346287644814537,-6.76699911397118,
41.8026573274865));
#193943=CARTESIAN_POINT('Ctrl Pts',(0.184489834657946,-6.7670952950118,
41.8114983521523));
#193944=CARTESIAN_POINT('Ctrl Pts',(0.37244640425339,-6.75935639738146,
41.8203393768181));
#193945=CARTESIAN_POINT('Ctrl Pts',(0.559755019492312,-6.74380925873153,
41.8291804014839));
#193946=CARTESIAN_POINT('Ctrl Pts',(0.74513470552573,-6.72842222659762,
41.8379303800937));
#193947=CARTESIAN_POINT('Ctrl Pts',(0.929879431232497,-6.70538706057469,
41.8466803587034));
#193948=CARTESIAN_POINT('Ctrl Pts',(1.11336163627216,-6.67478200894062,
41.8554303373131));
#193949=CARTESIAN_POINT('Ctrl Pts',(1.29684196301123,-6.64417727060934,
41.8641802263497));
#193950=CARTESIAN_POINT('Ctrl Pts',(1.47905951217929,-6.60600284890497,
41.8729301153862));
#193951=CARTESIAN_POINT('Ctrl Pts',(1.65939532067517,-6.56038841607121,
41.8816800044227));
#193952=CARTESIAN_POINT('Ctrl Pts',(1.83972934301246,-6.51477443503132,
41.8904298067949));
#193953=CARTESIAN_POINT('Ctrl Pts',(2.0181813840672,-6.46172066061999,41.8991796091671));
#193954=CARTESIAN_POINT('Ctrl Pts',(2.19414528354666,-6.40140730423319,
41.9079294115392));
#193955=CARTESIAN_POINT('Ctrl Pts',(2.37010749864455,-6.34109452518472,
41.9166791301556));
#193956=CARTESIAN_POINT('Ctrl Pts',(2.54358134866903,-6.27352239616324,
41.9254288487719));
#193957=CARTESIAN_POINT('Ctrl Pts',(2.71397759435987,-6.1989204396663,41.9341785673882));
#193958=CARTESIAN_POINT('Ctrl Pts',(2.88437226558544,-6.12431917249317,
41.9429282051569));
#193959=CARTESIAN_POINT('Ctrl Pts',(3.05168912681364,-6.04268832278592,
41.9516778429256));
#193960=CARTESIAN_POINT('Ctrl Pts',(3.21535986274252,-5.9543051612312,41.9604274806943));
#193961=CARTESIAN_POINT('Ctrl Pts',(3.37902914073247,-5.86592278697208,
41.9691770405234));
#193962=CARTESIAN_POINT('Ctrl Pts',(3.53905210621983,-5.7707883574169,41.9779266003525));
#193963=CARTESIAN_POINT('Ctrl Pts',(3.69488522832114,-5.66922500431358,
41.9866761601815));
#193964=CARTESIAN_POINT('Ctrl Pts',(3.85071701407354,-5.56766252216807,
41.9954256449786));
#193965=CARTESIAN_POINT('Ctrl Pts',(4.00235878822814,-5.45967138329069,
42.0041751297758));
#193966=CARTESIAN_POINT('Ctrl Pts',(4.14929549611731,-5.34561838199292,
42.0129246145729));
#193967=CARTESIAN_POINT('Ctrl Pts',(4.29623099276485,-5.23156632086691,
42.0216740272455));
#193968=CARTESIAN_POINT('Ctrl Pts',(4.43846127436411,-5.11145267304631,
42.030423439918));
#193969=CARTESIAN_POINT('Ctrl Pts',(4.57550326054814,-4.98568540049544,
42.0391728525906));
#193970=CARTESIAN_POINT('Ctrl Pts',(4.7125441625814,-4.85991912290012,42.0479221960459));
#193971=CARTESIAN_POINT('Ctrl Pts',(4.84439664019108,-4.72849950385063,
42.0566715395011));
#193972=CARTESIAN_POINT('Ctrl Pts',(4.97061286795079,-4.59187289860706,
42.0654208829564));
#193973=CARTESIAN_POINT('Ctrl Pts',(5.09682813913007,-4.45524732884316,
42.0741701601012));
#193974=CARTESIAN_POINT('Ctrl Pts',(5.21740705148149,-4.31341506235413,
42.082919437246));
#193975=CARTESIAN_POINT('Ctrl Pts',(5.33194007545994,-4.16685781275343,
42.0916687143908));
#193976=CARTESIAN_POINT('Ctrl Pts',(5.44647226944759,-4.0203016252147,42.100417928132));
#193977=CARTESIAN_POINT('Ctrl Pts',(5.55495848628365,-3.86902074887572,
42.1091671418731));
#193978=CARTESIAN_POINT('Ctrl Pts',(5.65703027292018,-3.71352898080312,
42.1179163556142));
#193979=CARTESIAN_POINT('Ctrl Pts',(5.75910135377216,-3.55803828789234,
42.1266655088581));
#193980=CARTESIAN_POINT('Ctrl Pts',(5.8547579359296,-3.39833700106354,42.135414662102));
#193981=CARTESIAN_POINT('Ctrl Pts',(5.94367514427595,-3.23496750823193,
42.1441638153458));
#193982=CARTESIAN_POINT('Ctrl Pts',(6.03259176732825,-3.07159909077361,
42.1529129109988));
#193983=CARTESIAN_POINT('Ctrl Pts',(6.11476896836098,-2.90456276731069,
42.1616620066517));
#193984=CARTESIAN_POINT('Ctrl Pts',(6.18992765548048,-2.73442583002683,
42.1704111023046));
#193985=CARTESIAN_POINT('Ctrl Pts',(6.265085872832,-2.56428995615813,42.1791601432726));
#193986=CARTESIAN_POINT('Ctrl Pts',(6.33322554827291,-2.39105376934855,
42.1879091842407));
#193987=CARTESIAN_POINT('Ctrl Pts',(6.39411526733147,-2.21530561053744,
42.1966582252087));
#193988=CARTESIAN_POINT('Ctrl Pts',(6.45500462602956,-2.03955849184755,
42.2054072143977));
#193989=CARTESIAN_POINT('Ctrl Pts',(6.5086440204084,-1.86129970164195,42.2141562035868));
#193990=CARTESIAN_POINT('Ctrl Pts',(6.55485128368692,-1.68113463135703,
42.2229051927758));
#193991=CARTESIAN_POINT('Ctrl Pts',(6.60199809554403,-1.49730620116532,
42.2318320782472));
#193992=CARTESIAN_POINT('Ctrl Pts',(6.64140720707935,-1.31149343245381,
42.2407589637186));
#193993=CARTESIAN_POINT('Ctrl Pts',(6.67293928722934,-1.12435326697228,
42.2496858491901));
#193994=CARTESIAN_POINT('Ctrl Pts',(6.70384625876298,-0.940923067003626,
42.2584357633675));
#193995=CARTESIAN_POINT('Ctrl Pts',(6.72718554579829,-0.756217899518716,
42.267185677545));
#193996=CARTESIAN_POINT('Ctrl Pts',(6.74287786815353,-0.570865181251564,
42.2759355917224));
#193997=CARTESIAN_POINT('Ctrl Pts',(6.75856988190862,-0.385516108071076,
42.2846853338269));
#193998=CARTESIAN_POINT('Ctrl Pts',(6.76661520773411,-0.199519795223544,
42.2934350759314));
#193999=CARTESIAN_POINT('Ctrl Pts',(6.76698651789579,-0.0135080204529134,
42.3021848180359));
#194000=CARTESIAN_POINT('Ctrl Pts',(6.76735782124896,0.172500343515658,
42.3109343997008));
#194001=CARTESIAN_POINT('Ctrl Pts',(6.7600553899517,0.358523882213577,42.3196839813658));
#194002=CARTESIAN_POINT('Ctrl Pts',(6.7451040274234,0.543930748566989,42.3284335630308));
#194003=CARTESIAN_POINT('Ctrl Pts',(6.73015291918002,0.729334461617808,
42.3371829958875));
#194004=CARTESIAN_POINT('Ctrl Pts',(6.7075531630656,0.914121237637212,42.3459324287441));
#194005=CARTESIAN_POINT('Ctrl Pts',(6.67738151874533,1.0976634516637,42.3546818616008));
#194006=CARTESIAN_POINT('Ctrl Pts',(6.64721034747522,1.28120278799909,42.3634311572784));
#194007=CARTESIAN_POINT('Ctrl Pts',(6.60946757205088,1.46349731860569,42.3721804529559));
#194008=CARTESIAN_POINT('Ctrl Pts',(6.56428138111464,1.64392790278397,42.3809297486334));
#194009=CARTESIAN_POINT('Ctrl Pts',(6.51909583859785,1.82435589779289,42.389678918759));
#194010=CARTESIAN_POINT('Ctrl Pts',(6.46646716392804,2.00291972192496,42.3984280888846));
#194011=CARTESIAN_POINT('Ctrl Pts',(6.40657409872806,2.17901292274891,42.4071772590102));
#194012=CARTESIAN_POINT('Ctrl Pts',(6.34668181341991,2.35510383059207,42.4159263152093));
#194013=CARTESIAN_POINT('Ctrl Pts',(6.27952541913957,2.52872390822811,42.4246753714084));
#194014=CARTESIAN_POINT('Ctrl Pts',(6.20533299175416,2.69928350890518,42.4334244276075));
#194015=CARTESIAN_POINT('Ctrl Pts',(6.12831602991443,2.87633637965847,42.4425065637657));
#194016=CARTESIAN_POINT('Ctrl Pts',(6.04371690605161,3.05009086601678,42.4515886999239));
#194017=CARTESIAN_POINT('Ctrl Pts',(5.95184520316519,3.21991112882942,42.4606708360821));
#194018=CARTESIAN_POINT('Ctrl Pts',(5.86333549509153,3.38351691183227,42.4694206164257));
#194019=CARTESIAN_POINT('Ctrl Pts',(5.76807618099238,3.54347103712216,42.4781703967693));
#194020=CARTESIAN_POINT('Ctrl Pts',(5.66639083308876,3.69923018027909,42.4869201771128));
#194021=CARTESIAN_POINT('Ctrl Pts',(5.56470914082053,3.85498372382262,42.4956696428977));
#194022=CARTESIAN_POINT('Ctrl Pts',(5.45660203371912,4.00654234702208,42.5044191086826));
#194023=CARTESIAN_POINT('Ctrl Pts',(5.34243669839054,4.15339127986877,42.5131685744676));
#194024=CARTESIAN_POINT('Ctrl Pts',(5.22827486050418,4.30023571401491,42.5219177722136));
#194025=CARTESIAN_POINT('Ctrl Pts',(5.10805534166926,4.44237052028683,42.5306669699596));
#194026=CARTESIAN_POINT('Ctrl Pts',(4.98218644339754,4.57931296628936,42.5394161677056));
#194027=CARTESIAN_POINT('Ctrl Pts',(4.85632073219396,4.71625194483556,42.5481651439172));
#194028=CARTESIAN_POINT('Ctrl Pts',(4.72480612170136,4.84799861524685,42.5569141201289));
#194029=CARTESIAN_POINT('Ctrl Pts',(4.58808925235138,4.97410554898645,42.5656630963405));
#194030=CARTESIAN_POINT('Ctrl Pts',(4.45136349473871,5.10022068121361,42.5744126413422));
#194031=CARTESIAN_POINT('Ctrl Pts',(4.309435012099,5.22069514871983,42.5831621863439));
#194032=CARTESIAN_POINT('Ctrl Pts',(4.16278587431598,5.335119751664,42.5919117313456));
#194033=CARTESIAN_POINT('Ctrl Pts',(4.01614535740258,5.44953762807982,42.6006607619993));
#194034=CARTESIAN_POINT('Ctrl Pts',(3.86478496657727,5.5579061753292,42.6094097926531));
#194035=CARTESIAN_POINT('Ctrl Pts',(3.70921874746993,5.65985735539489,42.6181588233068));
#194036=CARTESIAN_POINT('Ctrl Pts',(3.5536504160569,5.76180991977176,42.6269079727564));
#194037=CARTESIAN_POINT('Ctrl Pts',(3.39387638174305,5.85734478552939,42.635657122206));
#194038=CARTESIAN_POINT('Ctrl Pts',(3.23043927904314,5.94613749121354,42.6444062716556));
#194039=CARTESIAN_POINT('Ctrl Pts',(3.18691767070278,5.96978206944228,42.6467360795718));
#194040=CARTESIAN_POINT('Ctrl Pts',(3.14313645919552,5.99294880633466,42.6490658874879));
#194041=CARTESIAN_POINT('Ctrl Pts',(3.09910619832134,6.0156321173694,42.651395695404));
#194042=CARTESIAN_POINT('Origin',(0.,0.,4.30282021618968));
#194043=CARTESIAN_POINT('',(3.09910619832132,6.01563211736941,45.0457774706169));
#194044=CARTESIAN_POINT('',(3.09910619832132,6.01563211736941,44.6516492284231));
#194045=CARTESIAN_POINT('',(3.09910619832133,6.0156321173694,4.30282021618968));
#194046=CARTESIAN_POINT('',(-6.76699922072898,0.00324756113893609,43.6971797837735));
#194047=CARTESIAN_POINT('Ctrl Pts',(-6.76699922072936,0.00324756035794601,
43.6971797838101));
#194048=CARTESIAN_POINT('Ctrl Pts',(-6.76708539128521,-0.176307557950773,
43.7055896024739));
#194049=CARTESIAN_POINT('Ctrl Pts',(-6.76002065673009,-0.355840812135418,
43.7139994211378));
#194050=CARTESIAN_POINT('Ctrl Pts',(-6.74583735173559,-0.534759220517912,
43.7224092398016));
#194051=CARTESIAN_POINT('Ctrl Pts',(-6.73172457194684,-0.712787973240606,
43.7307772414001));
#194052=CARTESIAN_POINT('Ctrl Pts',(-6.71056392607303,-0.890207646468588,
43.7391452429986));
#194053=CARTESIAN_POINT('Ctrl Pts',(-6.6824392701373,-1.06644005969713,
43.7475132445971));
#194054=CARTESIAN_POINT('Ctrl Pts',(-6.65430116369288,-1.24275675540054,
43.7558852481602));
#194055=CARTESIAN_POINT('Ctrl Pts',(-6.61919245918884,-1.41788472534874,
43.7642572517233));
#194056=CARTESIAN_POINT('Ctrl Pts',(-6.57724817004016,-1.59125595354843,
43.7726292552864));
#194057=CARTESIAN_POINT('Ctrl Pts',(-6.53527761298665,-1.76473575669399,
43.7810065018754));
#194058=CARTESIAN_POINT('Ctrl Pts',(-6.48646301442609,-1.93645629632921,
43.7893837484644));
#194059=CARTESIAN_POINT('Ctrl Pts',(-6.43098936457008,-2.10586438138513,
43.7977609950534));
#194060=CARTESIAN_POINT('Ctrl Pts',(-6.37511427176604,-2.27649841211543,
43.8061988647774));
#194061=CARTESIAN_POINT('Ctrl Pts',(-6.31248349073343,-2.4447860605028,
43.8146367345015));
#194062=CARTESIAN_POINT('Ctrl Pts',(-6.24333507747812,-2.61018315647223,
43.8230746042255));
#194063=CARTESIAN_POINT('Ctrl Pts',(-6.17452783411554,-2.77476420321026,
43.8314708425227));
#194064=CARTESIAN_POINT('Ctrl Pts',(-6.09926733108904,-2.93648287925634,
43.8398670808199));
#194065=CARTESIAN_POINT('Ctrl Pts',(-6.01783402746916,-3.09482836645821,
43.8482633191171));
#194066=CARTESIAN_POINT('Ctrl Pts',(-5.93579506250964,-3.25435155044554,
43.8567220045546));
#194067=CARTESIAN_POINT('Ctrl Pts',(-5.84749129217044,-3.41045087005848,
43.865180689992));
#194068=CARTESIAN_POINT('Ctrl Pts',(-5.75325351341666,-3.56263427962496,
43.8736393754295));
#194069=CARTESIAN_POINT('Ctrl Pts',(-5.65901573466289,-3.71481768919144,
43.882098060867));
#194070=CARTESIAN_POINT('Ctrl Pts',(-5.55884418801034,-3.86308493565928,
43.8905567463044));
#194071=CARTESIAN_POINT('Ctrl Pts',(-5.4531104642186,-4.00697832100819,
43.8990154317419));
#194072=CARTESIAN_POINT('Ctrl Pts',(-5.3522439502868,-4.14424790385744,
43.9070847409644));
#194073=CARTESIAN_POINT('Ctrl Pts',(-5.24600592261595,-4.27795795198755,
43.9151540501869));
#194074=CARTESIAN_POINT('Ctrl Pts',(-5.1346786257687,-4.40764839909833,
43.9232233594094));
#194075=CARTESIAN_POINT('Ctrl Pts',(-5.0234901843183,-4.53717708697296,
43.9312826040102));
#194076=CARTESIAN_POINT('Ctrl Pts',(-4.90722534389093,-4.66269586987897,
43.939341848611));
#194077=CARTESIAN_POINT('Ctrl Pts',(-4.78621000370878,-4.78377286254249,
43.9474010932117));
#194078=CARTESIAN_POINT('Ctrl Pts',(-4.66531904592962,-4.90472540943516,
43.955452054332));
#194079=CARTESIAN_POINT('Ctrl Pts',(-4.53968756656092,-5.02124498958605,
43.9635030154522));
#194080=CARTESIAN_POINT('Ctrl Pts',(-4.40968210592735,-5.13293217612157,
43.9715539765725));
#194081=CARTESIAN_POINT('Ctrl Pts',(-4.27978178117675,-5.24452904082819,
43.9795984268516));
#194082=CARTESIAN_POINT('Ctrl Pts',(-4.14551479706261,-5.35130104816285,
43.9876428771306));
#194083=CARTESIAN_POINT('Ctrl Pts',(-4.0072848964897,-5.4528851774419,43.9956873274097));
#194084=CARTESIAN_POINT('Ctrl Pts',(-3.86913652570079,-5.55440939108704,
44.0037270329679));
#194085=CARTESIAN_POINT('Ctrl Pts',(-3.72703019139388,-5.65075159757475,
44.0117667385261));
#194086=CARTESIAN_POINT('Ctrl Pts',(-3.5814030120783,-5.74158875792028,
44.0198064440844));
#194087=CARTESIAN_POINT('Ctrl Pts',(-3.43263254795316,-5.83438658980803,
44.0280196823888));
#194088=CARTESIAN_POINT('Ctrl Pts',(-3.28018782247643,-5.92143876717896,
44.0362329206933));
#194089=CARTESIAN_POINT('Ctrl Pts',(-3.12456687615307,-6.00244707069101,
44.0444461589977));
#194090=CARTESIAN_POINT('Ctrl Pts',(-2.9722829910162,-6.08171827086433,
44.0524832765459));
#194091=CARTESIAN_POINT('Ctrl Pts',(-2.81695807331615,-6.15520200520335,
44.0605203940941));
#194092=CARTESIAN_POINT('Ctrl Pts',(-2.65908395749321,-6.22266514501642,
44.0685575116422));
#194093=CARTESIAN_POINT('Ctrl Pts',(-2.50119313959246,-6.29013542200082,
44.0765954794663));
#194094=CARTESIAN_POINT('Ctrl Pts',(-2.34075293012029,-6.3515836892884,
44.0846334472905));
#194095=CARTESIAN_POINT('Ctrl Pts',(-2.17827511616023,-6.40682499513738,
44.0926714151146));
#194096=CARTESIAN_POINT('Ctrl Pts',(-2.01574792023636,-6.46208309050427,
44.1007118259223));
#194097=CARTESIAN_POINT('Ctrl Pts',(-1.85118224066694,-6.51113034921,44.10875223673));
#194098=CARTESIAN_POINT('Ctrl Pts',(-1.6851048415235,-6.55383175501737,
44.1167926475377));
#194099=CARTESIAN_POINT('Ctrl Pts',(-1.5127506533799,-6.59814703312552,
44.1251369405255));
#194100=CARTESIAN_POINT('Ctrl Pts',(-1.33876867553726,-6.63562730071976,
44.1334812335133));
#194101=CARTESIAN_POINT('Ctrl Pts',(-1.16375790499993,-6.66618005596535,
44.1418255265011));
#194102=CARTESIAN_POINT('Ctrl Pts',(-0.994822856547196,-6.69567213334968,
44.1498801367167));
#194103=CARTESIAN_POINT('Ctrl Pts',(-0.824929623160702,-6.71870964961567,
44.1579347469322));
#194104=CARTESIAN_POINT('Ctrl Pts',(-0.654620370348223,-6.73526251683816,
44.1659893571478));
#194105=CARTESIAN_POINT('Ctrl Pts',(-0.484182191025886,-6.75182791481494,
44.174050064817));
#194106=CARTESIAN_POINT('Ctrl Pts',(-0.313327735545389,-6.76189886758439,
44.1821107724862));
#194107=CARTESIAN_POINT('Ctrl Pts',(-0.142598077855184,-6.76549737921699,
44.1901714801554));
#194108=CARTESIAN_POINT('Ctrl Pts',(0.0283722984240017,-6.76910096453542,
44.1982435529396));
#194109=CARTESIAN_POINT('Ctrl Pts',(0.19921715589738,-6.76621390754684,
44.2063156257237));
#194110=CARTESIAN_POINT('Ctrl Pts',(0.369401038750248,-6.75690993521227,
44.2143876985078));
#194111=CARTESIAN_POINT('Ctrl Pts',(0.387226507463855,-6.75593541479951,
44.2152331868024));
#194112=CARTESIAN_POINT('Ctrl Pts',(0.405044734747265,-6.75489054063013,
44.2160786750969));
#194113=CARTESIAN_POINT('Ctrl Pts',(0.422855112852365,-6.75377542960488,
44.2169241633914));
#194114=CARTESIAN_POINT('Ctrl Pts',(0.598389763461888,-6.74278517307849,
44.2252570854381));
#194115=CARTESIAN_POINT('Ctrl Pts',(0.773721088922039,-6.72493313061228,
44.2335900074848));
#194116=CARTESIAN_POINT('Ctrl Pts',(0.948279363318132,-6.70022799978515,
44.2419229295316));
#194117=CARTESIAN_POINT('Ctrl Pts',(1.12263135216511,-6.67555206443156,
44.2502460040852));
#194118=CARTESIAN_POINT('Ctrl Pts',(1.29621176825503,-6.64403922228022,
44.2585690786388));
#194119=CARTESIAN_POINT('Ctrl Pts',(1.46845310760402,-6.60575010659411,
44.2668921531925));
#194120=CARTESIAN_POINT('Ctrl Pts',(1.64052251534514,-6.56749921117062,
44.2752069196384));
#194121=CARTESIAN_POINT('Ctrl Pts',(1.81125517187407,-6.52248559348524,
44.2835216860844));
#194122=CARTESIAN_POINT('Ctrl Pts',(1.98009067900291,-6.47082142412583,
44.2918364525304));
#194123=CARTESIAN_POINT('Ctrl Pts',(2.14878862434689,-6.41919934908337,
44.3001444443699));
#194124=CARTESIAN_POINT('Ctrl Pts',(2.31559216901612,-6.36093762086397,
44.3084524362095));
#194125=CARTESIAN_POINT('Ctrl Pts',(2.47995284387544,-6.29619908295109,
44.316760428049));
#194126=CARTESIAN_POINT('Ctrl Pts',(2.64420973573751,-6.23150142318323,
44.3250631739361));
#194127=CARTESIAN_POINT('Ctrl Pts',(2.80602650900681,-6.16033523112452,
44.3333659198231));
#194128=CARTESIAN_POINT('Ctrl Pts',(2.96487134177183,-6.0829127008975,44.3416686657101));
#194129=CARTESIAN_POINT('Ctrl Pts',(3.12365125971659,-6.00552181079088,
44.3499680185296));
#194130=CARTESIAN_POINT('Ctrl Pts',(3.27946134495144,-5.92187982926044,
44.358267371349));
#194131=CARTESIAN_POINT('Ctrl Pts',(3.43179093234813,-5.83224656514565,
44.3665667241684));
#194132=CARTESIAN_POINT('Ctrl Pts',(3.58408812179778,-5.74263236452202,
44.3748643118548));
#194133=CARTESIAN_POINT('Ctrl Pts',(3.73290598846745,-5.64702959623125,
44.3831618995411));
#194134=CARTESIAN_POINT('Ctrl Pts',(3.87775939203867,-5.54574351169037,
44.3914594872275));
#194135=CARTESIAN_POINT('Ctrl Pts',(4.0226060587724,-5.44446213775951,44.3997566890099));
#194136=CARTESIAN_POINT('Ctrl Pts',(4.16348834482187,-5.33749817378009,
44.4080538907923));
#194137=CARTESIAN_POINT('Ctrl Pts',(4.29995081804031,-5.22519970550739,
44.4163510925747));
#194138=CARTESIAN_POINT('Ctrl Pts',(4.43642962034128,-5.11288779961398,
44.4246492871992));
#194139=CARTESIAN_POINT('Ctrl Pts',(4.56848728772864,-4.99524033900479,
44.4329474818238));
#194140=CARTESIAN_POINT('Ctrl Pts',(4.69570200726063,-4.87264524247442,
44.4412456764483));
#194141=CARTESIAN_POINT('Ctrl Pts',(4.82300619838821,-4.74996392338316,
44.4495497072899));
#194142=CARTESIAN_POINT('Ctrl Pts',(4.9454603847808,-4.62232825689607,44.4578537381314));
#194143=CARTESIAN_POINT('Ctrl Pts',(5.06267950072881,-4.49016316773682,
44.466157768973));
#194144=CARTESIAN_POINT('Ctrl Pts',(5.17994124077344,-4.35795001971374,
44.4744648193887));
#194145=CARTESIAN_POINT('Ctrl Pts',(5.29196389093938,-4.22120443144269,
44.4827718698045));
#194146=CARTESIAN_POINT('Ctrl Pts',(5.39840302243799,-4.0803840269431,44.4910789202202));
#194147=CARTESIAN_POINT('Ctrl Pts',(5.50495595533231,-3.93941306166431,
44.4993948522748));
#194148=CARTESIAN_POINT('Ctrl Pts',(5.60591323799116,-3.79435885764037,
44.5077107843295));
#194149=CARTESIAN_POINT('Ctrl Pts',(5.70097346544871,-3.64570851087271,
44.5160267163841));
#194150=CARTESIAN_POINT('Ctrl Pts',(5.77263188405087,-3.53365272204359,
44.522295442603));
#194151=CARTESIAN_POINT('Ctrl Pts',(5.84094021461499,-3.41955404417975,
44.5285641688219));
#194152=CARTESIAN_POINT('Ctrl Pts',(5.90578678435719,-3.30363004250052,
44.5348328950408));
#194153=CARTESIAN_POINT('Ctrl Pts',(5.99320022705266,-3.14736401149683,
44.5432831637642));
#194154=CARTESIAN_POINT('Ctrl Pts',(6.07448193940124,-2.98749380427392,
44.5517334324875));
#194155=CARTESIAN_POINT('Ctrl Pts',(6.1493359130113,-2.82452771785825,44.5601837012109));
#194156=CARTESIAN_POINT('Ctrl Pts',(6.22412382544997,-2.66170545454302,
44.5686265122854));
#194157=CARTESIAN_POINT('Ctrl Pts',(6.29249516810258,-2.49579305775209,
44.5770693233599));
#194158=CARTESIAN_POINT('Ctrl Pts',(6.35419972174159,-2.32732354781606,
44.5855121344344));
#194159=CARTESIAN_POINT('Ctrl Pts',(6.41585822025235,-2.15897978038082,
44.5939486439522));
#194160=CARTESIAN_POINT('Ctrl Pts',(6.47085973539428,-1.98808301478628,
44.6023851534699));
#194161=CARTESIAN_POINT('Ctrl Pts',(6.51900192249456,-1.81518674921131,
44.6108216629877));
#194162=CARTESIAN_POINT('Ctrl Pts',(6.56710966126934,-1.64241420021824,
44.6192521357289));
#194163=CARTESIAN_POINT('Ctrl Pts',(6.6083677735055,-1.46764532376163,44.6276826084701));
#194164=CARTESIAN_POINT('Ctrl Pts',(6.64262351808422,-1.29144949455812,
44.6361130812113));
#194165=CARTESIAN_POINT('Ctrl Pts',(6.67686453621108,-1.11532941146462,
44.6445399297151));
#194166=CARTESIAN_POINT('Ctrl Pts',(6.7041091246507,-0.937783923435001,
44.6529667782189));
#194167=CARTESIAN_POINT('Ctrl Pts',(6.72425533318508,-0.759393978203656,
44.6613936267227));
#194168=CARTESIAN_POINT('Ctrl Pts',(6.74439532330438,-0.581059095577448,
44.6698178741593));
#194169=CARTESIAN_POINT('Ctrl Pts',(6.75744126575737,-0.401880604658297,
44.6782421215959));
#194170=CARTESIAN_POINT('Ctrl Pts',(6.76334285848322,-0.222446349945432,
44.6866663690325));
#194171=CARTESIAN_POINT('Ctrl Pts',(6.76500570151503,-0.171888642225172,
44.6890399996436));
#194172=CARTESIAN_POINT('Ctrl Pts',(6.76610167319886,-0.121310658110363,
44.6914136302547));
#194173=CARTESIAN_POINT('Ctrl Pts',(6.76663039405615,-0.0707255981630307,
44.6937872608658));
#194174=CARTESIAN_POINT('Ctrl Pts',(6.76855020804263,0.112951486361858,
44.702406041803));
#194175=CARTESIAN_POINT('Ctrl Pts',(6.76298624196818,0.296639716696282,
44.7110248227403));
#194176=CARTESIAN_POINT('Ctrl Pts',(6.7499743874485,0.479723637930475,44.7196436036775));
#194177=CARTESIAN_POINT('Ctrl Pts',(6.736954716787,0.662917536561891,44.728267561864));
#194178=CARTESIAN_POINT('Ctrl Pts',(6.71647825069517,0.84550609823776,44.7368915200505));
#194179=CARTESIAN_POINT('Ctrl Pts',(6.68863272004142,1.02687941667527,44.745515478237));
#194180=CARTESIAN_POINT('Ctrl Pts',(6.65978122537314,1.21480513426844,44.7544509906081));
#194181=CARTESIAN_POINT('Ctrl Pts',(6.62301836171851,1.40142581027156,44.7633865029792));
#194182=CARTESIAN_POINT('Ctrl Pts',(6.57849929254961,1.58607567849844,44.7723220153503));
#194183=CARTESIAN_POINT('Ctrl Pts',(6.53545213559658,1.76462055841857,44.780962097245));
#194184=CARTESIAN_POINT('Ctrl Pts',(6.48515357156149,1.94132258415672,44.7896021791398));
#194185=CARTESIAN_POINT('Ctrl Pts',(6.42779458480289,2.1155958441013,44.7982422610345));
#194186=CARTESIAN_POINT('Ctrl Pts',(6.36749368273758,2.29880749713741,44.8073254886438));
#194187=CARTESIAN_POINT('Ctrl Pts',(6.29938922163399,2.47933433172568,44.8164087162531));
#194188=CARTESIAN_POINT('Ctrl Pts',(6.22376038338747,2.65651946918833,44.8254919438625));
#194189=CARTESIAN_POINT('Ctrl Pts',(6.14813154514096,2.83370460665094,44.8345751714718));
#194190=CARTESIAN_POINT('Ctrl Pts',(6.06497852743741,3.00754771169249,44.8436583990811));
#194191=CARTESIAN_POINT('Ctrl Pts',(5.97463653142741,3.17742148877562,44.8527416266904));
#194192=CARTESIAN_POINT('Ctrl Pts',(5.88467877765542,3.34657275934829,44.8617862215502));
#194193=CARTESIAN_POINT('Ctrl Pts',(5.78751076787639,3.51194501315713,44.87083081641));
#194194=CARTESIAN_POINT('Ctrl Pts',(5.68345990189301,3.67295147579904,44.8798754112698));
#194195=CARTESIAN_POINT('Ctrl Pts',(5.57950451895655,3.8338101896694,44.8889117062902));
#194196=CARTESIAN_POINT('Ctrl Pts',(5.46867901895975,3.9903109113421,44.8979480013106));
#194197=CARTESIAN_POINT('Ctrl Pts',(5.35135512372724,4.14189417293081,44.906984296331));
#194198=CARTESIAN_POINT('Ctrl Pts',(5.23423884232874,4.29320919604988,44.9160046009187));
#194199=CARTESIAN_POINT('Ctrl Pts',(5.11064727398898,4.43962394765089,44.9250249055064));
#194200=CARTESIAN_POINT('Ctrl Pts',(4.98099342848918,4.58061059961962,44.9340452100941));
#194201=CARTESIAN_POINT('Ctrl Pts',(4.85150285682168,4.72141970628777,44.9430541553604));
#194202=CARTESIAN_POINT('Ctrl Pts',(4.71596540390273,4.85681418032171,44.9520631006267));
#194203=CARTESIAN_POINT('Ctrl Pts',(4.57483371642635,4.9862997770941,44.961072045893));
#194204=CARTESIAN_POINT('Ctrl Pts',(4.43402250913482,5.11549133948817,44.9700605337518));
#194205=CARTESIAN_POINT('Ctrl Pts',(4.28764259918326,5.23880064719497,44.9790490216106));
#194206=CARTESIAN_POINT('Ctrl Pts',(4.13618240226534,5.35577110556365,44.9880375094694));
#194207=CARTESIAN_POINT('Ctrl Pts',(4.00329692485621,5.4583965842002,44.9959236704846));
#194208=CARTESIAN_POINT('Ctrl Pts',(3.86650145993055,5.55614306622334,45.0038098314999));
#194209=CARTESIAN_POINT('Ctrl Pts',(3.72614913619673,5.64872566291021,45.0116959925152));
#194210=CARTESIAN_POINT('Ctrl Pts',(3.58161445003416,5.7440671307268,45.0198171534412));
#194211=CARTESIAN_POINT('Ctrl Pts',(3.43337156207057,5.83388832813256,45.0279383143671));
#194212=CARTESIAN_POINT('Ctrl Pts',(3.28188888549178,5.91789610784826,45.036059475293));
#194213=CARTESIAN_POINT('Ctrl Pts',(3.22146616366386,5.9514047493628,45.0392988070677));
#194214=CARTESIAN_POINT('Ctrl Pts',(3.16052829945035,5.98398895658282,45.0425381388423));
#194215=CARTESIAN_POINT('Ctrl Pts',(3.09910619832133,6.01563211736941,45.0457774706169));
#194216=CARTESIAN_POINT('Ctrl Pts',(3.09910619832137,6.01563211736938,43.0457451347211));
#194217=CARTESIAN_POINT('Ctrl Pts',(2.9398432053638,6.0976805071326,43.0541676123953));
#194218=CARTESIAN_POINT('Ctrl Pts',(2.77728306715381,6.17341931069911,43.0625900900695));
#194219=CARTESIAN_POINT('Ctrl Pts',(2.61195574420795,6.24259370696981,43.0710125677437));
#194220=CARTESIAN_POINT('Ctrl Pts',(2.44662669862841,6.3117688240055,43.0794351331761));
#194221=CARTESIAN_POINT('Ctrl Pts',(2.27853071565575,6.37437926216612,43.0878576986086));
#194222=CARTESIAN_POINT('Ctrl Pts',(2.10821854588746,6.43021800274113,43.0962802640411));
#194223=CARTESIAN_POINT('Ctrl Pts',(1.93790130694559,6.48605840530113,43.1047030801629));
#194224=CARTESIAN_POINT('Ctrl Pts',(1.76536806660186,6.53512660429797,43.1131258962847));
#194225=CARTESIAN_POINT('Ctrl Pts',(1.59118572837604,6.57726515945742,43.1215487124066));
#194226=CARTESIAN_POINT('Ctrl Pts',(1.41697388813736,6.61941085180545,43.129972955137));
#194227=CARTESIAN_POINT('Ctrl Pts',(1.24111271735234,6.65462448186093,43.1383971978675));
#194228=CARTESIAN_POINT('Ctrl Pts',(1.06418068793334,6.68279944809282,43.146821440598));
#194229=CARTESIAN_POINT('Ctrl Pts',(0.887193981831948,6.71098312113538,
43.1552482866425));
#194230=CARTESIAN_POINT('Ctrl Pts',(0.709136086613573,6.73212374129672,
43.1636751326871));
#194231=CARTESIAN_POINT('Ctrl Pts',(0.530592361061849,6.74616637405147,
43.1721019787316));
#194232=CARTESIAN_POINT('Ctrl Pts',(0.35188828729745,6.7602216183447,43.1805363928366));
#194233=CARTESIAN_POINT('Ctrl Pts',(0.172697844219148,6.76716611134562,
43.1889708069416));
#194234=CARTESIAN_POINT('Ctrl Pts',(-0.00639066836027456,6.76699698236655,
43.1974052210466));
#194235=CARTESIAN_POINT('Ctrl Pts',(-0.185565022304428,6.76682777231995,
43.2058436779659));
#194236=CARTESIAN_POINT('Ctrl Pts',(-0.364637014990389,6.75953814839691,
43.2142821348853));
#194237=CARTESIAN_POINT('Ctrl Pts',(-0.54302114782077,6.74517731664776,
43.2227205918047));
#194238=CARTESIAN_POINT('Ctrl Pts',(-0.721605831932116,6.73080033949847,
43.2311685357973));
#194239=CARTESIAN_POINT('Ctrl Pts',(-0.899500779066923,6.70933630365108,
43.23961647979));
#194240=CARTESIAN_POINT('Ctrl Pts',(-1.07612714782113,6.6808861209964,43.2480644237827));
#194241=CARTESIAN_POINT('Ctrl Pts',(-1.18159592783921,6.66389768332968,
43.2531089386694));
#194242=CARTESIAN_POINT('Ctrl Pts',(-1.28661256810347,6.64441922430788,
43.2581534535561));
#194243=CARTESIAN_POINT('Ctrl Pts',(-1.39105602147073,6.62248081500657,
43.2631979684429));
#194244=CARTESIAN_POINT('Ctrl Pts',(-1.56165025698225,6.58664739469695,
43.2714375002937));
#194245=CARTESIAN_POINT('Ctrl Pts',(-1.73109537092469,6.54416838885696,
43.2796770321445));
#194246=CARTESIAN_POINT('Ctrl Pts',(-1.89883704638144,6.49512947301972,
43.2879165639953));
#194247=CARTESIAN_POINT('Ctrl Pts',(-2.06639254030146,6.44614498695186,
43.2961469505415));
#194248=CARTESIAN_POINT('Ctrl Pts',(-2.23224802183424,6.39061518765132,
43.3043773370878));
#194249=CARTESIAN_POINT('Ctrl Pts',(-2.39585840662889,6.32867691507362,
43.3126077236341));
#194250=CARTESIAN_POINT('Ctrl Pts',(-2.55931638192079,6.26679634043078,
43.3208304432519));
#194251=CARTESIAN_POINT('Ctrl Pts',(-2.72053309462844,6.19851930662708,
43.3290531628697));
#194252=CARTESIAN_POINT('Ctrl Pts',(-2.87897760889233,6.1240327340321,43.3372758824875));
#194253=CARTESIAN_POINT('Ctrl Pts',(-3.03728172990059,6.04961216190722,
43.3454913161832));
#194254=CARTESIAN_POINT('Ctrl Pts',(-3.19281822737472,5.96899316803299,
43.353706749879));
#194255=CARTESIAN_POINT('Ctrl Pts',(-3.34507530189061,5.88241108939876,
43.3619221835748));
#194256=CARTESIAN_POINT('Ctrl Pts',(-3.49725412809285,5.79587350722991,
43.3701333951755));
#194257=CARTESIAN_POINT('Ctrl Pts',(-3.64615657927168,5.70337911914984,
43.3783446067763));
#194258=CARTESIAN_POINT('Ctrl Pts',(-3.79129429437053,5.60520977069311,
43.3865558183771));
#194259=CARTESIAN_POINT('Ctrl Pts',(-3.93638333828836,5.50707334281892,
43.3947642763905));
#194260=CARTESIAN_POINT('Ctrl Pts',(-4.07770986661839,5.40326594483289,
43.402972734404));
#194261=CARTESIAN_POINT('Ctrl Pts',(-4.21481334735167,5.29411347129869,
43.4111811924175));
#194262=CARTESIAN_POINT('Ctrl Pts',(-4.27589594178423,5.24548366090626,
43.4148382397009));
#194263=CARTESIAN_POINT('Ctrl Pts',(-4.33614069485268,5.1957934790453,43.4184952869842));
#194264=CARTESIAN_POINT('Ctrl Pts',(-4.39550886582442,5.14507442224687,
43.4221523342676));
#194265=CARTESIAN_POINT('Ctrl Pts',(-4.53932626537561,5.02220921119109,
43.4310114084435));
#194266=CARTESIAN_POINT('Ctrl Pts',(-4.67784794423911,4.89343143470241,
43.4398704826195));
#194267=CARTESIAN_POINT('Ctrl Pts',(-4.81062718086157,4.75921791124927,
43.4487295567954));
#194268=CARTESIAN_POINT('Ctrl Pts',(-4.94365588295502,4.62475222758876,
43.4576052753893));
#194269=CARTESIAN_POINT('Ctrl Pts',(-5.07092039950944,4.48483057181061,
43.4664809939832));
#194270=CARTESIAN_POINT('Ctrl Pts',(-5.19201350524001,4.3399636820376,43.4753567125771));
#194271=CARTESIAN_POINT('Ctrl Pts',(-5.31345217648036,4.19468338309228,
43.4842577599641));
#194272=CARTESIAN_POINT('Ctrl Pts',(-5.42868402661054,4.04442980962973,
43.4931588073511));
#194273=CARTESIAN_POINT('Ctrl Pts',(-5.53734268853429,3.88974612921407,
43.5020598547381));
#194274=CARTESIAN_POINT('Ctrl Pts',(-5.6461490733983,3.73485215421465,43.510973003221));
#194275=CARTESIAN_POINT('Ctrl Pts',(-5.74836427551116,3.5755162572007,43.519886151704));
#194276=CARTESIAN_POINT('Ctrl Pts',(-5.84366668278929,3.41230841227144,
43.5287993001869));
#194277=CARTESIAN_POINT('Ctrl Pts',(-5.93918068747235,3.24873820129669,
43.5377322382968));
#194278=CARTESIAN_POINT('Ctrl Pts',(-6.02775106666007,3.08127907205079,
43.5466651764067));
#194279=CARTESIAN_POINT('Ctrl Pts',(-6.10910207358148,2.91052587251211,
43.5555981145166));
#194280=CARTESIAN_POINT('Ctrl Pts',(-6.1865364367665,2.74799358473288,43.5641009763752));
#194281=CARTESIAN_POINT('Ctrl Pts',(-6.25743014094712,2.58247711366446,
43.5726038382338));
#194282=CARTESIAN_POINT('Ctrl Pts',(-6.321586751586,2.41450407789517,43.5811067000924));
#194283=CARTESIAN_POINT('Ctrl Pts',(-6.3896604380815,2.23627546415156,43.5901287033858));
#194284=CARTESIAN_POINT('Ctrl Pts',(-6.45025510538802,2.05500312572533,
43.5991507066792));
#194285=CARTESIAN_POINT('Ctrl Pts',(-6.50311556953205,1.87130352677213,
43.6081727099725));
#194286=CARTESIAN_POINT('Ctrl Pts',(-6.55579193961244,1.68824368772661,
43.6171632928599));
#194287=CARTESIAN_POINT('Ctrl Pts',(-6.60078777408356,1.50277368155816,
43.6261538757472));
#194288=CARTESIAN_POINT('Ctrl Pts',(-6.63789736808551,1.31552557206748,
43.6351444586345));
#194289=CARTESIAN_POINT('Ctrl Pts',(-6.67492295241124,1.12870135977843,
43.6441146884035));
#194290=CARTESIAN_POINT('Ctrl Pts',(-6.70409785465102,0.940107305172852,
43.6530849181725));
#194291=CARTESIAN_POINT('Ctrl Pts',(-6.72526609179442,0.750389895028057,
43.6620551479416));
#194292=CARTESIAN_POINT('Ctrl Pts',(-6.74636212545597,0.561319598645588,
43.6709947808395));
#194293=CARTESIAN_POINT('Ctrl Pts',(-6.75950593593842,0.371133826403229,
43.6799344137374));
#194294=CARTESIAN_POINT('Ctrl Pts',(-6.76459261047664,0.180487712282064,
43.6888740466354));
#194295=CARTESIAN_POINT('Ctrl Pts',(-6.76616793920673,0.121445149484368,
43.6916426256814));
#194296=CARTESIAN_POINT('Ctrl Pts',(-6.76697085269131,0.0623585310693763,
43.6944112047275));
#194297=CARTESIAN_POINT('Ctrl Pts',(-6.76699922072898,0.00324756113897147,
43.6971797837735));
#194298=CARTESIAN_POINT('',(-6.767,4.1676968679568E-13,43.3028202161899));
#194299=CARTESIAN_POINT('Ctrl Pts',(3.09910619832134,6.0156321173694,42.651395695404));
#194300=CARTESIAN_POINT('Ctrl Pts',(2.93375330764829,6.10081787314652,42.6601451433063));
#194301=CARTESIAN_POINT('Ctrl Pts',(2.76488627843076,6.17918207037036,42.6688945912086));
#194302=CARTESIAN_POINT('Ctrl Pts',(2.5930786664671,6.25045854553994,42.6776440391109));
#194303=CARTESIAN_POINT('Ctrl Pts',(2.42127244185385,6.32173444515034,42.6863934163612));
#194304=CARTESIAN_POINT('Ctrl Pts',(2.24652594672474,6.38592262741835,42.6951427936115));
#194305=CARTESIAN_POINT('Ctrl Pts',(2.06943269687131,6.44280508110559,42.7038921708618));
#194306=CARTESIAN_POINT('Ctrl Pts',(1.89234081822081,6.49968709436165,42.7126414803672));
#194307=CARTESIAN_POINT('Ctrl Pts',(1.71290249405587,6.54926340459545,42.7213907898725));
#194308=CARTESIAN_POINT('Ctrl Pts',(1.53172716625051,6.59136563150385,42.7301400993779));
#194309=CARTESIAN_POINT('Ctrl Pts',(1.35055318107338,6.63346754640709,42.7388893440451));
#194310=CARTESIAN_POINT('Ctrl Pts',(1.16764249714434,6.66809542395773,42.7476385887123));
#194311=CARTESIAN_POINT('Ctrl Pts',(0.983616340614606,6.69513165624665,
42.7563878333796));
#194312=CARTESIAN_POINT('Ctrl Pts',(0.79959148671406,6.72216769715958,42.7651370161153));
#194313=CARTESIAN_POINT('Ctrl Pts',(0.614451459526898,6.74161215869369,
42.773886198851));
#194314=CARTESIAN_POINT('Ctrl Pts',(0.428825047910436,6.75339900185711,
42.7826353815867));
#194315=CARTESIAN_POINT('Ctrl Pts',(0.24319988859717,6.7651857655022,42.7913845052972));
#194316=CARTESIAN_POINT('Ctrl Pts',(0.0570886373920126,6.76931499599834,
42.8001336290077));
#194317=CARTESIAN_POINT('Ctrl Pts',(-0.128876626811083,6.76577266947847,
42.8088827527183));
#194318=CARTESIAN_POINT('Ctrl Pts',(-0.31484069818794,6.76223036567994,
42.8176318203098));
#194319=CARTESIAN_POINT('Ctrl Pts',(-0.500658497950882,6.75101660879225,
42.8263808879014));
#194320=CARTESIAN_POINT('Ctrl Pts',(-0.685698951925696,6.73216948296224,
42.8351299554929));
#194321=CARTESIAN_POINT('Ctrl Pts',(-0.870738280459434,6.71332247176299,
42.8438789698714));
#194322=CARTESIAN_POINT('Ctrl Pts',(-1.05499998761219,6.68684221356192,
42.8526279842499));
#194323=CARTESIAN_POINT('Ctrl Pts',(-1.23785829161398,6.65281863948526,
42.8613769986285));
#194324=CARTESIAN_POINT('Ctrl Pts',(-1.43007412917385,6.61705395368865,
42.8705737323277));
#194325=CARTESIAN_POINT('Ctrl Pts',(-1.62073882535776,6.57295372727794,
42.8797704660269));
#194326=CARTESIAN_POINT('Ctrl Pts',(-1.809136960915,6.52068343478283,42.8889671997261));
#194327=CARTESIAN_POINT('Ctrl Pts',(-1.98838356186096,6.47095219815204,
42.8977171974397));
#194328=CARTESIAN_POINT('Ctrl Pts',(-2.16557827572514,6.41382586850897,
42.9064671951534));
#194329=CARTESIAN_POINT('Ctrl Pts',(-2.34011918621678,6.34949849943286,
42.9152171928671));
#194330=CARTESIAN_POINT('Ctrl Pts',(-2.51465655691076,6.28517243495559,
42.9239670131254));
#194331=CARTESIAN_POINT('Ctrl Pts',(-2.68653996295306,6.21364572242384,
42.9327168333837));
#194332=CARTESIAN_POINT('Ctrl Pts',(-2.85518555379966,6.13516132252231,
42.941466653642));
#194333=CARTESIAN_POINT('Ctrl Pts',(-3.02382794858666,6.05667841000518,
42.9502163080795));
#194334=CARTESIAN_POINT('Ctrl Pts',(-3.18923239109257,5.97123819492094,
42.958965962517));
#194335=CARTESIAN_POINT('Ctrl Pts',(-3.35083705967673,5.87913088810727,
42.9677156169545));
#194336=CARTESIAN_POINT('Ctrl Pts',(-3.51243888042371,5.78702520443121,
42.9764651172035));
#194337=CARTESIAN_POINT('Ctrl Pts',(-3.67024081223657,5.68825280605804,
42.9852146174524));
#194338=CARTESIAN_POINT('Ctrl Pts',(-3.82370687544365,5.5831491768253,42.9939641177013));
#194339=CARTESIAN_POINT('Ctrl Pts',(-3.97717043817782,5.47804726008046,
43.0027134753918));
#194340=CARTESIAN_POINT('Ctrl Pts',(-4.1262980372243,5.3666144808426,43.0114628330823));
#194341=CARTESIAN_POINT('Ctrl Pts',(-4.27058317206879,5.24922931204599,
43.0202121907727));
#194342=CARTESIAN_POINT('Ctrl Pts',(-4.41486614774799,5.13184589986821,
43.0289614175328));
#194343=CARTESIAN_POINT('Ctrl Pts',(-4.5543065819437,5.00851045723074,43.0377106442929));
#194344=CARTESIAN_POINT('Ctrl Pts',(-4.68843089001795,4.87964187103167,
43.0464598710529));
#194345=CARTESIAN_POINT('Ctrl Pts',(-4.82255336917797,4.75077504208001,
43.0552089785089));
#194346=CARTESIAN_POINT('Ctrl Pts',(-4.95135966065106,4.61637541908125,
43.0639580859648));
#194347=CARTESIAN_POINT('Ctrl Pts',(-5.07441230869225,4.47689945401866,
43.0727071934207));
#194348=CARTESIAN_POINT('Ctrl Pts',(-5.19746344226398,4.33742520555538,
43.0814561931971));
#194349=CARTESIAN_POINT('Ctrl Pts',(-5.31476088454749,4.1928749549136,43.0902051929735));
#194350=CARTESIAN_POINT('Ctrl Pts',(-5.42590627628836,4.0437396158673,43.0989541927498));
#194351=CARTESIAN_POINT('Ctrl Pts',(-5.5370638067265,3.89458798906759,43.1077041480445));
#194352=CARTESIAN_POINT('Ctrl Pts',(-5.64206777071846,3.7408505015531,43.1164541033392));
#194353=CARTESIAN_POINT('Ctrl Pts',(-5.74056148163991,3.58304938223188,
43.1252040586339));
#194354=CARTESIAN_POINT('Ctrl Pts',(-5.83905138951862,3.42525435593318,
43.133953676075));
#194355=CARTESIAN_POINT('Ctrl Pts',(-5.93103139557628,3.26339625497228,
43.1427032935161));
#194356=CARTESIAN_POINT('Ctrl Pts',(-6.01618907820819,3.09802485065058,
43.1514529109572));
#194357=CARTESIAN_POINT('Ctrl Pts',(-6.10134392544964,2.93265895249682,
43.1602022370731));
#194358=CARTESIAN_POINT('Ctrl Pts',(-6.17967677261819,2.76378023986065,
43.168951563189));
#194359=CARTESIAN_POINT('Ctrl Pts',(-6.25092157009217,2.59196229227133,
43.1777008893049));
#194360=CARTESIAN_POINT('Ctrl Pts',(-6.32216437407745,2.42014915229113,
43.1864499706073));
#194361=CARTESIAN_POINT('Ctrl Pts',(-6.38631941548912,2.24539720662877,
43.1951990519098));
#194362=CARTESIAN_POINT('Ctrl Pts',(-6.44316881037528,2.06829994947717,
43.2039481332122));
#194363=CARTESIAN_POINT('Ctrl Pts',(-6.50002334524563,1.89118668024481,
43.2126980055546));
#194364=CARTESIAN_POINT('Ctrl Pts',(-6.54957082411088,1.71172794807733,
43.2214478778969));
#194365=CARTESIAN_POINT('Ctrl Pts',(-6.59164294296077,1.5305333425037,43.2301977502393));
#194366=CARTESIAN_POINT('Ctrl Pts',(-6.63371214082125,1.34935131693641,
43.2389470150942));
#194367=CARTESIAN_POINT('Ctrl Pts',(-6.6683069523968,1.16643393829817,43.2476962799491));
#194368=CARTESIAN_POINT('Ctrl Pts',(-6.69530988153979,0.982402458341639,
43.256445544804));
#194369=CARTESIAN_POINT('Ctrl Pts',(-6.72231419690474,0.798361530947818,
43.265195258811));
#194370=CARTESIAN_POINT('Ctrl Pts',(-6.7417258082927,0.613206671363342,
43.273944972818));
#194371=CARTESIAN_POINT('Ctrl Pts',(-6.75347878028173,0.427566795114374,
43.282694686825));
#194372=CARTESIAN_POINT('Ctrl Pts',(-6.76248992368216,0.285234494205584,
43.2894031966133));
#194373=CARTESIAN_POINT('Ctrl Pts',(-6.76699999999999,0.142617266091775,
43.2961117064016));
#194374=CARTESIAN_POINT('Ctrl Pts',(-6.767,4.16769702918876E-13,43.3028202161899));
#194375=CARTESIAN_POINT('Ctrl Pts',(-6.76699999999983,1.53523534223817E-6,
43.3028542630209));
#194376=CARTESIAN_POINT('Ctrl Pts',(-6.76700004292237,-0.189192154842816,
43.3117861533015));
#194377=CARTESIAN_POINT('Ctrl Pts',(-6.7590614542694,-0.378469857747368,
43.320718043582));
#194378=CARTESIAN_POINT('Ctrl Pts',(-6.74318913218751,-0.567176628175301,
43.3296499338625));
#194379=CARTESIAN_POINT('Ctrl Pts',(-6.72733425191513,-0.755676032124229,
43.3385720090493));
#194380=CARTESIAN_POINT('Ctrl Pts',(-6.70356305940782,-0.943605498803956,
43.3474940842361));
#194381=CARTESIAN_POINT('Ctrl Pts',(-6.67193243972188,-1.13031257614295,
43.3564161594229));
#194382=CARTESIAN_POINT('Ctrl Pts',(-6.64035725344944,-1.31669244488702,
43.3653225984607));
#194383=CARTESIAN_POINT('Ctrl Pts',(-6.6009501808069,-1.50185394688418,
43.3742290374985));
#194384=CARTESIAN_POINT('Ctrl Pts',(-6.55381956237659,-1.68515226131347,
43.3831354765363));
#194385=CARTESIAN_POINT('Ctrl Pts',(-6.5067453619389,-1.86823115738388,
43.3920312540672));
#194386=CARTESIAN_POINT('Ctrl Pts',(-6.45196612552911,-2.04945106631216,
43.4009270315981));
#194387=CARTESIAN_POINT('Ctrl Pts',(-6.38964113496009,-2.22817754373972,
43.409822809129));
#194388=CARTESIAN_POINT('Ctrl Pts',(-6.32742899935208,-2.40658039224321,
43.418702478633));
#194389=CARTESIAN_POINT('Ctrl Pts',(-6.25769846414383,-2.58249857695067,
43.427582148137));
#194390=CARTESIAN_POINT('Ctrl Pts',(-6.18065849880635,-2.75531296246594,
43.436461817641));
#194391=CARTESIAN_POINT('Ctrl Pts',(-6.15069230357275,-2.82253248408489,
43.4399157380679));
#194392=CARTESIAN_POINT('Ctrl Pts',(-6.11962074893652,-2.88928255697687,
43.4433696584948));
#194393=CARTESIAN_POINT('Ctrl Pts',(-6.08745817512892,-2.95552735836705,
43.4468235789217));
#194394=CARTESIAN_POINT('Ctrl Pts',(-6.01183187788457,-3.11129378025841,
43.4549450437778));
#194395=CARTESIAN_POINT('Ctrl Pts',(-5.9301986729754,-3.26420576152668,
43.463066508634));
#194396=CARTESIAN_POINT('Ctrl Pts',(-5.8428117574739,-3.41377207304834,
43.4711879734902));
#194397=CARTESIAN_POINT('Ctrl Pts',(-5.75543107394573,-3.56332771829053,
43.4793088591664));
#194398=CARTESIAN_POINT('Ctrl Pts',(-5.66229768186461,-3.70953785285899,
43.4874297448425));
#194399=CARTESIAN_POINT('Ctrl Pts',(-5.56370996621465,-3.85193722844023,
43.4955506305187));
#194400=CARTESIAN_POINT('Ctrl Pts',(-5.46511046651363,-3.99435362481866,
43.503672486873));
#194401=CARTESIAN_POINT('Ctrl Pts',(-5.36105555449261,-4.13295805483247,
43.5117943432272));
#194402=CARTESIAN_POINT('Ctrl Pts',(-5.25188600112966,-4.26731560013298,
43.5199161995814));
#194403=CARTESIAN_POINT('Ctrl Pts',(-5.14263679901109,-4.40177117103644,
43.5280439815416));
#194404=CARTESIAN_POINT('Ctrl Pts',(-5.02826573372788,-4.53197338423848,
43.5361717635017));
#194405=CARTESIAN_POINT('Ctrl Pts',(-4.9091532175445,-4.65752119551511,
43.5442995454619));
#194406=CARTESIAN_POINT('Ctrl Pts',(-4.78999217934918,-4.78312015030373,
43.5524306383783));
#194407=CARTESIAN_POINT('Ctrl Pts',(-4.66608610211582,-4.90406066824777,
43.5605617312947));
#194408=CARTESIAN_POINT('Ctrl Pts',(-4.53785086875385,-5.01997992953657,
43.5686928242112));
#194409=CARTESIAN_POINT('Ctrl Pts',(-4.40947567199396,-5.13602571185449,
43.5768327918757));
#194410=CARTESIAN_POINT('Ctrl Pts',(-4.27676216205594,-5.24703905648351,
43.5849727595403));
#194411=CARTESIAN_POINT('Ctrl Pts',(-4.14015835320787,-5.35269818039119,
43.5931127272048));
#194412=CARTESIAN_POINT('Ctrl Pts',(-4.06930971156866,-5.40749757045778,
43.5973344663853));
#194413=CARTESIAN_POINT('Ctrl Pts',(-3.9974150918705,-5.46085743637847,
43.6015562055658));
#194414=CARTESIAN_POINT('Ctrl Pts',(-3.92453983276044,-5.51273762309405,
43.6057779447463));
#194415=CARTESIAN_POINT('Ctrl Pts',(-3.77884574203878,-5.61645782556472,
43.6142181542039));
#194416=CARTESIAN_POINT('Ctrl Pts',(-3.62892939749098,-5.71447561839207,
43.6226583636615));
#194417=CARTESIAN_POINT('Ctrl Pts',(-3.47526558528633,-5.80644625495875,
43.6310985731191));
#194418=CARTESIAN_POINT('Ctrl Pts',(-3.32171819618477,-5.89834721014274,
43.6395323878677));
#194419=CARTESIAN_POINT('Ctrl Pts',(-3.16442928442298,-5.98420997156264,
43.6479662026162));
#194420=CARTESIAN_POINT('Ctrl Pts',(-3.00390273054915,-6.0637329579558,
43.6564000173647));
#194421=CARTESIAN_POINT('Ctrl Pts',(-2.84347312207337,-6.14320791872712,
43.6648287387533));
#194422=CARTESIAN_POINT('Ctrl Pts',(-2.67981006769599,-6.21635058991948,
43.6732574601418));
#194423=CARTESIAN_POINT('Ctrl Pts',(-2.51344251891016,-6.2829050370139,
43.6816861815304));
#194424=CARTESIAN_POINT('Ctrl Pts',(-2.34714989596315,-6.34942951042767,
43.6901111069321));
#194425=CARTESIAN_POINT('Ctrl Pts',(-2.17815551628463,-6.40937155213659,
43.6985360323338));
#194426=CARTESIAN_POINT('Ctrl Pts',(-2.00700916747056,-6.46252297494478,
43.7069609577356));
#194427=CARTESIAN_POINT('Ctrl Pts',(-1.83591363777016,-6.51565861530587,
43.7153833814933));
#194428=CARTESIAN_POINT('Ctrl Pts',(-1.66266773136378,-6.56200755903514,
43.723805805251));
#194429=CARTESIAN_POINT('Ctrl Pts',(-1.48783766182772,-6.60141106825253,
43.7322282290087));
#194430=CARTESIAN_POINT('Ctrl Pts',(-1.31300484271726,-6.64081519717385,
43.7406507852269));
#194431=CARTESIAN_POINT('Ctrl Pts',(-1.13658813447718,-6.67327359354366,
43.7490733414451));
#194432=CARTESIAN_POINT('Ctrl Pts',(-0.959165905965437,-6.69867821027653,
43.7574958976634));
#194433=CARTESIAN_POINT('Ctrl Pts',(-0.781737684097593,-6.7240836851821,
43.7659187383971));
#194434=CARTESIAN_POINT('Ctrl Pts',(-0.603304204417205,-6.74243485789718,
43.7743415791308));
#194435=CARTESIAN_POINT('Ctrl Pts',(-0.424451113328692,-6.7536753144043,
43.7827644198646));
#194436=CARTESIAN_POINT('Ctrl Pts',(-0.245567010679107,-6.76491771990823,
43.7911887210452));
#194437=CARTESIAN_POINT('Ctrl Pts',(-0.0662634844669385,-6.76904693017065,
43.7996130222259));
#194438=CARTESIAN_POINT('Ctrl Pts',(0.112871275286189,-6.76605860713719,
43.8080373234065));
#194439=CARTESIAN_POINT('Ctrl Pts',(0.292062112296732,-6.76306934862388,
43.8164642617733));
#194440=CARTESIAN_POINT('Ctrl Pts',(0.471083744130887,-6.75295812013209,
43.82489120014));
#194441=CARTESIAN_POINT('Ctrl Pts',(0.649350191357576,-6.73577266013216,
43.8333181385068));
#194442=CARTESIAN_POINT('Ctrl Pts',(0.827776922528825,-6.71857174824345,
43.8417526537504));
#194443=CARTESIAN_POINT('Ctrl Pts',(1.00544677998836,-6.69428392735286,
43.8501871689941));
#194444=CARTESIAN_POINT('Ctrl Pts',(1.18177995471074,-6.66300871518595,
43.8586216842377));
#194445=CARTESIAN_POINT('Ctrl Pts',(1.358198299867,-6.63171839682365,43.8670602734245));
#194446=CARTESIAN_POINT('Ctrl Pts',(1.53327834788571,-6.59343402240147,
43.8754988626113));
#194447=CARTESIAN_POINT('Ctrl Pts',(1.70645211213654,-6.54830590221507,
43.883937451798));
#194448=CARTESIAN_POINT('Ctrl Pts',(1.87981944547621,-6.50312733900029,
43.8923854734183));
#194449=CARTESIAN_POINT('Ctrl Pts',(2.05127591668672,-6.45108983649194,
43.9008334950386));
#194450=CARTESIAN_POINT('Ctrl Pts',(2.22026911063925,-6.39239345443796,
43.9092815166589));
#194451=CARTESIAN_POINT('Ctrl Pts',(2.31632213002314,-6.35903137285744,
43.9140832365712));
#194452=CARTESIAN_POINT('Ctrl Pts',(2.41157970716454,-6.32351896044428,
43.9188849564835));
#194453=CARTESIAN_POINT('Ctrl Pts',(2.50594349886653,-6.28589979084049,
43.9236866763959));
#194454=CARTESIAN_POINT('Ctrl Pts',(2.66786745142743,-6.22134701562412,
43.9319262082467));
#194455=CARTESIAN_POINT('Ctrl Pts',(2.82751985065107,-6.1504440960898,43.9401657400975));
#194456=CARTESIAN_POINT('Ctrl Pts',(2.98436927829437,-6.07337048192952,
43.9484052719484));
#194457=CARTESIAN_POINT('Ctrl Pts',(3.14104461403513,-5.9963824140943,43.9566356584947));
#194458=CARTESIAN_POINT('Ctrl Pts',(3.29492285631175,-5.91323744479937,
43.964866045041));
#194459=CARTESIAN_POINT('Ctrl Pts',(3.44549045535073,-5.82416384746231,
43.9730964315874));
#194460=CARTESIAN_POINT('Ctrl Pts',(3.59591779475377,-5.73517322568185,
43.9813191512051));
#194461=CARTESIAN_POINT('Ctrl Pts',(3.74304032822838,-5.64026515465837,
43.9895418708229));
#194462=CARTESIAN_POINT('Ctrl Pts',(3.88636703173365,-5.53971482069734,
43.9977645904408));
#194463=CARTESIAN_POINT('Ctrl Pts',(4.02956673745311,-5.43925358157673,
44.0059800241365));
#194464=CARTESIAN_POINT('Ctrl Pts',(4.16897702648647,-5.33316024751826,
44.0141954578323));
#194465=CARTESIAN_POINT('Ctrl Pts',(4.30413402933039,-5.2217544233294,44.0224108915281));
#194466=CARTESIAN_POINT('Ctrl Pts',(4.43922157196963,-5.11040585308364,
44.0306221031289));
#194467=CARTESIAN_POINT('Ctrl Pts',(4.57005990778635,-4.9937504559764,44.0388333147297));
#194468=CARTESIAN_POINT('Ctrl Pts',(4.69621623288276,-4.87214963789173,
44.0470445263305));
#194469=CARTESIAN_POINT('Ctrl Pts',(4.8223302521095,-4.75058959801106,44.055252984344));
#194470=CARTESIAN_POINT('Ctrl Pts',(4.94376513239408,-4.62408768760204,
44.0634614423575));
#194471=CARTESIAN_POINT('Ctrl Pts',(5.0601230393961,-4.4930439377078,44.0716699003711));
#194472=CARTESIAN_POINT('Ctrl Pts',(5.11196302773182,-4.43466108568667,
44.0753269476542));
#194473=CARTESIAN_POINT('Ctrl Pts',(5.16279577137245,-4.3753772209428,44.0789839949374));
#194474=CARTESIAN_POINT('Ctrl Pts',(5.2125885036707,-4.31523001604782,44.0826410422206));
#194475=CARTESIAN_POINT('Ctrl Pts',(5.33320972475314,-4.16952543298392,
44.0915001163965));
#194476=CARTESIAN_POINT('Ctrl Pts',(5.44759988295617,-4.01890384442965,
44.1003591905724));
#194477=CARTESIAN_POINT('Ctrl Pts',(5.55540062721881,-3.86391160239165,
44.1092182647483));
#194478=CARTESIAN_POINT('Ctrl Pts',(5.66340390738988,-3.70862816111607,
44.1180939833421));
#194479=CARTESIAN_POINT('Ctrl Pts',(5.7647928845205,-3.54895786881008,44.1269697019359));
#194480=CARTESIAN_POINT('Ctrl Pts',(5.85925393477225,-3.3854737228128,44.1358454205297));
#194481=CARTESIAN_POINT('Ctrl Pts',(5.95398455017322,-3.22152303925221,
44.1447464679167));
#194482=CARTESIAN_POINT('Ctrl Pts',(6.04174754497938,-3.05373694815608,
44.1536475153037));
#194483=CARTESIAN_POINT('Ctrl Pts',(6.12227510881517,-2.88271339053715,
44.1625485626907));
#194484=CARTESIAN_POINT('Ctrl Pts',(6.2029121509786,-2.7114573240457,44.1714617111737));
#194485=CARTESIAN_POINT('Ctrl Pts',(6.27629400830026,-2.53695523627329,
44.1803748596567));
#194486=CARTESIAN_POINT('Ctrl Pts',(6.34220155888343,-2.35982380412112,
44.1892880081397));
#194487=CARTESIAN_POINT('Ctrl Pts',(6.40825544225084,-2.18229909175425,
44.1982209462496));
#194488=CARTESIAN_POINT('Ctrl Pts',(6.46680173505636,-2.0021336021734,44.2071538843595));
#194489=CARTESIAN_POINT('Ctrl Pts',(6.51767076636749,-1.81996065376112,
44.2160868224694));
#194490=CARTESIAN_POINT('Ctrl Pts',(6.5660907084741,-1.64655842084732,44.2245896843281));
#194491=CARTESIAN_POINT('Ctrl Pts',(6.60755518447319,-1.47133765518869,
44.2330925461867));
#194492=CARTESIAN_POINT('Ctrl Pts',(6.64196113402503,-1.29485184252906,
44.2415954080454));
#194493=CARTESIAN_POINT('Ctrl Pts',(6.67523353421345,-1.1241805876189,44.2498181319113));
#194494=CARTESIAN_POINT('Ctrl Pts',(6.70196764817162,-0.951998966731906,
44.2580408557772));
#194495=CARTESIAN_POINT('Ctrl Pts',(6.72202969380216,-0.778849019799167,
44.266263579643));
#194496=CARTESIAN_POINT('Ctrl Pts',(6.74207050443702,-0.605882346219521,
44.2744776000343));
#194497=CARTESIAN_POINT('Ctrl Pts',(6.75545326882495,-0.431949740957379,
44.2826916204255));
#194498=CARTESIAN_POINT('Ctrl Pts',(6.76209501746225,-0.257604298900969,
44.2909056408167));
#194499=CARTESIAN_POINT('Ctrl Pts',(6.76873106950894,-0.0834083919538031,
44.2991126160886));
#194500=CARTESIAN_POINT('Ctrl Pts',(6.76863760704288,0.091199290158767,
44.3073195913606));
#194501=CARTESIAN_POINT('Ctrl Pts',(6.76178334459151,0.265659558090598,
44.3155265666325));
#194502=CARTESIAN_POINT('Ctrl Pts',(6.75493358525376,0.440005209108513,
44.3237281500855));
#194503=CARTESIAN_POINT('Ctrl Pts',(6.74133188731707,0.614203281693499,
44.3319297335385));
#194504=CARTESIAN_POINT('Ctrl Pts',(6.72099902742316,0.787693514875522,
44.3401313169915));
#194505=CARTESIAN_POINT('Ctrl Pts',(6.70067544555053,0.96110458329256,44.3483291580066));
#194506=CARTESIAN_POINT('Ctrl Pts',(6.67362686251875,1.13380810023515,44.3565269990216));
#194507=CARTESIAN_POINT('Ctrl Pts',(6.6399259981915,1.30524776902343,44.3647248400367));
#194508=CARTESIAN_POINT('Ctrl Pts',(6.60622810786051,1.47667230879515,44.3729219576178));
#194509=CARTESIAN_POINT('Ctrl Pts',(6.56587916626638,1.64683286919032,44.381119075199));
#194510=CARTESIAN_POINT('Ctrl Pts',(6.51900328847673,1.81518184346075,44.3893161927801));
#194511=CARTESIAN_POINT('Ctrl Pts',(6.47212793223347,1.98352894466121,44.3975132191592));
#194512=CARTESIAN_POINT('Ctrl Pts',(6.41872587965452,2.15006415391288,44.4057102455383));
#194513=CARTESIAN_POINT('Ctrl Pts',(6.35897152769573,2.31425368314605,44.4139072719174));
#194514=CARTESIAN_POINT('Ctrl Pts',(6.29920697541654,2.47847124022572,44.4221056975635));
#194515=CARTESIAN_POINT('Ctrl Pts',(6.23308808610291,2.64034198233027,44.4303041232096));
#194516=CARTESIAN_POINT('Ctrl Pts',(6.16083795604542,2.79935076032821,44.4385025488557));
#194517=CARTESIAN_POINT('Ctrl Pts',(6.08856235517795,2.95841559472862,44.4467038647464));
#194518=CARTESIAN_POINT('Ctrl Pts',(6.01015135621422,3.11461612869953,44.454905180637));
#194519=CARTESIAN_POINT('Ctrl Pts',(5.92587469883682,3.26746048999611,44.4631064965276));
#194520=CARTESIAN_POINT('Ctrl Pts',(5.8415020644539,3.4204789154353,44.4713171523442));
#194521=CARTESIAN_POINT('Ctrl Pts',(5.75125059964335,3.5701332177307,44.4795278081608));
#194522=CARTESIAN_POINT('Ctrl Pts',(5.6554347609124,3.71595837773565,44.4877384639774));
#194523=CARTESIAN_POINT('Ctrl Pts',(5.55956246022919,3.8618694689742,44.4959539581345));
#194524=CARTESIAN_POINT('Ctrl Pts',(5.45811945770854,4.00394662854382,44.5041694522917));
#194525=CARTESIAN_POINT('Ctrl Pts',(5.35146136878129,4.14175689996908,44.5123849464488));
#194526=CARTESIAN_POINT('Ctrl Pts',(5.24463779786639,4.2797809865664,44.5206131870963));
#194527=CARTESIAN_POINT('Ctrl Pts',(5.13258320123164,4.41352468047039,44.5288414277438));
#194528=CARTESIAN_POINT('Ctrl Pts',(5.01569191202018,4.54258997089715,44.5370696683913));
#194529=CARTESIAN_POINT('Ctrl Pts',(4.90945639194587,4.6598897144839,44.5445478254925));
#194530=CARTESIAN_POINT('Ctrl Pts',(4.79922641205564,4.77332546969481,44.5520259825937));
#194531=CARTESIAN_POINT('Ctrl Pts',(4.68532166476138,4.88262735601619,44.5595041396948));
#194532=CARTESIAN_POINT('Ctrl Pts',(4.56242623825974,5.0005566105555,44.5675725593896));
#194533=CARTESIAN_POINT('Ctrl Pts',(4.43485019286915,5.11405902250298,44.5756409790844));
#194534=CARTESIAN_POINT('Ctrl Pts',(4.30295035589384,5.22272986422934,44.5837093987791));
#194535=CARTESIAN_POINT('Ctrl Pts',(4.17119502834896,5.33128164620703,44.5917689787152));
#194536=CARTESIAN_POINT('Ctrl Pts',(4.03512561300381,5.4350121496199,44.5998285586512));
#194537=CARTESIAN_POINT('Ctrl Pts',(3.89513727967132,5.53355171409058,44.6078881385873));
#194538=CARTESIAN_POINT('Ctrl Pts',(3.7553109589693,5.6319772358145,44.6159383909335));
#194539=CARTESIAN_POINT('Ctrl Pts',(3.61157505317701,5.72522356704627,44.6239886432798));
#194540=CARTESIAN_POINT('Ctrl Pts',(3.46435904289281,5.81296012560957,44.6320388956261));
#194541=CARTESIAN_POINT('Ctrl Pts',(3.34482014189342,5.88420191356374,44.6385756732251));
#194542=CARTESIAN_POINT('Ctrl Pts',(3.22298741040076,5.95181155375775,44.6451124508241));
#194543=CARTESIAN_POINT('Ctrl Pts',(3.09910619832132,6.01563211736941,44.6516492284231));
#194544=CARTESIAN_POINT('Origin',(0.,0.,4.30282021618968));
#194545=CARTESIAN_POINT('',(3.09910619832128,6.01563211736943,47.0456420231655));
#194546=CARTESIAN_POINT('',(3.09910619832134,6.0156321173694,46.651350675134));
#194547=CARTESIAN_POINT('',(3.09910619832133,6.0156321173694,4.30282021618968));
#194548=CARTESIAN_POINT('',(-6.76699829542225,-0.00480309820322907,45.6971797838526));
#194549=CARTESIAN_POINT('Ctrl Pts',(-6.76699829542225,-0.00480309820322772,
45.6971797838526));
#194550=CARTESIAN_POINT('Ctrl Pts',(-6.76685365275678,-0.208587536770219,
45.7067503929135));
#194551=CARTESIAN_POINT('Ctrl Pts',(-6.75749973364958,-0.412056637524916,
45.7163210019745));
#194552=CARTESIAN_POINT('Ctrl Pts',(-6.73904578321651,-0.614451732613529,
45.7258916110354));
#194553=CARTESIAN_POINT('Ctrl Pts',(-6.72051194201249,-0.817723035766192,
45.7355036531401));
#194554=CARTESIAN_POINT('Ctrl Pts',(-6.69279918945737,-1.01991092176919,
45.7451156952449));
#194555=CARTESIAN_POINT('Ctrl Pts',(-6.65606837195544,-1.22026342559893,
45.7547277373496));
#194556=CARTESIAN_POINT('Ctrl Pts',(-6.61915583248788,-1.42160715296503,
45.7643873340502));
#194557=CARTESIAN_POINT('Ctrl Pts',(-6.57313583199955,-1.62109720207672,
45.7740469307509));
#194558=CARTESIAN_POINT('Ctrl Pts',(-6.51822114023457,-1.81798849473783,
45.7837065274516));
#194559=CARTESIAN_POINT('Ctrl Pts',(-6.47508857845154,-1.97263610491821,
45.791293625514));
#194560=CARTESIAN_POINT('Ctrl Pts',(-6.42646963323295,-2.1256808188579,
45.7988807235765));
#194561=CARTESIAN_POINT('Ctrl Pts',(-6.37248835238679,-2.27676990464447,
45.8064678216389));
#194562=CARTESIAN_POINT('Ctrl Pts',(-6.31398467118079,-2.44051681042375,
45.8146905455048));
#194563=CARTESIAN_POINT('Ctrl Pts',(-6.24908764947539,-2.6022251899042,
45.8229132693707));
#194564=CARTESIAN_POINT('Ctrl Pts',(-6.17795891737632,-2.76136064562572,
45.8311359932366));
#194565=CARTESIAN_POINT('Ctrl Pts',(-6.10690547263056,-2.92032766185836,
45.8393500136278));
#194566=CARTESIAN_POINT('Ctrl Pts',(-6.02963359751848,-3.07672685262557,
45.847564034019));
#194567=CARTESIAN_POINT('Ctrl Pts',(-5.94635425970498,-3.2300402502273,
45.8557780544103));
#194568=CARTESIAN_POINT('Ctrl Pts',(-5.86314635011295,-3.38322215178686,
45.8639850296822));
#194569=CARTESIAN_POINT('Ctrl Pts',(-5.77394140985738,-3.53332321781279,
45.8721920049542));
#194570=CARTESIAN_POINT('Ctrl Pts',(-5.67899796155401,-3.67984662080709,
45.8803989802261));
#194571=CARTESIAN_POINT('Ctrl Pts',(-5.58411688920132,-3.82627376084992,
45.8886005636791));
#194572=CARTESIAN_POINT('Ctrl Pts',(-5.48350501272984,-3.9691276197129,
45.8968021471321));
#194573=CARTESIAN_POINT('Ctrl Pts',(-5.3774661710349,-4.1079370223234,45.9050037305851));
#194574=CARTESIAN_POINT('Ctrl Pts',(-5.27147571557976,-4.24668308526578,
45.9132015716002));
#194575=CARTESIAN_POINT('Ctrl Pts',(-5.16006344573274,-4.38138808419242,
45.9213994126153));
#194576=CARTESIAN_POINT('Ctrl Pts',(-5.0435758439615,-4.51161076625722,
45.9295972536303));
#194577=CARTESIAN_POINT('Ctrl Pts',(-4.92709852185783,-4.64182195657645,
45.9377943712115));
#194578=CARTESIAN_POINT('Ctrl Pts',(-4.80554699253968,-4.76755134503546,
45.9459914887926));
#194579=CARTESIAN_POINT('Ctrl Pts',(-4.67930749869746,-4.88839138496845,
45.9541886063738));
#194580=CARTESIAN_POINT('Ctrl Pts',(-4.55306940941025,-5.00923008042137,
45.9623856327529));
#194581=CARTESIAN_POINT('Ctrl Pts',(-4.4221437179604,-5.12517928679488,
45.970582659132));
#194582=CARTESIAN_POINT('Ctrl Pts',(-4.2869528520441,-5.23586900565235,
45.9787796855111));
#194583=CARTESIAN_POINT('Ctrl Pts',(-4.1517389084755,-5.34657761971275,
45.9869781111572));
#194584=CARTESIAN_POINT('Ctrl Pts',(-4.01225861753204,-5.4520247302093,
45.9951765368034));
#194585=CARTESIAN_POINT('Ctrl Pts',(-3.86896677065171,-5.55188122419716,
46.0033749624495));
#194586=CARTESIAN_POINT('Ctrl Pts',(-3.72562440816134,-5.65177292124659,
46.0115762783402));
#194587=CARTESIAN_POINT('Ctrl Pts',(-3.578468107264,-5.74606987070758,46.0197775942309));
#194588=CARTESIAN_POINT('Ctrl Pts',(-3.42798088785504,-5.83448678398542,
46.0279789101215));
#194589=CARTESIAN_POINT('Ctrl Pts',(-3.27732228869389,-5.923004389327,46.0361895659381));
#194590=CARTESIAN_POINT('Ctrl Pts',(-3.12332550227137,-6.00562839835296,
46.0444002217547));
#194591=CARTESIAN_POINT('Ctrl Pts',(-2.96649829484811,-6.08211943870418,
46.0526108775713));
#194592=CARTESIAN_POINT('Ctrl Pts',(-2.80957867295087,-6.15865555337238,
46.0608263717285));
#194593=CARTESIAN_POINT('Ctrl Pts',(-2.64982563317626,-6.22905135093668,
46.0690418658856));
#194594=CARTESIAN_POINT('Ctrl Pts',(-2.4877659695276,-6.29311603904301,
46.0772573600428));
#194595=CARTESIAN_POINT('Ctrl Pts',(-2.3254548673288,-6.35728012469177,
46.0854856006903));
#194596=CARTESIAN_POINT('Ctrl Pts',(-2.1608303278032,-6.41509335217598,
46.0937138413378));
#194597=CARTESIAN_POINT('Ctrl Pts',(-1.99443460187551,-6.46641474225414,
46.1019420819853));
#194598=CARTESIAN_POINT('Ctrl Pts',(-1.84320745226529,-6.51305769231962,
46.1094202390864));
#194599=CARTESIAN_POINT('Ctrl Pts',(-1.69051766979617,-6.55433903623512,
46.1168983961874));
#194600=CARTESIAN_POINT('Ctrl Pts',(-1.53677791905916,-6.59018987795437,
46.1243765532884));
#194601=CARTESIAN_POINT('Ctrl Pts',(-1.3708849628497,-6.62887474694168,
46.132445862511));
#194602=CARTESIAN_POINT('Ctrl Pts',(-1.20322623801096,-6.66136239813277,
46.1405151717335));
#194603=CARTESIAN_POINT('Ctrl Pts',(-1.03431534275473,-6.68748688011739,
46.148584480956));
#194604=CARTESIAN_POINT('Ctrl Pts',(-0.865615125293458,-6.71357877777255,
46.1566437255568));
#194605=CARTESIAN_POINT('Ctrl Pts',(-0.69566620906036,-6.73332324163065,
46.1647029701575));
#194606=CARTESIAN_POINT('Ctrl Pts',(-0.524997028932897,-6.74660411759958,
46.1727622147583));
#194607=CARTESIAN_POINT('Ctrl Pts',(-0.354503266588588,-6.75987134317294,
46.1808131758786));
#194608=CARTESIAN_POINT('Ctrl Pts',(-0.183291082436059,-6.76668817269795,
46.1888641369989));
#194609=CARTESIAN_POINT('Ctrl Pts',(-0.0118986770931029,-6.76698953904049,
46.1969150981191));
#194610=CARTESIAN_POINT('Ctrl Pts',(0.159355122595911,-6.76729066166699,
46.2049595483982));
#194611=CARTESIAN_POINT('Ctrl Pts',(0.33078848215301,-6.761086807667,46.2130039986773));
#194612=CARTESIAN_POINT('Ctrl Pts',(0.501858614646054,-6.74836475977,46.2210484489564));
#194613=CARTESIAN_POINT('Ctrl Pts',(0.672827847761438,-6.73565021550145,
46.2290881545147));
#194614=CARTESIAN_POINT('Ctrl Pts',(0.843433909124399,-6.71642515822177,
46.2371278600729));
#194615=CARTESIAN_POINT('Ctrl Pts',(1.01313465791234,-6.69072844800451,
46.2451675656311));
#194616=CARTESIAN_POINT('Ctrl Pts',(1.1864983066362,-6.66447708803538,46.2533808039356));
#194617=CARTESIAN_POINT('Ctrl Pts',(1.3589167182694,-6.63147152425315,46.26159404224));
#194618=CARTESIAN_POINT('Ctrl Pts',(1.52981761192682,-6.59180908963833,
46.2698072805445));
#194619=CARTESIAN_POINT('Ctrl Pts',(1.69705378851112,-6.55299715731278,
46.2778443980927));
#194620=CARTESIAN_POINT('Ctrl Pts',(1.86283649359637,-6.50781105363439,
46.2858815156409));
#194621=CARTESIAN_POINT('Ctrl Pts',(2.02664048997135,-6.45639352304433,
46.293918633189));
#194622=CARTESIAN_POINT('Ctrl Pts',(2.19046181576765,-6.40497055280644,
46.3019566010132));
#194623=CARTESIAN_POINT('Ctrl Pts',(2.35230365951027,-6.34731495479433,
46.3099945688373));
#194624=CARTESIAN_POINT('Ctrl Pts',(2.51165695655697,-6.28361904737859,
46.3180325366614));
#194625=CARTESIAN_POINT('Ctrl Pts',(2.67105868593177,-6.21990378083351,
46.3260729474691));
#194626=CARTESIAN_POINT('Ctrl Pts',(2.827970016382,-6.15014468927429,46.3341133582769));
#194627=CARTESIAN_POINT('Ctrl Pts',(2.98190297929009,-6.07458176520005,
46.3421537690846));
#194628=CARTESIAN_POINT('Ctrl Pts',(3.14165374000358,-5.9961629887759,46.3504980620724));
#194629=CARTESIAN_POINT('Ctrl Pts',(3.29819620377378,-5.91149330051802,
46.3588423550602));
#194630=CARTESIAN_POINT('Ctrl Pts',(3.45101517644059,-5.82089196360633,
46.367186648048));
#194631=CARTESIAN_POINT('Ctrl Pts',(3.59852884358654,-5.73343596764627,
46.3752412582635));
#194632=CARTESIAN_POINT('Ctrl Pts',(3.74257294618498,-5.64045352622386,
46.3832958684791));
#194633=CARTESIAN_POINT('Ctrl Pts',(3.88271605159257,-5.54227435830322,
46.3913504786946));
#194634=CARTESIAN_POINT('Ctrl Pts',(4.02296524731073,-5.44402086736551,
46.3994111863639));
#194635=CARTESIAN_POINT('Ctrl Pts',(4.15930727032309,-5.34056304113514,
46.4074718940331));
#194636=CARTESIAN_POINT('Ctrl Pts',(4.29134539317149,-5.23226946138154,
46.4155326017024));
#194637=CARTESIAN_POINT('Ctrl Pts',(4.42356968186232,-5.12382319416866,
46.4236046744865));
#194638=CARTESIAN_POINT('Ctrl Pts',(4.55147768624772,-5.01052781545749,
46.4316767472706));
#194639=CARTESIAN_POINT('Ctrl Pts',(4.67471058271867,-4.89278754574711,
46.4397488200548));
#194640=CARTESIAN_POINT('Ctrl Pts',(4.68761829232993,-4.88045514705736,
46.4405943083492));
#194641=CARTESIAN_POINT('Ctrl Pts',(4.70047474908031,-4.86807401199892,
46.4414397966437));
#194642=CARTESIAN_POINT('Ctrl Pts',(4.71327956730438,-4.85564462460249,
46.4422852849381));
#194643=CARTESIAN_POINT('Ctrl Pts',(4.83948066645951,-4.73314367817709,
46.4506182069848));
#194644=CARTESIAN_POINT('Ctrl Pts',(4.96106501573664,-4.60556227232716,
46.4589511290316));
#194645=CARTESIAN_POINT('Ctrl Pts',(5.07760546832762,-4.47327751296625,
46.4672840510783));
#194646=CARTESIAN_POINT('Ctrl Pts',(5.19400819836504,-4.34114908211145,
46.4756071256319));
#194647=CARTESIAN_POINT('Ctrl Pts',(5.3053786777772,-4.20432862901411,46.4839302001855));
#194648=CARTESIAN_POINT('Ctrl Pts',(5.41132522199788,-4.06323126855581,
46.4922532747391));
#194649=CARTESIAN_POINT('Ctrl Pts',(5.51716601019195,-3.92227475173064,
46.5005680411851));
#194650=CARTESIAN_POINT('Ctrl Pts',(5.61759344235832,-3.77705010970675,
46.5088828076311));
#194651=CARTESIAN_POINT('Ctrl Pts',(5.71225474723509,-3.62800698768487,
46.517197574077));
#194652=CARTESIAN_POINT('Ctrl Pts',(5.80683892510071,-3.47908530124374,
46.5255055659166));
#194653=CARTESIAN_POINT('Ctrl Pts',(5.89566615120226,-3.32635162652708,
46.5338135577561));
#194654=CARTESIAN_POINT('Ctrl Pts',(5.97842566951192,-3.17028634576137,
46.5421215495957));
#194655=CARTESIAN_POINT('Ctrl Pts',(6.0611329306087,-3.01431960999408,46.5504242954828));
#194656=CARTESIAN_POINT('Ctrl Pts',(6.13777995680726,-2.85502576711637,
46.5587270413698));
#194657=CARTESIAN_POINT('Ctrl Pts',(6.20810073168352,-2.69291186362839,
46.5670297872569));
#194658=CARTESIAN_POINT('Ctrl Pts',(6.27839276870008,-2.53086421092651,
46.5753291400764));
#194659=CARTESIAN_POINT('Ctrl Pts',(6.34236356763179,-2.36599911268145,
46.5836284928958));
#194660=CARTESIAN_POINT('Ctrl Pts',(6.39979414854143,-2.19884602832825,
46.5919278457153));
#194661=CARTESIAN_POINT('Ctrl Pts',(6.45721251493014,-2.0317284946314,46.6002254334016));
#194662=CARTESIAN_POINT('Ctrl Pts',(6.50809332149035,-1.86232427311155,
46.608523021088));
#194663=CARTESIAN_POINT('Ctrl Pts',(6.55226653045999,-1.69118074545975,
46.6168206087743));
#194664=CARTESIAN_POINT('Ctrl Pts',(6.59643768502351,-1.5200451773454,46.6251178105567));
#194665=CARTESIAN_POINT('Ctrl Pts',(6.63390177686028,-1.34717080117684,
46.6334150123391));
#194666=CARTESIAN_POINT('Ctrl Pts',(6.66453919218751,-1.17311821902,46.6417122141216));
#194667=CARTESIAN_POINT('Ctrl Pts',(6.69518027358403,-0.999044809752956,
46.6500104087461));
#194668=CARTESIAN_POINT('Ctrl Pts',(6.71899299102571,-0.823793256288492,
46.6583086033706));
#194669=CARTESIAN_POINT('Ctrl Pts',(6.73590917402292,-0.647932557689332,
46.6666067979952));
#194670=CARTESIAN_POINT('Ctrl Pts',(6.75283725436887,-0.471948174210463,
46.6749108288368));
#194671=CARTESIAN_POINT('Ctrl Pts',(6.7628590748388,-0.295354136261364,
46.6832148596784));
#194672=CARTESIAN_POINT('Ctrl Pts',(6.76595844600158,-0.118723658046192,
46.6915188905199));
#194673=CARTESIAN_POINT('Ctrl Pts',(6.76905894418103,0.0579710478721898,
46.6998259409357));
#194674=CARTESIAN_POINT('Ctrl Pts',(6.76523197725446,0.234701872535052,
46.7081329913514));
#194675=CARTESIAN_POINT('Ctrl Pts',(6.75451349107595,0.41089718771603,46.7164400417672));
#194676=CARTESIAN_POINT('Ctrl Pts',(6.74378354502675,0.587280885425717,
46.7247559738218));
#194677=CARTESIAN_POINT('Ctrl Pts',(6.72614738650391,0.763127582691777,
46.7330719058764));
#194678=CARTESIAN_POINT('Ctrl Pts',(6.70169281114588,0.937871241181677,
46.7413878379311));
#194679=CARTESIAN_POINT('Ctrl Pts',(6.68325843280916,1.0695967226257,46.7476565641499));
#194680=CARTESIAN_POINT('Ctrl Pts',(6.66095058571782,1.20069552610051,46.7539252903687));
#194681=CARTESIAN_POINT('Ctrl Pts',(6.63482592046043,1.33092975216068,46.7601940165876));
#194682=CARTESIAN_POINT('Ctrl Pts',(6.59960976425492,1.5064860244823,46.7686442853109));
#194683=CARTESIAN_POINT('Ctrl Pts',(6.5573916916043,1.68079274914121,46.7770945540343));
#194684=CARTESIAN_POINT('Ctrl Pts',(6.50827738500053,1.85327129149801,46.7855448227576));
#194685=CARTESIAN_POINT('Ctrl Pts',(6.45920642343859,2.02559761568969,46.7939876338321));
#194686=CARTESIAN_POINT('Ctrl Pts',(6.40325144912586,2.19609865602286,46.8024304449066));
#194687=CARTESIAN_POINT('Ctrl Pts',(6.34056900696767,2.36420677350374,46.8108732559812));
#194688=CARTESIAN_POINT('Ctrl Pts',(6.27793334981569,2.53218941821985,46.8193097654989));
#194689=CARTESIAN_POINT('Ctrl Pts',(6.20858034987719,2.69778239076973,46.8277462750166));
#194690=CARTESIAN_POINT('Ctrl Pts',(6.1327162378131,2.86043362909605,46.8361827845343));
#194691=CARTESIAN_POINT('Ctrl Pts',(6.05690641060337,3.02296848170923,46.8446132572755));
#194692=CARTESIAN_POINT('Ctrl Pts',(5.97459490431643,3.18256549902456,46.8530437300167));
#194693=CARTESIAN_POINT('Ctrl Pts',(5.88603595655578,3.33869281577873,46.861474202758));
#194694=CARTESIAN_POINT('Ctrl Pts',(5.79751508004677,3.49475301382253,46.8699010512618));
#194695=CARTESIAN_POINT('Ctrl Pts',(5.70275227951128,3.64734619700503,46.8783278997656));
#194696=CARTESIAN_POINT('Ctrl Pts',(5.60204790286209,3.79596473825014,46.8867547482694));
#194697=CARTESIAN_POINT('Ctrl Pts',(5.50137461005746,3.94453740625928,46.8951789957061));
#194698=CARTESIAN_POINT('Ctrl Pts',(5.39476358425948,4.08913760474125,46.9036032431427));
#194699=CARTESIAN_POINT('Ctrl Pts',(5.28255889390558,4.22928605469281,46.9120274905793));
#194700=CARTESIAN_POINT('Ctrl Pts',(5.2509439051809,4.26877452572753,46.9144011211904));
#194701=CARTESIAN_POINT('Ctrl Pts',(5.21888509609938,4.30790975782307,46.9167747518014));
#194702=CARTESIAN_POINT('Ctrl Pts',(5.18639076284462,4.34668147614706,46.9191483824124));
#194703=CARTESIAN_POINT('Ctrl Pts',(5.068419892342,4.48744243054804,46.9277658624892));
#194704=CARTESIAN_POINT('Ctrl Pts',(4.94475829942727,4.62334654014516,46.9363833425661));
#194705=CARTESIAN_POINT('Ctrl Pts',(4.81583329022593,4.75394980208581,46.9450008226429));
#194706=CARTESIAN_POINT('Ctrl Pts',(4.68676484770896,4.88469836445349,46.9536278899499));
#194707=CARTESIAN_POINT('Ctrl Pts',(4.55242149739686,5.01013407351309,46.9622549572569));
#194708=CARTESIAN_POINT('Ctrl Pts',(4.41326701618101,5.12985021651595,46.9708820245639));
#194709=CARTESIAN_POINT('Ctrl Pts',(4.27403925901451,5.24962939963158,46.9795136347111));
#194710=CARTESIAN_POINT('Ctrl Pts',(4.12999554990547,5.36368281264469,46.9881452448582));
#194711=CARTESIAN_POINT('Ctrl Pts',(3.98163189657912,5.47164476552926,46.9967768550053));
#194712=CARTESIAN_POINT('Ctrl Pts',(3.83309584268652,5.57973217165925,47.0054184951998));
#194713=CARTESIAN_POINT('Ctrl Pts',(3.68023005886038,5.68171379226426,47.0140601353944));
#194714=CARTESIAN_POINT('Ctrl Pts',(3.52356004295536,5.77726696835869,47.0227017755889));
#194715=CARTESIAN_POINT('Ctrl Pts',(3.38492706465539,5.86181933986048,47.0303485247811));
#194716=CARTESIAN_POINT('Ctrl Pts',(3.24331589469917,5.9413388169842,47.0379952739733));
#194717=CARTESIAN_POINT('Ctrl Pts',(3.09910619832128,6.01563211736943,47.0456420231655));
#194718=CARTESIAN_POINT('Ctrl Pts',(3.09910619832133,6.01563211736941,45.0457774706169));
#194719=CARTESIAN_POINT('Ctrl Pts',(2.94511943075718,6.09496232515249,45.0538985576503));
#194720=CARTESIAN_POINT('Ctrl Pts',(2.78808765733465,6.16837455272572,45.0620196446837));
#194721=CARTESIAN_POINT('Ctrl Pts',(2.62851387184196,6.23563980883553,45.0701407317171));
#194722=CARTESIAN_POINT('Ctrl Pts',(2.4639351078096,6.30501481725996,45.0785165339357));
#194723=CARTESIAN_POINT('Ctrl Pts',(2.29665264882922,6.36785079448704,45.0868923361543));
#194724=CARTESIAN_POINT('Ctrl Pts',(2.12723915740466,6.42395069775635,45.0952681383728));
#194725=CARTESIAN_POINT('Ctrl Pts',(1.96281692221674,6.47839778701591,45.1033971729066));
#194726=CARTESIAN_POINT('Ctrl Pts',(1.79638781576152,6.52650003863257,45.1115262074403));
#194727=CARTESIAN_POINT('Ctrl Pts',(1.62848901668219,6.56812854034888,45.119655241974));
#194728=CARTESIAN_POINT('Ctrl Pts',(1.45294502964758,6.61165257509855,45.128154428035));
#194729=CARTESIAN_POINT('Ctrl Pts',(1.27579481701683,6.64809938942929,45.136653614096));
#194730=CARTESIAN_POINT('Ctrl Pts',(1.0976615919955,6.67738182444721,45.145152800157));
#194731=CARTESIAN_POINT('Ctrl Pts',(0.919528366974146,6.70666425946513,
45.153651986218));
#194732=CARTESIAN_POINT('Ctrl Pts',(0.740412585283084,6.72878231212951,
45.162151172279));
#194733=CARTESIAN_POINT('Ctrl Pts',(0.560940188315077,6.7437107815455,45.17065035834));
#194734=CARTESIAN_POINT('Ctrl Pts',(0.382713166174243,6.7585356609926,45.1790905677976));
#194735=CARTESIAN_POINT('Ctrl Pts',(0.203766007222725,6.76630176532737,
45.1875307772553));
#194736=CARTESIAN_POINT('Ctrl Pts',(0.0246829581155314,6.76695498371156,
45.1959709867129));
#194737=CARTESIAN_POINT('Ctrl Pts',(-0.154264409050907,6.76760770718604,
45.2044048014615));
#194738=CARTESIAN_POINT('Ctrl Pts',(-0.333347128852056,6.76115828623688,
45.21283861621));
#194739=CARTESIAN_POINT('Ctrl Pts',(-0.511977968558169,6.74760457938305,
45.2212724309585));
#194740=CARTESIAN_POINT('Ctrl Pts',(-0.69050092930322,6.73405905790087,
45.2297011523471));
#194741=CARTESIAN_POINT('Ctrl Pts',(-0.868572222323422,6.71341782926739,
45.2381298737356));
#194742=CARTESIAN_POINT('Ctrl Pts',(-1.04560635521803,6.68573080148518,
45.2465585951242));
#194743=CARTESIAN_POINT('Ctrl Pts',(-1.22256075843316,6.65805624292466,
45.2549835205258));
#194744=CARTESIAN_POINT('Ctrl Pts',(-1.39847860393442,6.62334226360043,
45.2634084459275));
#194745=CARTESIAN_POINT('Ctrl Pts',(-1.57278085347228,6.5816904657505,45.2718333713291));
#194746=CARTESIAN_POINT('Ctrl Pts',(-1.74703134680747,6.54005103572081,
45.2802557950869));
#194747=CARTESIAN_POINT('Ctrl Pts',(-1.91966687684997,6.49147797282548,
45.2886782188446));
#194748=CARTESIAN_POINT('Ctrl Pts',(-2.09011952060141,6.43612378606883,
45.2971006426024));
#194749=CARTESIAN_POINT('Ctrl Pts',(-2.26057484508011,6.38076872875086,
45.3055231988206));
#194750=CARTESIAN_POINT('Ctrl Pts',(-2.4288468955218,6.3186324311385,45.3139457550388));
#194751=CARTESIAN_POINT('Ctrl Pts',(-2.5943831703266,6.24991719669358,45.322368311257));
#194752=CARTESIAN_POINT('Ctrl Pts',(-2.75992503697877,6.18119964103476,
45.3307911519907));
#194753=CARTESIAN_POINT('Ctrl Pts',(-2.92273063557426,6.10590283315499,
45.3392139927244));
#194754=CARTESIAN_POINT('Ctrl Pts',(-3.08226756133981,6.02427719152367,
45.3476368334582));
#194755=CARTESIAN_POINT('Ctrl Pts',(-3.24183214941292,5.94263739672002,
45.3560611346388));
#194756=CARTESIAN_POINT('Ctrl Pts',(-3.39812663775679,5.85466673227387,
45.3644854358195));
#194757=CARTESIAN_POINT('Ctrl Pts',(-3.55064301529474,5.76066169618896,
45.3729097370002));
#194758=CARTESIAN_POINT('Ctrl Pts',(-3.70320713733692,5.6666272322884,45.381336675367));
#194759=CARTESIAN_POINT('Ctrl Pts',(-3.85199050670598,5.56655480548695,
45.3897636137339));
#194760=CARTESIAN_POINT('Ctrl Pts',(-3.99651359455045,5.4607845671271,45.3981905521007));
#194761=CARTESIAN_POINT('Ctrl Pts',(-4.14116662681661,5.35491922802825,
45.4066250673444));
#194762=CARTESIAN_POINT('Ctrl Pts',(-4.28155145412046,5.2433460378963,45.415059582588));
#194763=CARTESIAN_POINT('Ctrl Pts',(-4.4172202832284,5.12644652458558,45.4234940978317));
#194764=CARTESIAN_POINT('Ctrl Pts',(-4.55295464154302,5.00949054780852,
45.4319326870184));
#194765=CARTESIAN_POINT('Ctrl Pts',(-4.68396821151621,4.88720334070131,
45.4403712762052));
#194766=CARTESIAN_POINT('Ctrl Pts',(-4.80984929216416,4.76000407422808,
45.448809865392));
#194767=CARTESIAN_POINT('Ctrl Pts',(-4.93587107938033,4.63266262775311,
45.4572578870122));
#194768=CARTESIAN_POINT('Ctrl Pts',(-5.05674868504748,4.50039839360241,
45.4657059086325));
#194769=CARTESIAN_POINT('Ctrl Pts',(-5.17210919192994,4.36366537520395,
45.4741539302528));
#194770=CARTESIAN_POINT('Ctrl Pts',(-5.2376782526968,4.28594852188482,45.478955650165));
#194771=CARTESIAN_POINT('Ctrl Pts',(-5.30146570808013,4.20678857005627,
45.4837573700773));
#194772=CARTESIAN_POINT('Ctrl Pts',(-5.36340923190965,4.12627318667418,
45.4885590899895));
#194773=CARTESIAN_POINT('Ctrl Pts',(-5.4697014869505,3.98811246968441,45.4967986218403));
#194774=CARTESIAN_POINT('Ctrl Pts',(-5.57079909755088,3.84565059511103,
45.5050381536911));
#194775=CARTESIAN_POINT('Ctrl Pts',(-5.66633668219299,3.69931312597813,
45.5132776855419));
#194776=CARTESIAN_POINT('Ctrl Pts',(-5.76176822679321,3.55313808120856,
45.5215080720881));
#194777=CARTESIAN_POINT('Ctrl Pts',(-5.8516518405613,3.40309630255716,45.5297384586344));
#194778=CARTESIAN_POINT('Ctrl Pts',(-5.93566242842176,3.2496462170246,45.5379688451807));
#194779=CARTESIAN_POINT('Ctrl Pts',(-6.01959475711712,3.09633907627895,
45.5461915647984));
#194780=CARTESIAN_POINT('Ctrl Pts',(-6.09766478549532,2.93963026201029,
45.5544142844161));
#194781=CARTESIAN_POINT('Ctrl Pts',(-6.16959073445617,2.78000704483148,
45.5626370040338));
#194782=CARTESIAN_POINT('Ctrl Pts',(-6.24145295184508,2.62052526532145,
45.5708524377296));
#194783=CARTESIAN_POINT('Ctrl Pts',(-6.30718179475897,2.45813455305886,
45.5790678714254));
#194784=CARTESIAN_POINT('Ctrl Pts',(-6.36654150727517,2.29334651462496,
45.5872833051211));
#194785=CARTESIAN_POINT('Ctrl Pts',(-6.42587071350849,2.12864316444681,
45.5954945167219));
#194786=CARTESIAN_POINT('Ctrl Pts',(-6.47883718796481,1.96154527583867,
45.6037057283227));
#194787=CARTESIAN_POINT('Ctrl Pts',(-6.52525322510156,1.79258454425495,
45.6119169399235));
#194788=CARTESIAN_POINT('Ctrl Pts',(-6.57165369686032,1.62368047277868,
45.620125397937));
#194789=CARTESIAN_POINT('Ctrl Pts',(-6.61150801304833,1.45291514559708,
45.6283338559505));
#194790=CARTESIAN_POINT('Ctrl Pts',(-6.64467825451656,1.2808356233158,45.6365423139639));
#194791=CARTESIAN_POINT('Ctrl Pts',(-6.65945632139012,1.20417043864179,
45.6401993612473));
#194792=CARTESIAN_POINT('Ctrl Pts',(-6.67290833592412,1.12724457985017,
45.6438564085308));
#194793=CARTESIAN_POINT('Ctrl Pts',(-6.68502535051625,1.05010716736681,
45.6475134558142));
#194794=CARTESIAN_POINT('Ctrl Pts',(-6.7124521958382,0.87550674375319,45.6557911771468));
#194795=CARTESIAN_POINT('Ctrl Pts',(-6.73302212569519,0.699906920301995,
45.6640688984795));
#194796=CARTESIAN_POINT('Ctrl Pts',(-6.74668992367073,0.523893189342903,
45.6723466198121));
#194797=CARTESIAN_POINT('Ctrl Pts',(-6.76035772164626,0.34787945838381,
45.6806243411448));
#194798=CARTESIAN_POINT('Ctrl Pts',(-6.76712339837554,0.171452226019733,
45.6889020624775));
#194799=CARTESIAN_POINT('Ctrl Pts',(-6.76699829542289,-0.00480309729881822,
45.6971797838101));
#194800=CARTESIAN_POINT('',(-6.76699984541771,0.00144641512400706,45.302820216223));
#194801=CARTESIAN_POINT('Ctrl Pts',(3.09910619832132,6.01563211736941,44.6516492284231));
#194802=CARTESIAN_POINT('Ctrl Pts',(2.94672804361013,6.09413360724455,44.6596896898585));
#194803=CARTESIAN_POINT('Ctrl Pts',(2.79125002559318,6.16690088091477,44.6677301512939));
#194804=CARTESIAN_POINT('Ctrl Pts',(2.63315364174409,6.23368196966847,44.6757706127293));
#194805=CARTESIAN_POINT('Ctrl Pts',(2.46795317318091,6.30346387665885,44.6841723735049));
#194806=CARTESIAN_POINT('Ctrl Pts',(2.29989393689133,6.36670894231337,44.6925741342806));
#194807=CARTESIAN_POINT('Ctrl Pts',(2.12955192278888,6.42318438223178,44.7009758950562));
#194808=CARTESIAN_POINT('Ctrl Pts',(1.96660263550652,6.4772088267128,44.7090130251648));
#194809=CARTESIAN_POINT('Ctrl Pts',(1.8015649237697,6.52503873154561,44.7170501552734));
#194810=CARTESIAN_POINT('Ctrl Pts',(1.63496094949383,6.56652051650113,44.725087285382));
#194811=CARTESIAN_POINT('Ctrl Pts',(1.46834476877123,6.60800534067106,44.7331250043409));
#194812=CARTESIAN_POINT('Ctrl Pts',(1.30016245949996,6.64314102821417,44.7411627232999));
#194813=CARTESIAN_POINT('Ctrl Pts',(1.13094842483701,6.67182468747184,44.7492004422588));
#194814=CARTESIAN_POINT('Ctrl Pts',(0.96168846654374,6.70051613129518,44.7572403426043));
#194815=CARTESIAN_POINT('Ctrl Pts',(0.791396593721691,6.72275199893374,
44.7652802429499));
#194816=CARTESIAN_POINT('Ctrl Pts',(0.620614262965681,6.73848105559432,
44.7733201432954));
#194817=CARTESIAN_POINT('Ctrl Pts',(0.449751734246481,6.75421749848919,
44.7813638191114));
#194818=CARTESIAN_POINT('Ctrl Pts',(0.278398660528421,6.76344101428454,
44.7894074949273));
#194819=CARTESIAN_POINT('Ctrl Pts',(0.107098292709033,6.76615244845243,
44.7974511707433));
#194820=CARTESIAN_POINT('Ctrl Pts',(-0.0644124969663495,6.7688672132904,
44.8055047272455));
#194821=CARTESIAN_POINT('Ctrl Pts',(-0.235870078372894,6.76505392147229,
44.8135582837477));
#194822=CARTESIAN_POINT('Ctrl Pts',(-0.406733773147633,6.75476547614949,
44.8216118402499));
#194823=CARTESIAN_POINT('Ctrl Pts',(-0.577720687258337,6.74446961125519,
44.8296712046207));
#194824=CARTESIAN_POINT('Ctrl Pts',(-0.748112492369287,6.72768933119816,
44.8377305689915));
#194825=CARTESIAN_POINT('Ctrl Pts',(-0.917377468442388,6.70452888579013,
44.8457899333623));
#194826=CARTESIAN_POINT('Ctrl Pts',(-1.08689056063974,6.68133449077195,
44.8538611115076));
#194827=CARTESIAN_POINT('Ctrl Pts',(-1.25527316209345,6.65174132884393,
44.8619322896528));
#194828=CARTESIAN_POINT('Ctrl Pts',(-1.4220067907132,6.61590399621741,44.8700034677981));
#194829=CARTESIAN_POINT('Ctrl Pts',(-1.47302770806174,6.60493768065729,
44.8724732689802));
#194830=CARTESIAN_POINT('Ctrl Pts',(-1.52389435012713,6.59338702136638,
44.8749430701622));
#194831=CARTESIAN_POINT('Ctrl Pts',(-1.57459222930149,6.58125735034145,
44.8774128713443));
#194832=CARTESIAN_POINT('Ctrl Pts',(-1.74564303215994,6.54033275939186,
44.885745793391));
#194833=CARTESIAN_POINT('Ctrl Pts',(-1.9153170023392,6.4926828595889,44.8940787154377));
#194834=CARTESIAN_POINT('Ctrl Pts',(-2.08305434218415,6.43841390464358,
44.9024116374844));
#194835=CARTESIAN_POINT('Ctrl Pts',(-2.25059345717093,6.38420908244238,
44.910734712038));
#194836=CARTESIAN_POINT('Ctrl Pts',(-2.41620017272148,6.32340089356206,
44.9190577865916));
#194837=CARTESIAN_POINT('Ctrl Pts',(-2.57932578507492,6.25614637731948,
44.9273808611453));
#194838=CARTESIAN_POINT('Ctrl Pts',(-2.74228856515526,6.18895899465328,
44.9356956275913));
#194839=CARTESIAN_POINT('Ctrl Pts',(-2.9027748566236,6.11533823648511,44.9440103940372));
#194840=CARTESIAN_POINT('Ctrl Pts',(-3.06025179285158,6.03549069789265,
44.9523251604832));
#194841=CARTESIAN_POINT('Ctrl Pts',(-3.2176004218958,5.95570821652731,44.9606331523227));
#194842=CARTESIAN_POINT('Ctrl Pts',(-3.37194427237067,5.86970922054559,
44.9689411441623));
#194843=CARTESIAN_POINT('Ctrl Pts',(-3.52277091839561,5.77774818216458,
44.9772491360018));
#194844=CARTESIAN_POINT('Ctrl Pts',(-3.67350232727717,5.68584521115317,
44.9855518818889));
#194845=CARTESIAN_POINT('Ctrl Pts',(-3.82072066142304,5.58798788084392,
44.993854627776));
#194846=CARTESIAN_POINT('Ctrl Pts',(-3.96393835728736,5.48447642894251,
45.0021573736631));
#194847=CARTESIAN_POINT('Ctrl Pts',(-4.10709752464305,5.38100727887307,
45.0104567264826));
#194848=CARTESIAN_POINT('Ctrl Pts',(-4.2462590299019,5.27188881485649,45.018756079302));
#194849=CARTESIAN_POINT('Ctrl Pts',(-4.38096431699064,5.15746455666491,
45.0270554321214));
#194850=CARTESIAN_POINT('Ctrl Pts',(-4.51564095452497,5.04306463459318,
45.0353530198077));
#194851=CARTESIAN_POINT('Ctrl Pts',(-4.64586299704453,4.92336139158402,
45.0436506074941));
#194852=CARTESIAN_POINT('Ctrl Pts',(-4.77120482685568,4.79873874056393,
45.0519481951804));
#194853=CARTESIAN_POINT('Ctrl Pts',(-4.8965408272736,4.67412188548952,45.0602453969629));
#194854=CARTESIAN_POINT('Ctrl Pts',(-5.01699682069101,4.54458632372077,
45.0685425987453));
#194855=CARTESIAN_POINT('Ctrl Pts',(-5.13218380199773,4.4105530744468,45.0768398005277));
#194856=CARTESIAN_POINT('Ctrl Pts',(-5.24738456656427,4.27650378677094,
45.0851379951523));
#194857=CARTESIAN_POINT('Ctrl Pts',(-5.35731483641111,4.13795600340657,
45.0934361897769));
#194858=CARTESIAN_POINT('Ctrl Pts',(-5.46162555752576,3.99536422236839,
45.1017343844014));
#194859=CARTESIAN_POINT('Ctrl Pts',(-5.56600964158644,3.85267215486853,
45.110038415243));
#194860=CARTESIAN_POINT('Ctrl Pts',(-5.6647660737933,3.70593068757857,45.1183424460846));
#194861=CARTESIAN_POINT('Ctrl Pts',(-5.7575883482012,3.55562447576481,45.1266464769261));
#194862=CARTESIAN_POINT('Ctrl Pts',(-5.8504443753428,3.40526360847561,45.1349535273418));
#194863=CARTESIAN_POINT('Ctrl Pts',(-5.93736176738236,3.25133571294381,
45.1432605777576));
#194864=CARTESIAN_POINT('Ctrl Pts',(-6.01807966011595,3.09435069190592,
45.1515676281733));
#194865=CARTESIAN_POINT('Ctrl Pts',(-6.09888385389992,2.93719782738564,
45.1598835602279));
#194866=CARTESIAN_POINT('Ctrl Pts',(-6.17347515234348,2.77698161964319,
45.1681994922826));
#194867=CARTESIAN_POINT('Ctrl Pts',(-6.24164013118477,2.61423363010726,
45.1765154243372));
#194868=CARTESIAN_POINT('Ctrl Pts',(-6.2930243401069,2.49155073871459,45.1827841505562));
#194869=CARTESIAN_POINT('Ctrl Pts',(-6.34075779911307,2.3674296155873,45.1890528767751));
#194870=CARTESIAN_POINT('Ctrl Pts',(-6.38476779279172,2.24210375141953,
45.1953216029941));
#194871=CARTESIAN_POINT('Ctrl Pts',(-6.44765953403174,2.06300893315002,
45.2042798207604));
#194872=CARTESIAN_POINT('Ctrl Pts',(-6.50304972991107,1.88115764106677,
45.2132380385267));
#194873=CARTESIAN_POINT('Ctrl Pts',(-6.55071587795956,1.6971772112094,45.222196256293));
#194874=CARTESIAN_POINT('Ctrl Pts',(-6.59785592799697,1.5152273993522,45.2310556009441));
#194875=CARTESIAN_POINT('Ctrl Pts',(-6.63744147068533,1.33119547085567,
45.2399149455952));
#194876=CARTESIAN_POINT('Ctrl Pts',(-6.66930629363198,1.14570614108542,
45.2487742902462));
#194877=CARTESIAN_POINT('Ctrl Pts',(-6.70170454897727,0.957111631089739,
45.2577819445702));
#194878=CARTESIAN_POINT('Ctrl Pts',(-6.72612117866493,0.76701074401207,
45.2667895988941));
#194879=CARTESIAN_POINT('Ctrl Pts',(-6.74243476752652,0.576075000021326,
45.2757972532181));
#194880=CARTESIAN_POINT('Ctrl Pts',(-6.75874835638812,0.385139256030517,
45.284804907542));
#194881=CARTESIAN_POINT('Ctrl Pts',(-6.76695882283989,0.193368939904135,
45.2938125618659));
#194882=CARTESIAN_POINT('Ctrl Pts',(-6.76699984541756,0.00144641582902397,
45.3028202161899));
#194883=CARTESIAN_POINT('Ctrl Pts',(-6.76699984541771,0.00144641512391758,
45.302820216223));
#194884=CARTESIAN_POINT('Ctrl Pts',(-6.76703626799262,-0.168955259133196,
45.3108178151777));
#194885=CARTESIAN_POINT('Ctrl Pts',(-6.7606319637346,-0.339423633244816,
45.3188154141325));
#194886=CARTESIAN_POINT('Ctrl Pts',(-6.74779807270397,-0.509421407100884,
45.3268130130872));
#194887=CARTESIAN_POINT('Ctrl Pts',(-6.73496479099209,-0.679411109918256,
45.3348102323374));
#194888=CARTESIAN_POINT('Ctrl Pts',(-6.71570255732075,-0.848929879388188,
45.3428074515876));
#194889=CARTESIAN_POINT('Ctrl Pts',(-6.6900745042534,-1.01744391862089,
45.3508046708377));
#194890=CARTESIAN_POINT('Ctrl Pts',(-6.68636643998395,-1.04182582879324,
45.3519617701647));
#194891=CARTESIAN_POINT('Ctrl Pts',(-6.68252519855856,-1.06618671696161,
45.3531188694917));
#194892=CARTESIAN_POINT('Ctrl Pts',(-6.67855106060485,-1.09052497949101,
45.3542759688187));
#194893=CARTESIAN_POINT('Ctrl Pts',(-6.64894925924002,-1.27181119082858,
45.362894749756));
#194894=CARTESIAN_POINT('Ctrl Pts',(-6.61197259282066,-1.4518252175661,
45.3715135306932));
#194895=CARTESIAN_POINT('Ctrl Pts',(-6.56776194705422,-1.62996687292307,
45.3801323116304));
#194896=CARTESIAN_POINT('Ctrl Pts',(-6.52352474422171,-1.80821553688913,
45.388756269817));
#194897=CARTESIAN_POINT('Ctrl Pts',(-6.47204496319458,-1.98458928965325,
45.3973802280035));
#194898=CARTESIAN_POINT('Ctrl Pts',(-6.41351360988914,-2.15850229922666,
45.40600418619));
#194899=CARTESIAN_POINT('Ctrl Pts',(-6.35286771849596,-2.3386981924501,
45.4149396985611));
#194900=CARTESIAN_POINT('Ctrl Pts',(-6.28465137807912,-2.51625189068267,
45.4238752109322));
#194901=CARTESIAN_POINT('Ctrl Pts',(-6.20913160627264,-2.69053409121427,
45.4328107233033));
#194902=CARTESIAN_POINT('Ctrl Pts',(-6.13610870775519,-2.85905408456685,
45.4414508051981));
#194903=CARTESIAN_POINT('Ctrl Pts',(-6.05625776194166,-3.02451519146708,
45.4500908870928));
#194904=CARTESIAN_POINT('Ctrl Pts',(-5.96986738505975,-3.18637292305843,
45.4587309689875));
#194905=CARTESIAN_POINT('Ctrl Pts',(-5.87904608660028,-3.35653226116301,
45.4678141965968));
#194906=CARTESIAN_POINT('Ctrl Pts',(-5.78099712840625,-3.52270854534843,
45.4768974242061));
#194907=CARTESIAN_POINT('Ctrl Pts',(-5.67610818611867,-3.68430249293901,
45.4859806518155));
#194908=CARTESIAN_POINT('Ctrl Pts',(-5.5712192438311,-3.84589644052959,
45.4950638794248));
#194909=CARTESIAN_POINT('Ctrl Pts',(-5.45949056969796,-4.00290775509036,
45.5041471070341));
#194910=CARTESIAN_POINT('Ctrl Pts',(-5.34135995672453,-4.15477590402896,
45.5132303346434));
#194911=CARTESIAN_POINT('Ctrl Pts',(-5.22373177643027,-4.30599812792723,
45.5222749295032));
#194912=CARTESIAN_POINT('Ctrl Pts',(-5.09964806402658,-4.4522610308465,
45.531319524363));
#194913=CARTESIAN_POINT('Ctrl Pts',(-4.96953197896536,-4.59304266364255,
45.5403641192228));
#194914=CARTESIAN_POINT('Ctrl Pts',(-4.83953529589338,-4.73369510713048,
45.5494004142432));
#194915=CARTESIAN_POINT('Ctrl Pts',(-4.70351745344857,-4.86887614821844,
45.5584367092635));
#194916=CARTESIAN_POINT('Ctrl Pts',(-4.56194059478497,-4.99809833933397,
45.5674730042838));
#194917=CARTESIAN_POINT('Ctrl Pts',(-4.42061426747501,-5.12709186164892,
45.5764933088715));
#194918=CARTESIAN_POINT('Ctrl Pts',(-4.27374874289041,-5.25014743015173,
45.5855136134592));
#194919=CARTESIAN_POINT('Ctrl Pts',(-4.12184141577506,-5.36681584770723,
45.5945339180468));
#194920=CARTESIAN_POINT('Ctrl Pts',(-3.97012538642979,-5.48333734405397,
45.6035428633131));
#194921=CARTESIAN_POINT('Ctrl Pts',(-3.81338041342187,-5.59348759679608,
45.6125518085794));
#194922=CARTESIAN_POINT('Ctrl Pts',(-3.65213718322292,-5.69685729107906,
45.6215607538457));
#194923=CARTESIAN_POINT('Ctrl Pts',(-3.49126010226394,-5.79999225467007,
45.6305492417045));
#194924=CARTESIAN_POINT('Ctrl Pts',(-3.32590535321974,-5.89637726581379,
45.6395377295633));
#194925=CARTESIAN_POINT('Ctrl Pts',(-3.15663240641742,-5.98564623501551,
45.6485262174221));
#194926=CARTESIAN_POINT('Ctrl Pts',(-3.00811869254229,-6.06396746945018,
45.6564123784374));
#194927=CARTESIAN_POINT('Ctrl Pts',(-2.85658944393715,-6.13681155493424,
45.6642985394528));
#194928=CARTESIAN_POINT('Ctrl Pts',(-2.70244140676999,-6.20395836889441,
45.6721847004682));
#194929=CARTESIAN_POINT('Ctrl Pts',(-2.54369396754584,-6.27310868027126,
45.6803061653244));
#194930=CARTESIAN_POINT('Ctrl Pts',(-2.38223954086875,-6.33618420853312,
45.6884276301806));
#194931=CARTESIAN_POINT('Ctrl Pts',(-2.21858992398726,-6.39297643896661,
45.6965490950367));
#194932=CARTESIAN_POINT('Ctrl Pts',(-2.0549519777318,-6.44976461927829,
45.7046699807129));
#194933=CARTESIAN_POINT('Ctrl Pts',(-1.88911949904313,-6.50027027424077,
45.7127908663891));
#194934=CARTESIAN_POINT('Ctrl Pts',(-1.72162171742235,-6.54433401211305,
45.7209117520654));
#194935=CARTESIAN_POINT('Ctrl Pts',(-1.55410391502806,-6.58840301686175,
45.7290336084196));
#194936=CARTESIAN_POINT('Ctrl Pts',(-1.38492076778149,-6.62602847928742,
45.7371554647738));
#194937=CARTESIAN_POINT('Ctrl Pts',(-1.21461398060706,-6.65710161242217,
45.745277321128));
#194938=CARTESIAN_POINT('Ctrl Pts',(-1.044182939707,-6.68819741613055,45.7534051030882));
#194939=CARTESIAN_POINT('Ctrl Pts',(-0.872626982137431,-6.71273127679588,
45.7615328850484));
#194940=CARTESIAN_POINT('Ctrl Pts',(-0.700495898374002,-6.73064591969903,
45.7696606670085));
#194941=CARTESIAN_POINT('Ctrl Pts',(-0.528294694804394,-6.74856786036189,
45.777791759925));
#194942=CARTESIAN_POINT('Ctrl Pts',(-0.355518263194503,-6.75986518465779,
45.7859228528414));
#194943=CARTESIAN_POINT('Ctrl Pts',(-0.182718482227967,-6.76453272268324,
45.7940539457579));
#194944=CARTESIAN_POINT('Ctrl Pts',(-0.00973009752258797,-6.76920535513137,
45.8021939134224));
#194945=CARTESIAN_POINT('Ctrl Pts',(0.163281321721688,-6.76723375250431,
45.810333881087));
#194946=CARTESIAN_POINT('Ctrl Pts',(0.335766174274341,-6.75866481460748,
45.8184738487515));
#194947=CARTESIAN_POINT('Ctrl Pts',(0.425224276575121,-6.75422059291706,
45.822695587932));
#194948=CARTESIAN_POINT('Ctrl Pts',(0.514540838255739,-6.74800259950535,
45.8269173271125));
#194949=CARTESIAN_POINT('Ctrl Pts',(0.603640110343529,-6.74002282022728,
45.831139066293));
#194950=CARTESIAN_POINT('Ctrl Pts',(0.781769664727358,-6.72406944043441,
45.8395792757506));
#194951=CARTESIAN_POINT('Ctrl Pts',(0.959398397327153,-6.70103834344931,
45.8480194852082));
#194952=CARTESIAN_POINT('Ctrl Pts',(1.13594143568155,-6.67097639440448,
45.8564596946658));
#194953=CARTESIAN_POINT('Ctrl Pts',(1.31235071652922,-6.64093722173978,
45.8648935094144));
#194954=CARTESIAN_POINT('Ctrl Pts',(1.48767561530768,-6.6038778716359,45.8733273241629));
#194955=CARTESIAN_POINT('Ctrl Pts',(1.66133722834225,-6.5598969209679,45.8817611389114));
#194956=CARTESIAN_POINT('Ctrl Pts',(1.83489396343796,-6.51594253133071,
45.8901898603));
#194957=CARTESIAN_POINT('Ctrl Pts',(2.00678909292398,-6.46507495642847,
45.8986185816885));
#194958=CARTESIAN_POINT('Ctrl Pts',(2.17645435206196,-6.40744375343167,
45.9070473030771));
#194959=CARTESIAN_POINT('Ctrl Pts',(2.34604320019309,-6.34983850541393,
45.9154722284788));
#194960=CARTESIAN_POINT('Ctrl Pts',(2.51340386510166,-6.28547580994081,
45.9238971538806));
#194961=CARTESIAN_POINT('Ctrl Pts',(2.67798330409106,-6.21455504626112,
45.9323220792823));
#194962=CARTESIAN_POINT('Ctrl Pts',(2.84251387390282,-6.14365534134442,
45.94074450304));
#194963=CARTESIAN_POINT('Ctrl Pts',(3.00426455876845,-6.06620158341942,
45.9491669267977));
#194964=CARTESIAN_POINT('Ctrl Pts',(3.1627019950883,-5.98244139881575,45.9575893505553));
#194965=CARTESIAN_POINT('Ctrl Pts',(3.32114192317398,-5.89867989690494,
45.9660119067736));
#194966=CARTESIAN_POINT('Ctrl Pts',(3.47626820074634,-5.8086119200891,45.9744344629918));
#194967=CARTESIAN_POINT('Ctrl Pts',(3.62757119496527,-5.71253150761186,
45.98285701921));
#194968=CARTESIAN_POINT('Ctrl Pts',(3.77887930022777,-5.61644784952024,
45.9912798599437));
#194969=CARTESIAN_POINT('Ctrl Pts',(3.9263635829329,-5.51435152947949,45.9997027006775));
#194970=CARTESIAN_POINT('Ctrl Pts',(4.06954245923275,-5.40658054342131,
46.0081255414112));
#194971=CARTESIAN_POINT('Ctrl Pts',(4.2127461614971,-5.29879087081702,46.0165498425919));
#194972=CARTESIAN_POINT('Ctrl Pts',(4.35164270251472,-5.18532477110903,
46.0249741437725));
#194973=CARTESIAN_POINT('Ctrl Pts',(4.48578243166701,-5.06656145484762,
46.0333984449532));
#194974=CARTESIAN_POINT('Ctrl Pts',(4.6199641526039,-4.94776096031229,46.04182538332));
#194975=CARTESIAN_POINT('Ctrl Pts',(4.74938584317514,-4.82366016411711,
46.0502523216868));
#194976=CARTESIAN_POINT('Ctrl Pts',(4.87363339797939,-4.69467640014728,
46.0586792600536));
#194977=CARTESIAN_POINT('Ctrl Pts',(4.9979926669528,-4.56557666356095,46.0671137752973));
#194978=CARTESIAN_POINT('Ctrl Pts',(5.11716827269483,-4.43158542694702,
46.0755482905409));
#194979=CARTESIAN_POINT('Ctrl Pts',(5.23078446985143,-4.2931553465908,46.0839828057846));
#194980=CARTESIAN_POINT('Ctrl Pts',(5.34445554460447,-4.15465840332,46.0924213949713));
#194981=CARTESIAN_POINT('Ctrl Pts',(5.45256165018521,-4.01171860314079,
46.1008599841581));
#194982=CARTESIAN_POINT('Ctrl Pts',(5.55476905327486,-3.86481949963771,
46.1092985733449));
#194983=CARTESIAN_POINT('Ctrl Pts',(5.65709070111746,-3.71775619617181,
46.1177465949651));
#194984=CARTESIAN_POINT('Ctrl Pts',(5.75350028792251,-3.56672502468919,
46.1261946165854));
#194985=CARTESIAN_POINT('Ctrl Pts',(5.84370826213485,-3.41223720556717,
46.1346426382057));
#194986=CARTESIAN_POINT('Ctrl Pts',(5.89498102698885,-3.32442880845135,
46.139444358118));
#194987=CARTESIAN_POINT('Ctrl Pts',(5.944251136978,-3.23550415664104,46.1442460780302));
#194988=CARTESIAN_POINT('Ctrl Pts',(5.99147222024434,-3.14556030526206,
46.1490477979425));
#194989=CARTESIAN_POINT('Ctrl Pts',(6.07250144033901,-2.99122076822851,
46.1572873297933));
#194990=CARTESIAN_POINT('Ctrl Pts',(6.14767546819983,-2.83353443999638,
46.1655268616441));
#194991=CARTESIAN_POINT('Ctrl Pts',(6.21670730001626,-2.67298322963773,
46.1737663934949));
#194992=CARTESIAN_POINT('Ctrl Pts',(6.28566251132403,-2.51261021990161,
46.1819967800412));
#194993=CARTESIAN_POINT('Ctrl Pts',(6.34848896184637,-2.3493789836758,46.1902271665875));
#194994=CARTESIAN_POINT('Ctrl Pts',(6.40494497246148,-2.18379689983762,
46.1984575531339));
#194995=CARTESIAN_POINT('Ctrl Pts',(6.46134839208383,-2.01836906221835,
46.2066802727516));
#194996=CARTESIAN_POINT('Ctrl Pts',(6.51139307590824,-1.85059507310794,
46.2149029923694));
#194997=CARTESIAN_POINT('Ctrl Pts',(6.55488496484103,-1.68100330091912,
46.2231257119872));
#194998=CARTESIAN_POINT('Ctrl Pts',(6.59833831682685,-1.51156179925877,
46.231341145683));
#194999=CARTESIAN_POINT('Ctrl Pts',(6.63525035824642,-1.34030606820669,
46.2395565793787));
#195000=CARTESIAN_POINT('Ctrl Pts',(6.6654765442675,-1.16778056064477,46.2477720130745));
#195001=CARTESIAN_POINT('Ctrl Pts',(6.69568719637607,-0.995343717796904,
46.2559832246753));
#195002=CARTESIAN_POINT('Ctrl Pts',(6.71921877493554,-0.821638747792825,
46.2641944362761));
#195003=CARTESIAN_POINT('Ctrl Pts',(6.73597751835221,-0.647221656199521,
46.2724056478769));
#195004=CARTESIAN_POINT('Ctrl Pts',(6.7527306418111,-0.472863054474237,
46.2806141058905));
#195005=CARTESIAN_POINT('Ctrl Pts',(6.76271542062078,-0.297793160777767,
46.288822563904));
#195006=CARTESIAN_POINT('Ctrl Pts',(6.76588977680415,-0.122574581937041,
46.2970310219175));
#195007=CARTESIAN_POINT('Ctrl Pts',(6.76730402179845,-0.0445108790260286,
46.3006880692007));
#195008=CARTESIAN_POINT('Ctrl Pts',(6.7673671566835,0.0335822734222091,
46.304345116484));
#195009=CARTESIAN_POINT('Ctrl Pts',(6.76607878852531,0.111654948246415,
46.3080021637673));
#195010=CARTESIAN_POINT('Ctrl Pts',(6.76295775994808,0.300783379958654,
46.3168612379432));
#195011=CARTESIAN_POINT('Ctrl Pts',(6.75190560870376,0.489594982317368,
46.3257203121191));
#195012=CARTESIAN_POINT('Ctrl Pts',(6.73300540505689,0.677441669426068,
46.334579386295));
#195013=CARTESIAN_POINT('Ctrl Pts',(6.71406969172986,0.865641282667262,
46.343455104889));
#195014=CARTESIAN_POINT('Ctrl Pts',(6.68725648509868,1.05287209978896,46.3523308234829));
#195015=CARTESIAN_POINT('Ctrl Pts',(6.65270016103237,1.23849487984404,46.3612065420769));
#195016=CARTESIAN_POINT('Ctrl Pts',(6.61804522298096,1.42464737486621,46.3701075894639));
#195017=CARTESIAN_POINT('Ctrl Pts',(6.57560299673479,1.60918239336955,46.3790086368509));
#195018=CARTESIAN_POINT('Ctrl Pts',(6.52555888234382,1.79147153844647,46.3879096842379));
#195019=CARTESIAN_POINT('Ctrl Pts',(6.47544673229294,1.97400850811634,46.3968228327209));
#195020=CARTESIAN_POINT('Ctrl Pts',(6.41771212445246,2.15429325699545,46.4057359812039));
#195021=CARTESIAN_POINT('Ctrl Pts',(6.35258963012617,2.33171481772825,46.4146491296869));
#195022=CARTESIAN_POINT('Ctrl Pts',(6.28732254605501,2.50953030284104,46.4235820677968));
#195023=CARTESIAN_POINT('Ctrl Pts',(6.21463485592987,2.68446964016014,46.4325150059067));
#195024=CARTESIAN_POINT('Ctrl Pts',(6.13480951953011,2.85594137878962,46.4414479440166));
#195025=CARTESIAN_POINT('Ctrl Pts',(6.05882737347025,3.01915761159616,46.4499508058751));
#195026=CARTESIAN_POINT('Ctrl Pts',(5.97637876706631,3.17923211546311,46.4584536677335));
#195027=CARTESIAN_POINT('Ctrl Pts',(5.88774534609079,3.33567740340493,46.4669565295919));
#195028=CARTESIAN_POINT('Ctrl Pts',(5.80203966925059,3.48695498181656,46.4751785244403));
#195029=CARTESIAN_POINT('Ctrl Pts',(5.71038591012282,3.63512857379914,46.4834005192887));
#195030=CARTESIAN_POINT('Ctrl Pts',(5.61303486396487,3.77969954042842,46.4916225141371));
#195031=CARTESIAN_POINT('Ctrl Pts',(5.51578170093818,3.92412514591923,46.4998362420522));
#195032=CARTESIAN_POINT('Ctrl Pts',(5.41284285425992,4.06495504278447,46.5080499699674));
#195033=CARTESIAN_POINT('Ctrl Pts',(5.30451494138021,4.20171515415718,46.5162636978825));
#195034=CARTESIAN_POINT('Ctrl Pts',(5.19627624328738,4.33836263505576,46.5244706612809));
#195035=CARTESIAN_POINT('Ctrl Pts',(5.08265753808488,4.47094672502422,46.5326776246792));
#195036=CARTESIAN_POINT('Ctrl Pts',(4.96399869897026,4.59902227833499,46.5408845880776));
#195037=CARTESIAN_POINT('Ctrl Pts',(4.84541600183957,4.72701564706688,46.5490862851639));
#195038=CARTESIAN_POINT('Ctrl Pts',(4.72179985522649,4.8505059790308,46.5572879822502));
#195039=CARTESIAN_POINT('Ctrl Pts',(4.59353039710216,4.96908115157103,46.5654896793365));
#195040=CARTESIAN_POINT('Ctrl Pts',(4.46531758487443,5.08760395937018,46.5736877544188));
#195041=CARTESIAN_POINT('Ctrl Pts',(4.33245581749533,5.20121568852132,46.5818858295011));
#195042=CARTESIAN_POINT('Ctrl Pts',(4.19536213566963,5.30954099245778,46.5900839045835));
#195043=CARTESIAN_POINT('Ctrl Pts',(4.05830407533218,5.4178381498853,46.5982798495338));
#195044=CARTESIAN_POINT('Ctrl Pts',(3.91701657320311,5.52085139744787,46.6064757944842));
#195045=CARTESIAN_POINT('Ctrl Pts',(3.7719498318142,5.61824558614848,46.6146717394345));
#195046=CARTESIAN_POINT('Ctrl Pts',(3.62687458965975,5.71564548205086,46.622868164659));
#195047=CARTESIAN_POINT('Ctrl Pts',(3.47801996180599,5.80742545870113,46.6310645898836));
#195048=CARTESIAN_POINT('Ctrl Pts',(3.32586544744336,5.89329347865032,46.6392610151081));
#195049=CARTESIAN_POINT('Ctrl Pts',(3.25105656024912,5.93551168719234,46.6432909017834));
#195050=CARTESIAN_POINT('Ctrl Pts',(3.17545039875157,5.9763014568265,46.6473207884587));
#195051=CARTESIAN_POINT('Ctrl Pts',(3.09910619832134,6.0156321173694,46.651350675134));
#195052=CARTESIAN_POINT('Origin',(0.,0.,4.30282021618968));
#195053=CARTESIAN_POINT('',(3.09910619832136,6.01563211736939,49.0458451349191));
#195054=CARTESIAN_POINT('',(3.09910619832125,6.01563211736945,48.651281539311));
#195055=CARTESIAN_POINT('',(3.09910619832133,6.0156321173694,4.30282021618968));
#195056=CARTESIAN_POINT('',(-6.76699996850575,0.000652873004102149,47.6971797837837));
#195057=CARTESIAN_POINT('Ctrl Pts',(-6.76699996850581,0.000652872448132562,
47.69717978381));
#195058=CARTESIAN_POINT('Ctrl Pts',(-6.76701135541745,-0.117372066373527,
47.7027599263854));
#195059=CARTESIAN_POINT('Ctrl Pts',(-6.76393518322527,-0.235386287105458,
47.7083400689607));
#195060=CARTESIAN_POINT('Ctrl Pts',(-6.75777199804277,-0.353279807615802,
47.7139202115361));
#195061=CARTESIAN_POINT('Ctrl Pts',(-6.74867155662429,-0.527359126223625,
47.7221597433869));
#195062=CARTESIAN_POINT('Ctrl Pts',(-6.73282781940791,-0.701327768706293,
47.7303992752377));
#195063=CARTESIAN_POINT('Ctrl Pts',(-6.71023996551987,-0.874624836795691,
47.7386388070885));
#195064=CARTESIAN_POINT('Ctrl Pts',(-6.68767718257104,-1.04772955725079,
47.7468691936348));
#195065=CARTESIAN_POINT('Ctrl Pts',(-6.6583852334291,-1.22016383771851,
47.7550995801811));
#195066=CARTESIAN_POINT('Ctrl Pts',(-6.62241527335144,-1.39136801288573,
47.7633299667274));
#195067=CARTESIAN_POINT('Ctrl Pts',(-6.5864788207051,-1.562412704636,47.7715526863452));
#195068=CARTESIAN_POINT('Ctrl Pts',(-6.54387681875919,-1.73222922689334,
47.779775405963));
#195069=CARTESIAN_POINT('Ctrl Pts',(-6.49471208585917,-1.90026417158111,
47.7879981255808));
#195070=CARTESIAN_POINT('Ctrl Pts',(-6.44559091645483,-2.06815022520093,
47.7962135592766));
#195071=CARTESIAN_POINT('Ctrl Pts',(-6.38991870560588,-2.2342575072782,
47.8044289929724));
#195072=CARTESIAN_POINT('Ctrl Pts',(-6.32784905995541,-2.39804405181002,
47.8126444266682));
#195073=CARTESIAN_POINT('Ctrl Pts',(-6.26581131328305,-2.56174642277614,
47.820855638269));
#195074=CARTESIAN_POINT('Ctrl Pts',(-6.19738280553783,-2.72313009952606,
47.8290668498698));
#195075=CARTESIAN_POINT('Ctrl Pts',(-6.12276670973295,-2.88166910282668,
47.8372780614705));
#195076=CARTESIAN_POINT('Ctrl Pts',(-6.04817563604925,-3.04015494089387,
47.8454865194841));
#195077=CARTESIAN_POINT('Ctrl Pts',(-5.96740125923448,-3.19579768417759,
47.8536949774976));
#195078=CARTESIAN_POINT('Ctrl Pts',(-5.88069456558192,-3.34809205762554,
47.8619034355111));
#195079=CARTESIAN_POINT('Ctrl Pts',(-5.84206484024985,-3.4159425264658,
47.8655604827944));
#195080=CARTESIAN_POINT('Ctrl Pts',(-5.80225823542211,-3.48312867576308,
47.8692175300776));
#195081=CARTESIAN_POINT('Ctrl Pts',(-5.76129989740476,-3.54960737155026,
47.8728745773609));
#195082=CARTESIAN_POINT('Ctrl Pts',(-5.66207969965679,-3.71064977857462,
47.8817336515368));
#195083=CARTESIAN_POINT('Ctrl Pts',(-5.55620108325363,-3.86737147401267,
47.8905927257127));
#195084=CARTESIAN_POINT('Ctrl Pts',(-5.44406628293178,-4.01925755669445,
47.8994517998886));
#195085=CARTESIAN_POINT('Ctrl Pts',(-5.33172080388054,-4.1714290027676,
47.9083275184826));
#195086=CARTESIAN_POINT('Ctrl Pts',(-5.21309580497063,-4.31874647139722,
47.9172032370765));
#195087=CARTESIAN_POINT('Ctrl Pts',(-5.08863312498752,-4.46072885516254,
47.9260789556705));
#195088=CARTESIAN_POINT('Ctrl Pts',(-4.96381526368203,-4.60311641653475,
47.9349800030575));
#195089=CARTESIAN_POINT('Ctrl Pts',(-4.83312655610622,-4.7401382298894,
47.9438810504445));
#195090=CARTESIAN_POINT('Ctrl Pts',(-4.69704718270191,-4.87134855696778,
47.9527820978315));
#195091=CARTESIAN_POINT('Ctrl Pts',(-4.56078280752294,-5.00273726628556,
47.9616952463145));
#195092=CARTESIAN_POINT('Ctrl Pts',(-4.41911331812032,-5.12829853178341,
47.9706083947976));
#195093=CARTESIAN_POINT('Ctrl Pts',(-4.27255228179476,-5.24762670159858,
47.9795215432806));
#195094=CARTESIAN_POINT('Ctrl Pts',(-4.12566583989226,-5.36721981258036,
47.9884544813905));
#195095=CARTESIAN_POINT('Ctrl Pts',(-3.97386632979164,-5.48055198264083,
47.9973874195004));
#195096=CARTESIAN_POINT('Ctrl Pts',(-3.81769896731011,-5.58725904133676,
48.0063203576103));
#195097=CARTESIAN_POINT('Ctrl Pts',(-3.66905028155447,-5.6888286893346,
48.0148232194687));
#195098=CARTESIAN_POINT('Ctrl Pts',(-3.51644457724239,-5.78439603991769,
48.0233260813272));
#195099=CARTESIAN_POINT('Ctrl Pts',(-3.36037287420605,-5.87368565266309,
48.0318289431856));
#195100=CARTESIAN_POINT('Ctrl Pts',(-3.20944315916262,-5.9600335014135,
48.0400516670515));
#195101=CARTESIAN_POINT('Ctrl Pts',(-3.05498229824922,-6.04067509035055,
48.0482743909173));
#195102=CARTESIAN_POINT('Ctrl Pts',(-2.89746060097193,-6.11530956418523,
48.0564971147832));
#195103=CARTESIAN_POINT('Ctrl Pts',(-2.74010563507517,-6.1898650399576,
48.0647111351744));
#195104=CARTESIAN_POINT('Ctrl Pts',(-2.57969660576254,-6.25842590978019,
48.0729251555656));
#195105=CARTESIAN_POINT('Ctrl Pts',(-2.41673061829624,-6.32073588426138,
48.0811391759568));
#195106=CARTESIAN_POINT('Ctrl Pts',(-2.253904405844,-6.38299241582669,48.0893461512288));
#195107=CARTESIAN_POINT('Ctrl Pts',(-2.08852593613141,-6.43900860227001,
48.0975531265008));
#195108=CARTESIAN_POINT('Ctrl Pts',(-1.92111469273606,-6.48857513922384,
48.1057601017727));
#195109=CARTESIAN_POINT('Ctrl Pts',(-1.75381343518607,-6.53810911195224,
48.1139616852258));
#195110=CARTESIAN_POINT('Ctrl Pts',(-1.58448240682351,-6.58120177389115,
48.1221632686788));
#195111=CARTESIAN_POINT('Ctrl Pts',(-1.41365883454757,-6.61769277766093,
48.1303648521318));
#195112=CARTESIAN_POINT('Ctrl Pts',(-1.24291321022215,-6.65416713033907,
48.1385626931469));
#195113=CARTESIAN_POINT('Ctrl Pts',(-1.07067674890226,-6.68404575146301,
48.1467605341619));
#195114=CARTESIAN_POINT('Ctrl Pts',(-0.897499613741063,-6.7072187561861,
48.154958375177));
#195115=CARTESIAN_POINT('Ctrl Pts',(-0.724337760921886,-6.73038971596382,
48.1631554927581));
#195116=CARTESIAN_POINT('Ctrl Pts',(-0.550235753757301,-6.74685618198163,
48.1713526103393));
#195117=CARTESIAN_POINT('Ctrl Pts',(-0.375752040519851,-6.75655973140512,
48.1795497279205));
#195118=CARTESIAN_POINT('Ctrl Pts',(-0.20127026860789,-6.76626317286582,
48.1877467542996));
#195119=CARTESIAN_POINT('Ctrl Pts',(-0.0264071573010266,-6.76920382660556,
48.1959437806787));
#195120=CARTESIAN_POINT('Ctrl Pts',(0.148275774513133,-6.76537532548583,
48.2041408070578));
#195121=CARTESIAN_POINT('Ctrl Pts',(0.322988525441801,-6.76154617082479,
48.2123392327039));
#195122=CARTESIAN_POINT('Ctrl Pts',(0.497520676842875,-6.75094556702153,
48.2205376583501));
#195123=CARTESIAN_POINT('Ctrl Pts',(0.671312712364482,-6.73361925284003,
48.2287360839962));
#195124=CARTESIAN_POINT('Ctrl Pts',(0.845166015927335,-6.71628683049983,
48.2369373998869));
#195125=CARTESIAN_POINT('Ctrl Pts',(1.0182783270149,-6.69222401018458,48.2451387157775));
#195126=CARTESIAN_POINT('Ctrl Pts',(1.19009718442701,-6.66152817990128,
48.2533400316682));
#195127=CARTESIAN_POINT('Ctrl Pts',(1.36211171475564,-6.63079739220571,
48.2615506874848));
#195128=CARTESIAN_POINT('Ctrl Pts',(1.53282949495643,-6.59341856639132,
48.2697613433014));
#195129=CARTESIAN_POINT('Ctrl Pts',(1.70170912459192,-6.54954006440762,
48.277971999118));
#195130=CARTESIAN_POINT('Ctrl Pts',(1.87068827090139,-6.50563570588583,
48.2861874932751));
#195131=CARTESIAN_POINT('Ctrl Pts',(2.03782676451964,-6.45522413992352,
48.2944029874323));
#195132=CARTESIAN_POINT('Ctrl Pts',(2.20260034230712,-6.39850300711569,
48.3026184815894));
#195133=CARTESIAN_POINT('Ctrl Pts',(2.36762956933301,-6.34169387042643,
48.3108467222369));
#195134=CARTESIAN_POINT('Ctrl Pts',(2.5302862137073,-6.27855573355922,48.3190749628844));
#195135=CARTESIAN_POINT('Ctrl Pts',(2.69006666413196,-6.20933413036583,
48.3273032035319));
#195136=CARTESIAN_POINT('Ctrl Pts',(2.83528158444731,-6.14642274436639,
48.334781360633));
#195137=CARTESIAN_POINT('Ctrl Pts',(2.97812091338683,-6.07848714887653,
48.3422595177342));
#195138=CARTESIAN_POINT('Ctrl Pts',(3.11822635877642,-6.00574336576514,
48.3497376748353));
#195139=CARTESIAN_POINT('Ctrl Pts',(3.26940721086617,-5.92724914960935,
48.3578069840578));
#195140=CARTESIAN_POINT('Ctrl Pts',(3.41789934746328,-5.84289880365092,
48.3658762932804));
#195141=CARTESIAN_POINT('Ctrl Pts',(3.56320468417953,-5.75290025801257,
48.3739456025029));
#195142=CARTESIAN_POINT('Ctrl Pts',(3.70832878564812,-5.66301396502148,
48.3820048471037));
#195143=CARTESIAN_POINT('Ctrl Pts',(3.85027368283433,-5.56749368369514,
48.3900640917044));
#195144=CARTESIAN_POINT('Ctrl Pts',(3.98856240410905,-5.46659482205585,
48.3981233363052));
#195145=CARTESIAN_POINT('Ctrl Pts',(4.12670898899514,-5.3657996666312,48.4061742974255));
#195146=CARTESIAN_POINT('Ctrl Pts',(4.26120657738466,-5.2596371502495,48.4142252585457));
#195147=CARTESIAN_POINT('Ctrl Pts',(4.39160400129685,-5.14840784085658,
48.422276219666));
#195148=CARTESIAN_POINT('Ctrl Pts',(4.521895972344,-5.03726848300565,48.4303206699451));
#195149=CARTESIAN_POINT('Ctrl Pts',(4.64809409604339,-4.92107072851637,
48.4383651202242));
#195150=CARTESIAN_POINT('Ctrl Pts',(4.76977743883564,-4.80015751657948,
48.4464095705034));
#195151=CARTESIAN_POINT('Ctrl Pts',(4.89138901121838,-4.67931562081898,
48.4544492760616));
#195152=CARTESIAN_POINT('Ctrl Pts',(5.00849083967173,-4.55376406656954,
48.4624889816199));
#195153=CARTESIAN_POINT('Ctrl Pts',(5.1206963478992,-4.42388493437745,48.4705286871782));
#195154=CARTESIAN_POINT('Ctrl Pts',(5.23532375203256,-4.29120243055518,
48.4787419254826));
#195155=CARTESIAN_POINT('Ctrl Pts',(5.34484076078907,-4.15400366706386,
48.4869551637871));
#195156=CARTESIAN_POINT('Ctrl Pts',(5.44887592694491,-4.01273474487915,
48.4951684020915));
#195157=CARTESIAN_POINT('Ctrl Pts',(5.55068021272667,-3.87449512593499,
48.5032055196397));
#195158=CARTESIAN_POINT('Ctrl Pts',(5.64723515239597,-3.73235845615392,
48.5112426371879));
#195159=CARTESIAN_POINT('Ctrl Pts',(5.7382345678756,-3.58677474118985,48.519279754736));
#195160=CARTESIAN_POINT('Ctrl Pts',(5.82924361051464,-3.44117562439465,
48.5273177225601));
#195161=CARTESIAN_POINT('Ctrl Pts',(5.91469576054597,-3.29212905307198,
48.5353556903843));
#195162=CARTESIAN_POINT('Ctrl Pts',(5.99432936412382,-3.14011217544898,
48.5433936582083));
#195163=CARTESIAN_POINT('Ctrl Pts',(6.07398717078326,-2.98804909525914,
48.5514340690161));
#195164=CARTESIAN_POINT('Ctrl Pts',(6.14782273767134,-2.83301424259315,
48.5594744798238));
#195165=CARTESIAN_POINT('Ctrl Pts',(6.21562143990875,-2.67550726325806,
48.5675148906316));
#195166=CARTESIAN_POINT('Ctrl Pts',(6.28598255070105,-2.51204740845511,
48.5758591836193));
#195167=CARTESIAN_POINT('Ctrl Pts',(6.34984138638855,-2.34592532028708,
48.5842034766071));
#195168=CARTESIAN_POINT('Ctrl Pts',(6.40701419024083,-2.17771856906548,
48.5925477695949));
#195169=CARTESIAN_POINT('Ctrl Pts',(6.46220216729716,-2.01535132972001,
48.6006023798104));
#195170=CARTESIAN_POINT('Ctrl Pts',(6.51116052038201,-1.85104211643753,
48.6086569900259));
#195171=CARTESIAN_POINT('Ctrl Pts',(6.55377592327011,-1.6853219714835,48.6167116002415));
#195172=CARTESIAN_POINT('Ctrl Pts',(6.59642358662007,-1.51947637403921,
48.6247723079107));
#195173=CARTESIAN_POINT('Ctrl Pts',(6.63271866035056,-1.35221808076157,
48.63283301558));
#195174=CARTESIAN_POINT('Ctrl Pts',(6.66259945556137,-1.18408508763237,
48.6408937232492));
#195175=CARTESIAN_POINT('Ctrl Pts',(6.69252238090336,-1.01571503705519,
48.6489657960334));
#195176=CARTESIAN_POINT('Ctrl Pts',(6.71601293305232,-0.846468192526026,
48.6570378688175));
#195177=CARTESIAN_POINT('Ctrl Pts',(6.73306139370834,-0.676884974389522,
48.6651099416017));
#195178=CARTESIAN_POINT('Ctrl Pts',(6.73484709043169,-0.659122420744859,
48.665955429896));
#195179=CARTESIAN_POINT('Ctrl Pts',(6.73656215819896,-0.641356173871092,
48.6668009181904));
#195180=CARTESIAN_POINT('Ctrl Pts',(6.73820661880235,-0.623586852273408,
48.6676464064847));
#195181=CARTESIAN_POINT('Ctrl Pts',(6.75441401293016,-0.448456844340352,
48.6759793285314));
#195182=CARTESIAN_POINT('Ctrl Pts',(6.76381033163896,-0.27246969054077,
48.6843122505782));
#195183=CARTESIAN_POINT('Ctrl Pts',(6.76631632073985,-0.0961896443986176,
48.6926451726249));
#195184=CARTESIAN_POINT('Ctrl Pts',(6.76881934836934,0.0798820814776233,
48.7009682471785));
#195185=CARTESIAN_POINT('Ctrl Pts',(6.7644482623793,0.256245665240132,48.7092913217321));
#195186=CARTESIAN_POINT('Ctrl Pts',(6.75317546575908,0.43233104060391,48.7176143962857));
#195187=CARTESIAN_POINT('Ctrl Pts',(6.74191392166429,0.608240647236013,
48.7259291627317));
#195188=CARTESIAN_POINT('Ctrl Pts',(6.72376441472939,0.783872253675042,
48.7342439291776));
#195189=CARTESIAN_POINT('Ctrl Pts',(6.69875136458474,0.958654867756931,
48.7425586956236));
#195190=CARTESIAN_POINT('Ctrl Pts',(6.67375869427519,1.13329507454214,48.7508666874632));
#195191=CARTESIAN_POINT('Ctrl Pts',(6.64191367274921,1.30708732435082,48.7591746793027));
#195192=CARTESIAN_POINT('Ctrl Pts',(6.60329262589929,1.47946459800295,48.7674826711423));
#195193=CARTESIAN_POINT('Ctrl Pts',(6.56469596570982,1.65173302670177,48.7757854170294));
#195194=CARTESIAN_POINT('Ctrl Pts',(6.51933188282585,1.82258792124106,48.7840881629165));
#195195=CARTESIAN_POINT('Ctrl Pts',(6.46732803046758,1.99147110105278,48.7923909088036));
#195196=CARTESIAN_POINT('Ctrl Pts',(6.41534543042666,2.1602852636904,48.800690261623));
#195197=CARTESIAN_POINT('Ctrl Pts',(6.35672856991603,2.32712898517587,48.8089896144425));
#195198=CARTESIAN_POINT('Ctrl Pts',(6.29165540966437,2.49145764684875,48.8172889672619));
#195199=CARTESIAN_POINT('Ctrl Pts',(6.22659608938186,2.655751358573,48.8255865549483));
#195200=CARTESIAN_POINT('Ctrl Pts',(6.15508333299288,2.81753075286874,48.8338841426346));
#195201=CARTESIAN_POINT('Ctrl Pts',(6.07734393609153,2.97626942370001,48.842181730321));
#195202=CARTESIAN_POINT('Ctrl Pts',(5.99960815469194,3.13500071191746,48.8504789321034));
#195203=CARTESIAN_POINT('Ctrl Pts',(5.91564646300443,3.29069124612387,48.8587761338857));
#195204=CARTESIAN_POINT('Ctrl Pts',(5.82573255948691,3.442837368412,48.8670733356681));
#195205=CARTESIAN_POINT('Ctrl Pts',(5.73580789688236,3.59500169648709,48.8753715302927));
#195206=CARTESIAN_POINT('Ctrl Pts',(5.63992978073161,3.74362046834022,48.8836697249172));
#195207=CARTESIAN_POINT('Ctrl Pts',(5.53841645000472,3.88821710123254,48.8919679195418));
#195208=CARTESIAN_POINT('Ctrl Pts',(5.43683172376906,4.03291543062223,48.9002719503834));
#195209=CARTESIAN_POINT('Ctrl Pts',(5.3296040636254,4.17358568342901,48.9085759812249));
#195210=CARTESIAN_POINT('Ctrl Pts',(5.21709393807584,4.30978187862128,48.9168800120665));
#195211=CARTESIAN_POINT('Ctrl Pts',(5.1045429007476,4.44602759849913,48.9251870624823));
#195212=CARTESIAN_POINT('Ctrl Pts',(4.98670579675691,4.57779575468685,48.933494112898));
#195213=CARTESIAN_POINT('Ctrl Pts',(4.8639816687714,4.70467547508388,48.9418011633138));
#195214=CARTESIAN_POINT('Ctrl Pts',(4.74112632798099,4.83169085131545,48.9501170953684));
#195215=CARTESIAN_POINT('Ctrl Pts',(4.61337377080325,4.9538071039659,48.958433027423));
#195216=CARTESIAN_POINT('Ctrl Pts',(4.48115879339748,5.07065132585119,48.9667489594777));
#195217=CARTESIAN_POINT('Ctrl Pts',(4.3814923350924,5.15873098215957,48.9730176856966));
#195218=CARTESIAN_POINT('Ctrl Pts',(4.27929085903611,5.24381561418234,48.9792864119154));
#195219=CARTESIAN_POINT('Ctrl Pts',(4.17475210936812,5.32576133762361,48.9855551381343));
#195220=CARTESIAN_POINT('Ctrl Pts',(4.03381449903641,5.4362393610876,48.9940065429571));
#195221=CARTESIAN_POINT('Ctrl Pts',(3.88836913319198,5.5412132432926,49.0024579477799));
#195222=CARTESIAN_POINT('Ctrl Pts',(3.73887277406846,5.64031199308421,49.0109093526026));
#195223=CARTESIAN_POINT('Ctrl Pts',(3.58953094653658,5.73930830635079,49.0193520213662));
#195224=CARTESIAN_POINT('Ctrl Pts',(3.4361467509964,5.83244141481807,49.0277946901299));
#195225=CARTESIAN_POINT('Ctrl Pts',(3.27920823040502,5.91938192564426,49.0362373588935));
#195226=CARTESIAN_POINT('Ctrl Pts',(3.21967610070156,5.95236142454285,49.039439950902));
#195227=CARTESIAN_POINT('Ctrl Pts',(3.15963283954846,5.98445027557277,49.0426425429105));
#195228=CARTESIAN_POINT('Ctrl Pts',(3.09910619832136,6.01563211736939,49.0458451349191));
#195229=CARTESIAN_POINT('Ctrl Pts',(3.09910619832128,6.01563211736943,47.0456420231655));
#195230=CARTESIAN_POINT('Ctrl Pts',(2.93589454944422,6.09971475786413,47.0542963548475));
#195231=CARTESIAN_POINT('Ctrl Pts',(2.7693543383796,6.17710224807514,47.0629506865295));
#195232=CARTESIAN_POINT('Ctrl Pts',(2.60005473004366,6.24755987572569,47.0716050182115));
#195233=CARTESIAN_POINT('Ctrl Pts',(2.55768430450257,6.26519322819185,47.07377092822));
#195234=CARTESIAN_POINT('Ctrl Pts',(2.51514113168975,6.2823927721951,47.0759368382285));
#195235=CARTESIAN_POINT('Ctrl Pts',(2.47243429729718,6.29915531206753,47.0781027482371));
#195236=CARTESIAN_POINT('Ctrl Pts',(2.2940953943415,6.36915377985658,47.0871473430969));
#195237=CARTESIAN_POINT('Ctrl Pts',(2.11273661928173,6.43159254316305,47.0961919379567));
#195238=CARTESIAN_POINT('Ctrl Pts',(1.92898827293668,6.48623875931751,47.1052365328165));
#195239=CARTESIAN_POINT('Ctrl Pts',(1.74540854462305,6.54083482896684,47.1142728278369));
#195240=CARTESIAN_POINT('Ctrl Pts',(1.55944385080278,6.5876525604937,47.1233091228572));
#195241=CARTESIAN_POINT('Ctrl Pts',(1.37174040463728,6.62650867820194,47.1323454178775));
#195242=CARTESIAN_POINT('Ctrl Pts',(1.1843691144388,6.66529603696293,47.1413657224652));
#195243=CARTESIAN_POINT('Ctrl Pts',(0.995265448640978,6.69614986708242,
47.1503860270529));
#195244=CARTESIAN_POINT('Ctrl Pts',(0.805086409902682,6.71893777859194,
47.1594063316406));
#195245=CARTESIAN_POINT('Ctrl Pts',(0.615146864720306,6.7416969931536,47.1684152769069));
#195246=CARTESIAN_POINT('Ctrl Pts',(0.424134884659359,6.75641053168001,
47.1774242221732));
#195247=CARTESIAN_POINT('Ctrl Pts',(0.232715743612232,6.76299729281884,
47.1864331674395));
#195248=CARTESIAN_POINT('Ctrl Pts',(0.04173127491135,6.76956909681754,47.1954216552983));
#195249=CARTESIAN_POINT('Ctrl Pts',(-0.149658271927432,6.76805095142059,
47.2044101431571));
#195250=CARTESIAN_POINT('Ctrl Pts',(-0.340784934590754,6.75841361773279,
47.2133986310159));
#195251=CARTESIAN_POINT('Ctrl Pts',(-0.508472276417358,6.74995818380283,
47.2212847920312));
#195252=CARTESIAN_POINT('Ctrl Pts',(-0.675957051506147,6.73525362376994,
47.2291709530465));
#195253=CARTESIAN_POINT('Ctrl Pts',(-0.842785732964303,6.71431315983339,
47.2370571140618));
#195254=CARTESIAN_POINT('Ctrl Pts',(-1.01459217602766,6.69274788344573,
47.245178578918));
#195255=CARTESIAN_POINT('Ctrl Pts',(-1.18562567720486,6.66457705395441,
47.2533000437742));
#195256=CARTESIAN_POINT('Ctrl Pts',(-1.35533969976107,6.62988260063869,
47.2614215086304));
#195257=CARTESIAN_POINT('Ctrl Pts',(-1.52504161920968,6.59519062154811,
47.2695423943066));
#195258=CARTESIAN_POINT('Ctrl Pts',(-1.69342388870087,6.55397601864855,
47.2776632799828));
#195259=CARTESIAN_POINT('Ctrl Pts',(-1.85995005486183,6.50637186098516,
47.285784165659));
#195260=CARTESIAN_POINT('Ctrl Pts',(-2.02649612566183,6.45876201326358,
47.2939060220133));
#195261=CARTESIAN_POINT('Ctrl Pts',(-2.19118529961601,6.40476119180939,
47.3020278783675));
#195262=CARTESIAN_POINT('Ctrl Pts',(-2.35349622554594,6.34455234956266,
47.3101497347218));
#195263=CARTESIAN_POINT('Ctrl Pts',(-2.51592557151901,6.28429957968964,
47.318277516682));
#195264=CARTESIAN_POINT('Ctrl Pts',(-2.67597286024064,6.21782987027496,
47.3264052986422));
#195265=CARTESIAN_POINT('Ctrl Pts',(-2.8331360808695,6.14537459779918,47.3345330806024));
#195266=CARTESIAN_POINT('Ctrl Pts',(-2.99036332395316,6.07288980973834,
47.3426641735188));
#195267=CARTESIAN_POINT('Ctrl Pts',(-3.14470383092736,5.99441476425881,
47.3507952664353));
#195268=CARTESIAN_POINT('Ctrl Pts',(-3.2956803909903,5.91022670973306,47.3589263593518));
#195269=CARTESIAN_POINT('Ctrl Pts',(-3.44682173565884,5.82594676746422,
47.3670663270163));
#195270=CARTESIAN_POINT('Ctrl Pts',(-3.59459148762991,5.73594155201354,
47.3752062946809));
#195271=CARTESIAN_POINT('Ctrl Pts',(-3.73854097234446,5.64053192510261,
47.3833462623454));
#195272=CARTESIAN_POINT('Ctrl Pts',(-3.81319939909274,5.59104836733972,
47.3875680015258));
#195273=CARTESIAN_POINT('Ctrl Pts',(-3.88683073018327,5.54011175266949,
47.3917897407062));
#195274=CARTESIAN_POINT('Ctrl Pts',(-3.95937594541187,5.48777105233936,
47.3960114798866));
#195275=CARTESIAN_POINT('Ctrl Pts',(-4.10320066113873,5.38400285312451,
47.4043813004955));
#195276=CARTESIAN_POINT('Ctrl Pts',(-4.24306674454081,5.27448811926054,
47.4127511211043));
#195277=CARTESIAN_POINT('Ctrl Pts',(-4.37849989789952,5.15955692323419,
47.4211209417132));
#195278=CARTESIAN_POINT('Ctrl Pts',(-4.51382446214451,5.04471787803212,
47.4294840514733));
#195279=CARTESIAN_POINT('Ctrl Pts',(-4.64472292002328,4.92447124588934,
47.4378471612335));
#195280=CARTESIAN_POINT('Ctrl Pts',(-4.77075213347198,4.7991887940539,47.4462102709936));
#195281=CARTESIAN_POINT('Ctrl Pts',(-4.89670197423966,4.6739852445921,47.4545681137016));
#195282=CARTESIAN_POINT('Ctrl Pts',(-5.01778844097024,4.54375243716413,
47.4629259564095));
#195283=CARTESIAN_POINT('Ctrl Pts',(-5.13360329946691,4.40890078859827,
47.4712837991175));
#195284=CARTESIAN_POINT('Ctrl Pts',(-5.24936512419065,4.27411089110479,
47.4796378146142));
#195285=CARTESIAN_POINT('Ctrl Pts',(-5.35985993037371,4.1347066276499,47.4879918301109));
#195286=CARTESIAN_POINT('Ctrl Pts',(-5.46471782846359,3.99113368045625,
47.4963458456076));
#195287=CARTESIAN_POINT('Ctrl Pts',(-5.56975227083553,3.847319006284,47.5047139263649));
#195288=CARTESIAN_POINT('Ctrl Pts',(-5.66913058203875,3.69932185952979,
47.5130820071223));
#195289=CARTESIAN_POINT('Ctrl Pts',(-5.76252242132577,3.54762235077493,
47.5214500878796));
#195290=CARTESIAN_POINT('Ctrl Pts',(-5.85573510001801,3.39621385860593,
47.5298021155178));
#195291=CARTESIAN_POINT('Ctrl Pts',(-5.94298408360168,3.24111749420683,
47.5381541431559));
#195292=CARTESIAN_POINT('Ctrl Pts',(-6.02398508524712,3.08283841495467,
47.5465061707941));
#195293=CARTESIAN_POINT('Ctrl Pts',(-6.1049927121405,2.92454638971268,47.5548588815628));
#195294=CARTESIAN_POINT('Ctrl Pts',(-6.17975118257862,2.76307143517032,
47.5632115923314));
#195295=CARTESIAN_POINT('Ctrl Pts',(-6.24802278409988,2.59894214813812,
47.5715643031001));
#195296=CARTESIAN_POINT('Ctrl Pts',(-6.31631061892291,2.4347738352125,47.5799189999372));
#195297=CARTESIAN_POINT('Ctrl Pts',(-6.37810837926626,2.26795024759497,
47.5882736967743));
#195298=CARTESIAN_POINT('Ctrl Pts',(-6.43322689711854,2.09901898280853,
47.5966283936114));
#195299=CARTESIAN_POINT('Ctrl Pts',(-6.48850761428414,1.92959059770366,
47.6050076761258));
#195300=CARTESIAN_POINT('Ctrl Pts',(-6.53706961132309,1.7580424404529,47.6133869586401));
#195301=CARTESIAN_POINT('Ctrl Pts',(-6.57877280228418,1.58494082410858,
47.6217662411545));
#195302=CARTESIAN_POINT('Ctrl Pts',(-6.62040978814003,1.41211401193305,
47.6301322212987));
#195303=CARTESIAN_POINT('Ctrl Pts',(-6.655209693143,1.23773901200889,47.638498201443));
#195304=CARTESIAN_POINT('Ctrl Pts',(-6.68308464123356,1.06238819558019,
47.6468641815872));
#195305=CARTESIAN_POINT('Ctrl Pts',(-6.71102607338273,0.886619152939204,
47.6552501152867));
#195306=CARTESIAN_POINT('Ctrl Pts',(-6.73200944340711,0.709869976767763,
47.6636360489861));
#195307=CARTESIAN_POINT('Ctrl Pts',(-6.74599863286547,0.532720794954758,
47.6720219826855));
#195308=CARTESIAN_POINT('Ctrl Pts',(-6.75998782232383,0.355571613141753,
47.6804079163849));
#195309=CARTESIAN_POINT('Ctrl Pts',(-6.76698285604561,0.178022769645797,
47.6887938500843));
#195310=CARTESIAN_POINT('Ctrl Pts',(-6.76699996850575,0.000652873004196812,
47.6971797837837));
#195311=CARTESIAN_POINT('',(-6.76699998394344,-0.000466164701145535,47.302820216223));
#195312=CARTESIAN_POINT('Ctrl Pts',(3.09910619832134,6.0156321173694,46.651350675134));
#195313=CARTESIAN_POINT('Ctrl Pts',(2.94376773000356,6.09565868824486,46.6595503343105));
#195314=CARTESIAN_POINT('Ctrl Pts',(2.78537251701673,6.16964140625866,46.6677499934871));
#195315=CARTESIAN_POINT('Ctrl Pts',(2.62443560179651,6.23735735484372,46.6759496526637));
#195316=CARTESIAN_POINT('Ctrl Pts',(2.4634275737236,6.30510322493106,46.6841529350062));
#195317=CARTESIAN_POINT('Ctrl Pts',(2.29987593656179,6.36657667055195,46.6923562173487));
#195318=CARTESIAN_POINT('Ctrl Pts',(2.13431370578073,6.42160369419637,46.7005594996913));
#195319=CARTESIAN_POINT('Ctrl Pts',(1.96855810439084,6.47669498738473,46.7087723631665));
#195320=CARTESIAN_POINT('Ctrl Pts',(1.80078755988934,6.5253247082003,46.7169852266417));
#195321=CARTESIAN_POINT('Ctrl Pts',(1.63154910437626,6.56736907140211,46.7251980901169));
#195322=CARTESIAN_POINT('Ctrl Pts',(1.46219735665508,6.6094415800909,46.7334164514764));
#195323=CARTESIAN_POINT('Ctrl Pts',(1.29137608955599,6.64491987211678,46.7416348128359));
#195324=CARTESIAN_POINT('Ctrl Pts',(1.11964027288898,6.67373168919197,46.7498531741954));
#195325=CARTESIAN_POINT('Ctrl Pts',(0.94766179720174,6.70258421674583,46.7580831479229));
#195326=CARTESIAN_POINT('Ctrl Pts',(0.774766545646292,6.72475141133308,
46.7663131216504));
#195327=CARTESIAN_POINT('Ctrl Pts',(0.601513306138231,6.74021295973196,
46.774543095378));
#195328=CARTESIAN_POINT('Ctrl Pts',(0.529080969826472,6.74667700090492,
46.7779838173325));
#195329=CARTESIAN_POINT('Ctrl Pts',(0.456586049233609,6.75196962851049,
46.7814245392871));
#195330=CARTESIAN_POINT('Ctrl Pts',(0.384069221555972,6.75609205332886,
46.7848652612416));
#195331=CARTESIAN_POINT('Ctrl Pts',(0.21400005755518,6.76576011748679,46.7929345704641));
#195332=CARTESIAN_POINT('Ctrl Pts',(0.0432538459028244,6.7690199795768,
46.8010038796867));
#195333=CARTESIAN_POINT('Ctrl Pts',(-0.127634967030817,6.76579620703957,
46.8090731889092));
#195334=CARTESIAN_POINT('Ctrl Pts',(-0.298310635167999,6.76257645542291,
46.8171324335099));
#195335=CARTESIAN_POINT('Ctrl Pts',(-0.469128182337606,6.75288916681211,
46.8251916781107));
#195336=CARTESIAN_POINT('Ctrl Pts',(-0.639547083441763,6.73671051241339,
46.8332509227114));
#195337=CARTESIAN_POINT('Ctrl Pts',(-0.809790824006049,6.72054848681478,
46.8413018838317));
#195338=CARTESIAN_POINT('Ctrl Pts',(-0.979636365564611,6.69790840775643,
46.849352844952));
#195339=CARTESIAN_POINT('Ctrl Pts',(-1.14854232124391,6.66881845129343,
46.8574038060722));
#195340=CARTESIAN_POINT('Ctrl Pts',(-1.31731168206985,6.63975201998275,
46.8654482563513));
#195341=CARTESIAN_POINT('Ctrl Pts',(-1.48514260350749,6.60424615591976,
46.8734927066304));
#195342=CARTESIAN_POINT('Ctrl Pts',(-1.6514980704397,6.56238090355429,46.8815371569095));
#195343=CARTESIAN_POINT('Ctrl Pts',(-1.81775541876575,6.52054034385618,
46.8895768624678));
#195344=CARTESIAN_POINT('Ctrl Pts',(-1.98253868403992,6.47234795351275,
46.8976165680261));
#195345=CARTESIAN_POINT('Ctrl Pts',(-2.14532041684306,6.41793497233155,
46.9056562735843));
#195346=CARTESIAN_POINT('Ctrl Pts',(-2.3116157063202,6.36234751604255,46.9138695118888));
#195347=CARTESIAN_POINT('Ctrl Pts',(-2.47582168400813,6.3002679477279,46.9220827501932));
#195348=CARTESIAN_POINT('Ctrl Pts',(-2.6373912325011,6.23189028198719,46.9302959884977));
#195349=CARTESIAN_POINT('Ctrl Pts',(-2.7954961608265,6.16497887422606,46.9383331060458));
#195350=CARTESIAN_POINT('Ctrl Pts',(-2.95107622949768,6.09203690069045,
46.946370223594));
#195351=CARTESIAN_POINT('Ctrl Pts',(-3.1036384543481,6.01329504886395,46.9544073411422));
#195352=CARTESIAN_POINT('Ctrl Pts',(-3.25621681931218,5.93454486665004,
46.9624453089663));
#195353=CARTESIAN_POINT('Ctrl Pts',(-3.40577637266506,5.84999375566314,
46.9704832767905));
#195354=CARTESIAN_POINT('Ctrl Pts',(-3.55184856323456,5.75991847024319,
46.9785212446146));
#195355=CARTESIAN_POINT('Ctrl Pts',(-3.69796514959805,5.66981580819665,
46.9865616554223));
#195356=CARTESIAN_POINT('Ctrl Pts',(-3.840591945594,5.57418582575094,46.99460206623));
#195357=CARTESIAN_POINT('Ctrl Pts',(-3.97928935785062,5.47334862826193,
47.0026424770377));
#195358=CARTESIAN_POINT('Ctrl Pts',(-4.12322875002765,5.36870035343654,
47.0109867700255));
#195359=CARTESIAN_POINT('Ctrl Pts',(-4.26293557804433,5.2584438285581,47.0193310630133));
#195360=CARTESIAN_POINT('Ctrl Pts',(-4.397957017878,5.1429819238354,47.027675356001));
#195361=CARTESIAN_POINT('Ctrl Pts',(-4.52829101623976,5.03152842637964,
47.0357299662166));
#195362=CARTESIAN_POINT('Ctrl Pts',(-4.65425926856358,4.91522521355805,
47.0437845764321));
#195363=CARTESIAN_POINT('Ctrl Pts',(-4.77549326467682,4.79447109481602,
47.0518391866476));
#195364=CARTESIAN_POINT('Ctrl Pts',(-4.89681903663767,4.67362556350033,
47.0598998943169));
#195365=CARTESIAN_POINT('Ctrl Pts',(-5.01340316372495,4.54832268899797,
47.0679606019861));
#195366=CARTESIAN_POINT('Ctrl Pts',(-5.12491799040585,4.4189936175123,47.0760213096553));
#195367=CARTESIAN_POINT('Ctrl Pts',(-5.23659004631182,4.28948219978359,
47.0840933824395));
#195368=CARTESIAN_POINT('Ctrl Pts',(-5.34317831071259,4.15593354829151,
47.0921654552236));
#195369=CARTESIAN_POINT('Ctrl Pts',(-5.44439858121225,4.01880742122511,
47.1002375280078));
#195370=CARTESIAN_POINT('Ctrl Pts',(-5.45500063549913,4.00444450126718,
47.1010830163022));
#195371=CARTESIAN_POINT('Ctrl Pts',(-5.46554383960578,3.99004235446042,
47.1019285045966));
#195372=CARTESIAN_POINT('Ctrl Pts',(-5.47602789656972,3.97560152379363,
47.102773992891));
#195373=CARTESIAN_POINT('Ctrl Pts',(-5.58175609229637,3.8299705932821,47.1113004585698));
#195374=CARTESIAN_POINT('Ctrl Pts',(-5.68178758471567,3.67995942872403,
47.1198269242485));
#195375=CARTESIAN_POINT('Ctrl Pts',(-5.77575621167564,3.52603590215561,
47.1283533899272));
#195376=CARTESIAN_POINT('Ctrl Pts',(-5.8696048493169,3.37230892181418,47.1368689680912));
#195377=CARTESIAN_POINT('Ctrl Pts',(-5.95740588438657,3.21467981033767,
47.1453845462552));
#195378=CARTESIAN_POINT('Ctrl Pts',(-6.03883491479121,3.05364730640241,
47.1539001244192));
#195379=CARTESIAN_POINT('Ctrl Pts',(-6.12016969913281,2.89280118169139,
47.1624058466423));
#195380=CARTESIAN_POINT('Ctrl Pts',(-6.19514703415947,2.72855980311904,
47.1709115688653));
#195381=CARTESIAN_POINT('Ctrl Pts',(-6.26348690843292,2.56144895476944,
47.1794172910883));
#195382=CARTESIAN_POINT('Ctrl Pts',(-6.33175582951311,2.3945116075924,47.1879141823301));
#195383=CARTESIAN_POINT('Ctrl Pts',(-6.39340090554652,2.22471102761238,
47.1964110735718));
#195384=CARTESIAN_POINT('Ctrl Pts',(-6.44818878959137,2.05259599867782,
47.2049079648135));
#195385=CARTESIAN_POINT('Ctrl Pts',(-6.5029109822524,1.88068733789604,47.2133946681724));
#195386=CARTESIAN_POINT('Ctrl Pts',(-6.55079228728986,1.70647007132983,
47.2218813715313));
#195387=CARTESIAN_POINT('Ctrl Pts',(-6.5916480686147,1.53051126736398,47.2303680748902));
#195388=CARTESIAN_POINT('Ctrl Pts',(-6.6324745582664,1.35467861758255,47.2388486936821));
#195389=CARTESIAN_POINT('Ctrl Pts',(-6.66628549112995,1.17710723318183,
47.2473293124739));
#195390=CARTESIAN_POINT('Ctrl Pts',(-6.69294621220899,0.998378685909012,
47.2558099312658));
#195391=CARTESIAN_POINT('Ctrl Pts',(-6.71958695073797,0.819784097959,47.2642841937258));
#195392=CARTESIAN_POINT('Ctrl Pts',(-6.73908811962763,0.640034396317557,
47.2727584561858));
#195393=CARTESIAN_POINT('Ctrl Pts',(-6.75136621022658,0.459720888595186,
47.2812327186459));
#195394=CARTESIAN_POINT('Ctrl Pts',(-6.76179202415042,0.306609534324127,
47.2884285511605));
#195395=CARTESIAN_POINT('Ctrl Pts',(-6.7670105622296,0.15309194578801,47.2956243836752));
#195396=CARTESIAN_POINT('Ctrl Pts',(-6.76699998394349,-0.000466163995218723,
47.3028202161899));
#195397=CARTESIAN_POINT('Ctrl Pts',(-6.76699998394344,-0.000466164701054033,
47.302820216223));
#195398=CARTESIAN_POINT('Ctrl Pts',(-6.76698667745886,-0.193627467444925,
47.3118718800187));
#195399=CARTESIAN_POINT('Ctrl Pts',(-6.75869855779439,-0.386573833465984,
47.3209235438144));
#195400=CARTESIAN_POINT('Ctrl Pts',(-6.74221614043191,-0.578628132481847,
47.3299752076101));
#195401=CARTESIAN_POINT('Ctrl Pts',(-6.72567262469657,-0.771394354082396,
47.3390604248536));
#195402=CARTESIAN_POINT('Ctrl Pts',(-6.70087401106703,-0.96326166573528,
47.3481456420971));
#195403=CARTESIAN_POINT('Ctrl Pts',(-6.66795266219676,-1.15355810200577,
47.3572308593406));
#195404=CARTESIAN_POINT('Ctrl Pts',(-6.63497125451219,-1.34420169836295,
47.3663326508555));
#195405=CARTESIAN_POINT('Ctrl Pts',(-6.5938375346171,-1.53326847497989,
47.3754344423705));
#195406=CARTESIAN_POINT('Ctrl Pts',(-6.54473447929962,-1.72009871677959,
47.3845362338855));
#195407=CARTESIAN_POINT('Ctrl Pts',(-6.49551953809281,-1.90735466870306,
47.393658764681));
#195408=CARTESIAN_POINT('Ctrl Pts',(-6.43829899304615,-2.09236367814682,
47.4027812954766));
#195409=CARTESIAN_POINT('Ctrl Pts',(-6.3733058150232,-2.2744805974533,47.4119038262721));
#195410=CARTESIAN_POINT('Ctrl Pts',(-6.35245748865429,-2.33289954366425,
47.4148301256949));
#195411=CARTESIAN_POINT('Ctrl Pts',(-6.33080974255341,-2.39102105881993,
47.4177564251177));
#195412=CARTESIAN_POINT('Ctrl Pts',(-6.30837130107367,-2.44882431541956,
47.4206827245405));
#195413=CARTESIAN_POINT('Ctrl Pts',(-6.24357586053917,-2.61574265861571,
47.4291329932639));
#195414=CARTESIAN_POINT('Ctrl Pts',(-6.17209644062764,-2.78022941324602,
47.4375832619872));
#195415=CARTESIAN_POINT('Ctrl Pts',(-6.09413637121529,-2.9417326338454,
47.4460335307106));
#195416=CARTESIAN_POINT('Ctrl Pts',(-6.01624510420906,-3.10309332237344,
47.4544763417851));
#195417=CARTESIAN_POINT('Ctrl Pts',(-5.93188473095685,-3.26147542783308,
47.4629191528596));
#195418=CARTESIAN_POINT('Ctrl Pts',(-5.84130680522698,-3.4163465584172,
47.4713619639341));
#195419=CARTESIAN_POINT('Ctrl Pts',(-5.75079648517205,-3.57110209607701,
47.4797984734518));
#195420=CARTESIAN_POINT('Ctrl Pts',(-5.65407803039699,-3.72235159744624,
47.4882349829696));
#195421=CARTESIAN_POINT('Ctrl Pts',(-5.55144927382354,-3.86958653607387,
47.4966714924873));
#195422=CARTESIAN_POINT('Ctrl Pts',(-5.44889395364787,-4.01671612018018,
47.5051019652286));
#195423=CARTESIAN_POINT('Ctrl Pts',(-5.34043695652181,-4.15983660011802,
47.5135324379698));
#195424=CARTESIAN_POINT('Ctrl Pts',(-5.22641994845009,-4.29846757838685,
47.521962910711));
#195425=CARTESIAN_POINT('Ctrl Pts',(-5.11245195598136,-4.43703895957357,
47.5303897592148));
#195426=CARTESIAN_POINT('Ctrl Pts',(-4.99292892781845,-4.57112443103792,
47.5388166077186));
#195427=CARTESIAN_POINT('Ctrl Pts',(-4.86823380156747,-4.70027538057888,
47.5472434562224));
#195428=CARTESIAN_POINT('Ctrl Pts',(-4.74357716424851,-4.82938646583431,
47.5556677036591));
#195429=CARTESIAN_POINT('Ctrl Pts',(-4.61375184256928,-4.95356582834526,
47.5640919510957));
#195430=CARTESIAN_POINT('Ctrl Pts',(-4.47917898666345,-5.07240028048188,
47.5725161985324));
#195431=CARTESIAN_POINT('Ctrl Pts',(-4.44126150470596,-5.1058832824178,
47.5748898291433));
#195432=CARTESIAN_POINT('Ctrl Pts',(-4.40296734103366,-5.1389421792453,
47.5772634597543));
#195433=CARTESIAN_POINT('Ctrl Pts',(-4.36430643069116,-5.17156827074997,
47.5796370903653));
#195434=CARTESIAN_POINT('Ctrl Pts',(-4.22392657734108,-5.29003537098732,
47.5882558713025));
#195435=CARTESIAN_POINT('Ctrl Pts',(-4.07877158475177,-5.40274008166171,
47.5968746522398));
#195436=CARTESIAN_POINT('Ctrl Pts',(-3.92933878703287,-5.5093180791019,
47.605493433177));
#195437=CARTESIAN_POINT('Ctrl Pts',(-3.77981622594112,-5.61596009729702,
47.6141173913635));
#195438=CARTESIAN_POINT('Ctrl Pts',(-3.62601097911667,-5.71646788091598,
47.62274134955));
#195439=CARTESIAN_POINT('Ctrl Pts',(-3.46844912035301,-5.81052060486171,
47.6313653077365));
#195440=CARTESIAN_POINT('Ctrl Pts',(-3.3051950892284,-5.90797113281861,
47.6403008201077));
#195441=CARTESIAN_POINT('Ctrl Pts',(-3.13790827172861,-5.99849132695656,
47.6492363324788));
#195442=CARTESIAN_POINT('Ctrl Pts',(-2.96720075482661,-6.08177677003657,
47.6581718448499));
#195443=CARTESIAN_POINT('Ctrl Pts',(-2.80213725708672,-6.16230858723531,
47.6668119267446));
#195444=CARTESIAN_POINT('Ctrl Pts',(-2.63387593106464,-6.23607631465909,
47.6754520086393));
#195445=CARTESIAN_POINT('Ctrl Pts',(-2.46299011618518,-6.30285401128521,
47.6840920905341));
#195446=CARTESIAN_POINT('Ctrl Pts',(-2.28333964866977,-6.37305670439317,
47.6931753181434));
#195447=CARTESIAN_POINT('Ctrl Pts',(-2.10078877544895,-6.43553337455878,
47.7022585457527));
#195448=CARTESIAN_POINT('Ctrl Pts',(-1.91602172126667,-6.49008087496869,
47.711341773362));
#195449=CARTESIAN_POINT('Ctrl Pts',(-1.73125466708438,-6.5446283753786,
47.7204250009714));
#195450=CARTESIAN_POINT('Ctrl Pts',(-1.54427181634025,-6.59124664487992,
47.7295082285807));
#195451=CARTESIAN_POINT('Ctrl Pts',(-1.35577026679151,-6.62979456572254,
47.73859145619));
#195452=CARTESIAN_POINT('Ctrl Pts',(-1.16807045132442,-6.66817853469319,
47.7476360510498));
#195453=CARTESIAN_POINT('Ctrl Pts',(-0.978691667858135,-6.69859696376709,
47.7566806459097));
#195454=CARTESIAN_POINT('Ctrl Pts',(-0.788294806283688,-6.72092852948059,
47.7657252407695));
#195455=CARTESIAN_POINT('Ctrl Pts',(-0.598072663799427,-6.74323960246742,
47.7747615357898));
#195456=CARTESIAN_POINT('Ctrl Pts',(-0.406834544506014,-6.75747860040878,
47.7837978308102));
#195457=CARTESIAN_POINT('Ctrl Pts',(-0.215248516264292,-6.76357576110788,
47.7928341258306));
#195458=CARTESIAN_POINT('Ctrl Pts',(-0.024001514523603,-6.76966213240298,
47.8018544304183));
#195459=CARTESIAN_POINT('Ctrl Pts',(0.167591929322728,-6.76763542907804,
47.810874735006));
#195460=CARTESIAN_POINT('Ctrl Pts',(0.358861842538853,-6.7574778710677,
47.8198950395937));
#195461=CARTESIAN_POINT('Ctrl Pts',(0.549890888454496,-6.74733310452851,
47.82890398486));
#195462=CARTESIAN_POINT('Ctrl Pts',(0.740596979969487,-6.72907792986837,
47.8379129301263));
#195463=CARTESIAN_POINT('Ctrl Pts',(0.930310789523399,-6.70274651429519,
47.8469218753927));
#195464=CARTESIAN_POINT('Ctrl Pts',(1.11959379917794,-6.67647489179246,
47.8559103632515));
#195465=CARTESIAN_POINT('Ctrl Pts',(1.30788878937756,-6.64216366811312,
47.8648988511102));
#195466=CARTESIAN_POINT('Ctrl Pts',(1.49453267626538,-6.59989856585501,
47.873887338969));
#195467=CARTESIAN_POINT('Ctrl Pts',(1.65828699930971,-6.56281675554726,
47.8817734999843));
#195468=CARTESIAN_POINT('Ctrl Pts',(1.82077028321809,-6.51961309340796,
47.8896596609996));
#195469=CARTESIAN_POINT('Ctrl Pts',(1.98153798437442,-6.47037836733536,
47.8975458220148));
#195470=CARTESIAN_POINT('Ctrl Pts',(2.14710260224417,-6.41967459692935,
47.905667286871));
#195471=CARTESIAN_POINT('Ctrl Pts',(2.31077313961764,-6.36259562220991,
47.9137887517272));
#195472=CARTESIAN_POINT('Ctrl Pts',(2.4720252008872,-6.29931586810652,47.9219102165833));
#195473=CARTESIAN_POINT('Ctrl Pts',(2.63326576251149,-6.23604062678095,
47.9300311022595));
#195474=CARTESIAN_POINT('Ctrl Pts',(2.7920878506949,-6.16656562065507,47.9381519879358));
#195475=CARTESIAN_POINT('Ctrl Pts',(2.94798577226883,-6.09111392821548,
47.946272873612));
#195476=CARTESIAN_POINT('Ctrl Pts',(3.10390232810235,-6.01565321714107,
47.9543947299662));
#195477=CARTESIAN_POINT('Ctrl Pts',(3.25689369226613,-5.93421455785329,
47.9625165863205));
#195478=CARTESIAN_POINT('Ctrl Pts',(3.40647760320885,-5.84706758459627,
47.9706384426747));
#195479=CARTESIAN_POINT('Ctrl Pts',(3.55617064872238,-5.75985702998573,
47.9787662246349));
#195480=CARTESIAN_POINT('Ctrl Pts',(3.70245095899338,-5.66693002786138,
47.9868940065951));
#195481=CARTESIAN_POINT('Ctrl Pts',(3.84486362907688,-5.56860060282669,
47.9950217885552));
#195482=CARTESIAN_POINT('Ctrl Pts',(3.98733431278901,-5.47023112203893,
48.0031528814717));
#195483=CARTESIAN_POINT('Ctrl Pts',(4.12593392291485,-5.3664550509581,48.0112839743882));
#195484=CARTESIAN_POINT('Ctrl Pts',(4.26023985246192,-5.25762735456739,
48.0194150673046));
#195485=CARTESIAN_POINT('Ctrl Pts',(4.39469237131809,-5.14868087729426,
48.0275550349692));
#195486=CARTESIAN_POINT('Ctrl Pts',(4.52484157423164,-5.03467200313603,
48.0356950026337));
#195487=CARTESIAN_POINT('Ctrl Pts',(4.65030044578834,-4.91599377175162,
48.0438349702983));
#195488=CARTESIAN_POINT('Ctrl Pts',(4.71536884107114,-4.85444210963824,
48.0480567094787));
#195489=CARTESIAN_POINT('Ctrl Pts',(4.77917621034294,-4.79163501402767,
48.0522784486592));
#195490=CARTESIAN_POINT('Ctrl Pts',(4.84167280400669,-4.72763085053624,
48.0565001878396));
#195491=CARTESIAN_POINT('Ctrl Pts',(4.96661760006426,-4.59967208213843,
48.0649403972972));
#195492=CARTESIAN_POINT('Ctrl Pts',(5.08657922504885,-4.4666622832349,48.0733806067548));
#195493=CARTESIAN_POINT('Ctrl Pts',(5.20114384654871,-4.32901740438965,
48.0818208162125));
#195494=CARTESIAN_POINT('Ctrl Pts',(5.31562166837496,-4.19147681193231,
48.090254630961));
#195495=CARTESIAN_POINT('Ctrl Pts',(5.4247104253514,-4.04930839538647,48.0986884457095));
#195496=CARTESIAN_POINT('Ctrl Pts',(5.52803444804585,-3.90296350754378,
48.107122260458));
#195497=CARTESIAN_POINT('Ctrl Pts',(5.63129607116677,-3.75670700048953,
48.1155509818466));
#195498=CARTESIAN_POINT('Ctrl Pts',(5.7287997089068,-3.60627932236902,48.1239797032351));
#195499=CARTESIAN_POINT('Ctrl Pts',(5.82021092691212,-3.45216363549771,
48.1324084246236));
#195500=CARTESIAN_POINT('Ctrl Pts',(5.91158097665924,-3.29811735667639,
48.1408333500254));
#195501=CARTESIAN_POINT('Ctrl Pts',(5.9968639076614,-3.14038666718715,48.1492582754271));
#195502=CARTESIAN_POINT('Ctrl Pts',(6.07576924908423,-2.97948267856729,
48.1576832008288));
#195503=CARTESIAN_POINT('Ctrl Pts',(6.15465116085465,-2.81862646775885,
48.1661056245865));
#195504=CARTESIAN_POINT('Ctrl Pts',(6.22715911286567,-2.65459913599151,
48.1745280483442));
#195505=CARTESIAN_POINT('Ctrl Pts',(6.29304895945054,-2.48793564907907,
48.182950472102));
#195506=CARTESIAN_POINT('Ctrl Pts',(6.35893984229296,-2.32126954102991,
48.1913730283201));
#195507=CARTESIAN_POINT('Ctrl Pts',(6.41821228298509,-2.15196750260328,
48.1997955845383));
#195508=CARTESIAN_POINT('Ctrl Pts',(6.47067034617133,-1.98058432569255,
48.2082181407565));
#195509=CARTESIAN_POINT('Ctrl Pts',(6.5231301814009,-1.80919535942558,48.2166409814903));
#195510=CARTESIAN_POINT('Ctrl Pts',(6.56877508235097,-1.63572543342071,
48.225063822224));
#195511=CARTESIAN_POINT('Ctrl Pts',(6.60745900709423,-1.46074449154169,
48.2334866629578));
#195512=CARTESIAN_POINT('Ctrl Pts',(6.64614963929158,-1.28573320949829,
48.2419109641384));
#195513=CARTESIAN_POINT('Ctrl Pts',(6.67787681693145,-1.10921071493016,
48.250335265319));
#195514=CARTESIAN_POINT('Ctrl Pts',(6.702545559052,-0.931757494647768,48.2587595664996));
#195515=CARTESIAN_POINT('Ctrl Pts',(6.72722202360128,-0.754248723505163,
48.2671865048664));
#195516=CARTESIAN_POINT('Ctrl Pts',(6.74483560136085,-0.575808976013488,
48.2756134432332));
#195517=CARTESIAN_POINT('Ctrl Pts',(6.75534310595481,-0.397024584665557,
48.2840403816));
#195518=CARTESIAN_POINT('Ctrl Pts',(6.76586005811618,-0.218079443676738,
48.2924748968437));
#195519=CARTESIAN_POINT('Ctrl Pts',(6.76925815078355,-0.0387893729546224,
48.3009094120873));
#195520=CARTESIAN_POINT('Ctrl Pts',(6.76554630902837,0.140257407621158,
48.3093439273309));
#195521=CARTESIAN_POINT('Ctrl Pts',(6.76183267442182,0.319390669325824,
48.3177825165177));
#195522=CARTESIAN_POINT('Ctrl Pts',(6.75100227138573,0.498280073453796,
48.3262211057045));
#195523=CARTESIAN_POINT('Ctrl Pts',(6.7331160330511,0.676341249274491,48.3346596948913));
#195524=CARTESIAN_POINT('Ctrl Pts',(6.71520980194868,0.854601457204353,
48.3431077165115));
#195525=CARTESIAN_POINT('Ctrl Pts',(6.69023201777036,1.03203125595538,48.3515557381318));
#195526=CARTESIAN_POINT('Ctrl Pts',(6.65829516914972,1.20805398905742,48.3600037597521));
#195527=CARTESIAN_POINT('Ctrl Pts',(6.640142776927,1.30810248568076,48.3648054796644));
#195528=CARTESIAN_POINT('Ctrl Pts',(6.61974311859267,1.40769661893139,48.3696071995767));
#195529=CARTESIAN_POINT('Ctrl Pts',(6.59712408284742,1.50673250297279,48.374408919489));
#195530=CARTESIAN_POINT('Ctrl Pts',(6.5583108515756,1.67667355239676,48.3826484513398));
#195531=CARTESIAN_POINT('Ctrl Pts',(6.51287316133395,1.84534936240476,48.3908879831907));
#195532=CARTESIAN_POINT('Ctrl Pts',(6.46090637475389,2.01220720023176,48.3991275150415));
#195533=CARTESIAN_POINT('Ctrl Pts',(6.40899726767496,2.17887983752052,48.4073579015879));
#195534=CARTESIAN_POINT('Ctrl Pts',(6.35057359883229,2.34373818363682,48.4155882881342));
#195535=CARTESIAN_POINT('Ctrl Pts',(6.28578172588067,2.50623963231464,48.4238186746805));
#195536=CARTESIAN_POINT('Ctrl Pts',(6.22105020910515,2.66858970450639,48.4320413942983));
#195537=CARTESIAN_POINT('Ctrl Pts',(6.14996243340196,2.82858692306636,48.4402641139162));
#195538=CARTESIAN_POINT('Ctrl Pts',(6.07271458158104,2.98570370443101,48.448486833534));
#195539=CARTESIAN_POINT('Ctrl Pts',(5.99553517692233,3.14268126900754,48.4567022672298));
#195540=CARTESIAN_POINT('Ctrl Pts',(5.91220673142729,3.29678316513945,48.4649177009256));
#195541=CARTESIAN_POINT('Ctrl Pts',(5.82297350223552,3.44750179003042,48.4731331346213));
#195542=CARTESIAN_POINT('Ctrl Pts',(5.73378613199442,3.59814295725181,48.4813443462222));
#195543=CARTESIAN_POINT('Ctrl Pts',(5.63870020260684,3.74540401057651,48.489555557823));
#195544=CARTESIAN_POINT('Ctrl Pts',(5.53800606247838,3.88880159585864,48.4977667694238));
#195545=CARTESIAN_POINT('Ctrl Pts',(5.43734568960834,4.03215109350317,48.5059752274374));
#195546=CARTESIAN_POINT('Ctrl Pts',(5.33108105679396,4.1716394130846,48.5141836854509));
#195547=CARTESIAN_POINT('Ctrl Pts',(5.21954606773301,4.30681179607525,48.5223921434645));
#195548=CARTESIAN_POINT('Ctrl Pts',(5.16985479465303,4.36703404429181,48.5260491907476));
#195549=CARTESIAN_POINT('Ctrl Pts',(5.11911797420273,4.42640002356778,48.5297062380307));
#195550=CARTESIAN_POINT('Ctrl Pts',(5.06736777603006,4.48487155027345,48.5333632853138));
#195551=CARTESIAN_POINT('Ctrl Pts',(4.94206285740536,4.62645110270861,48.5422182468095));
#195552=CARTESIAN_POINT('Ctrl Pts',(4.81094435462351,4.76263729323991,48.5510732083052));
#195553=CARTESIAN_POINT('Ctrl Pts',(4.67449614862399,4.89299241328857,48.559928169801));
#195554=CARTESIAN_POINT('Ctrl Pts',(4.53765432310214,5.02372357580485,48.5688086756832));
#195555=CARTESIAN_POINT('Ctrl Pts',(4.39545221729934,5.14858982823487,48.5776891815655));
#195556=CARTESIAN_POINT('Ctrl Pts',(4.24840844994112,5.26719229214853,48.5865696874478));
#195557=CARTESIAN_POINT('Ctrl Pts',(4.10114695216991,5.38597037291365,48.5954633428586));
#195558=CARTESIAN_POINT('Ctrl Pts',(3.94902967639376,5.49846597893295,48.6043569982693));
#195559=CARTESIAN_POINT('Ctrl Pts',(3.7926047418606,5.60432317697833,48.6132506536801));
#195560=CARTESIAN_POINT('Ctrl Pts',(3.63584600571122,5.71040626806245,48.6221632876288));
#195561=CARTESIAN_POINT('Ctrl Pts',(3.47476144378922,5.80982247761136,48.6310759215775));
#195562=CARTESIAN_POINT('Ctrl Pts',(3.30992645411757,5.90226023387081,48.6399885555262));
#195563=CARTESIAN_POINT('Ctrl Pts',(3.24030697252026,5.94130211862853,48.6437528834545));
#195564=CARTESIAN_POINT('Ctrl Pts',(3.17001873308238,5.97909971782621,48.6475172113827));
#195565=CARTESIAN_POINT('Ctrl Pts',(3.09910619832125,6.01563211736945,48.651281539311));
#195566=CARTESIAN_POINT('Origin',(0.,0.,4.30282021618968));
#195567=CARTESIAN_POINT('',(3.0991061983214,6.01563211736937,51.0457552630242));
#195568=CARTESIAN_POINT('',(3.0991061983213,6.01563211736942,50.6516279712835));
#195569=CARTESIAN_POINT('',(3.09910619832133,6.0156321173694,4.30282021618968));
#195570=CARTESIAN_POINT('',(-6.767,4.15111738386043E-13,49.6971797838101));
#195571=CARTESIAN_POINT('Ctrl Pts',(-6.767,4.15112265940911E-13,49.6971797838101));
#195572=CARTESIAN_POINT('Ctrl Pts',(-6.76700000000001,-0.186007249526577,
49.7059292956213));
#195573=CARTESIAN_POINT('Ctrl Pts',(-6.75932637294521,-0.372014355749744,
49.7146788074325));
#195574=CARTESIAN_POINT('Ctrl Pts',(-6.74400518264181,-0.557389537487439,
49.7234283192437));
#195575=CARTESIAN_POINT('Ctrl Pts',(-6.72868405705085,-0.742763936251934,
49.7321777940993));
#195576=CARTESIAN_POINT('Ctrl Pts',(-6.70571545645721,-0.927506130242599,
49.740927268955));
#195577=CARTESIAN_POINT('Ctrl Pts',(-6.67517739404792,-1.11098863990213,
49.7496767438107));
#195578=CARTESIAN_POINT('Ctrl Pts',(-6.6446394580866,-1.29447038982159,
49.7584261824377));
#195579=CARTESIAN_POINT('Ctrl Pts',(-6.60653217008304,-1.47669218313911,
49.7671756210647));
#195580=CARTESIAN_POINT('Ctrl Pts',(-6.56098496092616,-1.65703510599528,
49.7759250596918));
#195581=CARTESIAN_POINT('Ctrl Pts',(-6.51543793658228,-1.83737729708945,
49.7846744628169));
#195582=CARTESIAN_POINT('Ctrl Pts',(-6.46245112167343,-2.01584035511174,
49.7934238659421));
#195583=CARTESIAN_POINT('Ctrl Pts',(-6.40220448374168,-2.1918181376104,
49.8021732690673));
#195584=CARTESIAN_POINT('Ctrl Pts',(-6.34195808526413,-2.36779522067386,
49.8109226374174));
#195585=CARTESIAN_POINT('Ctrl Pts',(-6.27445201433008,-2.54128677684402,
49.8196720057675));
#195586=CARTESIAN_POINT('Ctrl Pts',(-6.19991555071801,-2.71170355385042,
49.8284213741176));
#195587=CARTESIAN_POINT('Ctrl Pts',(-6.12537937716591,-2.88211966767692,
49.8371707084193));
#195588=CARTESIAN_POINT('Ctrl Pts',(-6.04381298052419,-3.04946076371985,
49.8459200427211));
#195589=CARTESIAN_POINT('Ctrl Pts',(-5.95549339335732,-3.21315848374731,
49.8546693770229));
#195590=CARTESIAN_POINT('Ctrl Pts',(-5.86717414255319,-3.37685558033647,
49.8634186780031));
#195591=CARTESIAN_POINT('Ctrl Pts',(-5.7721018887652,-3.53690907646883,
49.8721679789832));
#195592=CARTESIAN_POINT('Ctrl Pts',(-5.67059953346931,-3.69277536969386,
49.8809172799634));
#195593=CARTESIAN_POINT('Ctrl Pts',(-5.56909755631316,-3.84864108225021,
49.8896665483487));
#195594=CARTESIAN_POINT('Ctrl Pts',(-5.4611656819678,-4.00031938297612,
49.898415816734));
#195595=CARTESIAN_POINT('Ctrl Pts',(-5.34717048533531,-4.14729511859947,
49.9071650851192));
#195596=CARTESIAN_POINT('Ctrl Pts',(-5.23317570391759,-4.29427031888012,
49.9159143216363));
#195597=CARTESIAN_POINT('Ctrl Pts',(-5.1131178200343,-4.43654276189644,
49.9246635581533));
#195598=CARTESIAN_POINT('Ctrl Pts',(-4.98740458984663,-4.57362924351951,
49.9334127946704));
#195599=CARTESIAN_POINT('Ctrl Pts',(-4.86169180711654,-4.71071523720358,
49.9421620000458));
#195600=CARTESIAN_POINT('Ctrl Pts',(-4.73032391204085,-4.84261509523323,
49.9509112054212));
#195601=CARTESIAN_POINT('Ctrl Pts',(-4.59374707013515,-4.96888084538408,
49.9596604107967));
#195602=CARTESIAN_POINT('Ctrl Pts',(-4.45717070301353,-5.09514615659545,
49.9684095857571));
#195603=CARTESIAN_POINT('Ctrl Pts',(-4.31538563570941,-5.21577720459611,
49.9771587607176));
#195604=CARTESIAN_POINT('Ctrl Pts',(-4.16887341029401,-5.33036429232971,
49.985907935678));
#195605=CARTESIAN_POINT('Ctrl Pts',(-4.02236168203572,-5.44495099123716,
49.9946570809501));
#195606=CARTESIAN_POINT('Ctrl Pts',(-3.87112305348004,-5.55349359438715,
50.0034062262221));
#195607=CARTESIAN_POINT('Ctrl Pts',(-3.7156711701757,-5.65562346299019,
50.0121553714941));
#195608=CARTESIAN_POINT('Ctrl Pts',(-3.56021980145608,-5.75775299351775,
50.0209044878043));
#195609=CARTESIAN_POINT('Ctrl Pts',(-3.40055544538117,-5.85346967464008,
50.0296536041145));
#195610=CARTESIAN_POINT('Ctrl Pts',(-3.23722035986599,-5.94244842987039,
50.0384027204247));
#195611=CARTESIAN_POINT('Ctrl Pts',(-3.07388580146917,-6.03142689794664,
50.0471518084995));
#195612=CARTESIAN_POINT('Ctrl Pts',(-2.90688078896305,-6.11366734656912,
50.0559008965744));
#195613=CARTESIAN_POINT('Ctrl Pts',(-2.73677250721087,-6.18889046952479,
50.0646499846492));
#195614=CARTESIAN_POINT('Ctrl Pts',(-2.56666476031186,-6.26411335596449,
50.0733990452152));
#195615=CARTESIAN_POINT('Ctrl Pts',(-2.39345402574855,-6.33231884500673,
50.0821481057813));
#195616=CARTESIAN_POINT('Ctrl Pts',(-2.21772856065267,-6.39327529762839,
50.0908971663473));
#195617=CARTESIAN_POINT('Ctrl Pts',(-2.04200363348157,-6.45423156365225,
50.099646200131));
#195618=CARTESIAN_POINT('Ctrl Pts',(-1.8637642618889,-6.5079387437577,50.1083952339147));
#195619=CARTESIAN_POINT('Ctrl Pts',(-1.68361577752734,-6.5542144390965,
50.1171442676984));
#195620=CARTESIAN_POINT('Ctrl Pts',(-1.50346782967389,-6.60048999661961,
50.1258932754263));
#195621=CARTESIAN_POINT('Ctrl Pts',(-1.32141105794587,-6.63933404237792,
50.1346422831541));
#195622=CARTESIAN_POINT('Ctrl Pts',(-1.13806375486633,-6.67061465607627,
50.1433912908819));
#195623=CARTESIAN_POINT('Ctrl Pts',(-0.954716982599113,-6.70189517921352,
50.1521402732803));
#195624=CARTESIAN_POINT('Ctrl Pts',(-0.770079968898227,-6.72561226592273,
50.1608892556787));
#195625=CARTESIAN_POINT('Ctrl Pts',(-0.58477976555433,-6.74168536983136,
50.1696382380771));
#195626=CARTESIAN_POINT('Ctrl Pts',(-0.391489830647433,-6.75845151013875,
50.178764457087));
#195627=CARTESIAN_POINT('Ctrl Pts',(-0.197478578234526,-6.76689983031636,
50.1878906760968));
#195628=CARTESIAN_POINT('Ctrl Pts',(-0.00346287644759543,-6.76699911397118,
50.1970168951067));
#195629=CARTESIAN_POINT('Ctrl Pts',(0.184489834658524,-6.76709529501178,
50.2058579197725));
#195630=CARTESIAN_POINT('Ctrl Pts',(0.372446404253995,-6.75935639738143,
50.2146989444383));
#195631=CARTESIAN_POINT('Ctrl Pts',(0.559755019492944,-6.74380925873148,
50.2235399691041));
#195632=CARTESIAN_POINT('Ctrl Pts',(0.745134705526356,-6.72842222659755,
50.2322899477139));
#195633=CARTESIAN_POINT('Ctrl Pts',(0.929879431233118,-6.7053870605746,
50.2410399263236));
#195634=CARTESIAN_POINT('Ctrl Pts',(1.11336163627277,-6.67478200894052,
50.2497899049334));
#195635=CARTESIAN_POINT('Ctrl Pts',(1.29684196301187,-6.64417727060922,
50.2585397939699));
#195636=CARTESIAN_POINT('Ctrl Pts',(1.47905951217995,-6.60600284890482,
50.2672896830064));
#195637=CARTESIAN_POINT('Ctrl Pts',(1.65939532067585,-6.56038841607104,
50.276039572043));
#195638=CARTESIAN_POINT('Ctrl Pts',(1.83972934301301,-6.51477443503116,
50.2847893744151));
#195639=CARTESIAN_POINT('Ctrl Pts',(2.01818138406762,-6.46172066061986,
50.2935391767873));
#195640=CARTESIAN_POINT('Ctrl Pts',(2.19414528354694,-6.40140730423309,
50.3022889791594));
#195641=CARTESIAN_POINT('Ctrl Pts',(2.37010749864485,-6.3410945251846,50.3110386977758));
#195642=CARTESIAN_POINT('Ctrl Pts',(2.54358134866937,-6.2735223961631,50.3197884163921));
#195643=CARTESIAN_POINT('Ctrl Pts',(2.71397759436023,-6.19892043966614,
50.3285381350084));
#195644=CARTESIAN_POINT('Ctrl Pts',(2.88437226558593,-6.12431917249294,
50.3372877727771));
#195645=CARTESIAN_POINT('Ctrl Pts',(3.05168912681427,-6.04268832278561,
50.3460374105458));
#195646=CARTESIAN_POINT('Ctrl Pts',(3.21535986274326,-5.95430516123079,
50.3547870483145));
#195647=CARTESIAN_POINT('Ctrl Pts',(3.37902914073314,-5.86592278697169,
50.3635366081436));
#195648=CARTESIAN_POINT('Ctrl Pts',(3.53905210622044,-5.77078835741652,
50.3722861679727));
#195649=CARTESIAN_POINT('Ctrl Pts',(3.69488522832168,-5.66922500431322,
50.3810357278018));
#195650=CARTESIAN_POINT('Ctrl Pts',(3.85071701407415,-5.56766252216765,
50.3897852125989));
#195651=CARTESIAN_POINT('Ctrl Pts',(4.00235878822881,-5.45967138329021,
50.398534697396));
#195652=CARTESIAN_POINT('Ctrl Pts',(4.14929549611804,-5.34561838199236,
50.4072841821931));
#195653=CARTESIAN_POINT('Ctrl Pts',(4.29623099276555,-5.23156632086633,
50.4160335948657));
#195654=CARTESIAN_POINT('Ctrl Pts',(4.4384612743648,-5.11145267304571,50.4247830075383));
#195655=CARTESIAN_POINT('Ctrl Pts',(4.57550326054881,-4.98568540049482,
50.4335324202109));
#195656=CARTESIAN_POINT('Ctrl Pts',(4.71254416258202,-4.85991912289951,
50.4422817636661));
#195657=CARTESIAN_POINT('Ctrl Pts',(4.84439664019166,-4.72849950385004,
50.4510311071214));
#195658=CARTESIAN_POINT('Ctrl Pts',(4.97061286795133,-4.59187289860648,
50.4597804505766));
#195659=CARTESIAN_POINT('Ctrl Pts',(5.09682813913056,-4.45524732884259,
50.4685297277214));
#195660=CARTESIAN_POINT('Ctrl Pts',(5.21740705148195,-4.31341506235357,
50.4772790048663));
#195661=CARTESIAN_POINT('Ctrl Pts',(5.33194007546036,-4.16685781275289,
50.4860282820111));
#195662=CARTESIAN_POINT('Ctrl Pts',(5.4464722694481,-4.02030162521402,50.4947774957522));
#195663=CARTESIAN_POINT('Ctrl Pts',(5.55495848628422,-3.86902074887491,
50.5035267094933));
#195664=CARTESIAN_POINT('Ctrl Pts',(5.65703027292081,-3.71352898080216,
50.5122759232344));
#195665=CARTESIAN_POINT('Ctrl Pts',(5.75910135377274,-3.55803828789139,
50.5210250764783));
#195666=CARTESIAN_POINT('Ctrl Pts',(5.85475793593014,-3.39833700106261,
50.5297742297222));
#195667=CARTESIAN_POINT('Ctrl Pts',(5.94367514427645,-3.23496750823101,
50.5385233829661));
#195668=CARTESIAN_POINT('Ctrl Pts',(6.03259176732873,-3.07159909077266,
50.547272478619));
#195669=CARTESIAN_POINT('Ctrl Pts',(6.11476896836145,-2.9045627673097,50.5560215742719));
#195670=CARTESIAN_POINT('Ctrl Pts',(6.18992765548094,-2.7344258300258,50.5647706699249));
#195671=CARTESIAN_POINT('Ctrl Pts',(6.26508587283255,-2.5642899561568,50.5735197108929));
#195672=CARTESIAN_POINT('Ctrl Pts',(6.33322554827353,-2.39105376934691,
50.5822687518609));
#195673=CARTESIAN_POINT('Ctrl Pts',(6.39411526733215,-2.21530561053548,
50.591017792829));
#195674=CARTESIAN_POINT('Ctrl Pts',(6.45500462603017,-2.03955849184561,
50.599766782018));
#195675=CARTESIAN_POINT('Ctrl Pts',(6.50864402040895,-1.86129970164003,
50.608515771207));
#195676=CARTESIAN_POINT('Ctrl Pts',(6.55485128368741,-1.68113463135513,
50.6172647603961));
#195677=CARTESIAN_POINT('Ctrl Pts',(6.60199809554445,-1.49730620116344,
50.6261916458675));
#195678=CARTESIAN_POINT('Ctrl Pts',(6.64140720707972,-1.31149343245196,
50.6351185313389));
#195679=CARTESIAN_POINT('Ctrl Pts',(6.67293928722964,-1.12435326697046,
50.6440454168103));
#195680=CARTESIAN_POINT('Ctrl Pts',(6.70384625876323,-0.940923067001829,
50.6527953309878));
#195681=CARTESIAN_POINT('Ctrl Pts',(6.72718554579849,-0.756217899516949,
50.6615452451653));
#195682=CARTESIAN_POINT('Ctrl Pts',(6.74287786815367,-0.57086518124983,
50.6702951593427));
#195683=CARTESIAN_POINT('Ctrl Pts',(6.75856988190872,-0.385516108069375,
50.6790449014472));
#195684=CARTESIAN_POINT('Ctrl Pts',(6.76661520773416,-0.199519795221876,
50.6877946435517));
#195685=CARTESIAN_POINT('Ctrl Pts',(6.7669865178958,-0.0135080204512824,
50.6965443856562));
#195686=CARTESIAN_POINT('Ctrl Pts',(6.76735782124892,0.172500343517284,
50.7052939673211));
#195687=CARTESIAN_POINT('Ctrl Pts',(6.76005538995161,0.358523882215196,
50.7140435489861));
#195688=CARTESIAN_POINT('Ctrl Pts',(6.74510402742327,0.5439307485686,50.7227931306511));
#195689=CARTESIAN_POINT('Ctrl Pts',(6.73015291917986,0.729334461619347,
50.7315425635077));
#195690=CARTESIAN_POINT('Ctrl Pts',(6.7075531630654,0.914121237638676,50.7402919963644));
#195691=CARTESIAN_POINT('Ctrl Pts',(6.6773815187451,1.09766345166509,50.7490414292211));
#195692=CARTESIAN_POINT('Ctrl Pts',(6.64721034747495,1.28120278800047,50.7577907248986));
#195693=CARTESIAN_POINT('Ctrl Pts',(6.60946757205058,1.46349731860706,50.7665400205762));
#195694=CARTESIAN_POINT('Ctrl Pts',(6.5642813811143,1.64392790278533,50.7752893162537));
#195695=CARTESIAN_POINT('Ctrl Pts',(6.51909583859747,1.82435589779423,50.7840384863793));
#195696=CARTESIAN_POINT('Ctrl Pts',(6.46646716392763,2.00291972192628,50.7927876565049));
#195697=CARTESIAN_POINT('Ctrl Pts',(6.40657409872762,2.17901292275022,50.8015368266305));
#195698=CARTESIAN_POINT('Ctrl Pts',(6.34668181341944,2.35510383059333,50.8102858828296));
#195699=CARTESIAN_POINT('Ctrl Pts',(6.27952541913908,2.52872390822933,50.8190349390287));
#195700=CARTESIAN_POINT('Ctrl Pts',(6.20533299175365,2.69928350890634,50.8277839952278));
#195701=CARTESIAN_POINT('Ctrl Pts',(6.12831602991392,2.87633637965956,50.836866131386));
#195702=CARTESIAN_POINT('Ctrl Pts',(6.0437169060511,3.05009086601779,50.8459482675442));
#195703=CARTESIAN_POINT('Ctrl Pts',(5.95184520316468,3.21991112883036,50.8550304037024));
#195704=CARTESIAN_POINT('Ctrl Pts',(5.863335495091,3.38351691183319,50.8637801840459));
#195705=CARTESIAN_POINT('Ctrl Pts',(5.76807618099183,3.54347103712307,50.8725299643895));
#195706=CARTESIAN_POINT('Ctrl Pts',(5.66639083308818,3.69923018027997,50.8812797447331));
#195707=CARTESIAN_POINT('Ctrl Pts',(5.5647091408199,3.85498372382354,50.890029210518));
#195708=CARTESIAN_POINT('Ctrl Pts',(5.45660203371843,4.00654234702303,50.8987786763029));
#195709=CARTESIAN_POINT('Ctrl Pts',(5.34243669838979,4.15339127986974,50.9075281420878));
#195710=CARTESIAN_POINT('Ctrl Pts',(5.22827486050342,4.30023571401583,50.9162773398338));
#195711=CARTESIAN_POINT('Ctrl Pts',(5.1080553416685,4.4423705202877,50.9250265375798));
#195712=CARTESIAN_POINT('Ctrl Pts',(4.98218644339678,4.57931296629018,50.9337757353259));
#195713=CARTESIAN_POINT('Ctrl Pts',(4.85632073219318,4.71625194483636,50.9425247115375));
#195714=CARTESIAN_POINT('Ctrl Pts',(4.72480612170057,4.84799861524763,50.9512736877491));
#195715=CARTESIAN_POINT('Ctrl Pts',(4.58808925235057,4.9741055489872,50.9600226639607));
#195716=CARTESIAN_POINT('Ctrl Pts',(4.45136349473788,5.10022068121433,50.9687722089624));
#195717=CARTESIAN_POINT('Ctrl Pts',(4.30943501209815,5.22069514872053,50.9775217539641));
#195718=CARTESIAN_POINT('Ctrl Pts',(4.16278587431512,5.33511975166467,50.9862712989658));
#195719=CARTESIAN_POINT('Ctrl Pts',(4.01614535740155,5.44953762808059,50.9950203296196));
#195720=CARTESIAN_POINT('Ctrl Pts',(3.86478496657606,5.55790617533005,51.0037693602733));
#195721=CARTESIAN_POINT('Ctrl Pts',(3.70921874746854,5.6598573553958,51.0125183909271));
#195722=CARTESIAN_POINT('Ctrl Pts',(3.5536504160555,5.76180991977263,51.0212675403767));
#195723=CARTESIAN_POINT('Ctrl Pts',(3.39387638174163,5.85734478553022,51.0300166898263));
#195724=CARTESIAN_POINT('Ctrl Pts',(3.2304392790417,5.94613749121432,51.0387658392759));
#195725=CARTESIAN_POINT('Ctrl Pts',(3.18691767070183,5.96978206944278,51.041095647192));
#195726=CARTESIAN_POINT('Ctrl Pts',(3.14313645919507,5.99294880633489,51.0434254551081));
#195727=CARTESIAN_POINT('Ctrl Pts',(3.0991061983214,6.01563211736937,51.0457552630242));
#195728=CARTESIAN_POINT('Ctrl Pts',(3.09910619832136,6.01563211736939,49.0458451349191));
#195729=CARTESIAN_POINT('Ctrl Pts',(2.93972393993817,6.09774194975618,49.0542783857431));
#195730=CARTESIAN_POINT('Ctrl Pts',(2.77698811596646,6.17355927733608,49.0627116365671));
#195731=CARTESIAN_POINT('Ctrl Pts',(2.61142360477587,6.2428163321068,49.071144887391));
#195732=CARTESIAN_POINT('Ctrl Pts',(2.44594307296802,6.31203825758159,49.0795738606123));
#195733=CARTESIAN_POINT('Ctrl Pts',(2.27763701902433,6.37470641533421,49.0880028338337));
#195734=CARTESIAN_POINT('Ctrl Pts',(2.10705228741077,6.43060025643929,49.096431807055));
#195735=CARTESIAN_POINT('Ctrl Pts',(1.93652970878945,6.48647373247746,49.1048577091579));
#195736=CARTESIAN_POINT('Ctrl Pts',(1.76373042213216,6.53557770896233,49.1132836112607));
#195737=CARTESIAN_POINT('Ctrl Pts',(1.58921888533647,6.57774067096674,49.1217095133636));
#195738=CARTESIAN_POINT('Ctrl Pts',(1.43181293445047,6.61577082787403,49.1293095102288));
#195739=CARTESIAN_POINT('Ctrl Pts',(1.27301434684598,6.64815456842155,49.1369095070939));
#195740=CARTESIAN_POINT('Ctrl Pts',(1.11324685211149,6.67480115406174,49.1445095039591));
#195741=CARTESIAN_POINT('Ctrl Pts',(0.932062430270227,6.70501973025763,
49.1531282848963));
#195742=CARTESIAN_POINT('Ctrl Pts',(0.74971304937296,6.72784574542047,49.1617470658335));
#195743=CARTESIAN_POINT('Ctrl Pts',(0.566812338184386,6.74321976308662,
49.1703658467708));
#195744=CARTESIAN_POINT('Ctrl Pts',(0.383801759648514,6.75860301583188,
49.1789898049574));
#195745=CARTESIAN_POINT('Ctrl Pts',(0.200239492989446,6.76652531212785,
49.187613763144));
#195746=CARTESIAN_POINT('Ctrl Pts',(0.0167416779525153,6.7669792903643,
49.1962377213307));
#195747=CARTESIAN_POINT('Ctrl Pts',(-0.173385287049673,6.76744966928547,
49.2051732337018));
#195748=CARTESIAN_POINT('Ctrl Pts',(-0.363442695548515,6.75990206500124,
49.2141087460728));
#195749=CARTESIAN_POINT('Ctrl Pts',(-0.552748818302166,6.74438712885504,
49.2230442584439));
#195750=CARTESIAN_POINT('Ctrl Pts',(-0.735796005282449,6.72938515545645,
49.2316843403386));
#195751=CARTESIAN_POINT('Ctrl Pts',(-0.918140493494802,6.70693434116502,
49.2403244222333));
#195752=CARTESIAN_POINT('Ctrl Pts',(-1.09917392994075,6.67713304283647,
49.248964504128));
#195753=CARTESIAN_POINT('Ctrl Pts',(-1.28949248573411,6.64580325000922,
49.2580477317373));
#195754=CARTESIAN_POINT('Ctrl Pts',(-1.47836158572741,6.60634924265721,
49.2671309593466));
#195755=CARTESIAN_POINT('Ctrl Pts',(-1.66508915912587,6.55894557777098,
49.2762141869559));
#195756=CARTESIAN_POINT('Ctrl Pts',(-1.85181673252427,6.51154191288477,
49.2852974145652));
#195757=CARTESIAN_POINT('Ctrl Pts',(-2.03640241756047,6.45618873408586,
49.2943806421744));
#195758=CARTESIAN_POINT('Ctrl Pts',(-2.21817473501047,6.39312050918495,
49.3034638697837));
#195759=CARTESIAN_POINT('Ctrl Pts',(-2.39917393912359,6.33032052582097,
49.3125084646435));
#195760=CARTESIAN_POINT('Ctrl Pts',(-2.57755109173786,6.25981381777489,
49.3215530595033));
#195761=CARTESIAN_POINT('Ctrl Pts',(-2.75267595307432,6.18183339288325,
49.3305976543631));
#195762=CARTESIAN_POINT('Ctrl Pts',(-2.92764010978414,6.10392452730633,
49.3396339493834));
#195763=CARTESIAN_POINT('Ctrl Pts',(-3.09935771662874,6.0185557342239,49.3486702444037));
#195764=CARTESIAN_POINT('Ctrl Pts',(-3.26721867963455,5.92600802391012,
49.357706539424));
#195765=CARTESIAN_POINT('Ctrl Pts',(-3.43478259950343,5.8336240840269,49.3667268440117));
#195766=CARTESIAN_POINT('Ctrl Pts',(-3.59850329539956,5.73408670920529,
49.3757471485994));
#195767=CARTESIAN_POINT('Ctrl Pts',(-3.75779556841933,5.62772258253443,
49.3847674531871));
#195768=CARTESIAN_POINT('Ctrl Pts',(-3.91688724376425,5.52149240081956,
49.3937763984534));
#195769=CARTESIAN_POINT('Ctrl Pts',(-4.07156142823421,5.40845275555742,
49.4027853437196));
#195770=CARTESIAN_POINT('Ctrl Pts',(-4.22125999304436,5.28897467106084,
49.4117942889859));
#195771=CARTESIAN_POINT('Ctrl Pts',(-4.37061862410423,5.16976789600128,
49.4207827768446));
#195772=CARTESIAN_POINT('Ctrl Pts',(-4.51502400285251,5.04415201327701,
49.4297712647034));
#195773=CARTESIAN_POINT('Ctrl Pts',(-4.65394968488556,4.91253919379313,
49.4387597525621));
#195774=CARTESIAN_POINT('Ctrl Pts',(-4.77583785060568,4.79706705849472,
49.4466459135776));
#195775=CARTESIAN_POINT('Ctrl Pts',(-4.89350826159656,4.67697938905811,
49.454532074593));
#195776=CARTESIAN_POINT('Ctrl Pts',(-5.00662498621481,4.55258116318749,
49.4624182356085));
#195777=CARTESIAN_POINT('Ctrl Pts',(-5.12311683843922,4.42447119718552,
49.4705397004647));
#195778=CARTESIAN_POINT('Ctrl Pts',(-5.23472585164597,4.2918458514551,49.4786611653208));
#195779=CARTESIAN_POINT('Ctrl Pts',(-5.34109011845018,4.15512278357618,
49.486782630177));
#195780=CARTESIAN_POINT('Ctrl Pts',(-5.44744679991717,4.01840946606368,
49.4949035158532));
#195781=CARTESIAN_POINT('Ctrl Pts',(-5.54855925514299,3.87759929750489,
49.5030244015295));
#195782=CARTESIAN_POINT('Ctrl Pts',(-5.64410649347399,3.7331422274439,49.5111452872057));
#195783=CARTESIAN_POINT('Ctrl Pts',(-5.73966515243256,3.58866789063165,
49.51926714356));
#195784=CARTESIAN_POINT('Ctrl Pts',(-5.82965706891732,3.44054609040245,
49.5273889999143));
#195785=CARTESIAN_POINT('Ctrl Pts',(-5.91380516494978,3.28925485042028,
49.5355108562687));
#195786=CARTESIAN_POINT('Ctrl Pts',(-5.9980146543913,3.1378532302225,49.5436386382288));
#195787=CARTESIAN_POINT('Ctrl Pts',(-6.07637162967551,2.98327787215715,
49.551766420189));
#195788=CARTESIAN_POINT('Ctrl Pts',(-6.14864519539981,2.82603100851474,
49.5598942021491));
#195789=CARTESIAN_POINT('Ctrl Pts',(-6.2209482026883,2.66872008834513,49.5680252950656));
#195790=CARTESIAN_POINT('Ctrl Pts',(-6.28716272081908,2.50873583148082,
49.576156387982));
#195791=CARTESIAN_POINT('Ctrl Pts',(-6.347106525167,2.3465991899305,49.5842874808984));
#195792=CARTESIAN_POINT('Ctrl Pts',(-6.4071157556725,2.18428558301114,49.5924274485629));
#195793=CARTESIAN_POINT('Ctrl Pts',(-6.46084048863694,2.0198152468596,49.6005674162275));
#195794=CARTESIAN_POINT('Ctrl Pts',(-6.50814853973555,1.85372370776716,
49.608707383892));
#195795=CARTESIAN_POINT('Ctrl Pts',(-6.53268454050372,1.76758145425806,
49.6129291230724));
#195796=CARTESIAN_POINT('Ctrl Pts',(-6.55549535098424,1.68100328982057,
49.6171508622528));
#195797=CARTESIAN_POINT('Ctrl Pts',(-6.57656798188356,1.59406479782472,
49.6213726014332));
#195798=CARTESIAN_POINT('Ctrl Pts',(-6.63298328035275,1.3613145068032,49.6326749716525));
#195799=CARTESIAN_POINT('Ctrl Pts',(-6.67701699606666,1.12565713650379,
49.6439773418719));
#195800=CARTESIAN_POINT('Ctrl Pts',(-6.70845565815198,0.888207004368171,
49.6552797120912));
#195801=CARTESIAN_POINT('Ctrl Pts',(-6.73942658159803,0.654289611679238,
49.6664139277227));
#195802=CARTESIAN_POINT('Ctrl Pts',(-6.75817455604823,0.418631866523409,
49.6775481433541));
#195803=CARTESIAN_POINT('Ctrl Pts',(-6.76454365156374,0.182313428163557,
49.6886823589856));
#195804=CARTESIAN_POINT('Ctrl Pts',(-6.7661639096982,0.1221954928707,49.6915148339271));
#195805=CARTESIAN_POINT('Ctrl Pts',(-6.76698329674138,0.0620348961955091,
49.6943473088686));
#195806=CARTESIAN_POINT('Ctrl Pts',(-6.76699974721993,0.00184962846154336,
49.6971797838101));
#195807=CARTESIAN_POINT('',(-6.76699653643252,-0.00684659844694554,49.302820216166));
#195808=CARTESIAN_POINT('Ctrl Pts',(3.09910619832125,6.01563211736945,48.651281539311));
#195809=CARTESIAN_POINT('Ctrl Pts',(2.93077649148675,6.10235145585861,48.6602171699259));
#195810=CARTESIAN_POINT('Ctrl Pts',(2.75892788574672,6.18193830383501,48.6691528005408));
#195811=CARTESIAN_POINT('Ctrl Pts',(2.58416789816994,6.25414784555562,48.6780884311557));
#195812=CARTESIAN_POINT('Ctrl Pts',(2.4914045027765,6.29247699837079,48.6828315044834));
#195813=CARTESIAN_POINT('Ctrl Pts',(2.39782110739142,6.32872840195926,48.687574577811));
#195814=CARTESIAN_POINT('Ctrl Pts',(2.30351033261469,6.36287114025872,48.6923176511387));
#195815=CARTESIAN_POINT('Ctrl Pts',(2.14001054988095,6.42206194117319,48.7005403750046));
#195816=CARTESIAN_POINT('Ctrl Pts',(1.97401030601349,6.47502553674889,48.7087630988705));
#195817=CARTESIAN_POINT('Ctrl Pts',(1.80602453028676,6.52154616605621,48.7169858227363));
#195818=CARTESIAN_POINT('Ctrl Pts',(1.63821656181282,6.56801755485339,48.7251998431276));
#195819=CARTESIAN_POINT('Ctrl Pts',(1.46842758931484,6.60805946257521,48.7334138635188));
#195820=CARTESIAN_POINT('Ctrl Pts',(1.297191299762,6.64150462860802,48.74162788391));
#195821=CARTESIAN_POINT('Ctrl Pts',(1.12610187861514,6.67492110890934,48.749834859182));
#195822=CARTESIAN_POINT('Ctrl Pts',(0.953567962756425,6.70175204751753,
48.7580418344539));
#195823=CARTESIAN_POINT('Ctrl Pts',(0.78013723004385,6.72188031002483,48.7662488097259));
#195824=CARTESIAN_POINT('Ctrl Pts',(0.60682043786161,6.74199534866536,48.7744503931789));
#195825=CARTESIAN_POINT('Ctrl Pts',(0.43260835747718,6.75541644128931,48.7826519766319));
#195826=CARTESIAN_POINT('Ctrl Pts',(0.258057753170527,6.76207772774231,
48.7908535600849));
#195827=CARTESIAN_POINT('Ctrl Pts',(0.0835867974835264,6.76873597460531,
48.7990514011));
#195828=CARTESIAN_POINT('Ctrl Pts',(-0.091222016658833,6.76864054681347,
48.807249242115));
#195829=CARTESIAN_POINT('Ctrl Pts',(-0.265807832575272,6.76177751749802,
48.8154470831301));
#195830=CARTESIAN_POINT('Ctrl Pts',(-0.440378241837691,6.75491509382351,
48.8236442007112));
#195831=CARTESIAN_POINT('Ctrl Pts',(-0.614725333558899,6.74128626371388,
48.8318413182924));
#195832=CARTESIAN_POINT('Ctrl Pts',(-0.78828891228321,6.72092922078275,
48.8400384358735));
#195833=CARTESIAN_POINT('Ctrl Pts',(-0.961850559919425,6.70057240434639,
48.8482354622526));
#195834=CARTESIAN_POINT('Ctrl Pts',(-1.13462835540743,6.67348756492386,
48.8564324886317));
#195835=CARTESIAN_POINT('Ctrl Pts',(-1.30606800359344,6.63976470742672,
48.8646295150108));
#195836=CARTESIAN_POINT('Ctrl Pts',(-1.477536917252,6.60603609329528,48.872827940657));
#195837=CARTESIAN_POINT('Ctrl Pts',(-1.64766687641729,6.56566727280108,
48.8810263663031));
#195838=CARTESIAN_POINT('Ctrl Pts',(-1.81591449286919,6.51879924177664,
48.8892247919493));
#195839=CARTESIAN_POINT('Ctrl Pts',(-1.98422142275158,6.47191468805928,
48.8974261078399));
#195840=CARTESIAN_POINT('Ctrl Pts',(-2.15064434257303,6.41852645593345,
48.9056274237306));
#195841=CARTESIAN_POINT('Ctrl Pts',(-2.31465567054109,6.35882521593667,
48.9138287396212));
#195842=CARTESIAN_POINT('Ctrl Pts',(-2.47885377995708,6.2990559862212,48.9220393954378));
#195843=CARTESIAN_POINT('Ctrl Pts',(-2.64063447316435,6.23295950824151,
48.9302500512544));
#195844=CARTESIAN_POINT('Ctrl Pts',(-2.79948980530397,6.16077477513982,
48.938460707071));
#195845=CARTESIAN_POINT('Ctrl Pts',(-2.95843874704228,6.08854750532372,
48.9466762012282));
#195846=CARTESIAN_POINT('Ctrl Pts',(-3.11445857133242,6.01022498965705,
48.9548916953853));
#195847=CARTESIAN_POINT('Ctrl Pts',(-3.26706666612296,5.92609183181532,
48.9631071895425));
#195848=CARTESIAN_POINT('Ctrl Pts',(-3.41991153518071,5.84182813983106,
48.97133543019));
#195849=CARTESIAN_POINT('Ctrl Pts',(-3.56933378942484,5.75173597467379,
48.9795636708375));
#195850=CARTESIAN_POINT('Ctrl Pts',(-3.71487937457066,5.65614358307757,
48.987791911485));
#195851=CARTESIAN_POINT('Ctrl Pts',(-3.84715707495859,5.569265360545,48.9952700685861));
#195852=CARTESIAN_POINT('Ctrl Pts',(-3.97623291515218,5.47784464897183,
49.0027482256872));
#195853=CARTESIAN_POINT('Ctrl Pts',(-4.10179094787334,5.38215570379976,
49.0102263827882));
#195854=CARTESIAN_POINT('Ctrl Pts',(-4.23590552294086,5.27994573807888,
49.0182141621454));
#195855=CARTESIAN_POINT('Ctrl Pts',(-4.36646292588354,5.17251694764452,
49.0262019415026));
#195856=CARTESIAN_POINT('Ctrl Pts',(-4.49301282143286,5.06015066835365,
49.0341897208598));
#195857=CARTESIAN_POINT('Ctrl Pts',(-4.61940527170978,4.94792418798854,
49.0421675623337));
#195858=CARTESIAN_POINT('Ctrl Pts',(-4.74179985130257,4.83077268635996,
49.0501454038076));
#195859=CARTESIAN_POINT('Ctrl Pts',(-4.85977478472476,4.70902092177912,
49.0581232452815));
#195860=CARTESIAN_POINT('Ctrl Pts',(-4.97762971433009,4.58739300279864,
49.0660929717143));
#195861=CARTESIAN_POINT('Ctrl Pts',(-5.09107367901489,4.46117440049268,
49.0740626981471));
#195862=CARTESIAN_POINT('Ctrl Pts',(-5.1997177893047,4.33073018226584,49.08203242458));
#195863=CARTESIAN_POINT('Ctrl Pts',(-5.30827596765968,4.20038913874426,
49.0899958473668));
#195864=CARTESIAN_POINT('Ctrl Pts',(-5.41204160340074,4.06582942009886,
49.0979592701536));
#195865=CARTESIAN_POINT('Ctrl Pts',(-5.51066267351968,3.92745285123539,
49.1059226929404));
#195866=CARTESIAN_POINT('Ctrl Pts',(-5.61226389954651,3.78489478496254,
49.1141267564082));
#195867=CARTESIAN_POINT('Ctrl Pts',(-5.70840444721114,3.63828584246661,
49.1223308198759));
#195868=CARTESIAN_POINT('Ctrl Pts',(-5.79874377347859,3.48810258586861,
49.1305348833436));
#195869=CARTESIAN_POINT('Ctrl Pts',(-5.88636446989879,3.34243887464265,
49.1384920575248));
#195870=CARTESIAN_POINT('Ctrl Pts',(-5.96852785293425,3.19341322025949,
49.1464492317059));
#195871=CARTESIAN_POINT('Ctrl Pts',(-6.0449672588425,3.0414897401639,49.1544064058871));
#195872=CARTESIAN_POINT('Ctrl Pts',(-6.12140210458061,2.88957532341604,
49.1623631053645));
#195873=CARTESIAN_POINT('Ctrl Pts',(-6.19211348109745,2.7347637646725,49.170319804842));
#195874=CARTESIAN_POINT('Ctrl Pts',(-6.25688109669869,2.57754300483516,
49.1782765043194));
#195875=CARTESIAN_POINT('Ctrl Pts',(-6.32165806836643,2.42029953352586,
49.1862343531894));
#195876=CARTESIAN_POINT('Ctrl Pts',(-6.38048942633366,2.260646520787,49.1941922020593));
#195877=CARTESIAN_POINT('Ctrl Pts',(-6.43320345590825,2.09909082578392,
49.2021500509292));
#195878=CARTESIAN_POINT('Ctrl Pts',(-6.48593586589165,1.93747879929292,
49.2101106745541));
#195879=CARTESIAN_POINT('Ctrl Pts',(-6.53254658668755,1.77396313228821,
49.218071298179));
#195880=CARTESIAN_POINT('Ctrl Pts',(-6.57291415283513,1.60906449201382,
49.2260319218039));
#195881=CARTESIAN_POINT('Ctrl Pts',(-6.61332397791934,1.44399322698504,
49.2340008790373));
#195882=CARTESIAN_POINT('Ctrl Pts',(-6.64747751440874,1.27753646868631,
49.2419698362706));
#195883=CARTESIAN_POINT('Ctrl Pts',(-6.67530457567069,1.11022422151113,
49.2499387935039));
#195884=CARTESIAN_POINT('Ctrl Pts',(-6.70314910520335,0.942806945076842,
49.2579127532023));
#195885=CARTESIAN_POINT('Ctrl Pts',(-6.72465920715327,0.774533486416592,
49.2658867129007));
#195886=CARTESIAN_POINT('Ctrl Pts',(-6.73981672788629,0.605936856862318,
49.2738606725991));
#195887=CARTESIAN_POINT('Ctrl Pts',(-6.75499391063842,0.437121527283789,
49.2818449759514));
#195888=CARTESIAN_POINT('Ctrl Pts',(-6.76380205298423,0.267982567572156,
49.2898292793037));
#195889=CARTESIAN_POINT('Ctrl Pts',(-6.76627503343266,0.0990513601414978,
49.2978135826559));
#195890=CARTESIAN_POINT('Ctrl Pts',(-6.76679193541882,0.0637413856120705,
49.2994824604926));
#195891=CARTESIAN_POINT('Ctrl Pts',(-6.76703223858502,0.0284404633191816,
49.3011513383293));
#195892=CARTESIAN_POINT('Ctrl Pts',(-6.76699653643252,-0.0068465984469402,
49.302820216166));
#195893=CARTESIAN_POINT('Ctrl Pts',(-6.76699653643201,-0.00684659895290697,
49.3028202161899));
#195894=CARTESIAN_POINT('Ctrl Pts',(-6.76681601664308,-0.185267563115419,
49.3112585156058));
#195895=CARTESIAN_POINT('Ctrl Pts',(-6.75957966634908,-0.36344495759579,
49.3196968150218));
#195896=CARTESIAN_POINT('Ctrl Pts',(-6.74534153478688,-0.540977429361874,
49.3281351144377));
#195897=CARTESIAN_POINT('Ctrl Pts',(-6.73128120881953,-0.716292878015842,
49.3364680364845));
#195898=CARTESIAN_POINT('Ctrl Pts',(-6.7103637057022,-0.891284955468209,
49.3448009585312));
#195899=CARTESIAN_POINT('Ctrl Pts',(-6.68260769154779,-1.06538417524681,
49.3531338805779));
#195900=CARTESIAN_POINT('Ctrl Pts',(-6.65488447827121,-1.23927765196715,
49.3614569551315));
#195901=CARTESIAN_POINT('Ctrl Pts',(-6.62033890717343,-1.41228003226213,
49.3697800296851));
#195902=CARTESIAN_POINT('Ctrl Pts',(-6.57904153321619,-1.58382496009386,
49.3781031042387));
#195903=CARTESIAN_POINT('Ctrl Pts',(-6.5377853823702,-1.75519865147726,
49.3864178706847));
#195904=CARTESIAN_POINT('Ctrl Pts',(-6.48979093716717,-1.92511745270927,
49.3947326371306));
#195905=CARTESIAN_POINT('Ctrl Pts',(-6.43518015765482,-2.09302301433256,
49.4030474035766));
#195906=CARTESIAN_POINT('Ctrl Pts',(-6.38061387326331,-2.26079177186109,
49.4113553954161));
#195907=CARTESIAN_POINT('Ctrl Pts',(-6.31944210328963,-2.42655022880255,
49.4196633872557));
#195908=CARTESIAN_POINT('Ctrl Pts',(-6.25183726416639,-2.58975284967129,
49.4279713790952));
#195909=CARTESIAN_POINT('Ctrl Pts',(-6.18427511306904,-2.75285241877931,
49.4362741249823));
#195910=CARTESIAN_POINT('Ctrl Pts',(-6.11028812081249,-2.91339904746005,
49.4445768708694));
#195911=CARTESIAN_POINT('Ctrl Pts',(-6.03009775559501,-3.07086470850933,
49.4528796167565));
#195912=CARTESIAN_POINT('Ctrl Pts',(-5.94994016162442,-3.22826601836078,
49.461178969576));
#195913=CARTESIAN_POINT('Ctrl Pts',(-5.86358440374889,-3.38258855986731,
49.4694783223954));
#195914=CARTESIAN_POINT('Ctrl Pts',(-5.77129918736136,-3.53332629259769,
49.4777776752149));
#195915=CARTESIAN_POINT('Ctrl Pts',(-5.67903359849096,-3.68403196594145,
49.4860752629012));
#195916=CARTESIAN_POINT('Ctrl Pts',(-5.58084124504725,-3.83115405289675,
49.4943728505875));
#195917=CARTESIAN_POINT('Ctrl Pts',(-5.47703582137325,-3.97421282915174,
49.5026704382739));
#195918=CARTESIAN_POINT('Ctrl Pts',(-5.3732352254783,-4.11726495203411,
49.5109676400563));
#195919=CARTESIAN_POINT('Ctrl Pts',(-5.26382228400117,-4.25625385932584,
49.5192648418387));
#195920=CARTESIAN_POINT('Ctrl Pts',(-5.14915299918866,-4.39073027991318,
49.5275620436212));
#195921=CARTESIAN_POINT('Ctrl Pts',(-5.0344699930639,-4.52522279193214,
49.5358602382457));
#195922=CARTESIAN_POINT('Ctrl Pts',(-4.91452961647778,-4.65520147698483,
49.5441584328702));
#195923=CARTESIAN_POINT('Ctrl Pts',(-4.78972711030074,-4.78025137506912,
49.5524566274948));
#195924=CARTESIAN_POINT('Ctrl Pts',(-4.66483682906601,-4.9053892222047,
49.5607606583364));
#195925=CARTESIAN_POINT('Ctrl Pts',(-4.53507783128464,-5.02559110912605,
49.569064689178));
#195926=CARTESIAN_POINT('Ctrl Pts',(-4.40088171503481,-5.14047946501806,
49.5773687200195));
#195927=CARTESIAN_POINT('Ctrl Pts',(-4.26663680138383,-5.25540959747817,
49.5856757704353));
#195928=CARTESIAN_POINT('Ctrl Pts',(-4.12795182248836,-5.36502212728453,
49.593982820851));
#195929=CARTESIAN_POINT('Ctrl Pts',(-3.9852903595932,-5.46898068653872,
49.6022898712667));
#195930=CARTESIAN_POINT('Ctrl Pts',(-3.84247636751682,-5.57305039503813,
49.6106058033214));
#195931=CARTESIAN_POINT('Ctrl Pts',(-3.6956776825091,-5.67145385588585,
49.618921735376));
#195932=CARTESIAN_POINT('Ctrl Pts',(-3.54538660039247,-5.76389823416041,
49.6272376674306));
#195933=CARTESIAN_POINT('Ctrl Pts',(-3.43209399040731,-5.83358477008577,
49.6335063936495));
#195934=CARTESIAN_POINT('Ctrl Pts',(-3.3168174287625,-5.89988598161268,
49.6397751198684));
#195935=CARTESIAN_POINT('Ctrl Pts',(-3.19977640156996,-5.96269402031968,
49.6460438460873));
#195936=CARTESIAN_POINT('Ctrl Pts',(-3.04200461558026,-6.04735951479634,
49.6544941148106));
#195937=CARTESIAN_POINT('Ctrl Pts',(-2.88073650691223,-6.12583114690814,
49.6629443835339));
#195938=CARTESIAN_POINT('Ctrl Pts',(-2.71648547473006,-6.19782184848682,
49.6713946522573));
#195939=CARTESIAN_POINT('Ctrl Pts',(-2.55237939965628,-6.26974901582896,
49.6798374633318));
#195940=CARTESIAN_POINT('Ctrl Pts',(-2.38529595045556,-6.33520652042679,
49.6882802744063));
#195941=CARTESIAN_POINT('Ctrl Pts',(-2.21577244452717,-6.39395350890778,
49.6967230854808));
#195942=CARTESIAN_POINT('Ctrl Pts',(-2.04637546778268,-6.45265664973195,
49.7051595949985));
#195943=CARTESIAN_POINT('Ctrl Pts',(-1.87454237707326,-6.50465915059237,
49.7135961045163));
#195944=CARTESIAN_POINT('Ctrl Pts',(-1.70083012673447,-6.54976838369056,
49.722032614034));
#195945=CARTESIAN_POINT('Ctrl Pts',(-1.52724217685827,-6.59484533870513,
49.7304630867752));
#195946=CARTESIAN_POINT('Ctrl Pts',(-1.35177806961323,-6.63303878149209,
49.7388935595164));
#195947=CARTESIAN_POINT('Ctrl Pts',(-1.17500976540876,-6.66420595804137,
49.7473240322576));
#195948=CARTESIAN_POINT('Ctrl Pts',(-0.998317453419157,-6.69535973590592,
49.7557508807615));
#195949=CARTESIAN_POINT('Ctrl Pts',(-0.820322388132919,-6.71949321167944,
49.7641777292653));
#195950=CARTESIAN_POINT('Ctrl Pts',(-0.641607212394431,-6.7365146169962,
49.7726045777691));
#195951=CARTESIAN_POINT('Ctrl Pts',(-0.462947199648441,-6.753530768413,
49.7810288252058));
#195952=CARTESIAN_POINT('Ctrl Pts',(-0.28356784941739,-6.76343919580401,
49.7894530726424));
#195953=CARTESIAN_POINT('Ctrl Pts',(-0.104057796442262,-6.76619989174127,
49.797877320079));
#195954=CARTESIAN_POINT('Ctrl Pts',(-0.0534787316738465,-6.76697775023055,
49.80025095069));
#195955=CARTESIAN_POINT('Ctrl Pts',(-0.00288931352831388,-6.76718846934994,
49.802624581301));
#195956=CARTESIAN_POINT('Ctrl Pts',(0.0476972528130159,-6.76683190068101,
49.804998211912));
#195957=CARTESIAN_POINT('Ctrl Pts',(0.231379807142229,-6.7655371805875,
49.8136169928492));
#195958=CARTESIAN_POINT('Ctrl Pts',(0.414942543859155,-6.756759631352,49.8222357737864));
#195959=CARTESIAN_POINT('Ctrl Pts',(0.597770730378398,-6.74054590919036,
49.8308545547236));
#195960=CARTESIAN_POINT('Ctrl Pts',(0.780708740677443,-6.72432244754442,
49.8394785129101));
#195961=CARTESIAN_POINT('Ctrl Pts',(0.962911017213911,-6.70065392533793,
49.8481024710966));
#195962=CARTESIAN_POINT('Ctrl Pts',(1.14376928233591,-6.66963873300382,
49.8567264292831));
#195963=CARTESIAN_POINT('Ctrl Pts',(1.3311613394948,-6.63750306759342,49.8656619416542));
#195964=CARTESIAN_POINT('Ctrl Pts',(1.51711011063208,-6.59748008208997,
49.8745974540253));
#195965=CARTESIAN_POINT('Ctrl Pts',(1.70095264677661,-6.54973656671959,
49.8835329663965));
#195966=CARTESIAN_POINT('Ctrl Pts',(1.87871688703933,-6.50357157185346,
49.8921730482912));
#195967=CARTESIAN_POINT('Ctrl Pts',(2.05451165998388,-6.45018852914267,
49.9008131301858));
#195968=CARTESIAN_POINT('Ctrl Pts',(2.22775448583029,-6.38978864680695,
49.9094532120805));
#195969=CARTESIAN_POINT('Ctrl Pts',(2.40988285429204,-6.32629088306787,
49.9185364396899));
#195970=CARTESIAN_POINT('Ctrl Pts',(2.58919025776469,-6.25503773795242,
49.9276196672992));
#195971=CARTESIAN_POINT('Ctrl Pts',(2.76502480367359,-6.17631984559332,
49.9367028949086));
#195972=CARTESIAN_POINT('Ctrl Pts',(2.94085934958255,-6.09760195323419,
49.945786122518));
#195973=CARTESIAN_POINT('Ctrl Pts',(3.11322070614304,-6.0114195171545,49.9548693501273));
#195974=CARTESIAN_POINT('Ctrl Pts',(3.28148753969462,-5.91811866447682,
49.9639525777367));
#195975=CARTESIAN_POINT('Ctrl Pts',(3.44903870138265,-5.82521463863482,
49.9729971725966));
#195976=CARTESIAN_POINT('Ctrl Pts',(3.61268524976751,-5.72516759141924,
49.9820417674564));
#195977=CARTESIAN_POINT('Ctrl Pts',(3.77184622959922,-5.6183151407035,49.9910863623163));
#195978=CARTESIAN_POINT('Ctrl Pts',(3.93086115417876,-5.51156074393069,
50.0001226573367));
#195979=CARTESIAN_POINT('Ctrl Pts',(4.08539853090776,-5.3980135443738,50.0091589523571));
#195980=CARTESIAN_POINT('Ctrl Pts',(4.23490548248072,-5.27805499729349,
50.0181952473775));
#195981=CARTESIAN_POINT('Ctrl Pts',(4.38414786977883,-5.15830872626915,
50.0272155519652));
#195982=CARTESIAN_POINT('Ctrl Pts',(4.52837742223618,-5.03217391168751,
50.036235856553));
#195983=CARTESIAN_POINT('Ctrl Pts',(4.66707361998934,-4.90007273676623,
50.0452561611407));
#195984=CARTESIAN_POINT('Ctrl Pts',(4.80559515682386,-4.76813791761344,
50.0542651064071));
#195985=CARTESIAN_POINT('Ctrl Pts',(4.93859707330936,-4.63025189600761,
50.0632740516734));
#195986=CARTESIAN_POINT('Ctrl Pts',(5.06559312154925,-4.48687589831867,
50.0722829969398));
#195987=CARTESIAN_POINT('Ctrl Pts',(5.19230078864845,-4.343825477168,50.0812714847986));
#195988=CARTESIAN_POINT('Ctrl Pts',(5.31302965279278,-4.19531014204271,
50.0902599726574));
#195989=CARTESIAN_POINT('Ctrl Pts',(5.42733173623316,-4.04182622398296,
50.0992484605163));
#195990=CARTESIAN_POINT('Ctrl Pts',(5.52761608311355,-3.90716520980037,
50.1071346215313));
#195991=CARTESIAN_POINT('Ctrl Pts',(5.62295375801983,-3.76868018637237,
50.1150207825464));
#195992=CARTESIAN_POINT('Ctrl Pts',(5.71306609539626,-3.62672921371775,
50.1229069435614));
#195993=CARTESIAN_POINT('Ctrl Pts',(5.80586716548787,-3.48054276970326,
50.1310284084176));
#195994=CARTESIAN_POINT('Ctrl Pts',(5.89308350086692,-3.33074502271687,
50.1391498732738));
#195995=CARTESIAN_POINT('Ctrl Pts',(5.97443016494423,-3.17780949778373,
50.1472713381299));
#195996=CARTESIAN_POINT('Ctrl Pts',(6.05577102780719,-3.02488487940432,
50.1553922238061));
#195997=CARTESIAN_POINT('Ctrl Pts',(6.13124288118561,-2.86882325209378,
50.1635131094824));
#195998=CARTESIAN_POINT('Ctrl Pts',(6.20060663605718,-2.7101229390719,50.1716339951586));
#195999=CARTESIAN_POINT('Ctrl Pts',(6.26997868188088,-2.55140365682464,
50.1797558515128));
#196000=CARTESIAN_POINT('Ctrl Pts',(6.33324102986522,-2.39004539684763,
50.1878777078671));
#196001=CARTESIAN_POINT('Ctrl Pts',(6.39020266694267,-2.22656661148926,
50.1959995642213));
#196002=CARTESIAN_POINT('Ctrl Pts',(6.44720586252584,-2.06296855403155,
50.2041273461815));
#196003=CARTESIAN_POINT('Ctrl Pts',(6.49789904528797,-1.89724722734643,
50.2122551281417));
#196004=CARTESIAN_POINT('Ctrl Pts',(6.54214085162684,-1.7299370154648,50.2203829101018));
#196005=CARTESIAN_POINT('Ctrl Pts',(6.58640068043322,-1.56255864762147,
50.2285140030183));
#196006=CARTESIAN_POINT('Ctrl Pts',(6.62420381447888,-1.39359046152614,
50.2366450959348));
#196007=CARTESIAN_POINT('Ctrl Pts',(6.65546004985548,-1.22357693864249,
50.2447761888512));
#196008=CARTESIAN_POINT('Ctrl Pts',(6.68675040010672,-1.05337785310386,
50.2529161565158));
#196009=CARTESIAN_POINT('Ctrl Pts',(6.71147952713835,-0.882131513925039,
50.2610561241803));
#196010=CARTESIAN_POINT('Ctrl Pts',(6.72960902520342,-0.710388181138124,
50.2691960918449));
#196011=CARTESIAN_POINT('Ctrl Pts',(6.73901176676927,-0.621314663048547,
50.2734178310254));
#196012=CARTESIAN_POINT('Ctrl Pts',(6.74664012502561,-0.532107489665762,
50.2776395702059));
#196013=CARTESIAN_POINT('Ctrl Pts',(6.75249426252371,-0.442843352196272,
50.2818613093864));
#196014=CARTESIAN_POINT('Ctrl Pts',(6.76419800464635,-0.264384194705872,
50.290301518844));
#196015=CARTESIAN_POINT('Ctrl Pts',(6.76883145057379,-0.0853285350571334,
50.2987417283017));
#196016=CARTESIAN_POINT('Ctrl Pts',(6.76635072172373,0.0937385226508884,
50.3071819377593));
#196017=CARTESIAN_POINT('Ctrl Pts',(6.7638718723933,0.272669910533722,50.3156157525078));
#196018=CARTESIAN_POINT('Ctrl Pts',(6.75428959757382,0.451612347007539,
50.3240495672564));
#196019=CARTESIAN_POINT('Ctrl Pts',(6.73761203233686,0.62997865178875,50.3324833820049));
#196020=CARTESIAN_POINT('Ctrl Pts',(6.72094453903604,0.808237237367194,
50.3409121033935));
#196021=CARTESIAN_POINT('Ctrl Pts',(6.69719032904113,0.985920053713816,
50.349340824782));
#196022=CARTESIAN_POINT('Ctrl Pts',(6.66640954848244,1.16244257144261,50.3577695461705));
#196023=CARTESIAN_POINT('Ctrl Pts',(6.63564263045777,1.33888558990717,50.3661944715723));
#196024=CARTESIAN_POINT('Ctrl Pts',(6.5978555087356,1.5141690236913,50.374619396974));
#196025=CARTESIAN_POINT('Ctrl Pts',(6.55315990282209,1.68771570119044,50.3830443223758));
#196026=CARTESIAN_POINT('Ctrl Pts',(6.50847756853883,1.86121084683793,50.3914667461335));
#196027=CARTESIAN_POINT('Ctrl Pts',(6.45689092401229,2.03296994202092,50.3998891698912));
#196028=CARTESIAN_POINT('Ctrl Pts',(6.3985623932095,2.20242781952215,50.4083115936489));
#196029=CARTESIAN_POINT('Ctrl Pts',(6.34023294506684,2.37188836210795,50.4167341498671));
#196030=CARTESIAN_POINT('Ctrl Pts',(6.27516150101785,2.53904729728787,50.4251567060854));
#196031=CARTESIAN_POINT('Ctrl Pts',(6.20356000199686,2.70335574825526,50.4335792623036));
#196032=CARTESIAN_POINT('Ctrl Pts',(6.13195608426367,2.86766974959325,50.4420021030373));
#196033=CARTESIAN_POINT('Ctrl Pts',(6.05382180483552,3.02913276885523,50.4504249437711));
#196034=CARTESIAN_POINT('Ctrl Pts',(5.96941686060406,3.18721686496792,50.4588477845048));
#196035=CARTESIAN_POINT('Ctrl Pts',(5.88499728129378,3.34532837147972,50.4672720856855));
#196036=CARTESIAN_POINT('Ctrl Pts',(5.79430502657094,3.50005949253455,50.4756963868661));
#196037=CARTESIAN_POINT('Ctrl Pts',(5.69764543893034,3.65090748338496,50.4841206880467));
#196038=CARTESIAN_POINT('Ctrl Pts',(5.60095559247987,3.80180269645911,50.4925476264135));
#196039=CARTESIAN_POINT('Ctrl Pts',(5.49829486863055,3.94881207502123,50.5009745647804));
#196040=CARTESIAN_POINT('Ctrl Pts',(5.39001175810941,4.09146211609522,50.5094015031472));
#196041=CARTESIAN_POINT('Ctrl Pts',(5.28163128746083,4.23424041748709,50.5178360183908));
#196042=CARTESIAN_POINT('Ctrl Pts',(5.16761853085843,4.3726512834815,50.5262705336345));
#196043=CARTESIAN_POINT('Ctrl Pts',(5.04836279385075,4.50625366592511,50.5347050488782));
#196044=CARTESIAN_POINT('Ctrl Pts',(4.92904945530045,4.63992057946399,50.5431436380649));
#196045=CARTESIAN_POINT('Ctrl Pts',(4.80448831376961,4.7687741341678,50.5515822272517));
#196046=CARTESIAN_POINT('Ctrl Pts',(4.67510568055939,4.8924100273384,50.5600208164385));
#196047=CARTESIAN_POINT('Ctrl Pts',(4.54557842683734,5.01618411746565,50.5684688380588));
#196048=CARTESIAN_POINT('Ctrl Pts',(4.41121915937598,5.13472866788723,50.5769168596791));
#196049=CARTESIAN_POINT('Ctrl Pts',(4.27248833791398,5.24767876326181,50.5853648812994));
#196050=CARTESIAN_POINT('Ctrl Pts',(4.19363596539665,5.31187778480934,50.5901666012115));
#196051=CARTESIAN_POINT('Ctrl Pts',(4.11337189238453,5.37427022041562,50.5949683211236));
#196052=CARTESIAN_POINT('Ctrl Pts',(4.03178486308043,5.4347952875739,50.5997700410358));
#196053=CARTESIAN_POINT('Ctrl Pts',(3.88493003633055,5.54373905384864,50.6084130294104));
#196054=CARTESIAN_POINT('Ctrl Pts',(3.73344294290708,5.64688470195427,50.617056017785));
#196055=CARTESIAN_POINT('Ctrl Pts',(3.57782307109196,5.74382025066611,50.6256990061597));
#196056=CARTESIAN_POINT('Ctrl Pts',(3.4222031992769,5.84075579937792,50.6343419945343));
#196057=CARTESIAN_POINT('Ctrl Pts',(3.26245088247718,5.93148094036033,50.6429849829089));
#196058=CARTESIAN_POINT('Ctrl Pts',(3.0991061983213,6.01563211736942,50.6516279712835));
#196059=CARTESIAN_POINT('Origin',(0.,0.,4.30282021618968));
#196060=CARTESIAN_POINT('',(3.09910619832131,6.01563211736941,53.0454129677962));
#196061=CARTESIAN_POINT('',(3.09910619832128,6.01563211736943,52.6513490741792));
#196062=CARTESIAN_POINT('',(3.09910619832133,6.0156321173694,4.30282021618968));
#196063=CARTESIAN_POINT('',(-6.76699999999835,4.72499786567897E-6,51.6972805685448));
#196064=CARTESIAN_POINT('Ctrl Pts',(-6.76699999999835,4.72499786567896E-6,
51.6972805685448));
#196065=CARTESIAN_POINT('Ctrl Pts',(-6.7670001215516,-0.17408018574719,
51.705442029816));
#196066=CARTESIAN_POINT('Ctrl Pts',(-6.76027824898233,-0.348190866565372,
51.7136034910872));
#196067=CARTESIAN_POINT('Ctrl Pts',(-6.74685446399381,-0.521769912592487,
51.7217649523584));
#196068=CARTESIAN_POINT('Ctrl Pts',(-6.733429900442,-0.695359025994333,
51.7299268869845));
#196069=CARTESIAN_POINT('Ctrl Pts',(-6.71330267886051,-0.868416082426914,
51.7380888216106));
#196070=CARTESIAN_POINT('Ctrl Pts',(-6.68654482128806,-1.04038807802948,
51.7462507562368));
#196071=CARTESIAN_POINT('Ctrl Pts',(-6.65909310961529,-1.21681945435655,
51.7546243367987));
#196072=CARTESIAN_POINT('Ctrl Pts',(-6.62466227160216,-1.39210833402499,
51.7629979173606));
#196073=CARTESIAN_POINT('Ctrl Pts',(-6.58338601740211,-1.56566840227246,
51.7713714979226));
#196074=CARTESIAN_POINT('Ctrl Pts',(-6.54310963007841,-1.73502418971343,
51.7795422387162));
#196075=CARTESIAN_POINT('Ctrl Pts',(-6.49631578017444,-1.90273361408968,
51.7877129795098));
#196076=CARTESIAN_POINT('Ctrl Pts',(-6.44317926085405,-2.068267393859,51.7958837203034));
#196077=CARTESIAN_POINT('Ctrl Pts',(-6.38806405939049,-2.23996527203577,
51.8043587207495));
#196078=CARTESIAN_POINT('Ctrl Pts',(-6.32612486716165,-2.40932194435085,
51.8128337211956));
#196079=CARTESIAN_POINT('Ctrl Pts',(-6.25761121042792,-2.57576997015005,
51.8213087216417));
#196080=CARTESIAN_POINT('Ctrl Pts',(-6.1890975536942,-2.74221799594926,
51.8297837220878));
#196081=CARTESIAN_POINT('Ctrl Pts',(-6.11400965808697,-2.90575700593975,
51.8382587225339));
#196082=CARTESIAN_POINT('Ctrl Pts',(-6.03264948575606,-3.06584885178758,
51.84673372298));
#196083=CARTESIAN_POINT('Ctrl Pts',(-5.95162330760453,-3.22528349960904,
51.8551739324376));
#196084=CARTESIAN_POINT('Ctrl Pts',(-5.86421276379904,-3.38162221811784,
51.8636141418953));
#196085=CARTESIAN_POINT('Ctrl Pts',(-5.77067877548236,-3.53433946731173,
51.8720543513529));
#196086=CARTESIAN_POINT('Ctrl Pts',(-5.67721565301913,-3.68694101056392,
51.8804881661014));
#196087=CARTESIAN_POINT('Ctrl Pts',(-5.57763850795933,-3.83592627071905,
51.8889219808499));
#196088=CARTESIAN_POINT('Ctrl Pts',(-5.47225404880864,-3.98079447162215,
51.8973557955985));
#196089=CARTESIAN_POINT('Ctrl Pts',(-5.36693323357255,-4.12557518353985,
51.905784516987));
#196090=CARTESIAN_POINT('Ctrl Pts',(-5.25581229195834,-4.26624352415761,
51.9142132383756));
#196091=CARTESIAN_POINT('Ctrl Pts',(-5.13924130477004,-4.4023275447592,
51.9226419597641));
#196092=CARTESIAN_POINT('Ctrl Pts',(-5.02272281687667,-4.53835027811165,
51.9310668851659));
#196093=CARTESIAN_POINT('Ctrl Pts',(-4.90075939399643,-4.66979255520143,
51.9394918105676));
#196094=CARTESIAN_POINT('Ctrl Pts',(-4.77374171033594,-4.79621507889282,
51.9479167359693));
#196095=CARTESIAN_POINT('Ctrl Pts',(-4.64676174250258,-4.92260006348012,
51.956339159727));
#196096=CARTESIAN_POINT('Ctrl Pts',(-4.51473074288339,-5.0439680321168,
51.9647615834848));
#196097=CARTESIAN_POINT('Ctrl Pts',(-4.37807686013395,-5.15991589144238,
51.9731840072425));
#196098=CARTESIAN_POINT('Ctrl Pts',(-4.24142082821196,-5.27586557429432,
51.9816065634607));
#196099=CARTESIAN_POINT('Ctrl Pts',(-4.10014201781241,-5.38639475674505,
51.9900291196789));
#196100=CARTESIAN_POINT('Ctrl Pts',(-3.95470284318514,-5.49113962872038,
51.9984516758971));
#196101=CARTESIAN_POINT('Ctrl Pts',(-3.80925875559516,-5.59588803899721,
52.0068745166308));
#196102=CARTESIAN_POINT('Ctrl Pts',(-3.65965429414324,-5.69485155411564,
52.0152973573646));
#196103=CARTESIAN_POINT('Ctrl Pts',(-3.50638225324372,-5.78770874302928,
52.0237201980983));
#196104=CARTESIAN_POINT('Ctrl Pts',(-3.35308363631337,-5.880582032567,52.032144499279));
#196105=CARTESIAN_POINT('Ctrl Pts',(-3.19611645737286,-5.96734671216084,
52.0405688004596));
#196106=CARTESIAN_POINT('Ctrl Pts',(-3.03599990153993,-6.04772631638118,
52.0489931016403));
#196107=CARTESIAN_POINT('Ctrl Pts',(-2.8758332220041,-6.1281310830426,52.0574200400071));
#196108=CARTESIAN_POINT('Ctrl Pts',(-2.71251549795603,-6.20214663963946,
52.0658469783739));
#196109=CARTESIAN_POINT('Ctrl Pts',(-2.54658809276887,-6.26954369039469,
52.0742739167407));
#196110=CARTESIAN_POINT('Ctrl Pts',(-2.38051149798803,-6.33700133957009,
52.0827084319844));
#196111=CARTESIAN_POINT('Ctrl Pts',(-2.21182084286592,-6.39782846647733,
52.091142947228));
#196112=CARTESIAN_POINT('Ctrl Pts',(-2.04107602245292,-6.45184451692443,
52.0995774624717));
#196113=CARTESIAN_POINT('Ctrl Pts',(-1.87024873082868,-6.50588665758671,
52.1080160516584));
#196114=CARTESIAN_POINT('Ctrl Pts',(-1.6973656153603,-6.55311106785541,
52.1164546408452));
#196115=CARTESIAN_POINT('Ctrl Pts',(-1.52299963722095,-6.59338768047389,
52.124893230032));
#196116=CARTESIAN_POINT('Ctrl Pts',(-1.34843875736749,-6.63370931323289,
52.1333412516523));
#196117=CARTESIAN_POINT('Ctrl Pts',(-1.1723920296516,-6.66706756330533,
52.1417892732726));
#196118=CARTESIAN_POINT('Ctrl Pts',(-0.995441675805299,-6.69338366374362,
52.1502372948929));
#196119=CARTESIAN_POINT('Ctrl Pts',(-0.894865934439944,-6.7083413129028,
52.1550390148051));
#196120=CARTESIAN_POINT('Ctrl Pts',(-0.793998373723847,-6.72102487048139,
52.1598407347173));
#196121=CARTESIAN_POINT('Ctrl Pts',(-0.692946331705399,-6.73142736582488,
52.1646424546295));
#196122=CARTESIAN_POINT('Ctrl Pts',(-0.519545647361508,-6.74927757226717,
52.1728819864803));
#196123=CARTESIAN_POINT('Ctrl Pts',(-0.345214546491155,-6.76044806221027,
52.1811215183311));
#196124=CARTESIAN_POINT('Ctrl Pts',(-0.17050709286497,-6.76485153800752,
52.1893610501819));
#196125=CARTESIAN_POINT('Ctrl Pts',(0.00400644769779515,-6.7692501262544,
52.1975914367282));
#196126=CARTESIAN_POINT('Ctrl Pts',(0.178895156596411,-6.76689664695487,
52.2058218232745));
#196127=CARTESIAN_POINT('Ctrl Pts',(0.353598173914164,-6.7577553471108,
52.2140522098208));
#196128=CARTESIAN_POINT('Ctrl Pts',(0.528138448504477,-6.74862256274683,
52.2222749294386));
#196129=CARTESIAN_POINT('Ctrl Pts',(0.702493022673535,-6.73271456893072,
52.2304976490563));
#196130=CARTESIAN_POINT('Ctrl Pts',(0.876099252822407,-6.71004762272251,
52.2387203686741));
#196131=CARTESIAN_POINT('Ctrl Pts',(1.04955165534421,-6.68740076106165,
52.2469358023699));
#196132=CARTESIAN_POINT('Ctrl Pts',(1.22225668387424,-6.65800692939003,
52.2551512360656));
#196133=CARTESIAN_POINT('Ctrl Pts',(1.39365516884833,-6.62193432996299,
52.2633666697614));
#196134=CARTESIAN_POINT('Ctrl Pts',(1.56496556831073,-6.58588026905091,
52.2715778813622));
#196135=CARTESIAN_POINT('Ctrl Pts',(1.73497041406748,-6.54315434936632,
52.279789092963));
#196136=CARTESIAN_POINT('Ctrl Pts',(1.90311868934679,-6.49387621180593,
52.2880003045638));
#196137=CARTESIAN_POINT('Ctrl Pts',(2.07121057697315,-6.44461459941367,
52.2962087625773));
#196138=CARTESIAN_POINT('Ctrl Pts',(2.23744679320222,-6.38880524624889,
52.3044172205909));
#196139=CARTESIAN_POINT('Ctrl Pts',(2.40128940536313,-6.32661822711714,
52.3126256786044));
#196140=CARTESIAN_POINT('Ctrl Pts',(2.47428486671498,-6.29891255219076,
52.3162827258877));
#196141=CARTESIAN_POINT('Ctrl Pts',(2.54680541987644,-6.26994163894168,
52.3199397731709));
#196142=CARTESIAN_POINT('Ctrl Pts',(2.61880456934592,-6.23972368198888,
52.3235968204542));
#196143=CARTESIAN_POINT('Ctrl Pts',(2.79322008994097,-6.16652169651994,
52.3324558946301));
#196144=CARTESIAN_POINT('Ctrl Pts',(2.96439325302043,-6.0860746986052,52.341314968806));
#196145=CARTESIAN_POINT('Ctrl Pts',(3.13175329346485,-5.99870071839495,
52.3501740429818));
#196146=CARTESIAN_POINT('Ctrl Pts',(3.29942776975585,-5.91116258005375,
52.3590497615758));
#196147=CARTESIAN_POINT('Ctrl Pts',(3.46327457659115,-5.81667157085099,
52.3679254801698));
#196148=CARTESIAN_POINT('Ctrl Pts',(3.62275023178512,-5.7155900621109,52.3768011987638));
#196149=CARTESIAN_POINT('Ctrl Pts',(3.78268098543869,-5.61422009530575,
52.3857022461508));
#196150=CARTESIAN_POINT('Ctrl Pts',(3.9382154048476,-5.50622213235346,52.3946032935378));
#196151=CARTESIAN_POINT('Ctrl Pts',(4.0888390419843,-5.39200188137439,52.4035043409248));
#196152=CARTESIAN_POINT('Ctrl Pts',(4.23966745402118,-5.27762634639781,
52.4124174894078));
#196153=CARTESIAN_POINT('Ctrl Pts',(4.385571544924,-5.15701178724975,52.4213306378908));
#196154=CARTESIAN_POINT('Ctrl Pts',(4.52607132563768,-5.0306030806694,52.4302437863738));
#196155=CARTESIAN_POINT('Ctrl Pts',(4.66688305428365,-4.90391371219448,
52.4391767244837));
#196156=CARTESIAN_POINT('Ctrl Pts',(4.80226627894018,-4.77140463884942,
52.4481096625936));
#196157=CARTESIAN_POINT('Ctrl Pts',(4.93177711590503,-4.63355840354208,
52.4570426007034));
#196158=CARTESIAN_POINT('Ctrl Pts',(5.05505265440609,-4.50234877440141,
52.4655454625619));
#196159=CARTESIAN_POINT('Ctrl Pts',(5.17300782307301,-4.36630393741194,
52.4740483244205));
#196160=CARTESIAN_POINT('Ctrl Pts',(5.28529476372081,-4.22586656918855,
52.482551186279));
#196161=CARTESIAN_POINT('Ctrl Pts',(5.39388226308922,-4.0900560951897,52.4907739101448));
#196162=CARTESIAN_POINT('Ctrl Pts',(5.49737622324671,-3.94987683983684,
52.4989966340107));
#196163=CARTESIAN_POINT('Ctrl Pts',(5.59540686847251,-3.80574709830418,
52.5072193578766));
#196164=CARTESIAN_POINT('Ctrl Pts',(5.69333375158116,-3.66176991322049,
52.5154333782678));
#196165=CARTESIAN_POINT('Ctrl Pts',(5.78580863496937,-3.51385086272946,
52.523647398659));
#196166=CARTESIAN_POINT('Ctrl Pts',(5.87250164412075,-3.36244158905386,
52.5318614190502));
#196167=CARTESIAN_POINT('Ctrl Pts',(5.95912029716409,-3.21116217826367,
52.5400683943222));
#196168=CARTESIAN_POINT('Ctrl Pts',(6.03996677517237,-3.05639881573309,
52.5482753695941));
#196169=CARTESIAN_POINT('Ctrl Pts',(6.11475417616781,-2.89863249913444,
52.5564823448661));
#196170=CARTESIAN_POINT('Ctrl Pts',(6.18949244333358,-2.74096983185672,
52.5646839283191));
#196171=CARTESIAN_POINT('Ctrl Pts',(6.25817940944029,-2.58030846323823,
52.5728855117721));
#196172=CARTESIAN_POINT('Ctrl Pts',(6.32057380811288,-2.41715447090115,
52.5810870952251));
#196173=CARTESIAN_POINT('Ctrl Pts',(6.38293973579966,-2.25407492683349,
52.5892849362402));
#196174=CARTESIAN_POINT('Ctrl Pts',(6.4390186885944,-2.08850535939524,52.5974827772553));
#196175=CARTESIAN_POINT('Ctrl Pts',(6.48861726448096,-1.92097240872421,
52.6056806182703));
#196176=CARTESIAN_POINT('Ctrl Pts',(6.53821146344788,-1.75345424231358,
52.6138777358515));
#196177=CARTESIAN_POINT('Ctrl Pts',(6.58132631461898,-1.58397337905668,
52.6220748534326));
#196178=CARTESIAN_POINT('Ctrl Pts',(6.61781798503562,-1.41307258020921,
52.6302719710138));
#196179=CARTESIAN_POINT('Ctrl Pts',(6.65430924944177,-1.2421736828235,52.6384689973929));
#196180=CARTESIAN_POINT('Ctrl Pts',(6.68417740388642,-1.06985523201138,
52.646666023772));
#196181=CARTESIAN_POINT('Ctrl Pts',(6.70732957509223,-0.896671049545541,
52.6548630501511));
#196182=CARTESIAN_POINT('Ctrl Pts',(6.73048569847149,-0.723457303807981,
52.6630614757972));
#196183=CARTESIAN_POINT('Ctrl Pts',(6.74692350700062,-0.549377887665944,
52.6712599014433));
#196184=CARTESIAN_POINT('Ctrl Pts',(6.75660191893404,-0.374992678670986,
52.6794583270895));
#196185=CARTESIAN_POINT('Ctrl Pts',(6.7662837428612,-0.200545992520039,
52.6876596429801));
#196186=CARTESIAN_POINT('Ctrl Pts',(6.76920140349111,-0.0257936568339158,
52.6958609588707));
#196187=CARTESIAN_POINT('Ctrl Pts',(6.76536593848992,0.148703457661181,
52.7040622747613));
#196188=CARTESIAN_POINT('Ctrl Pts',(6.76152610553612,0.32339929516018,52.7122729305779));
#196189=CARTESIAN_POINT('Ctrl Pts',(6.75091779023594,0.497838971674598,
52.7204835863945));
#196190=CARTESIAN_POINT('Ctrl Pts',(6.73360410007997,0.671464685137079,
52.7286942422111));
#196191=CARTESIAN_POINT('Ctrl Pts',(6.71628020738587,0.845192712025799,
52.7369097363683));
#196192=CARTESIAN_POINT('Ctrl Pts',(6.69224311282282,1.01810546492956,52.7451252305254));
#196193=CARTESIAN_POINT('Ctrl Pts',(6.66160725564259,1.18965447570712,52.7533407246825));
#196194=CARTESIAN_POINT('Ctrl Pts',(6.63092386636619,1.36146964793175,52.76156896533));
#196195=CARTESIAN_POINT('Ctrl Pts',(6.59362133137818,1.53191649938276,52.7697972059776));
#196196=CARTESIAN_POINT('Ctrl Pts',(6.54986459478902,1.7004595819746,52.7780254466251));
#196197=CARTESIAN_POINT('Ctrl Pts',(6.51009670703936,1.85363833596687,52.7855036037262));
#196198=CARTESIAN_POINT('Ctrl Pts',(6.46499839601889,2.00524460684536,52.7929817608273));
#196199=CARTESIAN_POINT('Ctrl Pts',(6.414727853989,2.15489107828162,52.8004599179285));
#196200=CARTESIAN_POINT('Ctrl Pts',(6.36047336360953,2.31639705607734,52.8085307201541));
#196201=CARTESIAN_POINT('Ctrl Pts',(6.30001590092302,2.47614879841058,52.8166015223798));
#196202=CARTESIAN_POINT('Ctrl Pts',(6.23348418439502,2.6336218260975,52.8246723246055));
#196203=CARTESIAN_POINT('Ctrl Pts',(6.16703787316329,2.79089270913393,52.8327327665204));
#196204=CARTESIAN_POINT('Ctrl Pts',(6.09453296829489,2.94589035882531,52.8407932084354));
#196205=CARTESIAN_POINT('Ctrl Pts',(6.01614837033181,3.09810390176861,52.8488536503503));
#196206=CARTESIAN_POINT('Ctrl Pts',(5.93650414798612,3.25276348506982,52.8570436219106));
#196207=CARTESIAN_POINT('Ctrl Pts',(5.85078971948395,3.40454833549116,52.8652335934708));
#196208=CARTESIAN_POINT('Ctrl Pts',(5.75924492905679,3.55294059155704,52.8734235650311));
#196209=CARTESIAN_POINT('Ctrl Pts',(5.66933258222671,3.69868668952763,52.881467491507));
#196210=CARTESIAN_POINT('Ctrl Pts',(5.57379625129872,3.84115982554122,52.889511417983));
#196211=CARTESIAN_POINT('Ctrl Pts',(5.47291062215085,3.97989174751631,52.897555344459));
#196212=CARTESIAN_POINT('Ctrl Pts',(5.372079588008,4.11854859368486,52.9055949179046));
#196213=CARTESIAN_POINT('Ctrl Pts',(5.26590523497039,4.25346795360913,52.9136344913502));
#196214=CARTESIAN_POINT('Ctrl Pts',(5.15470620529812,4.38420949967735,52.9216740647958));
#196215=CARTESIAN_POINT('Ctrl Pts',(5.04354531918934,4.51490619869539,52.9297108805017));
#196216=CARTESIAN_POINT('Ctrl Pts',(4.92736342893566,4.64142765250874,52.9377476962076));
#196217=CARTESIAN_POINT('Ctrl Pts',(4.8065201043854,4.7633657728689,52.9457845119135));
#196218=CARTESIAN_POINT('Ctrl Pts',(4.68168382729436,4.88933302044253,52.954086883237));
#196219=CARTESIAN_POINT('Ctrl Pts',(4.55187304049737,5.01040852287378,52.9623892545606));
#196220=CARTESIAN_POINT('Ctrl Pts',(4.41752628628522,5.12618284008473,52.9706916258842));
#196221=CARTESIAN_POINT('Ctrl Pts',(4.28745632268326,5.23827160109707,52.9787296997639));
#196222=CARTESIAN_POINT('Ctrl Pts',(4.15313507913528,5.34539129234802,52.9867677736437));
#196223=CARTESIAN_POINT('Ctrl Pts',(4.01499456498667,5.44721099675123,52.9948058475235));
#196224=CARTESIAN_POINT('Ctrl Pts',(3.87004081697411,5.55405255489759,53.003240367569));
#196225=CARTESIAN_POINT('Ctrl Pts',(3.72088187097125,5.65505778981958,53.0116748876144));
#196226=CARTESIAN_POINT('Ctrl Pts',(3.56805102046256,5.74989573082644,53.0201094076599));
#196227=CARTESIAN_POINT('Ctrl Pts',(3.41522016995381,5.84473367183333,53.0285439277053));
#196228=CARTESIAN_POINT('Ctrl Pts',(3.25871784107602,5.9334041117776,53.0369784477508));
#196229=CARTESIAN_POINT('Ctrl Pts',(3.09910619832131,6.01563211736941,53.0454129677962));
#196230=CARTESIAN_POINT('Ctrl Pts',(3.0991061983214,6.01563211736937,51.0457552630242));
#196231=CARTESIAN_POINT('Ctrl Pts',(2.93375330764836,6.10081787314649,51.0545047109265));
#196232=CARTESIAN_POINT('Ctrl Pts',(2.76488627843083,6.17918207037033,51.0632541588288));
#196233=CARTESIAN_POINT('Ctrl Pts',(2.59307866646718,6.2504585455399,51.0720036067311));
#196234=CARTESIAN_POINT('Ctrl Pts',(2.4212724418539,6.32173444515032,51.0807529839814));
#196235=CARTESIAN_POINT('Ctrl Pts',(2.24652594672477,6.38592262741834,51.0895023612317));
#196236=CARTESIAN_POINT('Ctrl Pts',(2.06943269687131,6.44280508110559,51.098251738482));
#196237=CARTESIAN_POINT('Ctrl Pts',(1.89234081822085,6.49968709436164,51.1070010479874));
#196238=CARTESIAN_POINT('Ctrl Pts',(1.71290249405594,6.54926340459543,51.1157503574927));
#196239=CARTESIAN_POINT('Ctrl Pts',(1.53172716625062,6.59136563150383,51.1244996669981));
#196240=CARTESIAN_POINT('Ctrl Pts',(1.35055318107333,6.6334675464071,51.1332489116653));
#196241=CARTESIAN_POINT('Ctrl Pts',(1.16764249714414,6.66809542395777,51.1419981563326));
#196242=CARTESIAN_POINT('Ctrl Pts',(0.983616340614252,6.6951316562467,51.1507474009998));
#196243=CARTESIAN_POINT('Ctrl Pts',(0.799591486713773,6.72216769715962,
51.1594965837355));
#196244=CARTESIAN_POINT('Ctrl Pts',(0.614451459526678,6.74161215869371,
51.1682457664712));
#196245=CARTESIAN_POINT('Ctrl Pts',(0.428825047910284,6.75339900185712,
51.1769949492069));
#196246=CARTESIAN_POINT('Ctrl Pts',(0.243199888596927,6.76518576550222,
51.1857440729174));
#196247=CARTESIAN_POINT('Ctrl Pts',(0.0570886373916771,6.76931499599835,
51.194493196628));
#196248=CARTESIAN_POINT('Ctrl Pts',(-0.12887662681151,6.76577266947846,
51.2032423203385));
#196249=CARTESIAN_POINT('Ctrl Pts',(-0.314840698188554,6.76223036567991,
51.21199138793));
#196250=CARTESIAN_POINT('Ctrl Pts',(-0.500658497951682,6.7510166087922,
51.2207404555216));
#196251=CARTESIAN_POINT('Ctrl Pts',(-0.68569895192668,6.73216948296214,
51.2294895231131));
#196252=CARTESIAN_POINT('Ctrl Pts',(-0.870738280460442,6.71332247176286,
51.2382385374917));
#196253=CARTESIAN_POINT('Ctrl Pts',(-1.05499998761322,6.68684221356176,
51.2469875518702));
#196254=CARTESIAN_POINT('Ctrl Pts',(-1.23785829161503,6.65281863948507,
51.2557365662487));
#196255=CARTESIAN_POINT('Ctrl Pts',(-1.43007412917486,6.61705395368843,
51.2649332999479));
#196256=CARTESIAN_POINT('Ctrl Pts',(-1.62073882535873,6.5729537272777,51.2741300336471));
#196257=CARTESIAN_POINT('Ctrl Pts',(-1.80913696091594,6.52068343478257,
51.2833267673463));
#196258=CARTESIAN_POINT('Ctrl Pts',(-1.98838356186194,6.47095219815174,
51.29207676506));
#196259=CARTESIAN_POINT('Ctrl Pts',(-2.16557827572617,6.41382586850863,
51.3008267627737));
#196260=CARTESIAN_POINT('Ctrl Pts',(-2.34011918621786,6.34949849943246,
51.3095767604873));
#196261=CARTESIAN_POINT('Ctrl Pts',(-2.51465655691185,6.28517243495516,
51.3183265807457));
#196262=CARTESIAN_POINT('Ctrl Pts',(-2.68653996295416,6.21364572242336,
51.3270764010039));
#196263=CARTESIAN_POINT('Ctrl Pts',(-2.85518555380077,6.1351613225218,51.3358262212623));
#196264=CARTESIAN_POINT('Ctrl Pts',(-3.02382794858787,6.05667841000458,
51.3445758756998));
#196265=CARTESIAN_POINT('Ctrl Pts',(-3.18923239109387,5.97123819492025,
51.3533255301373));
#196266=CARTESIAN_POINT('Ctrl Pts',(-3.35083705967812,5.87913088810648,
51.3620751845748));
#196267=CARTESIAN_POINT('Ctrl Pts',(-3.51243888042504,5.7870252044304,51.3708246848237));
#196268=CARTESIAN_POINT('Ctrl Pts',(-3.67024081223785,5.68825280605722,
51.3795741850727));
#196269=CARTESIAN_POINT('Ctrl Pts',(-3.82370687544488,5.58314917682446,
51.3883236853216));
#196270=CARTESIAN_POINT('Ctrl Pts',(-3.97717043817909,5.47804726007953,
51.3970730430121));
#196271=CARTESIAN_POINT('Ctrl Pts',(-4.12629803722562,5.36661448084158,
51.4058224007025));
#196272=CARTESIAN_POINT('Ctrl Pts',(-4.27058317207016,5.24922931204488,
51.414571758393));
#196273=CARTESIAN_POINT('Ctrl Pts',(-4.41486614774942,5.13184589986699,
51.4233209851531));
#196274=CARTESIAN_POINT('Ctrl Pts',(-4.55430658194519,5.00851045722939,
51.4320702119132));
#196275=CARTESIAN_POINT('Ctrl Pts',(-4.68843089001949,4.8796418710302,51.4408194386733));
#196276=CARTESIAN_POINT('Ctrl Pts',(-4.82255336917937,4.75077504207858,
51.4495685461292));
#196277=CARTESIAN_POINT('Ctrl Pts',(-4.95135966065233,4.61637541907988,
51.4583176535851));
#196278=CARTESIAN_POINT('Ctrl Pts',(-5.0744123086934,4.47689945401736,51.467066761041));
#196279=CARTESIAN_POINT('Ctrl Pts',(-5.19746344226513,4.33742520555401,
51.4758157608174));
#196280=CARTESIAN_POINT('Ctrl Pts',(-5.31476088454863,4.19287495491215,
51.4845647605937));
#196281=CARTESIAN_POINT('Ctrl Pts',(-5.4259062762895,4.04373961586577,51.4933137603701));
#196282=CARTESIAN_POINT('Ctrl Pts',(-5.5370638067276,3.89458798906604,51.5020637156648));
#196283=CARTESIAN_POINT('Ctrl Pts',(-5.64206777071952,3.74085050155152,
51.5108136709595));
#196284=CARTESIAN_POINT('Ctrl Pts',(-5.74056148164091,3.58304938223027,
51.5195636262542));
#196285=CARTESIAN_POINT('Ctrl Pts',(-5.83905138951962,3.42525435593149,
51.5283132436953));
#196286=CARTESIAN_POINT('Ctrl Pts',(-5.93103139557725,3.26339625497051,
51.5370628611364));
#196287=CARTESIAN_POINT('Ctrl Pts',(-6.01618907820914,3.09802485064874,
51.5458124785775));
#196288=CARTESIAN_POINT('Ctrl Pts',(-6.1013439254504,2.93265895249521,51.5545618046934));
#196289=CARTESIAN_POINT('Ctrl Pts',(-6.17967677261879,2.76378023985929,
51.5633111308093));
#196290=CARTESIAN_POINT('Ctrl Pts',(-6.25092157009263,2.59196229227023,
51.5720604569251));
#196291=CARTESIAN_POINT('Ctrl Pts',(-6.32216437407792,2.4201491522899,51.5808095382276));
#196292=CARTESIAN_POINT('Ctrl Pts',(-6.3863194154896,2.24539720662741,51.58955861953));
#196293=CARTESIAN_POINT('Ctrl Pts',(-6.44316881037575,2.06829994947569,
51.5983077008325));
#196294=CARTESIAN_POINT('Ctrl Pts',(-6.50002334524603,1.8911866802434,51.6070575731748));
#196295=CARTESIAN_POINT('Ctrl Pts',(-6.54957082411122,1.71172794807601,
51.6158074455172));
#196296=CARTESIAN_POINT('Ctrl Pts',(-6.59164294296105,1.53053334250247,
51.6245573178595));
#196297=CARTESIAN_POINT('Ctrl Pts',(-6.63371214082145,1.34935131693539,
51.6333065827144));
#196298=CARTESIAN_POINT('Ctrl Pts',(-6.66830695239694,1.16643393829737,
51.6420558475693));
#196299=CARTESIAN_POINT('Ctrl Pts',(-6.69530988153987,0.982402458341065,
51.6508051124242));
#196300=CARTESIAN_POINT('Ctrl Pts',(-6.72231419690482,0.798361530947119,
51.6595548264312));
#196301=CARTESIAN_POINT('Ctrl Pts',(-6.74172580829277,0.613206671362522,
51.6683045404383));
#196302=CARTESIAN_POINT('Ctrl Pts',(-6.75347878028179,0.427566795113429,
51.6770542544453));
#196303=CARTESIAN_POINT('Ctrl Pts',(-6.76248992368217,0.285234494205065,
51.6837627642336));
#196304=CARTESIAN_POINT('Ctrl Pts',(-6.76699999999999,0.142617266091684,
51.6904712740218));
#196305=CARTESIAN_POINT('Ctrl Pts',(-6.767,7.53346691421078E-13,51.6971797838101));
#196306=CARTESIAN_POINT('',(-6.76699439492168,0.00870971288474031,51.3028202162293));
#196307=CARTESIAN_POINT('Ctrl Pts',(3.0991061983213,6.01563211736942,50.6516279712835));
#196308=CARTESIAN_POINT('Ctrl Pts',(2.94371706945757,6.09568478731625,50.6598500107166));
#196309=CARTESIAN_POINT('Ctrl Pts',(2.78507754112672,6.16978840847455,50.6680720501497));
#196310=CARTESIAN_POINT('Ctrl Pts',(2.62368229321237,6.23767426404136,50.6762940895828));
#196311=CARTESIAN_POINT('Ctrl Pts',(2.46242609187697,6.30550163402016,50.6845090454959));
#196312=CARTESIAN_POINT('Ctrl Pts',(2.29841922974917,6.36712177758301,50.692724001409));
#196313=CARTESIAN_POINT('Ctrl Pts',(2.13217947892454,6.42231264184897,50.7009389573222));
#196314=CARTESIAN_POINT('Ctrl Pts',(1.96602252369755,6.47747601834158,50.709149821782));
#196315=CARTESIAN_POINT('Ctrl Pts',(1.79763523168352,6.52621638114251,50.7173606862418));
#196316=CARTESIAN_POINT('Ctrl Pts',(1.62755415300313,6.56836025801282,50.7255715507016));
#196317=CARTESIAN_POINT('Ctrl Pts',(1.45752805383191,6.61049051167658,50.7337797609608));
#196318=CARTESIAN_POINT('Ctrl Pts',(1.28580960394632,6.64602844217198,50.74198797122));
#196319=CARTESIAN_POINT('Ctrl Pts',(1.11294935553933,6.67485076477404,50.7501961814792));
#196320=CARTESIAN_POINT('Ctrl Pts',(1.05308282713589,6.68483277284479,50.753038923273));
#196321=CARTESIAN_POINT('Ctrl Pts',(0.993079451021887,6.69400973202146,
50.7558816650668));
#196322=CARTESIAN_POINT('Ctrl Pts',(0.932962387151618,6.70237794996376,
50.7587244068605));
#196323=CARTESIAN_POINT('Ctrl Pts',(0.745614549499311,6.72845652791753,
50.7675834810364));
#196324=CARTESIAN_POINT('Ctrl Pts',(0.557356828514955,6.74664998063951,
50.7764425552123));
#196325=CARTESIAN_POINT('Ctrl Pts',(0.368842368325365,6.75694045462354,
50.7853016293882));
#196326=CARTESIAN_POINT('Ctrl Pts',(0.17997372739156,6.76725026233788,50.7941773479821));
#196327=CARTESIAN_POINT('Ctrl Pts',(-0.00915235787142143,6.76962740410089,
50.8030530665761));
#196328=CARTESIAN_POINT('Ctrl Pts',(-0.197883571541753,6.76410608226349,
50.81192878517));
#196329=CARTESIAN_POINT('Ctrl Pts',(-0.38715337077011,6.75856900413361,
50.820829832557));
#196330=CARTESIAN_POINT('Ctrl Pts',(-0.5760257826646,6.7450883643955,50.829730879944));
#196331=CARTESIAN_POINT('Ctrl Pts',(-0.763851338084534,6.72375045144497,
50.838631927331));
#196332=CARTESIAN_POINT('Ctrl Pts',(-0.951932244923655,6.70238352930908,
50.847545075814));
#196333=CARTESIAN_POINT('Ctrl Pts',(-1.13896319552895,6.67313803159433,
50.856458224297));
#196334=CARTESIAN_POINT('Ctrl Pts',(-1.3243043600039,6.63615151741389,50.86537137278));
#196335=CARTESIAN_POINT('Ctrl Pts',(-1.51005703254404,6.5990828830583,50.8743043108899));
#196336=CARTESIAN_POINT('Ctrl Pts',(-1.69411215942273,6.55423890568354,
50.8832372489998));
#196337=CARTESIAN_POINT('Ctrl Pts',(-1.87584173263627,6.50180796348986,
50.8921701871096));
#196338=CARTESIAN_POINT('Ctrl Pts',(-2.04882193664544,6.45190130869131,
50.9006730489682));
#196339=CARTESIAN_POINT('Ctrl Pts',(-2.21969506740445,6.3951210949578,50.9091759108267));
#196340=CARTESIAN_POINT('Ctrl Pts',(-2.38793604009994,6.33167043270509,
50.9176787726853));
#196341=CARTESIAN_POINT('Ctrl Pts',(-2.55063409216944,6.27031023616295,
50.9259014965511));
#196342=CARTESIAN_POINT('Ctrl Pts',(-2.71118205042307,6.20259335111222,
50.934124220417));
#196343=CARTESIAN_POINT('Ctrl Pts',(-2.86904842766212,6.12869073454759,
50.9423469442829));
#196344=CARTESIAN_POINT('Ctrl Pts',(-3.02674770868881,6.05486634139905,
50.9505609646741));
#196345=CARTESIAN_POINT('Ctrl Pts',(-3.18177073860635,5.97486940551333,
50.9587749850653));
#196346=CARTESIAN_POINT('Ctrl Pts',(-3.33360332083826,5.88891992637836,
50.9669890054566));
#196347=CARTESIAN_POINT('Ctrl Pts',(-3.48530567711517,5.80304416563004,
50.9751959807285));
#196348=CARTESIAN_POINT('Ctrl Pts',(-3.63382272513363,5.71122620531731,
50.9834029560005));
#196349=CARTESIAN_POINT('Ctrl Pts',(-3.77866223746558,5.61373322265599,
50.9916099312724));
#196350=CARTESIAN_POINT('Ctrl Pts',(-3.92340659312845,5.51630429093864,
50.9998115147254));
#196351=CARTESIAN_POINT('Ctrl Pts',(-4.06447792909981,5.41320796294226,
51.0080130981784));
#196352=CARTESIAN_POINT('Ctrl Pts',(-4.20141045945692,5.3047562763209,51.0162146816314));
#196353=CARTESIAN_POINT('Ctrl Pts',(-4.33828050657513,5.19635407693699,
51.0244125226465));
#196354=CARTESIAN_POINT('Ctrl Pts',(-4.47101522993291,5.08260160960884,
51.0326103636615));
#196355=CARTESIAN_POINT('Ctrl Pts',(-4.59917950748939,4.96385302541178,
51.0408082046765));
#196356=CARTESIAN_POINT('Ctrl Pts',(-4.72733247494833,4.84511492040671,
51.0490053222577));
#196357=CARTESIAN_POINT('Ctrl Pts',(-4.85091553121046,4.721381814058,51.0572024398388));
#196358=CARTESIAN_POINT('Ctrl Pts',(-4.96952795103427,4.59304702173722,
51.06539955742));
#196359=CARTESIAN_POINT('Ctrl Pts',(-5.0881390511629,4.46471365728383,51.0735965837991));
#196360=CARTESIAN_POINT('Ctrl Pts',(-5.20177938066244,4.3317789716239,51.0817936101782));
#196361=CARTESIAN_POINT('Ctrl Pts',(-5.31008638998706,4.19467180252212,
51.0899906365573));
#196362=CARTESIAN_POINT('Ctrl Pts',(-5.41841188777574,4.05754122864734,
51.0981890622034));
#196363=CARTESIAN_POINT('Ctrl Pts',(-5.52140202912524,3.91623703388157,
51.1063874878495));
#196364=CARTESIAN_POINT('Ctrl Pts',(-5.61873571006714,3.7712196993037,51.1145859134956));
#196365=CARTESIAN_POINT('Ctrl Pts',(-5.71610370468702,3.62615124081814,
51.1227872293863));
#196366=CARTESIAN_POINT('Ctrl Pts',(-5.80781106676032,3.47736733270664,
51.1309885452769));
#196367=CARTESIAN_POINT('Ctrl Pts',(-5.8935810039394,3.32535591328277,51.1391898611676));
#196368=CARTESIAN_POINT('Ctrl Pts',(-5.97944861871954,3.17317137829798,
51.1474005169842));
#196369=CARTESIAN_POINT('Ctrl Pts',(-6.0593651233506,3.0177523016584,51.1556111728008));
#196370=CARTESIAN_POINT('Ctrl Pts',(-6.13310006773624,2.85961056074664,
51.1638218286174));
#196371=CARTESIAN_POINT('Ctrl Pts',(-6.20687846233823,2.70137563073829,
51.1720373227745));
#196372=CARTESIAN_POINT('Ctrl Pts',(-6.27446789694731,2.54041516863319,
51.1802528169316));
#196373=CARTESIAN_POINT('Ctrl Pts',(-6.33568682700757,2.37725922652174,
51.1884683110888));
#196374=CARTESIAN_POINT('Ctrl Pts',(-6.39700073936435,2.21385014496376,
51.1966965517363));
#196375=CARTESIAN_POINT('Ctrl Pts',(-6.45192428225839,2.04823911658065,
51.2049247923838));
#196376=CARTESIAN_POINT('Ctrl Pts',(-6.50032598710557,1.88097077631737,
51.2131530330313));
#196377=CARTESIAN_POINT('Ctrl Pts',(-6.54431540942763,1.72895055958778,
51.2206311901325));
#196378=CARTESIAN_POINT('Ctrl Pts',(-6.58291845139467,1.57556175889647,
51.2281093472336));
#196379=CARTESIAN_POINT('Ctrl Pts',(-6.61607344889597,1.42121818128458,
51.2355875043348));
#196380=CARTESIAN_POINT('Ctrl Pts',(-6.66575370129441,1.18994602113622,
51.2467929563106));
#196381=CARTESIAN_POINT('Ctrl Pts',(-6.70334113414235,0.955893976418295,
51.2579984082865));
#196382=CARTESIAN_POINT('Ctrl Pts',(-6.72857472823353,0.720118828095116,
51.2692038602624));
#196383=CARTESIAN_POINT('Ctrl Pts',(-6.75380832232471,0.484343679771937,
51.2804093122382));
#196384=CARTESIAN_POINT('Ctrl Pts',(-6.76668789431658,0.246844735791887,
51.2916147642141));
#196385=CARTESIAN_POINT('Ctrl Pts',(-6.76699439492061,0.00870971372223031,
51.3028202161899));
#196386=CARTESIAN_POINT('Ctrl Pts',(-6.76699439492168,0.00870971288473129,
51.3028202162293));
#196387=CARTESIAN_POINT('Ctrl Pts',(-6.76721129645552,-0.159811509704027,
51.3107499883821));
#196388=CARTESIAN_POINT('Ctrl Pts',(-6.76112905601941,-0.32857630920491,
51.318679760535));
#196389=CARTESIAN_POINT('Ctrl Pts',(-6.74872017415013,-0.497056345919674,
51.3266095326878));
#196390=CARTESIAN_POINT('Ctrl Pts',(-6.73632102486479,-0.665404239697082,
51.33453308533));
#196391=CARTESIAN_POINT('Ctrl Pts',(-6.71760513327507,-0.833467434534488,
51.3424566379721));
#196392=CARTESIAN_POINT('Ctrl Pts',(-6.69259704942585,-1.00071661024312,
51.3503801906143));
#196393=CARTESIAN_POINT('Ctrl Pts',(-6.66760286110771,-1.16787285535639,
51.3582993406012));
#196394=CARTESIAN_POINT('Ctrl Pts',(-6.63632349363579,-1.33421560290597,
51.3662184905881));
#196395=CARTESIAN_POINT('Ctrl Pts',(-6.5988353961203,-1.49921993546972,
51.374137640575));
#196396=CARTESIAN_POINT('Ctrl Pts',(-6.56135387818638,-1.66419530792246,
51.3820554006623));
#196397=CARTESIAN_POINT('Ctrl Pts',(-6.51766587443334,-1.82783235690557,
51.3899731607495));
#196398=CARTESIAN_POINT('Ctrl Pts',(-6.46789907706397,-1.98961567367042,
51.3978909208368));
#196399=CARTESIAN_POINT('Ctrl Pts',(-6.41813475745096,-2.15139093567463,
51.4058082867198));
#196400=CARTESIAN_POINT('Ctrl Pts',(-6.36229235824538,-2.31131228174197,
51.4137256526029));
#196401=CARTESIAN_POINT('Ctrl Pts',(-6.30054953263265,-2.46887921673833,
51.421643018486));
#196402=CARTESIAN_POINT('Ctrl Pts',(-6.2387970222584,-2.62647086712754,
51.4295616262591));
#196403=CARTESIAN_POINT('Ctrl Pts',(-6.17114238463177,-2.78170701433539,
51.4374802340322));
#196404=CARTESIAN_POINT('Ctrl Pts',(-6.09781141086639,-2.93410718916465,
51.4453988418053));
#196405=CARTESIAN_POINT('Ctrl Pts',(-6.02445376858468,-3.08656278786656,
51.4533203293645));
#196406=CARTESIAN_POINT('Ctrl Pts',(-5.94541585065988,-3.2361800172617,
51.4612418169238));
#196407=CARTESIAN_POINT('Ctrl Pts',(-5.86096922732225,-3.38250332097126,
51.469163304483));
#196408=CARTESIAN_POINT('Ctrl Pts',(-5.77642537651826,-3.52899509375073,
51.4770939124325));
#196409=CARTESIAN_POINT('Ctrl Pts',(-5.68646058178355,-3.67218503831081,
51.4850245203821));
#196410=CARTESIAN_POINT('Ctrl Pts',(-5.59138988576118,-3.8116463825239,
51.4929551283316));
#196411=CARTESIAN_POINT('Ctrl Pts',(-5.49625815209595,-3.95119726422939,
51.5008908279197));
#196412=CARTESIAN_POINT('Ctrl Pts',(-5.39601422114059,-4.08701447504856,
51.5088265275077));
#196413=CARTESIAN_POINT('Ctrl Pts',(-5.29101265159158,-4.21870526591961,
51.5167622270957));
#196414=CARTESIAN_POINT('Ctrl Pts',(-5.18585329922107,-4.35059394473307,
51.52470985143));
#196415=CARTESIAN_POINT('Ctrl Pts',(-5.07592228849749,-4.47834353926268,
51.5326574757643));
#196416=CARTESIAN_POINT('Ctrl Pts',(-4.96161065321741,-4.60159849681386,
51.5406051000986));
#196417=CARTESIAN_POINT('Ctrl Pts',(-4.89980573467658,-4.66823880506016,
51.5449021453938));
#196418=CARTESIAN_POINT('Ctrl Pts',(-4.83672082785942,-4.73356591591269,
51.5491991906891));
#196419=CARTESIAN_POINT('Ctrl Pts',(-4.77242149879536,-4.79752874278371,
51.5534962359843));
#196420=CARTESIAN_POINT('Ctrl Pts',(-4.6477308660626,-4.92156682327407,
51.561829158031));
#196421=CARTESIAN_POINT('Ctrl Pts',(-4.51804134224386,-5.04089995580397,
51.5701620800777));
#196422=CARTESIAN_POINT('Ctrl Pts',(-4.38373745032378,-5.15510765810267,
51.5784950021244));
#196423=CARTESIAN_POINT('Ctrl Pts',(-4.24959227303486,-5.26918039459295,
51.5868180766781));
#196424=CARTESIAN_POINT('Ctrl Pts',(-4.11084385337876,-5.37813954342007,
51.5951411512317));
#196425=CARTESIAN_POINT('Ctrl Pts',(-3.96791409691977,-5.48160074425941,
51.6034642257853));
#196426=CARTESIAN_POINT('Ctrl Pts',(-3.82512701319462,-5.58495866994643,
51.6117789922312));
#196427=CARTESIAN_POINT('Ctrl Pts',(-3.67816718835495,-5.68282937887212,
51.6200937586772));
#196428=CARTESIAN_POINT('Ctrl Pts',(-3.52749037203691,-5.77486802231765,
51.6284085251232));
#196429=CARTESIAN_POINT('Ctrl Pts',(-3.37693632238244,-5.86683167561239,
51.6367165169627));
#196430=CARTESIAN_POINT('Ctrl Pts',(-3.2226716114118,-5.95297255114884,
51.6450245088022));
#196431=CARTESIAN_POINT('Ctrl Pts',(-3.0651819858386,-6.03298834688834,
51.6533325006417));
#196432=CARTESIAN_POINT('Ctrl Pts',(-2.90779180464315,-6.11295361789653,
51.6616352465288));
#196433=CARTESIAN_POINT('Ctrl Pts',(-2.74718107632359,-6.18680135958582,
51.6699379924159));
#196434=CARTESIAN_POINT('Ctrl Pts',(-2.58386142486764,-6.25427446927947,
51.678240738303));
#196435=CARTESIAN_POINT('Ctrl Pts',(-2.42060851694903,-6.32172000486323,
51.6865400911224));
#196436=CARTESIAN_POINT('Ctrl Pts',(-2.25464921283202,-6.38279596668328,
51.6948394439418));
#196437=CARTESIAN_POINT('Ctrl Pts',(-2.08651672289654,-6.4372926735603,
51.7031387967613));
#196438=CARTESIAN_POINT('Ctrl Pts',(-1.91841999192032,-6.49177778990225,
51.7114363844476));
#196439=CARTESIAN_POINT('Ctrl Pts',(-1.74815132669517,-6.53968633180688,
51.719733972134));
#196440=CARTESIAN_POINT('Ctrl Pts',(-1.57626100065361,-6.58085786640454,
51.7280315598203));
#196441=CARTESIAN_POINT('Ctrl Pts',(-1.40437866888195,-6.62202748619776,
51.7363287616027));
#196442=CARTESIAN_POINT('Ctrl Pts',(-1.23087516493557,-6.65646064218201,
51.7446259633851));
#196443=CARTESIAN_POINT('Ctrl Pts',(-1.05631309820776,-6.68404754909439,
51.7529231651675));
#196444=CARTESIAN_POINT('Ctrl Pts',(-0.88173014340526,-6.71163775705254,
51.761221359792));
#196445=CARTESIAN_POINT('Ctrl Pts',(-0.706088717132015,-6.73238002983325,
51.7695195544165));
#196446=CARTESIAN_POINT('Ctrl Pts',(-0.529958924265151,-6.74621616453192,
51.7778177490411));
#196447=CARTESIAN_POINT('Ctrl Pts',(-0.353705257260737,-6.76006203034549,
51.7861217798826));
#196448=CARTESIAN_POINT('Ctrl Pts',(-0.176962884594447,-6.76699202522156,
51.7944258107242));
#196449=CARTESIAN_POINT('Ctrl Pts',(-0.00030521600168854,-6.76699999311683,
51.8027298415658));
#196450=CARTESIAN_POINT('Ctrl Pts',(0.176416690181065,-6.76700796390945,
51.8110368919815));
#196451=CARTESIAN_POINT('Ctrl Pts',(0.353053483044433,-6.76008889831693,
51.8193439423972));
#196452=CARTESIAN_POINT('Ctrl Pts',(0.529034250924517,-6.74628873984421,
51.8276509928129));
#196453=CARTESIAN_POINT('Ctrl Pts',(0.705203171946611,-6.73247382667296,
51.8359669248676));
#196454=CARTESIAN_POINT('Ctrl Pts',(0.880714320129311,-6.71176315574064,
51.8442828569222));
#196455=CARTESIAN_POINT('Ctrl Pts',(1.05500328018712,-6.68425441457717,
51.8525987889768));
#196456=CARTESIAN_POINT('Ctrl Pts',(1.18638600029699,-6.66351774118342,
51.8588675151958));
#196457=CARTESIAN_POINT('Ctrl Pts',(1.31707435499131,-6.63891915865807,
51.8651362414147));
#196458=CARTESIAN_POINT('Ctrl Pts',(1.44683147260502,-6.61051947201425,
51.8714049676337));
#196459=CARTESIAN_POINT('Ctrl Pts',(1.62174460077588,-6.57223657762437,
51.879855236357));
#196460=CARTESIAN_POINT('Ctrl Pts',(1.79528584323523,-6.52697470531072,
51.8883055050804));
#196461=CARTESIAN_POINT('Ctrl Pts',(1.96687850332887,-6.4748496471457,51.8967557738037));
#196462=CARTESIAN_POINT('Ctrl Pts',(2.13831972707799,-6.42277059111307,
51.9051985848782));
#196463=CARTESIAN_POINT('Ctrl Pts',(2.30781548032498,-6.36384051783906,
51.9136413959527));
#196464=CARTESIAN_POINT('Ctrl Pts',(2.4748009504396,-6.29822588160374,51.9220842070271));
#196465=CARTESIAN_POINT('Ctrl Pts',(2.64166178571239,-6.23266021890968,
51.9305207165448));
#196466=CARTESIAN_POINT('Ctrl Pts',(2.80601576522364,-6.16042005987778,
51.9389572260625));
#196467=CARTESIAN_POINT('Ctrl Pts',(2.96731452036559,-6.0817212643484,51.9473937355802));
#196468=CARTESIAN_POINT('Ctrl Pts',(3.12849785756989,-6.00307878204146,
51.9558242083215));
#196469=CARTESIAN_POINT('Ctrl Pts',(3.28663003380628,-5.91798702661201,
51.9642546810627));
#196470=CARTESIAN_POINT('Ctrl Pts',(3.44118371426143,-5.8267095040599,51.9726851538039));
#196471=CARTESIAN_POINT('Ctrl Pts',(3.59567095250719,-5.73547122146796,
51.9811120023077));
#196472=CARTESIAN_POINT('Ctrl Pts',(3.74658247681241,-5.63805264135766,
51.9895388508115));
#196473=CARTESIAN_POINT('Ctrl Pts',(3.89341599374254,-5.53476294882354,
51.9979656993153));
#196474=CARTESIAN_POINT('Ctrl Pts',(4.04020418841084,-5.43150513812803,
52.0063899467519));
#196475=CARTESIAN_POINT('Ctrl Pts',(4.18291661503389,-5.32238001952461,
52.0148141941886));
#196476=CARTESIAN_POINT('Ctrl Pts',(4.32108008899238,-5.20773999586323,
52.0232384416253));
#196477=CARTESIAN_POINT('Ctrl Pts',(4.36000926974064,-5.17543882338809,
52.0256120722364));
#196478=CARTESIAN_POINT('Ctrl Pts',(4.39857749904668,-5.14270007998872,
52.0279857028475));
#196479=CARTESIAN_POINT('Ctrl Pts',(4.4367746488298,-5.10953224038182,52.0303593334587));
#196480=CARTESIAN_POINT('Ctrl Pts',(4.57547056253417,-4.98909802353581,
52.038978114396));
#196481=CARTESIAN_POINT('Ctrl Pts',(4.70920929362458,-4.86305725438358,
52.0475968953332));
#196482=CARTESIAN_POINT('Ctrl Pts',(4.83755419002768,-4.73184514312817,
52.0562156762705));
#196483=CARTESIAN_POINT('Ctrl Pts',(4.96597618242891,-4.60055421355612,
52.064839634457));
#196484=CARTESIAN_POINT('Ctrl Pts',(5.08899766130541,-4.4640859599079,52.0734635926436));
#196485=CARTESIAN_POINT('Ctrl Pts',(5.20622052148926,-4.32291069554116,
52.0820875508301));
#196486=CARTESIAN_POINT('Ctrl Pts',(5.32767824365046,-4.17663525055887,
52.0910230632012));
#196487=CARTESIAN_POINT('Ctrl Pts',(5.44291034106364,-4.02530663931312,
52.0999585755723));
#196488=CARTESIAN_POINT('Ctrl Pts',(5.5515216575626,-3.86948268966453,52.1088940879434));
#196489=CARTESIAN_POINT('Ctrl Pts',(5.65654201121118,-3.71881067107087,
52.1175341698381));
#196490=CARTESIAN_POINT('Ctrl Pts',(5.75537225130303,-3.5639360925001,52.1261742517328));
#196491=CARTESIAN_POINT('Ctrl Pts',(5.84770073397215,-3.40539059814019,
52.1348143336276));
#196492=CARTESIAN_POINT('Ctrl Pts',(5.94476470085616,-3.23871338034912,
52.1438975612369));
#196493=CARTESIAN_POINT('Ctrl Pts',(6.03464226453751,-3.06797914483941,
52.1529807888462));
#196494=CARTESIAN_POINT('Ctrl Pts',(6.11702720501719,-2.89383260972013,
52.1620640164555));
#196495=CARTESIAN_POINT('Ctrl Pts',(6.19941214549684,-2.71968607460092,
52.1711472440648));
#196496=CARTESIAN_POINT('Ctrl Pts',(6.27430434308154,-2.54212761024528,
52.1802304716741));
#196497=CARTESIAN_POINT('Ctrl Pts',(6.34145688008563,-2.36182421827169,
52.1893136992833));
#196498=CARTESIAN_POINT('Ctrl Pts',(6.40832380417191,-2.18228769200666,
52.1983582941431));
#196499=CARTESIAN_POINT('Ctrl Pts',(6.4675793353938,-1.99986404640702,52.2074028890029));
#196500=CARTESIAN_POINT('Ctrl Pts',(6.51900169662694,-1.81518756038461,
52.2164474838627));
#196501=CARTESIAN_POINT('Ctrl Pts',(6.57037686974953,-1.63068054410709,
52.2254837788831));
#196502=CARTESIAN_POINT('Ctrl Pts',(6.61393316033545,-1.44392504383055,
52.2345200739034));
#196503=CARTESIAN_POINT('Ctrl Pts',(6.64949862910018,-1.25557038098021,
52.2435563689238));
#196504=CARTESIAN_POINT('Ctrl Pts',(6.68500116197888,-1.06754902647664,
52.2525766735114));
#196505=CARTESIAN_POINT('Ctrl Pts',(6.71254106550225,-0.877934393694752,
52.2615969780991));
#196506=CARTESIAN_POINT('Ctrl Pts',(6.73199746713134,-0.687385701434986,
52.2706172826868));
#196507=CARTESIAN_POINT('Ctrl Pts',(6.75142936720212,-0.497076968237626,
52.2796262279531));
#196508=CARTESIAN_POINT('Ctrl Pts',(6.76279805626797,-0.305836758941343,
52.2886351732194));
#196509=CARTESIAN_POINT('Ctrl Pts',(6.7660340872941,-0.11433166479313,52.2976441184858));
#196510=CARTESIAN_POINT('Ctrl Pts',(6.76926276997881,0.076738561826771,
52.3066326063445));
#196511=CARTESIAN_POINT('Ctrl Pts',(6.76439565342507,0.268072235237285,
52.3156210942033));
#196512=CARTESIAN_POINT('Ctrl Pts',(6.75141519215947,0.459000983744335,
52.324609582062));
#196513=CARTESIAN_POINT('Ctrl Pts',(6.74002662389274,0.626514683139328,
52.3324957430774));
#196514=CARTESIAN_POINT('Ctrl Pts',(6.72239343122672,0.793716490812133,
52.3403819040927));
#196515=CARTESIAN_POINT('Ctrl Pts',(6.69853677078782,0.960153180697496,
52.3482680651081));
#196516=CARTESIAN_POINT('Ctrl Pts',(6.67396828569565,1.13155593611291,52.3563895299643));
#196517=CARTESIAN_POINT('Ctrl Pts',(6.64280878500894,1.30207027473601,52.3645109948204));
#196518=CARTESIAN_POINT('Ctrl Pts',(6.6051497495303,1.47115117723498,52.3726324596766));
#196519=CARTESIAN_POINT('Ctrl Pts',(6.5674933996951,1.64022002177731,52.3807533453528));
#196520=CARTESIAN_POINT('Ctrl Pts',(6.52333851792854,1.80785527638499,52.388874231029));
#196521=CARTESIAN_POINT('Ctrl Pts',(6.47282754051543,1.97352289845976,52.3969951167052));
#196522=CARTESIAN_POINT('Ctrl Pts',(6.42231052559608,2.13921032255288,52.4051169730595));
#196523=CARTESIAN_POINT('Ctrl Pts',(6.36543601016475,2.30292929588791,52.4132388294138));
#196524=CARTESIAN_POINT('Ctrl Pts',(6.30239604248319,2.46416174868702,52.4213606857681));
#196525=CARTESIAN_POINT('Ctrl Pts',(6.23931008162123,2.62551183468867,52.4294884677282));
#196526=CARTESIAN_POINT('Ctrl Pts',(6.17004981778485,2.78437143543766,52.4376162496884));
#196527=CARTESIAN_POINT('Ctrl Pts',(6.09485537691689,2.94024266591507,52.4457440316486));
#196528=CARTESIAN_POINT('Ctrl Pts',(6.01963030462878,3.09617739253786,52.453875124565));
#196529=CARTESIAN_POINT('Ctrl Pts',(5.93846640835912,3.24912099913245,52.4620062174814));
#196530=CARTESIAN_POINT('Ctrl Pts',(5.85164924493249,3.39860119965275,52.4701373103979));
#196531=CARTESIAN_POINT('Ctrl Pts',(5.7647373242001,3.54824455156507,52.4782772780624));
#196532=CARTESIAN_POINT('Ctrl Pts',(5.67216000784978,3.69441663817258,52.486417245727));
#196533=CARTESIAN_POINT('Ctrl Pts',(5.5742459600096,3.83667446851002,52.4945572133915));
#196534=CARTESIAN_POINT('Ctrl Pts',(5.52346350126786,3.91045553015699,52.498778952572));
#196535=CARTESIAN_POINT('Ctrl Pts',(5.47124618168525,3.983184225787,52.5030006917524));
#196536=CARTESIAN_POINT('Ctrl Pts',(5.41764399782902,4.05480240120122,52.5072224309329));
#196537=CARTESIAN_POINT('Ctrl Pts',(5.31047721113774,4.19798853981865,52.5156629493907));
#196538=CARTESIAN_POINT('Ctrl Pts',(5.1975510084198,4.33702963227614,52.5241034678485));
#196539=CARTESIAN_POINT('Ctrl Pts',(5.079212594634,4.47145260720847,52.5325439863063));
#196540=CARTESIAN_POINT('Ctrl Pts',(4.96096191138293,4.60577592726885,52.5409782473607));
#196541=CARTESIAN_POINT('Ctrl Pts',(4.83730723448576,4.73548770469269,52.5494125084151));
#196542=CARTESIAN_POINT('Ctrl Pts',(4.70863665742514,4.86014709945618,52.5578467694695));
#196543=CARTESIAN_POINT('Ctrl Pts',(4.58005485344859,4.98472048855166,52.5662752115139));
#196544=CARTESIAN_POINT('Ctrl Pts',(4.4464642901457,5.10424821561085,52.5747036535584));
#196545=CARTESIAN_POINT('Ctrl Pts',(4.30829074449172,5.21832538856356,52.5831320956028));
#196546=CARTESIAN_POINT('Ctrl Pts',(4.17017545649127,5.33235446353639,52.5915569839912));
#196547=CARTESIAN_POINT('Ctrl Pts',(4.02748129480552,5.44093735359852,52.5999818723796));
#196548=CARTESIAN_POINT('Ctrl Pts',(3.8806684656216,5.54370825891209,52.608406760768));
#196549=CARTESIAN_POINT('Ctrl Pts',(3.73389156471692,5.64645401395913,52.6168295874037));
#196550=CARTESIAN_POINT('Ctrl Pts',(3.58299827789504,5.74339042764865,52.6252524140394));
#196551=CARTESIAN_POINT('Ctrl Pts',(3.42847960027908,5.83419374296656,52.6336752406752));
#196552=CARTESIAN_POINT('Ctrl Pts',(3.32040276338655,5.897705386027,52.6395665185098));
#196553=CARTESIAN_POINT('Ctrl Pts',(3.21055297173536,5.95821747173756,52.6454577963445));
#196554=CARTESIAN_POINT('Ctrl Pts',(3.09910619832128,6.01563211736943,52.6513490741792));
#196555=CARTESIAN_POINT('Origin',(0.,0.,4.30282021618968));
#196556=CARTESIAN_POINT('',(3.09910619832139,6.01563211736937,55.0459882871872));
#196557=CARTESIAN_POINT('',(3.09910619832136,6.01563211736939,54.6512861468277));
#196558=CARTESIAN_POINT('',(3.09910619832133,6.0156321173694,4.30282021618968));
#196559=CARTESIAN_POINT('',(-6.7669990509716,-0.00358387352824917,53.6971797838396));
#196560=CARTESIAN_POINT('Ctrl Pts',(-6.7669990509716,-0.00358387352833798,
53.6971797838396));
#196561=CARTESIAN_POINT('Ctrl Pts',(-6.76689217047806,-0.20539350566186,
53.706683992129));
#196562=CARTESIAN_POINT('Ctrl Pts',(-6.75775334083001,-0.407019112576732,
53.7161882004184));
#196563=CARTESIAN_POINT('Ctrl Pts',(-6.73965675319555,-0.607713624255395,
53.7256924087078));
#196564=CARTESIAN_POINT('Ctrl Pts',(-6.7215721742797,-0.808274957018417,
53.7351903100976));
#196565=CARTESIAN_POINT('Ctrl Pts',(-6.69454179296501,-1.00790630788709,
53.7446882114873));
#196566=CARTESIAN_POINT('Ctrl Pts',(-6.6586905907916,-1.20587255383953,
53.754186112877));
#196567=CARTESIAN_POINT('Ctrl Pts',(-6.62455045966254,-1.39439046080544,
53.7632307077369));
#196568=CARTESIAN_POINT('Ctrl Pts',(-6.58239146852269,-1.58150599709402,
53.7722753025967));
#196569=CARTESIAN_POINT('Ctrl Pts',(-6.53234666004299,-1.76656053194482,
53.7813198974565));
#196570=CARTESIAN_POINT('Ctrl Pts',(-6.48234777555245,-1.95144525013112,
53.7903561924769));
#196571=CARTESIAN_POINT('Ctrl Pts',(-6.42447758343751,-2.13427251340943,
53.7993924874972));
#196572=CARTESIAN_POINT('Ctrl Pts',(-6.35891966107565,-2.31439619425575,
53.8084287825176));
#196573=CARTESIAN_POINT('Ctrl Pts',(-6.29347774859843,-2.49420113212362,
53.8174490871053));
#196574=CARTESIAN_POINT('Ctrl Pts',(-6.22037535266763,-2.67131181774264,
53.826469391693));
#196575=CARTESIAN_POINT('Ctrl Pts',(-6.13984501590862,-2.84509967850374,
53.8354896962807));
#196576=CARTESIAN_POINT('Ctrl Pts',(-6.05941609146528,-3.01866868721349,
53.844498641547));
#196577=CARTESIAN_POINT('Ctrl Pts',(-5.97157799337865,-3.18892300659289,
53.8535075868134));
#196578=CARTESIAN_POINT('Ctrl Pts',(-5.87661124923286,-3.35525397330661,
53.8625165320797));
#196579=CARTESIAN_POINT('Ctrl Pts',(-5.78186015445875,-3.52120723760687,
53.8715050199385));
#196580=CARTESIAN_POINT('Ctrl Pts',(-5.68001284330018,-3.68325472636994,
53.8804935077973));
#196581=CARTESIAN_POINT('Ctrl Pts',(-5.57139538336093,-3.84081273720349,
53.8894819956561));
#196582=CARTESIAN_POINT('Ctrl Pts',(-5.476098511228,-3.97904820708394,53.8973681566713));
#196583=CARTESIAN_POINT('Ctrl Pts',(-5.37559095502018,-4.11382804651479,
53.9052543176866));
#196584=CARTESIAN_POINT('Ctrl Pts',(-5.27012224682619,-4.24477331591543,
53.9131404787018));
#196585=CARTESIAN_POINT('Ctrl Pts',(-5.16150660920894,-4.37962567328717,
53.921261943558));
#196586=CARTESIAN_POINT('Ctrl Pts',(-5.04767669280879,-4.51034982672275,
53.9293834084142));
#196587=CARTESIAN_POINT('Ctrl Pts',(-4.92898935674534,-4.63652379710179,
53.9375048732703));
#196588=CARTESIAN_POINT('Ctrl Pts',(-4.81031048483593,-4.76268876941956,
53.9456257589465));
#196589=CARTESIAN_POINT('Ctrl Pts',(-4.68677513415301,-4.88430393830359,
53.9537466446227));
#196590=CARTESIAN_POINT('Ctrl Pts',(-4.55877837866638,-5.00098277283615,
53.9618675302989));
#196591=CARTESIAN_POINT('Ctrl Pts',(-4.43076632390726,-5.11767555382599,
53.9699893866532));
#196592=CARTESIAN_POINT('Ctrl Pts',(-4.29829207391614,-5.22943057977352,
53.9781112430074));
#196593=CARTESIAN_POINT('Ctrl Pts',(-4.16178521206458,-5.33590037844042,
53.9862330993617));
#196594=CARTESIAN_POINT('Ctrl Pts',(-4.02517875649533,-5.44244785615529,
53.9943608813218));
#196595=CARTESIAN_POINT('Ctrl Pts',(-3.88453410184469,-5.54370217959386,
54.002488663282));
#196596=CARTESIAN_POINT('Ctrl Pts',(-3.74031187162378,-5.63935777398368,
54.0106164452422));
#196597=CARTESIAN_POINT('Ctrl Pts',(-3.59603089062665,-5.7350523349074,
54.0187475381586));
#196598=CARTESIAN_POINT('Ctrl Pts',(-3.44816974160194,-5.82514343027827,
54.0268786310751));
#196599=CARTESIAN_POINT('Ctrl Pts',(-3.2972150485986,-5.90937068758552,
54.0350097239916));
#196600=CARTESIAN_POINT('Ctrl Pts',(-3.1460955948567,-5.99368987542401,
54.0431496916561));
#196601=CARTESIAN_POINT('Ctrl Pts',(-2.99187617918848,-6.07213227618284,
54.0512896593206));
#196602=CARTESIAN_POINT('Ctrl Pts',(-2.83506554149222,-6.14448471195457,
54.0594296269852));
#196603=CARTESIAN_POINT('Ctrl Pts',(-2.75373676472572,-6.18200981346452,
54.0636513661657));
#196604=CARTESIAN_POINT('Ctrl Pts',(-2.67171127792406,-6.21789757109083,
54.0678731053461));
#196605=CARTESIAN_POINT('Ctrl Pts',(-2.58906175767844,-6.25212349645519,
54.0720948445266));
#196606=CARTESIAN_POINT('Ctrl Pts',(-2.42382671291955,-6.32054884596341,
54.0805350539842));
#196607=CARTESIAN_POINT('Ctrl Pts',(-2.25575498027963,-6.3824704961414,
54.0889752634419));
#196608=CARTESIAN_POINT('Ctrl Pts',(-2.08538653745964,-6.43765889041833,
54.0974154728995));
#196609=CARTESIAN_POINT('Ctrl Pts',(-1.91514717397523,-6.49280547131041,
54.105849287648));
#196610=CARTESIAN_POINT('Ctrl Pts',(-1.74261488519324,-6.54122886327688,
54.1142831023966));
#196611=CARTESIAN_POINT('Ctrl Pts',(-1.56834832785497,-6.58274809806015,
54.1227169171451));
#196612=CARTESIAN_POINT('Ctrl Pts',(-1.39418701379491,-6.624242258495,54.1311456385336));
#196613=CARTESIAN_POINT('Ctrl Pts',(-1.21829384283528,-6.65884049728079,
54.1395743599222));
#196614=CARTESIAN_POINT('Ctrl Pts',(-1.04124167351343,-6.686411950915,54.1480030813107));
#196615=CARTESIAN_POINT('Ctrl Pts',(-0.864269241991779,-6.71397098737822,
54.1564280067125));
#196616=CARTESIAN_POINT('Ctrl Pts',(-0.686139181822217,-6.73450949732994,
54.1648529321142));
#196617=CARTESIAN_POINT('Ctrl Pts',(-0.507433955419252,-6.74794781995886,
54.1732778575159));
#196618=CARTESIAN_POINT('Ctrl Pts',(-0.328781792614159,-6.7613821522974,
54.1817002812736));
#196619=CARTESIAN_POINT('Ctrl Pts',(-0.149555136351088,-6.76772047671474,
54.1901227050314));
#196620=CARTESIAN_POINT('Ctrl Pts',(0.0296586264785453,-6.76693500529416,
54.1985451287891));
#196621=CARTESIAN_POINT('Ctrl Pts',(0.208875207824346,-6.76614952152037,
54.2069676850073));
#196622=CARTESIAN_POINT('Ctrl Pts',(0.388078561905396,-6.75824001286657,
54.2153902412255));
#196623=CARTESIAN_POINT('Ctrl Pts',(0.56668081765754,-6.74323081696741,
54.2238127974437));
#196624=CARTESIAN_POINT('Ctrl Pts',(0.745289106627769,-6.72822111405477,
54.2322356381774));
#196625=CARTESIAN_POINT('Ctrl Pts',(0.923295924362521,-6.70611127346617,
54.2406584789112));
#196626=CARTESIAN_POINT('Ctrl Pts',(1.10011788045682,-6.6769775833905,54.2490813196449));
#196627=CARTESIAN_POINT('Ctrl Pts',(1.27697049593126,-6.64783884178787,
54.2575056208255));
#196628=CARTESIAN_POINT('Ctrl Pts',(1.45263751104816,-6.61167387684255,
54.2659299220062));
#196629=CARTESIAN_POINT('Ctrl Pts',(1.62654472881587,-6.56861029786068,
54.2743542231868));
#196630=CARTESIAN_POINT('Ctrl Pts',(1.80050638738515,-6.52553323803661,
54.2827811615536));
#196631=CARTESIAN_POINT('Ctrl Pts',(1.97270682661158,-6.47555333871034,
54.2912080999204));
#196632=CARTESIAN_POINT('Ctrl Pts',(2.14258567628876,-6.41884846524377,
54.2996350382872));
#196633=CARTESIAN_POINT('Ctrl Pts',(2.31261726840537,-6.36209260696821,
54.3080695535309));
#196634=CARTESIAN_POINT('Ctrl Pts',(2.48032278330943,-6.29859979820912,
54.3165040687745));
#196635=CARTESIAN_POINT('Ctrl Pts',(2.64515947001497,-6.2285969831247,54.3249385840182));
#196636=CARTESIAN_POINT('Ctrl Pts',(2.8100757742525,-6.15856035608082,54.333377173205));
#196637=CARTESIAN_POINT('Ctrl Pts',(2.97212018312097,-6.08200758935251,
54.3418157623917));
#196638=CARTESIAN_POINT('Ctrl Pts',(3.13077285188469,-5.99921247747584,
54.3502543515785));
#196639=CARTESIAN_POINT('Ctrl Pts',(3.28960285843758,-5.91632481939614,
54.3587023731988));
#196640=CARTESIAN_POINT('Ctrl Pts',(3.4450332575324,-5.82718103540334,54.3671503948191));
#196641=CARTESIAN_POINT('Ctrl Pts',(3.59657053059673,-5.73209991350841,
54.3755984164394));
#196642=CARTESIAN_POINT('Ctrl Pts',(3.68270188468435,-5.6780573297178,54.3804001363516));
#196643=CARTESIAN_POINT('Ctrl Pts',(3.76757605959588,-5.62209741664671,
54.3852018562638));
#196644=CARTESIAN_POINT('Ctrl Pts',(3.85110698088934,-5.56428468194659,
54.3900035761761));
#196645=CARTESIAN_POINT('Ctrl Pts',(3.99444222307462,-5.465080672206,54.3982431080269));
#196646=CARTESIAN_POINT('Ctrl Pts',(4.13414038505795,-5.36019723159368,
54.4064826398777));
#196647=CARTESIAN_POINT('Ctrl Pts',(4.26972379138673,-5.24992835620318,
54.4147221717285));
#196648=CARTESIAN_POINT('Ctrl Pts',(4.4051567096104,-5.13978187155767,54.4229525582748));
#196649=CARTESIAN_POINT('Ctrl Pts',(4.53648369234045,-5.02426207683795,
54.4311829448211));
#196650=CARTESIAN_POINT('Ctrl Pts',(4.6632554213212,-4.90370654459649,54.4394133313674));
#196651=CARTESIAN_POINT('Ctrl Pts',(4.78990905745408,-4.78326331457134,
54.4476360509852));
#196652=CARTESIAN_POINT('Ctrl Pts',(4.91201563424525,-4.65779393302532,
54.455858770603));
#196653=CARTESIAN_POINT('Ctrl Pts',(5.02915830110851,-4.52767664287009,
54.4640814902208));
#196654=CARTESIAN_POINT('Ctrl Pts',(5.14619717112908,-4.39767464600858,
54.4722969239166));
#196655=CARTESIAN_POINT('Ctrl Pts',(5.25828066038809,-4.26303321235824,
54.4805123576123));
#196656=CARTESIAN_POINT('Ctrl Pts',(5.36502833791073,-4.124167786768,54.4887277913081));
#196657=CARTESIAN_POINT('Ctrl Pts',(5.47172115541633,-3.98537372722328,
54.4969390029089));
#196658=CARTESIAN_POINT('Ctrl Pts',(5.57308340612662,-3.84236028056674,
54.5051502145097));
#196659=CARTESIAN_POINT('Ctrl Pts',(5.66877430356654,-3.69557666612719,
54.5133614261105));
#196660=CARTESIAN_POINT('Ctrl Pts',(5.76443311155956,-3.54884227481258,
54.521569884124));
#196661=CARTESIAN_POINT('Ctrl Pts',(5.85442416079166,-3.39834053214902,
54.5297783421375));
#196662=CARTESIAN_POINT('Ctrl Pts',(5.93844940206025,-3.24455046180056,
54.537986800151));
#196663=CARTESIAN_POINT('Ctrl Pts',(5.9758844818036,-3.17603362733142,54.5416438474343));
#196664=CARTESIAN_POINT('Ctrl Pts',(6.01213599114525,-3.10686446862793,
54.5453008947176));
#196665=CARTESIAN_POINT('Ctrl Pts',(6.04718044105717,-3.03708704407623,
54.5489579420008));
#196666=CARTESIAN_POINT('Ctrl Pts',(6.13207444356175,-2.86805357744901,
54.5578170161767));
#196667=CARTESIAN_POINT('Ctrl Pts',(6.20979382233589,-2.69562484029854,
54.5666760903526));
#196668=CARTESIAN_POINT('Ctrl Pts',(6.28011180328,-2.52041360461001,54.5755351645285));
#196669=CARTESIAN_POINT('Ctrl Pts',(6.35056189756314,-2.34487318226009,
54.5844108831225));
#196670=CARTESIAN_POINT('Ctrl Pts',(6.41358270765095,-2.16654005458681,
54.5932866017164));
#196671=CARTESIAN_POINT('Ctrl Pts',(6.46899702095665,-1.98604293580326,
54.6021623203104));
#196672=CARTESIAN_POINT('Ctrl Pts',(6.52456947105544,-1.80503072924141,
54.6110633676974));
#196673=CARTESIAN_POINT('Ctrl Pts',(6.57249190950509,-1.62184242307575,
54.6199644150844));
#196674=CARTESIAN_POINT('Ctrl Pts',(6.61263736242461,-1.43712077191382,
54.6288654624714));
#196675=CARTESIAN_POINT('Ctrl Pts',(6.65283739363802,-1.25214798913337,
54.6377786109544));
#196676=CARTESIAN_POINT('Ctrl Pts',(6.68523927058451,-1.06563795189312,
54.6466917594375));
#196677=CARTESIAN_POINT('Ctrl Pts',(6.70976766854178,-0.878240760948553,
54.6556049079205));
#196678=CARTESIAN_POINT('Ctrl Pts',(6.73435052624963,-0.690427496997583,
54.6645378460304));
#196679=CARTESIAN_POINT('Ctrl Pts',(6.7510249054307,-0.501723397634979,
54.6734707841403));
#196680=CARTESIAN_POINT('Ctrl Pts',(6.75976740416614,-0.312783697741695,
54.6824037222502));
#196681=CARTESIAN_POINT('Ctrl Pts',(6.76808899535266,-0.132940498561066,
54.6909065841087));
#196682=CARTESIAN_POINT('Ctrl Pts',(6.76922448270502,0.0471159652347299,
54.6994094459671));
#196683=CARTESIAN_POINT('Ctrl Pts',(6.76319748642104,0.226823190322631,
54.7079123078255));
#196684=CARTESIAN_POINT('Ctrl Pts',(6.75736905747454,0.400609723986583,
54.7161350316914));
#196685=CARTESIAN_POINT('Ctrl Pts',(6.74483016277144,0.574402702958768,
54.7243577555573));
#196686=CARTESIAN_POINT('Ctrl Pts',(6.72557191694189,0.747643892533494,
54.7325804794232));
#196687=CARTESIAN_POINT('Ctrl Pts',(6.70633405531315,0.920701712177786,
54.7407944998144));
#196688=CARTESIAN_POINT('Ctrl Pts',(6.68039104454674,1.0932085518923,54.7490085202056));
#196689=CARTESIAN_POINT('Ctrl Pts',(6.64778599689748,1.26460679242751,54.7572225405969));
#196690=CARTESIAN_POINT('Ctrl Pts',(6.61520891441485,1.43585802565241,54.7654295158688));
#196691=CARTESIAN_POINT('Ctrl Pts',(6.57598124161398,1.60600220296919,54.7736364911408));
#196692=CARTESIAN_POINT('Ctrl Pts',(6.53019782579279,1.77448735019755,54.7818434664128));
#196693=CARTESIAN_POINT('Ctrl Pts',(6.48444448876211,1.9428618060466,54.7900450498658));
#196694=CARTESIAN_POINT('Ctrl Pts',(6.43214408145211,2.10957905792641,54.7982466333188));
#196695=CARTESIAN_POINT('Ctrl Pts',(6.37344242884872,2.27409775650718,54.8064482167718));
#196696=CARTESIAN_POINT('Ctrl Pts',(6.31476756220602,2.43854138409422,54.8146460577868));
#196697=CARTESIAN_POINT('Ctrl Pts',(6.24969738978208,2.60078811986705,54.8228438988019));
#196698=CARTESIAN_POINT('Ctrl Pts',(6.17842746963303,2.76031212048275,54.8310417398169));
#196699=CARTESIAN_POINT('Ctrl Pts',(6.10716383883211,2.91982204360303,54.8392388573981));
#196700=CARTESIAN_POINT('Ctrl Pts',(6.02970168845473,3.07660937938224,54.8474359749792));
#196701=CARTESIAN_POINT('Ctrl Pts',(5.94628471634663,3.23016827303818,54.8556330925604));
#196702=CARTESIAN_POINT('Ctrl Pts',(5.86286867234528,3.38372545818037,54.8638301189395));
#196703=CARTESIAN_POINT('Ctrl Pts',(5.77349810891769,3.53405395691857,54.8720271453186));
#196704=CARTESIAN_POINT('Ctrl Pts',(5.67846262915169,3.68067265174828,54.8802241716977));
#196705=CARTESIAN_POINT('Ctrl Pts',(5.58341092642758,3.82731637500895,54.8884225973438));
#196706=CARTESIAN_POINT('Ctrl Pts',(5.48269257594397,3.97024873156114,54.89662102299));
#196707=CARTESIAN_POINT('Ctrl Pts',(5.37664046332861,4.10901768408187,54.9048194486361));
#196708=CARTESIAN_POINT('Ctrl Pts',(5.27055096346976,4.24783555772722,54.9130207645268));
#196709=CARTESIAN_POINT('Ctrl Pts',(5.15912417356631,4.38248681863195,54.9212220804174));
#196710=CARTESIAN_POINT('Ctrl Pts',(5.04273321860242,4.51255256878009,54.9294233963081));
#196711=CARTESIAN_POINT('Ctrl Pts',(4.926209713824,4.64276644204537,54.9376340521247));
#196712=CARTESIAN_POINT('Ctrl Pts',(4.80471098912698,4.76838410399211,54.9458447079413));
#196713=CARTESIAN_POINT('Ctrl Pts',(4.67864772972981,4.88902284931193,54.9540553637579));
#196714=CARTESIAN_POINT('Ctrl Pts',(4.55251018430802,5.00973268412164,54.962270857915));
#196715=CARTESIAN_POINT('Ctrl Pts',(4.42180301076258,5.12545751644231,54.9704863520722));
#196716=CARTESIAN_POINT('Ctrl Pts',(4.28696981949483,5.23585511323036,54.9787018462293));
#196717=CARTESIAN_POINT('Ctrl Pts',(4.15192743204966,5.34642399392132,54.9869300868768));
#196718=CARTESIAN_POINT('Ctrl Pts',(4.01274652002538,5.45164890548821,54.9951583275243));
#196719=CARTESIAN_POINT('Ctrl Pts',(3.86990059370619,5.55123034964615,55.0033865681719));
#196720=CARTESIAN_POINT('Ctrl Pts',(3.74007645218726,5.64173398410144,55.010864725273));
#196721=CARTESIAN_POINT('Ctrl Pts',(3.60722555703865,5.72757662318511,55.0183428823742));
#196722=CARTESIAN_POINT('Ctrl Pts',(3.47171995776768,5.80856690887155,55.0258210394753));
#196723=CARTESIAN_POINT('Ctrl Pts',(3.34990852972529,5.88137233100985,55.0325434553793));
#196724=CARTESIAN_POINT('Ctrl Pts',(3.2256199413191,5.95045533836307,55.0392658712833));
#196725=CARTESIAN_POINT('Ctrl Pts',(3.09910619832139,6.01563211736937,55.0459882871872));
#196726=CARTESIAN_POINT('Ctrl Pts',(3.09910619832131,6.01563211736941,53.0454129677962));
#196727=CARTESIAN_POINT('Ctrl Pts',(2.94667468855627,6.09416109446034,53.0534680607862));
#196728=CARTESIAN_POINT('Ctrl Pts',(2.79140784790711,6.16681448736431,53.0615231537762));
#196729=CARTESIAN_POINT('Ctrl Pts',(2.63381441570988,6.23340281255743,53.0695782467662));
#196730=CARTESIAN_POINT('Ctrl Pts',(2.47472154848197,6.30062469757621,53.0777099805681));
#196731=CARTESIAN_POINT('Ctrl Pts',(2.31325796192262,6.36166538924136,53.0858417143701));
#196732=CARTESIAN_POINT('Ctrl Pts',(2.14996064585907,6.41638201958528,53.093973448172));
#196733=CARTESIAN_POINT('Ctrl Pts',(1.98666332979558,6.47109864992918,53.102105181974));
#196734=CARTESIAN_POINT('Ctrl Pts',(1.82153267172137,6.51949118168162,53.1102369157759));
#196735=CARTESIAN_POINT('Ctrl Pts',(1.65511355105797,6.56146996740092,53.1183686495779));
#196736=CARTESIAN_POINT('Ctrl Pts',(1.48457703408077,6.60448735551693,53.1267015716246));
#196737=CARTESIAN_POINT('Ctrl Pts',(1.31214340187037,6.64090728948818,53.1350344936713));
#196738=CARTESIAN_POINT('Ctrl Pts',(1.13835793945825,6.67056445899988,53.143367415718));
#196739=CARTESIAN_POINT('Ctrl Pts',(0.964777849319081,6.70018658092919,
53.1516904902716));
#196740=CARTESIAN_POINT('Ctrl Pts',(0.789849451455171,6.72306180095026,
53.1600135648252));
#196741=CARTESIAN_POINT('Ctrl Pts',(0.614131739318328,6.73907495185815,
53.1683366393788));
#196742=CARTESIAN_POINT('Ctrl Pts',(0.43858942891076,6.75507211841063,53.1766514058248));
#196743=CARTESIAN_POINT('Ctrl Pts',(0.262259718327668,6.76422083133051,
53.1849661722708));
#196744=CARTESIAN_POINT('Ctrl Pts',(0.0857105364293527,6.76645717520957,
53.1932809387167));
#196745=CARTESIAN_POINT('Ctrl Pts',(-0.090694798828944,6.76869169698699,
53.2015889305563));
#196746=CARTESIAN_POINT('Ctrl Pts',(-0.267318902673587,6.76402506751749,
53.2098969223959));
#196747=CARTESIAN_POINT('Ctrl Pts',(-0.443589768131856,6.75244526950117,
53.2182049142354));
#196748=CARTESIAN_POINT('Ctrl Pts',(-0.619749330088323,6.74087278336857,
53.2265076601225));
#196749=CARTESIAN_POINT('Ctrl Pts',(-0.795555751944949,6.72239585078345,
53.2348104060096));
#196750=CARTESIAN_POINT('Ctrl Pts',(-0.970437845322777,6.69705453078929,
53.2431131518967));
#196751=CARTESIAN_POINT('Ctrl Pts',(-1.1452484699622,6.67172356698502,53.2514125047161));
#196752=CARTESIAN_POINT('Ctrl Pts',(-1.31913517501728,6.6395338552691,53.2597118575355));
#196753=CARTESIAN_POINT('Ctrl Pts',(-1.49153241476046,6.60057725170449,
53.268011210355));
#196754=CARTESIAN_POINT('Ctrl Pts',(-1.66389298850354,6.56162893355578,
53.2763087980413));
#196755=CARTESIAN_POINT('Ctrl Pts',(-1.83476438888806,6.51591666741649,
53.2846063857276));
#196756=CARTESIAN_POINT('Ctrl Pts',(-2.00359153500685,6.46358336844578,
53.292903973414));
#196757=CARTESIAN_POINT('Ctrl Pts',(-2.17241082931851,6.41125250339035,
53.3012011751964));
#196758=CARTESIAN_POINT('Ctrl Pts',(-2.33918572658764,6.35230132228487,
53.3094983769789));
#196759=CARTESIAN_POINT('Ctrl Pts',(-2.50337638989166,6.28692258983145,
53.3177955787613));
#196760=CARTESIAN_POINT('Ctrl Pts',(-2.66758670022945,6.22153603416727,
53.3260937733858));
#196761=CARTESIAN_POINT('Ctrl Pts',(-2.82921183744743,6.14972052384547,
53.3343919680103));
#196762=CARTESIAN_POINT('Ctrl Pts',(-2.98773184815719,6.07171700621062,
53.3426901626349));
#196763=CARTESIAN_POINT('Ctrl Pts',(-3.14636334783892,5.99365862779225,
53.3509941934764));
#196764=CARTESIAN_POINT('Ctrl Pts',(-3.3018850446668,5.90940369950656,53.359298224318));
#196765=CARTESIAN_POINT('Ctrl Pts',(-3.45380070948755,5.81923961176572,
53.3676022551596));
#196766=CARTESIAN_POINT('Ctrl Pts',(-3.60577161502542,5.72904273788087,
53.3759093055753));
#196767=CARTESIAN_POINT('Ctrl Pts',(-3.75413357969917,5.63293260574036,
53.3842163559911));
#196768=CARTESIAN_POINT('Ctrl Pts',(-3.89841911554349,5.53124013215528,
53.3925234064068));
#196769=CARTESIAN_POINT('Ctrl Pts',(-4.04285891697658,5.42943893215338,
53.4008393384614));
#196770=CARTESIAN_POINT('Ctrl Pts',(-4.18321330120341,5.32204367222528,
53.409155270516));
#196771=CARTESIAN_POINT('Ctrl Pts',(-4.31904677820479,5.20942644901326,
53.4174712025706));
#196772=CARTESIAN_POINT('Ctrl Pts',(-4.42144093836636,5.12453319408754,
53.4237399287896));
#196773=CARTESIAN_POINT('Ctrl Pts',(-4.52126677450329,5.0366734265332,53.4300086550086));
#196774=CARTESIAN_POINT('Ctrl Pts',(-4.61835163230513,4.94602033966547,
53.4362773812276));
#196775=CARTESIAN_POINT('Ctrl Pts',(-4.74922241988468,4.82381960575584,
53.444727649951));
#196776=CARTESIAN_POINT('Ctrl Pts',(-4.87535123190647,4.69631775205162,
53.4531779186743));
#196777=CARTESIAN_POINT('Ctrl Pts',(-4.99630125840441,4.56390871241598,
53.4616281873977));
#196778=CARTESIAN_POINT('Ctrl Pts',(-5.11714454240011,4.43161652825049,
53.4700709984723));
#196779=CARTESIAN_POINT('Ctrl Pts',(-5.23281792802177,4.29442603381313,
53.4785138095468));
#196780=CARTESIAN_POINT('Ctrl Pts',(-5.34292068400844,4.15276866251839,
53.4869566206213));
#196781=CARTESIAN_POINT('Ctrl Pts',(-5.45294126135242,4.01121702164244,
53.4953931301392));
#196782=CARTESIAN_POINT('Ctrl Pts',(-5.55739929461045,3.86520541098306,
53.5038296396571));
#196783=CARTESIAN_POINT('Ctrl Pts',(-5.65593341103666,3.71519935534006,
53.5122661491749));
#196784=CARTESIAN_POINT('Ctrl Pts',(-5.7543970209993,3.56530063710344,53.5206966219162));
#196785=CARTESIAN_POINT('Ctrl Pts',(-5.84694498765805,3.41141345157195,
53.5291270946574));
#196786=CARTESIAN_POINT('Ctrl Pts',(-5.93325834557572,3.25403355923938,
53.5375575673987));
#196787=CARTESIAN_POINT('Ctrl Pts',(-6.01953459761426,3.09672132409688,
53.5459844159025));
#196788=CARTESIAN_POINT('Ctrl Pts',(-6.09958142491096,2.93591966565151,
53.5544112644063));
#196789=CARTESIAN_POINT('Ctrl Pts',(-6.17312471149832,2.77215084298976,
53.5628381129101));
#196790=CARTESIAN_POINT('Ctrl Pts',(-6.24664529789971,2.60843256991455,
53.5712623603468));
#196791=CARTESIAN_POINT('Ctrl Pts',(-6.31366621116775,2.44174926118961,
53.5796866077834));
#196792=CARTESIAN_POINT('Ctrl Pts',(-6.37396042614228,2.27264548180577,
53.5881108552201));
#196793=CARTESIAN_POINT('Ctrl Pts',(-6.39094902902823,2.22499850679036,
53.5904844858308));
#196794=CARTESIAN_POINT('Ctrl Pts',(-6.40740389402233,2.17715949500775,
53.5928581164416));
#196795=CARTESIAN_POINT('Ctrl Pts',(-6.42332063750646,2.12914090369416,
53.5952317470523));
#196796=CARTESIAN_POINT('Ctrl Pts',(-6.48028965164174,1.95727334736727,
53.6037274167821));
#196797=CARTESIAN_POINT('Ctrl Pts',(-6.53034517602241,1.78315182404982,
53.6122230865119));
#196798=CARTESIAN_POINT('Ctrl Pts',(-6.57333051505658,1.60736272814384,
53.6207187562417));
#196799=CARTESIAN_POINT('Ctrl Pts',(-6.61586491693437,1.43341774552887,
53.6291253022555));
#196800=CARTESIAN_POINT('Ctrl Pts',(-6.65147672476766,1.25784034745439,
53.6375318482693));
#196801=CARTESIAN_POINT('Ctrl Pts',(-6.68006557790762,1.08120898759385,
53.6459383942831));
#196802=CARTESIAN_POINT('Ctrl Pts',(-6.70910906690362,0.901768737530553,
53.6544786258709));
#196803=CARTESIAN_POINT('Ctrl Pts',(-6.73090428977837,0.721241075837371,
53.6630188574587));
#196804=CARTESIAN_POINT('Ctrl Pts',(-6.74540079315193,0.540238039891024,
53.6715590890465));
#196805=CARTESIAN_POINT('Ctrl Pts',(-6.7598972965255,0.359235003944613,
53.6800993206344));
#196806=CARTESIAN_POINT('Ctrl Pts',(-6.76709509095542,0.177756954509467,
53.6886395522222));
#196807=CARTESIAN_POINT('Ctrl Pts',(-6.76699905097193,-0.00358387290036924,
53.69717978381));
#196808=CARTESIAN_POINT('',(-6.76699985266004,-0.00141212569560718,53.3028202162272));
#196809=CARTESIAN_POINT('Ctrl Pts',(3.09910619832128,6.01563211736943,52.6513490741792));
#196810=CARTESIAN_POINT('Ctrl Pts',(2.93977317202945,6.09771658658964,52.6597717058748));
#196811=CARTESIAN_POINT('Ctrl Pts',(2.77717512720734,6.17346787802227,52.6681943375703));
#196812=CARTESIAN_POINT('Ctrl Pts',(2.61184631544113,6.24263949179484,52.6766169692659));
#196813=CARTESIAN_POINT('Ctrl Pts',(2.44649577225569,6.31182019773545,52.6850407080628));
#196814=CARTESIAN_POINT('Ctrl Pts',(2.27841405421461,6.37441937296258,52.6934644468596));
#196815=CARTESIAN_POINT('Ctrl Pts',(2.10815503505992,6.43023882512551,52.7018881856565));
#196816=CARTESIAN_POINT('Ctrl Pts',(1.93784986185947,6.48607340890122,52.7103142079719));
#196817=CARTESIAN_POINT('Ctrl Pts',(1.76536652769217,6.53512450156946,52.7187402302873));
#196818=CARTESIAN_POINT('Ctrl Pts',(1.59127404266256,6.57724379365311,52.7271662526027));
#196819=CARTESIAN_POINT('Ctrl Pts',(1.41702699399713,6.61940048029128,52.7355997557501));
#196820=CARTESIAN_POINT('Ctrl Pts',(1.2411682639919,6.65461298874775,52.7440332588976));
#196821=CARTESIAN_POINT('Ctrl Pts',(1.06427821797474,6.68278391650849,52.752466762045));
#196822=CARTESIAN_POINT('Ctrl Pts',(0.887309538935354,6.71096736710609,
52.7609040141419));
#196823=CARTESIAN_POINT('Ctrl Pts',(0.709308960135584,6.73210294950367,
52.7693412662388));
#196824=CARTESIAN_POINT('Ctrl Pts',(0.530862494699656,6.74614512234367,
52.7777785183357));
#196825=CARTESIAN_POINT('Ctrl Pts',(0.352204183006753,6.76020396562737,
52.7862257868836));
#196826=CARTESIAN_POINT('Ctrl Pts',(0.173099260154818,6.76715254952147,
52.7946730554315));
#196827=CARTESIAN_POINT('Ctrl Pts',(-0.00586430683023251,6.7669974589847,
52.8031203239794));
#196828=CARTESIAN_POINT('Ctrl Pts',(-0.161304619336367,6.76686275379354,
52.8104572701804));
#196829=CARTESIAN_POINT('Ctrl Pts',(-0.316638166327703,6.76136991059821,
52.8177942163814));
#196830=CARTESIAN_POINT('Ctrl Pts',(-0.471482715514754,6.75055501784637,
52.8251311625824));
#196831=CARTESIAN_POINT('Ctrl Pts',(-0.645376125660536,6.7384096850539,
52.8333706944332));
#196832=CARTESIAN_POINT('Ctrl Pts',(-0.81904087294918,6.71952402580645,
52.841610226284));
#196833=CARTESIAN_POINT('Ctrl Pts',(-0.991916130636073,6.69390703474316,
52.8498497581348));
#196834=CARTESIAN_POINT('Ctrl Pts',(-1.16459950886949,6.66831847674954,
52.8580801446811));
#196835=CARTESIAN_POINT('Ctrl Pts',(-1.33649479335783,6.63601351527784,
52.8663105312274));
#196836=CARTESIAN_POINT('Ctrl Pts',(-1.5070432996742,6.59705309156347,52.8745409177737));
#196837=CARTESIAN_POINT('Ctrl Pts',(-1.6774329333536,6.55812896101511,52.8827636373914));
#196838=CARTESIAN_POINT('Ctrl Pts',(-1.84647794244342,6.51256179407665,
52.8909863570092));
#196839=CARTESIAN_POINT('Ctrl Pts',(-2.01362680286849,6.46046407766266,
52.8992090766269));
#196840=CARTESIAN_POINT('Ctrl Pts',(-2.18062755736146,6.40841252357864,
52.9074245103227));
#196841=CARTESIAN_POINT('Ctrl Pts',(-2.34573517334649,6.34984205863469,
52.9156399440185));
#196842=CARTESIAN_POINT('Ctrl Pts',(-2.50841045583513,6.28491575003651,
52.9238553777143));
#196843=CARTESIAN_POINT('Ctrl Pts',(-2.67100213586083,6.22002280851921,
52.9320665893151));
#196844=CARTESIAN_POINT('Ctrl Pts',(-2.83116364219281,6.14878066029734,
52.9402778009159));
#196845=CARTESIAN_POINT('Ctrl Pts',(-2.98837263154654,6.07140165159773,
52.9484890125168));
#196846=CARTESIAN_POINT('Ctrl Pts',(-3.14552890168,5.99404859154788,52.9566974705303));
#196847=CARTESIAN_POINT('Ctrl Pts',(-3.29973430824302,5.91056292766706,
52.9649059285438));
#196848=CARTESIAN_POINT('Ctrl Pts',(-3.45048804566559,5.82120444982985,
52.9731143865574));
#196849=CARTESIAN_POINT('Ctrl Pts',(-3.51765212751514,5.78139329673992,
52.9767714338406));
#196850=CARTESIAN_POINT('Ctrl Pts',(-3.58413139685294,5.74041706956382,
52.9804284811239));
#196851=CARTESIAN_POINT('Ctrl Pts',(-3.6498831663623,5.6983016655759,52.9840855284071));
#196852=CARTESIAN_POINT('Ctrl Pts',(-3.80916461890021,5.59627851438966,
52.992944602583));
#196853=CARTESIAN_POINT('Ctrl Pts',(-3.96400950308699,5.48767357401941,
53.0018036767588));
#196854=CARTESIAN_POINT('Ctrl Pts',(-4.11391003546707,5.37289802807417,
53.0106627509346));
#196855=CARTESIAN_POINT('Ctrl Pts',(-4.26409220079215,5.25790684196739,
53.0195384695287));
#196856=CARTESIAN_POINT('Ctrl Pts',(-4.40931124407007,5.13672203928987,
53.0284141881227));
#196857=CARTESIAN_POINT('Ctrl Pts',(-4.54909386346712,5.00979381026463,
53.0372899067167));
#196858=CARTESIAN_POINT('Ctrl Pts',(-4.68927538296318,4.88250336393839,
53.0461909541037));
#196859=CARTESIAN_POINT('Ctrl Pts',(-4.8239892397493,4.74943686773294,53.0550920014907));
#196860=CARTESIAN_POINT('Ctrl Pts',(-4.95279816669417,4.61108222871712,
53.0639930488777));
#196861=CARTESIAN_POINT('Ctrl Pts',(-5.08178221114188,4.47253949467199,
53.0729061973607));
#196862=CARTESIAN_POINT('Ctrl Pts',(-5.20484511780985,4.32869445088134,
53.0818193458437));
#196863=CARTESIAN_POINT('Ctrl Pts',(-5.32159028407468,4.18006768467234,
53.0907324943267));
#196864=CARTESIAN_POINT('Ctrl Pts',(-5.43859465653232,4.0311109264007,53.0996654324366));
#196865=CARTESIAN_POINT('Ctrl Pts',(-5.54925307100242,3.87735141500615,
53.1085983705465));
#196866=CARTESIAN_POINT('Ctrl Pts',(-5.65321095375947,3.71934065558587,
53.1175313086564));
#196867=CARTESIAN_POINT('Ctrl Pts',(-5.75216378487853,3.56893732322435,
53.1260341705149));
#196868=CARTESIAN_POINT('Ctrl Pts',(-5.84504599221339,3.41468261487707,
53.1345370323734));
#196869=CARTESIAN_POINT('Ctrl Pts',(-5.93159077007427,3.25707229523228,
53.1430398942319));
#196870=CARTESIAN_POINT('Ctrl Pts',(-6.01739283086702,3.10081456874688,
53.1514697855336));
#196871=CARTESIAN_POINT('Ctrl Pts',(-6.09712353024838,2.94096957357786,
53.1598996768353));
#196872=CARTESIAN_POINT('Ctrl Pts',(-6.17047859025867,2.77803581099298,
53.168329568137));
#196873=CARTESIAN_POINT('Ctrl Pts',(-6.24373763717159,2.61531530943206,
53.176748425708));
#196874=CARTESIAN_POINT('Ctrl Pts',(-6.31063753670765,2.44951439765333,
53.185167283279));
#196875=CARTESIAN_POINT('Ctrl Pts',(-6.37091904262016,2.28115750275595,
53.19358614085));
#196876=CARTESIAN_POINT('Ctrl Pts',(-6.43113017293803,2.11299715597746,
53.2019951698327));
#196877=CARTESIAN_POINT('Ctrl Pts',(-6.48473819541337,1.94228708465093,
53.2104041988154));
#196878=CARTESIAN_POINT('Ctrl Pts',(-6.53153112594885,1.76957343751577,
53.218813227798));
#196879=CARTESIAN_POINT('Ctrl Pts',(-6.57826208234867,1.597088538161,53.227211119579));
#196880=CARTESIAN_POINT('Ctrl Pts',(-6.61819586128774,1.42260567571939,
53.2356090113601));
#196881=CARTESIAN_POINT('Ctrl Pts',(-6.65116970784568,1.24668781875657,
53.2440069031411));
#196882=CARTESIAN_POINT('Ctrl Pts',(-6.68411777619893,1.07090749038074,
53.2523982296409));
#196883=CARTESIAN_POINT('Ctrl Pts',(-6.71011669236257,0.893694729319301,
53.2607895561408));
#196884=CARTESIAN_POINT('Ctrl Pts',(-6.72905411009238,0.715625449134423,
53.2691808826406));
#196885=CARTESIAN_POINT('Ctrl Pts',(-6.74797629764367,0.537699378914352,
53.2775654605224));
#196886=CARTESIAN_POINT('Ctrl Pts',(-6.7598482762806,0.358918494063914,
53.2859500384041));
#196887=CARTESIAN_POINT('Ctrl Pts',(-6.76460915079576,0.17986672001878,
53.2943346162858));
#196888=CARTESIAN_POINT('Ctrl Pts',(-6.76621522951548,0.119463690468786,
53.2971631495872));
#196889=CARTESIAN_POINT('Ctrl Pts',(-6.76701246558696,0.0590298895209724,
53.2999916828885));
#196890=CARTESIAN_POINT('Ctrl Pts',(-6.76699985266021,-0.00141212489864533,
53.3028202161899));
#196891=CARTESIAN_POINT('Ctrl Pts',(-6.76699985266004,-0.00141212569551268,
53.3028202162272));
#196892=CARTESIAN_POINT('Ctrl Pts',(-6.76696059829612,-0.189521637263152,
53.3116232652798));
#196893=CARTESIAN_POINT('Ctrl Pts',(-6.75907349606841,-0.37741475106076,
53.3204263143324));
#196894=CARTESIAN_POINT('Ctrl Pts',(-6.74341788589126,-0.564450366499948,
53.329229363385));
#196895=CARTESIAN_POINT('Ctrl Pts',(-6.72772898176318,-0.751883740603923,
53.3380511334123));
#196896=CARTESIAN_POINT('Ctrl Pts',(-6.7042385751046,-0.938455706213667,
53.3468729034397));
#196897=CARTESIAN_POINT('Ctrl Pts',(-6.67307728490789,-1.1235339557158,
53.3556946734671));
#196898=CARTESIAN_POINT('Ctrl Pts',(-6.64181218264434,-1.30922878288483,
53.3645458327198));
#196899=CARTESIAN_POINT('Ctrl Pts',(-6.60282509282124,-1.49341966888789,
53.3733969919725));
#196900=CARTESIAN_POINT('Ctrl Pts',(-6.5562977086742,-1.67548481199724,
53.3822481512252));
#196901=CARTESIAN_POINT('Ctrl Pts',(-6.50969360393261,-1.85785016854612,
53.391113905457));
#196902=CARTESIAN_POINT('Ctrl Pts',(-6.4555244405932,-2.03808252365794,
53.3999796596888));
#196903=CARTESIAN_POINT('Ctrl Pts',(-6.39402102355469,-2.21557761099464,
53.4088454139206));
#196904=CARTESIAN_POINT('Ctrl Pts',(-6.33234674120663,-2.39356580512929,
53.4177357984887));
#196905=CARTESIAN_POINT('Ctrl Pts',(-6.26329752910282,-2.56880126419075,
53.4266261830567));
#196906=CARTESIAN_POINT('Ctrl Pts',(-6.18715265651196,-2.74069899934616,
53.4355165676248));
#196907=CARTESIAN_POINT('Ctrl Pts',(-6.11454534236484,-2.90461066447783,
53.4439939203769));
#196908=CARTESIAN_POINT('Ctrl Pts',(-6.03548680304529,-3.06548754111755,
53.4524712731291));
#196909=CARTESIAN_POINT('Ctrl Pts',(-5.95025661522847,-3.22284582518771,
53.4609486258813));
#196910=CARTESIAN_POINT('Ctrl Pts',(-5.86912884330557,-3.37262992524929,
53.4690179351038));
#196911=CARTESIAN_POINT('Ctrl Pts',(-5.78219288923522,-3.51962324273108,
53.4770872443263));
#196912=CARTESIAN_POINT('Ctrl Pts',(-5.68966536748213,-3.66333140816859,
53.4851565535488));
#196913=CARTESIAN_POINT('Ctrl Pts',(-5.59725325269687,-3.80686033046512,
53.4932157981496));
#196914=CARTESIAN_POINT('Ctrl Pts',(-5.49926364647894,-3.94711194384287,
53.5012750427503));
#196915=CARTESIAN_POINT('Ctrl Pts',(-5.39596026446172,-4.08361381919865,
53.5093342873511));
#196916=CARTESIAN_POINT('Ctrl Pts',(-5.29276306008153,-4.21997539472793,
53.5173852484714));
#196917=CARTESIAN_POINT('Ctrl Pts',(-5.18426317190447,-4.35259460688288,
53.5254362095916));
#196918=CARTESIAN_POINT('Ctrl Pts',(-5.07076901702374,-4.48102561652933,
53.5334871707119));
#196919=CARTESIAN_POINT('Ctrl Pts',(-4.95736664527389,-4.60935276355679,
53.541531620991));
#196920=CARTESIAN_POINT('Ctrl Pts',(-4.83897829136152,-4.73349817116958,
53.5495760712701));
#196921=CARTESIAN_POINT('Ctrl Pts',(-4.71595420805213,-4.85304697149692,
53.5576205215492));
#196922=CARTESIAN_POINT('Ctrl Pts',(-4.59300268593878,-4.97252526039509,
53.5656602271075));
#196923=CARTESIAN_POINT('Ctrl Pts',(-4.46542114435501,-5.08741207969262,
53.5736999326657));
#196924=CARTESIAN_POINT('Ctrl Pts',(-4.33359837019655,-5.19732759847115,
53.5817396382239));
#196925=CARTESIAN_POINT('Ctrl Pts',(-4.19893027193389,-5.3096155849587,
53.5899528765284));
#196926=CARTESIAN_POINT('Ctrl Pts',(-4.05983603445047,-5.41671492673835,
53.5981661148328));
#196927=CARTESIAN_POINT('Ctrl Pts',(-3.91676819051835,-5.51826203996726,
53.6063793531373));
#196928=CARTESIAN_POINT('Ctrl Pts',(-3.77676822504537,-5.61763162543941,
53.6144164706855));
#196929=CARTESIAN_POINT('Ctrl Pts',(-3.63296366592209,-5.71168447253263,
53.6224535882337));
#196930=CARTESIAN_POINT('Ctrl Pts',(-3.48580980782958,-5.80012232488584,
53.6304907057818));
#196931=CARTESIAN_POINT('Ctrl Pts',(-3.33864038179446,-5.88856953340156,
53.6385286736059));
#196932=CARTESIAN_POINT('Ctrl Pts',(-3.18812127145481,-5.97140037180547,
53.6465666414301));
#196933=CARTESIAN_POINT('Ctrl Pts',(-3.03473413076102,-6.04836157612904,
53.6546046092542));
#196934=CARTESIAN_POINT('Ctrl Pts',(-2.88130037103585,-6.12534617131043,
53.6626450200619));
#196935=CARTESIAN_POINT('Ctrl Pts',(-2.72499717963609,-6.19645741400195,
53.6706854308697));
#196936=CARTESIAN_POINT('Ctrl Pts',(-2.56632788166806,-6.26148945569448,
53.6787258416774));
#196937=CARTESIAN_POINT('Ctrl Pts',(-2.40166177914262,-6.32897934177779,
53.6870701346652));
#196938=CARTESIAN_POINT('Ctrl Pts',(-2.23444763687034,-6.38992136092001,
53.6954144276531));
#196939=CARTESIAN_POINT('Ctrl Pts',(-2.0652661523553,-6.44414189166685,
53.7037587206409));
#196940=CARTESIAN_POINT('Ctrl Pts',(-1.9019580188266,-6.49648008754321,
53.7118133308564));
#196941=CARTESIAN_POINT('Ctrl Pts',(-1.7368172234552,-6.5425556299749,53.7198679410719));
#196942=CARTESIAN_POINT('Ctrl Pts',(-1.57037671033177,-6.58226450301472,
53.7279225512875));
#196943=CARTESIAN_POINT('Ctrl Pts',(-1.40381019938871,-6.62200343623237,
53.7359832589568));
#196944=CARTESIAN_POINT('Ctrl Pts',(-1.23594237548614,-6.65536603123967,
53.744043966626));
#196945=CARTESIAN_POINT('Ctrl Pts',(-1.06731223174368,-6.68230002319339,
53.7521046742953));
#196946=CARTESIAN_POINT('Ctrl Pts',(-0.898444329601532,-6.70927199046209,
53.7601767470794));
#196947=CARTESIAN_POINT('Ctrl Pts',(-0.728812330485791,-6.72979722612918,
53.7682488198635));
#196948=CARTESIAN_POINT('Ctrl Pts',(-0.558956742052996,-6.74387547041859,
53.7763208926477));
#196949=CARTESIAN_POINT('Ctrl Pts',(-0.54116565968643,-6.7453500595448,
53.7771663809422));
#196950=CARTESIAN_POINT('Ctrl Pts',(-0.523372120621158,-6.74675396590074,
53.7780118692366));
#196951=CARTESIAN_POINT('Ctrl Pts',(-0.505576742886304,-6.74808722209876,
53.7788573575311));
#196952=CARTESIAN_POINT('Ctrl Pts',(-0.33018993218177,-6.76122746311562,
53.7871902795778));
#196953=CARTESIAN_POINT('Ctrl Pts',(-0.154065296644953,-6.76754267212398,
53.7955232016245));
#196954=CARTESIAN_POINT('Ctrl Pts',(0.0222316097009473,-6.76696348117308,
53.8038561236712));
#196955=CARTESIAN_POINT('Ctrl Pts',(0.198320175856137,-6.76638497468543,
53.8121791982249));
#196956=CARTESIAN_POINT('Ctrl Pts',(0.374580262292695,-6.75892829984617,
53.8205022727785));
#196957=CARTESIAN_POINT('Ctrl Pts',(0.550441407086462,-6.74457583969257,
53.8288253473321));
#196958=CARTESIAN_POINT('Ctrl Pts',(0.72612700697635,-6.73023770618992,
53.8371401137781));
#196959=CARTESIAN_POINT('Ctrl Pts',(0.901414113975392,-6.70901752941434,
53.845454880224));
#196960=CARTESIAN_POINT('Ctrl Pts',(1.07573225068254,-6.68094971728133,
53.85376964667));
#196961=CARTESIAN_POINT('Ctrl Pts',(1.24990835853327,-6.65290477390618,
53.8620776385095));
#196962=CARTESIAN_POINT('Ctrl Pts',(1.42311672716742,-6.61802336733466,
53.8703856303491));
#196963=CARTESIAN_POINT('Ctrl Pts',(1.59479175988844,-6.57639173427131,
53.8786936221886));
#196964=CARTESIAN_POINT('Ctrl Pts',(1.76635839107584,-6.53478638885619,
53.8869963680757));
#196965=CARTESIAN_POINT('Ctrl Pts',(1.93639327866725,-6.48643939302725,
53.8952991139628));
#196966=CARTESIAN_POINT('Ctrl Pts',(2.10434056142242,-6.43148814828671,
53.9036018598499));
#196967=CARTESIAN_POINT('Ctrl Pts',(2.2722192094751,-6.37655936036876,53.9119012126693));
#196968=CARTESIAN_POINT('Ctrl Pts',(2.43801162247627,-6.3150318094134,53.9202005654887));
#196969=CARTESIAN_POINT('Ctrl Pts',(2.60117637936824,-6.24709295940254,
53.9284999183082));
#196970=CARTESIAN_POINT('Ctrl Pts',(2.76430643385417,-6.17916855884512,
53.9367975059945));
#196971=CARTESIAN_POINT('Ctrl Pts',(2.92480962461324,-6.10483570943703,
53.9450950936809));
#196972=CARTESIAN_POINT('Ctrl Pts',(3.08216359500454,-6.02433038383758,
53.9533926813672));
#196973=CARTESIAN_POINT('Ctrl Pts',(3.23951024718267,-5.94382880237712,
53.9616898831496));
#196974=CARTESIAN_POINT('Ctrl Pts',(3.39370766122959,-5.85715547537241,
53.9699870849321));
#196975=CARTESIAN_POINT('Ctrl Pts',(3.54425704592219,-5.76459287308574,
53.9782842867145));
#196976=CARTESIAN_POINT('Ctrl Pts',(3.69482444533538,-5.67201919476963,
53.986582481339));
#196977=CARTESIAN_POINT('Ctrl Pts',(3.8417426495365,-5.57355501967024,53.9948806759636));
#196978=CARTESIAN_POINT('Ctrl Pts',(3.98454071775745,-5.46952687794228,
54.0031788705881));
#196979=CARTESIAN_POINT('Ctrl Pts',(4.12743921752462,-5.3654255720094,54.0114829014297));
#196980=CARTESIAN_POINT('Ctrl Pts',(4.26621150951494,-5.25575268520299,
54.0197869322713));
#196981=CARTESIAN_POINT('Ctrl Pts',(4.4004179889734,-5.14087643523158,54.0280909631128));
#196982=CARTESIAN_POINT('Ctrl Pts',(4.5346732696016,-5.0259584130939,54.0363980135286));
#196983=CARTESIAN_POINT('Ctrl Pts',(4.66435916913934,-4.90583348844042,
54.0447050639443));
#196984=CARTESIAN_POINT('Ctrl Pts',(4.7890718614116,-4.78090783285305,54.0530121143601));
#196985=CARTESIAN_POINT('Ctrl Pts',(4.91391789259978,-4.65584861065604,
54.0613280464147));
#196986=CARTESIAN_POINT('Ctrl Pts',(5.03377985200776,-4.52597865372332,
54.0696439784693));
#196987=CARTESIAN_POINT('Ctrl Pts',(5.1482924982285,-4.39173921729013,54.077959910524));
#196988=CARTESIAN_POINT('Ctrl Pts',(5.23461456327614,-4.29054667876992,
54.0842286367428));
#196989=CARTESIAN_POINT('Ctrl Pts',(5.31789770134732,-4.18687192182626,
54.0904973629616));
#196990=CARTESIAN_POINT('Ctrl Pts',(5.39800151058386,-4.08091517820873,
54.0967660891804));
#196991=CARTESIAN_POINT('Ctrl Pts',(5.50598177486445,-3.93808505206145,
54.1052163579038));
#196992=CARTESIAN_POINT('Ctrl Pts',(5.60838135925249,-3.79084536638939,
54.1136666266271));
#196993=CARTESIAN_POINT('Ctrl Pts',(5.7048374661404,-3.63965911658232,54.1221168953505));
#196994=CARTESIAN_POINT('Ctrl Pts',(5.80120844724159,-3.48860629376989,
54.130559706425));
#196995=CARTESIAN_POINT('Ctrl Pts',(5.89164622820041,-3.33361412725735,
54.1390025174995));
#196996=CARTESIAN_POINT('Ctrl Pts',(5.975829985486,-3.17517637062358,54.147445328574));
#196997=CARTESIAN_POINT('Ctrl Pts',(6.05995090958461,-3.0168568689776,54.1558818380917));
#196998=CARTESIAN_POINT('Ctrl Pts',(6.13782696010525,-2.85509719565438,
54.1643183476095));
#196999=CARTESIAN_POINT('Ctrl Pts',(6.20918193447105,-2.69041794237223,
54.1727548571272));
#197000=CARTESIAN_POINT('Ctrl Pts',(6.28048585051319,-2.52585652595691,
54.1811853298684));
#197001=CARTESIAN_POINT('Ctrl Pts',(6.3452778663386,-2.35838000017359,54.1896158026096));
#197002=CARTESIAN_POINT('Ctrl Pts',(6.40332874287388,-2.1885314735423,54.1980462753508));
#197003=CARTESIAN_POINT('Ctrl Pts',(6.46135466349469,-2.0187559643322,54.2064731238546));
#197004=CARTESIAN_POINT('Ctrl Pts',(6.51264511504258,-1.84661080030151,
54.2148999723585));
#197005=CARTESIAN_POINT('Ctrl Pts',(6.55701958718149,-1.67265750628106,
54.2233268208623));
#197006=CARTESIAN_POINT('Ctrl Pts',(6.60138036250554,-1.49875790543027,
54.2317510682989));
#197007=CARTESIAN_POINT('Ctrl Pts',(6.63882933368537,-1.32305160850205,
54.2401753157356));
#197008=CARTESIAN_POINT('Ctrl Pts',(6.669236208392,-1.14611404173981,54.2485995631722));
#197009=CARTESIAN_POINT('Ctrl Pts',(6.67780370229957,-1.0962598051607,54.2509731937832));
#197010=CARTESIAN_POINT('Ctrl Pts',(6.68581243581901,-1.04630789009901,
54.2533468243942));
#197011=CARTESIAN_POINT('Ctrl Pts',(6.69326022616024,-0.996271320926859,
54.2557204550053));
#197012=CARTESIAN_POINT('Ctrl Pts',(6.72030355510934,-0.814585836023446,
54.2643392359425));
#197013=CARTESIAN_POINT('Ctrl Pts',(6.73993506892834,-0.631864935886169,
54.2729580168797));
#197014=CARTESIAN_POINT('Ctrl Pts',(6.75210607839452,-0.44872319541984,
54.2815767978169));
#197015=CARTESIAN_POINT('Ctrl Pts',(6.76428439891208,-0.265471442823568,
54.2902007560035));
#197016=CARTESIAN_POINT('Ctrl Pts',(6.76899325123443,-0.0817986488975172,
54.29882471419));
#197017=CARTESIAN_POINT('Ctrl Pts',(6.76623605695892,0.101679012136382,
54.3074486723765));
#197018=CARTESIAN_POINT('Ctrl Pts',(6.7633792546617,0.291785095043078,54.3163841847476));
#197019=CARTESIAN_POINT('Ctrl Pts',(6.75250691412112,0.481681322143884,
54.3253196971188));
#197020=CARTESIAN_POINT('Ctrl Pts',(6.7336816087822,0.670686954956127,54.3342552094899));
#197021=CARTESIAN_POINT('Ctrl Pts',(6.71547871530889,0.85344358694677,54.3428952913846));
#197022=CARTESIAN_POINT('Ctrl Pts',(6.68984041836846,1.03536727747079,54.3515353732793));
#197023=CARTESIAN_POINT('Ctrl Pts',(6.65687570557249,1.21585148787129,54.360175455174));
#197024=CARTESIAN_POINT('Ctrl Pts',(6.62222024824564,1.40559264807541,54.3692586827833));
#197025=CARTESIAN_POINT('Ctrl Pts',(6.57946718504263,1.59374240549075,54.3783419103926));
#197026=CARTESIAN_POINT('Ctrl Pts',(6.52880315705344,1.77961184994062,54.387425138002));
#197027=CARTESIAN_POINT('Ctrl Pts',(6.47813912906425,1.96548129439049,54.3965083656113));
#197028=CARTESIAN_POINT('Ctrl Pts',(6.4195642862191,2.14907006667625,54.4055915932206));
#197029=CARTESIAN_POINT('Ctrl Pts',(6.35332481091391,2.32971089344274,54.41467482083));
#197030=CARTESIAN_POINT('Ctrl Pts',(6.287367065096,2.5095834193241,54.4237194156898));
#197031=CARTESIAN_POINT('Ctrl Pts',(6.21374965904559,2.68669943209794,54.4327640105496));
#197032=CARTESIAN_POINT('Ctrl Pts',(6.13271659374217,2.86043286599063,54.4418086054094));
#197033=CARTESIAN_POINT('Ctrl Pts',(6.05175788903143,3.03400687211068,54.4508449004298));
#197034=CARTESIAN_POINT('Ctrl Pts',(5.96339721182486,3.20420428118829,54.4598811954501));
#197035=CARTESIAN_POINT('Ctrl Pts',(5.86792620564945,3.37042001018455,54.4689174904705));
#197036=CARTESIAN_POINT('Ctrl Pts',(5.77262414290605,3.53634160741416,54.4779377950582));
#197037=CARTESIAN_POINT('Ctrl Pts',(5.67023699474511,3.69829538829857,54.4869580996459));
#197038=CARTESIAN_POINT('Ctrl Pts',(5.56110163486589,3.85570196030398,54.4959784042336));
#197039=CARTESIAN_POINT('Ctrl Pts',(5.45210370977234,4.01291030930898,54.5049873494999));
#197040=CARTESIAN_POINT('Ctrl Pts',(5.33637466731163,4.16558268229743,54.5139962947663));
#197041=CARTESIAN_POINT('Ctrl Pts',(5.21429524190593,4.31316752865423,54.5230052400326));
#197042=CARTESIAN_POINT('Ctrl Pts',(5.09249303303122,4.46041724106853,54.5319937278914));
#197043=CARTESIAN_POINT('Ctrl Pts',(4.96436937687443,4.6026023040594,54.5409822157502));
#197044=CARTESIAN_POINT('Ctrl Pts',(4.83034559369141,4.73920356658226,54.549970703609));
#197045=CARTESIAN_POINT('Ctrl Pts',(4.71275816957089,4.85905237408636,54.5578568646242));
#197046=CARTESIAN_POINT('Ctrl Pts',(4.59062972628005,4.97460330359925,54.5657430256395));
#197047=CARTESIAN_POINT('Ctrl Pts',(4.46427107342755,5.0855258118466,54.5736291866548));
#197048=CARTESIAN_POINT('Ctrl Pts',(4.33414306896021,5.19975720259742,54.5817505964091));
#197049=CARTESIAN_POINT('Ctrl Pts',(4.19958588311641,5.30902755291757,54.5898720061635));
#197050=CARTESIAN_POINT('Ctrl Pts',(4.06102343394452,5.41298232668032,54.5979934159179));
#197051=CARTESIAN_POINT('Ctrl Pts',(3.92247874117177,5.51692377892294,54.6061137849358));
#197052=CARTESIAN_POINT('Ctrl Pts',(3.77993010237479,5.61555079450149,54.6142341539537));
#197053=CARTESIAN_POINT('Ctrl Pts',(3.63383292729056,5.7085503638436,54.6223545229715));
#197054=CARTESIAN_POINT('Ctrl Pts',(3.4877063293019,5.80156866262,54.6304765273725));
#197055=CARTESIAN_POINT('Ctrl Pts',(3.33803007852441,5.88895705803541,54.6385985317734));
#197056=CARTESIAN_POINT('Ctrl Pts',(3.18528699900472,5.97044686216798,54.6467205361743));
#197057=CARTESIAN_POINT('Ctrl Pts',(3.15666658312933,5.98571611096938,54.6482424063921));
#197058=CARTESIAN_POINT('Ctrl Pts',(3.12793856017337,6.00077839134618,54.6497642766099));
#197059=CARTESIAN_POINT('Ctrl Pts',(3.09910619832136,6.01563211736939,54.6512861468277));
#197060=CARTESIAN_POINT('Origin',(0.,0.,4.30282021618968));
#197061=CARTESIAN_POINT('',(3.09910619832134,6.0156321173694,57.0459010634246));
#197062=CARTESIAN_POINT('',(3.09910619832132,6.01563211736941,56.6514148629243));
#197063=CARTESIAN_POINT('',(3.09910619832133,6.0156321173694,4.30282021618968));
#197064=CARTESIAN_POINT('',(-6.76699969835165,0.00202052189306006,55.6971797838405));
#197065=CARTESIAN_POINT('Ctrl Pts',(-6.76699969835165,0.0020205218929699,
55.6971797838405));
#197066=CARTESIAN_POINT('Ctrl Pts',(-6.76705147928238,-0.171400782706949,
55.7053523960128));
#197067=CARTESIAN_POINT('Ctrl Pts',(-6.76043245233308,-0.3450005055368,
55.713525008185));
#197068=CARTESIAN_POINT('Ctrl Pts',(-6.7471277734586,-0.518223705192626,
55.7216976203573));
#197069=CARTESIAN_POINT('Ctrl Pts',(-6.73371132132619,-0.692902161420724,
55.7299388910441));
#197070=CARTESIAN_POINT('Ctrl Pts',(-6.71349632062296,-0.867197368685377,
55.7381801617309));
#197071=CARTESIAN_POINT('Ctrl Pts',(-6.68652127016635,-1.04053942914863,
55.7464214324177));
#197072=CARTESIAN_POINT('Ctrl Pts',(-6.65980533644719,-1.21221640174707,
55.7545835391684));
#197073=CARTESIAN_POINT('Ctrl Pts',(-6.6264587095387,-1.38295809180124,
55.762745645919));
#197074=CARTESIAN_POINT('Ctrl Pts',(-6.58657088360599,-1.55221551185195,
55.7709077526696));
#197075=CARTESIAN_POINT('Ctrl Pts',(-6.54610275210948,-1.72393536298964,
55.7791886053245));
#197076=CARTESIAN_POINT('Ctrl Pts',(-6.49890164906467,-1.89412704152559,
55.7874694579794));
#197077=CARTESIAN_POINT('Ctrl Pts',(-6.44511484732756,-2.06222782561915,
55.7957503106343));
#197078=CARTESIAN_POINT('Ctrl Pts',(-6.39132804559047,-2.23032860971264,
55.8040311632892));
#197079=CARTESIAN_POINT('Ctrl Pts',(-6.33095565914911,-2.39633812586347,
55.8123120159441));
#197080=CARTESIAN_POINT('Ctrl Pts',(-6.26419778537996,-2.55970996514075,
55.820592868599));
#197081=CARTESIAN_POINT('Ctrl Pts',(-6.19471563011998,-2.72974874649895,
55.8292116495363));
#197082=CARTESIAN_POINT('Ctrl Pts',(-6.11833139665957,-2.89689470834243,
55.8378304304735));
#197083=CARTESIAN_POINT('Ctrl Pts',(-6.03531691208284,-3.06059451262772,
55.8464492114108));
#197084=CARTESIAN_POINT('Ctrl Pts',(-5.95225256121027,-3.22439265038952,
55.8550731695973));
#197085=CARTESIAN_POINT('Ctrl Pts',(-5.86255014843089,-3.3847402280458,
55.8636971277838));
#197086=CARTESIAN_POINT('Ctrl Pts',(-5.76652712834069,-3.54110913106486,
55.8723210859703));
#197087=CARTESIAN_POINT('Ctrl Pts',(-5.66703512416222,-3.70312710902409,
55.8812565983414));
#197088=CARTESIAN_POINT('Ctrl Pts',(-5.56075750837659,-3.86087327613705,
55.8901921107126));
#197089=CARTESIAN_POINT('Ctrl Pts',(-5.44809555685882,-4.01379419045561,
55.8991276230837));
#197090=CARTESIAN_POINT('Ctrl Pts',(-5.33915849235693,-4.16165915535622,
55.9077677049784));
#197091=CARTESIAN_POINT('Ctrl Pts',(-5.2242527262714,-4.30501262187923,
55.9164077868731));
#197092=CARTESIAN_POINT('Ctrl Pts',(-5.10378157334828,-4.44338864511654,
55.9250478687678));
#197093=CARTESIAN_POINT('Ctrl Pts',(-4.97713151196047,-4.58886190915005,
55.9341310963771));
#197094=CARTESIAN_POINT('Ctrl Pts',(-4.84433044693398,-4.72883345181669,
55.9432143239864));
#197095=CARTESIAN_POINT('Ctrl Pts',(-4.70589051354589,-4.86280613170202,
55.9522975515957));
#197096=CARTESIAN_POINT('Ctrl Pts',(-4.56745058015781,-4.99677881158735,
55.9613807792051));
#197097=CARTESIAN_POINT('Ctrl Pts',(-4.42337209068111,-5.12475239633751,
55.9704640068144));
#197098=CARTESIAN_POINT('Ctrl Pts',(-4.27420733716871,-5.24627874201258,
55.9795472344237));
#197099=CARTESIAN_POINT('Ctrl Pts',(-4.12567701062539,-5.36728821229094,
55.9885918292835));
#197100=CARTESIAN_POINT('Ctrl Pts',(-3.97196698339277,-5.48201759816239,
55.9976364241433));
#197101=CARTESIAN_POINT('Ctrl Pts',(-3.81360663819394,-5.59005307748711,
56.0066810190031));
#197102=CARTESIAN_POINT('Ctrl Pts',(-3.65539161353856,-5.69798941725421,
56.0157173140235));
#197103=CARTESIAN_POINT('Ctrl Pts',(-3.49253498714845,-5.79924398047969,
56.0247536090438));
#197104=CARTESIAN_POINT('Ctrl Pts',(-3.32559640039692,-5.89344530658146,
56.0337899040641));
#197105=CARTESIAN_POINT('Ctrl Pts',(-3.15895322456582,-5.98747993604951,
56.0428102086518));
#197106=CARTESIAN_POINT('Ctrl Pts',(-2.98824271939455,-6.07448613511232,
56.0518305132395));
#197107=CARTESIAN_POINT('Ctrl Pts',(-2.81405030747951,-6.15413762171228,
56.0608508178272));
#197108=CARTESIAN_POINT('Ctrl Pts',(-2.64007725707004,-6.23368880273733,
56.0698597630935));
#197109=CARTESIAN_POINT('Ctrl Pts',(-2.46263126614196,-6.30590365609888,
56.0788687083598));
#197110=CARTESIAN_POINT('Ctrl Pts',(-2.28232126275601,-6.37050222930436,
56.087877653626));
#197111=CARTESIAN_POINT('Ctrl Pts',(-2.10242070521609,-6.43495411282561,
56.0968661414848));
#197112=CARTESIAN_POINT('Ctrl Pts',(-1.91966934043858,-6.4918241583365,
56.1058546293436));
#197113=CARTESIAN_POINT('Ctrl Pts',(-1.73469445945225,-6.54088099053527,
56.1148431172023));
#197114=CARTESIAN_POINT('Ctrl Pts',(-1.57240445937941,-6.58392160912446,
56.1227292782177));
#197115=CARTESIAN_POINT('Ctrl Pts',(-1.40840329791828,-6.62094853192503,
56.1306154392331));
#197116=CARTESIAN_POINT('Ctrl Pts',(-1.2431269650968,-6.65183616369565,
56.1385016002484));
#197117=CARTESIAN_POINT('Ctrl Pts',(-1.07291918897449,-6.68364540718268,
56.1466230651046));
#197118=CARTESIAN_POINT('Ctrl Pts',(-0.901434902148291,-6.70892768419305,
56.1547445299608));
#197119=CARTESIAN_POINT('Ctrl Pts',(-0.729219616686332,-6.72759449956965,
56.1628659948169));
#197120=CARTESIAN_POINT('Ctrl Pts',(-0.557016612709089,-6.74625998372756,
56.1709868804931));
#197121=CARTESIAN_POINT('Ctrl Pts',(-0.384083077987967,-6.75831090650958,
56.1791077661693));
#197122=CARTESIAN_POINT('Ctrl Pts',(-0.210970502884236,-6.76371055315888,
56.1872286518455));
#197123=CARTESIAN_POINT('Ctrl Pts',(-0.0378372358778278,-6.76911084522035,
56.1953505081997));
#197124=CARTESIAN_POINT('Ctrl Pts',(0.135474748084897,-6.76785826787115,
56.203472364554));
#197125=CARTESIAN_POINT('Ctrl Pts',(0.308413143192804,-6.75996821982958,
56.2115942209082));
#197126=CARTESIAN_POINT('Ctrl Pts',(0.481477712014817,-6.75207241530655,
56.2197220028684));
#197127=CARTESIAN_POINT('Ctrl Pts',(0.654167781411757,-6.73752948477339,
56.2278497848286));
#197128=CARTESIAN_POINT('Ctrl Pts',(0.825934711704664,-6.71640684086375,
56.2359775667887));
#197129=CARTESIAN_POINT('Ctrl Pts',(0.997771613460076,-6.69527559237414,
56.2441086597052));
#197130=CARTESIAN_POINT('Ctrl Pts',(1.16868426532264,-6.66755934643257,
56.2522397526216));
#197131=CARTESIAN_POINT('Ctrl Pts',(1.3381336713158,-6.63337676283286,56.260370845538));
#197132=CARTESIAN_POINT('Ctrl Pts',(1.50776802425461,-6.59915687037158,
56.2685108132026));
#197133=CARTESIAN_POINT('Ctrl Pts',(1.67593558595926,-6.55845662963263,
56.2766507808671));
#197134=CARTESIAN_POINT('Ctrl Pts',(1.8421112508722,-6.51144493483666,56.2847907485317));
#197135=CARTESIAN_POINT('Ctrl Pts',(1.92829713567188,-6.48706263725991,
56.2890124877122));
#197136=CARTESIAN_POINT('Ctrl Pts',(2.01394750765826,-6.46098342309908,
56.2932342268927));
#197137=CARTESIAN_POINT('Ctrl Pts',(2.0989912316564,-6.43323595163659,56.2974559660732));
#197138=CARTESIAN_POINT('Ctrl Pts',(2.26901283008087,-6.37776249364934,
56.3058961755308));
#197139=CARTESIAN_POINT('Ctrl Pts',(2.43695994872582,-6.31550365160833,
56.3143363849885));
#197140=CARTESIAN_POINT('Ctrl Pts',(2.60227310043975,-6.24663619164168,
56.3227765944461));
#197141=CARTESIAN_POINT('Ctrl Pts',(2.76746100294989,-6.17782090897877,
56.3312104091947));
#197142=CARTESIAN_POINT('Ctrl Pts',(2.93001860993022,-6.10240711730429,
56.3396442239432));
#197143=CARTESIAN_POINT('Ctrl Pts',(3.08940384182834,-6.02062064093863,
56.3480780386918));
#197144=CARTESIAN_POINT('Ctrl Pts',(3.24869281759735,-5.93888355716433,
56.3565067600803));
#197145=CARTESIAN_POINT('Ctrl Pts',(3.40481294187678,-5.85078161330139,
56.3649354814689));
#197146=CARTESIAN_POINT('Ctrl Pts',(3.55724393009326,-5.75658793225768,
56.3733642028574));
#197147=CARTESIAN_POINT('Ctrl Pts',(3.70960626898648,-5.66243667259123,
56.3817891282592));
#197148=CARTESIAN_POINT('Ctrl Pts',(3.85828250134583,-5.56219932097617,
56.390214053661));
#197149=CARTESIAN_POINT('Ctrl Pts',(4.00277834447115,-5.45619414290152,
56.3986389790627));
#197150=CARTESIAN_POINT('Ctrl Pts',(4.14723128191518,-5.35022044133364,
56.4070614028204));
#197151=CARTESIAN_POINT('Ctrl Pts',(4.28750603694678,-5.23848252577955,
56.4154838265782));
#197152=CARTESIAN_POINT('Ctrl Pts',(4.42313831937298,-5.12134127037971,
56.4239062503359));
#197153=CARTESIAN_POINT('Ctrl Pts',(4.55877273490465,-5.00419817268502,
56.4323288065541));
#197154=CARTESIAN_POINT('Ctrl Pts',(4.68976427528127,-4.88165177824237,
56.4407513627723));
#197155=CARTESIAN_POINT('Ctrl Pts',(4.81568218028241,-4.75410287420355,
56.4491739189905));
#197156=CARTESIAN_POINT('Ctrl Pts',(4.94160433881428,-4.62654966153854,
56.4575967597243));
#197157=CARTESIAN_POINT('Ctrl Pts',(5.06245228576555,-4.49399383960433,
56.466019600458));
#197158=CARTESIAN_POINT('Ctrl Pts',(5.17783244871321,-4.35687274694277,
56.4744424411918));
#197159=CARTESIAN_POINT('Ctrl Pts',(5.29323261757138,-4.21972787868374,
56.4828667423724));
#197160=CARTESIAN_POINT('Ctrl Pts',(5.40316289750295,-4.07801641674895,
56.4912910435531));
#197161=CARTESIAN_POINT('Ctrl Pts',(5.50727007468458,-3.9322087081542,56.4997153447337));
#197162=CARTESIAN_POINT('Ctrl Pts',(5.61140984210758,-3.78635535517118,
56.5081422831005));
#197163=CARTESIAN_POINT('Ctrl Pts',(5.70972267867272,-3.63640347031142,
56.5165692214673));
#197164=CARTESIAN_POINT('Ctrl Pts',(5.80189855636353,-3.48285258684126,
56.5249961598341));
#197165=CARTESIAN_POINT('Ctrl Pts',(5.89415731175491,-3.32916364182546,
56.5334306750778));
#197166=CARTESIAN_POINT('Ctrl Pts',(5.98026791079522,-3.1718695185201,56.5418651903215));
#197167=CARTESIAN_POINT('Ctrl Pts',(6.05996562668506,-3.01149557585522,
56.5502997055651));
#197168=CARTESIAN_POINT('Ctrl Pts',(6.13970183725431,-2.85104417120237,
56.5587382947519));
#197169=CARTESIAN_POINT('Ctrl Pts',(6.21301884605309,-2.68751028248184,
56.5671768839387));
#197170=CARTESIAN_POINT('Ctrl Pts',(6.27969979472655,-2.5214399632177,56.5756154731255));
#197171=CARTESIAN_POINT('Ctrl Pts',(6.3464552776145,-2.35518401490897,56.5840634947458));
#197172=CARTESIAN_POINT('Ctrl Pts',(6.40655976202181,-2.18638628346224,
56.5925115163661));
#197173=CARTESIAN_POINT('Ctrl Pts',(6.45984564847592,-2.01560988235987,
56.6009595379864));
#197174=CARTESIAN_POINT('Ctrl Pts',(6.49013249118527,-1.9185433166547,56.6057612578985));
#197175=CARTESIAN_POINT('Ctrl Pts',(6.51821743525438,-1.82083777252419,
56.6105629778105));
#197176=CARTESIAN_POINT('Ctrl Pts',(6.54407704261625,-1.72259822950766,
56.6153646977226));
#197177=CARTESIAN_POINT('Ctrl Pts',(6.58845094663599,-1.55402366486885,
56.6236042295735));
#197178=CARTESIAN_POINT('Ctrl Pts',(6.62636848229945,-1.38349984522596,
56.6318437614243));
#197179=CARTESIAN_POINT('Ctrl Pts',(6.6576579632165,-1.21156074747406,56.6400832932751));
#197180=CARTESIAN_POINT('Ctrl Pts',(6.68891271499639,-1.03981249010473,
56.6483136798214));
#197181=CARTESIAN_POINT('Ctrl Pts',(6.71355399724992,-0.866652429542697,
56.6565440663677));
#197182=CARTESIAN_POINT('Ctrl Pts',(6.73146000388173,-0.692629205376576,
56.664774452914));
#197183=CARTESIAN_POINT('Ctrl Pts',(6.74934933036471,-0.518768090682325,
56.6729971725319));
#197184=CARTESIAN_POINT('Ctrl Pts',(6.76051584013589,-0.344045765660869,
56.6812198921497));
#197185=CARTESIAN_POINT('Ctrl Pts',(6.76488884012532,-0.169020651838755,
56.6894426117675));
#197186=CARTESIAN_POINT('Ctrl Pts',(6.7692579653217,0.00584937712268896,
56.6976580454633));
#197187=CARTESIAN_POINT('Ctrl Pts',(6.76684556938897,0.181021305712984,
56.7058734791591));
#197188=CARTESIAN_POINT('Ctrl Pts',(6.75763281889859,0.35593213530774,56.7140889128549));
#197189=CARTESIAN_POINT('Ctrl Pts',(6.74842480304663,0.530753074317118,
56.7223001244557));
#197190=CARTESIAN_POINT('Ctrl Pts',(6.73242341162174,0.705312827026527,
56.7305113360565));
#197191=CARTESIAN_POINT('Ctrl Pts',(6.70966189177258,0.879048518623898,
56.7387225476572));
#197192=CARTESIAN_POINT('Ctrl Pts',(6.68690800488117,1.05272594885721,56.7469310056707));
#197193=CARTESIAN_POINT('Ctrl Pts',(6.65739855175781,1.2255795159683,56.7551394636843));
#197194=CARTESIAN_POINT('Ctrl Pts',(6.62121862778495,1.39705149621392,56.7633479216978));
#197195=CARTESIAN_POINT('Ctrl Pts',(6.60509968163741,1.47344600764146,56.7670049689811));
#197196=CARTESIAN_POINT('Ctrl Pts',(6.58765740095151,1.54956638132596,56.7706620162643));
#197197=CARTESIAN_POINT('Ctrl Pts',(6.56890259347102,1.62536387233434,56.7743190635476));
#197198=CARTESIAN_POINT('Ctrl Pts',(6.52346970246536,1.8089807476912,56.7831781377235));
#197199=CARTESIAN_POINT('Ctrl Pts',(6.47037849510245,1.99051117195333,56.7920372118994));
#197200=CARTESIAN_POINT('Ctrl Pts',(6.4098551901401,2.16934216790115,56.8008962860752));
#197201=CARTESIAN_POINT('Ctrl Pts',(6.34921817406361,2.3485091513137,56.8097720046692));
#197202=CARTESIAN_POINT('Ctrl Pts',(6.28112123841151,2.5249663253962,56.8186477232632));
#197203=CARTESIAN_POINT('Ctrl Pts',(6.20583861966574,2.6981208324805,56.8275234418573));
#197204=CARTESIAN_POINT('Ctrl Pts',(6.13034116559747,2.87176947360253,56.8364244892443));
#197205=CARTESIAN_POINT('Ctrl Pts',(6.04761709727592,3.04209634800314,56.8453255366313));
#197206=CARTESIAN_POINT('Ctrl Pts',(5.95798794656755,3.20853060271456,56.8542265840183));
#197207=CARTESIAN_POINT('Ctrl Pts',(5.86823694379943,3.37519112707807,56.8631397325013));
#197208=CARTESIAN_POINT('Ctrl Pts',(5.77156223505374,3.53794823540166,56.8720528809843));
#197209=CARTESIAN_POINT('Ctrl Pts',(5.66832936572089,3.69625908205935,56.8809660294673));
#197210=CARTESIAN_POINT('Ctrl Pts',(5.56486729118965,3.85492142208588,56.8898989675772));
#197211=CARTESIAN_POINT('Ctrl Pts',(5.45481807376652,4.00911753676417,56.8988319056871));
#197212=CARTESIAN_POINT('Ctrl Pts',(5.33859004174419,4.1583344461683,56.907764843797));
#197213=CARTESIAN_POINT('Ctrl Pts',(5.22795780762323,4.30036730836828,56.9162677056554));
#197214=CARTESIAN_POINT('Ctrl Pts',(5.11172782731296,4.43788898361679,56.9247705675139));
#197215=CARTESIAN_POINT('Ctrl Pts',(4.9902838460473,4.57048751621524,56.9332734293723));
#197216=CARTESIAN_POINT('Ctrl Pts',(4.87281800056972,4.69874252381987,56.9414977633143));
#197217=CARTESIAN_POINT('Ctrl Pts',(4.75024823342919,4.82263683442815,56.9497220972564));
#197218=CARTESIAN_POINT('Ctrl Pts',(4.62293103387865,4.94174034688203,56.9579464311984));
#197219=CARTESIAN_POINT('Ctrl Pts',(4.49578303534043,5.06068557408499,56.9661598352297));
#197220=CARTESIAN_POINT('Ctrl Pts',(4.36390043775118,5.17485244816821,56.974373239261));
#197221=CARTESIAN_POINT('Ctrl Pts',(4.22767853481257,5.28384549417231,56.9825866432922));
#197222=CARTESIAN_POINT('Ctrl Pts',(4.09156113004649,5.39275492972993,56.9907937466796));
#197223=CARTESIAN_POINT('Ctrl Pts',(3.95111132471011,5.49649821510977,56.9990008500669));
#197224=CARTESIAN_POINT('Ctrl Pts',(3.80676015048628,5.59471770124907,57.0072079534542));
#197225=CARTESIAN_POINT('Ctrl Pts',(3.66250955706071,5.6928687501597,57.0154093383081));
#197226=CARTESIAN_POINT('Ctrl Pts',(3.51436330622302,5.78550346700239,57.023610723162));
#197227=CARTESIAN_POINT('Ctrl Pts',(3.36278419189374,5.87230546538151,57.0318121080159));
#197228=CARTESIAN_POINT('Ctrl Pts',(3.27598619290921,5.92201046465206,57.0365084264855));
#197229=CARTESIAN_POINT('Ctrl Pts',(3.18806313841968,5.96980368254101,57.041204744955));
#197230=CARTESIAN_POINT('Ctrl Pts',(3.09910619832134,6.0156321173694,57.0459010634246));
#197231=CARTESIAN_POINT('Ctrl Pts',(3.09910619832139,6.01563211736937,55.0459882871872));
#197232=CARTESIAN_POINT('Ctrl Pts',(2.947404464696,6.09378513168305,55.054049088509));
#197233=CARTESIAN_POINT('Ctrl Pts',(2.79250277190683,6.16632044368588,55.0621098898309));
#197234=CARTESIAN_POINT('Ctrl Pts',(2.63486444203576,6.23295903821737,55.0701706911527));
#197235=CARTESIAN_POINT('Ctrl Pts',(2.47739390984294,6.29952669948375,55.0782229121771));
#197236=CARTESIAN_POINT('Ctrl Pts',(2.31719287792394,6.36020998984401,55.0862751332016));
#197237=CARTESIAN_POINT('Ctrl Pts',(2.15475029648333,6.41477514491389,55.094327354226));
#197238=CARTESIAN_POINT('Ctrl Pts',(1.99244502452738,6.46929417714297,55.1023727688681));
#197239=CARTESIAN_POINT('Ctrl Pts',(1.82790232583838,6.51770524871838,55.1104181835102));
#197240=CARTESIAN_POINT('Ctrl Pts',(1.66163211870152,6.55982223098306,55.1184635981523));
#197241=CARTESIAN_POINT('Ctrl Pts',(1.4954660560798,6.6019128329793,55.1265039734923));
#197242=CARTESIAN_POINT('Ctrl Pts',(1.32757499961367,6.6377171020729,55.1345443488323));
#197243=CARTESIAN_POINT('Ctrl Pts',(1.15848495344206,6.66709844029983,55.1425847241723));
#197244=CARTESIAN_POINT('Ctrl Pts',(0.982230612909521,6.69772465698377,
55.1509657677953));
#197245=CARTESIAN_POINT('Ctrl Pts',(0.804673857516982,6.72137163588897,
55.1593468114183));
#197246=CARTESIAN_POINT('Ctrl Pts',(0.626423866829409,6.73794346511356,
55.1677278550413));
#197247=CARTESIAN_POINT('Ctrl Pts',(0.455488382986473,6.75383526760814,
55.1757649816705));
#197248=CARTESIAN_POINT('Ctrl Pts',(0.283915829244434,6.7632209944559,55.1838021082997));
#197249=CARTESIAN_POINT('Ctrl Pts',(0.112249562627997,6.76606894996569,
55.1918392349289));
#197250=CARTESIAN_POINT('Ctrl Pts',(-0.0594298949380122,6.76891712431427,
55.1998769791362));
#197251=CARTESIAN_POINT('Ctrl Pts',(-0.231202706125807,6.76522652047594,
55.2079147233436));
#197252=CARTESIAN_POINT('Ctrl Pts',(-0.402525040730363,6.75501758632685,
55.2159524675509));
#197253=CARTESIAN_POINT('Ctrl Pts',(-0.573894483692988,6.74480584503574,
55.22399242189));
#197254=CARTESIAN_POINT('Ctrl Pts',(-0.744812830711291,6.72807222796632,
55.2320323762291));
#197255=CARTESIAN_POINT('Ctrl Pts',(-0.914741050811109,6.70488909751392,
55.2400723305681));
#197256=CARTESIAN_POINT('Ctrl Pts',(-1.08474967562401,6.68169499753008,
55.2481160891619));
#197257=CARTESIAN_POINT('Ctrl Pts',(-1.25376687149422,6.65204536028967,
55.2561598477556));
#197258=CARTESIAN_POINT('Ctrl Pts',(-1.42126362542262,6.61606368674385,
55.2642036063493));
#197259=CARTESIAN_POINT('Ctrl Pts',(-1.58896631887206,6.58003777324446,
55.2722572548529));
#197260=CARTESIAN_POINT('Ctrl Pts',(-1.75514447369032,6.53766436007929,
55.2803109033565));
#197261=CARTESIAN_POINT('Ctrl Pts',(-1.91928334731617,6.48911707651471,
55.28836455186));
#197262=CARTESIAN_POINT('Ctrl Pts',(-2.08354111776461,6.44053462688841,
55.2964240341627));
#197263=CARTESIAN_POINT('Ctrl Pts',(-2.24575631385013,6.38576952076682,
55.3044835164654));
#197264=CARTESIAN_POINT('Ctrl Pts',(-2.40543451991011,6.32504338091248,
55.3125429987681));
#197265=CARTESIAN_POINT('Ctrl Pts',(-2.56534597916378,6.26422853411179,
55.3206142541238));
#197266=CARTESIAN_POINT('Ctrl Pts',(-2.72271271096822,6.19743541973706,
55.3286855094795));
#197267=CARTESIAN_POINT('Ctrl Pts',(-2.87706458077591,6.12493170558209,
55.3367567648352));
#197268=CARTESIAN_POINT('Ctrl Pts',(-2.92151436012792,6.10405230774645,
55.339081100265));
#197269=CARTESIAN_POINT('Ctrl Pts',(-2.96571429885978,6.08269960050195,
55.3414054356949));
#197270=CARTESIAN_POINT('Ctrl Pts',(-3.0096536315685,6.06088063056736,55.3437297711247));
#197271=CARTESIAN_POINT('Ctrl Pts',(-3.16717953318606,5.98265793806318,
55.3520626931714));
#197272=CARTESIAN_POINT('Ctrl Pts',(-3.32185622138896,5.8981896526874,55.3603956152181));
#197273=CARTESIAN_POINT('Ctrl Pts',(-3.47316195721547,5.80770479784839,
55.3687285372648));
#197274=CARTESIAN_POINT('Ctrl Pts',(-3.62428888635416,5.71732687416505,
55.3770516118184));
#197275=CARTESIAN_POINT('Ctrl Pts',(-3.7720525027817,5.62094672200501,55.385374686372));
#197276=CARTESIAN_POINT('Ctrl Pts',(-3.91595326226002,5.51884037165374,
55.3936977609256));
#197277=CARTESIAN_POINT('Ctrl Pts',(-4.05971037974752,5.41683594404069,
55.4020125273716));
#197278=CARTESIAN_POINT('Ctrl Pts',(-4.19961204049332,5.30911690624783,
55.4103272938175));
#197279=CARTESIAN_POINT('Ctrl Pts',(-4.33518524188114,5.19600403373361,
55.4186420602635));
#197280=CARTESIAN_POINT('Ctrl Pts',(-4.47064798254955,5.08298332197937,
55.426950052103));
#197281=CARTESIAN_POINT('Ctrl Pts',(-4.60178902506593,4.96457775430237,
55.4352580439425));
#197282=CARTESIAN_POINT('Ctrl Pts',(-4.72816601867455,4.84115018356705,
55.4435660357821));
#197283=CARTESIAN_POINT('Ctrl Pts',(-4.85446321349336,4.71780054925428,
55.4518687816692));
#197284=CARTESIAN_POINT('Ctrl Pts',(-4.97600210613736,4.58943547386822,
55.4601715275563));
#197285=CARTESIAN_POINT('Ctrl Pts',(-5.09237483349377,4.45645683870037,
55.4684742734434));
#197286=CARTESIAN_POINT('Ctrl Pts',(-5.20870000302462,4.32353254766347,
55.4767736262628));
#197287=CARTESIAN_POINT('Ctrl Pts',(-5.31986298531551,4.18599871508608,
55.4850729790822));
#197288=CARTESIAN_POINT('Ctrl Pts',(-5.42549388793494,4.04429290135873,
55.4933723319017));
#197289=CARTESIAN_POINT('Ctrl Pts',(-5.53110232463386,3.90261722608016,
55.501669919588));
#197290=CARTESIAN_POINT('Ctrl Pts',(-5.63118081787038,3.75677161614816,
55.5099675072743));
#197291=CARTESIAN_POINT('Ctrl Pts',(-5.72540062926587,3.60722561456891,
55.5182650949607));
#197292=CARTESIAN_POINT('Ctrl Pts',(-5.81961605868946,3.45768656807019,
55.5265622967431));
#197293=CARTESIAN_POINT('Ctrl Pts',(-5.90797316393929,3.3044477672898,55.5348594985255));
#197294=CARTESIAN_POINT('Ctrl Pts',(-5.990187204686,3.14800671105004,55.5431567003079));
#197295=CARTESIAN_POINT('Ctrl Pts',(-6.07241108315444,2.99154693509328,
55.5514548949324));
#197296=CARTESIAN_POINT('Ctrl Pts',(-6.14849027108658,2.8318844483687,55.5597530895569));
#197297=CARTESIAN_POINT('Ctrl Pts',(-6.2181864667203,2.66954042207578,55.5680512841815));
#197298=CARTESIAN_POINT('Ctrl Pts',(-6.28793168050111,2.50708221733614,
55.576355315023));
#197299=CARTESIAN_POINT('Ctrl Pts',(-6.35128479419908,2.341939024593,55.5846593458646));
#197300=CARTESIAN_POINT('Ctrl Pts',(-6.40805573101609,2.174651868275,55.5929633767062));
#197301=CARTESIAN_POINT('Ctrl Pts',(-6.46484731130831,2.00730388174247,
55.6012704271219));
#197302=CARTESIAN_POINT('Ctrl Pts',(-6.51505183945978,1.83781070956437,
55.6095774775377));
#197303=CARTESIAN_POINT('Ctrl Pts',(-6.55852937811859,1.66672775112055,
55.6178845279534));
#197304=CARTESIAN_POINT('Ctrl Pts',(-6.60205340160396,1.49546187612038,
55.626200460008));
#197305=CARTESIAN_POINT('Ctrl Pts',(-6.63883598675889,1.32260315792511,
55.6345163920627));
#197306=CARTESIAN_POINT('Ctrl Pts',(-6.66878828373765,1.14871747034836,
55.6428323241173));
#197307=CARTESIAN_POINT('Ctrl Pts',(-6.69136696140792,1.01763874559964,
55.6491010503363));
#197308=CARTESIAN_POINT('Ctrl Pts',(-6.71006541001522,0.885976661707472,
55.6553697765552));
#197309=CARTESIAN_POINT('Ctrl Pts',(-6.72486509888574,0.753975067086791,
55.6616385027742));
#197310=CARTESIAN_POINT('Ctrl Pts',(-6.75028615237594,0.527239246691952,
55.672406136197));
#197311=CARTESIAN_POINT('Ctrl Pts',(-6.76424264559793,0.299157940462259,
55.6831737696197));
#197312=CARTESIAN_POINT('Ctrl Pts',(-6.76663034842965,0.0707299633175301,
55.6939414030424));
#197313=CARTESIAN_POINT('Ctrl Pts',(-6.76686971674843,0.0478299524261698,
55.6950208632983));
#197314=CARTESIAN_POINT('Ctrl Pts',(-6.76699285898682,0.0249264676522418,
55.6961003235541));
#197315=CARTESIAN_POINT('Ctrl Pts',(-6.76699969835146,0.00202052254068524,
55.69717978381));
#197316=CARTESIAN_POINT('',(-6.76699843275197,-0.00460555451873011,55.3028202161608));
#197317=CARTESIAN_POINT('Ctrl Pts',(3.09910619832136,6.01563211736939,54.6512861468277));
#197318=CARTESIAN_POINT('Ctrl Pts',(2.94511279802101,6.09496574217557,54.6594144427633));
#197319=CARTESIAN_POINT('Ctrl Pts',(2.78814145528455,6.16834620428235,54.6675427386989));
#197320=CARTESIAN_POINT('Ctrl Pts',(2.62870208357314,6.23556046845977,54.6756710346345));
#197321=CARTESIAN_POINT('Ctrl Pts',(2.46919265465219,6.30280426639501,54.6838029021204));
#197322=CARTESIAN_POINT('Ctrl Pts',(2.30721337762719,6.36387633741049,54.6919347696062));
#197323=CARTESIAN_POINT('Ctrl Pts',(2.1432911071522,6.41861295218853,54.7000666370921));
#197324=CARTESIAN_POINT('Ctrl Pts',(1.97919583167376,6.47340733647037,54.7082070870223));
#197325=CARTESIAN_POINT('Ctrl Pts',(1.81315381883384,6.52185281089454,54.7163475369525));
#197326=CARTESIAN_POINT('Ctrl Pts',(1.64570456140892,6.56383618751702,54.7244879868827));
#197327=CARTESIAN_POINT('Ctrl Pts',(1.59019589955145,6.57775348456813,54.7271865087483));
#197328=CARTESIAN_POINT('Ctrl Pts',(1.53453266244973,6.59096108701847,54.7298850306139));
#197329=CARTESIAN_POINT('Ctrl Pts',(1.47873466302612,6.6034561251185,54.7325835524796));
#197330=CARTESIAN_POINT('Ctrl Pts',(1.30421437899526,6.64253705312163,54.7410237619372));
#197331=CARTESIAN_POINT('Ctrl Pts',(1.1280145363046,6.67472421685401,54.7494639713948));
#197332=CARTESIAN_POINT('Ctrl Pts',(0.950706475874524,6.69988404352868,
54.7579041808524));
#197333=CARTESIAN_POINT('Ctrl Pts',(0.773532752568601,6.7250248079072,54.766337995601));
#197334=CARTESIAN_POINT('Ctrl Pts',(0.595252814277275,6.74314880207744,
54.7747718103495));
#197335=CARTESIAN_POINT('Ctrl Pts',(0.416448073417482,6.75417352472876,
54.783205625098));
#197336=CARTESIAN_POINT('Ctrl Pts',(0.237751316541259,6.76519158931573,
54.7916343464866));
#197337=CARTESIAN_POINT('Ctrl Pts',(0.058530720978724,6.76911890946073,
54.8000630678751));
#197338=CARTESIAN_POINT('Ctrl Pts',(-0.120626900306542,6.76592478164829,
54.8084917892637));
#197339=CARTESIAN_POINT('Ctrl Pts',(-0.299703835573495,6.76273209235381,
54.8169167146654));
#197340=CARTESIAN_POINT('Ctrl Pts',(-0.478717520236171,6.75242435590935,
54.8253416400671));
#197341=CARTESIAN_POINT('Ctrl Pts',(-0.657080458865021,6.73502295991467,
54.8337665654688));
#197342=CARTESIAN_POINT('Ctrl Pts',(-0.835390435531868,6.71762673098037,
54.8421889892265));
#197343=CARTESIAN_POINT('Ctrl Pts',(-1.01304971995069,6.6931410753592,54.8506114129842));
#197344=CARTESIAN_POINT('Ctrl Pts',(-1.18947485924251,6.66163932971682,
54.859033836742));
#197345=CARTESIAN_POINT('Ctrl Pts',(-1.36590277319424,6.63013708864261,
54.8674563929602));
#197346=CARTESIAN_POINT('Ctrl Pts',(-1.54109617385986,6.59161858913544,
54.8758789491784));
#197347=CARTESIAN_POINT('Ctrl Pts',(-1.71448006877979,6.5462086045097,54.8843015053966));
#197348=CARTESIAN_POINT('Ctrl Pts',(-1.88786982064052,6.50079708592609,
54.8927243461303));
#197349=CARTESIAN_POINT('Ctrl Pts',(-2.05944962214071,6.44849370240205,
54.9011471868641));
#197350=CARTESIAN_POINT('Ctrl Pts',(-2.22865780254383,6.38947364022738,
54.9095700275978));
#197351=CARTESIAN_POINT('Ctrl Pts',(-2.39789532216493,6.33044334449032,
54.9179943287784));
#197352=CARTESIAN_POINT('Ctrl Pts',(-2.56476008589129,6.26469415806114,
54.9264186299591));
#197353=CARTESIAN_POINT('Ctrl Pts',(-2.72870827975019,6.19245025204263,
54.9348429311397));
#197354=CARTESIAN_POINT('Ctrl Pts',(-2.89270779678703,6.12018373042369,
54.9432698695065));
#197355=CARTESIAN_POINT('Ctrl Pts',(-3.0537886185245,6.04141857013837,54.9516968078733));
#197356=CARTESIAN_POINT('Ctrl Pts',(-3.2114291698959,5.95642608337766,54.9601237462401));
#197357=CARTESIAN_POINT('Ctrl Pts',(-3.36921145993829,5.87135717768786,
54.9685582614837));
#197358=CARTESIAN_POINT('Ctrl Pts',(-3.52354700495028,5.78004991598772,
54.9769927767274));
#197359=CARTESIAN_POINT('Ctrl Pts',(-3.67394000319246,5.68282094148163,
54.985427291971));
#197360=CARTESIAN_POINT('Ctrl Pts',(-3.8244056425414,5.58554500454777,54.9938658811578));
#197361=CARTESIAN_POINT('Ctrl Pts',(-3.97092466174838,5.48234183817236,
55.0023044703446));
#197362=CARTESIAN_POINT('Ctrl Pts',(-4.11303185905277,5.37357031464342,
55.0107430595314));
#197363=CARTESIAN_POINT('Ctrl Pts',(-4.25529790005259,5.26467720916027,
55.0191910811517));
#197364=CARTESIAN_POINT('Ctrl Pts',(-4.39314200545948,5.15020351876856,
55.027639102772));
#197365=CARTESIAN_POINT('Ctrl Pts',(-4.52613262437603,5.03054792905892,
55.0360871243923));
#197366=CARTESIAN_POINT('Ctrl Pts',(-4.60172235788968,4.96253761214141,
55.0408888443045));
#197367=CARTESIAN_POINT('Ctrl Pts',(-4.67574478522353,4.89285391469649,
55.0456905642168));
#197368=CARTESIAN_POINT('Ctrl Pts',(-4.74812616704887,4.82157514737516,
55.0504922841291));
#197369=CARTESIAN_POINT('Ctrl Pts',(-4.87232930922572,4.69926404127934,
55.0587318159799));
#197370=CARTESIAN_POINT('Ctrl Pts',(-4.99197543961657,4.57198122209799,
55.0669713478307));
#197371=CARTESIAN_POINT('Ctrl Pts',(-5.10664436501536,4.44009823418997,
55.0752108796815));
#197372=CARTESIAN_POINT('Ctrl Pts',(-5.22118601592096,4.30836162718147,
55.0834412662278));
#197373=CARTESIAN_POINT('Ctrl Pts',(-5.33076123027508,4.17203528429697,
55.0916716527742));
#197374=CARTESIAN_POINT('Ctrl Pts',(-5.43498522373034,4.03152881892625,
55.0999020393205));
#197375=CARTESIAN_POINT('Ctrl Pts',(-5.53911212843965,3.89115324084999,
55.1081247589383));
#197376=CARTESIAN_POINT('Ctrl Pts',(-5.63789752891919,3.74660557932165,
55.116347478556));
#197377=CARTESIAN_POINT('Ctrl Pts',(-5.73099560100306,3.59832994891847,
55.1245701981738));
#197378=CARTESIAN_POINT('Ctrl Pts',(-5.82401118148764,3.45018570140663,
55.1327856318696));
#197379=CARTESIAN_POINT('Ctrl Pts',(-5.91134928901013,3.29832036897575,
55.1410010655654));
#197380=CARTESIAN_POINT('Ctrl Pts',(-5.99270635831043,3.14320847273383,
55.1492164992612));
#197381=CARTESIAN_POINT('Ctrl Pts',(-6.0740216163948,2.98817629196154,55.157427710862));
#197382=CARTESIAN_POINT('Ctrl Pts',(-6.14936179306817,2.82990118471906,
55.1656389224628));
#197383=CARTESIAN_POINT('Ctrl Pts',(-6.2184681714375,2.66888414900661,55.1738501340636));
#197384=CARTESIAN_POINT('Ctrl Pts',(-6.28755137534065,2.5079211095234,55.1820585920771));
#197385=CARTESIAN_POINT('Ctrl Pts',(-6.35040480512318,2.3442182999833,55.1902670500907));
#197386=CARTESIAN_POINT('Ctrl Pts',(-6.40681695851238,2.17829875364198,
55.1984755081042));
#197387=CARTESIAN_POINT('Ctrl Pts',(-6.43194980465131,2.10437797276225,
55.2021325553874));
#197388=CARTESIAN_POINT('Ctrl Pts',(-6.45580476048543,2.03001746222543,
55.2057896026706));
#197389=CARTESIAN_POINT('Ctrl Pts',(-6.47836623906171,1.95526465538182,
55.2094466499538));
#197390=CARTESIAN_POINT('Ctrl Pts',(-6.52931529549927,1.78645546311793,
55.2177051117296));
#197391=CARTESIAN_POINT('Ctrl Pts',(-6.57363637656756,1.61573891659319,
55.2259635735053));
#197392=CARTESIAN_POINT('Ctrl Pts',(-6.61120997214735,1.44367299073559,
55.2342220352811));
#197393=CARTESIAN_POINT('Ctrl Pts',(-6.64880347265179,1.27151591152317,
55.2424848720456));
#197394=CARTESIAN_POINT('Ctrl Pts',(-6.67964229747292,1.09800837206614,
55.2507477088102));
#197395=CARTESIAN_POINT('Ctrl Pts',(-6.70365853353092,0.923716009289684,
55.2590105455747));
#197396=CARTESIAN_POINT('Ctrl Pts',(-6.7277071374903,0.749188743841748,
55.2672845185841));
#197397=CARTESIAN_POINT('Ctrl Pts',(-6.74491474196548,0.573874889902926,
55.2755584915935));
#197398=CARTESIAN_POINT('Ctrl Pts',(-6.7552654380163,0.398343899090347,
55.2838324646029));
#197399=CARTESIAN_POINT('Ctrl Pts',(-6.76318329661703,0.264069879403348,
55.2901617151222));
#197400=CARTESIAN_POINT('Ctrl Pts',(-6.76708981864431,0.129668871660295,
55.2964909656416));
#197401=CARTESIAN_POINT('Ctrl Pts',(-6.76699843275197,-0.00460555451873829,
55.3028202161609));
#197402=CARTESIAN_POINT('Ctrl Pts',(-6.76699843275155,-0.00460555513501829,
55.3028202161899));
#197403=CARTESIAN_POINT('Ctrl Pts',(-6.7668369231588,-0.241913573155351,
55.31400612805));
#197404=CARTESIAN_POINT('Ctrl Pts',(-6.75418850557821,-0.478814946071242,
55.32519203991));
#197405=CARTESIAN_POINT('Ctrl Pts',(-6.72920402485982,-0.714214387848929,
55.33637795177));
#197406=CARTESIAN_POINT('Ctrl Pts',(-6.7053621412692,-0.938848477763353,
55.3470523064395));
#197407=CARTESIAN_POINT('Ctrl Pts',(-6.6702870947623,-1.1621154726341,55.357726661109));
#197408=CARTESIAN_POINT('Ctrl Pts',(-6.62415141723983,-1.38307881246136,
55.3684010157785));
#197409=CARTESIAN_POINT('Ctrl Pts',(-6.58861194451494,-1.55329243043991,
55.3766237396444));
#197410=CARTESIAN_POINT('Ctrl Pts',(-6.54646027510188,-1.72236182502713,
55.3848464635103));
#197411=CARTESIAN_POINT('Ctrl Pts',(-6.49778336986864,-1.88973550484151,
55.3930691873761));
#197412=CARTESIAN_POINT('Ctrl Pts',(-6.44915798749064,-2.05693202528564,
55.4012832077674));
#197413=CARTESIAN_POINT('Ctrl Pts',(-6.39402122217541,-2.22243606350356,
55.4094972281586));
#197414=CARTESIAN_POINT('Ctrl Pts',(-6.33251115686558,-2.38570564994363,
55.4177112485498));
#197415=CARTESIAN_POINT('Ctrl Pts',(-6.27105384839404,-2.54883520097445,
55.4259182238217));
#197416=CARTESIAN_POINT('Ctrl Pts',(-6.20323425237369,-2.70973378326702,
55.4341251990937));
#197417=CARTESIAN_POINT('Ctrl Pts',(-6.1292404527537,-2.86787385920784,
55.4423321743657));
#197418=CARTESIAN_POINT('Ctrl Pts',(-6.05529526558349,-3.0259100402745,
55.4505337578186));
#197419=CARTESIAN_POINT('Ctrl Pts',(-5.97518410601595,-3.1811910010899,
55.4587353412716));
#197420=CARTESIAN_POINT('Ctrl Pts',(-5.88914345903629,-3.33320841215939,
55.4669369247246));
#197421=CARTESIAN_POINT('Ctrl Pts',(-5.80314207298519,-3.48515645665709,
55.4751347657396));
#197422=CARTESIAN_POINT('Ctrl Pts',(-5.71121676619947,-3.63384360667496,
55.4833326067547));
#197423=CARTESIAN_POINT('Ctrl Pts',(-5.61365036159667,-3.77878533628806,
55.4915304477697));
#197424=CARTESIAN_POINT('Ctrl Pts',(-5.51609256692457,-3.92371427524588,
55.4997275653508));
#197425=CARTESIAN_POINT('Ctrl Pts',(-5.41289485905208,-4.06489815000376,
55.507924682932));
#197426=CARTESIAN_POINT('Ctrl Pts',(-5.3043840605631,-4.20188038121555,
55.5161218005132));
#197427=CARTESIAN_POINT('Ctrl Pts',(-5.19587446937759,-4.33886108834747,
55.5243188268922));
#197428=CARTESIAN_POINT('Ctrl Pts',(-5.08205212728753,-4.47163996310305,
55.5325158532713));
#197429=CARTESIAN_POINT('Ctrl Pts',(-4.96328484087391,-4.59979266797442,
55.5407128796504));
#197430=CARTESIAN_POINT('Ctrl Pts',(-4.84449728038244,-4.72796724905426,
55.5489113052965));
#197431=CARTESIAN_POINT('Ctrl Pts',(-4.72076333774359,-4.8515138237245,
55.5571097309427));
#197432=CARTESIAN_POINT('Ctrl Pts',(-4.59248847504029,-4.97004412521882,
55.5653081565888));
#197433=CARTESIAN_POINT('Ctrl Pts',(-4.46416839076231,-5.08861621297405,
55.5735094724795));
#197434=CARTESIAN_POINT('Ctrl Pts',(-4.33130446091504,-5.20216826146719,
55.5817107883702));
#197435=CARTESIAN_POINT('Ctrl Pts',(-4.19433610899009,-5.31035155190519,
55.5899121042608));
#197436=CARTESIAN_POINT('Ctrl Pts',(-4.05721177304013,-5.41865804500166,
55.5981227600774));
#197437=CARTESIAN_POINT('Ctrl Pts',(-3.91597395857713,-5.5215833424832,
55.606333415894));
#197438=CARTESIAN_POINT('Ctrl Pts',(-3.77109288751936,-5.6188208223524,
55.6145440717106));
#197439=CARTESIAN_POINT('Ctrl Pts',(-3.62612644155663,-5.7161156019126,
55.6227595658677));
#197440=CARTESIAN_POINT('Ctrl Pts',(-3.47751276448229,-5.80771569480692,
55.6309750600249));
#197441=CARTESIAN_POINT('Ctrl Pts',(-3.32574757645875,-5.89335999729176,
55.639190554182));
#197442=CARTESIAN_POINT('Ctrl Pts',(-3.17374692195308,-5.97913717848801,
55.6474187948295));
#197443=CARTESIAN_POINT('Ctrl Pts',(-3.01858530398695,-6.0589399390686,
55.655647035477));
#197444=CARTESIAN_POINT('Ctrl Pts',(-2.86078057254186,-6.13255440381633,
55.6638752761245));
#197445=CARTESIAN_POINT('Ctrl Pts',(-2.71736126535138,-6.19945819964448,
55.6713534332258));
#197446=CARTESIAN_POINT('Ctrl Pts',(-2.57175919926442,-6.2612510582797,
55.678831590327));
#197447=CARTESIAN_POINT('Ctrl Pts',(-2.42437372432431,-6.31780824691648,
55.6863097474282));
#197448=CARTESIAN_POINT('Ctrl Pts',(-2.26533735264849,-6.37883631007286,
55.6943790566507));
#197449=CARTESIAN_POINT('Ctrl Pts',(-2.10370356158937,-6.43396718238844,
55.7024483658733));
#197450=CARTESIAN_POINT('Ctrl Pts',(-1.93995839993024,-6.48296617348418,
55.7105176750958));
#197451=CARTESIAN_POINT('Ctrl Pts',(-1.77641747299214,-6.53190404952055,
55.7185769196965));
#197452=CARTESIAN_POINT('Ctrl Pts',(-1.61077076827496,-6.5747251564444,
55.7266361642973));
#197453=CARTESIAN_POINT('Ctrl Pts',(-1.44352584780147,-6.61124210165753,
55.7346954088981));
#197454=CARTESIAN_POINT('Ctrl Pts',(-1.27645282557682,-6.64772151389855,
55.7427463700183));
#197455=CARTESIAN_POINT('Ctrl Pts',(-1.10778521803332,-6.67790957996122,
55.7507973311386));
#197456=CARTESIAN_POINT('Ctrl Pts',(-0.938047253761767,-6.70166817663408,
55.7588482922589));
#197457=CARTESIAN_POINT('Ctrl Pts',(-0.768446557191717,-6.72540755964447,
55.766892742538));
#197458=CARTESIAN_POINT('Ctrl Pts',(-0.597777594383516,-6.74272777059752,
55.7749371928171));
#197459=CARTESIAN_POINT('Ctrl Pts',(-0.426576234246035,-6.75354142034951,
55.7829816430962));
#197460=CARTESIAN_POINT('Ctrl Pts',(-0.255475850885913,-6.76434869207096,
55.7910213486544));
#197461=CARTESIAN_POINT('Ctrl Pts',(-0.0838440667595212,-6.76865701875375,
55.7990610542127));
#197462=CARTESIAN_POINT('Ctrl Pts',(0.0877767609437413,-6.76643068687164,
55.8071007597709));
#197463=CARTESIAN_POINT('Ctrl Pts',(0.263101932459457,-6.76415630080612,
55.8153139980754));
#197464=CARTESIAN_POINT('Ctrl Pts',(0.43841527417324,-6.75506189990469,
55.8235272363798));
#197465=CARTESIAN_POINT('Ctrl Pts',(0.613136568790696,-6.73916556763607,
55.8317404746843));
#197466=CARTESIAN_POINT('Ctrl Pts',(0.784111223483176,-6.72361010871817,
55.8397775922324));
#197467=CARTESIAN_POINT('Ctrl Pts',(0.954518579036146,-6.70154152370596,
55.8478147097806));
#197468=CARTESIAN_POINT('Ctrl Pts',(1.12381880315425,-6.67302931940786,
55.8558518273288));
#197469=CARTESIAN_POINT('Ctrl Pts',(1.29313693815969,-6.64451409869983,
55.8638897951529));
#197470=CARTESIAN_POINT('Ctrl Pts',(1.46134734003895,-6.60955396329149,
55.871927762977));
#197471=CARTESIAN_POINT('Ctrl Pts',(1.62791941120203,-6.56826974100727,
55.8799657308011));
#197472=CARTESIAN_POINT('Ctrl Pts',(1.79454210869888,-6.52697297118849,
55.8880061416089));
#197473=CARTESIAN_POINT('Ctrl Pts',(1.95952512189877,-6.47934837844146,
55.8960465524166));
#197474=CARTESIAN_POINT('Ctrl Pts',(2.12235222507528,-6.4255669036061,55.9040869632243));
#197475=CARTESIAN_POINT('Ctrl Pts',(2.29133327439528,-6.36975279235335,
55.9124312562121));
#197476=CARTESIAN_POINT('Ctrl Pts',(2.45799184433616,-6.30730745515342,
55.9207755491999));
#197477=CARTESIAN_POINT('Ctrl Pts',(2.62177388937024,-6.2384766307983,55.9291198421877));
#197478=CARTESIAN_POINT('Ctrl Pts',(2.77987003184592,-6.17203535628801,
55.9371744524032));
#197479=CARTESIAN_POINT('Ctrl Pts',(2.93528572203134,-6.09964474121615,
55.9452290626188));
#197480=CARTESIAN_POINT('Ctrl Pts',(3.08754845635011,-6.02157234696139,
55.9532836728343));
#197481=CARTESIAN_POINT('Ctrl Pts',(3.23992645570963,-5.94344085080131,
55.9613443805036));
#197482=CARTESIAN_POINT('Ctrl Pts',(3.38914642329934,-5.85961919297991,
55.9694050881728));
#197483=CARTESIAN_POINT('Ctrl Pts',(3.53476491456139,-5.7704181823145,55.9774657958421));
#197484=CARTESIAN_POINT('Ctrl Pts',(3.68058871917186,-5.68109140356825,
55.9855378686262));
#197485=CARTESIAN_POINT('Ctrl Pts',(3.82280060830583,-5.5863703445995,55.9936099414104));
#197486=CARTESIAN_POINT('Ctrl Pts',(3.96098980629043,-5.48660630576528,
56.0016820141945));
#197487=CARTESIAN_POINT('Ctrl Pts',(3.97546407484964,-5.47615678068157,
56.0025275024889));
#197488=CARTESIAN_POINT('Ctrl Pts',(3.98989424395179,-5.46565196249461,
56.0033729907833));
#197489=CARTESIAN_POINT('Ctrl Pts',(4.00427986530766,-5.45509227788969,
56.0042184790777));
#197490=CARTESIAN_POINT('Ctrl Pts',(4.14606096641492,-5.35101865648716,
56.0125514011244));
#197491=CARTESIAN_POINT('Ctrl Pts',(4.28396418126854,-5.24128045693582,
56.0208843231711));
#197492=CARTESIAN_POINT('Ctrl Pts',(4.417514765497,-5.12619276818733,56.0292172452178));
#197493=CARTESIAN_POINT('Ctrl Pts',(4.55090752532126,-5.01124108517787,
56.0375403197714));
#197494=CARTESIAN_POINT('Ctrl Pts',(4.67995763994972,-4.89095273169111,
56.045863394325));
#197495=CARTESIAN_POINT('Ctrl Pts',(4.80422029083322,-4.76568530194204,
56.0541864688786));
#197496=CARTESIAN_POINT('Ctrl Pts',(4.92835890252025,-4.64054291436146,
56.0625012353246));
#197497=CARTESIAN_POINT('Ctrl Pts',(5.04771932795627,-4.51043159808899,
56.0708160017705));
#197498=CARTESIAN_POINT('Ctrl Pts',(5.16189056914938,-4.37574847907494,
56.0791307682165));
#197499=CARTESIAN_POINT('Ctrl Pts',(5.27596878725769,-4.24117509556933,
56.087438760056));
#197500=CARTESIAN_POINT('Ctrl Pts',(5.38486602170394,-4.10203759588203,
56.0957467518955));
#197501=CARTESIAN_POINT('Ctrl Pts',(5.48820868701037,-3.95876930469861,
56.1040547437351));
#197502=CARTESIAN_POINT('Ctrl Pts',(5.59148609819536,-3.81559147805318,
56.1123574896221));
#197503=CARTESIAN_POINT('Ctrl Pts',(5.68921572698593,-3.66828833938926,
56.1206602355092));
#197504=CARTESIAN_POINT('Ctrl Pts',(5.7810646566209,-3.51732575061917,56.1289629813963));
#197505=CARTESIAN_POINT('Ctrl Pts',(5.87287605052535,-3.36642485544827,
56.1372623342157));
#197506=CARTESIAN_POINT('Ctrl Pts',(5.95881135337727,-3.21186778683285,
56.1455616870352));
#197507=CARTESIAN_POINT('Ctrl Pts',(6.0385811743165,-3.05414904698352,56.1538610398546));
#197508=CARTESIAN_POINT('Ctrl Pts',(6.11833402955332,-2.89646385126372,
56.1621586275409));
#197509=CARTESIAN_POINT('Ctrl Pts',(6.19192385834307,-2.73561863422694,
56.1704562152273));
#197510=CARTESIAN_POINT('Ctrl Pts',(6.25910729815888,-2.5721323508199,56.1787538029136));
#197511=CARTESIAN_POINT('Ctrl Pts',(6.32628761340949,-2.40865367082751,
56.187051004696));
#197512=CARTESIAN_POINT('Ctrl Pts',(6.3870620013392,-2.24253449106635,56.1953482064784));
#197513=CARTESIAN_POINT('Ctrl Pts',(6.44123523920145,-2.07431376442173,
56.2036454082608));
#197514=CARTESIAN_POINT('Ctrl Pts',(6.49541495942661,-1.90607290850588,
56.2119436028854));
#197515=CARTESIAN_POINT('Ctrl Pts',(6.54299184956379,-1.73573033593956,
56.2202417975099));
#197516=CARTESIAN_POINT('Ctrl Pts',(6.58382049658707,-1.56384035909041,
56.2285399921345));
#197517=CARTESIAN_POINT('Ctrl Pts',(6.6246778588738,-1.39182949001658,56.236844022976));
#197518=CARTESIAN_POINT('Ctrl Pts',(6.65877741387089,-1.21826938090844,
56.2451480538176));
#197519=CARTESIAN_POINT('Ctrl Pts',(6.68602466338608,-1.04372563473027,
56.2534520846592));
#197520=CARTESIAN_POINT('Ctrl Pts',(6.71328182075112,-0.869118419642034,
56.2617591350749));
#197521=CARTESIAN_POINT('Ctrl Pts',(6.73368166003576,-0.693527199420231,
56.2700661854906));
#197522=CARTESIAN_POINT('Ctrl Pts',(6.74718154470948,-0.517523142218622,
56.2783732359064));
#197523=CARTESIAN_POINT('Ctrl Pts',(6.76069586303831,-0.341330906975363,
56.286689167961));
#197524=CARTESIAN_POINT('Ctrl Pts',(6.76729546774921,-0.164725300483295,
56.2950051000156));
#197525=CARTESIAN_POINT('Ctrl Pts',(6.76698984921282,0.0117209492236127,
56.3033210320702));
#197526=CARTESIAN_POINT('Ctrl Pts',(6.76675946746853,0.14472988009398,56.3095897582892));
#197527=CARTESIAN_POINT('Ctrl Pts',(6.76260629585194,0.277648229017697,
56.3158584845082));
#197528=CARTESIAN_POINT('Ctrl Pts',(6.75455388823963,0.410232581430221,
56.3221272107271));
#197529=CARTESIAN_POINT('Ctrl Pts',(6.74369920966265,0.588956833736392,
56.3305774794505));
#197530=CARTESIAN_POINT('Ctrl Pts',(6.72573748134582,0.767401716643068,
56.3390277481738));
#197531=CARTESIAN_POINT('Ctrl Pts',(6.7006941879843,0.944979576029759,56.3474780168972));
#197532=CARTESIAN_POINT('Ctrl Pts',(6.6756729961788,1.12240071693104,56.3559208279717));
#197533=CARTESIAN_POINT('Ctrl Pts',(6.64358274223863,1.29895603264581,56.3643636390462));
#197534=CARTESIAN_POINT('Ctrl Pts',(6.60450079961785,1.47406179919539,56.3728064501208));
#197535=CARTESIAN_POINT('Ctrl Pts',(6.56544802703039,1.64903687006553,56.3812429596385));
#197536=CARTESIAN_POINT('Ctrl Pts',(6.51941404047306,1.82256422594958,56.3896794691562));
#197537=CARTESIAN_POINT('Ctrl Pts',(6.46652756365981,1.99406877224131,56.398115978674));
#197538=CARTESIAN_POINT('Ctrl Pts',(6.4136789299665,2.16545059780162,56.4065464514152));
#197539=CARTESIAN_POINT('Ctrl Pts',(6.35398768396143,2.33481218480885,56.4149769241564));
#197540=CARTESIAN_POINT('Ctrl Pts',(6.28763286896952,2.50159187419814,56.4234073968976));
#197541=CARTESIAN_POINT('Ctrl Pts',(6.22130657973267,2.66829986545113,56.4318342454015));
#197542=CARTESIAN_POINT('Ctrl Pts',(6.14832255464118,2.83242786428337,56.4402610939053));
#197543=CARTESIAN_POINT('Ctrl Pts',(6.06890883103224,2.99343191013574,56.4486879424092));
#197544=CARTESIAN_POINT('Ctrl Pts',(5.98951961960386,3.15438625978872,56.4571121898458));
#197545=CARTESIAN_POINT('Ctrl Pts',(5.9037048139639,3.31221828238127,56.4655364372824));
#197546=CARTESIAN_POINT('Ctrl Pts',(5.81173964072859,3.46640611417415,56.4739606847191));
#197547=CARTESIAN_POINT('Ctrl Pts',(5.78582737355267,3.50985034585596,56.47633431533));
#197548=CARTESIAN_POINT('Ctrl Pts',(5.75942711228635,3.55300541318139,56.478707945941));
#197549=CARTESIAN_POINT('Ctrl Pts',(5.73254566861582,3.59586000245198,56.481081576552));
#197550=CARTESIAN_POINT('Ctrl Pts',(5.63493769490564,3.75146733047175,56.4897003574892));
#197551=CARTESIAN_POINT('Ctrl Pts',(5.53102585618159,3.90304125123259,56.4983191384264));
#197552=CARTESIAN_POINT('Ctrl Pts',(5.42117282916198,4.05008322832456,56.5069379193637));
#197553=CARTESIAN_POINT('Ctrl Pts',(5.3112538140971,4.19721353263796,56.5155618775502));
#197554=CARTESIAN_POINT('Ctrl Pts',(5.19538667047351,4.33980621669734,56.5241858357367));
#197555=CARTESIAN_POINT('Ctrl Pts',(5.07397470201981,4.47739541734511,56.5328097939232));
#197556=CARTESIAN_POINT('Ctrl Pts',(4.94817653339984,4.6199552463621,56.5417453062943));
#197557=CARTESIAN_POINT('Ctrl Pts',(4.81642568281949,4.75714306734963,56.5506808186655));
#197558=CARTESIAN_POINT('Ctrl Pts',(4.67921237661769,4.88848243675968,56.5596163310366));
#197559=CARTESIAN_POINT('Ctrl Pts',(4.5465356868671,5.01547939681854,56.5682564129313));
#197560=CARTESIAN_POINT('Ctrl Pts',(4.40875222440379,5.13700827781193,56.576896494826));
#197561=CARTESIAN_POINT('Ctrl Pts',(4.26633922204371,5.25267918708648,56.5855365767207));
#197562=CARTESIAN_POINT('Ctrl Pts',(4.11662192413715,5.37428280259902,56.59461980433));
#197563=CARTESIAN_POINT('Ctrl Pts',(3.96178803430437,5.48941152268209,56.6037030319393));
#197564=CARTESIAN_POINT('Ctrl Pts',(3.80242734332519,5.59766337847614,56.6127862595487));
#197565=CARTESIAN_POINT('Ctrl Pts',(3.64306665234607,5.70591523427016,56.621869487158));
#197566=CARTESIAN_POINT('Ctrl Pts',(3.47917950770841,5.80729005040436,56.6309527147673));
#197567=CARTESIAN_POINT('Ctrl Pts',(3.31138686120923,5.90144101515985,56.6400359423767));
#197568=CARTESIAN_POINT('Ctrl Pts',(3.24132002024662,5.94075656808565,56.6438289158925));
#197569=CARTESIAN_POINT('Ctrl Pts',(3.17054541902039,5.97882838214224,56.6476218894084));
#197570=CARTESIAN_POINT('Ctrl Pts',(3.09910619832132,6.01563211736941,56.6514148629243));
#197571=CARTESIAN_POINT('Origin',(0.,0.,4.30282021618968));
#197572=CARTESIAN_POINT('',(3.09910619832129,6.01563211736943,59.0457552630241));
#197573=CARTESIAN_POINT('',(3.0991061983213,6.01563211736942,58.6514477063419));
#197574=CARTESIAN_POINT('',(3.09910619832133,6.0156321173694,4.30282021618968));
#197575=CARTESIAN_POINT('',(-6.76799881069709,0.0013588597829734,57.6954514518074));
#197576=CARTESIAN_POINT('Ctrl Pts',(-6.767,1.1904414001692E-12,57.69717978381));
#197577=CARTESIAN_POINT('Ctrl Pts',(-6.76700000000003,-0.186007249525739,
57.7059292956212));
#197578=CARTESIAN_POINT('Ctrl Pts',(-6.75932637294526,-0.372014355748844,
57.7146788074324));
#197579=CARTESIAN_POINT('Ctrl Pts',(-6.74400518264189,-0.557389537486478,
57.7234283192436));
#197580=CARTESIAN_POINT('Ctrl Pts',(-6.72868405705096,-0.742763936250848,
57.7321777940992));
#197581=CARTESIAN_POINT('Ctrl Pts',(-6.70571545645737,-0.927506130241391,
57.7409272689549));
#197582=CARTESIAN_POINT('Ctrl Pts',(-6.67517739404815,-1.1109886399008,
57.7496767438106));
#197583=CARTESIAN_POINT('Ctrl Pts',(-6.64463945808684,-1.2944703898204,
57.7584261824376));
#197584=CARTESIAN_POINT('Ctrl Pts',(-6.60653217008328,-1.47669218313805,
57.7671756210646));
#197585=CARTESIAN_POINT('Ctrl Pts',(-6.56098496092639,-1.65703510599435,
57.7759250596917));
#197586=CARTESIAN_POINT('Ctrl Pts',(-6.51543793658254,-1.83737729708852,
57.7846744628168));
#197587=CARTESIAN_POINT('Ctrl Pts',(-6.46245112167372,-2.01584035511082,
57.793423865942));
#197588=CARTESIAN_POINT('Ctrl Pts',(-6.40220448374199,-2.1918181376095,
57.8021732690672));
#197589=CARTESIAN_POINT('Ctrl Pts',(-6.3419580852644,-2.36779522067315,
57.8109226374173));
#197590=CARTESIAN_POINT('Ctrl Pts',(-6.2744520143303,-2.54128677684349,
57.8196720057674));
#197591=CARTESIAN_POINT('Ctrl Pts',(-6.19991555071816,-2.71170355385007,
57.8284213741175));
#197592=CARTESIAN_POINT('Ctrl Pts',(-6.12537937716599,-2.88211966767675,
57.8371707084193));
#197593=CARTESIAN_POINT('Ctrl Pts',(-6.04381298052419,-3.04946076371986,
57.845920042721));
#197594=CARTESIAN_POINT('Ctrl Pts',(-5.95549339335722,-3.21315848374749,
57.8546693770228));
#197595=CARTESIAN_POINT('Ctrl Pts',(-5.867174142553,-3.37685558033682,57.863418678003));
#197596=CARTESIAN_POINT('Ctrl Pts',(-5.77210188876489,-3.53690907646934,
57.8721679789832));
#197597=CARTESIAN_POINT('Ctrl Pts',(-5.67059953346888,-3.69277536969452,
57.8809172799634));
#197598=CARTESIAN_POINT('Ctrl Pts',(-5.56909755631268,-3.84864108225091,
57.8896665483486));
#197599=CARTESIAN_POINT('Ctrl Pts',(-5.46116568196727,-4.00031938297686,
57.8984158167339));
#197600=CARTESIAN_POINT('Ctrl Pts',(-5.34717048533471,-4.14729511860024,
57.9071650851192));
#197601=CARTESIAN_POINT('Ctrl Pts',(-5.23317570391704,-4.29427031888077,
57.9159143216363));
#197602=CARTESIAN_POINT('Ctrl Pts',(-5.11311782003383,-4.43654276189698,
57.9246635581533));
#197603=CARTESIAN_POINT('Ctrl Pts',(-4.98740458984623,-4.57362924351994,
57.9334127946703));
#197604=CARTESIAN_POINT('Ctrl Pts',(-4.86169180711613,-4.71071523720401,
57.9421620000458));
#197605=CARTESIAN_POINT('Ctrl Pts',(-4.73032391204042,-4.84261509523364,
57.9509112054212));
#197606=CARTESIAN_POINT('Ctrl Pts',(-4.59374707013471,-4.96888084538448,
57.9596604107967));
#197607=CARTESIAN_POINT('Ctrl Pts',(-4.45717070301289,-5.09514615659601,
57.9684095857571));
#197608=CARTESIAN_POINT('Ctrl Pts',(-4.31538563570856,-5.21577720459682,
57.9771587607176));
#197609=CARTESIAN_POINT('Ctrl Pts',(-4.16887341029293,-5.33036429233055,
57.985907935678));
#197610=CARTESIAN_POINT('Ctrl Pts',(-4.02236168203482,-5.44495099123782,
57.9946570809501));
#197611=CARTESIAN_POINT('Ctrl Pts',(-3.87112305347933,-5.55349359438764,
58.0034062262221));
#197612=CARTESIAN_POINT('Ctrl Pts',(-3.7156711701752,-5.65562346299052,
58.0121553714941));
#197613=CARTESIAN_POINT('Ctrl Pts',(-3.56021980145573,-5.75775299351796,
58.0209044878043));
#197614=CARTESIAN_POINT('Ctrl Pts',(-3.40055544538098,-5.85346967464019,
58.0296536041144));
#197615=CARTESIAN_POINT('Ctrl Pts',(-3.23722035986597,-5.94244842987041,
58.0384027204246));
#197616=CARTESIAN_POINT('Ctrl Pts',(-3.07388580146891,-6.03142689794677,
58.0471518084995));
#197617=CARTESIAN_POINT('Ctrl Pts',(-2.90688078896256,-6.11366734656935,
58.0559008965743));
#197618=CARTESIAN_POINT('Ctrl Pts',(-2.73677250721014,-6.18889046952511,
58.0646499846492));
#197619=CARTESIAN_POINT('Ctrl Pts',(-2.566664760311,-6.26411335596484,58.0733990452152));
#197620=CARTESIAN_POINT('Ctrl Pts',(-2.39345402574757,-6.33231884500711,
58.0821481057813));
#197621=CARTESIAN_POINT('Ctrl Pts',(-2.21772856065155,-6.39327529762878,
58.0908971663473));
#197622=CARTESIAN_POINT('Ctrl Pts',(-2.04200363348044,-6.4542315636526,
58.099646200131));
#197623=CARTESIAN_POINT('Ctrl Pts',(-1.86376426188776,-6.50793874375803,
58.1083952339147));
#197624=CARTESIAN_POINT('Ctrl Pts',(-1.68361577752619,-6.55421443909679,
58.1171442676984));
#197625=CARTESIAN_POINT('Ctrl Pts',(-1.50346782967279,-6.60048999661986,
58.1258932754262));
#197626=CARTESIAN_POINT('Ctrl Pts',(-1.32141105794483,-6.63933404237812,
58.1346422831541));
#197627=CARTESIAN_POINT('Ctrl Pts',(-1.13806375486535,-6.67061465607644,
58.1433912908819));
#197628=CARTESIAN_POINT('Ctrl Pts',(-0.954716982598694,-6.70189517921356,
58.1521402732803));
#197629=CARTESIAN_POINT('Ctrl Pts',(-0.770079968898376,-6.7256122659227,
58.1608892556786));
#197630=CARTESIAN_POINT('Ctrl Pts',(-0.584779765555054,-6.7416853698313,
58.169638238077));
#197631=CARTESIAN_POINT('Ctrl Pts',(-0.391489830648159,-6.75845151013871,
58.1787644570869));
#197632=CARTESIAN_POINT('Ctrl Pts',(-0.197478578235256,-6.76689983031634,
58.1878906760967));
#197633=CARTESIAN_POINT('Ctrl Pts',(-0.00346287644832417,-6.76699911397118,
58.1970168951066));
#197634=CARTESIAN_POINT('Ctrl Pts',(0.184489834657796,-6.7670952950118,
58.2058579197724));
#197635=CARTESIAN_POINT('Ctrl Pts',(0.372446404253271,-6.75935639738147,
58.2146989444382));
#197636=CARTESIAN_POINT('Ctrl Pts',(0.559755019492222,-6.74380925873154,
58.223539969104));
#197637=CARTESIAN_POINT('Ctrl Pts',(0.7451347055257,-6.72842222659762,58.2322899477138));
#197638=CARTESIAN_POINT('Ctrl Pts',(0.929879431232527,-6.70538706057469,
58.2410399263235));
#197639=CARTESIAN_POINT('Ctrl Pts',(1.11336163627224,-6.67478200894061,
58.2497899049333));
#197640=CARTESIAN_POINT('Ctrl Pts',(1.29684196301129,-6.64417727060933,
58.2585397939698));
#197641=CARTESIAN_POINT('Ctrl Pts',(1.47905951217931,-6.60600284890497,
58.2672896830063));
#197642=CARTESIAN_POINT('Ctrl Pts',(1.65939532067515,-6.56038841607122,
58.2760395720429));
#197643=CARTESIAN_POINT('Ctrl Pts',(1.83972934301232,-6.51477443503135,
58.284789374415));
#197644=CARTESIAN_POINT('Ctrl Pts',(2.01818138406693,-6.46172066062007,
58.2935391767872));
#197645=CARTESIAN_POINT('Ctrl Pts',(2.19414528354626,-6.40140730423332,
58.3022889791593));
#197646=CARTESIAN_POINT('Ctrl Pts',(2.37010749864418,-6.34109452518486,
58.3110386977757));
#197647=CARTESIAN_POINT('Ctrl Pts',(2.5435813486687,-6.27352239616337,58.319788416392));
#197648=CARTESIAN_POINT('Ctrl Pts',(2.71397759435957,-6.19892043966643,
58.3285381350083));
#197649=CARTESIAN_POINT('Ctrl Pts',(2.88437226558517,-6.1243191724933,58.337287772777));
#197650=CARTESIAN_POINT('Ctrl Pts',(3.0516891268134,-6.04268832278604,58.3460374105457));
#197651=CARTESIAN_POINT('Ctrl Pts',(3.2153598627423,-5.95430516123131,58.3547870483144));
#197652=CARTESIAN_POINT('Ctrl Pts',(3.37902914073225,-5.8659227869722,58.3635366081435));
#197653=CARTESIAN_POINT('Ctrl Pts',(3.53905210621962,-5.77078835741703,
58.3722861679726));
#197654=CARTESIAN_POINT('Ctrl Pts',(3.69488522832093,-5.66922500431372,
58.3810357278016));
#197655=CARTESIAN_POINT('Ctrl Pts',(3.8507170140734,-5.56766252216817,58.3897852125988));
#197656=CARTESIAN_POINT('Ctrl Pts',(4.00235878822809,-5.45967138329074,
58.3985346973959));
#197657=CARTESIAN_POINT('Ctrl Pts',(4.14929549611733,-5.34561838199291,
58.407284182193));
#197658=CARTESIAN_POINT('Ctrl Pts',(4.29623099276496,-5.23156632086682,
58.4160335948656));
#197659=CARTESIAN_POINT('Ctrl Pts',(4.43846127436432,-5.11145267304613,
58.4247830075382));
#197660=CARTESIAN_POINT('Ctrl Pts',(4.57550326054843,-4.98568540049517,
58.4335324202108));
#197661=CARTESIAN_POINT('Ctrl Pts',(4.71254416258175,-4.85991912289978,
58.442281763666));
#197662=CARTESIAN_POINT('Ctrl Pts',(4.84439664019148,-4.72849950385022,
58.4510311071213));
#197663=CARTESIAN_POINT('Ctrl Pts',(4.97061286795124,-4.59187289860657,
58.4597804505765));
#197664=CARTESIAN_POINT('Ctrl Pts',(5.09682813913048,-4.45524732884269,
58.4685297277214));
#197665=CARTESIAN_POINT('Ctrl Pts',(5.21740705148187,-4.31341506235366,
58.4772790048662));
#197666=CARTESIAN_POINT('Ctrl Pts',(5.33194007546028,-4.16685781275299,
58.486028282011));
#197667=CARTESIAN_POINT('Ctrl Pts',(5.44647226944806,-4.02030162521407,
58.4947774957521));
#197668=CARTESIAN_POINT('Ctrl Pts',(5.55495848628422,-3.8690207488749,58.5035267094933));
#197669=CARTESIAN_POINT('Ctrl Pts',(5.65703027292085,-3.7135289808021,58.5122759232344));
#197670=CARTESIAN_POINT('Ctrl Pts',(5.75910135377282,-3.55803828789128,
58.5210250764783));
#197671=CARTESIAN_POINT('Ctrl Pts',(5.85475793593024,-3.39833700106244,
58.5297742297221));
#197672=CARTESIAN_POINT('Ctrl Pts',(5.94367514427657,-3.23496750823078,
58.538523382966));
#197673=CARTESIAN_POINT('Ctrl Pts',(6.03259176732892,-3.07159909077231,
58.547272478619));
#197674=CARTESIAN_POINT('Ctrl Pts',(6.11476896836168,-2.90456276730922,
58.5560215742719));
#197675=CARTESIAN_POINT('Ctrl Pts',(6.1899276554812,-2.73442583002521,58.5647706699248));
#197676=CARTESIAN_POINT('Ctrl Pts',(6.26508587283272,-2.56428995615637,
58.5735197108929));
#197677=CARTESIAN_POINT('Ctrl Pts',(6.33322554827363,-2.39105376934665,
58.5822687518609));
#197678=CARTESIAN_POINT('Ctrl Pts',(6.39411526733217,-2.21530561053541,
58.5910177928289));
#197679=CARTESIAN_POINT('Ctrl Pts',(6.4550046260302,-2.03955849184554,58.599766782018));
#197680=CARTESIAN_POINT('Ctrl Pts',(6.50864402040897,-1.86129970163995,
58.608515771207));
#197681=CARTESIAN_POINT('Ctrl Pts',(6.55485128368743,-1.68113463135505,
58.617264760396));
#197682=CARTESIAN_POINT('Ctrl Pts',(6.60199809554447,-1.49730620116336,
58.6261916458674));
#197683=CARTESIAN_POINT('Ctrl Pts',(6.64140720707974,-1.31149343245187,
58.6351185313388));
#197684=CARTESIAN_POINT('Ctrl Pts',(6.67293928722966,-1.12435326697037,
58.6440454168103));
#197685=CARTESIAN_POINT('Ctrl Pts',(6.70384625876325,-0.940923067001745,
58.6527953309877));
#197686=CARTESIAN_POINT('Ctrl Pts',(6.7271855457985,-0.756217899516862,
58.6615452451652));
#197687=CARTESIAN_POINT('Ctrl Pts',(6.74287786815368,-0.570865181249742,
58.6702951593427));
#197688=CARTESIAN_POINT('Ctrl Pts',(6.75856988190873,-0.385516108069222,
58.6790449014471));
#197689=CARTESIAN_POINT('Ctrl Pts',(6.76661520773417,-0.199519795221659,
58.6877946435516));
#197690=CARTESIAN_POINT('Ctrl Pts',(6.7669865178958,-0.0135080204510007,
58.6965443856561));
#197691=CARTESIAN_POINT('Ctrl Pts',(6.76735782124891,0.172500343517631,
58.7052939673211));
#197692=CARTESIAN_POINT('Ctrl Pts',(6.76005538995159,0.358523882215608,
58.7140435489861));
#197693=CARTESIAN_POINT('Ctrl Pts',(6.74510402742323,0.543930748569076,
58.722793130651));
#197694=CARTESIAN_POINT('Ctrl Pts',(6.7301529191798,0.729334461619886,58.7315425635077));
#197695=CARTESIAN_POINT('Ctrl Pts',(6.70755316306532,0.914121237639279,
58.7402919963644));
#197696=CARTESIAN_POINT('Ctrl Pts',(6.677381518745,1.09766345166576,58.7490414292211));
#197697=CARTESIAN_POINT('Ctrl Pts',(6.64721034747483,1.28120278800113,58.7577907248986));
#197698=CARTESIAN_POINT('Ctrl Pts',(6.60946757205044,1.46349731860771,58.7665400205761));
#197699=CARTESIAN_POINT('Ctrl Pts',(6.56428138111414,1.64392790278598,58.7752893162536));
#197700=CARTESIAN_POINT('Ctrl Pts',(6.51909583859729,1.82435589779488,58.7840384863792));
#197701=CARTESIAN_POINT('Ctrl Pts',(6.46646716392743,2.00291972192693,58.7927876565048));
#197702=CARTESIAN_POINT('Ctrl Pts',(6.4065740987274,2.17901292275086,58.8015368266304));
#197703=CARTESIAN_POINT('Ctrl Pts',(6.34668181341923,2.3551038305939,58.8102858828295));
#197704=CARTESIAN_POINT('Ctrl Pts',(6.27952541913887,2.52872390822984,58.8190349390287));
#197705=CARTESIAN_POINT('Ctrl Pts',(6.20533299175345,2.69928350890679,58.8277839952278));
#197706=CARTESIAN_POINT('Ctrl Pts',(6.12831602991371,2.87633637966001,58.836866131386));
#197707=CARTESIAN_POINT('Ctrl Pts',(6.04371690605088,3.05009086601823,58.8459482675441));
#197708=CARTESIAN_POINT('Ctrl Pts',(5.95184520316445,3.21991112883079,58.8550304037023));
#197709=CARTESIAN_POINT('Ctrl Pts',(5.86333549509076,3.38351691183362,58.8637801840459));
#197710=CARTESIAN_POINT('Ctrl Pts',(5.76807618099157,3.54347103712348,58.8725299643895));
#197711=CARTESIAN_POINT('Ctrl Pts',(5.66639083308792,3.69923018028039,58.881279744733));
#197712=CARTESIAN_POINT('Ctrl Pts',(5.56470914081962,3.85498372382395,58.8900292105179));
#197713=CARTESIAN_POINT('Ctrl Pts',(5.45660203371814,4.00654234702343,58.8987786763029));
#197714=CARTESIAN_POINT('Ctrl Pts',(5.34243669838949,4.15339127987014,58.9075281420878));
#197715=CARTESIAN_POINT('Ctrl Pts',(5.22827486050311,4.30023571401621,58.9162773398338));
#197716=CARTESIAN_POINT('Ctrl Pts',(5.10805534166817,4.44237052028808,58.9250265375798));
#197717=CARTESIAN_POINT('Ctrl Pts',(4.98218644339644,4.57931296629055,58.9337757353258));
#197718=CARTESIAN_POINT('Ctrl Pts',(4.8563207321927,4.71625194483686,58.9425247115375));
#197719=CARTESIAN_POINT('Ctrl Pts',(4.72480612169994,4.84799861524825,58.9512736877491));
#197720=CARTESIAN_POINT('Ctrl Pts',(4.58808925234978,4.97410554898793,58.9600226639607));
#197721=CARTESIAN_POINT('Ctrl Pts',(4.45136349473707,5.10022068121504,58.9687722089624));
#197722=CARTESIAN_POINT('Ctrl Pts',(4.30943501209732,5.22069514872121,58.9775217539641));
#197723=CARTESIAN_POINT('Ctrl Pts',(4.16278587431427,5.33511975166534,58.9862712989658));
#197724=CARTESIAN_POINT('Ctrl Pts',(4.01614535740073,5.44953762808119,58.9950203296196));
#197725=CARTESIAN_POINT('Ctrl Pts',(3.86478496657528,5.55790617533059,59.0037693602733));
#197726=CARTESIAN_POINT('Ctrl Pts',(3.7092187474678,5.65985735539629,59.012518390927));
#197727=CARTESIAN_POINT('Ctrl Pts',(3.55365041605485,5.76180991977303,59.0212675403766));
#197728=CARTESIAN_POINT('Ctrl Pts',(3.39387638174108,5.85734478553053,59.0300166898263));
#197729=CARTESIAN_POINT('Ctrl Pts',(3.23043927904125,5.94613749121457,59.0387658392759));
#197730=CARTESIAN_POINT('Ctrl Pts',(3.1869176707015,5.96978206944296,59.041095647192));
#197731=CARTESIAN_POINT('Ctrl Pts',(3.14313645919485,5.99294880633501,59.0434254551081));
#197732=CARTESIAN_POINT('Ctrl Pts',(3.09910619832129,6.01563211736943,59.0457552630241));
#197733=CARTESIAN_POINT('Ctrl Pts',(3.09910619832134,6.0156321173694,57.0459010634246));
#197734=CARTESIAN_POINT('Ctrl Pts',(2.93708941130078,6.09909919432674,57.0544544424911));
#197735=CARTESIAN_POINT('Ctrl Pts',(2.77164155858761,6.17604560811617,57.0630078215577));
#197736=CARTESIAN_POINT('Ctrl Pts',(2.60333644578525,6.24619310860994,57.0715612006242));
#197737=CARTESIAN_POINT('Ctrl Pts',(2.44204607508404,6.31341695089267,57.0797580857777));
#197738=CARTESIAN_POINT('Ctrl Pts',(2.27813215886749,6.37439700936649,57.0879549709313));
#197739=CARTESIAN_POINT('Ctrl Pts',(2.1121209293986,6.42893725117895,57.0961518560848));
#197740=CARTESIAN_POINT('Ctrl Pts',(1.94609294049766,6.48348299902543,57.1043495687434));
#197741=CARTESIAN_POINT('Ctrl Pts',(1.77796755733578,6.53158752260565,57.112547281402));
#197742=CARTESIAN_POINT('Ctrl Pts',(1.60828684773392,6.57310447318511,57.1207449940607));
#197743=CARTESIAN_POINT('Ctrl Pts',(1.43855815497868,6.61463316413395,57.1289450249092));
#197744=CARTESIAN_POINT('Ctrl Pts',(1.26727360808535,6.64957048589982,57.1371450557577));
#197745=CARTESIAN_POINT('Ctrl Pts',(1.09498620479806,6.67782106763141,57.1453450866062));
#197746=CARTESIAN_POINT('Ctrl Pts',(0.92261875341179,6.7060847751361,57.1535489273495));
#197747=CARTESIAN_POINT('Ctrl Pts',(0.749247871090595,6.72765549585866,
57.1617527680928));
#197748=CARTESIAN_POINT('Ctrl Pts',(0.575432475817302,6.74248963408731,
57.1699566088361));
#197749=CARTESIAN_POINT('Ctrl Pts',(0.401412906582284,6.75734119738216,
57.1781700863015));
#197750=CARTESIAN_POINT('Ctrl Pts',(0.226948139060304,6.76544034478136,
57.186383563767));
#197751=CARTESIAN_POINT('Ctrl Pts',(0.0525988345949597,6.76679557564726,
57.1945970412324));
#197752=CARTESIAN_POINT('Ctrl Pts',(-0.12187074230351,6.76815174140024,
57.2028161846506));
#197753=CARTESIAN_POINT('Ctrl Pts',(-0.296224340113023,6.76275472968003,
57.2110353280687));
#197754=CARTESIAN_POINT('Ctrl Pts',(-0.469905747545066,6.75066497379511,
57.2192544714869));
#197755=CARTESIAN_POINT('Ctrl Pts',(-0.643826689135678,6.73855854422275,
57.2274849504051));
#197756=CARTESIAN_POINT('Ctrl Pts',(-0.817073234136335,6.71974097753192,
57.2357154293233));
#197757=CARTESIAN_POINT('Ctrl Pts',(-0.989097810834744,6.69432405255392,
57.2439459082416));
#197758=CARTESIAN_POINT('Ctrl Pts',(-1.03951258960042,6.68687518289667,
57.2463579925016));
#197759=CARTESIAN_POINT('Ctrl Pts',(-1.08982250582229,6.67885983380128,
57.2487700767617));
#197760=CARTESIAN_POINT('Ctrl Pts',(-1.14001402095487,6.67028163063797,
57.2511821610217));
#197761=CARTESIAN_POINT('Ctrl Pts',(-1.30792310384148,6.64158438525373,
57.2592514702443));
#197762=CARTESIAN_POINT('Ctrl Pts',(-1.47505567297142,6.60649022861081,
57.2673207794668));
#197763=CARTESIAN_POINT('Ctrl Pts',(-1.64087397246921,6.56504543826417,
57.2753900886893));
#197764=CARTESIAN_POINT('Ctrl Pts',(-1.8064854514793,6.52365234083548,57.2834493332901));
#197765=CARTESIAN_POINT('Ctrl Pts',(-1.97078556511015,6.47592445964785,
57.2915085778908));
#197766=CARTESIAN_POINT('Ctrl Pts',(-2.13324219989485,6.42195972555012,
57.2995678224915));
#197767=CARTESIAN_POINT('Ctrl Pts',(-2.29553185794315,6.36805045767076,
57.3076187836118));
#197768=CARTESIAN_POINT('Ctrl Pts',(-2.45598145665742,6.30791721029896,
57.3156697447321));
#197769=CARTESIAN_POINT('Ctrl Pts',(-2.61406969909475,6.24170878912776,
57.3237207058524));
#197770=CARTESIAN_POINT('Ctrl Pts',(-2.77203009500253,6.17555391094459,
57.3317651561315));
#197771=CARTESIAN_POINT('Ctrl Pts',(-2.92763259301981,6.10333378089565,
57.3398096064106));
#197772=CARTESIAN_POINT('Ctrl Pts',(-3.08037178251789,6.02524677349132,
57.3478540566897));
#197773=CARTESIAN_POINT('Ctrl Pts',(-3.23302088446625,5.94720582281405,
57.355893762248));
#197774=CARTESIAN_POINT('Ctrl Pts',(-3.38280970842921,5.86330505275075,
57.3639334678062));
#197775=CARTESIAN_POINT('Ctrl Pts',(-3.52925364102936,5.77379058654546,
57.3719731733645));
#197776=CARTESIAN_POINT('Ctrl Pts',(-3.67885848762091,5.68234399844453,
57.3801864116689));
#197777=CARTESIAN_POINT('Ctrl Pts',(-3.82497203811319,5.58503877621496,
57.3883996499734));
#197778=CARTESIAN_POINT('Ctrl Pts',(-3.9671045819061,5.48218662909424,57.3966128882778));
#197779=CARTESIAN_POINT('Ctrl Pts',(-4.10618930336944,5.38153999425293,
57.404650005826));
#197780=CARTESIAN_POINT('Ctrl Pts',(-4.24146171358088,5.27558215213335,
57.4126871233742));
#197781=CARTESIAN_POINT('Ctrl Pts',(-4.37249307772857,5.1646484183549,57.4207242409224));
#197782=CARTESIAN_POINT('Ctrl Pts',(-4.50353830416122,5.05370294849295,
57.4287622087465));
#197783=CARTESIAN_POINT('Ctrl Pts',(-4.63034130590809,4.93778078013822,
57.4368001765706));
#197784=CARTESIAN_POINT('Ctrl Pts',(-4.75250748493224,4.81725664726959,
57.4448381443947));
#197785=CARTESIAN_POINT('Ctrl Pts',(-4.87471079398519,4.69669588344007,
57.4528785552024));
#197786=CARTESIAN_POINT('Ctrl Pts',(-4.99227420935914,4.57153063329252,
57.4609189660102));
#197787=CARTESIAN_POINT('Ctrl Pts',(-5.10484107074446,4.44217138823353,
57.4689593768179));
#197788=CARTESIAN_POINT('Ctrl Pts',(-5.22166232460481,4.30792309330691,
57.4773036698057));
#197789=CARTESIAN_POINT('Ctrl Pts',(-5.33310166985868,4.16915792692092,
57.4856479627935));
#197790=CARTESIAN_POINT('Ctrl Pts',(-5.4388081030987,4.02637000506262,57.4939922557813));
#197791=CARTESIAN_POINT('Ctrl Pts',(-5.54084480270537,3.88853914800367,
57.5020468659968));
#197792=CARTESIAN_POINT('Ctrl Pts',(-5.63753981844651,3.74696050612187,
57.5101014762123));
#197793=CARTESIAN_POINT('Ctrl Pts',(-5.72862340538127,3.60210533984195,
57.5181560864279));
#197794=CARTESIAN_POINT('Ctrl Pts',(-5.81977594387776,3.4571405161553,57.5262167940971));
#197795=CARTESIAN_POINT('Ctrl Pts',(-5.90530841004553,3.30889455068405,
57.5342775017664));
#197796=CARTESIAN_POINT('Ctrl Pts',(-5.98499812208102,3.15786106070021,
57.5423382094356));
#197797=CARTESIAN_POINT('Ctrl Pts',(-6.06480019183685,3.00661462254282,
57.5504102822198));
#197798=CARTESIAN_POINT('Ctrl Pts',(-6.13874291127432,2.8525731519391,57.558482355004));
#197799=CARTESIAN_POINT('Ctrl Pts',(-6.2066523592396,2.69624841057822,57.5665544277882));
#197800=CARTESIAN_POINT('Ctrl Pts',(-6.2137653579533,2.67987458164076,57.5673999160825));
#197801=CARTESIAN_POINT('Ctrl Pts',(-6.22081221150533,2.66347571459303,
57.5682454043769));
#197802=CARTESIAN_POINT('Ctrl Pts',(-6.2277927521944,2.64705240516974,57.5690908926713));
#197803=CARTESIAN_POINT('Ctrl Pts',(-6.30728184109723,2.46003624682668,
57.5787186704022));
#197804=CARTESIAN_POINT('Ctrl Pts',(-6.37837738907553,2.26935700482112,
57.5883464481332));
#197805=CARTESIAN_POINT('Ctrl Pts',(-6.44078272410078,2.0757184059802,57.5979742258642));
#197806=CARTESIAN_POINT('Ctrl Pts',(-6.50285624708936,1.88310939247571,
57.6075508122582));
#197807=CARTESIAN_POINT('Ctrl Pts',(-6.5563316696614,1.68757250775811,57.6171273986522));
#197808=CARTESIAN_POINT('Ctrl Pts',(-6.60096333987442,1.48982280343468,
57.6267039850461));
#197809=CARTESIAN_POINT('Ctrl Pts',(-6.6454136680469,1.29287657195301,57.6362416610047));
#197810=CARTESIAN_POINT('Ctrl Pts',(-6.68109188231582,1.09373556062145,
57.6457793369633));
#197811=CARTESIAN_POINT('Ctrl Pts',(-6.70780239938444,0.893127074280214,
57.6553170129219));
#197812=CARTESIAN_POINT('Ctrl Pts',(-6.73431424062455,0.694010736411043,
57.6647837465746));
#197813=CARTESIAN_POINT('Ctrl Pts',(-6.75199122402378,0.493448781645467,
57.6742504802273));
#197814=CARTESIAN_POINT('Ctrl Pts',(-6.76068966814693,0.29217154380841,
57.68371721388));
#197815=CARTESIAN_POINT('Ctrl Pts',(-6.76481299855797,0.19675993409133,
57.68820473719));
#197816=CARTESIAN_POINT('Ctrl Pts',(-6.76691950451404,0.101187865534849,
57.6926922605));
#197817=CARTESIAN_POINT('Ctrl Pts',(-6.76699773672647,0.00553454053396756,
57.69717978381));
#197818=CARTESIAN_POINT('',(-6.76699833040872,0.00475355083741498,57.3028202162319));
#197819=CARTESIAN_POINT('Ctrl Pts',(3.09910619832132,6.01563211736941,56.6514148629243));
#197820=CARTESIAN_POINT('Ctrl Pts',(2.9288158558623,6.10336152726886,56.6604562095772));
#197821=CARTESIAN_POINT('Ctrl Pts',(2.75474742236709,6.18388246268263,56.6694975562302));
#197822=CARTESIAN_POINT('Ctrl Pts',(2.57750328655722,6.2568974586281,56.6785389028831));
#197823=CARTESIAN_POINT('Ctrl Pts',(2.40043744629085,6.32983900645453,56.6875711545564));
#197824=CARTESIAN_POINT('Ctrl Pts',(2.22020250089245,6.39528959756098,56.6966034062296));
#197825=CARTESIAN_POINT('Ctrl Pts',(2.03742186377874,6.45299939167798,56.7056356579029));
#197826=CARTESIAN_POINT('Ctrl Pts',(1.8549763315794,6.51060338227049,56.7146513500983));
#197827=CARTESIAN_POINT('Ctrl Pts',(1.66999465320859,6.56049484068034,56.7236670422936));
#197828=CARTESIAN_POINT('Ctrl Pts',(1.48311635673492,6.60247339050945,56.732682734489));
#197829=CARTESIAN_POINT('Ctrl Pts',(1.29648441379771,6.64439660184072,56.7416865416891));
#197830=CARTESIAN_POINT('Ctrl Pts',(1.10796107345928,6.67842766797474,56.7506903488893));
#197831=CARTESIAN_POINT('Ctrl Pts',(0.918199525888249,6.70441635272293,
56.7596941560894));
#197832=CARTESIAN_POINT('Ctrl Pts',(0.728849668397189,6.73034865469053,
56.7686784294158));
#197833=CARTESIAN_POINT('Ctrl Pts',(0.538267200699625,6.74827336726381,
56.7776627027423));
#197834=CARTESIAN_POINT('Ctrl Pts',(0.347113800198479,6.75809152125893,
56.7866469760687));
#197835=CARTESIAN_POINT('Ctrl Pts',(0.259573056317174,6.7625878498726,56.7907614201129));
#197836=CARTESIAN_POINT('Ctrl Pts',(0.171912726692458,6.76538470783889,
56.7948758641572));
#197837=CARTESIAN_POINT('Ctrl Pts',(0.0841970533280191,6.76647617717013,
56.7989903082014));
#197838=CARTESIAN_POINT('Ctrl Pts',(-0.0889441416684437,6.76863061886869,
56.8071117730576));
#197839=CARTESIAN_POINT('Ctrl Pts',(-0.262223833179623,6.76413588094265,
56.8152332379138));
#197840=CARTESIAN_POINT('Ctrl Pts',(-0.435089414198062,6.75299831198356,
56.82335470277));
#197841=CARTESIAN_POINT('Ctrl Pts',(-0.607942667356204,6.74186153729707,
56.8314755884462));
#197842=CARTESIAN_POINT('Ctrl Pts',(-0.780381503416446,6.72408289872817,
56.8395964741224));
#197843=CARTESIAN_POINT('Ctrl Pts',(-0.951856303852425,6.69972078349661,
56.8477173597986));
#197844=CARTESIAN_POINT('Ctrl Pts',(-1.12335160043043,6.67535575629564,
56.8558392161529));
#197845=CARTESIAN_POINT('Ctrl Pts',(-1.29388226956476,6.64440573820314,
56.8639610725071));
#197846=CARTESIAN_POINT('Ctrl Pts',(-1.46290682470662,6.60698059799079,
56.8720829288614));
#197847=CARTESIAN_POINT('Ctrl Pts',(-1.63205469807292,6.56952815285914,
56.8802107108216));
#197848=CARTESIAN_POINT('Ctrl Pts',(-1.79969390486481,6.52559122939987,
56.8883384927817));
#197849=CARTESIAN_POINT('Ctrl Pts',(-1.96529548865556,6.47533031144127,
56.8964662747419));
#197850=CARTESIAN_POINT('Ctrl Pts',(-2.13096453237613,6.4250489190529,56.9045973676583));
#197851=CARTESIAN_POINT('Ctrl Pts',(-2.29459395275117,6.36843851679601,
56.9127284605748));
#197852=CARTESIAN_POINT('Ctrl Pts',(-2.45567308105799,6.30570842324375,
56.9208595534912));
#197853=CARTESIAN_POINT('Ctrl Pts',(-2.61692802050191,6.24290986241585,
56.9289995211558));
#197854=CARTESIAN_POINT('Ctrl Pts',(-2.77562677276144,6.17397841504057,
56.9371394888204));
#197855=CARTESIAN_POINT('Ctrl Pts',(-2.93128096700278,6.09917050855994,
56.9452794564849));
#197856=CARTESIAN_POINT('Ctrl Pts',(-3.01200996219032,6.06037189377348,
56.9495011956653));
#197857=CARTESIAN_POINT('Ctrl Pts',(-3.09192042237868,6.01999331053127,
56.9537229348457));
#197858=CARTESIAN_POINT('Ctrl Pts',(-3.17094717972885,5.9780751905082,56.9579446740261));
#197859=CARTESIAN_POINT('Ctrl Pts',(-3.32893950381451,5.89427140776661,
56.9663848834837));
#197860=CARTESIAN_POINT('Ctrl Pts',(-3.48372465004122,5.80413841391356,
56.9748250929413));
#197861=CARTESIAN_POINT('Ctrl Pts',(-3.63478172484608,5.70794628677644,
56.9832653023989));
#197862=CARTESIAN_POINT('Ctrl Pts',(-3.78572435153768,5.61182703942649,
56.9916991171475));
#197863=CARTESIAN_POINT('Ctrl Pts',(-3.93294425710903,5.5096579885086,57.000132931896));
#197864=CARTESIAN_POINT('Ctrl Pts',(-4.07594610930425,5.40175455884915,
57.0085667466445));
#197865=CARTESIAN_POINT('Ctrl Pts',(-4.21886159964126,5.29391629436448,
57.0169954680331));
#197866=CARTESIAN_POINT('Ctrl Pts',(-4.35756384961711,5.18035075571406,
57.0254241894216));
#197867=CARTESIAN_POINT('Ctrl Pts',(-4.49158710898992,5.0614162289181,57.0338529108102));
#197868=CARTESIAN_POINT('Ctrl Pts',(-4.62555000920494,4.94253526586851,
57.0422778362119));
#197869=CARTESIAN_POINT('Ctrl Pts',(-4.754837871411,4.81829035686463,57.0507027616137));
#197870=CARTESIAN_POINT('Ctrl Pts',(-4.87901830230743,4.68907980373006,
57.0591276870154));
#197871=CARTESIAN_POINT('Ctrl Pts',(-5.00316185985319,4.5599076175588,57.0675501107731));
#197872=CARTESIAN_POINT('Ctrl Pts',(-5.12220077962333,4.42577296785309,
57.0759725345309));
#197873=CARTESIAN_POINT('Ctrl Pts',(-5.23573952232929,4.28711099160251,
57.0843949582886));
#197874=CARTESIAN_POINT('Ctrl Pts',(-5.34928005067248,4.14844683459864,
57.0928175145069));
#197875=CARTESIAN_POINT('Ctrl Pts',(-5.45732001275269,4.00525546253049,
57.101240070725));
#197876=CARTESIAN_POINT('Ctrl Pts',(-5.5595037461799,3.85800558530073,57.1096626269433));
#197877=CARTESIAN_POINT('Ctrl Pts',(-5.66169093139295,3.71075073394229,
57.118085467677));
#197878=CARTESIAN_POINT('Ctrl Pts',(-5.75802130319094,3.5594373780211,57.1265083084108));
#197879=CARTESIAN_POINT('Ctrl Pts',(-5.84818210335718,3.40456386134447,
57.1349311491445));
#197880=CARTESIAN_POINT('Ctrl Pts',(-5.93835853661733,3.24966349095508,
57.1433554503251));
#197881=CARTESIAN_POINT('Ctrl Pts',(-6.02236309766209,3.09120201736223,
57.1517797515058));
#197882=CARTESIAN_POINT('Ctrl Pts',(-6.0999284488278,2.92970338416388,57.1602040526864));
#197883=CARTESIAN_POINT('Ctrl Pts',(-6.17751808144624,2.76815419461056,
57.1686309910532));
#197884=CARTESIAN_POINT('Ctrl Pts',(-6.24866434094537,2.60356625044192,
57.17705792942));
#197885=CARTESIAN_POINT('Ctrl Pts',(-6.31314744019751,2.43648484467433,
57.1854848677868));
#197886=CARTESIAN_POINT('Ctrl Pts',(-6.37768851786137,2.26925321172088,
57.1939193830305));
#197887=CARTESIAN_POINT('Ctrl Pts',(-6.43555434405825,2.09952394891718,
57.2023538982741));
#197888=CARTESIAN_POINT('Ctrl Pts',(-6.48657419007526,1.92786002517027,
57.2107884135178));
#197889=CARTESIAN_POINT('Ctrl Pts',(-6.53761867911499,1.75611318627751,
57.2192270027045));
#197890=CARTESIAN_POINT('Ctrl Pts',(-6.58181050603663,1.58243014458215,
57.2276655918913));
#197891=CARTESIAN_POINT('Ctrl Pts',(-6.61902964998118,1.4073860496218,57.2361041810781));
#197892=CARTESIAN_POINT('Ctrl Pts',(-6.65629039650801,1.23214629496615,
57.2445522026984));
#197893=CARTESIAN_POINT('Ctrl Pts',(-6.6865628251688,1.05554277504005,57.2530002243187));
#197894=CARTESIAN_POINT('Ctrl Pts',(-6.70977836961247,0.878159000796931,
57.261448245939));
#197895=CARTESIAN_POINT('Ctrl Pts',(-6.72297371250336,0.777336910231834,
57.2662499658513));
#197896=CARTESIAN_POINT('Ctrl Pts',(-6.73389020537125,0.67626284025593,
57.2710516857635));
#197897=CARTESIAN_POINT('Ctrl Pts',(-6.74252275698126,0.57504423446365,
57.2758534056758));
#197898=CARTESIAN_POINT('Ctrl Pts',(-6.75868310423,0.385560534680092,57.2848423425139));
#197899=CARTESIAN_POINT('Ctrl Pts',(-6.76686449420557,0.195278323762471,
57.2938312793519));
#197900=CARTESIAN_POINT('Ctrl Pts',(-6.7669983304081,0.00475355172657754,
57.3028202161899));
#197901=CARTESIAN_POINT('Ctrl Pts',(-6.76699833040872,0.00475355083741949,
57.3028202162319));
#197902=CARTESIAN_POINT('Ctrl Pts',(-6.76711724571589,-0.164530361876449,
57.3108070117694));
#197903=CARTESIAN_POINT('Ctrl Pts',(-6.76087979991684,-0.334076059823817,
57.3187938073069));
#197904=CARTESIAN_POINT('Ctrl Pts',(-6.74825359655539,-0.503351166262,57.3267806028444));
#197905=CARTESIAN_POINT('Ctrl Pts',(-6.73563867023757,-0.672475085307733,
57.334760265007));
#197906=CARTESIAN_POINT('Ctrl Pts',(-6.71664636501254,-0.841328517593721,
57.3427399271696));
#197907=CARTESIAN_POINT('Ctrl Pts',(-6.69129630022003,-1.00937744311123,
57.3507195893322));
#197908=CARTESIAN_POINT('Ctrl Pts',(-6.66596532811808,-1.17729980066293,
57.3586932415212));
#197909=CARTESIAN_POINT('Ctrl Pts',(-6.63428618501412,-1.34441848357119,
57.3666668937102));
#197910=CARTESIAN_POINT('Ctrl Pts',(-6.59633041995841,-1.5102032945042,
57.3746405458993));
#197911=CARTESIAN_POINT('Ctrl Pts',(-6.55839134800311,-1.67591519260062,
57.3826106912435));
#197912=CARTESIAN_POINT('Ctrl Pts',(-6.51418123128944,-1.84029401639184,
57.3905808365877));
#197913=CARTESIAN_POINT('Ctrl Pts',(-6.46382293043131,-2.00281854495867,
57.3985509819319));
#197914=CARTESIAN_POINT('Ctrl Pts',(-6.41347226683219,-2.16531842531661,
57.4065199185367));
#197915=CARTESIAN_POINT('Ctrl Pts',(-6.35697538289133,-2.32596420604132,
57.4144888551415));
#197916=CARTESIAN_POINT('Ctrl Pts',(-6.29450531389351,-2.48424875029986,
57.4224577917463));
#197917=CARTESIAN_POINT('Ctrl Pts',(-6.26223400319354,-2.56601670395697,
57.4265744516643));
#197918=CARTESIAN_POINT('Ctrl Pts',(-6.22836947764888,-2.64715478973649,
57.4306911115824));
#197919=CARTESIAN_POINT('Ctrl Pts',(-6.19294068818362,-2.72759502724284,
57.4348077715005));
#197920=CARTESIAN_POINT('Ctrl Pts',(-6.11669774364076,-2.90070284886974,
57.4436668456763));
#197921=CARTESIAN_POINT('Ctrl Pts',(-6.03326763538907,-3.07044202604806,
57.4525259198522));
#197922=CARTESIAN_POINT('Ctrl Pts',(-5.94297833293132,-3.23624744639666,
57.4613849940281));
#197923=CARTESIAN_POINT('Ctrl Pts',(-5.8525193950385,-3.40236438177365,
57.4702607126221));
#197924=CARTESIAN_POINT('Ctrl Pts',(-5.75517563289851,-3.56453256269319,
57.4791364312161));
#197925=CARTESIAN_POINT('Ctrl Pts',(-5.65131887296307,-3.72221493147446,
57.4880121498101));
#197926=CARTESIAN_POINT('Ctrl Pts',(-5.54716573518003,-3.88034728118229,
57.4969131971971));
#197927=CARTESIAN_POINT('Ctrl Pts',(-5.43646254941413,-4.03396798383621,
57.5058142445841));
#197928=CARTESIAN_POINT('Ctrl Pts',(-5.31962396419665,-4.18256976983586,
57.514715291971));
#197929=CARTESIAN_POINT('Ctrl Pts',(-5.20262653531977,-4.33137358200209,
57.523628440454));
#197930=CARTESIAN_POINT('Ctrl Pts',(-5.07947721033135,-4.47514464785269,
57.5325415889371));
#197931=CARTESIAN_POINT('Ctrl Pts',(-4.9506291973722,-4.61341083691078,
57.5414547374201));
#197932=CARTESIAN_POINT('Ctrl Pts',(-4.82149510659183,-4.75198401471636,
57.55038767553));
#197933=CARTESIAN_POINT('Ctrl Pts',(-4.68663719769362,-4.88502767839387,
57.5593206136398));
#197934=CARTESIAN_POINT('Ctrl Pts',(-4.54654570739704,-5.01210645642623,
57.5682535517497));
#197935=CARTESIAN_POINT('Ctrl Pts',(-4.41319892105528,-5.1330670274572,
57.5767564136082));
#197936=CARTESIAN_POINT('Ctrl Pts',(-4.27511077058095,-5.24862343007156,
57.5852592754667));
#197937=CARTESIAN_POINT('Ctrl Pts',(-4.13272995211554,-5.35843560592895,
57.5937621373252));
#197938=CARTESIAN_POINT('Ctrl Pts',(-3.99504005740441,-5.46462987489557,
57.6019848611911));
#197939=CARTESIAN_POINT('Ctrl Pts',(-3.85307118423185,-5.56565493352219,
57.6102075850569));
#197940=CARTESIAN_POINT('Ctrl Pts',(-3.70724803457597,-5.66114838262809,
57.6184303089228));
#197941=CARTESIAN_POINT('Ctrl Pts',(-3.56157923378442,-5.75654075515284,
57.626644329314));
#197942=CARTESIAN_POINT('Ctrl Pts',(-3.41206457795247,-5.84641298249386,
57.6348583497052));
#197943=CARTESIAN_POINT('Ctrl Pts',(-3.25916141275307,-5.93044314411844,
57.6430723700964));
#197944=CARTESIAN_POINT('Ctrl Pts',(-3.10638939174153,-6.01440123354434,
57.6512793453684));
#197945=CARTESIAN_POINT('Ctrl Pts',(-2.95023496211614,-6.09252706471693,
57.6594863206403));
#197946=CARTESIAN_POINT('Ctrl Pts',(-2.79118406851032,-6.16454219676483,
57.6676932959123));
#197947=CARTESIAN_POINT('Ctrl Pts',(-2.63223766816786,-6.23651001630799,
57.6758948793652));
#197948=CARTESIAN_POINT('Ctrl Pts',(-2.47039891984656,-6.30237498590982,
57.6840964628182));
#197949=CARTESIAN_POINT('Ctrl Pts',(-2.30617804569328,-6.36190473219792,
57.6922980462711));
#197950=CARTESIAN_POINT('Ctrl Pts',(-2.14203210663384,-6.4214073146608,
57.7004958872862));
#197951=CARTESIAN_POINT('Ctrl Pts',(-1.97550654382605,-6.47458031100016,
57.7086937283012));
#197952=CARTESIAN_POINT('Ctrl Pts',(-1.8071313011859,-6.52123956470502,
57.7168915693163));
#197953=CARTESIAN_POINT('Ctrl Pts',(-1.63877091713554,-6.56789470087634,
57.7250886868974));
#197954=CARTESIAN_POINT('Ctrl Pts',(-1.46856152152535,-6.60803713537928,
57.7332858044786));
#197955=CARTESIAN_POINT('Ctrl Pts',(-1.2970483094915,-6.64153255528009,
57.7414829220597));
#197956=CARTESIAN_POINT('Ctrl Pts',(-1.12553700573313,-6.67502760250705,
57.7496799484388));
#197957=CARTESIAN_POINT('Ctrl Pts',(-0.95272226641788,-6.70187571260162,
57.7578769748179));
#197958=CARTESIAN_POINT('Ctrl Pts',(-0.779159453741085,-6.72199371806058,
57.766074001197));
#197959=CARTESIAN_POINT('Ctrl Pts',(-0.60556701315866,-6.74211515774809,
57.7742724268432));
#197960=CARTESIAN_POINT('Ctrl Pts',(-0.431226601256352,-6.75550416261753,
57.7824708524893));
#197961=CARTESIAN_POINT('Ctrl Pts',(-0.256698728759893,-6.76212945473932,
57.7906692781354));
#197962=CARTESIAN_POINT('Ctrl Pts',(-0.0821093288132859,-6.76875708251859,
57.7988705940261));
#197963=CARTESIAN_POINT('Ctrl Pts',(0.0926673050172221,-6.76861623408654,
57.8070719099167));
#197964=CARTESIAN_POINT('Ctrl Pts',(0.267070581042112,-6.76172776032442,
57.8152732258074));
#197965=CARTESIAN_POINT('Ctrl Pts',(0.441672473204208,-6.75483144174377,
57.823483881624));
#197966=CARTESIAN_POINT('Ctrl Pts',(0.61589979917764,-6.74117215991515,
57.8316945374406));
#197967=CARTESIAN_POINT('Ctrl Pts',(0.789195946652915,-6.72082277387126,
57.8399051932572));
#197968=CARTESIAN_POINT('Ctrl Pts',(0.962594213349496,-6.70046139642718,
57.8481206874143));
#197969=CARTESIAN_POINT('Ctrl Pts',(1.13505985384755,-6.67340211189372,
57.8563361815715));
#197970=CARTESIAN_POINT('Ctrl Pts',(1.30604648660982,-6.63976893986637,
57.8645516757286));
#197971=CARTESIAN_POINT('Ctrl Pts',(1.47729840827921,-6.60608358535372,
57.8727799163761));
#197972=CARTESIAN_POINT('Ctrl Pts',(1.64706638757443,-6.56580404349757,
57.8810081570236));
#197973=CARTESIAN_POINT('Ctrl Pts',(1.81481794482534,-6.51910460317519,
57.8892363976711));
#197974=CARTESIAN_POINT('Ctrl Pts',(1.96727732865149,-6.47666226753757,
57.8967145547723));
#197975=CARTESIAN_POINT('Ctrl Pts',(2.11807119090478,-6.42891784237976,
57.9041927118735));
#197976=CARTESIAN_POINT('Ctrl Pts',(2.26681504283588,-6.37603627354589,
57.9116708689747));
#197977=CARTESIAN_POINT('Ctrl Pts',(2.42731717189511,-6.31897438980659,
57.9197401781972));
#197978=CARTESIAN_POINT('Ctrl Pts',(2.58595747511384,-6.25574346628744,
57.9278094874198));
#197979=CARTESIAN_POINT('Ctrl Pts',(2.74221409488188,-6.18648129859221,
57.9358787966423));
#197980=CARTESIAN_POINT('Ctrl Pts',(2.89827582017616,-6.11730551964482,
57.9439380412431));
#197981=CARTESIAN_POINT('Ctrl Pts',(3.05195944088801,-6.04211361378504,
57.9519972858438));
#197982=CARTESIAN_POINT('Ctrl Pts',(3.2027575147074,-5.96109329754075,57.9600565304446));
#197983=CARTESIAN_POINT('Ctrl Pts',(3.35340059473218,-5.88015625587642,
57.9681074915649));
#197984=CARTESIAN_POINT('Ctrl Pts',(3.50116370400768,-5.79340290029704,
57.9761584526852));
#197985=CARTESIAN_POINT('Ctrl Pts',(3.64555877954429,-5.70106921418146,
57.9842094138054));
#197986=CARTESIAN_POINT('Ctrl Pts',(3.78983708226455,-5.60881019864956,
57.9922538640845));
#197987=CARTESIAN_POINT('Ctrl Pts',(3.93075245962766,-5.51098003460954,
58.0002983143636));
#197988=CARTESIAN_POINT('Ctrl Pts',(4.06784099874613,-5.40786081634135,
58.0083427646427));
#197989=CARTESIAN_POINT('Ctrl Pts',(4.20484868127066,-5.30480241912218,
58.016382470201));
#197990=CARTESIAN_POINT('Ctrl Pts',(4.33803372136174,-5.19646140151004,
58.0244221757592));
#197991=CARTESIAN_POINT('Ctrl Pts',(4.46696088237514,-5.08316333352868,
58.0324618813175));
#197992=CARTESIAN_POINT('Ctrl Pts',(4.59867086723058,-4.96741978732257,
58.0406751196219));
#197993=CARTESIAN_POINT('Ctrl Pts',(4.72593673940524,-4.84650298249286,
58.0488883579264));
#197994=CARTESIAN_POINT('Ctrl Pts',(4.84832948585928,-4.72080397777195,
58.0571015962308));
#197995=CARTESIAN_POINT('Ctrl Pts',(4.96809770076211,-4.59780040242414,
58.065138713779));
#197996=CARTESIAN_POINT('Ctrl Pts',(5.08319940323806,-4.47021792965405,
58.0731758313272));
#197997=CARTESIAN_POINT('Ctrl Pts',(5.19326970059408,-4.33846042011351,
58.0812129488753));
#197998=CARTESIAN_POINT('Ctrl Pts',(5.30335164268751,-4.20668897146643,
58.0892509166994));
#197999=CARTESIAN_POINT('Ctrl Pts',(5.40840088015366,-4.07074189324922,
58.0972888845236));
#198000=CARTESIAN_POINT('Ctrl Pts',(5.50809291020161,-3.93105602765806,
58.1053268523476));
#198001=CARTESIAN_POINT('Ctrl Pts',(5.60781523969898,-3.7913277072707,58.1133672631554));
#198002=CARTESIAN_POINT('Ctrl Pts',(5.70217690391183,-3.64785864159494,
58.1214076739631));
#198003=CARTESIAN_POINT('Ctrl Pts',(5.79089690691449,-3.50111439594426,
58.1294480847709));
#198004=CARTESIAN_POINT('Ctrl Pts',(5.88297002564342,-3.34882404545615,
58.1377923777587));
#198005=CARTESIAN_POINT('Ctrl Pts',(5.96896647493851,-3.19300649258926,
58.1461366707464));
#198006=CARTESIAN_POINT('Ctrl Pts',(6.04862517023485,-3.03420871892517,
58.1544809637342));
#198007=CARTESIAN_POINT('Ctrl Pts',(6.12551841233805,-2.88092381248301,
58.1625355739498));
#198008=CARTESIAN_POINT('Ctrl Pts',(6.19650648129406,-2.72486250410686,
58.1705901841653));
#198009=CARTESIAN_POINT('Ctrl Pts',(6.26140442885749,-2.56653532574244,
58.1786447943808));
#198010=CARTESIAN_POINT('Ctrl Pts',(6.32635150508414,-2.40808829146705,
58.1867055020501));
#198011=CARTESIAN_POINT('Ctrl Pts',(6.3851991527014,-2.24737232020921,58.1947662097193));
#198012=CARTESIAN_POINT('Ctrl Pts',(6.43781262294535,-2.08491190025995,
58.2028269173886));
#198013=CARTESIAN_POINT('Ctrl Pts',(6.49050027502996,-1.92222242085252,
58.2108989901727));
#198014=CARTESIAN_POINT('Ctrl Pts',(6.53693611201876,-1.75778394157787,
58.2189710629568));
#198015=CARTESIAN_POINT('Ctrl Pts',(6.5770365347422,-1.59213046596888,58.2270431357409));
#198016=CARTESIAN_POINT('Ctrl Pts',(6.581236749349,-1.57477952299459,58.2278886240354));
#198017=CARTESIAN_POINT('Ctrl Pts',(6.58536750530445,-1.55741525391307,
58.2287341123298));
#198018=CARTESIAN_POINT('Ctrl Pts',(6.5894287395351,-1.54003827439088,58.2295796006243));
#198019=CARTESIAN_POINT('Ctrl Pts',(6.62945525259258,-1.36877509225432,
58.237912522671));
#198020=CARTESIAN_POINT('Ctrl Pts',(6.66285212335729,-1.19573053691983,
58.2462454447177));
#198021=CARTESIAN_POINT('Ctrl Pts',(6.68946360899263,-1.02145270275391,
58.2545783667644));
#198022=CARTESIAN_POINT('Ctrl Pts',(6.71604364630531,-0.847380822725198,
58.262901441318));
#198023=CARTESIAN_POINT('Ctrl Pts',(6.73585422025224,-0.672078908217391,
58.2712245158716));
#198024=CARTESIAN_POINT('Ctrl Pts',(6.74878996331768,-0.496107882443526,
58.2795475904253));
#198025=CARTESIAN_POINT('Ctrl Pts',(6.76171279390168,-0.320312511256482,
58.2878623568712));
#198026=CARTESIAN_POINT('Ctrl Pts',(6.76777444049541,-0.143849704344839,
58.2961771233172));
#198027=CARTESIAN_POINT('Ctrl Pts',(6.76692093589621,0.0327115779142395,
58.3044918897632));
#198028=CARTESIAN_POINT('Ctrl Pts',(6.76606812670532,0.209129003673223,
58.3127998816027));
#198029=CARTESIAN_POINT('Ctrl Pts',(6.75831139469508,0.385644398463105,
58.3211078734423));
#198030=CARTESIAN_POINT('Ctrl Pts',(6.74364873418873,0.561685632604875,
58.3294158652818));
#198031=CARTESIAN_POINT('Ctrl Pts',(6.72899533219164,0.737615708243444,
58.3377186111689));
#198032=CARTESIAN_POINT('Ctrl Pts',(6.70744472073708,0.913071874136868,
58.346021357056));
#198033=CARTESIAN_POINT('Ctrl Pts',(6.6790469481925,1.08748373037968,58.3543241029432));
#198034=CARTESIAN_POINT('Ctrl Pts',(6.65066078091265,1.26182431005451,58.3626234557626));
#198035=CARTESIAN_POINT('Ctrl Pts',(6.61543308402124,1.43512108759843,58.370922808582));
#198036=CARTESIAN_POINT('Ctrl Pts',(6.57346559623067,1.60681021131051,58.3792221614015));
#198037=CARTESIAN_POINT('Ctrl Pts',(6.53150703422064,1.77846281962653,58.3875197490878));
#198038=CARTESIAN_POINT('Ctrl Pts',(6.48281161960978,1.94850811753511,58.3958173367742));
#198039=CARTESIAN_POINT('Ctrl Pts',(6.42753195926004,2.11639361005716,58.4041149244605));
#198040=CARTESIAN_POINT('Ctrl Pts',(6.37225486985472,2.2842712945669,58.412412126243));
#198041=CARTESIAN_POINT('Ctrl Pts',(6.3103942538806,2.44998904347843,58.4207093280254));
#198042=CARTESIAN_POINT('Ctrl Pts',(6.2421522933486,2.61301047580045,58.4290065298079));
#198043=CARTESIAN_POINT('Ctrl Pts',(6.17390216699228,2.77605141524631,58.4373047244324));
#198044=CARTESIAN_POINT('Ctrl Pts',(6.09926930941793,2.93639507453469,58.445602919057));
#198045=CARTESIAN_POINT('Ctrl Pts',(6.01850372995083,3.09352579633143,58.4539011136815));
#198046=CARTESIAN_POINT('Ctrl Pts',(5.93768134711018,3.25076702999653,58.4622051445231));
#198047=CARTESIAN_POINT('Ctrl Pts',(5.85071778296393,3.4047905010508,58.4705091753646));
#198048=CARTESIAN_POINT('Ctrl Pts',(5.75790906763323,3.55510508548862,58.4788132062062));
#198049=CARTESIAN_POINT('Ctrl Pts',(5.66506660449923,3.70547432844651,58.4871202566219));
#198050=CARTESIAN_POINT('Ctrl Pts',(5.56637494291118,3.8521317046498,58.4954273070377));
#198051=CARTESIAN_POINT('Ctrl Pts',(5.46217312977042,3.99461558856594,58.5037343574534));
#198052=CARTESIAN_POINT('Ctrl Pts',(5.35785990730502,4.13725181180134,58.5120502895081));
#198053=CARTESIAN_POINT('Ctrl Pts',(5.24802497389089,4.27570535068261,58.5203662215627));
#198054=CARTESIAN_POINT('Ctrl Pts',(5.13304799000972,4.40954729334625,58.5286821536173));
#198055=CARTESIAN_POINT('Ctrl Pts',(5.04637589737093,4.51044019261978,58.5349508798361));
#198056=CARTESIAN_POINT('Ctrl Pts',(4.95678269050299,4.60871324893425,58.541219606055));
#198057=CARTESIAN_POINT('Ctrl Pts',(4.86444455754876,4.70419686519753,58.5474883322738));
#198058=CARTESIAN_POINT('Ctrl Pts',(4.73683470814911,4.83615372312458,58.5561516134461));
#198059=CARTESIAN_POINT('Ctrl Pts',(4.60374100709286,4.96302963095883,58.5648148946185));
#198060=CARTESIAN_POINT('Ctrl Pts',(4.46559664161901,5.08436187090977,58.5734781757908));
#198061=CARTESIAN_POINT('Ctrl Pts',(4.3309786271445,5.20259691566106,58.581920313161));
#198062=CARTESIAN_POINT('Ctrl Pts',(4.19156490220754,5.31556759914414,58.5903624505313));
#198063=CARTESIAN_POINT('Ctrl Pts',(4.04779465364802,5.42288183919754,58.5988045879015));
#198064=CARTESIAN_POINT('Ctrl Pts',(3.89837526115711,5.53441276242443,58.6075784409749));
#198065=CARTESIAN_POINT('Ctrl Pts',(3.74425028870485,5.63983344997825,58.6163522940483));
#198066=CARTESIAN_POINT('Ctrl Pts',(3.58595203971155,5.73874872850246,58.6251261471217));
#198067=CARTESIAN_POINT('Ctrl Pts',(3.42765379071826,5.83766400702666,58.6339000001951));
#198068=CARTESIAN_POINT('Ctrl Pts',(3.26518258774288,5.93007363277307,58.6426738532685));
#198069=CARTESIAN_POINT('Ctrl Pts',(3.0991061983213,6.01563211736942,58.6514477063419));
#198070=CARTESIAN_POINT('Origin',(0.,0.,4.30282021618968));
#198071=CARTESIAN_POINT('',(3.09910619832126,6.01563211736944,61.0457854935189));
#198072=CARTESIAN_POINT('',(3.09910619832132,6.01563211736941,60.6513956954041));
#198073=CARTESIAN_POINT('',(3.09910619832133,6.0156321173694,4.30282021618968));
#198074=CARTESIAN_POINT('',(-6.76699745956572,-0.00415705027770917,59.69717978381));
#198075=CARTESIAN_POINT('Ctrl Pts',(-6.76699494557931,-0.00827082245302645,
59.69717978381));
#198076=CARTESIAN_POINT('Ctrl Pts',(-6.76674793991816,-0.210365120819723,
59.7066512595226));
#198077=CARTESIAN_POINT('Ctrl Pts',(-6.75744417315915,-0.412020284934577,
59.7161227352352));
#198078=CARTESIAN_POINT('Ctrl Pts',(-6.73922359742326,-0.612498411372184,
59.7255942109478));
#198079=CARTESIAN_POINT('Ctrl Pts',(-6.72088520849356,-0.814272817834613,
59.7351269286771));
#198080=CARTESIAN_POINT('Ctrl Pts',(-6.69351444453166,-1.01485482244309,
59.7446596464064));
#198081=CARTESIAN_POINT('Ctrl Pts',(-6.65730215415095,-1.21351432967937,
59.7541923641357));
#198082=CARTESIAN_POINT('Ctrl Pts',(-6.62079334179662,-1.41380054730992,
59.7638031399013));
#198083=CARTESIAN_POINT('Ctrl Pts',(-6.57529770100836,-1.61213256130308,
59.7734139156668));
#198084=CARTESIAN_POINT('Ctrl Pts',(-6.52105806976313,-1.80778611864821,
59.7830246914324));
#198085=CARTESIAN_POINT('Ctrl Pts',(-6.49956088822673,-1.88533089437641,
59.7868337990276));
#198086=CARTESIAN_POINT('Ctrl Pts',(-6.47669068445561,-1.96245519968619,
59.7906429066228));
#198087=CARTESIAN_POINT('Ctrl Pts',(-6.45246456311846,-2.03911501924253,
59.794452014218));
#198088=CARTESIAN_POINT('Ctrl Pts',(-6.3994667478689,-2.20681842076402,
59.8027849362647));
#198089=CARTESIAN_POINT('Ctrl Pts',(-6.33985870359495,-2.37266971007358,
59.8111178583114));
#198090=CARTESIAN_POINT('Ctrl Pts',(-6.27378626625729,-2.53611807401024,
59.8194507803581));
#198091=CARTESIAN_POINT('Ctrl Pts',(-6.20779191051785,-2.69937328161732,
59.8277738549118));
#198092=CARTESIAN_POINT('Ctrl Pts',(-6.13534850917667,-2.8602309008722,
59.8360969294654));
#198093=CARTESIAN_POINT('Ctrl Pts',(-6.05665176517554,-3.01815479977354,
59.844420004019));
#198094=CARTESIAN_POINT('Ctrl Pts',(-5.97803357640252,-3.17592105876156,
59.852734770465));
#198095=CARTESIAN_POINT('Ctrl Pts',(-5.89317463545723,-3.33075912231229,
59.8610495369109));
#198096=CARTESIAN_POINT('Ctrl Pts',(-5.80231894786804,-3.48215218323547,
59.8693643033569));
#198097=CARTESIAN_POINT('Ctrl Pts',(-5.7115372865945,-3.63342189392255,
59.8776722951964));
#198098=CARTESIAN_POINT('Ctrl Pts',(-5.61476879262656,-3.7812518978611,
59.885980287036));
#198099=CARTESIAN_POINT('Ctrl Pts',(-5.5123037719867,-3.92514918510637,
59.8942882788755));
#198100=CARTESIAN_POINT('Ctrl Pts',(-5.40990345129323,-4.06895561064379,
59.9025910247626));
#198101=CARTESIAN_POINT('Ctrl Pts',(-5.30181397354251,-4.2088339856821,
59.9108937706497));
#198102=CARTESIAN_POINT('Ctrl Pts',(-5.18836952418654,-4.34431935756251,
59.9191965165367));
#198103=CARTESIAN_POINT('Ctrl Pts',(-5.07497143596165,-4.47974936088924,
59.9274958693562));
#198104=CARTESIAN_POINT('Ctrl Pts',(-4.95622295970471,-4.61078967194648,
59.9357952221756));
#198105=CARTESIAN_POINT('Ctrl Pts',(-4.83249938808486,-4.73700735318824,
59.944094574995));
#198106=CARTESIAN_POINT('Ctrl Pts',(-4.70880213039263,-4.86319819004711,
59.9523921626814));
#198107=CARTESIAN_POINT('Ctrl Pts',(-4.58013212874796,-4.98456819219664,
59.9606897503678));
#198108=CARTESIAN_POINT('Ctrl Pts',(-4.44690262161451,-5.10072015247631,
59.9689873380541));
#198109=CARTESIAN_POINT('Ctrl Pts',(-4.31367931071456,-5.21686671076447,
59.9772845398365));
#198110=CARTESIAN_POINT('Ctrl Pts',(-4.17589717921879,-5.32779548229528,
59.985581741619));
#198111=CARTESIAN_POINT('Ctrl Pts',(-4.0340038712678,-5.43314842118237,
59.9938789434014));
#198112=CARTESIAN_POINT('Ctrl Pts',(-3.89209358438091,-5.53851396658925,
60.0021771380259));
#198113=CARTESIAN_POINT('Ctrl Pts',(-3.7460714204525,-5.63830214297072,
60.0104753326505));
#198114=CARTESIAN_POINT('Ctrl Pts',(-3.59641557339867,-5.73219713752201,
60.0187735272751));
#198115=CARTESIAN_POINT('Ctrl Pts',(-3.44665447164329,-5.82615816951737,
60.0270775581167));
#198116=CARTESIAN_POINT('Ctrl Pts',(-3.29325487521143,-5.91421755254508,
60.0353815889583));
#198117=CARTESIAN_POINT('Ctrl Pts',(-3.13672202977063,-5.99610406080078,
60.0436856197998));
#198118=CARTESIAN_POINT('Ctrl Pts',(-2.98013226467893,-6.07802034524468,
60.0519926702156));
#198119=CARTESIAN_POINT('Ctrl Pts',(-2.8204072913917,-6.15375912639602,
60.0602997206313));
#198120=CARTESIAN_POINT('Ctrl Pts',(-2.65807428976598,-6.22309650174936,
60.0686067710471));
#198121=CARTESIAN_POINT('Ctrl Pts',(-2.49556772676425,-6.29250801045916,
60.0769227031017));
#198122=CARTESIAN_POINT('Ctrl Pts',(-2.3304478871435,-6.35550430868761,
60.0852386351563));
#198123=CARTESIAN_POINT('Ctrl Pts',(-2.16326017726427,-6.4119103553826,
60.093554567211));
#198124=CARTESIAN_POINT('Ctrl Pts',(-2.03723053037763,-6.45443043148374,
60.0998232934297));
#198125=CARTESIAN_POINT('Ctrl Pts',(-1.9100261967052,-6.49320663306443,
60.1060920196485));
#198126=CARTESIAN_POINT('Ctrl Pts',(-1.78188525111659,-6.52818305134385,
60.1123607458673));
#198127=CARTESIAN_POINT('Ctrl Pts',(-1.60915072947773,-6.57533140702662,
60.1208110145907));
#198128=CARTESIAN_POINT('Ctrl Pts',(-1.43439713546218,-6.61565982502612,
60.129261283314));
#198129=CARTESIAN_POINT('Ctrl Pts',(-1.25818914927755,-6.64900361442526,
60.1377115520374));
#198130=CARTESIAN_POINT('Ctrl Pts',(-1.08213667261888,-6.68231797679902,
60.1461543631119));
#198131=CARTESIAN_POINT('Ctrl Pts',(-0.904632686421212,-6.70865993551441,
60.1545971741864));
#198132=CARTESIAN_POINT('Ctrl Pts',(-0.726254821983576,-6.7279151996399,
60.1630399852609));
#198133=CARTESIAN_POINT('Ctrl Pts',(-0.548010095458443,-6.74715609199523,
60.1714764947786));
#198134=CARTESIAN_POINT('Ctrl Pts',(-0.368893119497846,-6.75932079836543,
60.1799130042963));
#198135=CARTESIAN_POINT('Ctrl Pts',(-0.1894898534267,-6.76434642781166,
60.188349513814));
#198136=CARTESIAN_POINT('Ctrl Pts',(-0.0102149600456931,-6.7693684611496,
60.1967799865552));
#198137=CARTESIAN_POINT('Ctrl Pts',(0.169345484178861,-6.76726159781441,
60.2052104592965));
#198138=CARTESIAN_POINT('Ctrl Pts',(0.348602074366175,-6.75801491517647,
60.2136409320377));
#198139=CARTESIAN_POINT('Ctrl Pts',(0.527781602631672,-6.74877220766231,
60.2220677805415));
#198140=CARTESIAN_POINT('Ctrl Pts',(0.706657206732951,-6.73239581682857,
60.2304946290454));
#198141=CARTESIAN_POINT('Ctrl Pts',(0.884640499077104,-6.70892690282079,
60.2389214775492));
#198142=CARTESIAN_POINT('Ctrl Pts',(1.06256885433471,-6.6854652328287,60.2473457249859));
#198143=CARTESIAN_POINT('Ctrl Pts',(1.23960511874426,-6.65491544875998,
60.2557699724225));
#198144=CARTESIAN_POINT('Ctrl Pts',(1.41516666697177,-6.61737049776511,
60.2641942198592));
#198145=CARTESIAN_POINT('Ctrl Pts',(1.4646331941756,-6.60679176706636,60.2665678504702));
#198146=CARTESIAN_POINT('Ctrl Pts',(1.51398269264356,-6.59565800615915,
60.2689414810813));
#198147=CARTESIAN_POINT('Ctrl Pts',(1.5632022599082,-6.5839720302123,60.2713151116923));
#198148=CARTESIAN_POINT('Ctrl Pts',(1.74192116676137,-6.54153962044519,
60.2799338926296));
#198149=CARTESIAN_POINT('Ctrl Pts',(1.91884610224507,-6.4918416236436,60.2885526735668));
#198150=CARTESIAN_POINT('Ctrl Pts',(2.09338843199052,-6.43506129518657,
60.2971714545041));
#198151=CARTESIAN_POINT('Ctrl Pts',(2.26803560825225,-6.37824685913146,
60.3057954126907));
#198152=CARTESIAN_POINT('Ctrl Pts',(2.44029703324883,-6.31434169519958,
60.3144193708772));
#198153=CARTESIAN_POINT('Ctrl Pts',(2.60960195902574,-6.24357802989993,
60.3230433290638));
#198154=CARTESIAN_POINT('Ctrl Pts',(2.78502329410652,-6.17025791481696,
60.3319788414349));
#198155=CARTESIAN_POINT('Ctrl Pts',(2.95727019985895,-6.08957465562102,
60.340914353806));
#198156=CARTESIAN_POINT('Ctrl Pts',(3.12573397915408,-6.00183939234978,
60.3498498661771));
#198157=CARTESIAN_POINT('Ctrl Pts',(3.28862792288728,-5.9170048771886,60.3584899480718));
#198158=CARTESIAN_POINT('Ctrl Pts',(3.44798465443273,-5.82557740016303,
60.3671300299665));
#198159=CARTESIAN_POINT('Ctrl Pts',(3.60328161292256,-5.72788360723,60.3757701118613));
#198160=CARTESIAN_POINT('Ctrl Pts',(3.76654367897481,-5.62517914585595,
60.3848533394706));
#198161=CARTESIAN_POINT('Ctrl Pts',(3.92531826187956,-5.51554891529997,
60.3939365670799));
#198162=CARTESIAN_POINT('Ctrl Pts',(4.07903519798477,-5.39942227035461,
60.4030197946892));
#198163=CARTESIAN_POINT('Ctrl Pts',(4.23275213408994,-5.28329562540929,
60.4121030222984));
#198164=CARTESIAN_POINT('Ctrl Pts',(4.38141114567018,-5.16067283878569,
60.4211862499077));
#198165=CARTESIAN_POINT('Ctrl Pts',(4.52448428868086,-5.032030496875,60.430269477517));
#198166=CARTESIAN_POINT('Ctrl Pts',(4.66694891353778,-4.90393529608911,
60.4393140723768));
#198167=CARTESIAN_POINT('Ctrl Pts',(4.8040072327267,-4.76975399487583,60.4483586672366));
#198168=CARTESIAN_POINT('Ctrl Pts',(4.93516874599835,-4.62994583645652,
60.4574032620964));
#198169=CARTESIAN_POINT('Ctrl Pts',(5.06620989793573,-4.49026597402946,
60.4664395571167));
#198170=CARTESIAN_POINT('Ctrl Pts',(5.19136488491325,-4.34496973675022,
60.475475852137));
#198171=CARTESIAN_POINT('Ctrl Pts',(5.31018039595455,-4.19455279647545,
60.4845121471573));
#198172=CARTESIAN_POINT('Ctrl Pts',(5.42878565363185,-4.0444020307718,60.493532451745));
#198173=CARTESIAN_POINT('Ctrl Pts',(5.54107368942041,-3.88914884314024,
60.5025527563327));
#198174=CARTESIAN_POINT('Ctrl Pts',(5.64663185528263,-3.72932134454882,
60.5115730609204));
#198175=CARTESIAN_POINT('Ctrl Pts',(5.7520570911402,-3.56969511764452,60.5205820061867));
#198176=CARTESIAN_POINT('Ctrl Pts',(5.85076923947305,-3.4055062735836,60.5295909514529));
#198177=CARTESIAN_POINT('Ctrl Pts',(5.94239780336344,-3.23731329138552,
60.5385998967192));
#198178=CARTESIAN_POINT('Ctrl Pts',(6.03381829818286,-3.06950223984383,
60.547588384578));
#198179=CARTESIAN_POINT('Ctrl Pts',(6.11818720265059,-2.89770540819866,
60.5565768724368));
#198180=CARTESIAN_POINT('Ctrl Pts',(6.19517918465154,-2.72250690909321,
60.5655653602955));
#198181=CARTESIAN_POINT('Ctrl Pts',(6.26272905249322,-2.5687943386013,60.573451521311));
#198182=CARTESIAN_POINT('Ctrl Pts',(6.32460099297568,-2.41246380110435,
60.5813376823264));
#198183=CARTESIAN_POINT('Ctrl Pts',(6.38060368627001,-2.25392670660728,
60.5892238433418));
#198184=CARTESIAN_POINT('Ctrl Pts',(6.43827736355753,-2.09065925127133,
60.597345308198));
#198185=CARTESIAN_POINT('Ctrl Pts',(6.48969896103663,-1.92512413876695,
60.6054667730541));
#198186=CARTESIAN_POINT('Ctrl Pts',(6.53469692774071,-1.75784671191094,
60.6135882379103));
#198187=CARTESIAN_POINT('Ctrl Pts',(6.57969168542751,-1.5905812143974,60.6217091235865));
#198188=CARTESIAN_POINT('Ctrl Pts',(6.6182636296851,-1.42157400364193,60.6298300092627));
#198189=CARTESIAN_POINT('Ctrl Pts',(6.65029144888128,-1.25136431343414,
60.6379508949389));
#198190=CARTESIAN_POINT('Ctrl Pts',(6.68232309631771,-1.08113427830118,
60.6460727512932));
#198191=CARTESIAN_POINT('Ctrl Pts',(6.70780899459909,-0.90970183760193,
60.6541946076474));
#198192=CARTESIAN_POINT('Ctrl Pts',(6.72667919659345,-0.737615066357041,
60.6623164640017));
#198193=CARTESIAN_POINT('Ctrl Pts',(6.74556316605373,-0.565402742732858,
60.6704442459619));
#198194=CARTESIAN_POINT('Ctrl Pts',(6.7578217589761,-0.392535499461082,
60.678572027922));
#198195=CARTESIAN_POINT('Ctrl Pts',(6.76343698538826,-0.219565809456372,
60.6866998098822));
#198196=CARTESIAN_POINT('Ctrl Pts',(6.76905449923494,-0.0465256580289172,
60.6948309027986));
#198197=CARTESIAN_POINT('Ctrl Pts',(6.76802325441362,0.126616657394339,
60.7029619957151));
#198198=CARTESIAN_POINT('Ctrl Pts',(6.76037738222586,0.299310290316055,
60.7110930886316));
#198199=CARTESIAN_POINT('Ctrl Pts',(6.75272316488814,0.472192411120845,
60.7192330562961));
#198200=CARTESIAN_POINT('Ctrl Pts',(6.73843993045061,0.644624506798774,
60.7273730239606));
#198201=CARTESIAN_POINT('Ctrl Pts',(6.71761358568088,0.816061709355177,
60.7355129916252));
#198202=CARTESIAN_POINT('Ctrl Pts',(6.70681214280997,0.90497645506959,60.7397347308056));
#198203=CARTESIAN_POINT('Ctrl Pts',(6.69425150488015,0.993623744972743,
60.7439564699861));
#198204=CARTESIAN_POINT('Ctrl Pts',(6.67994901988375,1.08192887555241,60.7481782091665));
#198205=CARTESIAN_POINT('Ctrl Pts',(6.65135441875996,1.25847511816318,60.7566186268942));
#198206=CARTESIAN_POINT('Ctrl Pts',(6.61573536456724,1.43401789943923,60.7650590446218));
#198207=CARTESIAN_POINT('Ctrl Pts',(6.57318024761848,1.60797712431437,60.7734994623495));
#198208=CARTESIAN_POINT('Ctrl Pts',(6.53065765213538,1.78180340609445,60.7819334297423));
#198209=CARTESIAN_POINT('Ctrl Pts',(6.48120963969021,1.95404822115737,60.7903673971351));
#198210=CARTESIAN_POINT('Ctrl Pts',(6.4249757583338,2.12414112168259,60.7988013645279));
#198211=CARTESIAN_POINT('Ctrl Pts',(6.36877620683777,2.29413018328751,60.8072301831222));
#198212=CARTESIAN_POINT('Ctrl Pts',(6.30579915012798,2.46196963365099,60.8156590017165));
#198213=CARTESIAN_POINT('Ctrl Pts',(6.23623422950004,2.6271032782919,60.8240878203108));
#198214=CARTESIAN_POINT('Ctrl Pts',(6.16670109436923,2.79216147032049,60.8325127876222));
#198215=CARTESIAN_POINT('Ctrl Pts',(6.0905862266872,2.95451601501969,60.8409377549336));
#198216=CARTESIAN_POINT('Ctrl Pts',(6.00812787707466,3.11362945976529,60.849362722245));
#198217=CARTESIAN_POINT('Ctrl Pts',(5.92568748457082,3.27270825407906,60.8577858548356));
#198218=CARTESIAN_POINT('Ctrl Pts',(5.83690651507366,3.42854705848998,60.8662089874261));
#198219=CARTESIAN_POINT('Ctrl Pts',(5.74207001323417,3.58063136375653,60.8746321200167));
#198220=CARTESIAN_POINT('Ctrl Pts',(5.64724439076035,3.73269822235713,60.8830542863302));
#198221=CARTESIAN_POINT('Ctrl Pts',(5.54636479713171,3.88101115746608,60.8914764526436));
#198222=CARTESIAN_POINT('Ctrl Pts',(5.43976076561801,4.0250828330412,60.8998986189571));
#198223=CARTESIAN_POINT('Ctrl Pts',(5.33315408214735,4.16915809264479,60.9083209947863));
#198224=CARTESIAN_POINT('Ctrl Pts',(5.2208228754521,4.3089916144373,60.9167433706155));
#198225=CARTESIAN_POINT('Ctrl Pts',(5.10313850903089,4.44412717613324,60.9251657464447));
#198226=CARTESIAN_POINT('Ctrl Pts',(4.98543478604954,4.57928496473754,60.9335895075745));
#198227=CARTESIAN_POINT('Ctrl Pts',(4.86237636728863,4.7097430015437,60.9420132687043));
#198228=CARTESIAN_POINT('Ctrl Pts',(4.73437343314789,4.83507985409791,60.9504370298341));
#198229=CARTESIAN_POINT('Ctrl Pts',(4.60628018313717,4.96050514139743,60.9588667345723));
#198230=CARTESIAN_POINT('Ctrl Pts',(4.4732356842172,5.08080178964516,60.9672964393106));
#198231=CARTESIAN_POINT('Ctrl Pts',(4.33568613525387,5.1955860821054,60.9757261440488));
#198232=CARTESIAN_POINT('Ctrl Pts',(4.19808791635887,5.31041098933838,60.9841588315169));
#198233=CARTESIAN_POINT('Ctrl Pts',(4.05598172897378,5.41971944265584,60.992591518985));
#198234=CARTESIAN_POINT('Ctrl Pts',(3.90984552507733,5.52316910568858,61.0010242064531));
#198235=CARTESIAN_POINT('Ctrl Pts',(3.76356343867773,5.62672203878986,61.0094653119691));
#198236=CARTESIAN_POINT('Ctrl Pts',(3.61324357220252,5.72440430589957,61.0179064174851));
#198237=CARTESIAN_POINT('Ctrl Pts',(3.45939246949101,5.81591718837441,61.026347523001));
#198238=CARTESIAN_POINT('Ctrl Pts',(3.34129762227779,5.88616172795481,61.032826846507));
#198239=CARTESIAN_POINT('Ctrl Pts',(3.22112276878836,5.95277217140621,61.039306170013));
#198240=CARTESIAN_POINT('Ctrl Pts',(3.09910619832126,6.01563211736944,61.0457854935189));
#198241=CARTESIAN_POINT('Ctrl Pts',(3.09910619832129,6.01563211736943,59.0457552630241));
#198242=CARTESIAN_POINT('Ctrl Pts',(2.93375330764824,6.10081787314654,59.0545047109264));
#198243=CARTESIAN_POINT('Ctrl Pts',(2.76488627843071,6.17918207037038,59.0632541588287));
#198244=CARTESIAN_POINT('Ctrl Pts',(2.59307866646706,6.25045854553995,59.072003606731));
#198245=CARTESIAN_POINT('Ctrl Pts',(2.42127244185373,6.32173444515039,59.0807529839813));
#198246=CARTESIAN_POINT('Ctrl Pts',(2.24652594672453,6.38592262741843,59.0895023612316));
#198247=CARTESIAN_POINT('Ctrl Pts',(2.06943269687101,6.44280508110568,59.0982517384819));
#198248=CARTESIAN_POINT('Ctrl Pts',(1.89234081822054,6.49968709436173,59.1070010479873));
#198249=CARTESIAN_POINT('Ctrl Pts',(1.71290249405563,6.54926340459551,59.1157503574927));
#198250=CARTESIAN_POINT('Ctrl Pts',(1.53172716625031,6.5913656315039,59.124499666998));
#198251=CARTESIAN_POINT('Ctrl Pts',(1.35055318107301,6.63346754640717,59.1332489116653));
#198252=CARTESIAN_POINT('Ctrl Pts',(1.16764249714382,6.66809542395783,59.1419981563325));
#198253=CARTESIAN_POINT('Ctrl Pts',(0.98361634061393,6.69513165624674,59.1507474009997));
#198254=CARTESIAN_POINT('Ctrl Pts',(0.799591486713385,6.72216769715966,
59.1594965837354));
#198255=CARTESIAN_POINT('Ctrl Pts',(0.614451459526225,6.74161215869375,
59.1682457664711));
#198256=CARTESIAN_POINT('Ctrl Pts',(0.428825047909765,6.75339900185715,
59.1769949492068));
#198257=CARTESIAN_POINT('Ctrl Pts',(0.243199888596534,6.76518576550223,
59.1857440729174));
#198258=CARTESIAN_POINT('Ctrl Pts',(0.0570886373914115,6.76931499599835,
59.1944931966279));
#198259=CARTESIAN_POINT('Ctrl Pts',(-0.128876626811648,6.76577266947846,
59.2032423203384));
#198260=CARTESIAN_POINT('Ctrl Pts',(-0.314840698188693,6.76223036567991,
59.21199138793));
#198261=CARTESIAN_POINT('Ctrl Pts',(-0.500658497951821,6.75101660879219,
59.2207404555215));
#198262=CARTESIAN_POINT('Ctrl Pts',(-0.685698951926819,6.73216948296212,
59.2294895231131));
#198263=CARTESIAN_POINT('Ctrl Pts',(-0.870738280460326,6.71332247176287,
59.2382385374916));
#198264=CARTESIAN_POINT('Ctrl Pts',(-1.05499998761285,6.68684221356181,
59.2469875518701));
#198265=CARTESIAN_POINT('Ctrl Pts',(-1.23785829161442,6.65281863948518,
59.2557365662486));
#198266=CARTESIAN_POINT('Ctrl Pts',(-1.43007412917425,6.61705395368857,
59.2649332999478));
#198267=CARTESIAN_POINT('Ctrl Pts',(-1.62073882535812,6.57295372727785,
59.274130033647));
#198268=CARTESIAN_POINT('Ctrl Pts',(-1.80913696091533,6.52068343478274,
59.2833267673462));
#198269=CARTESIAN_POINT('Ctrl Pts',(-1.98838356186122,6.47095219815195,
59.2920767650599));
#198270=CARTESIAN_POINT('Ctrl Pts',(-2.16557827572533,6.4138258685089,59.3008267627735));
#198271=CARTESIAN_POINT('Ctrl Pts',(-2.34011918621691,6.34949849943281,
59.3095767604872));
#198272=CARTESIAN_POINT('Ctrl Pts',(-2.51465655691092,6.28517243495553,
59.3183265807455));
#198273=CARTESIAN_POINT('Ctrl Pts',(-2.68653996295324,6.21364572242376,
59.3270764010038));
#198274=CARTESIAN_POINT('Ctrl Pts',(-2.85518555379986,6.13516132252222,
59.3358262212621));
#198275=CARTESIAN_POINT('Ctrl Pts',(-3.02382794858685,6.05667841000508,
59.3445758756996));
#198276=CARTESIAN_POINT('Ctrl Pts',(-3.18923239109276,5.97123819492084,
59.3533255301371));
#198277=CARTESIAN_POINT('Ctrl Pts',(-3.35083705967692,5.87913088810717,
59.3620751845746));
#198278=CARTESIAN_POINT('Ctrl Pts',(-3.51243888042386,5.78702520443111,
59.3708246848236));
#198279=CARTESIAN_POINT('Ctrl Pts',(-3.67024081223669,5.68825280605797,
59.3795741850725));
#198280=CARTESIAN_POINT('Ctrl Pts',(-3.82370687544374,5.58314917682524,
59.3883236853215));
#198281=CARTESIAN_POINT('Ctrl Pts',(-3.97717043817797,5.47804726008034,
59.3970730430119));
#198282=CARTESIAN_POINT('Ctrl Pts',(-4.12629803722453,5.36661448084242,
59.4058224007024));
#198283=CARTESIAN_POINT('Ctrl Pts',(-4.27058317206909,5.24922931204575,
59.4145717583929));
#198284=CARTESIAN_POINT('Ctrl Pts',(-4.41486614774827,5.13184589986797,
59.423320985153));
#198285=CARTESIAN_POINT('Ctrl Pts',(-4.55430658194398,5.00851045723048,
59.432070211913));
#198286=CARTESIAN_POINT('Ctrl Pts',(-4.68843089001822,4.87964187103142,
59.4408194386731));
#198287=CARTESIAN_POINT('Ctrl Pts',(-4.82255336917814,4.75077504207983,
59.449568546129));
#198288=CARTESIAN_POINT('Ctrl Pts',(-4.95135966065113,4.61637541908117,
59.4583176535849));
#198289=CARTESIAN_POINT('Ctrl Pts',(-5.07441230869223,4.47689945401868,
59.4670667610409));
#198290=CARTESIAN_POINT('Ctrl Pts',(-5.197463442264,4.33742520555536,59.4758157608172));
#198291=CARTESIAN_POINT('Ctrl Pts',(-5.31476088454755,4.19287495491353,
59.4845647605936));
#198292=CARTESIAN_POINT('Ctrl Pts',(-5.42590627628845,4.04373961586718,
59.49331376037));
#198293=CARTESIAN_POINT('Ctrl Pts',(-5.53706380672659,3.89458798906747,
59.5020637156647));
#198294=CARTESIAN_POINT('Ctrl Pts',(-5.64206777071855,3.74085050155298,
59.5108136709594));
#198295=CARTESIAN_POINT('Ctrl Pts',(-5.74056148163998,3.58304938223176,
59.5195636262541));
#198296=CARTESIAN_POINT('Ctrl Pts',(-5.83905138951869,3.42525435593306,
59.5283132436952));
#198297=CARTESIAN_POINT('Ctrl Pts',(-5.93103139557634,3.26339625497216,
59.5370628611363));
#198298=CARTESIAN_POINT('Ctrl Pts',(-6.01618907820825,3.09802485065046,
59.5458124785774));
#198299=CARTESIAN_POINT('Ctrl Pts',(-6.10134392544956,2.93265895249697,
59.5545618046932));
#198300=CARTESIAN_POINT('Ctrl Pts',(-6.179676772618,2.76378023986106,59.5633111308091));
#198301=CARTESIAN_POINT('Ctrl Pts',(-6.25092157009188,2.59196229227202,
59.572060456925));
#198302=CARTESIAN_POINT('Ctrl Pts',(-6.32216437407723,2.42014915229171,
59.5808095382274));
#198303=CARTESIAN_POINT('Ctrl Pts',(-6.38631941548896,2.24539720662924,
59.5895586195299));
#198304=CARTESIAN_POINT('Ctrl Pts',(-6.44316881037516,2.06829994947753,
59.5983077008323));
#198305=CARTESIAN_POINT('Ctrl Pts',(-6.50002334524549,1.89118668024526,
59.6070575731747));
#198306=CARTESIAN_POINT('Ctrl Pts',(-6.54957082411074,1.71172794807788,
59.615807445517));
#198307=CARTESIAN_POINT('Ctrl Pts',(-6.59164294296062,1.53053334250435,
59.6245573178594));
#198308=CARTESIAN_POINT('Ctrl Pts',(-6.6337121408212,1.34935131693673,59.6333065827143));
#198309=CARTESIAN_POINT('Ctrl Pts',(-6.66830695239682,1.16643393829814,
59.6420558475692));
#198310=CARTESIAN_POINT('Ctrl Pts',(-6.69530988153984,0.982402458341267,
59.6508051124241));
#198311=CARTESIAN_POINT('Ctrl Pts',(-6.72231419690479,0.798361530947385,
59.6595548264311));
#198312=CARTESIAN_POINT('Ctrl Pts',(-6.74172580829274,0.613206671362852,
59.6683045404382));
#198313=CARTESIAN_POINT('Ctrl Pts',(-6.75347878028177,0.427566795113822,
59.6770542544452));
#198314=CARTESIAN_POINT('Ctrl Pts',(-6.76248992368215,0.285234494205521,
59.6837627642335));
#198315=CARTESIAN_POINT('Ctrl Pts',(-6.76699999999997,0.142617266092203,
59.6904712740217));
#198316=CARTESIAN_POINT('Ctrl Pts',(-6.767,1.33634611793382E-12,59.69717978381));
#198317=CARTESIAN_POINT('',(-6.767,1.48494633473231E-12,59.3028202161899));
#198318=CARTESIAN_POINT('Ctrl Pts',(3.0991061983213,6.01563211736942,58.6514477063419));
#198319=CARTESIAN_POINT('Ctrl Pts',(2.93960420746614,6.09780363299062,58.6598742324576));
#198320=CARTESIAN_POINT('Ctrl Pts',(2.77677729812525,6.17365583256632,58.6683007585734));
#198321=CARTESIAN_POINT('Ctrl Pts',(2.6111549264028,6.24292871578095,58.6767272846892));
#198322=CARTESIAN_POINT('Ctrl Pts',(2.44558185079483,6.31218098050096,58.6851513027199));
#198323=CARTESIAN_POINT('Ctrl Pts',(2.27721527777857,6.37485770660371,58.6935753207507));
#198324=CARTESIAN_POINT('Ctrl Pts',(2.10660567906555,6.43074657508199,58.7019993387814));
#198325=CARTESIAN_POINT('Ctrl Pts',(2.07660891871999,6.44057301513211,58.7034804585538));
#198326=CARTESIAN_POINT('Ctrl Pts',(2.04654286662022,6.45018974321123,58.7049615783262));
#198327=CARTESIAN_POINT('Ctrl Pts',(2.01641057233741,6.45959576163756,58.7064426980986));
#198328=CARTESIAN_POINT('Ctrl Pts',(1.8410678023596,6.51433030358304,58.7150614790358));
#198329=CARTESIAN_POINT('Ctrl Pts',(1.66355914988804,6.56190132396065,58.7236802599731));
#198330=CARTESIAN_POINT('Ctrl Pts',(1.48448433243295,6.60216595268258,58.7322990409103));
#198331=CARTESIAN_POINT('Ctrl Pts',(1.30530194582427,6.64245476812208,58.7409229990969));
#198332=CARTESIAN_POINT('Ctrl Pts',(1.12455181347335,6.6754283662573,58.7495469572834));
#198333=CARTESIAN_POINT('Ctrl Pts',(0.942843268204863,6.70099511801052,
58.75817091547));
#198334=CARTESIAN_POINT('Ctrl Pts',(0.754570213180525,6.7274855092715,58.7671064278411));
#198335=CARTESIAN_POINT('Ctrl Pts',(0.565268564308852,6.74602386384453,
58.7760419402122));
#198336=CARTESIAN_POINT('Ctrl Pts',(0.375620567336058,6.75656704173015,
58.7849774525833));
#198337=CARTESIAN_POINT('Ctrl Pts',(0.192242809356957,6.76676163568053,
58.7936175344779));
#198338=CARTESIAN_POINT('Ctrl Pts',(0.00854154427682233,6.76948131428951,
58.8022576163726));
#198339=CARTESIAN_POINT('Ctrl Pts',(-0.174867137869492,6.76474023773961,
58.8108976982673));
#198340=CARTESIAN_POINT('Ctrl Pts',(-0.367682764592293,6.75975599361543,
58.8199809258766));
#198341=CARTESIAN_POINT('Ctrl Pts',(-0.560174614704952,6.74652560175623,
58.829064153486));
#198342=CARTESIAN_POINT('Ctrl Pts',(-0.751633238131505,6.72512724603304,
58.8381473810953));
#198343=CARTESIAN_POINT('Ctrl Pts',(-0.943091861558059,6.70372889030986,
58.8472306087046));
#198344=CARTESIAN_POINT('Ctrl Pts',(-1.13351688027741,6.67416266347395,
58.8563138363139));
#198345=CARTESIAN_POINT('Ctrl Pts',(-1.32221104142195,6.63656891487928,
58.8653970639232));
#198346=CARTESIAN_POINT('Ctrl Pts',(-1.51010264927044,6.59913505987465,
58.874441658783));
#198347=CARTESIAN_POINT('Ctrl Pts',(-1.69645177588442,6.5537081134136,58.8834862536429));
#198348=CARTESIAN_POINT('Ctrl Pts',(-1.88060221952506,6.50043262344265,
58.8925308485027));
#198349=CARTESIAN_POINT('Ctrl Pts',(-2.06458367614873,6.4472060221192,58.9015671435232));
#198350=CARTESIAN_POINT('Ctrl Pts',(-2.24637024969716,6.38614532271716,
58.9106034385436));
#198351=CARTESIAN_POINT('Ctrl Pts',(-2.42531912408078,6.31744538135219,
58.919639733564));
#198352=CARTESIAN_POINT('Ctrl Pts',(-2.60395133439687,6.24886700992134,
58.9286600381518));
#198353=CARTESIAN_POINT('Ctrl Pts',(-2.77975565110537,6.17267647587612,
58.9376803427395));
#198354=CARTESIAN_POINT('Ctrl Pts',(-2.95210766720634,6.08911728588156,
58.9467006473272));
#198355=CARTESIAN_POINT('Ctrl Pts',(-3.12424263942437,6.00566332245447,
58.9557095925936));
#198356=CARTESIAN_POINT('Ctrl Pts',(-3.29293377373124,5.91485932502222,
58.96471853786));
#198357=CARTESIAN_POINT('Ctrl Pts',(-3.45757740906046,5.81699642946038,
58.9737274831264));
#198358=CARTESIAN_POINT('Ctrl Pts',(-3.62184717354777,5.71935575981746,
58.9827159709853));
#198359=CARTESIAN_POINT('Ctrl Pts',(-3.7820875809945,5.61468830916453,58.9917044588441));
#198360=CARTESIAN_POINT('Ctrl Pts',(-3.93772072437835,5.50333030962173,
59.0006929467029));
#198361=CARTESIAN_POINT('Ctrl Pts',(-4.07426738798728,5.40562899116779,
59.008579107718));
#198362=CARTESIAN_POINT('Ctrl Pts',(-4.20726776641211,5.30277825801675,
59.0164652687331));
#198363=CARTESIAN_POINT('Ctrl Pts',(-4.33634734476151,5.19503423526542,
59.0243514297482));
#198364=CARTESIAN_POINT('Ctrl Pts',(-4.46927834340681,5.08407539324297,
59.0324728946044));
#198365=CARTESIAN_POINT('Ctrl Pts',(-4.59799052346479,4.96797531200298,
59.0405943594606));
#198366=CARTESIAN_POINT('Ctrl Pts',(-4.72206821525421,4.84709818040505,
59.0487158243168));
#198367=CARTESIAN_POINT('Ctrl Pts',(-4.84613705847835,4.72622966912536,
59.056836709993));
#198368=CARTESIAN_POINT('Ctrl Pts',(-4.9655718094636,4.60058504159022,59.0649575956692));
#198369=CARTESIAN_POINT('Ctrl Pts',(-5.0799929100406,4.47056607533512,59.0730784813454));
#198370=CARTESIAN_POINT('Ctrl Pts',(-5.19442768721103,4.34053156809562,
59.0812003376997));
#198371=CARTESIAN_POINT('Ctrl Pts',(-5.30384737966787,4.20612195669019,
59.089322194054));
#198372=CARTESIAN_POINT('Ctrl Pts',(-5.40791208583435,4.06777283926804,
59.0974440504083));
#198373=CARTESIAN_POINT('Ctrl Pts',(-5.51205271632277,3.92932278404173,
59.1055718323684));
#198374=CARTESIAN_POINT('Ctrl Pts',(-5.61083033696595,3.78692777515107,
59.1136996143286));
#198375=CARTESIAN_POINT('Ctrl Pts',(-5.70394748042142,3.64105371295098,
59.1218273962888));
#198376=CARTESIAN_POINT('Ctrl Pts',(-5.79710255633991,3.49512022708019,
59.1299584892052));
#198377=CARTESIAN_POINT('Ctrl Pts',(-5.88459237392545,3.34570517872564,
59.1380895821217));
#198378=CARTESIAN_POINT('Ctrl Pts',(-5.96616511616956,3.19329967378595,
59.1462206750381));
#198379=CARTESIAN_POINT('Ctrl Pts',(-6.04782689165323,3.04072782460603,
59.1543606427027));
#198380=CARTESIAN_POINT('Ctrl Pts',(-6.12355853245191,2.88515932847609,
59.1625006103673));
#198381=CARTESIAN_POINT('Ctrl Pts',(-6.19315579594797,2.72710657787994,
59.1706405780319));
#198382=CARTESIAN_POINT('Ctrl Pts',(-6.22925194598829,2.64513358766136,
59.1748623172122));
#198383=CARTESIAN_POINT('Ctrl Pts',(-6.26369881085293,2.56249264663979,
59.1790840563926));
#198384=CARTESIAN_POINT('Ctrl Pts',(-6.29647317771066,2.47925684880979,
59.1833057955729));
#198385=CARTESIAN_POINT('Ctrl Pts',(-6.373791420635,2.2828946836898,59.1932653306243));
#198386=CARTESIAN_POINT('Ctrl Pts',(-6.44192552376281,2.08289773371365,
59.2032248656757));
#198387=CARTESIAN_POINT('Ctrl Pts',(-6.5005853984413,1.88007406172517,59.2131844007271));
#198388=CARTESIAN_POINT('Ctrl Pts',(-6.55661410572472,1.68634797195297,
59.2226972044474));
#198389=CARTESIAN_POINT('Ctrl Pts',(-6.60399976692655,1.4900433177012,59.2322100081678));
#198390=CARTESIAN_POINT('Ctrl Pts',(-6.64253932075502,1.29188249164675,
59.2417228118881));
#198391=CARTESIAN_POINT('Ctrl Pts',(-6.68098477670612,1.09420549353679,
59.2512123892202));
#198392=CARTESIAN_POINT('Ctrl Pts',(-6.71062720877404,0.894681494081056,
59.2607019665523));
#198393=CARTESIAN_POINT('Ctrl Pts',(-6.73131431791604,0.694043625011065,
59.2701915438844));
#198394=CARTESIAN_POINT('Ctrl Pts',(-6.7519070606708,0.494320986325281,
59.2796378335284));
#198395=CARTESIAN_POINT('Ctrl Pts',(-6.76362593898087,0.293494741529154,
59.2890841231724));
#198396=CARTESIAN_POINT('Ctrl Pts',(-6.76637046870224,0.0923021141375346,
59.2985304128164));
#198397=CARTESIAN_POINT('Ctrl Pts',(-6.76678592257535,0.0618465298379839,
59.2999603472742));
#198398=CARTESIAN_POINT('Ctrl Pts',(-6.76699582823407,0.0313825743895913,
59.3013902817321));
#198399=CARTESIAN_POINT('Ctrl Pts',(-6.76699993843214,0.000912830451469524,
59.3028202161899));
#198400=CARTESIAN_POINT('Ctrl Pts',(-6.767,1.48494626510862E-12,59.3028202161899));
#198401=CARTESIAN_POINT('Ctrl Pts',(-6.76700000000004,-0.186007249525479,
59.3115697280011));
#198402=CARTESIAN_POINT('Ctrl Pts',(-6.75932637294528,-0.372014355748617,
59.3203192398123));
#198403=CARTESIAN_POINT('Ctrl Pts',(-6.7440051826419,-0.557389537486286,
59.3290687516235));
#198404=CARTESIAN_POINT('Ctrl Pts',(-6.72868405705097,-0.742763936250755,
59.3378182264792));
#198405=CARTESIAN_POINT('Ctrl Pts',(-6.70571545645737,-0.927506130241397,
59.3465677013348));
#198406=CARTESIAN_POINT('Ctrl Pts',(-6.67517739404813,-1.1109886399009,
59.3553171761905));
#198407=CARTESIAN_POINT('Ctrl Pts',(-6.64463945808683,-1.29447038982047,
59.3640666148175));
#198408=CARTESIAN_POINT('Ctrl Pts',(-6.60653217008327,-1.47669218313809,
59.3728160534445));
#198409=CARTESIAN_POINT('Ctrl Pts',(-6.56098496092639,-1.65703510599436,
59.3815654920716));
#198410=CARTESIAN_POINT('Ctrl Pts',(-6.51543793658257,-1.83737729708838,
59.3903148951967));
#198411=CARTESIAN_POINT('Ctrl Pts',(-6.4624511216738,-2.01584035511053,
59.3990642983219));
#198412=CARTESIAN_POINT('Ctrl Pts',(-6.40220448374214,-2.19181813760906,
59.407813701447));
#198413=CARTESIAN_POINT('Ctrl Pts',(-6.34195808526463,-2.36779522067251,
59.4165630697971));
#198414=CARTESIAN_POINT('Ctrl Pts',(-6.27445201433063,-2.54128677684266,
59.4253124381472));
#198415=CARTESIAN_POINT('Ctrl Pts',(-6.19991555071861,-2.71170355384904,
59.4340618064973));
#198416=CARTESIAN_POINT('Ctrl Pts',(-6.12537937716646,-2.88211966767577,
59.4428111407991));
#198417=CARTESIAN_POINT('Ctrl Pts',(-6.04381298052467,-3.04946076371892,
59.4515604751009));
#198418=CARTESIAN_POINT('Ctrl Pts',(-5.95549339335771,-3.21315848374659,
59.4603098094027));
#198419=CARTESIAN_POINT('Ctrl Pts',(-5.86717414255346,-3.37685558033602,
59.4690591103829));
#198420=CARTESIAN_POINT('Ctrl Pts',(-5.77210188876532,-3.53690907646864,
59.4778084113631));
#198421=CARTESIAN_POINT('Ctrl Pts',(-5.67059953346928,-3.69277536969392,
59.4865577123432));
#198422=CARTESIAN_POINT('Ctrl Pts',(-5.56909755631311,-3.84864108225029,
59.4953069807285));
#198423=CARTESIAN_POINT('Ctrl Pts',(-5.46116568196773,-4.00031938297623,
59.5040562491138));
#198424=CARTESIAN_POINT('Ctrl Pts',(-5.34717048533521,-4.1472951185996,
59.5128055174991));
#198425=CARTESIAN_POINT('Ctrl Pts',(-5.23317570391758,-4.29427031888012,
59.5215547540161));
#198426=CARTESIAN_POINT('Ctrl Pts',(-5.11311782003439,-4.43654276189633,
59.5303039905332));
#198427=CARTESIAN_POINT('Ctrl Pts',(-4.98740458984683,-4.57362924351928,
59.5390532270502));
#198428=CARTESIAN_POINT('Ctrl Pts',(-4.86169180711664,-4.71071523720349,
59.5478024324257));
#198429=CARTESIAN_POINT('Ctrl Pts',(-4.73032391204083,-4.84261509523324,
59.5565516378011));
#198430=CARTESIAN_POINT('Ctrl Pts',(-4.59374707013501,-4.9688808453842,
59.5653008431765));
#198431=CARTESIAN_POINT('Ctrl Pts',(-4.45717070301346,-5.09514615659551,
59.574050018137));
#198432=CARTESIAN_POINT('Ctrl Pts',(-4.31538563570941,-5.2157772045961,
59.5827991930974));
#198433=CARTESIAN_POINT('Ctrl Pts',(-4.16887341029408,-5.33036429232966,
59.5915483680579));
#198434=CARTESIAN_POINT('Ctrl Pts',(-4.02236168203597,-5.44495099123697,
59.6002975133299));
#198435=CARTESIAN_POINT('Ctrl Pts',(-3.87112305348047,-5.55349359438684,
59.6090466586019));
#198436=CARTESIAN_POINT('Ctrl Pts',(-3.71567117017634,-5.65562346298977,
59.617795803874));
#198437=CARTESIAN_POINT('Ctrl Pts',(-3.56021980145696,-5.7577529935172,
59.6265449201841));
#198438=CARTESIAN_POINT('Ctrl Pts',(-3.40055544538231,-5.85346967463941,
59.6352940364943));
#198439=CARTESIAN_POINT('Ctrl Pts',(-3.23722035986741,-5.94244842986962,
59.6440431528044));
#198440=CARTESIAN_POINT('Ctrl Pts',(-3.07388580147068,-6.03142689794586,
59.6527922408793));
#198441=CARTESIAN_POINT('Ctrl Pts',(-2.90688078896467,-6.11366734656834,
59.6615413289541));
#198442=CARTESIAN_POINT('Ctrl Pts',(-2.7367725072126,-6.18889046952402,
59.670290417029));
#198443=CARTESIAN_POINT('Ctrl Pts',(-2.56666476031357,-6.26411335596379,
59.679039477595));
#198444=CARTESIAN_POINT('Ctrl Pts',(-2.39345402575025,-6.33231884500609,
59.687788538161));
#198445=CARTESIAN_POINT('Ctrl Pts',(-2.21772856065436,-6.39327529762781,
59.6965375987271));
#198446=CARTESIAN_POINT('Ctrl Pts',(-2.04200363348324,-6.45423156365172,
59.7052866325108));
#198447=CARTESIAN_POINT('Ctrl Pts',(-1.86376426189055,-6.50793874375723,
59.7140356662945));
#198448=CARTESIAN_POINT('Ctrl Pts',(-1.68361577752896,-6.55421443909608,
59.7227847000782));
#198449=CARTESIAN_POINT('Ctrl Pts',(-1.50346782967561,-6.60048999661922,
59.731533707806));
#198450=CARTESIAN_POINT('Ctrl Pts',(-1.32141105794769,-6.63933404237755,
59.7402827155338));
#198451=CARTESIAN_POINT('Ctrl Pts',(-1.13806375486826,-6.67061465607594,
59.7490317232617));
#198452=CARTESIAN_POINT('Ctrl Pts',(-0.954716982601011,-6.70189517921325,
59.7577807056601));
#198453=CARTESIAN_POINT('Ctrl Pts',(-0.770079968900096,-6.72561226592252,
59.7665296880585));
#198454=CARTESIAN_POINT('Ctrl Pts',(-0.584779765556168,-6.7416853698312,
59.7752786704569));
#198455=CARTESIAN_POINT('Ctrl Pts',(-0.391489830649242,-6.75845151013865,
59.7844048894667));
#198456=CARTESIAN_POINT('Ctrl Pts',(-0.197478578236303,-6.76689983031631,
59.7935311084766));
#198457=CARTESIAN_POINT('Ctrl Pts',(-0.00346287644933841,-6.76699911397118,
59.8026573274865));
#198458=CARTESIAN_POINT('Ctrl Pts',(0.184489834656752,-6.76709529501183,
59.8114983521523));
#198459=CARTESIAN_POINT('Ctrl Pts',(0.372446404252195,-6.75935639738152,
59.8203393768181));
#198460=CARTESIAN_POINT('Ctrl Pts',(0.559755019491118,-6.74380925873163,
59.8291804014839));
#198461=CARTESIAN_POINT('Ctrl Pts',(0.74513470552457,-6.72842222659775,
59.8379303800937));
#198462=CARTESIAN_POINT('Ctrl Pts',(0.929879431231373,-6.70538706057485,
59.8466803587034));
#198463=CARTESIAN_POINT('Ctrl Pts',(1.11336163627107,-6.6747820089408,59.8554303373131));
#198464=CARTESIAN_POINT('Ctrl Pts',(1.29684196301015,-6.64417727060955,
59.8641802263497));
#198465=CARTESIAN_POINT('Ctrl Pts',(1.47905951217821,-6.60600284890521,
59.8729301153862));
#198466=CARTESIAN_POINT('Ctrl Pts',(1.65939532067409,-6.56038841607149,
59.8816800044227));
#198467=CARTESIAN_POINT('Ctrl Pts',(1.8397293430113,-6.51477443503164,59.8904298067949));
#198468=CARTESIAN_POINT('Ctrl Pts',(2.01818138406596,-6.46172066062038,
59.899179609167));
#198469=CARTESIAN_POINT('Ctrl Pts',(2.19414528354533,-6.40140730423364,
59.9079294115392));
#198470=CARTESIAN_POINT('Ctrl Pts',(2.37010749864323,-6.34109452518521,
59.9166791301555));
#198471=CARTESIAN_POINT('Ctrl Pts',(2.54358134866773,-6.27352239616377,
59.9254288487718));
#198472=CARTESIAN_POINT('Ctrl Pts',(2.71397759435858,-6.19892043966686,
59.9341785673882));
#198473=CARTESIAN_POINT('Ctrl Pts',(2.88437226558423,-6.12431917249374,
59.9429282051569));
#198474=CARTESIAN_POINT('Ctrl Pts',(3.0516891268125,-6.0426883227865,59.9516778429256));
#198475=CARTESIAN_POINT('Ctrl Pts',(3.21535986274144,-5.95430516123178,
59.9604274806943));
#198476=CARTESIAN_POINT('Ctrl Pts',(3.37902914073127,-5.86592278697276,
59.9691770405234));
#198477=CARTESIAN_POINT('Ctrl Pts',(3.53905210621852,-5.7707883574177,59.9779266003524));
#198478=CARTESIAN_POINT('Ctrl Pts',(3.69488522831972,-5.6692250043145,59.9866761601815));
#198479=CARTESIAN_POINT('Ctrl Pts',(3.85071701407214,-5.56766252216904,
59.9954256449786));
#198480=CARTESIAN_POINT('Ctrl Pts',(4.00235878822677,-5.4596713832917,60.0041751297757));
#198481=CARTESIAN_POINT('Ctrl Pts',(4.14929549611596,-5.34561838199397,
60.0129246145728));
#198482=CARTESIAN_POINT('Ctrl Pts',(4.29623099276355,-5.23156632086797,
60.0216740272454));
#198483=CARTESIAN_POINT('Ctrl Pts',(4.43846127436287,-5.11145267304739,
60.030423439918));
#198484=CARTESIAN_POINT('Ctrl Pts',(4.57550326054695,-4.98568540049653,
60.0391728525906));
#198485=CARTESIAN_POINT('Ctrl Pts',(4.71254416258024,-4.85991912290124,
60.0479221960459));
#198486=CARTESIAN_POINT('Ctrl Pts',(4.84439664018995,-4.72849950385179,
60.0566715395011));
#198487=CARTESIAN_POINT('Ctrl Pts',(4.97061286794969,-4.59187289860825,
60.0654208829563));
#198488=CARTESIAN_POINT('Ctrl Pts',(5.09682813912891,-4.45524732884448,
60.0741701601012));
#198489=CARTESIAN_POINT('Ctrl Pts',(5.21740705148029,-4.31341506235557,
60.082919437246));
#198490=CARTESIAN_POINT('Ctrl Pts',(5.3319400754587,-4.16685781275501,60.0916687143908));
#198491=CARTESIAN_POINT('Ctrl Pts',(5.44647226944652,-4.02030162521616,
60.1004179281319));
#198492=CARTESIAN_POINT('Ctrl Pts',(5.55495848628272,-3.86902074887706,
60.1091671418731));
#198493=CARTESIAN_POINT('Ctrl Pts',(5.65703027291939,-3.71352898080432,
60.1179163556142));
#198494=CARTESIAN_POINT('Ctrl Pts',(5.75910135377141,-3.55803828789356,
60.1266655088581));
#198495=CARTESIAN_POINT('Ctrl Pts',(5.85475793592888,-3.39833700106478,
60.1354146621019));
#198496=CARTESIAN_POINT('Ctrl Pts',(5.94367514427526,-3.23496750823319,
60.1441638153458));
#198497=CARTESIAN_POINT('Ctrl Pts',(6.0325917673276,-3.0715990907749,60.1529129109987));
#198498=CARTESIAN_POINT('Ctrl Pts',(6.11476896836036,-2.90456276731199,
60.1616620066517));
#198499=CARTESIAN_POINT('Ctrl Pts',(6.1899276554799,-2.73442583002815,60.1704111023046));
#198500=CARTESIAN_POINT('Ctrl Pts',(6.26508587283144,-2.56428995615949,
60.1791601432726));
#198501=CARTESIAN_POINT('Ctrl Pts',(6.33322554827237,-2.39105376934996,
60.1879091842406));
#198502=CARTESIAN_POINT('Ctrl Pts',(6.39411526733096,-2.21530561053889,
60.1966582252087));
#198503=CARTESIAN_POINT('Ctrl Pts',(6.45500462602905,-2.03955849184915,
60.2054072143977));
#198504=CARTESIAN_POINT('Ctrl Pts',(6.50864402040791,-1.86129970164368,
60.2141562035867));
#198505=CARTESIAN_POINT('Ctrl Pts',(6.55485128368644,-1.6811346313589,60.2229051927757));
#198506=CARTESIAN_POINT('Ctrl Pts',(6.60199809554361,-1.49730620116714,
60.2318320782472));
#198507=CARTESIAN_POINT('Ctrl Pts',(6.64140720707901,-1.31149343245558,
60.2407589637186));
#198508=CARTESIAN_POINT('Ctrl Pts',(6.67293928722905,-1.124353266974,60.24968584919));
#198509=CARTESIAN_POINT('Ctrl Pts',(6.70384625876274,-0.940923067005351,
60.2584357633675));
#198510=CARTESIAN_POINT('Ctrl Pts',(6.7271855457981,-0.756217899520448,
60.2671856775449));
#198511=CARTESIAN_POINT('Ctrl Pts',(6.74287786815338,-0.570865181253302,
60.2759355917224));
#198512=CARTESIAN_POINT('Ctrl Pts',(6.75856988190852,-0.385516108072819,
60.2846853338269));
#198513=CARTESIAN_POINT('Ctrl Pts',(6.76661520773406,-0.19951979522529,
60.2934350759314));
#198514=CARTESIAN_POINT('Ctrl Pts',(6.76698651789579,-0.0135080204546609,
60.3021848180358));
#198515=CARTESIAN_POINT('Ctrl Pts',(6.767357821249,0.172500343513941,60.3109343997008));
#198516=CARTESIAN_POINT('Ctrl Pts',(6.76005538995179,0.358523882211893,
60.3196839813658));
#198517=CARTESIAN_POINT('Ctrl Pts',(6.74510402742353,0.54393074856534,60.3284335630308));
#198518=CARTESIAN_POINT('Ctrl Pts',(6.7301529191802,0.729334461616193,60.3371829958874));
#198519=CARTESIAN_POINT('Ctrl Pts',(6.70755316306582,0.914121237635632,
60.3459324287441));
#198520=CARTESIAN_POINT('Ctrl Pts',(6.67738151874559,1.09766345166216,60.3546818616008));
#198521=CARTESIAN_POINT('Ctrl Pts',(6.64721034747551,1.28120278799758,60.3634311572783));
#198522=CARTESIAN_POINT('Ctrl Pts',(6.60946757205121,1.46349731860422,60.3721804529559));
#198523=CARTESIAN_POINT('Ctrl Pts',(6.564281381115,1.64392790278255,60.3809297486334));
#198524=CARTESIAN_POINT('Ctrl Pts',(6.51909583859825,1.82435589779144,60.389678918759));
#198525=CARTESIAN_POINT('Ctrl Pts',(6.46646716392849,2.00291972192349,60.3984280888846));
#198526=CARTESIAN_POINT('Ctrl Pts',(6.40657409872857,2.17901292274742,60.4071772590102));
#198527=CARTESIAN_POINT('Ctrl Pts',(6.34668181342048,2.35510383059053,60.4159263152093));
#198528=CARTESIAN_POINT('Ctrl Pts',(6.27952541914021,2.52872390822653,60.4246753714084));
#198529=CARTESIAN_POINT('Ctrl Pts',(6.20533299175486,2.69928350890356,60.4334244276075));
#198530=CARTESIAN_POINT('Ctrl Pts',(6.12831602991515,2.87633637965696,60.4425065637657));
#198531=CARTESIAN_POINT('Ctrl Pts',(6.04371690605232,3.05009086601537,60.4515886999239));
#198532=CARTESIAN_POINT('Ctrl Pts',(5.95184520316589,3.21991112882812,60.4606708360821));
#198533=CARTESIAN_POINT('Ctrl Pts',(5.86333549509226,3.38351691183101,60.4694206164257));
#198534=CARTESIAN_POINT('Ctrl Pts',(5.76807618099313,3.54347103712095,60.4781703967692));
#198535=CARTESIAN_POINT('Ctrl Pts',(5.66639083308952,3.69923018027793,60.4869201771128));
#198536=CARTESIAN_POINT('Ctrl Pts',(5.56470914082134,3.85498372382145,60.4956696428977));
#198537=CARTESIAN_POINT('Ctrl Pts',(5.45660203371999,4.00654234702091,60.5044191086826));
#198538=CARTESIAN_POINT('Ctrl Pts',(5.34243669839146,4.15339127986759,60.5131685744675));
#198539=CARTESIAN_POINT('Ctrl Pts',(5.22827486050517,4.3002357140137,60.5219177722136));
#198540=CARTESIAN_POINT('Ctrl Pts',(5.10805534167032,4.4423705202856,60.5306669699596));
#198541=CARTESIAN_POINT('Ctrl Pts',(4.98218644339868,4.57931296628811,60.5394161677056));
#198542=CARTESIAN_POINT('Ctrl Pts',(4.85632073219498,4.71625194483451,60.5481651439172));
#198543=CARTESIAN_POINT('Ctrl Pts',(4.72480612170226,4.84799861524599,60.5569141201289));
#198544=CARTESIAN_POINT('Ctrl Pts',(4.58808925235213,4.97410554898575,60.5656630963405));
#198545=CARTESIAN_POINT('Ctrl Pts',(4.45136349473951,5.10022068121291,60.5744126413422));
#198546=CARTESIAN_POINT('Ctrl Pts',(4.30943501209983,5.22069514871914,60.5831621863439));
#198547=CARTESIAN_POINT('Ctrl Pts',(4.16278587431686,5.33511975166331,60.5919117313456));
#198548=CARTESIAN_POINT('Ctrl Pts',(4.01614535740335,5.44953762807926,60.6006607619993));
#198549=CARTESIAN_POINT('Ctrl Pts',(3.86478496657793,5.55790617532875,60.6094097926531));
#198550=CARTESIAN_POINT('Ctrl Pts',(3.70921874747046,5.65985735539454,60.6181588233068));
#198551=CARTESIAN_POINT('Ctrl Pts',(3.55365041605759,5.76180991977134,60.6269079727564));
#198552=CARTESIAN_POINT('Ctrl Pts',(3.39387638174388,5.85734478552891,60.635657122206));
#198553=CARTESIAN_POINT('Ctrl Pts',(3.23043927904413,5.946137491213,60.6444062716557));
#198554=CARTESIAN_POINT('Ctrl Pts',(3.18691767070344,5.96978206944193,60.6467360795718));
#198555=CARTESIAN_POINT('Ctrl Pts',(3.14313645919583,5.9929488063345,60.6490658874879));
#198556=CARTESIAN_POINT('Ctrl Pts',(3.09910619832132,6.01563211736941,60.6513956954041));
#198557=CARTESIAN_POINT('Origin',(0.,0.,4.30282021618968));
#198558=CARTESIAN_POINT('',(3.09910619832125,6.01563211736945,63.0457521963359));
#198559=CARTESIAN_POINT('',(3.09910619832141,6.01563211736936,62.6510873080017));
#198560=CARTESIAN_POINT('',(3.09910619832133,6.0156321173694,4.30282021618968));
#198561=CARTESIAN_POINT('',(-6.76699974432514,0.00186018910577019,61.6971797837854));
#198562=CARTESIAN_POINT('Ctrl Pts',(-6.76699974432528,0.00186018858652958,
61.69717978381));
#198563=CARTESIAN_POINT('Ctrl Pts',(-6.76700888267723,-0.0313833361700197,
61.698754657245));
#198564=CARTESIAN_POINT('Ctrl Pts',(-6.76677305573693,-0.0646273068054331,
61.70032953068));
#198565=CARTESIAN_POINT('Ctrl Pts',(-6.7662922309777,-0.097869530553651,
61.701904404115));
#198566=CARTESIAN_POINT('Ctrl Pts',(-6.76382858940636,-0.268195460695293,
61.7099737133375));
#198567=CARTESIAN_POINT('Ctrl Pts',(-6.75492480586881,-0.438740522579581,
61.71804302256));
#198568=CARTESIAN_POINT('Ctrl Pts',(-6.7395436862802,-0.608966255814484,
61.7261123317825));
#198569=CARTESIAN_POINT('Ctrl Pts',(-6.72418175112818,-0.778979671294108,
61.7341715763833));
#198570=CARTESIAN_POINT('Ctrl Pts',(-6.70235858813183,-0.948674183693938,
61.742230820984));
#198571=CARTESIAN_POINT('Ctrl Pts',(-6.67408890878531,-1.11750894297491,
61.7502900655848));
#198572=CARTESIAN_POINT('Ctrl Pts',(-6.64584828567779,-1.28617016993328,
61.758341026705));
#198573=CARTESIAN_POINT('Ctrl Pts',(-6.61117439294617,-1.45397303739914,
61.7663919878253));
#198574=CARTESIAN_POINT('Ctrl Pts',(-6.57013387633598,-1.62037953795473,
61.7744429489456));
#198575=CARTESIAN_POINT('Ctrl Pts',(-6.52912654933898,-1.78665146497562,
61.7824873992246));
#198576=CARTESIAN_POINT('Ctrl Pts',(-6.48176293499712,-1.95152891222019,
61.7905318495037));
#198577=CARTESIAN_POINT('Ctrl Pts',(-6.42816110462577,-2.11448192543149,
61.7985762997828));
#198578=CARTESIAN_POINT('Ctrl Pts',(-6.37459088930749,-2.27733882684724,
61.8066160053411));
#198579=CARTESIAN_POINT('Ctrl Pts',(-6.31478989880819,-2.4382732002311,
61.8146557108993));
#198580=CARTESIAN_POINT('Ctrl Pts',(-6.24892658892837,-2.59676827733706,
61.8226954164575));
#198581=CARTESIAN_POINT('Ctrl Pts',(-6.18164165471705,-2.75868438594671,
61.830908654762));
#198582=CARTESIAN_POINT('Ctrl Pts',(-6.10802981782756,-2.91805431215768,
61.8391218930664));
#198583=CARTESIAN_POINT('Ctrl Pts',(-6.02832354973824,-3.07434613855879,
61.8473351313709));
#198584=CARTESIAN_POINT('Ctrl Pts',(-5.9503264647624,-3.22728651774173,
61.8553722489191));
#198585=CARTESIAN_POINT('Ctrl Pts',(-5.86649385885111,-3.37727912908345,
61.8634093664673));
#198586=CARTESIAN_POINT('Ctrl Pts',(-5.77709092958998,-3.5238486617971,
61.8714464840154));
#198587=CARTESIAN_POINT('Ctrl Pts',(-5.68767854206744,-3.67043370063529,
61.8794844518396));
#198588=CARTESIAN_POINT('Ctrl Pts',(-5.59269485227502,-3.81359462072695,
61.8875224196637));
#198589=CARTESIAN_POINT('Ctrl Pts',(-5.4924492683956,-3.95288376177452,
61.8955603874878));
#198590=CARTESIAN_POINT('Ctrl Pts',(-5.39217321682531,-4.09221523704097,
61.9036007982955));
#198591=CARTESIAN_POINT('Ctrl Pts',(-5.28663230600283,-4.22767228787798,
61.9116412091032));
#198592=CARTESIAN_POINT('Ctrl Pts',(-5.17617712363885,-4.35883922446308,
61.9196816199109));
#198593=CARTESIAN_POINT('Ctrl Pts',(-5.06154735835593,-4.49496353146103,
61.9280259128988));
#198594=CARTESIAN_POINT('Ctrl Pts',(-4.94162488735914,-4.62646676344811,
61.9363702058866));
#198595=CARTESIAN_POINT('Ctrl Pts',(-4.81684379510684,-4.75292592552638,
61.9447144988744));
#198596=CARTESIAN_POINT('Ctrl Pts',(-4.69639463760129,-4.8749948965239,
61.9527691090899));
#198597=CARTESIAN_POINT('Ctrl Pts',(-4.57141886569017,-4.9923639484135,
61.9608237193054));
#198598=CARTESIAN_POINT('Ctrl Pts',(-4.44234051109221,-5.10469389714104,
61.968878329521));
#198599=CARTESIAN_POINT('Ctrl Pts',(-4.31316444235635,-5.21710888122664,
61.9769390371902));
#198600=CARTESIAN_POINT('Ctrl Pts',(-4.17987989599693,-5.32447693396655,
61.9849997448595));
#198601=CARTESIAN_POINT('Ctrl Pts',(-4.0429402500153,-5.42650192433452,
61.9930604525288));
#198602=CARTESIAN_POINT('Ctrl Pts',(-3.90580752733713,-5.52867076382641,
62.0011325253129));
#198603=CARTESIAN_POINT('Ctrl Pts',(-3.76500972787653,-5.62548130090922,
62.0092045980971));
#198604=CARTESIAN_POINT('Ctrl Pts',(-3.6210256756095,-5.71668278432316,
62.0172766708812));
#198605=CARTESIAN_POINT('Ctrl Pts',(-3.60594444009007,-5.72623544678425,
62.0181221591757));
#198606=CARTESIAN_POINT('Ctrl Pts',(-3.59082826677618,-5.73572661583186,
62.0189676474702));
#198607=CARTESIAN_POINT('Ctrl Pts',(-3.57567771841961,-5.74515603391218,
62.0198131357647));
#198608=CARTESIAN_POINT('Ctrl Pts',(-3.42635768733166,-5.83809002994699,
62.0281460578114));
#198609=CARTESIAN_POINT('Ctrl Pts',(-3.27322051995201,-5.92531833426816,
62.0364789798581));
#198610=CARTESIAN_POINT('Ctrl Pts',(-3.11673520276891,-6.00651734999751,
62.0448119019049));
#198611=CARTESIAN_POINT('Ctrl Pts',(-2.96043481328268,-6.0876204081812,
62.0531349764585));
#198612=CARTESIAN_POINT('Ctrl Pts',(-2.80079446225958,-6.16270821275327,
62.0614580510121));
#198613=CARTESIAN_POINT('Ctrl Pts',(-2.63831147126212,-6.23150074866454,
62.0697811255657));
#198614=CARTESIAN_POINT('Ctrl Pts',(-2.47599067107149,-6.3002246157457,
62.0780958920117));
#198615=CARTESIAN_POINT('Ctrl Pts',(-2.31083320259564,-6.36266559899581,
62.0864106584577));
#198616=CARTESIAN_POINT('Ctrl Pts',(-2.14336051423539,-6.41858977548937,
62.0947254249036));
#198617=CARTESIAN_POINT('Ctrl Pts',(-1.97602427727905,-6.47446838674796,
62.1030334167432));
#198618=CARTESIAN_POINT('Ctrl Pts',(-1.80637690779052,-6.52384066150702,
62.1113414085827));
#198619=CARTESIAN_POINT('Ctrl Pts',(-1.63495955161181,-6.56652086455174,
62.1196494004222));
#198620=CARTESIAN_POINT('Ctrl Pts',(-1.46365043426143,-6.60917411784484,
62.1279521463093));
#198621=CARTESIAN_POINT('Ctrl Pts',(-1.29057389421217,-6.64514363672157,
62.1362548921963));
#198622=CARTESIAN_POINT('Ctrl Pts',(-1.11628616519195,-6.67429353545385,
62.1445576380834));
#198623=CARTESIAN_POINT('Ctrl Pts',(-0.942069662011984,-6.70343152155154,
62.1528569909028));
#198624=CARTESIAN_POINT('Ctrl Pts',(-0.766643298753215,-6.72575538342788,
62.1611563437222));
#198625=CARTESIAN_POINT('Ctrl Pts',(-0.590573717251133,-6.74118028868033,
62.1694556965417));
#198626=CARTESIAN_POINT('Ctrl Pts',(-0.414541582794685,-6.75660191331425,
62.177753284228));
#198627=CARTESIAN_POINT('Ctrl Pts',(-0.237866849011761,-6.76512747415664,
62.1860508719144));
#198628=CARTESIAN_POINT('Ctrl Pts',(-0.0611217481314931,-6.76672395860104,
62.1943484596007));
#198629=CARTESIAN_POINT('Ctrl Pts',(0.115615132693807,-6.7683203687962,
62.2026456613831));
#198630=CARTESIAN_POINT('Ctrl Pts',(0.292422026227014,-6.76298834178729,
62.2109428631655));
#198631=CARTESIAN_POINT('Ctrl Pts',(0.468726030304149,-6.75074698892762,
62.219240064948));
#198632=CARTESIAN_POINT('Ctrl Pts',(0.645051130896099,-6.73850417126922,
62.2275382595725));
#198633=CARTESIAN_POINT('Ctrl Pts',(0.820872875120574,-6.71935040502058,
62.235836454197));
#198634=CARTESIAN_POINT('Ctrl Pts',(0.995622617714268,-6.69335675151831,
62.2441346488216));
#198635=CARTESIAN_POINT('Ctrl Pts',(1.17049526383936,-6.66734481637648,
62.2524386796632));
#198636=CARTESIAN_POINT('Ctrl Pts',(1.34429405725153,-6.63448343276056,
62.2607427105047));
#198637=CARTESIAN_POINT('Ctrl Pts',(1.51645879770513,-6.59489512538772,
62.2690467413463));
#198638=CARTESIAN_POINT('Ctrl Pts',(1.68868614199685,-6.55529242261673,
62.2773537917621));
#198639=CARTESIAN_POINT('Ctrl Pts',(1.85927791168808,-6.50895800586749,
62.2856608421778));
#198640=CARTESIAN_POINT('Ctrl Pts',(2.02768801864551,-6.45606461391469,
62.2939678925935));
#198641=CARTESIAN_POINT('Ctrl Pts',(2.19627818443031,-6.40311466999893,
62.3022838246482));
#198642=CARTESIAN_POINT('Ctrl Pts',(2.36268169710778,-6.34359185088309,
62.3105997567028));
#198643=CARTESIAN_POINT('Ctrl Pts',(2.52637039754753,-6.27771786674071,
62.3189156887574));
#198644=CARTESIAN_POINT('Ctrl Pts',(2.64976241679885,-6.22806065828575,
62.3251844149763));
#198645=CARTESIAN_POINT('Ctrl Pts',(2.77161212861598,-6.17479543469104,
62.3314531411952));
#198646=CARTESIAN_POINT('Ctrl Pts',(2.89170231692055,-6.11803454634872,
62.337721867414));
#198647=CARTESIAN_POINT('Ctrl Pts',(3.05358438462945,-6.04152063543249,
62.3461721361374));
#198648=CARTESIAN_POINT('Ctrl Pts',(3.21256520260729,-5.95851280788114,
62.3546224048607));
#198649=CARTESIAN_POINT('Ctrl Pts',(3.36810870078526,-5.86925317052303,
62.3630726735841));
#198650=CARTESIAN_POINT('Ctrl Pts',(3.52351492654881,-5.78007230782329,
62.3715154846586));
#198651=CARTESIAN_POINT('Ctrl Pts',(3.67548959267449,-5.68465079682643,
62.3799582957331));
#198652=CARTESIAN_POINT('Ctrl Pts',(3.82351956618513,-5.58327745387953,
62.3884011068076));
#198653=CARTESIAN_POINT('Ctrl Pts',(3.97143905288291,-5.48197977410615,
62.3968376163253));
#198654=CARTESIAN_POINT('Ctrl Pts',(4.11541944346791,-5.37473930466906,
62.405274125843));
#198655=CARTESIAN_POINT('Ctrl Pts',(4.25497470436759,-5.26188932468101,
62.4137106353607));
#198656=CARTESIAN_POINT('Ctrl Pts',(4.39443010596926,-5.14912009492559,
62.4221411081019));
#198657=CARTESIAN_POINT('Ctrl Pts',(4.52946643660968,-5.03074956898987,
62.4305715808431));
#198658=CARTESIAN_POINT('Ctrl Pts',(4.65962884076262,-4.90715274536397,
62.4390020535843));
#198659=CARTESIAN_POINT('Ctrl Pts',(4.7897352884504,-4.78360905567796,62.4474289020881));
#198660=CARTESIAN_POINT('Ctrl Pts',(4.9149717466706,-4.65484377522036,62.4558557505919));
#198661=CARTESIAN_POINT('Ctrl Pts',(5.03491800266433,-4.52127080658156,
62.4642825990957));
#198662=CARTESIAN_POINT('Ctrl Pts',(5.15482723553273,-4.3877390671476,62.4727068465323));
#198663=CARTESIAN_POINT('Ctrl Pts',(5.26944930127381,-4.24940284532616,
62.4811310939689));
#198664=CARTESIAN_POINT('Ctrl Pts',(5.37840204215944,-4.10671163741688,
62.4895553414056));
#198665=CARTESIAN_POINT('Ctrl Pts',(5.40910075594672,-4.0665067144754,62.4919289720167));
#198666=CARTESIAN_POINT('Ctrl Pts',(5.43934962480274,-4.02595625746157,
62.4943026026278));
#198667=CARTESIAN_POINT('Ctrl Pts',(5.46914067786036,-3.98507079557857,
62.4966762332389));
#198668=CARTESIAN_POINT('Ctrl Pts',(5.57731360038267,-3.83661347545612,
62.5052950141761));
#198669=CARTESIAN_POINT('Ctrl Pts',(5.67939881289885,-3.68380335449862,
62.5139137951133));
#198670=CARTESIAN_POINT('Ctrl Pts',(5.77506832117722,-3.52716244107573,
62.5225325760505));
#198671=CARTESIAN_POINT('Ctrl Pts',(5.87079529754818,-3.37042743440748,
62.531156534237));
#198672=CARTESIAN_POINT('Ctrl Pts',(5.9600987199737,-3.20985730249598,62.5397804924236));
#198673=CARTESIAN_POINT('Ctrl Pts',(6.04269602840139,-3.04599962382501,
62.5484044506101));
#198674=CARTESIAN_POINT('Ctrl Pts',(6.12827729576277,-2.87622232630165,
62.5573399629813));
#198675=CARTESIAN_POINT('Ctrl Pts',(6.20665872006912,-2.70291584292701,
62.5662754753524));
#198676=CARTESIAN_POINT('Ctrl Pts',(6.27758023075002,-2.5267123790603,62.5752109877235));
#198677=CARTESIAN_POINT('Ctrl Pts',(6.34615689820091,-2.35633464416332,
62.5838510696182));
#198678=CARTESIAN_POINT('Ctrl Pts',(6.40775898527662,-2.18324872818015,
62.5924911515129));
#198679=CARTESIAN_POINT('Ctrl Pts',(6.46220194008558,-2.0080426005327,62.6011312334076));
#198680=CARTESIAN_POINT('Ctrl Pts',(6.51943724830169,-1.82385023344974,
62.610214461017));
#198681=CARTESIAN_POINT('Ctrl Pts',(6.56875965702786,-1.63731483298587,
62.6192976886263));
#198682=CARTESIAN_POINT('Ctrl Pts',(6.61001524464286,-1.44913334982983,
62.6283809162356));
#198683=CARTESIAN_POINT('Ctrl Pts',(6.65127083225785,-1.26095186667384,
62.6374641438449));
#198684=CARTESIAN_POINT('Ctrl Pts',(6.68445956512924,-1.07112468860344,
62.6465473714543));
#198685=CARTESIAN_POINT('Ctrl Pts',(6.7094903097447,-0.88035719082765,62.6556305990636));
#198686=CARTESIAN_POINT('Ctrl Pts',(6.73441459369128,-0.690401064656113,
62.6646751939234));
#198687=CARTESIAN_POINT('Ctrl Pts',(6.75127402270358,-0.49933729491443,
62.6737197887833));
#198688=CARTESIAN_POINT('Ctrl Pts',(6.75999462970576,-0.307833731662577,
62.6827643836431));
#198689=CARTESIAN_POINT('Ctrl Pts',(6.76870723417835,-0.116505903073646,
62.6918006786634));
#198690=CARTESIAN_POINT('Ctrl Pts',(6.76929591702558,0.0752606758338459,
62.7008369736838));
#198691=CARTESIAN_POINT('Ctrl Pts',(6.76173865261451,0.26679466587419,62.7098732687042));
#198692=CARTESIAN_POINT('Ctrl Pts',(6.75419476137546,0.457989721499053,
62.7188935732919));
#198693=CARTESIAN_POINT('Ctrl Pts',(6.73853371694772,0.648952772738747,
62.7279138778796));
#198694=CARTESIAN_POINT('Ctrl Pts',(6.71478547954788,0.839014280958885,
62.7369341824673));
#198695=CARTESIAN_POINT('Ctrl Pts',(6.6910671484399,1.02883644362932,62.7459431277336));
#198696=CARTESIAN_POINT('Ctrl Pts',(6.65928197802554,1.21775909363292,62.7549520729999));
#198697=CARTESIAN_POINT('Ctrl Pts',(6.61951169806382,1.40511703398552,62.7639610182662));
#198698=CARTESIAN_POINT('Ctrl Pts',(6.5798317279884,1.59204952411984,62.772949506125));
#198699=CARTESIAN_POINT('Ctrl Pts',(6.53220289169279,1.77742416466695,62.7819379939839));
#198700=CARTESIAN_POINT('Ctrl Pts',(6.47675789903176,1.96058565671835,62.7909264818427));
#198701=CARTESIAN_POINT('Ctrl Pts',(6.42811254883714,2.12128465757279,62.7988126428579));
#198702=CARTESIAN_POINT('Ctrl Pts',(6.37345136413233,2.28028003127382,62.8066988038731));
#198703=CARTESIAN_POINT('Ctrl Pts',(6.31289654940264,2.43713482526926,62.8145849648884));
#198704=CARTESIAN_POINT('Ctrl Pts',(6.2505349264596,2.59866978435746,62.8227064297445));
#198705=CARTESIAN_POINT('Ctrl Pts',(6.18194911347087,2.75786161962484,62.8308278946007));
#198706=CARTESIAN_POINT('Ctrl Pts',(6.10735042438937,2.91419968322539,62.8389493594569));
#198707=CARTESIAN_POINT('Ctrl Pts',(6.03275705529221,3.0705265976213,62.8470702451331));
#198708=CARTESIAN_POINT('Ctrl Pts',(5.9521518219221,3.22399981523457,62.8551911308093));
#198709=CARTESIAN_POINT('Ctrl Pts',(5.86579323692356,3.37413080683927,62.8633120164855));
#198710=CARTESIAN_POINT('Ctrl Pts',(5.77942432960469,3.52427974339045,62.8714338728398));
#198711=CARTESIAN_POINT('Ctrl Pts',(5.68730088493318,3.67108534163933,62.8795557291941));
#198712=CARTESIAN_POINT('Ctrl Pts',(5.58972618509928,3.81408575881762,62.8876775855483));
#198713=CARTESIAN_POINT('Ctrl Pts',(5.49208029597166,3.95719050733098,62.8958053675085));
#198714=CARTESIAN_POINT('Ctrl Pts',(5.3889754147992,4.09648422712913,62.9039331494687));
#198715=CARTESIAN_POINT('Ctrl Pts',(5.28075715399485,4.23153552277802,62.9120609314289));
#198716=CARTESIAN_POINT('Ctrl Pts',(5.17249480909339,4.36664183330505,62.9201920243453));
#198717=CARTESIAN_POINT('Ctrl Pts',(5.05911517217354,4.49750199832047,62.9283231172618));
#198718=CARTESIAN_POINT('Ctrl Pts',(4.94100239287162,4.6237197529302,62.9364542101782));
#198719=CARTESIAN_POINT('Ctrl Pts',(4.82276069840703,4.75007526894444,62.9445941778428));
#198720=CARTESIAN_POINT('Ctrl Pts',(4.69977580325369,4.87177799681061,62.9527341455073));
#198721=CARTESIAN_POINT('Ctrl Pts',(4.57246730136593,4.98846988343514,62.9608741131719));
#198722=CARTESIAN_POINT('Ctrl Pts',(4.50643960782099,5.04899134127162,62.9650958523523));
#198723=CARTESIAN_POINT('Ctrl Pts',(4.43924943815944,5.10816559862391,62.9693175915328));
#198724=CARTESIAN_POINT('Ctrl Pts',(4.37095855157181,5.16594718715177,62.9735393307132));
#198725=CARTESIAN_POINT('Ctrl Pts',(4.23442476346711,5.28146976356893,62.9819798426394));
#198726=CARTESIAN_POINT('Ctrl Pts',(4.09320717501415,5.39166184854721,62.9904203545656));
#198727=CARTESIAN_POINT('Ctrl Pts',(3.94775019044169,5.49614023054977,62.9988608664918));
#198728=CARTESIAN_POINT('Ctrl Pts',(3.8024168135024,5.60052982805321,63.0072942057703));
#198729=CARTESIAN_POINT('Ctrl Pts',(3.6528514942629,5.6992152109744,63.0157275450489));
#198730=CARTESIAN_POINT('Ctrl Pts',(3.49953110373262,5.79185385295658,63.0241608843274));
#198731=CARTESIAN_POINT('Ctrl Pts',(3.368685805096,5.87091268351086,63.0313579883302));
#198732=CARTESIAN_POINT('Ctrl Pts',(3.23510629795606,5.94556819997437,63.0385550923331));
#198733=CARTESIAN_POINT('Ctrl Pts',(3.09910619832125,6.01563211736945,63.0457521963359));
#198734=CARTESIAN_POINT('Ctrl Pts',(3.09910619832126,6.01563211736944,61.0457854935189));
#198735=CARTESIAN_POINT('Ctrl Pts',(2.971669387342,6.08128443837155,61.052552642618));
#198736=CARTESIAN_POINT('Ctrl Pts',(2.84222364202814,6.14284547814351,61.059319791717));
#198737=CARTESIAN_POINT('Ctrl Pts',(2.71104814989807,6.20020216839212,61.066086940816));
#198738=CARTESIAN_POINT('Ctrl Pts',(2.55133175682986,6.27003841246547,61.0743264726669));
#198739=CARTESIAN_POINT('Ctrl Pts',(2.38869389354897,6.33379606301573,61.0825660045177));
#198740=CARTESIAN_POINT('Ctrl Pts',(2.22363567814493,6.39122315139136,61.0908055363685));
#198741=CARTESIAN_POINT('Ctrl Pts',(2.05876066582408,6.44858649971248,61.0990359229148));
#198742=CARTESIAN_POINT('Ctrl Pts',(1.89147098367788,6.49963316084281,61.1072663094612));
#198743=CARTESIAN_POINT('Ctrl Pts',(1.72228992832713,6.54415818900972,61.1154966960075));
#198744=CARTESIAN_POINT('Ctrl Pts',(1.55326647177858,6.58864174036297,61.1237194156253));
#198745=CARTESIAN_POINT('Ctrl Pts',(1.38235549301942,6.62661566748188,61.1319421352431));
#198746=CARTESIAN_POINT('Ctrl Pts',(1.21009783489472,6.65792401803919,61.1401648548609));
#198747=CARTESIAN_POINT('Ctrl Pts',(1.03799280946576,6.68920462714224,61.1483802885566));
#198748=CARTESIAN_POINT('Ctrl Pts',(0.864543831775616,6.71383136785693,
61.1565957222524));
#198749=CARTESIAN_POINT('Ctrl Pts',(0.690304263422528,6.73169882153834,
61.1648111559482));
#198750=CARTESIAN_POINT('Ctrl Pts',(0.516154240677573,6.749557092736,61.173022367549));
#198751=CARTESIAN_POINT('Ctrl Pts',(0.341214789640626,6.76066295895982,
61.1812335791498));
#198752=CARTESIAN_POINT('Ctrl Pts',(0.166047180039049,6.76496247838826,
61.1894447907506));
#198753=CARTESIAN_POINT('Ctrl Pts',(-0.00906168801186097,6.76926055599514,
61.1976532487642));
#198754=CARTESIAN_POINT('Ctrl Pts',(-0.184398206791257,6.76675682496721,
61.2058617067777));
#198755=CARTESIAN_POINT('Ctrl Pts',(-0.359398201402664,6.75744936590934,
61.2140701647912));
#198756=CARTESIAN_POINT('Ctrl Pts',(-0.437364520265389,6.75330268966333,
61.2177272120744));
#198757=CARTESIAN_POINT('Ctrl Pts',(-0.515264028797898,6.74780623484948,
61.2213842593576));
#198758=CARTESIAN_POINT('Ctrl Pts',(-0.593046898541615,6.74096316383128,
61.2250413066408));
#198759=CARTESIAN_POINT('Ctrl Pts',(-0.78147328718548,6.72438605419979,
61.2339003808167));
#198760=CARTESIAN_POINT('Ctrl Pts',(-0.969019035950057,6.69992049979116,
61.2427594549926));
#198761=CARTESIAN_POINT('Ctrl Pts',(-1.15504361701545,6.66769549715581,
61.2516185291685));
#198762=CARTESIAN_POINT('Ctrl Pts',(-1.34141770084286,6.63540995022377,
61.2604942477624));
#198763=CARTESIAN_POINT('Ctrl Pts',(-1.5262646500587,6.59533586513905,61.2693699663564));
#198764=CARTESIAN_POINT('Ctrl Pts',(-1.70895641178248,6.54765278421417,
61.2782456849503));
#198765=CARTESIAN_POINT('Ctrl Pts',(-1.89216952417524,6.49983362924904,
61.2871467323373));
#198766=CARTESIAN_POINT('Ctrl Pts',(-2.07321488906964,6.44436209174639,
61.2960477797243));
#198767=CARTESIAN_POINT('Ctrl Pts',(-2.25147890250826,6.3814678367567,61.3049488271113));
#198768=CARTESIAN_POINT('Ctrl Pts',(-2.42998526831839,6.31848807616463,
61.3138619755943));
#198769=CARTESIAN_POINT('Ctrl Pts',(-2.60570248706574,6.2480655324972,61.3227751240773));
#198770=CARTESIAN_POINT('Ctrl Pts',(-2.77803784061023,6.17047767649618,
61.3316882725603));
#198771=CARTESIAN_POINT('Ctrl Pts',(-2.95075582576348,6.09271755423898,
61.3406212106702));
#198772=CARTESIAN_POINT('Ctrl Pts',(-3.12007668965096,6.00776040569,61.3495541487801));
#198773=CARTESIAN_POINT('Ctrl Pts',(-3.28543062583687,5.91593057792374,
61.35848708689));
#198774=CARTESIAN_POINT('Ctrl Pts',(-3.44282359776378,5.82852189666068,
61.3669899487485));
#198775=CARTESIAN_POINT('Ctrl Pts',(-3.59662246647734,5.73488682059762,
61.3754928106071));
#198776=CARTESIAN_POINT('Ctrl Pts',(-3.74636103213043,5.63534098497461,
61.3839956724656));
#198777=CARTESIAN_POINT('Ctrl Pts',(-3.89071306068689,5.53937610616163,
61.3921926613473));
#198778=CARTESIAN_POINT('Ctrl Pts',(-4.03157407539767,5.4377291067025,61.4003896502289));
#198779=CARTESIAN_POINT('Ctrl Pts',(-4.1684661687206,5.33068277054936,61.4085866391106));
#198780=CARTESIAN_POINT('Ctrl Pts',(-4.30521276970425,5.2237502059186,61.4167749160275));
#198781=CARTESIAN_POINT('Ctrl Pts',(-4.43799856612345,5.11142995130479,
61.4249631929445));
#198782=CARTESIAN_POINT('Ctrl Pts',(-4.56637335098806,4.99404880026078,
61.4331514698614));
#198783=CARTESIAN_POINT('Ctrl Pts',(-4.69463793991919,4.87676840829905,
61.4413327180241));
#198784=CARTESIAN_POINT('Ctrl Pts',(-4.8184987922927,4.75443601332382,61.4495139661867));
#198785=CARTESIAN_POINT('Ctrl Pts',(-4.93753757986241,4.62741954521594,
61.4576952143494));
#198786=CARTESIAN_POINT('Ctrl Pts',(-5.05649851333387,4.50048614879242,
61.465871111788));
#198787=CARTESIAN_POINT('Ctrl Pts',(-5.17064341706586,4.36887504342546,
61.4740470092267));
#198788=CARTESIAN_POINT('Ctrl Pts',(-5.2795897143172,4.23299202083775,61.4822229066654));
#198789=CARTESIAN_POINT('Ctrl Pts',(-5.38848701873598,4.09717010444952,
61.4903951274267));
#198790=CARTESIAN_POINT('Ctrl Pts',(-5.49219014816907,3.95708037907291,
61.4985673481881));
#198791=CARTESIAN_POINT('Ctrl Pts',(-5.59035580617994,3.81316285520436,
61.5067395689495));
#198792=CARTESIAN_POINT('Ctrl Pts',(-5.68851400498286,3.66925626704143,
61.5149111687372));
#198793=CARTESIAN_POINT('Ctrl Pts',(-5.78113535964076,3.52152275299368,
61.5230827685248));
#198794=CARTESIAN_POINT('Ctrl Pts',(-5.86791885457339,3.37043280843012,
61.5312543683125));
#198795=CARTESIAN_POINT('Ctrl Pts',(-5.95470251620644,3.21934257364135,
61.5394259837968));
#198796=CARTESIAN_POINT('Ctrl Pts',(-6.0356481148912,3.0648962084235,61.5475975992811));
#198797=CARTESIAN_POINT('Ctrl Pts',(-6.11049980374545,2.90759026488032,
61.5557692147654));
#198798=CARTESIAN_POINT('Ctrl Pts',(-6.18536549273228,2.75025489910103,
61.5639423586548));
#198799=CARTESIAN_POINT('Ctrl Pts',(-6.25413484616501,2.59005921596141,
61.5721155025442));
#198800=CARTESIAN_POINT('Ctrl Pts',(-6.3165995158996,2.4275212781224,61.5802886464335));
#198801=CARTESIAN_POINT('Ctrl Pts',(-6.3790874324696,2.26492285020627,61.588464832038));
#198802=CARTESIAN_POINT('Ctrl Pts',(-6.43526586246192,2.09998076852402,
61.5966410176425));
#198803=CARTESIAN_POINT('Ctrl Pts',(-6.48497581727025,1.93322984909193,
61.604817203247));
#198804=CARTESIAN_POINT('Ctrl Pts',(-6.53474271347514,1.76628792103258,
61.6130027544489));
#198805=CARTESIAN_POINT('Ctrl Pts',(-6.57802623055246,1.59753336300356,
61.6211883056509));
#198806=CARTESIAN_POINT('Ctrl Pts',(-6.61471793604195,1.42751379208924,
61.6293738568529));
#198807=CARTESIAN_POINT('Ctrl Pts',(-6.65143212392997,1.25739004374022,
61.6375644236523));
#198808=CARTESIAN_POINT('Ctrl Pts',(-6.68154638808421,1.08600009285269,
61.6457549904517));
#198809=CARTESIAN_POINT('Ctrl Pts',(-6.70500403871336,0.913898156709823,
61.6539455572511));
#198810=CARTESIAN_POINT('Ctrl Pts',(-6.72849721039538,0.741535612969445,
61.6621485267229));
#198811=CARTESIAN_POINT('Ctrl Pts',(-6.7453135950495,0.568459289010249,
61.6703514961947));
#198812=CARTESIAN_POINT('Ctrl Pts',(-6.75544856672205,0.39522609019773,
61.6785544656666));
#198813=CARTESIAN_POINT('Ctrl Pts',(-6.76311924712526,0.264114080589015,
61.6847629050395));
#198814=CARTESIAN_POINT('Ctrl Pts',(-6.76696371925884,0.132912249167229,
61.6909713444125));
#198815=CARTESIAN_POINT('Ctrl Pts',(-6.76699974432514,0.00186018910577469,
61.6971797837854));
#198816=CARTESIAN_POINT('',(-6.76699994399638,-0.00056233818115236,61.3028202161899));
#198817=CARTESIAN_POINT('Ctrl Pts',(3.09910619832132,6.01563211736941,60.6513956954041));
#198818=CARTESIAN_POINT('Ctrl Pts',(2.93375330764824,6.10081787314654,60.6601451433064));
#198819=CARTESIAN_POINT('Ctrl Pts',(2.76488627843068,6.1791820703704,60.6688945912087));
#198820=CARTESIAN_POINT('Ctrl Pts',(2.59307866646699,6.25045854553998,60.677644039111));
#198821=CARTESIAN_POINT('Ctrl Pts',(2.42127244185368,6.3217344451504,60.6863934163613));
#198822=CARTESIAN_POINT('Ctrl Pts',(2.24652594672451,6.38592262741843,60.6951427936116));
#198823=CARTESIAN_POINT('Ctrl Pts',(2.06943269687102,6.44280508110568,60.7038921708619));
#198824=CARTESIAN_POINT('Ctrl Pts',(1.89234081822058,6.49968709436172,60.7126414803672));
#198825=CARTESIAN_POINT('Ctrl Pts',(1.7129024940557,6.5492634045955,60.7213907898726));
#198826=CARTESIAN_POINT('Ctrl Pts',(1.5317271662504,6.59136563150388,60.7301400993779));
#198827=CARTESIAN_POINT('Ctrl Pts',(1.3505531810732,6.63346754640713,60.7388893440452));
#198828=CARTESIAN_POINT('Ctrl Pts',(1.1676424971441,6.66809542395777,60.7476385887124));
#198829=CARTESIAN_POINT('Ctrl Pts',(0.983616340614309,6.69513165624669,
60.7563878333796));
#198830=CARTESIAN_POINT('Ctrl Pts',(0.799591486713858,6.7221676971596,60.7651370161153));
#198831=CARTESIAN_POINT('Ctrl Pts',(0.614451459526792,6.7416121586937,60.773886198851));
#198832=CARTESIAN_POINT('Ctrl Pts',(0.428825047910427,6.75339900185711,
60.7826353815867));
#198833=CARTESIAN_POINT('Ctrl Pts',(0.243199888597162,6.7651857655022,60.7913845052973));
#198834=CARTESIAN_POINT('Ctrl Pts',(0.0570886373920053,6.76931499599834,
60.8001336290078));
#198835=CARTESIAN_POINT('Ctrl Pts',(-0.128876626811089,6.76577266947847,
60.8088827527183));
#198836=CARTESIAN_POINT('Ctrl Pts',(-0.314840698188105,6.76223036567993,
60.8176318203099));
#198837=CARTESIAN_POINT('Ctrl Pts',(-0.500658497951205,6.75101660879223,
60.8263808879014));
#198838=CARTESIAN_POINT('Ctrl Pts',(-0.685698951926176,6.73216948296219,
60.835129955493));
#198839=CARTESIAN_POINT('Ctrl Pts',(-0.870738280459975,6.71332247176292,
60.8438789698715));
#198840=CARTESIAN_POINT('Ctrl Pts',(-1.05499998761279,6.68684221356183,
60.85262798425));
#198841=CARTESIAN_POINT('Ctrl Pts',(-1.23785829161464,6.65281863948514,
60.8613769986286));
#198842=CARTESIAN_POINT('Ctrl Pts',(-1.43007412917444,6.61705395368852,
60.8705737323277));
#198843=CARTESIAN_POINT('Ctrl Pts',(-1.62073882535828,6.57295372727781,
60.8797704660269));
#198844=CARTESIAN_POINT('Ctrl Pts',(-1.80913696091546,6.52068343478271,
60.8889671997261));
#198845=CARTESIAN_POINT('Ctrl Pts',(-1.98838356186138,6.4709521981519,60.8977171974398));
#198846=CARTESIAN_POINT('Ctrl Pts',(-2.16557827572553,6.41382586850884,
60.9064671951535));
#198847=CARTESIAN_POINT('Ctrl Pts',(-2.34011918621713,6.34949849943273,
60.9152171928671));
#198848=CARTESIAN_POINT('Ctrl Pts',(-2.51465655691111,6.28517243495545,
60.9239670131255));
#198849=CARTESIAN_POINT('Ctrl Pts',(-2.6865399629534,6.21364572242369,60.9327168333838));
#198850=CARTESIAN_POINT('Ctrl Pts',(-2.8551855538,6.13516132252216,60.9414666536421));
#198851=CARTESIAN_POINT('Ctrl Pts',(-3.0238279485869,6.05667841000506,60.9502163080796));
#198852=CARTESIAN_POINT('Ctrl Pts',(-3.18923239109273,5.97123819492085,
60.9589659625171));
#198853=CARTESIAN_POINT('Ctrl Pts',(-3.3508370596768,5.87913088810723,60.9677156169546));
#198854=CARTESIAN_POINT('Ctrl Pts',(-3.51243888042383,5.78702520443113,
60.9764651172035));
#198855=CARTESIAN_POINT('Ctrl Pts',(-3.67024081223675,5.68825280605793,
60.9852146174524));
#198856=CARTESIAN_POINT('Ctrl Pts',(-3.82370687544387,5.58314917682514,
60.9939641177014));
#198857=CARTESIAN_POINT('Ctrl Pts',(-3.97717043817798,5.47804726008034,
61.0027134753919));
#198858=CARTESIAN_POINT('Ctrl Pts',(-4.1262980372244,5.36661448084251,61.0114628330823));
#198859=CARTESIAN_POINT('Ctrl Pts',(-4.27058317206885,5.24922931204595,
61.0202121907728));
#198860=CARTESIAN_POINT('Ctrl Pts',(-4.41486614774807,5.13184589986815,
61.0289614175329));
#198861=CARTESIAN_POINT('Ctrl Pts',(-4.5543065819438,5.00851045723065,61.0377106442929));
#198862=CARTESIAN_POINT('Ctrl Pts',(-4.68843089001807,4.87964187103156,
61.046459871053));
#198863=CARTESIAN_POINT('Ctrl Pts',(-4.82255336917802,4.75077504207996,
61.0552089785089));
#198864=CARTESIAN_POINT('Ctrl Pts',(-4.95135966065103,4.61637541908127,
61.0639580859649));
#198865=CARTESIAN_POINT('Ctrl Pts',(-5.07441230869217,4.47689945401876,
61.0727071934208));
#198866=CARTESIAN_POINT('Ctrl Pts',(-5.19746344226367,4.33742520555575,
61.0814561931971));
#198867=CARTESIAN_POINT('Ctrl Pts',(-5.31476088454696,4.19287495491425,
61.0902051929735));
#198868=CARTESIAN_POINT('Ctrl Pts',(-5.42590627628765,4.04373961586825,
61.0989541927498));
#198869=CARTESIAN_POINT('Ctrl Pts',(-5.53706380672587,3.89458798906849,
61.1077041480445));
#198870=CARTESIAN_POINT('Ctrl Pts',(-5.64206777071792,3.74085050155394,
61.1164541033392));
#198871=CARTESIAN_POINT('Ctrl Pts',(-5.74056148163943,3.58304938223265,
61.1252040586339));
#198872=CARTESIAN_POINT('Ctrl Pts',(-5.83905138951818,3.42525435593393,
61.133953676075));
#198873=CARTESIAN_POINT('Ctrl Pts',(-5.93103139557587,3.26339625497302,
61.1427032935161));
#198874=CARTESIAN_POINT('Ctrl Pts',(-6.01618907820782,3.0980248506513,61.1514529109573));
#198875=CARTESIAN_POINT('Ctrl Pts',(-6.10134392544923,2.93265895249767,
61.1602022370731));
#198876=CARTESIAN_POINT('Ctrl Pts',(-6.17967677261775,2.76378023986162,
61.168951563189));
#198877=CARTESIAN_POINT('Ctrl Pts',(-6.25092157009171,2.59196229227244,
61.1777008893049));
#198878=CARTESIAN_POINT('Ctrl Pts',(-6.32216437407705,2.42014915229216,
61.1864499706073));
#198879=CARTESIAN_POINT('Ctrl Pts',(-6.38631941548879,2.24539720662972,
61.1951990519098));
#198880=CARTESIAN_POINT('Ctrl Pts',(-6.443168810375,2.06829994947804,61.2039481332122));
#198881=CARTESIAN_POINT('Ctrl Pts',(-6.50002334524539,1.89118668024562,
61.2126980055546));
#198882=CARTESIAN_POINT('Ctrl Pts',(-6.54957082411068,1.71172794807809,
61.2214478778969));
#198883=CARTESIAN_POINT('Ctrl Pts',(-6.5916429429606,1.5305333425044,61.2301977502393));
#198884=CARTESIAN_POINT('Ctrl Pts',(-6.63371214082117,1.34935131693687,
61.2389470150942));
#198885=CARTESIAN_POINT('Ctrl Pts',(-6.66830695239677,1.16643393829838,
61.2476962799491));
#198886=CARTESIAN_POINT('Ctrl Pts',(-6.69530988153979,0.982402458341598,
61.256445544804));
#198887=CARTESIAN_POINT('Ctrl Pts',(-6.72231419690476,0.798361530947682,
61.265195258811));
#198888=CARTESIAN_POINT('Ctrl Pts',(-6.74172580829272,0.613206671363114,
61.2739449728181));
#198889=CARTESIAN_POINT('Ctrl Pts',(-6.75347878028175,0.42756679511405,
61.2826946868251));
#198890=CARTESIAN_POINT('Ctrl Pts',(-6.76248992368214,0.285234494205772,
61.2894031966134));
#198891=CARTESIAN_POINT('Ctrl Pts',(-6.76699999999997,0.142617266092478,
61.2961117064016));
#198892=CARTESIAN_POINT('Ctrl Pts',(-6.767,1.6338561345563E-12,61.3028202161899));
#198893=CARTESIAN_POINT('Ctrl Pts',(-6.76699986576577,-0.00134785983437084,
61.3028202161899));
#198894=CARTESIAN_POINT('Ctrl Pts',(-6.76696237706181,-0.189561832946977,
61.3116407746007));
#198895=CARTESIAN_POINT('Ctrl Pts',(-6.759067555259,-0.377645677084734,
61.3204613330115));
#198896=CARTESIAN_POINT('Ctrl Pts',(-6.74337774695477,-0.564929696400553,
61.3292818914223));
#198897=CARTESIAN_POINT('Ctrl Pts',(-6.72825252948937,-0.7454743827994,
61.3377850459251));
#198898=CARTESIAN_POINT('Ctrl Pts',(-6.70588363470456,-0.9252754993788,
61.3462882004278));
#198899=CARTESIAN_POINT('Ctrl Pts',(-6.67637932502589,-1.10374277273595,
61.3547913549306));
#198900=CARTESIAN_POINT('Ctrl Pts',(-6.64684860413504,-1.28236980367006,
61.3633021211558));
#198901=CARTESIAN_POINT('Ctrl Pts',(-6.61016978531227,-1.45966029532048,
61.3718128873811));
#198902=CARTESIAN_POINT('Ctrl Pts',(-6.56650166905042,-1.6350366449588,
61.3803236536064));
#198903=CARTESIAN_POINT('Ctrl Pts',(-6.5227698219134,-1.81066894537313,
61.3888468407608));
#198904=CARTESIAN_POINT('Ctrl Pts',(-6.47202838418072,-1.98438121467708,
61.3973700279153));
#198905=CARTESIAN_POINT('Ctrl Pts',(-6.41448557730058,-2.1556121586693,
61.4058932150697));
#198906=CARTESIAN_POINT('Ctrl Pts',(-6.4082435225972,-2.17418672910234,
61.4068177824196));
#198907=CARTESIAN_POINT('Ctrl Pts',(-6.4019214808727,-2.1927321220714,61.4077423497696));
#198908=CARTESIAN_POINT('Ctrl Pts',(-6.39551975129775,-2.21124763668847,
61.4086669171195));
#198909=CARTESIAN_POINT('Ctrl Pts',(-6.33707951056536,-2.3802724476926,
61.4171071265771));
#198910=CARTESIAN_POINT('Ctrl Pts',(-6.27189122696682,-2.54710435637577,
61.4255473360348));
#198911=CARTESIAN_POINT('Ctrl Pts',(-6.20014143025623,-2.7111870545612,
61.4339875454924));
#198912=CARTESIAN_POINT('Ctrl Pts',(-6.12844599464654,-2.87514543579355,
61.4424213602409));
#198913=CARTESIAN_POINT('Ctrl Pts',(-6.05019908904357,-3.03635845426718,
61.4508551749895));
#198914=CARTESIAN_POINT('Ctrl Pts',(-5.96563598925893,-3.19428806522809,
61.459288989738));
#198915=CARTESIAN_POINT('Ctrl Pts',(-5.88112395892767,-3.35212229914009,
61.4677177111265));
#198916=CARTESIAN_POINT('Ctrl Pts',(-5.79030349615835,-3.50667678551837,
61.4761464325151));
#198917=CARTESIAN_POINT('Ctrl Pts',(-5.69345678670816,-3.65743609894784,
61.4845751539036));
#198918=CARTESIAN_POINT('Ctrl Pts',(-5.59665369346201,-3.80812751591481,
61.4930000793053));
#198919=CARTESIAN_POINT('Ctrl Pts',(-5.49382994488778,-3.95502688778638,
61.5014250047071));
#198920=CARTESIAN_POINT('Ctrl Pts',(-5.38531240739392,-4.0976455770075,
61.5098499301088));
#198921=CARTESIAN_POINT('Ctrl Pts',(-5.27682709241016,-4.24022191793856,
61.5182723538665));
#198922=CARTESIAN_POINT('Ctrl Pts',(-5.16265156180884,-4.37851984591891,
61.5266947776243));
#198923=CARTESIAN_POINT('Ctrl Pts',(-5.04315475927423,-4.51208145693422,
61.5351172013821));
#198924=CARTESIAN_POINT('Ctrl Pts',(-4.92365607739932,-4.64564516848874,
61.5435397576003));
#198925=CARTESIAN_POINT('Ctrl Pts',(-4.79883617372676,-4.77447216134442,
61.5519623138185));
#198926=CARTESIAN_POINT('Ctrl Pts',(-4.66910331208577,-4.89813875477918,
61.5603848700367));
#198927=CARTESIAN_POINT('Ctrl Pts',(-4.53936606804406,-5.02180952569497,
61.5688077107704));
#198928=CARTESIAN_POINT('Ctrl Pts',(-4.40471577645939,-5.14031931932873,
61.5772305515042));
#198929=CARTESIAN_POINT('Ctrl Pts',(-4.26559659618971,-5.253282276689,61.5856533922379));
#198930=CARTESIAN_POINT('Ctrl Pts',(-4.12645329387145,-5.36626482083765,
61.5940776934186));
#198931=CARTESIAN_POINT('Ctrl Pts',(-3.98283981695724,-5.47369840096132,
61.6025019945992));
#198932=CARTESIAN_POINT('Ctrl Pts',(-3.83523262147287,-5.57523808811699,
61.6109262957798));
#198933=CARTESIAN_POINT('Ctrl Pts',(-3.68757921828049,-5.67680956177331,
61.6193532341466));
#198934=CARTESIAN_POINT('Ctrl Pts',(-3.53592987864075,-5.77248327495003,
61.6277801725134));
#198935=CARTESIAN_POINT('Ctrl Pts',(-3.38078948463484,-5.86195798864019,
61.6362071108802));
#198936=CARTESIAN_POINT('Ctrl Pts',(-3.22550959991312,-5.95151315134518,
61.6446416261238));
#198937=CARTESIAN_POINT('Ctrl Pts',(-3.06673267804151,-6.03485801066074,
61.6530761413674));
#198938=CARTESIAN_POINT('Ctrl Pts',(-2.90498863006585,-6.11173707379401,
61.6615106566111));
#198939=CARTESIAN_POINT('Ctrl Pts',(-2.74316645832919,-6.18865327017347,
61.6699492457979));
#198940=CARTESIAN_POINT('Ctrl Pts',(-2.57837460676043,-6.25909730608732,
61.6783878349847));
#198941=CARTESIAN_POINT('Ctrl Pts',(-2.41116284016113,-6.32286191200046,
61.6868264241714));
#198942=CARTESIAN_POINT('Ctrl Pts',(-2.24376416863754,-6.38669779231661,
61.6952744457917));
#198943=CARTESIAN_POINT('Ctrl Pts',(-2.07394049172099,-6.44383921289698,
61.7037224674121));
#198944=CARTESIAN_POINT('Ctrl Pts',(-1.90225776955778,-6.49412845408505,
61.7121704890324));
#198945=CARTESIAN_POINT('Ctrl Pts',(-1.80467606550361,-6.5227120517173,
61.7169722089446));
#198946=CARTESIAN_POINT('Ctrl Pts',(-1.70649401278955,-6.54908290613419,
61.7217739288568));
#198947=CARTESIAN_POINT('Ctrl Pts',(-1.60781698503205,-6.57321941993742,
61.726575648769));
#198948=CARTESIAN_POINT('Ctrl Pts',(-1.43849171658337,-6.6146365741832,
61.7348151806199));
#198949=CARTESIAN_POINT('Ctrl Pts',(-1.2673304742322,-6.64956423790568,
61.7430547124707));
#198950=CARTESIAN_POINT('Ctrl Pts',(-1.09487015751772,-6.67784009528359,
61.7512942443215));
#198951=CARTESIAN_POINT('Ctrl Pts',(-0.922601259701609,-6.706084568436,
61.7595246308678));
#198952=CARTESIAN_POINT('Ctrl Pts',(-0.749036506673693,-6.72769187903942,
61.7677550174141));
#198953=CARTESIAN_POINT('Ctrl Pts',(-0.574726585545867,-6.74254984051781,
61.7759854039605));
#198954=CARTESIAN_POINT('Ctrl Pts',(-0.400579040960036,-6.75739396122117,
61.7842081235783));
#198955=CARTESIAN_POINT('Ctrl Pts',(-0.225688063228557,-6.76550122398285,
61.7924308431961));
#198956=CARTESIAN_POINT('Ctrl Pts',(-0.0506132254557434,-6.76681071860363,
61.8006535628139));
#198957=CARTESIAN_POINT('Ctrl Pts',(0.124306483397012,-6.76811905291783,
61.8088689965097));
#198958=CARTESIAN_POINT('Ctrl Pts',(0.299409373049765,-6.76264162146797,
61.8170844302054));
#198959=CARTESIAN_POINT('Ctrl Pts',(0.474132201514215,-6.75036944585163,
61.8252998639012));
#198960=CARTESIAN_POINT('Ctrl Pts',(0.648765236012361,-6.73810357718061,
61.833511075502));
#198961=CARTESIAN_POINT('Ctrl Pts',(0.823018244159236,-6.71904994378684,
61.8417222871029));
#198962=CARTESIAN_POINT('Ctrl Pts',(0.996329019139121,-6.69325163770355,
61.8499334987037));
#198963=CARTESIAN_POINT('Ctrl Pts',(1.16958167524828,-6.66746198294859,
61.8581419567172));
#198964=CARTESIAN_POINT('Ctrl Pts',(1.3418923759856,-6.63493221353315,61.8663504147307));
#198965=CARTESIAN_POINT('Ctrl Pts',(1.51270497212881,-6.59575717164427,
61.8745588727443));
#198966=CARTESIAN_POINT('Ctrl Pts',(1.58880571353783,-6.57830383506496,
61.8782159200274));
#198967=CARTESIAN_POINT('Ctrl Pts',(1.66460920161152,-6.55953216383277,
61.8818729673106));
#198968=CARTESIAN_POINT('Ctrl Pts',(1.74006688801004,-6.53945381704398,
61.8855300145937));
#198969=CARTESIAN_POINT('Ctrl Pts',(1.9228605981222,-6.49081469653002,61.8943890887696));
#198970=CARTESIAN_POINT('Ctrl Pts',(2.10343416063342,-6.43455494400628,
61.9032481629455));
#198971=CARTESIAN_POINT('Ctrl Pts',(2.28117865088128,-6.37091147032852,
61.9121072371214));
#198972=CARTESIAN_POINT('Ctrl Pts',(2.45925708726672,-6.30714842336785,
61.9209829557153));
#198973=CARTESIAN_POINT('Ctrl Pts',(2.63449558509462,-6.23597401919902,
61.9298586743092));
#198974=CARTESIAN_POINT('Ctrl Pts',(2.80630617645485,-6.15767282696892,
61.9387343929031));
#198975=CARTESIAN_POINT('Ctrl Pts',(2.97860706669801,-6.07914818526007,
61.9476354402901));
#198976=CARTESIAN_POINT('Ctrl Pts',(3.14746023740388,-5.99345616483172,
61.9565364876771));
#198977=CARTESIAN_POINT('Ctrl Pts',(3.3123005496344,-5.9009282379039,61.9654375350641));
#198978=CARTESIAN_POINT('Ctrl Pts',(3.47736496453052,-5.80827451799022,
61.9743506835471));
#198979=CARTESIAN_POINT('Ctrl Pts',(3.63840540035195,-5.7087664597678,61.9832638320301));
#198980=CARTESIAN_POINT('Ctrl Pts',(3.79488549142437,-5.60277905212911,
61.9921769805131));
#198981=CARTESIAN_POINT('Ctrl Pts',(3.95171301108731,-5.49655632346399,
62.0011099186229));
#198982=CARTESIAN_POINT('Ctrl Pts',(4.10395971820272,-5.38382561686846,
62.0100428567328));
#198983=CARTESIAN_POINT('Ctrl Pts',(4.25111985689851,-5.26500417495401,
62.0189757948427));
#198984=CARTESIAN_POINT('Ctrl Pts',(4.39119497160725,-5.15190339064156,
62.0274786567013));
#198985=CARTESIAN_POINT('Ctrl Pts',(4.52666163290563,-5.03328466039966,
62.0359815185599));
#198986=CARTESIAN_POINT('Ctrl Pts',(4.65711466349043,-4.90953887968131,
62.0444843804185));
#198987=CARTESIAN_POINT('Ctrl Pts',(4.78326974701439,-4.7898700668352,62.0527071042844));
#198988=CARTESIAN_POINT('Ctrl Pts',(4.90497722864513,-4.66517639283559,
62.0609298281503));
#198989=CARTESIAN_POINT('Ctrl Pts',(5.02181355715097,-4.53582160112307,
62.0691525520162));
#198990=CARTESIAN_POINT('Ctrl Pts',(5.13852621836105,-4.40660372707556,
62.0773665724074));
#198991=CARTESIAN_POINT('Ctrl Pts',(5.25037775515071,-4.27273482376444,
62.0855805927986));
#198992=CARTESIAN_POINT('Ctrl Pts',(5.35697957741249,-4.13461712945534,
62.0937946131898));
#198993=CARTESIAN_POINT('Ctrl Pts',(5.46348996788871,-3.99661789791863,
62.1020015884618));
#198994=CARTESIAN_POINT('Ctrl Pts',(5.56475939331671,-3.85437741541928,
62.1102085637338));
#198995=CARTESIAN_POINT('Ctrl Pts',(5.66043781350638,-3.70833288142086,
62.1184155390057));
#198996=CARTESIAN_POINT('Ctrl Pts',(5.75605337488338,-3.56238429576674,
62.1266171224587));
#198997=CARTESIAN_POINT('Ctrl Pts',(5.84608505167637,-3.41263693567997,
62.1348187059117));
#198998=CARTESIAN_POINT('Ctrl Pts',(5.93022457683854,-3.25955909108275,
62.1430202893647));
#198999=CARTESIAN_POINT('Ctrl Pts',(6.01432570856698,-3.10655109694012,
62.1512181303798));
#199000=CARTESIAN_POINT('Ctrl Pts',(6.09253987263445,-2.95021595966294,
62.1594159713948));
#199001=CARTESIAN_POINT('Ctrl Pts',(6.16460340125909,-2.79104888978764,
62.1676138124099));
#199002=CARTESIAN_POINT('Ctrl Pts',(6.23666057050211,-2.63189586590981,
62.175810929991));
#199003=CARTESIAN_POINT('Ctrl Pts',(6.30256802977629,-2.46991173022405,
62.1840080475722));
#199004=CARTESIAN_POINT('Ctrl Pts',(6.3621090071535,-2.30561444762482,62.1922051651534));
#199005=CARTESIAN_POINT('Ctrl Pts',(6.42164932207101,-2.14131899301588,
62.2004021915324));
#199006=CARTESIAN_POINT('Ctrl Pts',(6.47482317290785,-1.97471077975065,
62.2085992179115));
#199007=CARTESIAN_POINT('Ctrl Pts',(6.52146275381584,-1.80632570445994,
62.2167962442906));
#199008=CARTESIAN_POINT('Ctrl Pts',(6.56811029629741,-1.6379118851252,62.2249946699368));
#199009=CARTESIAN_POINT('Ctrl Pts',(6.60822125080081,-1.46772094528846,
62.2331930955829));
#199010=CARTESIAN_POINT('Ctrl Pts',(6.64167828662358,-1.2963018695477,62.241391521229));
#199011=CARTESIAN_POINT('Ctrl Pts',(6.6751471172736,-1.12482236232115,62.2495928371197));
#199012=CARTESIAN_POINT('Ctrl Pts',(6.70195728778965,-0.952114208696751,
62.2577941530104));
#199013=CARTESIAN_POINT('Ctrl Pts',(6.7220429603744,-0.778734511166019,
62.265995468901));
#199014=CARTESIAN_POINT('Ctrl Pts',(6.74215150717799,-0.605157363182644,
62.2742061247176));
#199015=CARTESIAN_POINT('Ctrl Pts',(6.75552021523821,-0.430907500224963,
62.2824167805342));
#199016=CARTESIAN_POINT('Ctrl Pts',(6.76213524652309,-0.256546112288071,
62.2906274363508));
#199017=CARTESIAN_POINT('Ctrl Pts',(6.76875417588565,-0.0820819774095412,
62.2988429305079));
#199018=CARTESIAN_POINT('Ctrl Pts',(6.76861149569004,0.0924934552098535,
62.3070584246651));
#199019=CARTESIAN_POINT('Ctrl Pts',(6.76174549413847,0.266621215393907,
62.3152739188222));
#199020=CARTESIAN_POINT('Ctrl Pts',(6.75486883985914,0.441019138002136,
62.3235021594698));
#199021=CARTESIAN_POINT('Ctrl Pts',(6.74124804625857,0.614967642646063,
62.3317304001173));
#199022=CARTESIAN_POINT('Ctrl Pts',(6.72097321320831,0.787913743588968,
62.3399586407648));
#199023=CARTESIAN_POINT('Ctrl Pts',(6.7025466268647,0.945094138313558,62.3474367978658));
#199024=CARTESIAN_POINT('Ctrl Pts',(6.67862454825568,1.10144647497973,62.3549149549669));
#199025=CARTESIAN_POINT('Ctrl Pts',(6.64931066512028,1.25656542954104,62.3623931120679));
#199026=CARTESIAN_POINT('Ctrl Pts',(6.6176772789028,1.42395839404954,62.3704629890842));
#199027=CARTESIAN_POINT('Ctrl Pts',(6.57966065066864,1.59046289650428,62.3785328661005));
#199028=CARTESIAN_POINT('Ctrl Pts',(6.53531647488157,1.75554195994901,62.3866027431168));
#199029=CARTESIAN_POINT('Ctrl Pts',(6.4910282548947,1.92041271799784,62.3946624371402));
#199030=CARTESIAN_POINT('Ctrl Pts',(6.44042847067859,2.08386126021791,62.4027221311636));
#199031=CARTESIAN_POINT('Ctrl Pts',(6.38362437276625,2.2453571803668,62.410781825187));
#199032=CARTESIAN_POINT('Ctrl Pts',(6.32687948517417,2.40668476362619,62.4188331181077));
#199033=CARTESIAN_POINT('Ctrl Pts',(6.26394327721674,2.56606342631572,62.4268844110283));
#199034=CARTESIAN_POINT('Ctrl Pts',(6.19497368113208,2.72297449310141,62.434935703949));
#199035=CARTESIAN_POINT('Ctrl Pts',(6.12606086135194,2.87975638948426,62.4429803689831));
#199036=CARTESIAN_POINT('Ctrl Pts',(6.05112468911279,3.03407439342175,62.4510250340171));
#199037=CARTESIAN_POINT('Ctrl Pts',(5.97037237837069,3.18542660621593,62.4590696990512));
#199038=CARTESIAN_POINT('Ctrl Pts',(5.88966799418435,3.3366889913606,62.4671095895707));
#199039=CARTESIAN_POINT('Ctrl Pts',(5.80315451859122,3.48498876107766,62.4751494800902));
#199040=CARTESIAN_POINT('Ctrl Pts',(5.71108654476726,3.62984565486997,62.4831893706097));
#199041=CARTESIAN_POINT('Ctrl Pts',(5.61904760808922,3.7746568625177,62.4912267254431));
#199042=CARTESIAN_POINT('Ctrl Pts',(5.52145785861991,3.91602703986738,62.4992640802766));
#199043=CARTESIAN_POINT('Ctrl Pts',(5.41861692502185,4.05350214257582,62.50730143511));
#199044=CARTESIAN_POINT('Ctrl Pts',(5.31578805542593,4.19096111843793,62.5153378471023));
#199045=CARTESIAN_POINT('Ctrl Pts',(5.20770945131625,4.32452563004555,62.5233742590946));
#199046=CARTESIAN_POINT('Ctrl Pts',(5.09472290864114,4.45377227574191,62.5314106710869));
#199047=CARTESIAN_POINT('Ctrl Pts',(4.98172723908565,4.58302936178492,62.5394477322483));
#199048=CARTESIAN_POINT('Ctrl Pts',(4.86382308829119,4.70796760708525,62.5474847934097));
#199049=CARTESIAN_POINT('Ctrl Pts',(4.74139110618502,4.8281983573782,62.555521854571));
#199050=CARTESIAN_POINT('Ctrl Pts',(4.61886417636146,4.94852234830244,62.5635651485859));
#199051=CARTESIAN_POINT('Ctrl Pts',(4.49180266700234,5.06413128877575,62.5716084426008));
#199052=CARTESIAN_POINT('Ctrl Pts',(4.36062298791606,5.17467449771075,62.5796517366157));
#199053=CARTESIAN_POINT('Ctrl Pts',(4.22939315943916,5.28525996680834,62.5876981055451));
#199054=CARTESIAN_POINT('Ctrl Pts',(4.0940423186118,5.39077561596903,62.5957444744745));
#199055=CARTESIAN_POINT('Ctrl Pts',(3.95501784946542,5.49091274838801,62.6037908434039));
#199056=CARTESIAN_POINT('Ctrl Pts',(3.81581422947476,5.59117892033454,62.6118475811108));
#199057=CARTESIAN_POINT('Ctrl Pts',(3.67292783343855,5.68605252033276,62.6199043188176));
#199058=CARTESIAN_POINT('Ctrl Pts',(3.52683359618341,5.77526915258778,62.6279610565245));
#199059=CARTESIAN_POINT('Ctrl Pts',(3.38704947209315,5.86063233342477,62.6356698070169));
#199060=CARTESIAN_POINT('Ctrl Pts',(3.24432906216674,5.94081685794192,62.6433785575093));
#199061=CARTESIAN_POINT('Ctrl Pts',(3.09910619832141,6.01563211736936,62.6510873080018));
#199062=CARTESIAN_POINT('Origin',(0.,0.,4.30282021618968));
#199063=CARTESIAN_POINT('',(3.09910619832142,6.01563211736936,65.0458684084508));
#199064=CARTESIAN_POINT('',(3.09910619832139,6.01563211736938,64.6516994535812));
#199065=CARTESIAN_POINT('',(3.09910619832133,6.0156321173694,4.30282021618968));
#199066=CARTESIAN_POINT('',(-6.7669979781149,0.00523107913431084,63.6971797837701));
#199067=CARTESIAN_POINT('Ctrl Pts',(-6.76699797811555,0.00523107828453301,
63.69717978381));
#199068=CARTESIAN_POINT('Ctrl Pts',(-6.76713328191249,-0.169799856163699,
63.7053954717453));
#199069=CARTESIAN_POINT('Ctrl Pts',(-6.76047344531109,-0.344918086105988,
63.7136111596805));
#199070=CARTESIAN_POINT('Ctrl Pts',(-6.74702499707155,-0.519560091704129,
63.7218268476158));
#199071=CARTESIAN_POINT('Ctrl Pts',(-6.73301302667077,-0.70152001522752,
63.7303867925343));
#199072=CARTESIAN_POINT('Ctrl Pts',(-6.71163121841307,-0.882962538116192,
63.7389467374529));
#199073=CARTESIAN_POINT('Ctrl Pts',(-6.6829470971477,-1.06325307275606,
63.7475066823715));
#199074=CARTESIAN_POINT('Ctrl Pts',(-6.65542018410509,-1.23627011669901,
63.7557212920241));
#199075=CARTESIAN_POINT('Ctrl Pts',(-6.62116869467487,-1.40822592771657,
63.7639359016767));
#199076=CARTESIAN_POINT('Ctrl Pts',(-6.58030494640585,-1.57856764578107,
63.7721505113294));
#199077=CARTESIAN_POINT('Ctrl Pts',(-6.53943488854242,-1.74893566557253,
63.7803663893643));
#199078=CARTESIAN_POINT('Ctrl Pts',(-6.49195062043139,-1.91768874898435,
63.7885822673992));
#199079=CARTESIAN_POINT('Ctrl Pts',(-6.43801499756835,-2.08428690229655,
63.7967981454341));
#199080=CARTESIAN_POINT('Ctrl Pts',(-6.38406140330354,-2.2509405662748,
63.8050167610075));
#199081=CARTESIAN_POINT('Ctrl Pts',(-6.32365228135544,-2.41543753051153,
63.813235376581));
#199082=CARTESIAN_POINT('Ctrl Pts',(-6.25699953357942,-2.57725548535394,
63.8214539921544));
#199083=CARTESIAN_POINT('Ctrl Pts',(-6.19031265947404,-2.73915629128662,
63.8296768156741));
#199084=CARTESIAN_POINT('Ctrl Pts',(-6.11737592623212,-2.8983750258755,
63.8378996391938));
#199085=CARTESIAN_POINT('Ctrl Pts',(-6.03844831996388,-3.05441170884433,
63.8461224627135));
#199086=CARTESIAN_POINT('Ctrl Pts',(-5.95942328610895,-3.21064100220864,
63.8543554364188));
#199087=CARTESIAN_POINT('Ctrl Pts',(-5.87439277112278,-3.36368008137496,
63.8625884101241));
#199088=CARTESIAN_POINT('Ctrl Pts',(-5.78366093910566,-3.51305495850314,
63.8708213838294));
#199089=CARTESIAN_POINT('Ctrl Pts',(-5.69286329287895,-3.66253818778569,
63.8790603294923));
#199090=CARTESIAN_POINT('Ctrl Pts',(-5.59635628255329,-3.80835162114177,
63.8872992751553));
#199091=CARTESIAN_POINT('Ctrl Pts',(-5.49448584051031,-3.95005244882036,
63.8955382208182));
#199092=CARTESIAN_POINT('Ctrl Pts',(-5.3924709029499,-4.09195426840597,
63.9037888528024));
#199093=CARTESIAN_POINT('Ctrl Pts',(-5.28507755990454,-4.22973155355144,
63.9120394847866));
#199094=CARTESIAN_POINT('Ctrl Pts',(-5.17269082950643,-4.36297588605989,
63.9202901167709));
#199095=CARTESIAN_POINT('Ctrl Pts',(-5.14101877497245,-4.40052588640781,
63.9226152530678));
#199096=CARTESIAN_POINT('Ctrl Pts',(-5.10895036825335,-4.4377161192415,
63.9249403893648));
#199097=CARTESIAN_POINT('Ctrl Pts',(-5.07649472080399,-4.47453800404569,
63.9272655256617));
#199098=CARTESIAN_POINT('Ctrl Pts',(-4.96385846131697,-4.60232714700078,
63.9353348348842));
#199099=CARTESIAN_POINT('Ctrl Pts',(-4.84618732405444,-4.72609466676973,
63.9434041441068));
#199100=CARTESIAN_POINT('Ctrl Pts',(-4.72380322017864,-4.84540732416068,
63.9514734533293));
#199101=CARTESIAN_POINT('Ctrl Pts',(-4.60157176254317,-4.96457116623986,
63.95953269793));
#199102=CARTESIAN_POINT('Ctrl Pts',(-4.47463929844225,-5.0792909445658,
63.9675919425308));
#199103=CARTESIAN_POINT('Ctrl Pts',(-4.34336872409291,-5.18916535933974,
63.9756511871316));
#199104=CARTESIAN_POINT('Ctrl Pts',(-4.21223307271646,-5.29892684261506,
63.9837021482519));
#199105=CARTESIAN_POINT('Ctrl Pts',(-4.0767684679249,-5.40385263551516,
63.9917531093721));
#199106=CARTESIAN_POINT('Ctrl Pts',(-3.93737541017347,-5.50357737107068,
63.9998040704924));
#199107=CARTESIAN_POINT('Ctrl Pts',(-3.79809508008873,-5.60322145887422,
64.0078485207715));
#199108=CARTESIAN_POINT('Ctrl Pts',(-3.6548929221624,-5.69767264488414,
64.0158929710506));
#199109=CARTESIAN_POINT('Ctrl Pts',(-3.50820326619095,-5.78660512244331,
64.0239374213297));
#199110=CARTESIAN_POINT('Ctrl Pts',(-3.36160012967582,-5.875485146477,64.031977126888));
#199111=CARTESIAN_POINT('Ctrl Pts',(-3.21151390820272,-5.9588527488499,
64.0400168324462));
#199112=CARTESIAN_POINT('Ctrl Pts',(-3.05840863208465,-6.0364249054544,
64.0480565380045));
#199113=CARTESIAN_POINT('Ctrl Pts',(-2.90199866043684,-6.1156714155865,
64.056269776309));
#199114=CARTESIAN_POINT('Ctrl Pts',(-2.74243814764586,-6.18886922066618,
64.0644830146134));
#199115=CARTESIAN_POINT('Ctrl Pts',(-2.58024960638838,-6.25576541829476,
64.0726962529179));
#199116=CARTESIAN_POINT('Ctrl Pts',(-2.42153895868367,-6.32122712583771,
64.080733370466));
#199117=CARTESIAN_POINT('Ctrl Pts',(-2.26031221230842,-6.38065460705794,
64.0887704880142));
#199118=CARTESIAN_POINT('Ctrl Pts',(-2.09707992906674,-6.43385924396124,
64.0968076055624));
#199119=CARTESIAN_POINT('Ctrl Pts',(-1.93383037688703,-6.48706950957693,
64.1048455733865));
#199120=CARTESIAN_POINT('Ctrl Pts',(-1.76857522058572,-6.53405550412845,
64.1128835412106));
#199121=CARTESIAN_POINT('Ctrl Pts',(-1.60184062597471,-6.5746783654394,
64.1209215090347));
#199122=CARTESIAN_POINT('Ctrl Pts',(-1.43505535563428,-6.61531357327708,
64.1289619198425));
#199123=CARTESIAN_POINT('Ctrl Pts',(-1.26679011476239,-6.6495817099803,
64.1370023306502));
#199124=CARTESIAN_POINT('Ctrl Pts',(-1.09758156123894,-6.67739497981273,
64.1450427414579));
#199125=CARTESIAN_POINT('Ctrl Pts',(-0.921977878740528,-6.70625943437602,
64.1533870344457));
#199126=CARTESIAN_POINT('Ctrl Pts',(-0.745358626195725,-6.72817150190247,
64.1617313274335));
#199127=CARTESIAN_POINT('Ctrl Pts',(-0.568328641914355,-6.74309213601444,
64.1700756204213));
#199128=CARTESIAN_POINT('Ctrl Pts',(-0.397444479296954,-6.75749478128549,
64.1781302306368));
#199129=CARTESIAN_POINT('Ctrl Pts',(-0.226177995334895,-6.76538334120345,
64.1861848408523));
#199130=CARTESIAN_POINT('Ctrl Pts',(-0.0550718885309028,-6.7667759004635,
64.1942394510679));
#199131=CARTESIAN_POINT('Ctrl Pts',(0.116163748012738,-6.76816951391058,
64.2023001587371));
#199132=CARTESIAN_POINT('Ctrl Pts',(0.2872383948486,-6.76305734633575,64.2103608664064));
#199133=CARTESIAN_POINT('Ctrl Pts',(0.457615057850005,-6.75150927266111,
64.2184215740756));
#199134=CARTESIAN_POINT('Ctrl Pts',(0.628231941739058,-6.73994491689443,
64.2264936468598));
#199135=CARTESIAN_POINT('Ctrl Pts',(0.798148510376524,-6.7219265893989,
64.2345657196439));
#199136=CARTESIAN_POINT('Ctrl Pts',(0.966837950055704,-6.69757518646354,
64.2426377924281));
#199137=CARTESIAN_POINT('Ctrl Pts',(0.984506887198725,-6.69502456202239,
64.2434832807225));
#199138=CARTESIAN_POINT('Ctrl Pts',(1.00216237568927,-6.69240450255315,
64.2443287690169));
#199139=CARTESIAN_POINT('Ctrl Pts',(1.01980382053253,-6.68971517836352,
64.2451742573113));
#199140=CARTESIAN_POINT('Ctrl Pts',(1.19367350701362,-6.66320986897132,
64.253507179358));
#199141=CARTESIAN_POINT('Ctrl Pts',(1.36673248224403,-6.62988780120963,
64.2618401014047));
#199142=CARTESIAN_POINT('Ctrl Pts',(1.53841403349182,-6.58980813541301,
64.2701730234514));
#199143=CARTESIAN_POINT('Ctrl Pts',(1.70989269877938,-6.5497758340619,64.278496098005));
#199144=CARTESIAN_POINT('Ctrl Pts',(1.87999684680696,-6.50300192152489,
64.2868191725586));
#199145=CARTESIAN_POINT('Ctrl Pts',(2.04816658128681,-6.44959709247794,
64.2951422471122));
#199146=CARTESIAN_POINT('Ctrl Pts',(2.216168448443,-6.39624557222493,64.3034570135582));
#199147=CARTESIAN_POINT('Ctrl Pts',(2.38223941952868,-6.33627642728021,
64.3117717800042));
#199148=CARTESIAN_POINT('Ctrl Pts',(2.54583124403592,-6.26985105699414,
64.3200865464502));
#199149=CARTESIAN_POINT('Ctrl Pts',(2.70928977914283,-6.20347980798093,
64.3283945382897));
#199150=CARTESIAN_POINT('Ctrl Pts',(2.87027287155391,-6.1306629456,64.3367025301292));
#199151=CARTESIAN_POINT('Ctrl Pts',(3.02824864419703,-6.05161128534532,
64.3450105219688));
#199152=CARTESIAN_POINT('Ctrl Pts',(3.18612466549118,-5.97260954103419,
64.3533132678558));
#199153=CARTESIAN_POINT('Ctrl Pts',(3.34099684106431,-5.88738099982339,
64.3616160137429));
#199154=CARTESIAN_POINT('Ctrl Pts',(3.49235424968499,-5.79618415810844,
64.36991875963));
#199155=CARTESIAN_POINT('Ctrl Pts',(3.64364980335661,-5.7050245856362,64.3782181124494));
#199156=CARTESIAN_POINT('Ctrl Pts',(3.79143315461349,-5.60790175193272,
64.3865174652688));
#199157=CARTESIAN_POINT('Ctrl Pts',(3.93521867601476,-5.50511970550547,
64.3948168180883));
#199158=CARTESIAN_POINT('Ctrl Pts',(4.07897361664801,-5.40235951909506,
64.4031144057746));
#199159=CARTESIAN_POINT('Ctrl Pts',(4.21873213849263,-5.29394272004307,
64.411411993461));
#199160=CARTESIAN_POINT('Ctrl Pts',(4.35403806620837,-5.18021635822371,
64.4197095811473));
#199161=CARTESIAN_POINT('Ctrl Pts',(4.48933770112075,-5.066495285586,64.4280067829297));
#199162=CARTESIAN_POINT('Ctrl Pts',(4.62018488836009,-4.9474653662196,64.4363039847121));
#199163=CARTESIAN_POINT('Ctrl Pts',(4.74615684040595,-4.82351368260398,
64.4446011864945));
#199164=CARTESIAN_POINT('Ctrl Pts',(4.87214386623956,-4.69954716694567,
64.4528993811191));
#199165=CARTESIAN_POINT('Ctrl Pts',(4.99325424689754,-4.57065795793107,
64.4611975757436));
#199166=CARTESIAN_POINT('Ctrl Pts',(5.1091022123032,-4.43726983450844,64.4694957703681));
#199167=CARTESIAN_POINT('Ctrl Pts',(5.225031654934,-4.30378789766299,64.4777998012097));
#199168=CARTESIAN_POINT('Ctrl Pts',(5.3356910583431,-4.16580098682759,64.4861038320513));
#199169=CARTESIAN_POINT('Ctrl Pts',(5.44073453503616,-4.02376648418679,
64.4944078628929));
#199170=CARTESIAN_POINT('Ctrl Pts',(5.54581620842777,-3.88168033389254,
64.5027149133086));
#199171=CARTESIAN_POINT('Ctrl Pts',(5.64527768402938,-3.73554394235127,
64.5110219637242));
#199172=CARTESIAN_POINT('Ctrl Pts',(5.73881644959561,-3.58584366054223,
64.5193290141399));
#199173=CARTESIAN_POINT('Ctrl Pts',(5.83245522388936,-3.43598332386606,
64.5276449461946));
#199174=CARTESIAN_POINT('Ctrl Pts',(5.92015845780619,-3.28255178282144,
64.5359608782492));
#199175=CARTESIAN_POINT('Ctrl Pts',(6.00166910580818,-3.12606093101009,
64.5442768103038));
#199176=CARTESIAN_POINT('Ctrl Pts',(6.06311356361502,-3.00809480293999,
64.5505455365228));
#199177=CARTESIAN_POINT('Ctrl Pts',(6.12104004933156,-2.88839075719545,
64.5568142627418));
#199178=CARTESIAN_POINT('Ctrl Pts',(6.17535661332451,-2.76717540070542,
64.5630829889607));
#199179=CARTESIAN_POINT('Ctrl Pts',(6.24857556496458,-2.60377660165715,
64.5715332576841));
#199180=CARTESIAN_POINT('Ctrl Pts',(6.31536746712272,-2.43733129013988,
64.5799835264075));
#199181=CARTESIAN_POINT('Ctrl Pts',(6.37548252872376,-2.26837199902002,
64.5884337951309));
#199182=CARTESIAN_POINT('Ctrl Pts',(6.43554453674333,-2.09956182020709,
64.5968766062054));
#199183=CARTESIAN_POINT('Ctrl Pts',(6.48894133846522,-1.92824239494811,
64.60531941728));
#199184=CARTESIAN_POINT('Ctrl Pts',(6.53547094308591,-1.75496682364076,
64.6137622283545));
#199185=CARTESIAN_POINT('Ctrl Pts',(6.58196581887717,-1.58182058198945,
64.6221987378723));
#199186=CARTESIAN_POINT('Ctrl Pts',(6.62160362934667,-1.40672142396835,
64.63063524739));
#199187=CARTESIAN_POINT('Ctrl Pts',(6.65423188485467,-1.23023860392345,
64.6390717569077));
#199188=CARTESIAN_POINT('Ctrl Pts',(6.68683679309019,-1.05388206683248,
64.647502229649));
#199189=CARTESIAN_POINT('Ctrl Pts',(6.71244209087706,-0.876144167867102,
64.6559327023902));
#199190=CARTESIAN_POINT('Ctrl Pts',(6.73094610410198,-0.697605578872706,
64.6643631751315));
#199191=CARTESIAN_POINT('Ctrl Pts',(6.74944216250176,-0.519143743133937,
64.6727900236353));
#199192=CARTESIAN_POINT('Ctrl Pts',(6.76084298812794,-0.339882232780162,
64.6812168721391));
#199193=CARTESIAN_POINT('Ctrl Pts',(6.76509852362996,-0.160408745334515,
64.689643720643));
#199194=CARTESIAN_POINT('Ctrl Pts',(6.76935274560013,0.0190093450545052,
64.6980679680796));
#199195=CARTESIAN_POINT('Ctrl Pts',(6.76646606787668,0.198638950950581,
64.7064922155163));
#199196=CARTESIAN_POINT('Ctrl Pts',(6.75644048928006,0.3778900829832,64.7149164629529));
#199197=CARTESIAN_POINT('Ctrl Pts',(6.75361566481618,0.428396193734256,
64.7172900935638));
#199198=CARTESIAN_POINT('Ctrl Pts',(6.75022440287827,0.478872257101879,
64.7196637241747));
#199199=CARTESIAN_POINT('Ctrl Pts',(6.74626749549761,0.529305090843154,
64.7220373547856));
#199200=CARTESIAN_POINT('Ctrl Pts',(6.73189975110381,0.712429433805857,
64.7306561357227));
#199201=CARTESIAN_POINT('Ctrl Pts',(6.71007669283438,0.894901562660722,
64.7392749166599));
#199202=CARTESIAN_POINT('Ctrl Pts',(6.6808886211682,1.07611162596884,64.747893697597));
#199203=CARTESIAN_POINT('Ctrl Pts',(6.6516830164047,1.25743054106107,64.7565176557835));
#199204=CARTESIAN_POINT('Ctrl Pts',(6.61510361741735,1.43748557733641,64.76514161397));
#199205=CARTESIAN_POINT('Ctrl Pts',(6.57129186811685,1.61567700485629,64.7737655721564));
#199206=CARTESIAN_POINT('Ctrl Pts',(6.52589734979804,1.80030588067048,64.7827010845276));
#199207=CARTESIAN_POINT('Ctrl Pts',(6.4727382702726,1.98293363628355,64.7916365968987));
#199208=CARTESIAN_POINT('Ctrl Pts',(6.41202819173572,2.16291087851218,64.8005721092699));
#199209=CARTESIAN_POINT('Ctrl Pts',(6.35332534084163,2.33693762117996,64.8092121911645));
#199210=CARTESIAN_POINT('Ctrl Pts',(6.28756296160559,2.5084860426836,64.8178522730591));
#199211=CARTESIAN_POINT('Ctrl Pts',(6.21498321831187,2.67698946507115,64.8264923549537));
#199212=CARTESIAN_POINT('Ctrl Pts',(6.1386808943046,2.85413534831456,64.8355755825631));
#199213=CARTESIAN_POINT('Ctrl Pts',(6.05484368962889,3.02791532052571,64.8446588101726));
#199214=CARTESIAN_POINT('Ctrl Pts',(5.96380790906726,3.19769983327811,64.853742037782));
#199215=CARTESIAN_POINT('Ctrl Pts',(5.87277212850563,3.36748434603051,64.8628252653914));
#199216=CARTESIAN_POINT('Ctrl Pts',(5.77453799868445,3.53327308287001,64.8719084930009));
#199217=CARTESIAN_POINT('Ctrl Pts',(5.66949500109843,3.69447092728038,64.8809917206103));
#199218=CARTESIAN_POINT('Ctrl Pts',(5.56489877199312,3.85498316562754,64.8900363154704));
#199219=CARTESIAN_POINT('Ctrl Pts',(5.45345561315619,4.01109218780394,64.8990809103304));
#199220=CARTESIAN_POINT('Ctrl Pts',(5.3355436438952,4.16224254748441,64.9081255051905));
#199221=CARTESIAN_POINT('Ctrl Pts',(5.21773987742674,4.31325420291703,64.917161800211));
#199222=CARTESIAN_POINT('Ctrl Pts',(5.09347929828821,4.4593160932476,64.9261980952316));
#199223=CARTESIAN_POINT('Ctrl Pts',(4.96318175308897,4.59990389962711,64.9352343902522));
#199224=CARTESIAN_POINT('Ctrl Pts',(4.83311477961333,4.74024292485895,64.9442546948401));
#199225=CARTESIAN_POINT('Ctrl Pts',(4.69703233393514,4.87512703523263,64.953274999428));
#199226=CARTESIAN_POINT('Ctrl Pts',(4.55539258376835,5.00406708665545,64.9622953040159));
#199227=CARTESIAN_POINT('Ctrl Pts',(4.4139312013527,5.13284476313072,64.9713042492825));
#199228=CARTESIAN_POINT('Ctrl Pts',(4.2669266561315,5.2556931592491,64.980313194549));
#199229=CARTESIAN_POINT('Ctrl Pts',(4.11487362009876,5.37216009540067,64.9893221398155));
#199230=CARTESIAN_POINT('Ctrl Pts',(3.96316586432145,5.48836255979612,64.9983106276745));
#199231=CARTESIAN_POINT('Ctrl Pts',(3.80643268948294,5.59821234500969,65.0072991155336));
#199232=CARTESIAN_POINT('Ctrl Pts',(3.64520105873866,5.70129794357132,65.0162876033926));
#199233=CARTESIAN_POINT('Ctrl Pts',(3.50374249300808,5.79174136867774,65.0241737644067));
#199234=CARTESIAN_POINT('Ctrl Pts',(3.35882177251838,5.87697844240007,65.0320599254209));
#199235=CARTESIAN_POINT('Ctrl Pts',(3.21081588693835,5.95675669640655,65.039946086435));
#199236=CARTESIAN_POINT('Ctrl Pts',(3.17376623700652,5.97672722914266,65.0419201937736));
#199237=CARTESIAN_POINT('Ctrl Pts',(3.13652736059032,5.99635365191914,65.0438943011122));
#199238=CARTESIAN_POINT('Ctrl Pts',(3.09910619832142,6.01563211736936,65.0458684084508));
#199239=CARTESIAN_POINT('Ctrl Pts',(3.09910619832125,6.01563211736945,63.0457521963359));
#199240=CARTESIAN_POINT('Ctrl Pts',(2.93989560984711,6.09765350962745,63.0541775957781));
#199241=CARTESIAN_POINT('Ctrl Pts',(2.77736734802791,6.17338115804527,63.0626029952203));
#199242=CARTESIAN_POINT('Ctrl Pts',(2.61204854936917,6.24255487566897,63.0710283946625));
#199243=CARTESIAN_POINT('Ctrl Pts',(2.44678254603495,6.31170650234537,63.0794511034144));
#199244=CARTESIAN_POINT('Ctrl Pts',(2.27872809028716,6.37430824348362,63.0878738121662));
#199245=CARTESIAN_POINT('Ctrl Pts',(2.10843344773471,6.43014754080134,63.0962965209181));
#199246=CARTESIAN_POINT('Ctrl Pts',(1.93814073881744,6.48598620408367,63.104719134033));
#199247=CARTESIAN_POINT('Ctrl Pts',(1.76560820845957,6.53506246626283,63.113141747148));
#199248=CARTESIAN_POINT('Ctrl Pts',(1.59140111308797,6.57721304940492,63.121564360263));
#199249=CARTESIAN_POINT('Ctrl Pts',(1.41719168729634,6.61936419640787,63.1299870860498));
#199250=CARTESIAN_POINT('Ctrl Pts',(1.24130797598144,6.65458940095232,63.1384098118365));
#199251=CARTESIAN_POINT('Ctrl Pts',(1.06432747400704,6.68277607196843,63.1468325376233));
#199252=CARTESIAN_POINT('Ctrl Pts',(0.887319896724574,6.7109670551138,63.1552565519582));
#199253=CARTESIAN_POINT('Ctrl Pts',(0.709215523668136,6.73211730545359,
63.1636805662931));
#199254=CARTESIAN_POINT('Ctrl Pts',(0.530599419496047,6.74616581889524,
63.172104580628));
#199255=CARTESIAN_POINT('Ctrl Pts',(0.351931046830005,6.76021844335836,
63.1805310600852));
#199256=CARTESIAN_POINT('Ctrl Pts',(0.172750976923394,6.76716516146341,
63.1889575395424));
#199257=CARTESIAN_POINT('Ctrl Pts',(-0.0063528875793088,6.76699701794078,
63.1973840189996));
#199258=CARTESIAN_POINT('Ctrl Pts',(-0.185616827994484,6.76682872413816,
63.2058180297091));
#199259=CARTESIAN_POINT('Ctrl Pts',(-0.364804092962102,6.75953286179767,
63.2142520404186));
#199260=CARTESIAN_POINT('Ctrl Pts',(-0.543327885455411,6.74515261568532,
63.2226860511281));
#199261=CARTESIAN_POINT('Ctrl Pts',(-0.721934564639815,6.73076569297822,
63.2311239776587));
#199262=CARTESIAN_POINT('Ctrl Pts',(-0.899876825311956,6.70928786130205,
63.2395619041894));
#199263=CARTESIAN_POINT('Ctrl Pts',(-1.07657472139828,6.6808140124723,63.24799983072));
#199264=CARTESIAN_POINT('Ctrl Pts',(-1.25347601309279,6.6523073876111,63.2564474700839));
#199265=CARTESIAN_POINT('Ctrl Pts',(-1.42912974948983,6.6167887129663,63.2648951094477));
#199266=CARTESIAN_POINT('Ctrl Pts',(-1.60296658039716,6.57440393816275,
63.2733427488116));
#199267=CARTESIAN_POINT('Ctrl Pts',(-1.72715789565616,6.54412369834052,
63.2793778533286));
#199268=CARTESIAN_POINT('Ctrl Pts',(-1.85042214059953,6.51034016194635,
63.2854129578456));
#199269=CARTESIAN_POINT('Ctrl Pts',(-1.97255701527909,6.47312195323657,
63.2914480623626));
#199270=CARTESIAN_POINT('Ctrl Pts',(-2.13930378613897,6.42230914374357,
63.2996875942134));
#199271=CARTESIAN_POINT('Ctrl Pts',(-2.30431693438982,6.36497875493986,
63.3079271260642));
#199272=CARTESIAN_POINT('Ctrl Pts',(-2.46705191850273,6.30126525639193,
63.316166657915));
#199273=CARTESIAN_POINT('Ctrl Pts',(-2.62960627815627,6.23762247537466,
63.3243970444613));
#199274=CARTESIAN_POINT('Ctrl Pts',(-2.78988718005324,6.16761082026071,
63.3326274310076));
#199275=CARTESIAN_POINT('Ctrl Pts',(-2.94736381379206,6.09141490535238,
63.3408578175538));
#199276=CARTESIAN_POINT('Ctrl Pts',(-3.10469375185753,6.01528996993338,
63.3490805371716));
#199277=CARTESIAN_POINT('Ctrl Pts',(-3.25922430568567,5.93299240171641,
63.3573032567893));
#199278=CARTESIAN_POINT('Ctrl Pts',(-3.41044319650045,5.84475544428027,
63.3655259764071));
#199279=CARTESIAN_POINT('Ctrl Pts',(-3.5615280964841,5.75659667114504,63.3737414101029));
#199280=CARTESIAN_POINT('Ctrl Pts',(-3.70930687570434,5.66250917658713,
63.3819568437987));
#199281=CARTESIAN_POINT('Ctrl Pts',(-3.85329060785493,5.56277273411534,
63.3901722774944));
#199282=CARTESIAN_POINT('Ctrl Pts',(-3.99720034354836,5.46308754842986,
63.3983834890953));
#199283=CARTESIAN_POINT('Ctrl Pts',(-4.13731862462951,5.35775939881728,
63.4065947006961));
#199284=CARTESIAN_POINT('Ctrl Pts',(-4.27318399314307,5.24711230685468,
63.414805912297));
#199285=CARTESIAN_POINT('Ctrl Pts',(-4.40900379990856,5.13650231982164,
63.4230143703105));
#199286=CARTESIAN_POINT('Ctrl Pts',(-4.54057325953186,5.02057716818818,
63.4312228283241));
#199287=CARTESIAN_POINT('Ctrl Pts',(-4.66746253781183,4.89970228260077,
63.4394312863376));
#199288=CARTESIAN_POINT('Ctrl Pts',(-4.72399448201461,4.8458498816716,63.4430883336209));
#199289=CARTESIAN_POINT('Ctrl Pts',(-4.77959789758538,4.79101554368635,
63.4467453809042));
#199290=CARTESIAN_POINT('Ctrl Pts',(-4.83423698792236,4.73523407495378,
63.4504024281874));
#199291=CARTESIAN_POINT('Ctrl Pts',(-4.96659834852405,4.60010534106987,
63.4592615023634));
#199292=CARTESIAN_POINT('Ctrl Pts',(-5.09316077763605,4.45955669194881,
63.4681205765393));
#199293=CARTESIAN_POINT('Ctrl Pts',(-5.21352157412158,4.31410266407382,
63.4769796507152));
#199294=CARTESIAN_POINT('Ctrl Pts',(-5.33410850432773,4.16837535734506,
63.4858553693091));
#199295=CARTESIAN_POINT('Ctrl Pts',(-5.44847035155232,4.01772445350142,
63.494731087903));
#199296=CARTESIAN_POINT('Ctrl Pts',(-5.55624676190952,3.86269477447675,
63.5036068064969));
#199297=CARTESIAN_POINT('Ctrl Pts',(-5.66433073569032,3.70722268455082,
63.5125078538839));
#199298=CARTESIAN_POINT('Ctrl Pts',(-5.76579151634374,3.5473470278303,63.5214089012709));
#199299=CARTESIAN_POINT('Ctrl Pts',(-5.86031232171138,3.3836413066396,63.5303099486579));
#199300=CARTESIAN_POINT('Ctrl Pts',(-5.95496162941053,3.21971302527529,
63.5392230971409));
#199301=CARTESIAN_POINT('Ctrl Pts',(-6.04265199088647,3.05194450580542,
63.5481362456239));
#199302=CARTESIAN_POINT('Ctrl Pts',(-6.12311357881597,2.88093198477844,
63.5570493941069));
#199303=CARTESIAN_POINT('Ctrl Pts',(-6.20375381347223,2.70953976919284,
63.5659823322168));
#199304=CARTESIAN_POINT('Ctrl Pts',(-6.27713306111496,2.53488938112438,
63.5749152703266));
#199305=CARTESIAN_POINT('Ctrl Pts',(-6.34302938388745,2.35759776788587,
63.5838482084365));
#199306=CARTESIAN_POINT('Ctrl Pts',(-6.40575312859799,2.18884185829608,
63.592351070295));
#199307=CARTESIAN_POINT('Ctrl Pts',(-6.46169745694369,2.0176932339583,63.6008539321535));
#199308=CARTESIAN_POINT('Ctrl Pts',(-6.51071347235249,1.84469484764495,
63.609356794012));
#199309=CARTESIAN_POINT('Ctrl Pts',(-6.56661490996948,1.64739487497929,
63.6190540775996));
#199310=CARTESIAN_POINT('Ctrl Pts',(-6.61358342331807,1.44741283947396,
63.6287513611871));
#199311=CARTESIAN_POINT('Ctrl Pts',(-6.65139328240953,1.2454944410624,63.6384486447746));
#199312=CARTESIAN_POINT('Ctrl Pts',(-6.68955888603213,1.04167623747579,
63.6482371679405));
#199313=CARTESIAN_POINT('Ctrl Pts',(-6.71839248848192,0.835885082081672,
63.6580256911065));
#199314=CARTESIAN_POINT('Ctrl Pts',(-6.73771199660313,0.628908618823391,
63.6678142142724));
#199315=CARTESIAN_POINT('Ctrl Pts',(-6.75703150472433,0.42193215556511,
63.6776027374383));
#199316=CARTESIAN_POINT('Ctrl Pts',(-6.76683677133875,0.213770445537998,
63.6873912606042));
#199317=CARTESIAN_POINT('Ctrl Pts',(-6.7669979781149,0.00523107913429214,
63.6971797837701));
#199318=CARTESIAN_POINT('',(-6.76699985002101,-0.00142471597195355,63.3028202161558));
#199319=CARTESIAN_POINT('Ctrl Pts',(3.09910619832141,6.01563211736936,62.6510873080018));
#199320=CARTESIAN_POINT('Ctrl Pts',(2.94704750109924,6.09396903057741,62.659158919634));
#199321=CARTESIAN_POINT('Ctrl Pts',(2.79224544225794,6.16641885136224,62.6672305312663));
#199322=CARTESIAN_POINT('Ctrl Pts',(2.63521336584288,6.23281152582709,62.6753021428986));
#199323=CARTESIAN_POINT('Ctrl Pts',(2.60279053890997,6.2465197964106,62.6769687098383));
#199324=CARTESIAN_POINT('Ctrl Pts',(2.57027268699037,6.259970017224,62.678635276778));
#199325=CARTESIAN_POINT('Ctrl Pts',(2.5376643900067,6.27316096108588,62.6803018437177));
#199326=CARTESIAN_POINT('Ctrl Pts',(2.37462119601859,6.33911637176053,62.6886347657644));
#199327=CARTESIAN_POINT('Ctrl Pts',(2.20879568825379,6.39879610100219,62.6969676878111));
#199328=CARTESIAN_POINT('Ctrl Pts',(2.04070539182329,6.45196175622449,62.7053006098578));
#199329=CARTESIAN_POINT('Ctrl Pts',(1.87281373736084,6.50506458253512,62.7136236844114));
#199330=CARTESIAN_POINT('Ctrl Pts',(1.70266295480959,6.55166856592118,62.7219467589651));
#199331=CARTESIAN_POINT('Ctrl Pts',(1.53079101222576,6.59158310854751,62.7302698335187));
#199332=CARTESIAN_POINT('Ctrl Pts',(1.35909063251716,6.63145780840722,62.7385845999646));
#199333=CARTESIAN_POINT('Ctrl Pts',(1.1856728525344,6.66465629283506,62.7468993664106));
#199334=CARTESIAN_POINT('Ctrl Pts',(1.01109150694816,6.69103751032508,62.7552141328566));
#199335=CARTESIAN_POINT('Ctrl Pts',(0.836652404672212,6.71739723324081,
62.7635221246961));
#199336=CARTESIAN_POINT('Ctrl Pts',(0.661051968390811,6.73695070523883,
62.7718301165357));
#199337=CARTESIAN_POINT('Ctrl Pts',(0.484855176277834,6.74960772623392,
62.7801381083752));
#199338=CARTESIAN_POINT('Ctrl Pts',(0.308769640893683,6.7622567551496,62.7884408542623));
#199339=CARTESIAN_POINT('Ctrl Pts',(0.132088846190396,6.76801798651536,
62.7967436001494));
#199340=CARTESIAN_POINT('Ctrl Pts',(-0.0446159123753718,6.7668529184816,
62.8050463460365));
#199341=CARTESIAN_POINT('Ctrl Pts',(-0.221248457337557,6.76568832657402,
62.8133456988559));
#199342=CARTESIAN_POINT('Ctrl Pts',(-0.397904599277771,6.75760307765305,
62.8216450516754));
#199343=CARTESIAN_POINT('Ctrl Pts',(-0.574011542342586,6.74261075172351,
62.8299444044948));
#199344=CARTESIAN_POINT('Ctrl Pts',(-0.750081030415655,6.72762161441013,
62.8382419921812));
#199345=CARTESIAN_POINT('Ctrl Pts',(-0.925601205865563,6.70572835620025,
62.8465395798675));
#199346=CARTESIAN_POINT('Ctrl Pts',(-1.10000265022993,6.67699656803021,
62.8548371675539));
#199347=CARTESIAN_POINT('Ctrl Pts',(-1.27439598353772,6.64826611611721,
62.8631343693363));
#199348=CARTESIAN_POINT('Ctrl Pts',(-1.44767034621451,6.61269782473572,
62.8714315711187));
#199349=CARTESIAN_POINT('Ctrl Pts',(-1.61926459693325,6.57040875175347,
62.8797287729011));
#199350=CARTESIAN_POINT('Ctrl Pts',(-1.79087938059843,6.52811461846607,
62.8880269675257));
#199351=CARTESIAN_POINT('Ctrl Pts',(-1.96081331407444,6.47909818492569,
62.8963251621502));
#199352=CARTESIAN_POINT('Ctrl Pts',(-2.12851835721448,6.42352695977848,
62.9046233567748));
#199353=CARTESIAN_POINT('Ctrl Pts',(-2.29634134926671,6.3679166507407,62.9129273876164));
#199354=CARTESIAN_POINT('Ctrl Pts',(-2.4619319879509,6.30574244785182,62.9212314184579));
#199355=CARTESIAN_POINT('Ctrl Pts',(-2.62475937696367,6.23722111304716,
62.9295354492995));
#199356=CARTESIAN_POINT('Ctrl Pts',(-2.78764597449635,6.16867486199935,
62.9378424997152));
#199357=CARTESIAN_POINT('Ctrl Pts',(-2.94776700192038,6.09377702065205,
62.946149550131));
#199358=CARTESIAN_POINT('Ctrl Pts',(-3.1046140757391,6.01279140173037,62.9544566005467));
#199359=CARTESIAN_POINT('Ctrl Pts',(-3.26162884555125,5.9317191955139,62.9627725326013));
#199360=CARTESIAN_POINT('Ctrl Pts',(-3.41536236199939,5.84454637321634,
62.9710884646559));
#199361=CARTESIAN_POINT('Ctrl Pts',(-3.56533230169483,5.75158191965406,
62.9794043967106));
#199362=CARTESIAN_POINT('Ctrl Pts',(-3.67838282770091,5.68150333993049,
62.9856731229294));
#199363=CARTESIAN_POINT('Ctrl Pts',(-3.78929525749684,5.60813461886252,
62.9919418491483));
#199364=CARTESIAN_POINT('Ctrl Pts',(-3.89787485526575,5.53162368682894,
62.9982105753671));
#199365=CARTESIAN_POINT('Ctrl Pts',(-4.0442405995954,5.42848663579396,63.0066608440905));
#199366=CARTESIAN_POINT('Ctrl Pts',(-4.1866346144784,5.31944928235414,63.0151111128138));
#199367=CARTESIAN_POINT('Ctrl Pts',(-4.32457027994008,5.20484206233571,
63.0235613815371));
#199368=CARTESIAN_POINT('Ctrl Pts',(-4.46238421249748,5.09033598707702,
63.0320041926116));
#199369=CARTESIAN_POINT('Ctrl Pts',(-4.59574738424135,4.97027005382572,
63.0404470036862));
#199370=CARTESIAN_POINT('Ctrl Pts',(-4.72420378140878,4.84501678343047,
63.0488898147607));
#199371=CARTESIAN_POINT('Ctrl Pts',(-4.85256430111656,4.71985699974079,
63.0573263242784));
#199372=CARTESIAN_POINT('Ctrl Pts',(-4.97602511025851,4.58951782771408,
63.0657628337962));
#199373=CARTESIAN_POINT('Ctrl Pts',(-5.09416451673034,4.45441094607194,
63.074199343314));
#199374=CARTESIAN_POINT('Ctrl Pts',(-5.21221938809949,4.31940074067403,
63.0826298160552));
#199375=CARTESIAN_POINT('Ctrl Pts',(-5.32496023423207,4.17962987956021,
63.0910602887964));
#199376=CARTESIAN_POINT('Ctrl Pts',(-5.43200323254407,4.03554579724115,
63.0994907615376));
#199377=CARTESIAN_POINT('Ctrl Pts',(-5.53900021336142,3.89152365627831,
63.1079176100414));
#199378=CARTESIAN_POINT('Ctrl Pts',(-5.64030403212136,3.74319225628524,
63.1163444585452));
#199379=CARTESIAN_POINT('Ctrl Pts',(-5.73557166646664,3.59103141991616,
63.1247713070491));
#199380=CARTESIAN_POINT('Ctrl Pts',(-5.83080989509528,3.43891755016349,
63.1331955544857));
#199381=CARTESIAN_POINT('Ctrl Pts',(-5.92001547912602,3.28297688195782,
63.1416198019224));
#199382=CARTESIAN_POINT('Ctrl Pts',(-6.0028889905621,3.1237177796639,63.150044049359));
#199383=CARTESIAN_POINT('Ctrl Pts',(-6.02623957529533,3.0788446579847,63.15241767997));
#199384=CARTESIAN_POINT('Ctrl Pts',(-6.04908773166963,3.0337082493871,63.1547913105809));
#199385=CARTESIAN_POINT('Ctrl Pts',(-6.07142741218927,2.98832029383009,
63.1571649411919));
#199386=CARTESIAN_POINT('Ctrl Pts',(-6.15179288111495,2.82504023578669,
63.1657039145644));
#199387=CARTESIAN_POINT('Ctrl Pts',(-6.22554386788738,2.65856491521556,
63.1742428879368));
#199388=CARTESIAN_POINT('Ctrl Pts',(-6.29244860583804,2.48945366353481,
63.1827818613093));
#199389=CARTESIAN_POINT('Ctrl Pts',(-6.35938647625348,2.32025866483163,
63.1913250633395));
#199390=CARTESIAN_POINT('Ctrl Pts',(-6.41947121772726,2.14842542445335,
63.1998682653696));
#199391=CARTESIAN_POINT('Ctrl Pts',(-6.47252014396247,1.97453082680419,
63.2084114673998));
#199392=CARTESIAN_POINT('Ctrl Pts',(-6.5256272545327,1.80044550066633,63.2169640396579));
#199393=CARTESIAN_POINT('Ctrl Pts',(-6.57168303404136,1.62429460107207,
63.2255166119159));
#199394=CARTESIAN_POINT('Ctrl Pts',(-6.61055500926353,1.4466690946795,63.234069184174));
#199395=CARTESIAN_POINT('Ctrl Pts',(-6.64944878854188,1.26894395464352,
63.2426265537382));
#199396=CARTESIAN_POINT('Ctrl Pts',(-6.68115066323215,1.08974286753986,
63.2511839233024));
#199397=CARTESIAN_POINT('Ctrl Pts',(-6.70557961935685,0.909665305739452,
63.2597412928667));
#199398=CARTESIAN_POINT('Ctrl Pts',(-6.73003791924544,0.729371436970054,
63.2683089414387));
#199399=CARTESIAN_POINT('Ctrl Pts',(-6.74720580367184,0.548199303442522,
63.2768765900108));
#199400=CARTESIAN_POINT('Ctrl Pts',(-6.75705416573981,0.366753324808809,
63.2854442385829));
#199401=CARTESIAN_POINT('Ctrl Pts',(-6.76371195976512,0.244090292709951,
63.2912362311072));
#199402=CARTESIAN_POINT('Ctrl Pts',(-6.76702568878971,0.121302162455473,
63.2970282236315));
#199403=CARTESIAN_POINT('Ctrl Pts',(-6.76699985002101,-0.00142471597195272,
63.3028202161558));
#199404=CARTESIAN_POINT('Ctrl Pts',(-6.76699985002086,-0.00142471669502992,
63.3028202161899));
#199405=CARTESIAN_POINT('Ctrl Pts',(-6.76698007373462,-0.0953564621888831,
63.3072532464654));
#199406=CARTESIAN_POINT('Ctrl Pts',(-6.76500440002413,-0.189266792552925,
63.311686276741));
#199407=CARTESIAN_POINT('Ctrl Pts',(-6.76107620035431,-0.283085875667693,
63.3161193070166));
#199408=CARTESIAN_POINT('Ctrl Pts',(-6.75306159807707,-0.474502478789027,
63.3251639018765));
#199409=CARTESIAN_POINT('Ctrl Pts',(-6.73691165593163,-0.665627526396733,
63.3342084967363));
#199410=CARTESIAN_POINT('Ctrl Pts',(-6.71266801146048,-0.855790376152495,
63.3432530915961));
#199411=CARTESIAN_POINT('Ctrl Pts',(-6.6884466143493,-1.04577872156024,
63.3522893866164));
#199412=CARTESIAN_POINT('Ctrl Pts',(-6.65614637350505,-1.23480639618576,
63.3613256816367));
#199413=CARTESIAN_POINT('Ctrl Pts',(-6.61586069696472,-1.42220822608981,
63.370361976657));
#199414=CARTESIAN_POINT('Ctrl Pts',(-6.57564630908804,-1.60927843376065,
63.3793822812447));
#199415=CARTESIAN_POINT('Ctrl Pts',(-6.52747475296321,-1.79472830955393,
63.3884025858324));
#199416=CARTESIAN_POINT('Ctrl Pts',(-6.47149034390523,-1.97790336688663,
63.3974228904201));
#199417=CARTESIAN_POINT('Ctrl Pts',(-6.41557643633529,-2.16084775081699,
63.4064318356864));
#199418=CARTESIAN_POINT('Ctrl Pts',(-6.35186937996053,-2.34152280640211,
63.4154407809527));
#199419=CARTESIAN_POINT('Ctrl Pts',(-6.28056374857452,-2.51928720079541,
63.424449726219));
#199420=CARTESIAN_POINT('Ctrl Pts',(-6.20942003718207,-2.69664792988155,
63.4334382140778));
#199421=CARTESIAN_POINT('Ctrl Pts',(-6.1307122811609,-2.87111097051372,
63.4424267019366));
#199422=CARTESIAN_POINT('Ctrl Pts',(-6.04468358232521,-3.04205348236485,
63.4514151897954));
#199423=CARTESIAN_POINT('Ctrl Pts',(-5.96920523918043,-3.19203200978827,
63.4593013508107));
#199424=CARTESIAN_POINT('Ctrl Pts',(-5.88809225212156,-3.33930066668055,
63.467187511826));
#199425=CARTESIAN_POINT('Ctrl Pts',(-5.80153993560371,-3.48344992437029,
63.4750736728414));
#199426=CARTESIAN_POINT('Ctrl Pts',(-5.71240510872753,-3.63190024488659,
63.4831951376975));
#199427=CARTESIAN_POINT('Ctrl Pts',(-5.61754001569764,-3.7769749438643,
63.4913166025537));
#199428=CARTESIAN_POINT('Ctrl Pts',(-5.51724039658921,-3.91820716734633,
63.4994380674098));
#199429=CARTESIAN_POINT('Ctrl Pts',(-5.41694793031973,-4.05942931889232,
63.507558953086));
#199430=CARTESIAN_POINT('Ctrl Pts',(-5.31122192196806,-4.19680924220401,
63.5156798387622));
#199431=CARTESIAN_POINT('Ctrl Pts',(-5.20040081889535,-4.32990996705851,
63.5238007244384));
#199432=CARTESIAN_POINT('Ctrl Pts',(-5.08956646953165,-4.46302660125593,
63.5319225807927));
#199433=CARTESIAN_POINT('Ctrl Pts',(-4.97363604799523,-4.59186273787047,
63.540044437147));
#199434=CARTESIAN_POINT('Ctrl Pts',(-4.85298753256088,-4.71601537410648,
63.5481662935012));
#199435=CARTESIAN_POINT('Ctrl Pts',(-4.73225099346262,-4.84025859056958,
63.5562940754614));
#199436=CARTESIAN_POINT('Ctrl Pts',(-4.60678974079254,-4.95981121904418,
63.5644218574216));
#199437=CARTESIAN_POINT('Ctrl Pts',(-4.47701823570153,-5.07430751109902,
63.5725496393817));
#199438=CARTESIAN_POINT('Ctrl Pts',(-4.34719386652271,-5.18885044468764,
63.5806807322981));
#199439=CARTESIAN_POINT('Ctrl Pts',(-4.21305602853732,-5.29833270478728,
63.5888118252146));
#199440=CARTESIAN_POINT('Ctrl Pts',(-4.07505112596264,-5.40242976083824,
63.596942918131));
#199441=CARTESIAN_POINT('Ctrl Pts',(-3.93689559680428,-5.50664043447546,
63.6050828857956));
#199442=CARTESIAN_POINT('Ctrl Pts',(-3.7948648730645,-5.60545395541145,
63.6132228534601));
#199443=CARTESIAN_POINT('Ctrl Pts',(-3.64943372661247,-5.69858951628063,
63.6213628211247));
#199444=CARTESIAN_POINT('Ctrl Pts',(-3.5740068460226,-5.74689364507099,
63.6255845603051));
#199445=CARTESIAN_POINT('Ctrl Pts',(-3.49766569458399,-5.79367120624689,
63.6298062994856));
#199446=CARTESIAN_POINT('Ctrl Pts',(-3.42047891288538,-5.83888799400249,
63.6340280386661));
#199447=CARTESIAN_POINT('Ctrl Pts',(-3.26616511540881,-5.92928655804038,
63.6424682481237));
#199448=CARTESIAN_POINT('Ctrl Pts',(-3.10815110810223,-6.01363092103054,
63.6509084575814));
#199449=CARTESIAN_POINT('Ctrl Pts',(-2.94694036471961,-6.09161977529673,
63.659348667039));
#199450=CARTESIAN_POINT('Ctrl Pts',(-2.78585176235865,-6.16954954145169,
63.6677824817875));
#199451=CARTESIAN_POINT('Ctrl Pts',(-2.62157155114009,-6.24113325303317,
63.676216296536));
#199452=CARTESIAN_POINT('Ctrl Pts',(-2.45462835877894,-6.30611517657886,
63.6846501112846));
#199453=CARTESIAN_POINT('Ctrl Pts',(-2.28778598696022,-6.37105785615966,
63.6930788326731));
#199454=CARTESIAN_POINT('Ctrl Pts',(-2.11828415023037,-6.42940657561799,
63.7015075540616));
#199455=CARTESIAN_POINT('Ctrl Pts',(-1.94667240273159,-6.48095329071605,
63.7099362754501));
#199456=CARTESIAN_POINT('Ctrl Pts',(-1.77513794286605,-6.53247679106531,
63.7183612008519));
#199457=CARTESIAN_POINT('Ctrl Pts',(-1.60149578573184,-6.57720429930089,
63.7267861262536));
#199458=CARTESIAN_POINT('Ctrl Pts',(-1.42631200754099,-6.61497717737139,
63.7352110516553));
#199459=CARTESIAN_POINT('Ctrl Pts',(-1.25118024731205,-6.65273883940264,
63.7436334754131));
#199460=CARTESIAN_POINT('Ctrl Pts',(-1.074508104543,-6.68354991924383,63.7520558991708));
#199461=CARTESIAN_POINT('Ctrl Pts',(-0.896873633896095,-6.70730248943806,
63.7604783229285));
#199462=CARTESIAN_POINT('Ctrl Pts',(-0.719236369570615,-6.7310554331918,
63.7689008791467));
#199463=CARTESIAN_POINT('Ctrl Pts',(-0.540637076705376,-6.74774959471769,
63.7773234353649));
#199464=CARTESIAN_POINT('Ctrl Pts',(-0.361661424485507,-6.75732861521764,
63.7857459915831));
#199465=CARTESIAN_POINT('Ctrl Pts',(-0.182679726434212,-6.76690795929871,
63.7941688323169));
#199466=CARTESIAN_POINT('Ctrl Pts',(-0.00332197677035101,-6.76937166511965,
63.8025916730506));
#199467=CARTESIAN_POINT('Ctrl Pts',(0.175823482853185,-6.76471544877369,
63.8110145137843));
#199468=CARTESIAN_POINT('Ctrl Pts',(0.355000004732227,-6.76005842508055,
63.8194388149649));
#199469=CARTESIAN_POINT('Ctrl Pts',(0.533963829738483,-6.74827902659319,
63.8278631161456));
#199470=CARTESIAN_POINT('Ctrl Pts',(0.71212869830463,-6.72942506586194,
63.8362874173262));
#199471=CARTESIAN_POINT('Ctrl Pts',(0.89034934050912,-6.71056520299075,
63.844714355693));
#199472=CARTESIAN_POINT('Ctrl Pts',(1.06777019604266,-6.68462639753977,
63.8531412940599));
#199473=CARTESIAN_POINT('Ctrl Pts',(1.24381182296976,-6.6517081376922,63.8615682324267));
#199474=CARTESIAN_POINT('Ctrl Pts',(1.42001173344752,-6.61876028019127,
63.8700027476703));
#199475=CARTESIAN_POINT('Ctrl Pts',(1.5948296092077,-6.57882049040694,63.8784372629139));
#199476=CARTESIAN_POINT('Ctrl Pts',(1.76769674382886,-6.53203928508218,
63.8868717781576));
#199477=CARTESIAN_POINT('Ctrl Pts',(1.94064737475684,-6.48523548403451,
63.8953103673443));
#199478=CARTESIAN_POINT('Ctrl Pts',(2.11164506577398,-6.43158377198406,
63.9037489565311));
#199479=CARTESIAN_POINT('Ctrl Pts',(2.28013738826408,-6.37128421047439,
63.9121875457179));
#199480=CARTESIAN_POINT('Ctrl Pts',(2.44881804705034,-6.31091724769736,
63.9206355673382));
#199481=CARTESIAN_POINT('Ctrl Pts',(2.6149874303068,-6.24388770752694,63.9290835889585));
#199482=CARTESIAN_POINT('Ctrl Pts',(2.7781130291179,-6.17044382499714,63.9375316105788));
#199483=CARTESIAN_POINT('Ctrl Pts',(2.8708310015874,-6.12869950081945,63.942333330491));
#199484=CARTESIAN_POINT('Ctrl Pts',(2.96256607040804,-6.08488381200273,
63.9471350504033));
#199485=CARTESIAN_POINT('Ctrl Pts',(3.05322414153299,-6.03904887722894,
63.9519367703156));
#199486=CARTESIAN_POINT('Ctrl Pts',(3.20878924699882,-5.96039822457744,
63.9601763021664));
#199487=CARTESIAN_POINT('Ctrl Pts',(3.36152890175195,-5.8756237564737,63.9684158340172));
#199488=CARTESIAN_POINT('Ctrl Pts',(3.51092968437654,-5.78495131797699,
63.9766553658681));
#199489=CARTESIAN_POINT('Ctrl Pts',(3.66016464257403,-5.69437951954991,
63.9848857524144));
#199490=CARTESIAN_POINT('Ctrl Pts',(3.80606780616563,-5.5979229686101,63.9931161389607));
#199491=CARTESIAN_POINT('Ctrl Pts',(3.94814787931328,-5.495854558035,64.0013465255071));
#199492=CARTESIAN_POINT('Ctrl Pts',(4.09009559928871,-5.39388122819587,
64.0095692451249));
#199493=CARTESIAN_POINT('Ctrl Pts',(4.2282270339751,-5.28630665614089,64.0177919647427));
#199494=CARTESIAN_POINT('Ctrl Pts',(4.36207748268065,-5.1734484664574,64.0260146843605));
#199495=CARTESIAN_POINT('Ctrl Pts',(4.49580933024509,-5.0606902772611,64.0342301180563));
#199496=CARTESIAN_POINT('Ctrl Pts',(4.62526748109972,-4.94265802998371,
64.0424455517521));
#199497=CARTESIAN_POINT('Ctrl Pts',(4.75001821919929,-4.8197111860852,64.0506609854479));
#199498=CARTESIAN_POINT('Ctrl Pts',(4.87470484510672,-4.69682752731729,
64.0588721970487));
#199499=CARTESIAN_POINT('Ctrl Pts',(4.9946886235279,-4.56903455133817,64.0670834086495));
#199500=CARTESIAN_POINT('Ctrl Pts',(5.10957048674683,-4.4367306027035,64.0752946202503));
#199501=CARTESIAN_POINT('Ctrl Pts',(5.22441382492784,-4.30447102151289,
64.0835030782639));
#199502=CARTESIAN_POINT('Ctrl Pts',(5.33415842307217,-4.16770374960559,
64.0917115362774));
#199503=CARTESIAN_POINT('Ctrl Pts',(5.43844346888631,-4.02686250519282,
64.099919994291));
#199504=CARTESIAN_POINT('Ctrl Pts',(5.48490473394169,-3.9641146554287,64.1035770415741));
#199505=CARTESIAN_POINT('Ctrl Pts',(5.53028285833373,-3.90055861502764,
64.1072340888572));
#199506=CARTESIAN_POINT('Ctrl Pts',(5.57454854343968,-3.83623481252576,
64.1108911361403));
#199507=CARTESIAN_POINT('Ctrl Pts',(5.68178067839527,-3.68041256207988,
64.1197502103162));
#199508=CARTESIAN_POINT('Ctrl Pts',(5.78237046120215,-3.52024494104774,
64.1286092844921));
#199509=CARTESIAN_POINT('Ctrl Pts',(5.87600937643769,-3.3563079131713,64.137468358668));
#199510=CARTESIAN_POINT('Ctrl Pts',(5.96982422035596,-3.19206288060161,
64.1463440772619));
#199511=CARTESIAN_POINT('Ctrl Pts',(6.05666196990865,-3.02403451340599,
64.1552197958559));
#199512=CARTESIAN_POINT('Ctrl Pts',(6.13626102253946,-2.85282135144545,
64.1640955144498));
#199513=CARTESIAN_POINT('Ctrl Pts',(6.21608722837607,-2.68111959549629,
64.1729965618368));
#199514=CARTESIAN_POINT('Ctrl Pts',(6.28863328939886,-2.50621509397389,
64.1818976092238));
#199515=CARTESIAN_POINT('Ctrl Pts',(6.35368544705852,-2.32872717161902,
64.1907986566108));
#199516=CARTESIAN_POINT('Ctrl Pts',(6.41882604401885,-2.15099795199912,
64.1997118050938));
#199517=CARTESIAN_POINT('Ctrl Pts',(6.47645230324947,-1.97067854131893,
64.2086249535769));
#199518=CARTESIAN_POINT('Ctrl Pts',(6.52640062368902,-1.78840261102236,
64.2175381020599));
#199519=CARTESIAN_POINT('Ctrl Pts',(6.57645984305797,-1.60572197831846,
64.2264710401698));
#199520=CARTESIAN_POINT('Ctrl Pts',(6.61880695747251,-1.42107638823298,
64.2354039782797));
#199521=CARTESIAN_POINT('Ctrl Pts',(6.65332909720839,-1.23511170516685,
64.2443369163896));
#199522=CARTESIAN_POINT('Ctrl Pts',(6.68618916873535,-1.05810029064291,
64.2528397782481));
#199523=CARTESIAN_POINT('Ctrl Pts',(6.71195996542605,-0.879893990178444,
64.2613426401067));
#199524=CARTESIAN_POINT('Ctrl Pts',(6.73058789011606,-0.701053245783138,
64.2698455019653));
#199525=CARTESIAN_POINT('Ctrl Pts',(6.74860209327117,-0.528104645466156,
64.2780682258312));
#199526=CARTESIAN_POINT('Ctrl Pts',(6.75996987356229,-0.354231136869663,
64.2862909496971));
#199527=CARTESIAN_POINT('Ctrl Pts',(6.76460601849349,-0.179984484224986,
64.2945136735629));
#199528=CARTESIAN_POINT('Ctrl Pts',(6.76923725622233,-0.00592226575934016,
64.3027276939542));
#199529=CARTESIAN_POINT('Ctrl Pts',(6.76715103770652,0.168511954645426,
64.3109417143454));
#199530=CARTESIAN_POINT('Ctrl Pts',(6.75831374290271,0.342759905024563,
64.3191557347366));
#199531=CARTESIAN_POINT('Ctrl Pts',(6.74948402779712,0.516858403913161,
64.3273627100086));
#199532=CARTESIAN_POINT('Ctrl Pts',(6.73391478647192,0.690770594724244,
64.3355696852805));
#199533=CARTESIAN_POINT('Ctrl Pts',(6.71162441967599,0.86393671597462,64.3437766605525));
#199534=CARTESIAN_POINT('Ctrl Pts',(6.6893486972062,1.03698907053911,64.3519782440055));
#199535=CARTESIAN_POINT('Ctrl Pts',(6.66036069033445,1.20929597735572,64.3601798274585));
#199536=CARTESIAN_POINT('Ctrl Pts',(6.62473075200399,1.38030122199928,64.3683814109115));
#199537=CARTESIAN_POINT('Ctrl Pts',(6.5891170718551,1.55122843579444,64.3765792519265));
#199538=CARTESIAN_POINT('Ctrl Pts',(6.54686757127822,1.72085482026698,64.3847770929416));
#199539=CARTESIAN_POINT('Ctrl Pts',(6.49810399063429,1.88863271360599,64.3929749339566));
#199540=CARTESIAN_POINT('Ctrl Pts',(6.44934471322425,2.05639580106923,64.4011720515378));
#199541=CARTESIAN_POINT('Ctrl Pts',(6.39407259256909,2.22231037571562,64.4093691691189));
#199542=CARTESIAN_POINT('Ctrl Pts',(6.33245979173458,2.38584198681826,64.4175662867001));
#199543=CARTESIAN_POINT('Ctrl Pts',(6.27084767641108,2.54937177844962,64.4257633130792));
#199544=CARTESIAN_POINT('Ctrl Pts',(6.20289514693037,2.71051832317652,64.4339603394583));
#199545=CARTESIAN_POINT('Ctrl Pts',(6.12882322554851,2.86876539124013,64.4421573658374));
#199546=CARTESIAN_POINT('Ctrl Pts',(6.05473865977661,3.02703947274709,64.4503557914835));
#199547=CARTESIAN_POINT('Ctrl Pts',(5.97453277306417,3.1824127664959,64.4585542171297));
#199548=CARTESIAN_POINT('Ctrl Pts',(5.88847344329453,3.33439192471657,64.4667526427758));
#199549=CARTESIAN_POINT('Ctrl Pts',(5.80238377446761,3.48642466114196,64.4749539586665));
#199550=CARTESIAN_POINT('Ctrl Pts',(5.71043672867051,3.63506056642938,64.4831552745571));
#199551=CARTESIAN_POINT('Ctrl Pts',(5.61294458048369,3.7798336122664,64.4913565904477));
#199552=CARTESIAN_POINT('Ctrl Pts',(5.51534140505971,3.92477153036843,64.4995672462643));
#199553=CARTESIAN_POINT('Ctrl Pts',(5.41218071175398,4.06583750235549,64.5077779020809));
#199554=CARTESIAN_POINT('Ctrl Pts',(5.30381693588577,4.20259621075012,64.5159885578975));
#199555=CARTESIAN_POINT('Ctrl Pts',(5.19538930386982,4.33943550773829,64.5242040520547));
#199556=CARTESIAN_POINT('Ctrl Pts',(5.08175271078018,4.47196220973772,64.5324195462119));
#199557=CARTESIAN_POINT('Ctrl Pts',(4.96329974703248,4.59977658382527,64.540635040369));
#199558=CARTESIAN_POINT('Ctrl Pts',(4.8446630013318,4.72778926426622,64.5488632810165));
#199559=CARTESIAN_POINT('Ctrl Pts',(4.72119520535234,4.85107475263417,64.557091521664));
#199560=CARTESIAN_POINT('Ctrl Pts',(4.59332441746952,4.9692715558599,64.5653197623115));
#199561=CARTESIAN_POINT('Ctrl Pts',(4.47711028599368,5.07669357974457,64.5727979194126));
#199562=CARTESIAN_POINT('Ctrl Pts',(4.35725989585569,5.17991277858773,64.5802760765137));
#199563=CARTESIAN_POINT('Ctrl Pts',(4.23411560178897,5.27868866961173,64.5877542336147));
#199564=CARTESIAN_POINT('Ctrl Pts',(4.10121601260401,5.38528942962222,64.5958247984275));
#199565=CARTESIAN_POINT('Ctrl Pts',(3.96404432174565,5.48706334156706,64.6038953632403));
#199566=CARTESIAN_POINT('Ctrl Pts',(3.82299214193917,5.58363860602308,64.6119659280531));
#199567=CARTESIAN_POINT('Ctrl Pts',(3.68214381142925,5.68007429943702,64.6200248292464));
#199568=CARTESIAN_POINT('Ctrl Pts',(3.53742646164195,5.77132609532913,64.6280837304396));
#199569=CARTESIAN_POINT('Ctrl Pts',(3.38926637153549,5.85706090652801,64.6361426316329));
#199570=CARTESIAN_POINT('Ctrl Pts',(3.29393078808783,5.91222811276787,64.641328238949));
#199571=CARTESIAN_POINT('Ctrl Pts',(3.1971704820577,5.96511180235815,64.6465138462651));
#199572=CARTESIAN_POINT('Ctrl Pts',(3.09910619832139,6.01563211736938,64.6516994535812));
#199573=CARTESIAN_POINT('Origin',(0.,0.,4.30282021618968));
#199574=CARTESIAN_POINT('',(3.09910619832127,6.01563211736944,67.045599963736));
#199575=CARTESIAN_POINT('',(3.09910619832135,6.0156321173694,66.651425676538));
#199576=CARTESIAN_POINT('',(3.09910619832133,6.0156321173694,4.30282021618968));
#199577=CARTESIAN_POINT('',(-6.76699920770444,-0.00327458815153042,65.6971797838342));
#199578=CARTESIAN_POINT('Ctrl Pts',(-6.76699920770444,-0.00327458815152907,
65.6971797838342));
#199579=CARTESIAN_POINT('Ctrl Pts',(-6.76690542650691,-0.197075231149046,
65.7062649518173));
#199580=CARTESIAN_POINT('Ctrl Pts',(-6.75848210553396,-0.390632917290863,
65.7153501198004));
#199581=CARTESIAN_POINT('Ctrl Pts',(-6.74181645938078,-0.583266515430461,
65.7244352877836));
#199582=CARTESIAN_POINT('Ctrl Pts',(-6.72495810982722,-0.778127518919279,
65.7336255067648));
#199583=CARTESIAN_POINT('Ctrl Pts',(-6.69966572931804,-0.972042707940345,
65.7428157257461));
#199584=CARTESIAN_POINT('Ctrl Pts',(-6.66608169134746,-1.16432121181491,
65.7520059447274));
#199585=CARTESIAN_POINT('Ctrl Pts',(-6.63266310140719,-1.35565247701127,
65.7611508891163));
#199586=CARTESIAN_POINT('Ctrl Pts',(-6.59103450047461,-1.54536296153818,
65.7702958335053));
#199587=CARTESIAN_POINT('Ctrl Pts',(-6.54138605026677,-1.73278894888422,
65.7794407778942));
#199588=CARTESIAN_POINT('Ctrl Pts',(-6.49136890235314,-1.92160679300023,
65.7886536341717));
#199589=CARTESIAN_POINT('Ctrl Pts',(-6.43321240571779,-2.1081058685722,
65.7978664904491));
#199590=CARTESIAN_POINT('Ctrl Pts',(-6.36716032525063,-2.29162789138077,
65.8070793467265));
#199591=CARTESIAN_POINT('Ctrl Pts',(-6.30110824478346,-2.4751499141894,
65.816292203004));
#199592=CARTESIAN_POINT('Ctrl Pts',(-6.22716070257162,-2.65569469998394,
65.8255050592814));
#199593=CARTESIAN_POINT('Ctrl Pts',(-6.14560918242237,-2.83262718636356,
65.8347179155589));
#199594=CARTESIAN_POINT('Ctrl Pts',(-6.07282224090383,-2.99054422476176,
65.8429406394255));
#199595=CARTESIAN_POINT('Ctrl Pts',(-5.99384780368116,-3.14586409371244,
65.851163363292));
#199596=CARTESIAN_POINT('Ctrl Pts',(-5.90889423041982,-3.29806882489,65.8593860871586));
#199597=CARTESIAN_POINT('Ctrl Pts',(-5.82403057763788,-3.45011245251572,
65.8676001075505));
#199598=CARTESIAN_POINT('Ctrl Pts',(-5.73320056469686,-3.59904719765596,
65.8758141279424));
#199599=CARTESIAN_POINT('Ctrl Pts',(-5.63666023840997,-3.74437583005874,
65.8840281483343));
#199600=CARTESIAN_POINT('Ctrl Pts',(-5.54020271421983,-3.88957981490807,
65.892235123607));
#199601=CARTESIAN_POINT('Ctrl Pts',(-5.43804482825019,-4.03118354977133,
65.9004420988796));
#199602=CARTESIAN_POINT('Ctrl Pts',(-5.33048812136502,-4.16871507637383,
65.9086490741523));
#199603=CARTESIAN_POINT('Ctrl Pts',(-5.22300207708986,-4.30615624750794,
65.9168506576059));
#199604=CARTESIAN_POINT('Ctrl Pts',(-5.1101244971274,-4.43953025781604,
65.9250522410596));
#199605=CARTESIAN_POINT('Ctrl Pts',(-4.99219978659632,-4.56839471704314,
65.9332538245133));
#199606=CARTESIAN_POINT('Ctrl Pts',(-4.87432888590749,-4.69720037454673,
65.941451665529));
#199607=CARTESIAN_POINT('Ctrl Pts',(-4.75141568454248,-4.8215003163931,
65.9496495065448));
#199608=CARTESIAN_POINT('Ctrl Pts',(-4.62384441123766,-4.94088573645113,
65.9578473475605));
#199609=CARTESIAN_POINT('Ctrl Pts',(-4.49628439569947,-5.06026062111853,
65.9660444651423));
#199610=CARTESIAN_POINT('Ctrl Pts',(-4.36406738285808,-5.17472159665961,
65.9742415827242));
#199611=CARTESIAN_POINT('Ctrl Pts',(-4.22761421767973,-5.28389695456604,
65.9824387003061));
#199612=CARTESIAN_POINT('Ctrl Pts',(-4.09116257069484,-5.39307109777499,
65.9906357266859));
#199613=CARTESIAN_POINT('Ctrl Pts',(-3.95047514476605,-5.49695951546655,
65.9988327530656));
#199614=CARTESIAN_POINT('Ctrl Pts',(-3.80600549940807,-5.5952311067976,
66.0070297794454));
#199615=CARTESIAN_POINT('Ctrl Pts',(-3.66151119247102,-5.69351947350465,
66.0152282050923));
#199616=CARTESIAN_POINT('Ctrl Pts',(-3.51323367650264,-5.78618890177864,
66.0234266307391));
#199617=CARTESIAN_POINT('Ctrl Pts',(-3.36165512354724,-5.87295188387651,
66.0316250563859));
#199618=CARTESIAN_POINT('Ctrl Pts',(-3.21002313361495,-5.95974545309491,
66.0398263722773));
#199619=CARTESIAN_POINT('Ctrl Pts',(-3.05508809975564,-6.04062825014876,
66.0480276881687));
#199620=CARTESIAN_POINT('Ctrl Pts',(-2.89735642705186,-6.11535892116082,
66.05622900406));
#199621=CARTESIAN_POINT('Ctrl Pts',(-2.73944512437668,-6.19017469789748,
66.0644396598773));
#199622=CARTESIAN_POINT('Ctrl Pts',(-2.57873114460146,-6.25882419757173,
66.0726503156946));
#199623=CARTESIAN_POINT('Ctrl Pts',(-2.4157414720476,-6.32111399519336,
66.0808609715119));
#199624=CARTESIAN_POINT('Ctrl Pts',(-2.25265575362824,-6.38344049868371,
66.0890764656697));
#199625=CARTESIAN_POINT('Ctrl Pts',(-2.08729200866785,-6.439399714989,66.0972919598276));
#199626=CARTESIAN_POINT('Ctrl Pts',(-1.92019186851095,-6.48884829442825,
66.1055074539854));
#199627=CARTESIAN_POINT('Ctrl Pts',(-1.75283246941213,-6.53837359424831,
66.1137356946336));
#199628=CARTESIAN_POINT('Ctrl Pts',(-1.58373163888332,-6.58136798231884,
66.1219639352818));
#199629=CARTESIAN_POINT('Ctrl Pts',(-1.41344198922957,-6.61773909602689,
66.13019217593));
#199630=CARTESIAN_POINT('Ctrl Pts',(-1.25867588480477,-6.65079463166063,
66.1376703330228));
#199631=CARTESIAN_POINT('Ctrl Pts',(-1.10292812370035,-6.67838002420534,
66.1451484901156));
#199632=CARTESIAN_POINT('Ctrl Pts',(-0.946615852892707,-6.70046322481157,
66.1526266472084));
#199633=CARTESIAN_POINT('Ctrl Pts',(-0.777947017418176,-6.72429211367971,
66.1606959564304));
#199634=CARTESIAN_POINT('Ctrl Pts',(-0.608068646005757,-6.74179166845406,
66.1687652656524));
#199635=CARTESIAN_POINT('Ctrl Pts',(-0.437507024395419,-6.7528421130369,
66.1768345748744));
#199636=CARTESIAN_POINT('Ctrl Pts',(-0.26715813948428,-6.76387877471194,
66.1848938194746));
#199637=CARTESIAN_POINT('Ctrl Pts',(-0.09612806766793,-6.76848230737992,
66.1929530640749));
#199638=CARTESIAN_POINT('Ctrl Pts',(0.0750465407677626,-6.76658385130332,
66.2010123086751));
#199639=CARTESIAN_POINT('Ctrl Pts',(0.24604521192923,-6.76468734650436,
66.2090632697949));
#199640=CARTESIAN_POINT('Ctrl Pts',(0.417187754117139,-6.75630215615335,
66.2171142309146));
#199641=CARTESIAN_POINT('Ctrl Pts',(0.587932317773019,-6.74141117198158,
66.2251651920344));
#199642=CARTESIAN_POINT('Ctrl Pts',(0.75853879968691,-6.72653223020221,
66.2332096423129));
#199643=CARTESIAN_POINT('Ctrl Pts',(0.928747573812776,-6.70515799850142,
66.2412540925915));
#199644=CARTESIAN_POINT('Ctrl Pts',(1.09801681797997,-6.67732342090999,
66.2492985428701));
#199645=CARTESIAN_POINT('Ctrl Pts',(1.26718622495699,-6.64950526051255,
66.2573382484278));
#199646=CARTESIAN_POINT('Ctrl Pts',(1.43541683785557,-6.61523439997803,
66.2653779539856));
#199647=CARTESIAN_POINT('Ctrl Pts',(1.6021720938859,-6.57459759845219,66.2734176595433));
#199648=CARTESIAN_POINT('Ctrl Pts',(1.77252667298302,-6.53308367328674,
66.2816308978481));
#199649=CARTESIAN_POINT('Ctrl Pts',(1.94134108426297,-6.48492590695746,
66.2898441361528));
#199650=CARTESIAN_POINT('Ctrl Pts',(2.10805392617354,-6.430271972813,66.2980573744576));
#199651=CARTESIAN_POINT('Ctrl Pts',(2.27119185757413,-6.37679001151325,
66.3060944920053));
#199652=CARTESIAN_POINT('Ctrl Pts',(2.43231707074948,-6.31708779256848,
66.3141316095529));
#199653=CARTESIAN_POINT('Ctrl Pts',(2.59091904766208,-6.25135405240031,
66.3221687271006));
#199654=CARTESIAN_POINT('Ctrl Pts',(2.74953780365543,-6.18561335802038,
66.3302066949242));
#199655=CARTESIAN_POINT('Ctrl Pts',(2.90563244664924,-6.11384001482513,
66.3382446627478));
#199656=CARTESIAN_POINT('Ctrl Pts',(3.0587129614512,-6.03627070461974,66.3462826305714));
#199657=CARTESIAN_POINT('Ctrl Pts',(3.21184000209162,-5.95867781873457,
66.3543230413786));
#199658=CARTESIAN_POINT('Ctrl Pts',(3.36195075799938,-5.8752856282353,66.3623634521859));
#199659=CARTESIAN_POINT('Ctrl Pts',(3.50858045251912,-5.78637643160214,
66.3704038629931));
#199660=CARTESIAN_POINT('Ctrl Pts',(3.66075192251652,-5.69410696877423,
66.3787481559819));
#199661=CARTESIAN_POINT('Ctrl Pts',(3.80917368031177,-5.59589555959404,
66.3870924489706));
#199662=CARTESIAN_POINT('Ctrl Pts',(3.95336085692254,-5.49210587433934,
66.3954367419593));
#199663=CARTESIAN_POINT('Ctrl Pts',(4.09254239179647,-5.39191938038484,
66.4034913521744));
#199664=CARTESIAN_POINT('Ctrl Pts',(4.22777818736746,-5.28653571229999,
66.4115459623895));
#199665=CARTESIAN_POINT('Ctrl Pts',(4.35866773324423,-5.17632153089195,
66.4196005726045));
#199666=CARTESIAN_POINT('Ctrl Pts',(4.48965636435639,-5.06602391579152,
66.4276612802733));
#199667=CARTESIAN_POINT('Ctrl Pts',(4.61629192016794,-4.95088875587905,
66.4357219879421));
#199668=CARTESIAN_POINT('Ctrl Pts',(4.7382119034419,-4.83131834576045,66.4437826956108));
#199669=CARTESIAN_POINT('Ctrl Pts',(4.8603037865879,-4.71157934852719,66.4518547683945));
#199670=CARTESIAN_POINT('Ctrl Pts',(4.97766657782695,-4.58739289333984,
66.4599268411782));
#199671=CARTESIAN_POINT('Ctrl Pts',(5.08997869338911,-4.45919341370667,
66.4679989139619));
#199672=CARTESIAN_POINT('Ctrl Pts',(5.10174253423307,-4.44576549217625,
66.4688444022605));
#199673=CARTESIAN_POINT('Ctrl Pts',(5.11345100424188,-4.43229356882661,
66.4696898905592));
#199674=CARTESIAN_POINT('Ctrl Pts',(5.12510376216945,-4.41877815996646,
66.4705353788579));
#199675=CARTESIAN_POINT('Ctrl Pts',(5.23995044138292,-4.28557365718281,
66.4788683009027));
#199676=CARTESIAN_POINT('Ctrl Pts',(5.34974824041682,-4.14771789045397,
66.4872012229475));
#199677=CARTESIAN_POINT('Ctrl Pts',(5.45410511793379,-4.00562434116437,
66.4955341449923));
#199678=CARTESIAN_POINT('Ctrl Pts',(5.55833867092831,-3.86369871199201,
66.503857219544));
#199679=CARTESIAN_POINT('Ctrl Pts',(5.65714390696477,-3.7175455546957,66.5121802940957));
#199680=CARTESIAN_POINT('Ctrl Pts',(5.75016747625841,-3.56761306688099,
66.5205033686474));
#199681=CARTESIAN_POINT('Ctrl Pts',(5.8430981892616,-3.41783024193927,66.5288181350915));
#199682=CARTESIAN_POINT('Ctrl Pts',(5.93025855144572,-3.26427589640551,
66.5371329015355));
#199683=CARTESIAN_POINT('Ctrl Pts',(6.01133703373258,-3.10742917326769,
66.5454476679795));
#199684=CARTESIAN_POINT('Ctrl Pts',(6.0923494558588,-2.95071024383589,66.5537556598172));
#199685=CARTESIAN_POINT('Ctrl Pts',(6.16728971288715,-2.79070458971096,
66.5620636516548));
#199686=CARTESIAN_POINT('Ctrl Pts',(6.23589084995342,-2.62791824596337,
66.5703716434924));
#199687=CARTESIAN_POINT('Ctrl Pts',(6.30444866989683,-2.46523469112503,
66.5786743893776));
#199688=CARTESIAN_POINT('Ctrl Pts',(6.36667521211871,-2.29977426554493,
66.5869771352627));
#199689=CARTESIAN_POINT('Ctrl Pts',(6.42235044863246,-2.13206559818182,
66.5952798811479));
#199690=CARTESIAN_POINT('Ctrl Pts',(6.47800293245139,-1.96442546800629,
66.6035792339654));
#199691=CARTESIAN_POINT('Ctrl Pts',(6.52710933585228,-1.79453925648026,
66.611878586783));
#199692=CARTESIAN_POINT('Ctrl Pts',(6.569498468757,-1.62295374826254,66.6201779396005));
#199693=CARTESIAN_POINT('Ctrl Pts',(6.61187858620445,-1.45140473340319,
66.6284755272849));
#199694=CARTESIAN_POINT('Ctrl Pts',(6.64754419595931,-1.27815747942175,
66.6367731149694));
#199695=CARTESIAN_POINT('Ctrl Pts',(6.67637444601388,-1.10377228476385,
66.6450707026538));
#199696=CARTESIAN_POINT('Ctrl Pts',(6.7052033552322,-0.929395200406484,
66.6533679044343));
#199697=CARTESIAN_POINT('Ctrl Pts',(6.72719748165547,-0.753880624083096,
66.6616651062149));
#199698=CARTESIAN_POINT('Ctrl Pts',(6.74228737057286,-0.57779755331233,
66.6699623079954));
#199699=CARTESIAN_POINT('Ctrl Pts',(6.7573790651445,-0.401693412462954,
66.6782605026181));
#199700=CARTESIAN_POINT('Ctrl Pts',(6.76556484688301,-0.225020988278597,
66.6865586972408));
#199701=CARTESIAN_POINT('Ctrl Pts',(6.76682724616212,-0.0483530826106249,
66.6948568918634));
#199702=CARTESIAN_POINT('Ctrl Pts',(6.76809053330137,0.128439075655805,
66.7031609227031));
#199703=CARTESIAN_POINT('Ctrl Pts',(6.76242070568186,0.305226360734584,
66.7114649535429));
#199704=CARTESIAN_POINT('Ctrl Pts',(6.74985244375693,0.481436379502573,
66.7197689843826));
#199705=CARTESIAN_POINT('Ctrl Pts',(6.73727961166603,0.657710473083544,
66.7280760347965));
#199706=CARTESIAN_POINT('Ctrl Pts',(6.71780337770929,0.83340653552811,66.7363830852104));
#199707=CARTESIAN_POINT('Ctrl Pts',(6.69151021186395,1.0079583743987,66.7446901356244));
#199708=CARTESIAN_POINT('Ctrl Pts',(6.66518893418664,1.18269683864544,66.7530060676772));
#199709=CARTESIAN_POINT('Ctrl Pts',(6.63203622137704,1.35628829190802,66.76132199973));
#199710=CARTESIAN_POINT('Ctrl Pts',(6.59218969367674,1.52817670528714,66.7696379317829));
#199711=CARTESIAN_POINT('Ctrl Pts',(6.56215253461373,1.65774984281592,66.7759066580244));
#199712=CARTESIAN_POINT('Ctrl Pts',(6.52831269653172,1.78635544844846,66.7821753842659));
#199713=CARTESIAN_POINT('Ctrl Pts',(6.49074769299697,1.91376158020129,66.7884441105074));
#199714=CARTESIAN_POINT('Ctrl Pts',(6.44010991381911,2.08550556951401,66.7968943792489));
#199715=CARTESIAN_POINT('Ctrl Pts',(6.38260852795585,2.25538432239095,66.8053446479904));
#199716=CARTESIAN_POINT('Ctrl Pts',(6.31840008856451,2.4228308485794,66.813794916732));
#199717=CARTESIAN_POINT('Ctrl Pts',(6.25424831530007,2.59012959752562,66.8222377278245));
#199718=CARTESIAN_POINT('Ctrl Pts',(6.18340140471071,2.75500009003148,66.8306805389171));
#199719=CARTESIAN_POINT('Ctrl Pts',(6.10606559760062,2.91689079634432,66.8391233500096));
#199720=CARTESIAN_POINT('Ctrl Pts',(6.02878751249635,3.07866067044965,66.8475598595453));
#199721=CARTESIAN_POINT('Ctrl Pts',(5.94503032796038,3.23745489367703,66.8559963690809));
#199722=CARTESIAN_POINT('Ctrl Pts',(5.85504839435968,3.39274185574236,66.8644328786165));
#199723=CARTESIAN_POINT('Ctrl Pts',(5.76513084767753,3.54791770162495,66.8728633513753));
#199724=CARTESIAN_POINT('Ctrl Pts',(5.66899760227697,3.69959100601353,66.8812938241341));
#199725=CARTESIAN_POINT('Ctrl Pts',(5.56694903640641,3.84725453096799,66.8897242968929));
#199726=CARTESIAN_POINT('Ctrl Pts',(5.46494434094009,3.99485457576989,66.8981511454141));
#199727=CARTESIAN_POINT('Ctrl Pts',(5.35702958269231,4.1384480053,66.9065779939354));
#199728=CARTESIAN_POINT('Ctrl Pts',(5.2435489204202,4.27755581134369,66.9150048424566));
#199729=CARTESIAN_POINT('Ctrl Pts',(5.13010328558069,4.41662067976962,66.9234290899102));
#199730=CARTESIAN_POINT('Ctrl Pts',(5.01109538216323,4.55120242920022,66.9318533373639));
#199731=CARTESIAN_POINT('Ctrl Pts',(4.88691040477964,4.68085416304081,66.9402775848175));
#199732=CARTESIAN_POINT('Ctrl Pts',(4.85191983117837,4.71738505937837,66.9426512153224));
#199733=CARTESIAN_POINT('Ctrl Pts',(4.81651849292903,4.75352476956623,66.9450248458273));
#199734=CARTESIAN_POINT('Ctrl Pts',(4.78071556426013,4.7892637945347,66.9473984763321));
#199735=CARTESIAN_POINT('Ctrl Pts',(4.65068866603528,4.91905861118802,66.956018883197));
#199736=CARTESIAN_POINT('Ctrl Pts',(4.51542036286421,5.0435076761011,66.9646392900618));
#199737=CARTESIAN_POINT('Ctrl Pts',(4.37537611229567,5.162206202386,66.9732596969266));
#199738=CARTESIAN_POINT('Ctrl Pts',(4.23526607529101,5.28096048785404,66.9818841532675));
#199739=CARTESIAN_POINT('Ctrl Pts',(4.09037584969622,5.39395865182629,66.9905086096085));
#199740=CARTESIAN_POINT('Ctrl Pts',(3.94120298921011,5.50083702702064,66.9991330659494));
#199741=CARTESIAN_POINT('Ctrl Pts',(3.79187566396558,5.60782607209389,67.0077664526987));
#199742=CARTESIAN_POINT('Ctrl Pts',(3.63825708990562,5.70868248803072,67.0163998394481));
#199743=CARTESIAN_POINT('Ctrl Pts',(3.48087406380763,5.80308579567038,67.0250332261974));
#199744=CARTESIAN_POINT('Ctrl Pts',(3.35589972543279,5.87804934927062,67.0318888053769));
#199745=CARTESIAN_POINT('Ctrl Pts',(3.22855226664415,5.94894467623928,67.0387443845565));
#199746=CARTESIAN_POINT('Ctrl Pts',(3.09910619832127,6.01563211736944,67.045599963736));
#199747=CARTESIAN_POINT('Ctrl Pts',(3.09910619832142,6.01563211736936,65.0458684084508));
#199748=CARTESIAN_POINT('Ctrl Pts',(2.94516114955274,6.09494083265172,65.0539895899452));
#199749=CARTESIAN_POINT('Ctrl Pts',(2.78812931881981,6.16835713904708,65.0621107714396));
#199750=CARTESIAN_POINT('Ctrl Pts',(2.62850896512945,6.23564187716342,65.0702319529339));
#199751=CARTESIAN_POINT('Ctrl Pts',(2.46889259069812,6.30292493790344,65.0783529319711));
#199752=CARTESIAN_POINT('Ctrl Pts',(2.30668815948071,6.36407659300713,65.0864739110084));
#199753=CARTESIAN_POINT('Ctrl Pts',(2.14241424949784,6.4189056842696,65.0945948900456));
#199754=CARTESIAN_POINT('Ctrl Pts',(1.97811308399406,6.4737438725058,65.1027172164757));
#199755=CARTESIAN_POINT('Ctrl Pts',(1.81174210374682,6.52225729344709,65.1108395429059));
#199756=CARTESIAN_POINT('Ctrl Pts',(1.64383534460238,6.56430456025892,65.1189618693361));
#199757=CARTESIAN_POINT('Ctrl Pts',(1.47580182462047,6.60638357056207,65.1270903276987));
#199758=CARTESIAN_POINT('Ctrl Pts',(1.30623056605353,6.64198659017616,65.1352187860613));
#199759=CARTESIAN_POINT('Ctrl Pts',(1.13566669900318,6.67102317105669,65.1433472444239));
#199760=CARTESIAN_POINT('Ctrl Pts',(0.96502626010918,6.70007278743278,65.1514793519243));
#199761=CARTESIAN_POINT('Ctrl Pts',(0.79339268720288,6.72255004250854,65.1596114594246));
#199762=CARTESIAN_POINT('Ctrl Pts',(0.621316279714828,6.73841636295661,
65.167743566925));
#199763=CARTESIAN_POINT('Ctrl Pts',(0.449060062493121,6.75429926277715,
65.1758841719998));
#199764=CARTESIAN_POINT('Ctrl Pts',(0.276360451521886,6.7635574159956,65.1840247770746));
#199765=CARTESIAN_POINT('Ctrl Pts',(0.103768411007834,6.76620433602747,
65.1921653821493));
#199766=CARTESIAN_POINT('Ctrl Pts',(0.0561708232495194,6.7669343060083,
65.1944104055195));
#199767=CARTESIAN_POINT('Ctrl Pts',(0.00858139259991337,6.76716176248498,
65.1966554288896));
#199768=CARTESIAN_POINT('Ctrl Pts',(-0.0389883963188912,6.76688768230658,
65.1989004522597));
#199769=CARTESIAN_POINT('Ctrl Pts',(-0.217827952145001,6.76585727249229,
65.2073406617175));
#199770=CARTESIAN_POINT('Ctrl Pts',(-0.396759164286741,6.75773204046498,
65.2157808711752));
#199771=CARTESIAN_POINT('Ctrl Pts',(-0.575195289471173,6.74250987236728,
65.2242210806329));
#199772=CARTESIAN_POINT('Ctrl Pts',(-0.753496222855277,6.72729923731709,
65.2326548953815));
#199773=CARTESIAN_POINT('Ctrl Pts',(-0.931302485939268,6.70500241309035,
65.2410887101301));
#199774=CARTESIAN_POINT('Ctrl Pts',(-1.10802896737074,6.67566931531718,
65.2495225248788));
#199775=CARTESIAN_POINT('Ctrl Pts',(-1.28464871992387,6.64635393242521,
65.2579512462674));
#199776=CARTESIAN_POINT('Ctrl Pts',(-1.46018966272657,6.61001080215337,
65.266379967656));
#199777=CARTESIAN_POINT('Ctrl Pts',(-1.63407303125078,6.56674153051107,
65.2748086890447));
#199778=CARTESIAN_POINT('Ctrl Pts',(-1.80787808908676,6.52349174576088,
65.2832336144465));
#199779=CARTESIAN_POINT('Ctrl Pts',(-1.98002673802562,6.47332211952744,
65.2916585398483));
#199780=CARTESIAN_POINT('Ctrl Pts',(-2.14995122414666,6.4163851765453,65.3000834652502));
#199781=CARTESIAN_POINT('Ctrl Pts',(-2.31982525396339,6.35946514005961,
65.3085058890078));
#199782=CARTESIAN_POINT('Ctrl Pts',(-2.48747612213423,6.29578189993621,
65.3169283127655));
#199783=CARTESIAN_POINT('Ctrl Pts',(-2.65235165830439,6.22553770213385,
65.3253507365232));
#199784=CARTESIAN_POINT('Ctrl Pts',(-2.81722978749479,6.15529239959132,
65.3337732927415));
#199785=CARTESIAN_POINT('Ctrl Pts',(-2.97933218814459,6.07848605776204,
65.3421958489597));
#199786=CARTESIAN_POINT('Ctrl Pts',(-3.13812646407643,5.99536915422755,
65.350618405178));
#199787=CARTESIAN_POINT('Ctrl Pts',(-3.29692610410909,5.91224944298827,
65.3590412459118));
#199788=CARTESIAN_POINT('Ctrl Pts',(-3.45241710098796,5.82281889954178,
65.3674640866457));
#199789=CARTESIAN_POINT('Ctrl Pts',(-3.6040913408839,5.72737414585128,65.3758869273795));
#199790=CARTESIAN_POINT('Ctrl Pts',(-3.75579187976612,5.63191284287549,
65.3843112285603));
#199791=CARTESIAN_POINT('Ctrl Pts',(-3.9036740599332,5.53043542824901,65.392735529741));
#199792=CARTESIAN_POINT('Ctrl Pts',(-4.04725814945114,5.42328226000651,
65.4011598309217));
#199793=CARTESIAN_POINT('Ctrl Pts',(-4.19088718726476,5.31609554798974,
65.4095867692886));
#199794=CARTESIAN_POINT('Ctrl Pts',(-4.33021518465237,5.20322973938779,
65.4180137076555));
#199795=CARTESIAN_POINT('Ctrl Pts',(-4.46479464896943,5.0850661492781,65.4264406460225));
#199796=CARTESIAN_POINT('Ctrl Pts',(-4.59949511714048,4.96679631524867,
65.4348751612662));
#199797=CARTESIAN_POINT('Ctrl Pts',(-4.72943827015068,4.84321940203399,
65.4433096765099));
#199798=CARTESIAN_POINT('Ctrl Pts',(-4.8542118934293,4.71475512552768,65.4517441917537));
#199799=CARTESIAN_POINT('Ctrl Pts',(-4.9790457834363,4.58622879967588,65.4601827809405));
#199800=CARTESIAN_POINT('Ctrl Pts',(-5.09870493747933,4.45281064726322,
65.4686213701273));
#199801=CARTESIAN_POINT('Ctrl Pts',(-5.21281642764112,4.31495468014612,
65.4770599593141));
#199802=CARTESIAN_POINT('Ctrl Pts',(-5.3270554686324,4.17694462124623,65.4855079809345));
#199803=CARTESIAN_POINT('Ctrl Pts',(-5.43573424864483,4.03448709788232,
65.4939560025548));
#199804=CARTESIAN_POINT('Ctrl Pts',(-5.53852155820174,3.88806737973181,
65.5024040241752));
#199805=CARTESIAN_POINT('Ctrl Pts',(-5.59694421537717,3.80484476174419,
65.5072057440866));
#199806=CARTESIAN_POINT('Ctrl Pts',(-5.65346437173352,3.7203426353821,65.512007463998));
#199807=CARTESIAN_POINT('Ctrl Pts',(-5.70802771665664,3.63465384677545,
65.5168091839094));
#199808=CARTESIAN_POINT('Ctrl Pts',(-5.80165592211089,3.48761580290016,
65.5250487157605));
#199809=CARTESIAN_POINT('Ctrl Pts',(-5.88972869975506,3.3367539508084,65.5332882476116));
#199810=CARTESIAN_POINT('Ctrl Pts',(-5.9719198253901,3.1825245637878,65.5415277794628));
#199811=CARTESIAN_POINT('Ctrl Pts',(-6.05401972462032,3.02846636060714,
65.5497581660094));
#199812=CARTESIAN_POINT('Ctrl Pts',(-6.13025080472018,2.87104837626483,
65.5579885525561));
#199813=CARTESIAN_POINT('Ctrl Pts',(-6.20032988223659,2.71075604794014,
65.5662189391027));
#199814=CARTESIAN_POINT('Ctrl Pts',(-6.27034367833743,2.55061303822049,
65.5744416587208));
#199815=CARTESIAN_POINT('Ctrl Pts',(-6.33421674317225,2.38760134111947,
65.5826643783388));
#199816=CARTESIAN_POINT('Ctrl Pts',(-6.39171159530326,2.22223128464746,
65.5908870979569));
#199817=CARTESIAN_POINT('Ctrl Pts',(-6.44915550285331,2.05700775795885,
65.599102531653));
#199818=CARTESIAN_POINT('Ctrl Pts',(-6.50023234535129,1.88943037170787,
65.6073179653491));
#199819=CARTESIAN_POINT('Ctrl Pts',(-6.54475264039243,1.72002961488351,
65.6155333990451));
#199820=CARTESIAN_POINT('Ctrl Pts',(-6.58925005545882,1.55071591689458,
65.6237446106462));
#199821=CARTESIAN_POINT('Ctrl Pts',(-6.62719754359413,1.37958105796757,
65.6319558222473));
#199822=CARTESIAN_POINT('Ctrl Pts',(-6.65845526421439,1.2071712780114,65.6401670338484));
#199823=CARTESIAN_POINT('Ctrl Pts',(-6.68970250272006,1.03481931478131,
65.6483754918623));
#199824=CARTESIAN_POINT('Ctrl Pts',(-6.71426437929343,0.861193632037482,
65.6565839498761));
#199825=CARTESIAN_POINT('Ctrl Pts',(-6.73205200567082,0.686851361608561,
65.6647924078899));
#199826=CARTESIAN_POINT('Ctrl Pts',(-6.73997678162466,0.609178073272046,
65.6684494551713));
#199827=CARTESIAN_POINT('Ctrl Pts',(-6.74655761967025,0.53136266984976,
65.6721065024528));
#199828=CARTESIAN_POINT('Ctrl Pts',(-6.75178996115178,0.453454871503358,
65.6757635497342));
#199829=CARTESIAN_POINT('Ctrl Pts',(-6.76200376127612,0.301374835586867,
65.6829022944261));
#199830=CARTESIAN_POINT('Ctrl Pts',(-6.76707289703235,0.149005845051979,
65.690041039118));
#199831=CARTESIAN_POINT('Ctrl Pts',(-6.76699920770469,-0.00327458763509952,
65.69717978381));
#199832=CARTESIAN_POINT('',(-6.76699956272236,0.00243271768895434,65.3028202162318));
#199833=CARTESIAN_POINT('Ctrl Pts',(3.09910619832139,6.01563211736938,64.6516994535812));
#199834=CARTESIAN_POINT('Ctrl Pts',(2.94693875536856,6.09402505371204,64.6597460182975));
#199835=CARTESIAN_POINT('Ctrl Pts',(2.79163034931604,6.16672520808967,64.6677925830138));
#199836=CARTESIAN_POINT('Ctrl Pts',(2.63365580949279,6.23346982643895,64.6758391477302));
#199837=CARTESIAN_POINT('Ctrl Pts',(2.47578674824321,6.3001698798403,64.6838803398075));
#199838=CARTESIAN_POINT('Ctrl Pts',(2.31525543930568,6.36092216788117,64.6919215318849));
#199839=CARTESIAN_POINT('Ctrl Pts',(2.15256031046411,6.41551035458713,64.6999627239623));
#199840=CARTESIAN_POINT('Ctrl Pts',(1.98993821690109,6.47007403617453,64.7080003062776));
#199841=CARTESIAN_POINT('Ctrl Pts',(1.82515459071054,6.51847900726484,64.7160378885929));
#199842=CARTESIAN_POINT('Ctrl Pts',(1.65872668409159,6.56055750584373,64.7240754709082));
#199843=CARTESIAN_POINT('Ctrl Pts',(1.49230647245128,6.60263405887662,64.7321126815969));
#199844=CARTESIAN_POINT('Ctrl Pts',(1.32424249096148,6.6383846199015,64.7401498922857));
#199845=CARTESIAN_POINT('Ctrl Pts',(1.15506613979514,6.66769159549981,64.7481871029745));
#199846=CARTESIAN_POINT('Ctrl Pts',(0.985884552355947,6.69699947819488,
64.7562245624276));
#199847=CARTESIAN_POINT('Ctrl Pts',(0.815590894709271,6.71986331380237,
64.7642620218806));
#199848=CARTESIAN_POINT('Ctrl Pts',(0.644725380944703,6.73621690440307,
64.7722994813336));
#199849=CARTESIAN_POINT('Ctrl Pts',(0.473820727341555,6.75257424108971,
64.7803387819122));
#199850=CARTESIAN_POINT('Ctrl Pts',(0.302344328702447,6.76241832863058,
64.7883780824908));
#199851=CARTESIAN_POINT('Ctrl Pts',(0.130839972253854,6.76573498606475,
64.7964173830694));
#199852=CARTESIAN_POINT('Ctrl Pts',(-0.0407376591175529,6.76905306053475,
64.8044601184245));
#199853=CARTESIAN_POINT('Ctrl Pts',(-0.212342899062803,6.7658381466579,
64.8125028537795));
#199854=CARTESIAN_POINT('Ctrl Pts',(-0.383433663236555,6.75612815345424,
64.8205455891346));
#199855=CARTESIAN_POINT('Ctrl Pts',(-0.554732208459059,6.7464063679567,
64.8285980919835));
#199856=CARTESIAN_POINT('Ctrl Pts',(-0.725514657581686,6.73017377492276,
64.8366505948325));
#199857=CARTESIAN_POINT('Ctrl Pts',(-0.895244939809831,6.70752007061812,
64.8447030976814));
#199858=CARTESIAN_POINT('Ctrl Pts',(-1.06509117150887,6.68485089067181,
64.8527611015136));
#199859=CARTESIAN_POINT('Ctrl Pts',(-1.23388343868523,6.65575192782333,
64.8608191053458));
#199860=CARTESIAN_POINT('Ctrl Pts',(-1.40109804990698,6.62036352888169,
64.868877109178));
#199861=CARTESIAN_POINT('Ctrl Pts',(-1.56856798368071,6.58492109485148,
64.8769474168997));
#199862=CARTESIAN_POINT('Ctrl Pts',(-1.73445509191011,6.54317014206269,
64.8850177246215));
#199863=CARTESIAN_POINT('Ctrl Pts',(-1.89825211904073,6.49530044667353,
64.8930880323432));
#199864=CARTESIAN_POINT('Ctrl Pts',(-1.98332680267741,6.47043736300005,
64.8972796766502));
#199865=CARTESIAN_POINT('Ctrl Pts',(-2.06783799326545,6.44392443317852,
64.9014713209572));
#199866=CARTESIAN_POINT('Ctrl Pts',(-2.15171708220286,6.4157932165989,64.9056629652642));
#199867=CARTESIAN_POINT('Ctrl Pts',(-2.31846737356143,6.35986880658982,
64.9139958873109));
#199868=CARTESIAN_POINT('Ctrl Pts',(-2.48325016122551,6.29736759062251,
64.9223288093576));
#199869=CARTESIAN_POINT('Ctrl Pts',(-2.64551726842098,6.22844502123013,
64.9306617314043));
#199870=CARTESIAN_POINT('Ctrl Pts',(-2.80759261524595,6.15960390160087,
64.9389848059579));
#199871=CARTESIAN_POINT('Ctrl Pts',(-2.96715788637728,6.08435668026371,
64.9473078805115));
#199872=CARTESIAN_POINT('Ctrl Pts',(-3.12368045659504,6.0029084121854,64.9556309550651));
#199873=CARTESIAN_POINT('Ctrl Pts',(-3.28004678570824,5.92154144591137,
64.9639457215111));
#199874=CARTESIAN_POINT('Ctrl Pts',(-3.43337615830418,5.83398592477317,
64.9722604879571));
#199875=CARTESIAN_POINT('Ctrl Pts',(-3.58315611628153,5.74049486075497,
64.980575254403));
#199876=CARTESIAN_POINT('Ctrl Pts',(-3.73281403832754,5.64707997027311,
64.9888832462426));
#199877=CARTESIAN_POINT('Ctrl Pts',(-3.87892801431128,5.54773935666794,
64.9971912380821));
#199878=CARTESIAN_POINT('Ctrl Pts',(-4.02101018996412,5.44277190889024,
65.0054992299216));
#199879=CARTESIAN_POINT('Ctrl Pts',(-4.1630026500332,5.33787074117765,65.0138019758087));
#199880=CARTESIAN_POINT('Ctrl Pts',(-4.30096810421492,5.2273500261231,65.0221047216957));
#199881=CARTESIAN_POINT('Ctrl Pts',(-4.43444751909432,5.1115520344019,65.0304074675828));
#199882=CARTESIAN_POINT('Ctrl Pts',(-4.56787238519079,4.9958013656295,65.0387068204023));
#199883=CARTESIAN_POINT('Ctrl Pts',(-4.69681460257618,4.8747779451232,65.0470061732217));
#199884=CARTESIAN_POINT('Ctrl Pts',(-4.8208478673979,4.74886458423538,65.0553055260411));
#199885=CARTESIAN_POINT('Ctrl Pts',(-4.94485475242528,4.62297800300681,
65.0636031137275));
#199886=CARTESIAN_POINT('Ctrl Pts',(-5.06395452086855,4.49220380103383,
65.0719007014138));
#199887=CARTESIAN_POINT('Ctrl Pts',(-5.17775725781825,4.35696210439229,
65.0801982891002));
#199888=CARTESIAN_POINT('Ctrl Pts',(-5.29155470203395,4.22172669756719,
65.0884954908826));
#199889=CARTESIAN_POINT('Ctrl Pts',(-5.40005538181477,4.0820244763973,65.096792692665));
#199890=CARTESIAN_POINT('Ctrl Pts',(-5.50290913960771,3.93830928206788,
65.1050898944474));
#199891=CARTESIAN_POINT('Ctrl Pts',(-5.60577520486862,3.79457689079602,
65.1133880890719));
#199892=CARTESIAN_POINT('Ctrl Pts',(-5.70299279973539,3.64683085277139,
65.1216862836964));
#199893=CARTESIAN_POINT('Ctrl Pts',(-5.7942545278726,3.49555481522288,65.129984478321));
#199894=CARTESIAN_POINT('Ctrl Pts',(-5.88558044144718,3.34417238347352,
65.1382885091626));
#199895=CARTESIAN_POINT('Ctrl Pts',(-5.97094193825195,3.18925528955587,
65.1465925400041));
#199896=CARTESIAN_POINT('Ctrl Pts',(-6.05007667551407,3.03131344806185,
65.1548965708457));
#199897=CARTESIAN_POINT('Ctrl Pts',(-6.12924018834468,2.87331417456723,
65.1632036212614));
#199898=CARTESIAN_POINT('Ctrl Pts',(-6.20217227953624,2.71228827560603,
65.1715106716772));
#199899=CARTESIAN_POINT('Ctrl Pts',(-6.26865830620369,2.54876676847128,
65.1798177220929));
#199900=CARTESIAN_POINT('Ctrl Pts',(-6.33521541765463,2.38507042924754,
65.1881336541475));
#199901=CARTESIAN_POINT('Ctrl Pts',(-6.39531257017017,2.21887347594715,
65.1964495862022));
#199902=CARTESIAN_POINT('Ctrl Pts',(-6.44878429378962,2.05072429452921,
65.2047655182568));
#199903=CARTESIAN_POINT('Ctrl Pts',(-6.48909241483055,1.92396986997085,
65.2110342444758));
#199904=CARTESIAN_POINT('Ctrl Pts',(-6.52563667831421,1.79610645408708,
65.2173029706947));
#199905=CARTESIAN_POINT('Ctrl Pts',(-6.55836535018998,1.66737306366255,
65.2235716969137));
#199906=CARTESIAN_POINT('Ctrl Pts',(-6.60705778437594,1.47584857514759,
65.2328980618821));
#199907=CARTESIAN_POINT('Ctrl Pts',(-6.64737822743416,1.28210408866333,
65.2422244268506));
#199908=CARTESIAN_POINT('Ctrl Pts',(-6.6791523671754,1.0868360759817,65.251550791819));
#199909=CARTESIAN_POINT('Ctrl Pts',(-6.71082043881711,0.8922199049289,65.2608460236139));
#199910=CARTESIAN_POINT('Ctrl Pts',(-6.73399911643487,0.696090530314812,
65.2701412554088));
#199911=CARTESIAN_POINT('Ctrl Pts',(-6.74856552832742,0.499151590071463,
65.2794364872037));
#199912=CARTESIAN_POINT('Ctrl Pts',(-6.76078028658603,0.334007176709741,
65.2872310635324));
#199913=CARTESIAN_POINT('Ctrl Pts',(-6.76693993610197,0.168293790692667,
65.2950256398612));
#199914=CARTESIAN_POINT('Ctrl Pts',(-6.76699956272204,0.00243271858094791,
65.3028202161899));
#199915=CARTESIAN_POINT('Ctrl Pts',(-6.76699956272236,0.00243271768885066,
65.3028202162319));
#199916=CARTESIAN_POINT('Ctrl Pts',(-6.76706085584476,-0.16806406225308,
65.3108326458402));
#199917=CARTESIAN_POINT('Ctrl Pts',(-6.76067426950852,-0.338686686387149,
65.3188450754485));
#199918=CARTESIAN_POINT('Ctrl Pts',(-6.74783765965278,-0.508896766517312,
65.3268575050568));
#199919=CARTESIAN_POINT('Ctrl Pts',(-6.73500553438279,-0.679047382216446,
65.3348671354504));
#199920=CARTESIAN_POINT('Ctrl Pts',(-6.71572789968542,-0.848785364849528,
65.3428767658439));
#199921=CARTESIAN_POINT('Ctrl Pts',(-6.69005467462822,-1.01757429728013,
65.3508863962375));
#199922=CARTESIAN_POINT('Ctrl Pts',(-6.664383039394,-1.18635277740006,65.358895530632));
#199923=CARTESIAN_POINT('Ctrl Pts',(-6.6323166558608,-1.35418195066118,
65.3669046650266));
#199924=CARTESIAN_POINT('Ctrl Pts',(-6.59395706489379,-1.520532546951,65.3749137994211));
#199925=CARTESIAN_POINT('Ctrl Pts',(-6.5818041366329,-1.57323506050504,
65.3774512205269));
#199926=CARTESIAN_POINT('Ctrl Pts',(-6.56901992964328,-1.62578924170528,
65.3799886416327));
#199927=CARTESIAN_POINT('Ctrl Pts',(-6.5556087376292,-1.67817850037464,
65.3825260627384));
#199928=CARTESIAN_POINT('Ctrl Pts',(-6.51005535044735,-1.85612749863156,
65.3911448436755));
#199929=CARTESIAN_POINT('Ctrl Pts',(-6.45726888221967,-2.03215565675692,
65.3997636246127));
#199930=CARTESIAN_POINT('Ctrl Pts',(-6.39744286101652,-2.20567763737787,
65.4083824055498));
#199931=CARTESIAN_POINT('Ctrl Pts',(-6.33758090268591,-2.37930385159831,
65.4170063637363));
#199932=CARTESIAN_POINT('Ctrl Pts',(-6.27067105148898,-2.55042059634021,
65.4256303219227));
#199933=CARTESIAN_POINT('Ctrl Pts',(-6.1969554861256,-2.71846127487183,
65.4342542801092));
#199934=CARTESIAN_POINT('Ctrl Pts',(-6.12057682889995,-2.89257268977132,
65.4431897924804));
#199935=CARTESIAN_POINT('Ctrl Pts',(-6.03689170568422,-3.06338131077366,
65.4521253048515));
#199936=CARTESIAN_POINT('Ctrl Pts',(-5.9462218607113,-3.23028397872371,
65.4610608172227));
#199937=CARTESIAN_POINT('Ctrl Pts',(-5.85854978849024,-3.39166842536938,
65.4697008991173));
#199938=CARTESIAN_POINT('Ctrl Pts',(-5.7643476630778,-3.5494008285431,65.4783409810119));
#199939=CARTESIAN_POINT('Ctrl Pts',(-5.66395122491822,-3.70296442350551,
65.4869810629065));
#199940=CARTESIAN_POINT('Ctrl Pts',(-5.55840550091867,-3.86440422263979,
65.4960642905159));
#199941=CARTESIAN_POINT('Ctrl Pts',(-5.44601359654986,-4.02123602892285,
65.5051475181254));
#199942=CARTESIAN_POINT('Ctrl Pts',(-5.3272147783848,-4.17289727946407,
65.5142307457348));
#199943=CARTESIAN_POINT('Ctrl Pts',(-5.2084159602197,-4.32455853000534,
65.5233139733443));
#199944=CARTESIAN_POINT('Ctrl Pts',(-5.08321050578771,-4.47104895189418,
65.5323972009538));
#199945=CARTESIAN_POINT('Ctrl Pts',(-4.95208416720997,-4.61184902190742,
65.5414804285632));
#199946=CARTESIAN_POINT('Ctrl Pts',(-4.82151553468037,-4.75205024159449,
65.5505250234233));
#199947=CARTESIAN_POINT('Ctrl Pts',(-4.68495634081004,-4.88673948031103,
65.5595696182834));
#199948=CARTESIAN_POINT('Ctrl Pts',(-4.54287434196174,-5.01543434940042,
65.5686142131435));
#199949=CARTESIAN_POINT('Ctrl Pts',(-4.40092272571211,-5.14401112068995,
65.5776505081641));
#199950=CARTESIAN_POINT('Ctrl Pts',(-4.25345859902276,-5.2666043451153,
65.5866868031847));
#199951=CARTESIAN_POINT('Ctrl Pts',(-4.1009854905234,-5.38276945507762,
65.5957230982053));
#199952=CARTESIAN_POINT('Ctrl Pts',(-3.94878219514641,-5.49872900176823,
65.6047434027933));
#199953=CARTESIAN_POINT('Ctrl Pts',(-3.79158780679507,-5.60828300454349,
65.6137637073812));
#199954=CARTESIAN_POINT('Ctrl Pts',(-3.62993757666583,-5.71102812018199,
65.6227840119692));
#199955=CARTESIAN_POINT('Ctrl Pts',(-3.46849091359974,-5.8136438483063,
65.6317929572358));
#199956=CARTESIAN_POINT('Ctrl Pts',(-3.30259980708626,-5.90946767376026,
65.6408019025023));
#199957=CARTESIAN_POINT('Ctrl Pts',(-3.13282913410349,-5.99813892941072,
65.6498108477689));
#199958=CARTESIAN_POINT('Ctrl Pts',(-2.96344397437972,-6.08660883141073,
65.6587993356279));
#199959=CARTESIAN_POINT('Ctrl Pts',(-2.79019704353166,-6.16795847405367,
65.6677878234869));
#199960=CARTESIAN_POINT('Ctrl Pts',(-2.61367805787869,-6.24187279666636,
65.6767763113459));
#199961=CARTESIAN_POINT('Ctrl Pts',(-2.45880694221107,-6.30672244195804,
65.68466247236));
#199962=CARTESIAN_POINT('Ctrl Pts',(-2.30141762078234,-6.36584921646203,
65.692548633374));
#199963=CARTESIAN_POINT('Ctrl Pts',(-2.14192478858306,-6.41906902907683,
65.700434794388));
#199964=CARTESIAN_POINT('Ctrl Pts',(-1.97767307863398,-6.47387679131049,
65.708556259244));
#199965=CARTESIAN_POINT('Ctrl Pts',(-1.81126346644537,-6.52239374843791,
65.7166777240999));
#199966=CARTESIAN_POINT('Ctrl Pts',(-1.64322421643041,-6.56445756894937,
65.7247991889559));
#199967=CARTESIAN_POINT('Ctrl Pts',(-1.47519695008643,-6.60651838969152,
65.7329200746319));
#199968=CARTESIAN_POINT('Ctrl Pts',(-1.30554063263069,-6.64212690155737,
65.741040960308));
#199969=CARTESIAN_POINT('Ctrl Pts',(-1.13479653816351,-6.67117124776243,
65.749161845984));
#199970=CARTESIAN_POINT('Ctrl Pts',(-0.964032034895708,-6.70021906559719,
65.757283702338));
#199971=CARTESIAN_POINT('Ctrl Pts',(-0.792179856911885,-6.72270109521926,
65.7654055586921));
#199972=CARTESIAN_POINT('Ctrl Pts',(-0.61978921934128,-6.7385569911954,
65.7735274150461));
#199973=CARTESIAN_POINT('Ctrl Pts',(-0.447272807694267,-6.75442445543707,
65.781655197006));
#199974=CARTESIAN_POINT('Ctrl Pts',(-0.274217516847378,-6.76365609695529,
65.789782978966));
#199975=CARTESIAN_POINT('Ctrl Pts',(-0.101176049930937,-6.76624359648102,
65.7979107609259));
#199976=CARTESIAN_POINT('Ctrl Pts',(0.0719359076474961,-6.76883215005788,
65.8060418538421));
#199977=CARTESIAN_POINT('Ctrl Pts',(0.245033664242083,-6.76477117525787,
65.8141729467584));
#199978=CARTESIAN_POINT('Ctrl Pts',(0.417567054982159,-6.75410443764335,
65.8223040396746));
#199979=CARTESIAN_POINT('Ctrl Pts',(0.590288758708181,-6.74342605773047,
65.830444007339));
#199980=CARTESIAN_POINT('Ctrl Pts',(0.762444502348168,-6.72612755096827,
65.8385839750033));
#199981=CARTESIAN_POINT('Ctrl Pts',(0.933491004658623,-6.7023043458367,
65.8467239426677));
#199982=CARTESIAN_POINT('Ctrl Pts',(1.02220311636091,-6.68994860160228,
65.8509456818493));
#199983=CARTESIAN_POINT('Ctrl Pts',(1.1106170283355,-6.67583861200521,65.855167421031));
#199984=CARTESIAN_POINT('Ctrl Pts',(1.19865835208879,-6.65999302964859,
65.8593891602127));
#199985=CARTESIAN_POINT('Ctrl Pts',(1.37467282892736,-6.62831413421854,
65.8678293696704));
#199986=CARTESIAN_POINT('Ctrl Pts',(1.5495611299319,-6.5896297672765,65.8762695791281));
#199987=CARTESIAN_POINT('Ctrl Pts',(1.72274483837265,-6.54403844899007,
65.8847097885858));
#199988=CARTESIAN_POINT('Ctrl Pts',(1.89579733449684,-6.49848167288167,
65.8931436033344));
#199989=CARTESIAN_POINT('Ctrl Pts',(2.06714749120149,-6.44602846173389,
65.901577418083));
#199990=CARTESIAN_POINT('Ctrl Pts',(2.23622742046157,-6.38682831489745,
65.9100112328316));
#199991=CARTESIAN_POINT('Ctrl Pts',(2.40520523875857,-6.32766392028798,
65.9184399542203));
#199992=CARTESIAN_POINT('Ctrl Pts',(2.57191524901281,-6.26176082325196,
65.9268686756089));
#199993=CARTESIAN_POINT('Ctrl Pts',(2.73580467884222,-6.18931835982162,
65.9352973969975));
#199994=CARTESIAN_POINT('Ctrl Pts',(2.89962029888659,-6.11690852181844,
65.9437223223993));
#199995=CARTESIAN_POINT('Ctrl Pts',(3.06061756680526,-6.03796532419842,
65.9521472478012));
#199996=CARTESIAN_POINT('Ctrl Pts',(3.21826328826953,-5.95273637979851,
65.960572173203));
#199997=CARTESIAN_POINT('Ctrl Pts',(3.37586219941044,-5.86753274274223,
65.9689945969607));
#199998=CARTESIAN_POINT('Ctrl Pts',(3.53011125567466,-5.77604723944603,
65.9774170207185));
#199999=CARTESIAN_POINT('Ctrl Pts',(3.68050114070233,-5.67857379570688,
65.9858394444762));
#200000=CARTESIAN_POINT('Ctrl Pts',(3.8308933909307,-5.58109881899059,65.9942620006945));
#200001=CARTESIAN_POINT('Ctrl Pts',(3.97742606526254,-5.47763588942274,
66.0026845569128));
#200002=CARTESIAN_POINT('Ctrl Pts',(4.1196175984539,-5.36852305969798,66.0111071131311));
#200003=CARTESIAN_POINT('Ctrl Pts',(4.26181393490254,-5.25940654412089,
66.0195299538649));
#200004=CARTESIAN_POINT('Ctrl Pts',(4.39966857307213,-5.14463995078146,
66.0279527945988));
#200005=CARTESIAN_POINT('Ctrl Pts',(4.5327317823673,-5.02460262997158,66.0363756353326));
#200006=CARTESIAN_POINT('Ctrl Pts',(4.66581806365872,-4.90454449574056,
66.0447999365133));
#200007=CARTESIAN_POINT('Ctrl Pts',(4.79411101204902,-4.77921403542229,
66.0532242376941));
#200008=CARTESIAN_POINT('Ctrl Pts',(4.91719635750109,-4.64902882135377,
66.0616485388748));
#200009=CARTESIAN_POINT('Ctrl Pts',(5.04032023421727,-4.51880285344207,
66.0700754772417));
#200010=CARTESIAN_POINT('Ctrl Pts',(5.15823302871722,-4.38371934408376,
66.0785024156087));
#200011=CARTESIAN_POINT('Ctrl Pts',(5.27055925530196,-4.24423068839936,
66.0869293539756));
#200012=CARTESIAN_POINT('Ctrl Pts',(5.38298647728311,-4.10461661488063,
66.0953638692193));
#200013=CARTESIAN_POINT('Ctrl Pts',(5.48981688513591,-3.96058974081905,
66.103798384463));
#200014=CARTESIAN_POINT('Ctrl Pts',(5.59071633299359,-3.8126342447183,66.1122328997068));
#200015=CARTESIAN_POINT('Ctrl Pts',(5.69166451614895,-3.66460728484547,
66.1206714888936));
#200016=CARTESIAN_POINT('Ctrl Pts',(5.78667584490498,-3.51264819841815,
66.1291100780805));
#200017=CARTESIAN_POINT('Ctrl Pts',(5.87546075862826,-3.35726821594872,
66.1375486672673));
#200018=CARTESIAN_POINT('Ctrl Pts',(5.96434491379795,-3.20171455381279,
66.1459966888877));
#200019=CARTESIAN_POINT('Ctrl Pts',(6.04698858884251,-3.04273264866924,
66.1544447105081));
#200020=CARTESIAN_POINT('Ctrl Pts',(6.12314868321863,-2.88085737293569,
66.1628927321284));
#200021=CARTESIAN_POINT('Ctrl Pts',(6.16643685860994,-2.78885006405733,
66.1676944520397));
#200022=CARTESIAN_POINT('Ctrl Pts',(6.20763132310783,-2.69590839671385,
66.172496171951));
#200023=CARTESIAN_POINT('Ctrl Pts',(6.24669448972815,-2.6021331541641,66.1772978918623));
#200024=CARTESIAN_POINT('Ctrl Pts',(6.3137250978264,-2.4412191250029,66.1855374237134));
#200025=CARTESIAN_POINT('Ctrl Pts',(6.37462691919696,-2.27749044476659,
66.1937769555645));
#200026=CARTESIAN_POINT('Ctrl Pts',(6.42915679304084,-2.11145256411241,
66.2020164874156));
#200027=CARTESIAN_POINT('Ctrl Pts',(6.48362614253585,-1.94559897390137,
66.2102468739621));
#200028=CARTESIAN_POINT('Ctrl Pts',(6.53173751680025,-1.77744162189617,
66.2184772605087));
#200029=CARTESIAN_POINT('Ctrl Pts',(6.57329515882468,-1.60750731101666,
66.2267076470553));
#200030=CARTESIAN_POINT('Ctrl Pts',(6.61481408827214,-1.43773130062703,
66.2349303666733));
#200031=CARTESIAN_POINT('Ctrl Pts',(6.64979135976002,-1.26618197162173,
66.2431530862913));
#200032=CARTESIAN_POINT('Ctrl Pts',(6.67808050927068,-1.09340281310184,
66.2513758059093));
#200033=CARTESIAN_POINT('Ctrl Pts',(6.70634459255683,-0.920776749364022,
66.2595912396054));
#200034=CARTESIAN_POINT('Ctrl Pts',(6.72793230796884,-0.746923377912297,
66.2678066733014));
#200035=CARTESIAN_POINT('Ctrl Pts',(6.74274793650412,-0.572397820374476,
66.2760221069974));
#200036=CARTESIAN_POINT('Ctrl Pts',(6.75755595095667,-0.397961955422491,
66.2842333185984));
#200037=CARTESIAN_POINT('Ctrl Pts',(6.76559877987904,-0.222854946145419,
66.2924445301994));
#200038=CARTESIAN_POINT('Ctrl Pts',(6.76683231159713,-0.047638920275371,
66.3006557418004));
#200039=CARTESIAN_POINT('Ctrl Pts',(6.76806542965676,0.12751834780896,66.3088641998142));
#200040=CARTESIAN_POINT('Ctrl Pts',(6.76249379686454,0.302784204143018,
66.3170726578279));
#200041=CARTESIAN_POINT('Ctrl Pts',(6.7501253668455,0.47759452663206,66.3252811158417));
#200042=CARTESIAN_POINT('Ctrl Pts',(6.74461496119987,0.555476342390058,
66.3289381631235));
#200043=CARTESIAN_POINT('Ctrl Pts',(6.7377561528153,0.633267737723453,66.3325952104053));
#200044=CARTESIAN_POINT('Ctrl Pts',(6.72955297553951,0.710918947143271,
66.336252257687));
#200045=CARTESIAN_POINT('Ctrl Pts',(6.70968105418944,0.899026393130531,
66.3451113318621));
#200046=CARTESIAN_POINT('Ctrl Pts',(6.68193730666842,1.08611529098033,66.3539704060371));
#200047=CARTESIAN_POINT('Ctrl Pts',(6.6464619186312,1.27154746831774,66.3628294802121));
#200048=CARTESIAN_POINT('Ctrl Pts',(6.61091987947707,1.45732803540973,66.3717051988051));
#200049=CARTESIAN_POINT('Ctrl Pts',(6.56761721875264,1.64144540693416,66.3805809173982));
#200050=CARTESIAN_POINT('Ctrl Pts',(6.51674444183085,1.82327476806617,66.3894566359913));
#200051=CARTESIAN_POINT('Ctrl Pts',(6.4657264883781,2.00562301881799,66.3983576833773));
#200052=CARTESIAN_POINT('Ctrl Pts',(6.40709525846708,2.1856699418529,66.4072587307633));
#200053=CARTESIAN_POINT('Ctrl Pts',(6.34109111968594,2.36280604617479,66.4161597781494));
#200054=CARTESIAN_POINT('Ctrl Pts',(6.27499724737285,2.54018296946001,66.4250729266314));
#200055=CARTESIAN_POINT('Ctrl Pts',(6.20151054009244,2.714640928483,66.4339860751134));
#200056=CARTESIAN_POINT('Ctrl Pts',(6.12091879831441,2.88559215143812,66.4428992235955));
#200057=CARTESIAN_POINT('Ctrl Pts',(6.04014812083256,3.05692293285325,66.4518321617044));
#200058=CARTESIAN_POINT('Ctrl Pts',(5.95224096672325,3.22473116949826,66.4607650998133));
#200059=CARTESIAN_POINT('Ctrl Pts',(5.8575316046697,3.38845281807135,66.4696980379221));
#200060=CARTESIAN_POINT('Ctrl Pts',(5.76738202422048,3.54429208896595,66.4782008997854));
#200061=CARTESIAN_POINT('Ctrl Pts',(5.67106989706527,3.69642884877683,66.4867037616486));
#200062=CARTESIAN_POINT('Ctrl Pts',(5.56891896833363,3.84440249247317,66.4952066235118));
#200063=CARTESIAN_POINT('Ctrl Pts',(5.4701325162687,3.98750242745548,66.5034294323134));
#200064=CARTESIAN_POINT('Ctrl Pts',(5.36569539072126,4.1269826741663,66.511652241115));
#200065=CARTESIAN_POINT('Ctrl Pts',(5.25590168574291,4.26236864546051,66.5198750499166));
#200066=CARTESIAN_POINT('Ctrl Pts',(5.14622034499035,4.39761606108934,66.5280894433947));
#200067=CARTESIAN_POINT('Ctrl Pts',(5.03119356381535,4.52877726773737,66.5363038368728));
#200068=CARTESIAN_POINT('Ctrl Pts',(4.91115889954411,4.65540624042937,66.5445182303509));
#200069=CARTESIAN_POINT('Ctrl Pts',(4.79122524308017,4.78192865627839,66.5527257115102));
#200070=CARTESIAN_POINT('Ctrl Pts',(4.66629234101214,4.9039261742029,66.5609331926694));
#200071=CARTESIAN_POINT('Ctrl Pts',(4.53673826381348,5.02098545363863,66.5691406738287));
#200072=CARTESIAN_POINT('Ctrl Pts',(4.40728078818542,5.13795744820852,66.5773420351066));
#200073=CARTESIAN_POINT('Ctrl Pts',(4.27320926950222,5.24999830259124,66.5855433963846));
#200074=CARTESIAN_POINT('Ctrl Pts',(4.13493883468289,5.35673126388017,66.5937447576626));
#200075=CARTESIAN_POINT('Ctrl Pts',(3.99672785226157,5.4634183329977,66.6019425925859));
#200076=CARTESIAN_POINT('Ctrl Pts',(3.85432183299172,5.56480183594365,66.6101404275092));
#200077=CARTESIAN_POINT('Ctrl Pts',(3.70816941121728,5.66054490466355,66.6183382624324));
#200078=CARTESIAN_POINT('Ctrl Pts',(3.56204877618386,5.75626715019016,66.6265343144058));
#200079=CARTESIAN_POINT('Ctrl Pts',(3.4121836610716,5.84635120811245,66.6347303663791));
#200080=CARTESIAN_POINT('Ctrl Pts',(3.25905222577131,5.93050314810599,66.6429264183524));
#200081=CARTESIAN_POINT('Ctrl Pts',(3.20612009010448,5.95959150540919,66.6457595044142));
#200082=CARTESIAN_POINT('Ctrl Pts',(3.15279792204455,5.98797145751809,66.6485925904762));
#200083=CARTESIAN_POINT('Ctrl Pts',(3.09910619832135,6.0156321173694,66.651425676538));
#200084=CARTESIAN_POINT('Origin',(0.,0.,4.30282021618968));
#200085=CARTESIAN_POINT('',(3.09910619832131,6.01563211736941,69.0457552630242));
#200086=CARTESIAN_POINT('',(3.09910619832137,6.01563211736939,68.6512130080706));
#200087=CARTESIAN_POINT('',(3.09910619832133,6.0156321173694,4.30282021618968));
#200088=CARTESIAN_POINT('',(-6.76699999999839,-4.66729631973904E-6,67.6970790042622));
#200089=CARTESIAN_POINT('Ctrl Pts',(-6.767,2.1130229668672E-12,67.69717978381));
#200090=CARTESIAN_POINT('Ctrl Pts',(-6.76700000000006,-0.186007249524881,
67.7059292956212));
#200091=CARTESIAN_POINT('Ctrl Pts',(-6.75932637294531,-0.372014355748052,
67.7146788074324));
#200092=CARTESIAN_POINT('Ctrl Pts',(-6.74400518264195,-0.557389537485753,
67.7234283192436));
#200093=CARTESIAN_POINT('Ctrl Pts',(-6.72868405705103,-0.742763936250253,
67.7321777940992));
#200094=CARTESIAN_POINT('Ctrl Pts',(-6.70571545645744,-0.927506130240924,
67.7409272689549));
#200095=CARTESIAN_POINT('Ctrl Pts',(-6.6751773940482,-1.11098863990046,
67.7496767438106));
#200096=CARTESIAN_POINT('Ctrl Pts',(-6.64463945808692,-1.29447038982,67.7584261824376));
#200097=CARTESIAN_POINT('Ctrl Pts',(-6.60653217008338,-1.47669218313759,
67.7671756210647));
#200098=CARTESIAN_POINT('Ctrl Pts',(-6.56098496092652,-1.65703510599384,
67.7759250596917));
#200099=CARTESIAN_POINT('Ctrl Pts',(-6.51543793658267,-1.83737729708808,
67.7846744628169));
#200100=CARTESIAN_POINT('Ctrl Pts',(-6.46245112167384,-2.01584035511044,
67.793423865942));
#200101=CARTESIAN_POINT('Ctrl Pts',(-6.4022044837421,-2.19181813760918,
67.8021732690672));
#200102=CARTESIAN_POINT('Ctrl Pts',(-6.3419580852645,-2.3677952206729,67.8109226374173));
#200103=CARTESIAN_POINT('Ctrl Pts',(-6.27445201433038,-2.5412867768433,
67.8196720057674));
#200104=CARTESIAN_POINT('Ctrl Pts',(-6.19991555071822,-2.71170355384994,
67.8284213741175));
#200105=CARTESIAN_POINT('Ctrl Pts',(-6.1253793771661,-2.88211966767651,
67.8371707084193));
#200106=CARTESIAN_POINT('Ctrl Pts',(-6.04381298052437,-3.0494607637195,
67.8459200427211));
#200107=CARTESIAN_POINT('Ctrl Pts',(-5.95549339335747,-3.21315848374703,
67.8546693770228));
#200108=CARTESIAN_POINT('Ctrl Pts',(-5.86717414255332,-3.37685558033625,
67.863418678003));
#200109=CARTESIAN_POINT('Ctrl Pts',(-5.7721018887653,-3.53690907646867,
67.8721679789832));
#200110=CARTESIAN_POINT('Ctrl Pts',(-5.67059953346938,-3.69277536969376,
67.8809172799634));
#200111=CARTESIAN_POINT('Ctrl Pts',(-5.56909755631334,-3.84864108224995,
67.8896665483486));
#200112=CARTESIAN_POINT('Ctrl Pts',(-5.4611656819681,-4.00031938297571,
67.8984158167339));
#200113=CARTESIAN_POINT('Ctrl Pts',(-5.34717048533573,-4.14729511859892,
67.9071650851192));
#200114=CARTESIAN_POINT('Ctrl Pts',(-5.2331757039181,-4.29427031887948,
67.9159143216362));
#200115=CARTESIAN_POINT('Ctrl Pts',(-5.11311782003492,-4.43654276189572,
67.9246635581532));
#200116=CARTESIAN_POINT('Ctrl Pts',(-4.98740458984735,-4.57362924351871,
67.9334127946703));
#200117=CARTESIAN_POINT('Ctrl Pts',(-4.86169180711733,-4.71071523720276,
67.9421620000457));
#200118=CARTESIAN_POINT('Ctrl Pts',(-4.7303239120417,-4.84261509523238,
67.9509112054212));
#200119=CARTESIAN_POINT('Ctrl Pts',(-4.59374707013607,-4.96888084538322,
67.9596604107966));
#200120=CARTESIAN_POINT('Ctrl Pts',(-4.45717070301462,-5.09514615659448,
67.9684095857571));
#200121=CARTESIAN_POINT('Ctrl Pts',(-4.31538563571067,-5.21577720459505,
67.9771587607175));
#200122=CARTESIAN_POINT('Ctrl Pts',(-4.16887341029545,-5.33036429232858,
67.9859079356779));
#200123=CARTESIAN_POINT('Ctrl Pts',(-4.02236168203755,-5.44495099123579,
67.9946570809499));
#200124=CARTESIAN_POINT('Ctrl Pts',(-3.87112305348227,-5.55349359438558,
68.003406226222));
#200125=CARTESIAN_POINT('Ctrl Pts',(-3.71567117017836,-5.65562346298844,
68.012155371494));
#200126=CARTESIAN_POINT('Ctrl Pts',(-3.56021980145894,-5.75775299351597,
68.0209044878041));
#200127=CARTESIAN_POINT('Ctrl Pts',(-3.40055544538425,-5.85346967463829,
68.0296536041143));
#200128=CARTESIAN_POINT('Ctrl Pts',(-3.23722035986929,-5.9424484298686,
68.0384027204245));
#200129=CARTESIAN_POINT('Ctrl Pts',(-3.07388580147251,-6.03142689794493,
68.0471518084993));
#200130=CARTESIAN_POINT('Ctrl Pts',(-2.90688078896643,-6.11366734656751,
68.0559008965742));
#200131=CARTESIAN_POINT('Ctrl Pts',(-2.7367725072143,-6.18889046952327,
68.064649984649));
#200132=CARTESIAN_POINT('Ctrl Pts',(-2.56666476031555,-6.26411335596296,
68.0733990452151));
#200133=CARTESIAN_POINT('Ctrl Pts',(-2.39345402575253,-6.33231884500522,
68.0821481057811));
#200134=CARTESIAN_POINT('Ctrl Pts',(-2.21772856065693,-6.39327529762692,
68.0908971663471));
#200135=CARTESIAN_POINT('Ctrl Pts',(-2.0420036334863,-6.45423156365074,
68.0996462001308));
#200136=CARTESIAN_POINT('Ctrl Pts',(-1.8637642618941,-6.5079387437562,68.1083952339145));
#200137=CARTESIAN_POINT('Ctrl Pts',(-1.683615777533,-6.55421443909504,68.1171442676981));
#200138=CARTESIAN_POINT('Ctrl Pts',(-1.50346782967971,-6.60048999661828,
68.125893275426));
#200139=CARTESIAN_POINT('Ctrl Pts',(-1.32141105795185,-6.63933404237672,
68.1346422831538));
#200140=CARTESIAN_POINT('Ctrl Pts',(-1.13806375487247,-6.67061465607522,
68.1433912908816));
#200141=CARTESIAN_POINT('Ctrl Pts',(-0.954716982605532,-6.7018951792126,
68.15214027328));
#200142=CARTESIAN_POINT('Ctrl Pts',(-0.77007996890492,-6.72561226592196,
68.1608892556784));
#200143=CARTESIAN_POINT('Ctrl Pts',(-0.584779765561294,-6.74168536983076,
68.1696382380768));
#200144=CARTESIAN_POINT('Ctrl Pts',(-0.391489830654349,-6.75845151013835,
68.1787644570866));
#200145=CARTESIAN_POINT('Ctrl Pts',(-0.197478578241385,-6.76689983031616,
68.1878906760965));
#200146=CARTESIAN_POINT('Ctrl Pts',(-0.00346287645438857,-6.76699911397118,
68.1970168951064));
#200147=CARTESIAN_POINT('Ctrl Pts',(0.184489834651796,-6.76709529501197,
68.2058579197722));
#200148=CARTESIAN_POINT('Ctrl Pts',(0.372446404247341,-6.7593563973818,
68.214698944438));
#200149=CARTESIAN_POINT('Ctrl Pts',(0.55975501948637,-6.74380925873203,
68.2235399691038));
#200150=CARTESIAN_POINT('Ctrl Pts',(0.745134705519926,-6.72842222659826,
68.2322899477135));
#200151=CARTESIAN_POINT('Ctrl Pts',(0.929879431226838,-6.70538706057548,
68.2410399263233));
#200152=CARTESIAN_POINT('Ctrl Pts',(1.11336163626664,-6.67478200894154,
68.2497899049331));
#200153=CARTESIAN_POINT('Ctrl Pts',(1.29684196300578,-6.64417727061041,
68.2585397939696));
#200154=CARTESIAN_POINT('Ctrl Pts',(1.47905951217389,-6.60600284890618,
68.2672896830061));
#200155=CARTESIAN_POINT('Ctrl Pts',(1.65939532066983,-6.56038841607256,
68.2760395720427));
#200156=CARTESIAN_POINT('Ctrl Pts',(1.83972934300704,-6.51477443503284,
68.2847893744148));
#200157=CARTESIAN_POINT('Ctrl Pts',(2.0181813840617,-6.46172066062171,68.293539176787));
#200158=CARTESIAN_POINT('Ctrl Pts',(2.19414528354108,-6.4014073042351,68.3022889791591));
#200159=CARTESIAN_POINT('Ctrl Pts',(2.37010749863917,-6.34109452518673,
68.3110386977754));
#200160=CARTESIAN_POINT('Ctrl Pts',(2.54358134866386,-6.27352239616534,
68.3197884163918));
#200161=CARTESIAN_POINT('Ctrl Pts',(2.71397759435491,-6.19892043966847,
68.3285381350081));
#200162=CARTESIAN_POINT('Ctrl Pts',(2.88437226558068,-6.12431917249542,
68.3372877727768));
#200163=CARTESIAN_POINT('Ctrl Pts',(3.05168912680908,-6.04268832278823,
68.3460374105455));
#200164=CARTESIAN_POINT('Ctrl Pts',(3.21535986273816,-5.95430516123355,
68.3547870483143));
#200165=CARTESIAN_POINT('Ctrl Pts',(3.37902914072811,-5.86592278697458,
68.3635366081433));
#200166=CARTESIAN_POINT('Ctrl Pts',(3.5390521062155,-5.77078835741955,68.3722861679724));
#200167=CARTESIAN_POINT('Ctrl Pts',(3.69488522831682,-5.66922500431639,
68.3810357278015));
#200168=CARTESIAN_POINT('Ctrl Pts',(3.85071701406938,-5.56766252217095,
68.3897852125986));
#200169=CARTESIAN_POINT('Ctrl Pts',(4.00235878822414,-5.45967138329363,
68.3985346973957));
#200170=CARTESIAN_POINT('Ctrl Pts',(4.14929549611346,-5.34561838199591,
68.4072841821928));
#200171=CARTESIAN_POINT('Ctrl Pts',(4.29623099276113,-5.23156632086997,
68.4160335948654));
#200172=CARTESIAN_POINT('Ctrl Pts',(4.43846127436053,-5.11145267304943,
68.424783007538));
#200173=CARTESIAN_POINT('Ctrl Pts',(4.57550326054469,-4.98568540049861,
68.4335324202106));
#200174=CARTESIAN_POINT('Ctrl Pts',(4.71254416257801,-4.85991912290341,
68.4422817636658));
#200175=CARTESIAN_POINT('Ctrl Pts',(4.84439664018775,-4.72849950385404,
68.4510311071211));
#200176=CARTESIAN_POINT('Ctrl Pts',(4.97061286794753,-4.59187289861059,
68.4597804505763));
#200177=CARTESIAN_POINT('Ctrl Pts',(5.09682813912688,-4.4552473288468,68.4685297277211));
#200178=CARTESIAN_POINT('Ctrl Pts',(5.21740705147838,-4.31341506235788,
68.477279004866));
#200179=CARTESIAN_POINT('Ctrl Pts',(5.33194007545692,-4.16685781275729,
68.4860282820108));
#200180=CARTESIAN_POINT('Ctrl Pts',(5.44647226944478,-4.02030162521851,
68.4947774957519));
#200181=CARTESIAN_POINT('Ctrl Pts',(5.55495848628103,-3.86902074887949,
68.503526709493));
#200182=CARTESIAN_POINT('Ctrl Pts',(5.65703027291775,-3.71352898080683,
68.5122759232341));
#200183=CARTESIAN_POINT('Ctrl Pts',(5.75910135376981,-3.55803828789614,
68.521025076478));
#200184=CARTESIAN_POINT('Ctrl Pts',(5.85475793592734,-3.39833700106744,
68.5297742297219));
#200185=CARTESIAN_POINT('Ctrl Pts',(5.94367514427378,-3.23496750823591,
68.5385233829658));
#200186=CARTESIAN_POINT('Ctrl Pts',(6.03259176732621,-3.07159909077763,
68.5472724786187));
#200187=CARTESIAN_POINT('Ctrl Pts',(6.11476896835906,-2.90456276731473,
68.5560215742716));
#200188=CARTESIAN_POINT('Ctrl Pts',(6.18992765547868,-2.7344258300309,68.5647706699246));
#200189=CARTESIAN_POINT('Ctrl Pts',(6.26508587283039,-2.56428995616207,
68.5735197108926));
#200190=CARTESIAN_POINT('Ctrl Pts',(6.33322554827147,-2.39105376935236,
68.5822687518606));
#200191=CARTESIAN_POINT('Ctrl Pts',(6.3941152673302,-2.21530561054111,68.5910177928287));
#200192=CARTESIAN_POINT('Ctrl Pts',(6.45500462602829,-2.03955849185153,
68.5997667820177));
#200193=CARTESIAN_POINT('Ctrl Pts',(6.50864402040717,-1.86129970164624,
68.6085157712067));
#200194=CARTESIAN_POINT('Ctrl Pts',(6.55485128368574,-1.68113463136163,
68.6172647603957));
#200195=CARTESIAN_POINT('Ctrl Pts',(6.601998095543,-1.49730620116987,68.6261916458672));
#200196=CARTESIAN_POINT('Ctrl Pts',(6.64140720707847,-1.31149343245829,
68.6351185313386));
#200197=CARTESIAN_POINT('Ctrl Pts',(6.67293928722859,-1.12435326697669,
68.64404541681));
#200198=CARTESIAN_POINT('Ctrl Pts',(6.70384625876235,-0.940923067008094,
68.6527953309875));
#200199=CARTESIAN_POINT('Ctrl Pts',(6.72718554579778,-0.756217899523231,
68.6615452451649));
#200200=CARTESIAN_POINT('Ctrl Pts',(6.74287786815314,-0.570865181256125,
68.6702951593424));
#200201=CARTESIAN_POINT('Ctrl Pts',(6.75856988190837,-0.385516108075555,
68.6790449014469));
#200202=CARTESIAN_POINT('Ctrl Pts',(6.76661520773398,-0.199519795227935,
68.6877946435514));
#200203=CARTESIAN_POINT('Ctrl Pts',(6.76698651789579,-0.0135080204572116,
68.6965443856559));
#200204=CARTESIAN_POINT('Ctrl Pts',(6.76735782124907,0.17250034351142,68.7052939673208));
#200205=CARTESIAN_POINT('Ctrl Pts',(6.76005538995192,0.358523882209404,
68.7140435489858));
#200206=CARTESIAN_POINT('Ctrl Pts',(6.74510402742373,0.543930748562886,
68.7227931306508));
#200207=CARTESIAN_POINT('Ctrl Pts',(6.73015291918047,0.729334461613647,
68.7315425635074));
#200208=CARTESIAN_POINT('Ctrl Pts',(6.70755316306617,0.914121237632997,
68.7402919963641));
#200209=CARTESIAN_POINT('Ctrl Pts',(6.67738151874603,1.09766345165944,68.7490414292208));
#200210=CARTESIAN_POINT('Ctrl Pts',(6.64721034747604,1.28120278799484,68.7577907248983));
#200211=CARTESIAN_POINT('Ctrl Pts',(6.60946757205182,1.46349731860147,68.7665400205758));
#200212=CARTESIAN_POINT('Ctrl Pts',(6.56428138111569,1.64392790277978,68.7752893162534));
#200213=CARTESIAN_POINT('Ctrl Pts',(6.51909583859903,1.82435589778866,68.784038486379));
#200214=CARTESIAN_POINT('Ctrl Pts',(6.46646716392936,2.00291972192069,68.7927876565046));
#200215=CARTESIAN_POINT('Ctrl Pts',(6.40657409872952,2.17901292274462,68.8015368266302));
#200216=CARTESIAN_POINT('Ctrl Pts',(6.34668181342152,2.35510383058773,68.8102858828293));
#200217=CARTESIAN_POINT('Ctrl Pts',(6.27952541914134,2.52872390822373,68.8190349390284));
#200218=CARTESIAN_POINT('Ctrl Pts',(6.20533299175608,2.69928350890075,68.8277839952275));
#200219=CARTESIAN_POINT('Ctrl Pts',(6.12831602991641,2.87633637965428,68.8368661313857));
#200220=CARTESIAN_POINT('Ctrl Pts',(6.04371690605362,3.05009086601281,68.8459482675439));
#200221=CARTESIAN_POINT('Ctrl Pts',(5.95184520316721,3.21991112882568,68.8550304037021));
#200222=CARTESIAN_POINT('Ctrl Pts',(5.86333549509366,3.38351691182858,68.8637801840457));
#200223=CARTESIAN_POINT('Ctrl Pts',(5.76807618099461,3.54347103711853,68.8725299643892));
#200224=CARTESIAN_POINT('Ctrl Pts',(5.66639083309109,3.69923018027552,68.8812797447328));
#200225=CARTESIAN_POINT('Ctrl Pts',(5.56470914082296,3.85498372381912,68.8900292105177));
#200226=CARTESIAN_POINT('Ctrl Pts',(5.45660203372165,4.00654234701864,68.8987786763026));
#200227=CARTESIAN_POINT('Ctrl Pts',(5.34243669839317,4.1533912798654,68.9075281420876));
#200228=CARTESIAN_POINT('Ctrl Pts',(5.228274860507,4.30023571401148,68.9162773398336));
#200229=CARTESIAN_POINT('Ctrl Pts',(5.10805534167227,4.44237052028335,68.9250265375796));
#200230=CARTESIAN_POINT('Ctrl Pts',(4.98218644340076,4.57931296628585,68.9337757353256));
#200231=CARTESIAN_POINT('Ctrl Pts',(4.85632073219728,4.71625194483214,68.9425247115372));
#200232=CARTESIAN_POINT('Ctrl Pts',(4.72480612170478,4.84799861524352,68.9512736877488));
#200233=CARTESIAN_POINT('Ctrl Pts',(4.58808925235489,4.97410554898321,68.9600226639604));
#200234=CARTESIAN_POINT('Ctrl Pts',(4.45136349474231,5.10022068121047,68.9687722089622));
#200235=CARTESIAN_POINT('Ctrl Pts',(4.30943501210268,5.22069514871679,68.9775217539639));
#200236=CARTESIAN_POINT('Ctrl Pts',(4.16278587431975,5.33511975166106,68.9862712989656));
#200237=CARTESIAN_POINT('Ctrl Pts',(4.01614535740648,5.44953762807695,68.9950203296193));
#200238=CARTESIAN_POINT('Ctrl Pts',(3.8647849665813,5.5579061753264,69.003769360273));
#200239=CARTESIAN_POINT('Ctrl Pts',(3.70921874747409,5.65985735539216,69.0125183909267));
#200240=CARTESIAN_POINT('Ctrl Pts',(3.55365041606115,5.76180991976914,69.0212675403763));
#200241=CARTESIAN_POINT('Ctrl Pts',(3.39387638174737,5.85734478552689,69.030016689826));
#200242=CARTESIAN_POINT('Ctrl Pts',(3.23043927904753,5.94613749121116,69.0387658392756));
#200243=CARTESIAN_POINT('Ctrl Pts',(3.18691767070571,5.96978206944073,69.0410956471918));
#200244=CARTESIAN_POINT('Ctrl Pts',(3.14313645919698,5.99294880633391,69.043425455108));
#200245=CARTESIAN_POINT('Ctrl Pts',(3.09910619832131,6.01563211736941,69.0457552630242));
#200246=CARTESIAN_POINT('Ctrl Pts',(3.09910619832127,6.01563211736944,67.045599963736));
#200247=CARTESIAN_POINT('Ctrl Pts',(2.93588559344356,6.09971937177612,67.0542442724815));
#200248=CARTESIAN_POINT('Ctrl Pts',(2.76932797444242,6.17711490518632,67.062888581227));
#200249=CARTESIAN_POINT('Ctrl Pts',(2.60000172269813,6.2475819355945,67.0715328899725));
#200250=CARTESIAN_POINT('Ctrl Pts',(2.4304853058764,6.31812810534557,67.0801869068738));
#200251=CARTESIAN_POINT('Ctrl Pts',(2.25819432564532,6.38173011083379,67.0888409237752));
#200252=CARTESIAN_POINT('Ctrl Pts',(2.0837152003389,6.43820005621731,67.0974949406765));
#200253=CARTESIAN_POINT('Ctrl Pts',(2.02418527645254,6.45746683982048,67.1004475745033));
#200254=CARTESIAN_POINT('Ctrl Pts',(1.96440075258064,6.47590382425444,67.1034002083301));
#200255=CARTESIAN_POINT('Ctrl Pts',(1.90438525386509,6.49350489372736,67.1063528421569));
#200256=CARTESIAN_POINT('Ctrl Pts',(1.72054400935479,6.54742100849549,67.1153974371184));
#200257=CARTESIAN_POINT('Ctrl Pts',(1.53436482360287,6.59353950868748,67.12444203208));
#200258=CARTESIAN_POINT('Ctrl Pts',(1.34649615449113,6.63168433400902,67.1334866270416));
#200259=CARTESIAN_POINT('Ctrl Pts',(1.15879988446168,6.66979415544773,67.1425229221633));
#200260=CARTESIAN_POINT('Ctrl Pts',(0.96941745932348,6.69994486335135,67.151559217285));
#200261=CARTESIAN_POINT('Ctrl Pts',(0.779008793363627,6.72201117968887,
67.1605955124067));
#200262=CARTESIAN_POINT('Ctrl Pts',(0.58893707052117,6.74403844794327,67.1696158170932));
#200263=CARTESIAN_POINT('Ctrl Pts',(0.397842969209742,6.75800986447361,
67.1786361217796));
#200264=CARTESIAN_POINT('Ctrl Pts',(0.206392640552195,6.76385179301897,
67.1876564264661));
#200265=CARTESIAN_POINT('Ctrl Pts',(0.0151834064377996,6.76968636478879,
67.1966653718289));
#200266=CARTESIAN_POINT('Ctrl Pts',(-0.176380922700902,6.76741187189506,
67.2056743171917));
#200267=CARTESIAN_POINT('Ctrl Pts',(-0.367630502967207,6.75700649794627,
67.2146832625546));
#200268=CARTESIAN_POINT('Ctrl Pts',(-0.558445795822093,6.74662475240445,
67.2236717505048));
#200269=CARTESIAN_POINT('Ctrl Pts',(-0.748947529360054,6.72814899347496,
67.2326602384551));
#200270=CARTESIAN_POINT('Ctrl Pts',(-0.938467778612769,6.70160930139214,
67.2416487264054));
#200271=CARTESIAN_POINT('Ctrl Pts',(-1.10474570174047,6.67832437591647,
67.2495348869309));
#200272=CARTESIAN_POINT('Ctrl Pts',(-1.27026797150988,6.64883287419998,
67.2574210474564));
#200273=CARTESIAN_POINT('Ctrl Pts',(-1.43458401800579,6.61318816421266,
67.2653072079818));
#200274=CARTESIAN_POINT('Ctrl Pts',(-1.60380286441234,6.57647990088002,
67.2734286727758));
#200275=CARTESIAN_POINT('Ctrl Pts',(-1.7716663356137,6.53326059095723,67.2815501375697));
#200276=CARTESIAN_POINT('Ctrl Pts',(-1.93763730760377,6.4836602829098,67.2896716023637));
#200277=CARTESIAN_POINT('Ctrl Pts',(-2.10359644341587,6.43406351209582,
67.2977924879774));
#200278=CARTESIAN_POINT('Ctrl Pts',(-2.26766299798987,6.37808675442341,
67.3059133735911));
#200279=CARTESIAN_POINT('Ctrl Pts',(-2.42931442370919,6.31591010312516,
67.3140342592048));
#200280=CARTESIAN_POINT('Ctrl Pts',(-2.59098517139225,6.2537260199407,67.3221561154964));
#200281=CARTESIAN_POINT('Ctrl Pts',(-2.75023987405961,6.18534070007898,
67.330277971788));
#200282=CARTESIAN_POINT('Ctrl Pts',(-2.90657544825129,6.11098258577316,
67.3383998280796));
#200283=CARTESIAN_POINT('Ctrl Pts',(-3.06302508294209,6.03657022070787,
67.3465276099769));
#200284=CARTESIAN_POINT('Ctrl Pts',(-3.21655100441934,5.9561765151777,67.3546553918742));
#200285=CARTESIAN_POINT('Ctrl Pts',(-3.36667368540554,5.87007643016664,
67.3627831737716));
#200286=CARTESIAN_POINT('Ctrl Pts',(-3.5168575207906,5.78394127118204,67.3709142666251));
#200287=CARTESIAN_POINT('Ctrl Pts',(-3.66363504208972,5.6920952933114,67.3790453594787));
#200288=CARTESIAN_POINT('Ctrl Pts',(-3.80655549026008,5.59485695076924,
67.3871764523322));
#200289=CARTESIAN_POINT('Ctrl Pts',(-3.94963193013018,5.4975124766376,67.3953164199339));
#200290=CARTESIAN_POINT('Ctrl Pts',(-4.08884259415968,5.39476409964222,
67.4034563875357));
#200291=CARTESIAN_POINT('Ctrl Pts',(-4.2237690128558,5.28697118642037,67.4115963551374));
#200292=CARTESIAN_POINT('Ctrl Pts',(-4.29374769420603,5.23106511554811,
67.4158180946938));
#200293=CARTESIAN_POINT('Ctrl Pts',(-4.36257453206647,5.1738027417705,67.4200398342501));
#200294=CARTESIAN_POINT('Ctrl Pts',(-4.43019507901427,5.11523807479943,
67.4242615738065));
#200295=CARTESIAN_POINT('Ctrl Pts',(-4.56329035016489,4.99996719069407,
67.4325710832136));
#200296=CARTESIAN_POINT('Ctrl Pts',(-4.69201063712768,4.87938866675348,
67.4408805926207));
#200297=CARTESIAN_POINT('Ctrl Pts',(-4.81591620892539,4.7538658025453,67.4491901020279));
#200298=CARTESIAN_POINT('Ctrl Pts',(-4.93971855124055,4.62844751523495,
67.4574926885312));
#200299=CARTESIAN_POINT('Ctrl Pts',(-5.05871392679581,4.49809334240074,
67.4657952750345));
#200300=CARTESIAN_POINT('Ctrl Pts',(-5.17249707351925,4.36320559043862,
67.4740978615378));
#200301=CARTESIAN_POINT('Ctrl Pts',(-5.28620647825334,4.2284052581995,67.4823950671982));
#200302=CARTESIAN_POINT('Ctrl Pts',(-5.394710161456,4.08907746784305,67.4906922728585));
#200303=CARTESIAN_POINT('Ctrl Pts',(-5.49764087114487,3.94566012878929,
67.4989894785188));
#200304=CARTESIAN_POINT('Ctrl Pts',(-5.60052808452494,3.80230339482496,
67.5072831779581));
#200305=CARTESIAN_POINT('Ctrl Pts',(-5.69784681356272,3.65486083838874,
67.5155768773975));
#200306=CARTESIAN_POINT('Ctrl Pts',(-5.78927097556485,3.50380230199743,
67.5238705768368));
#200307=CARTESIAN_POINT('Ctrl Pts',(-5.88067469871569,3.35277753636094,
67.5321624221307));
#200308=CARTESIAN_POINT('Ctrl Pts',(-5.96618629940749,3.19813869939004,
67.5404542674246));
#200309=CARTESIAN_POINT('Ctrl Pts',(-6.045523690687,3.0403835786529,67.5487461127185));
#200310=CARTESIAN_POINT('Ctrl Pts',(-6.12485665051338,2.88263726945358,
67.5570374948648));
#200311=CARTESIAN_POINT('Ctrl Pts',(-6.19801593138472,2.72177533498301,
67.5653288770111));
#200312=CARTESIAN_POINT('Ctrl Pts',(-6.26476589907955,2.55831921966943,
67.5736202591574));
#200313=CARTESIAN_POINT('Ctrl Pts',(-6.33152333219865,2.39484482315973,
67.5819125686252));
#200314=CARTESIAN_POINT('Ctrl Pts',(-6.39186989237051,2.22877599084022,
67.5902048780931));
#200315=CARTESIAN_POINT('Ctrl Pts',(-6.44561842696355,2.06065331727293,
67.598497187561));
#200316=CARTESIAN_POINT('Ctrl Pts',(-6.49940622500276,1.89240782964956,
67.6067955545828));
#200317=CARTESIAN_POINT('Ctrl Pts',(-6.5465862588529,1.72210583522364,67.6150939216046));
#200318=CARTESIAN_POINT('Ctrl Pts',(-6.58702126478448,1.55030315012163,
67.6233922886263));
#200319=CARTESIAN_POINT('Ctrl Pts',(-6.62747075214523,1.37843893545242,
67.6316936276327));
#200320=CARTESIAN_POINT('Ctrl Pts',(-6.66117032425106,1.20507330023746,
67.6399949666391));
#200321=CARTESIAN_POINT('Ctrl Pts',(-6.6880340124061,1.03077157940018,67.6482963056455));
#200322=CARTESIAN_POINT('Ctrl Pts',(-6.71492875010227,0.856268397452345,
67.656607239491));
#200323=CARTESIAN_POINT('Ctrl Pts',(-6.73497176834432,0.680827314055356,
67.6649181733365));
#200324=CARTESIAN_POINT('Ctrl Pts',(-6.748128959665,0.505019349857625,67.673229107182));
#200325=CARTESIAN_POINT('Ctrl Pts',(-6.76071469570443,0.336847239481363,
67.6811790728754));
#200326=CARTESIAN_POINT('Ctrl Pts',(-6.76700011610791,0.168339715120327,
67.6891290385688));
#200327=CARTESIAN_POINT('Ctrl Pts',(-6.76699999999839,-4.66729631973905E-6,
67.6970790042622));
#200328=CARTESIAN_POINT('',(-6.76699969105987,0.00204479721649499,67.3028202162187));
#200329=CARTESIAN_POINT('Ctrl Pts',(3.09910619832135,6.0156321173694,66.651425676538));
#200330=CARTESIAN_POINT('Ctrl Pts',(2.9437528555786,6.09566635118397,66.6596230179432));
#200331=CARTESIAN_POINT('Ctrl Pts',(2.78530404469065,6.16967521411631,66.6678203593483));
#200332=CARTESIAN_POINT('Ctrl Pts',(2.62427106360847,6.23742658351241,66.6760177007535));
#200333=CARTESIAN_POINT('Ctrl Pts',(2.46320047430483,6.30519377580694,66.6842169565952));
#200334=CARTESIAN_POINT('Ctrl Pts',(2.29954484324433,6.36670042414967,66.692416212437));
#200335=CARTESIAN_POINT('Ctrl Pts',(2.13383456016875,6.42176292538345,66.7006154682787));
#200336=CARTESIAN_POINT('Ctrl Pts',(1.96805544484949,6.47684829831496,66.7088181299029));
#200337=CARTESIAN_POINT('Ctrl Pts',(1.80022031761879,6.52548407900047,66.7170207915271));
#200338=CARTESIAN_POINT('Ctrl Pts',(1.63087384812159,6.56753679026719,66.7252234531513));
#200339=CARTESIAN_POINT('Ctrl Pts',(1.46133097115867,6.609638274127,66.7334356281949));
#200340=CARTESIAN_POINT('Ctrl Pts',(1.29027359919294,6.645141352039,66.7416478032385));
#200341=CARTESIAN_POINT('Ctrl Pts',(1.11825667107228,6.67396366618836,66.749859978282));
#200342=CARTESIAN_POINT('Ctrl Pts',(0.946128679145179,6.70280458964527,
66.7580774555678));
#200343=CARTESIAN_POINT('Ctrl Pts',(0.773040251134529,6.72495610647834,
66.7662949328536));
#200344=CARTESIAN_POINT('Ctrl Pts',(0.599550408877115,6.74038784545929,
66.7745124101394));
#200345=CARTESIAN_POINT('Ctrl Pts',(0.425808467513748,6.75584200839053,
66.7827418282896));
#200346=CARTESIAN_POINT('Ctrl Pts',(0.251664304072191,6.76455687037831,
66.7909712464398));
#200347=CARTESIAN_POINT('Ctrl Pts',(0.0776769903517417,6.76655416627769,
66.7992006645899));
#200348=CARTESIAN_POINT('Ctrl Pts',(-0.0203850106945762,6.7676798738272,
66.8038388947804));
#200349=CARTESIAN_POINT('Ctrl Pts',(-0.118397260002335,6.76667260349463,
66.8084771249708));
#200350=CARTESIAN_POINT('Ctrl Pts',(-0.216260647502554,6.76354347456581,
66.8131153551613));
#200351=CARTESIAN_POINT('Ctrl Pts',(-0.386517383979043,6.75809960742568,
66.8211846643833));
#200352=CARTESIAN_POINT('Ctrl Pts',(-0.55688051997641,6.7462127497999,66.8292539736053));
#200353=CARTESIAN_POINT('Ctrl Pts',(-0.726811026680727,6.72785513603669,
66.8373232828273));
#200354=CARTESIAN_POINT('Ctrl Pts',(-0.896529583857726,6.70952041920727,
66.8453825274275));
#200355=CARTESIAN_POINT('Ctrl Pts',(-1.06581621913016,6.68473104453334,
66.8534417720278));
#200356=CARTESIAN_POINT('Ctrl Pts',(-1.23413042271984,6.6535111858114,66.861501016628));
#200357=CARTESIAN_POINT('Ctrl Pts',(-1.40227162902586,6.62232341559203,
66.8695519777477));
#200358=CARTESIAN_POINT('Ctrl Pts',(-1.56944202887194,6.5847183816347,66.8776029388675));
#200359=CARTESIAN_POINT('Ctrl Pts',(-1.7351048634845,6.5407721342906,66.8856538999872));
#200360=CARTESIAN_POINT('Ctrl Pts',(-1.90063372596885,6.49686142643427,
66.8936983502658));
#200361=CARTESIAN_POINT('Ctrl Pts',(-2.06465709094783,6.44661980711828,
66.9017428005445));
#200362=CARTESIAN_POINT('Ctrl Pts',(-2.2266471514926,6.3901746034635,66.9097872508231));
#200363=CARTESIAN_POINT('Ctrl Pts',(-2.38854166820264,6.33376269192054,
66.9178269563808));
#200364=CARTESIAN_POINT('Ctrl Pts',(-2.54840491639844,6.27115460239405,
66.9258666619385));
#200365=CARTESIAN_POINT('Ctrl Pts',(-2.70572315484147,6.20252780802752,
66.9339063674962));
#200366=CARTESIAN_POINT('Ctrl Pts',(-2.86643702337129,6.1324197409871,66.942119605801));
#200367=CARTESIAN_POINT('Ctrl Pts',(-3.02449438234326,6.05603029676614,
66.9503328441057));
#200368=CARTESIAN_POINT('Ctrl Pts',(-3.17936746390975,5.97360121948495,
66.9585460824105));
#200369=CARTESIAN_POINT('Ctrl Pts',(-3.33091952112869,5.89293971194427,
66.9665831999582));
#200370=CARTESIAN_POINT('Ctrl Pts',(-3.47942214373032,5.80649516123075,
66.9746203175059));
#200371=CARTESIAN_POINT('Ctrl Pts',(-3.62440473451101,5.71454104197828,
66.9826574350535));
#200372=CARTESIAN_POINT('Ctrl Pts',(-3.7694026635282,5.62257719456451,66.9906954028771));
#200373=CARTESIAN_POINT('Ctrl Pts',(-3.91087950363473,5.52510281804308,
66.9987333707007));
#200374=CARTESIAN_POINT('Ctrl Pts',(-4.04839307754145,5.42243510700815,
67.0067713385243));
#200375=CARTESIAN_POINT('Ctrl Pts',(-4.18594844601779,5.31973619212421,
67.0148117493315));
#200376=CARTESIAN_POINT('Ctrl Pts',(-4.31953785142545,5.21184102430835,
67.0228521601387));
#200377=CARTESIAN_POINT('Ctrl Pts',(-4.44875180267221,5.09910741191248,
67.030892570946));
#200378=CARTESIAN_POINT('Ctrl Pts',(-4.58284931252452,4.98211310477244,
67.0392368639347));
#200379=CARTESIAN_POINT('Ctrl Pts',(-4.71223383576047,4.85990776844361,
67.0475811569234));
#200380=CARTESIAN_POINT('Ctrl Pts',(-4.83649003847436,4.73293282307475,
67.0559254499121));
#200381=CARTESIAN_POINT('Ctrl Pts',(-4.95643252863061,4.61036597488237,
67.0639800601272));
#200382=CARTESIAN_POINT('Ctrl Pts',(-5.07159660629193,4.4833554512275,67.0720346703422));
#200383=CARTESIAN_POINT('Ctrl Pts',(-5.18165055964601,4.3523311544183,67.0800892805573));
#200384=CARTESIAN_POINT('Ctrl Pts',(-5.29178782539577,4.22120767036752,
67.088149988226));
#200385=CARTESIAN_POINT('Ctrl Pts',(-5.39680703669563,4.08606465611705,
67.0962106958946));
#200386=CARTESIAN_POINT('Ctrl Pts',(-5.49642004171115,3.94736060236154,
67.1042714035632));
#200387=CARTESIAN_POINT('Ctrl Pts',(-5.59617349509784,3.80846098419732,
67.1123434763469));
#200388=CARTESIAN_POINT('Ctrl Pts',(-5.69050532990209,3.66599061758706,
67.1204155491306));
#200389=CARTESIAN_POINT('Ctrl Pts',(-5.77917321239657,3.52043264118459,
67.1284876219143));
#200390=CARTESIAN_POINT('Ctrl Pts',(-5.78846049945894,3.50518654899161,
67.1293331102131));
#200391=CARTESIAN_POINT('Ctrl Pts',(-5.79768569113277,3.489906600452,67.130178598512));
#200392=CARTESIAN_POINT('Ctrl Pts',(-5.8068485397515,3.47459336273842,67.1310240868108));
#200393=CARTESIAN_POINT('Ctrl Pts',(-5.90234831954787,3.3149911592679,67.1398361876887));
#200394=CARTESIAN_POINT('Ctrl Pts',(-5.99134678333706,3.15131174780054,
67.1486482885667));
#200395=CARTESIAN_POINT('Ctrl Pts',(-6.07350709161056,2.98409125332256,
67.1574603894447));
#200396=CARTESIAN_POINT('Ctrl Pts',(-6.15553653987655,2.81713709761112,
67.1662584549374));
#200397=CARTESIAN_POINT('Ctrl Pts',(-6.23074943337021,2.64665335945228,
67.17505652043));
#200398=CARTESIAN_POINT('Ctrl Pts',(-6.29885384418314,2.47320222578328,
67.1838545859227));
#200399=CARTESIAN_POINT('Ctrl Pts',(-6.36684939253087,2.30002834754862,
67.1926385880222));
#200400=CARTESIAN_POINT('Ctrl Pts',(-6.42775901957409,2.12389679511523,
67.2014225901218));
#200401=CARTESIAN_POINT('Ctrl Pts',(-6.48133772067748,1.94539208143841,
67.2102065922214));
#200402=CARTESIAN_POINT('Ctrl Pts',(-6.53479274991776,1.76729939735657,
67.2189703188405));
#200403=CARTESIAN_POINT('Ctrl Pts',(-6.58095053711646,1.58684475049073,
67.2277340454596));
#200404=CARTESIAN_POINT('Ctrl Pts',(-6.61961510243933,1.40462980730055,
67.2364977720788));
#200405=CARTESIAN_POINT('Ctrl Pts',(-6.65822430976861,1.22267575036558,
67.2452489512319));
#200406=CARTESIAN_POINT('Ctrl Pts',(-6.68936163055062,1.03896669613739,
67.2540001303849));
#200407=CARTESIAN_POINT('Ctrl Pts',(-6.71288087981851,0.854119015926434,
67.262751309538));
#200408=CARTESIAN_POINT('Ctrl Pts',(-6.73635188671799,0.669650492795929,
67.2714845383899));
#200409=CARTESIAN_POINT('Ctrl Pts',(-6.75223596278394,0.484048281077616,
67.2802177672417));
#200410=CARTESIAN_POINT('Ctrl Pts',(-6.76043799091104,0.297938200046067,
67.2889509960935));
#200411=CARTESIAN_POINT('Ctrl Pts',(-6.76477986473802,0.199417873457771,
67.2935740694589));
#200412=CARTESIAN_POINT('Ctrl Pts',(-6.76696986347182,0.100755425632308,
67.2981971428244));
#200413=CARTESIAN_POINT('Ctrl Pts',(-6.76699969105968,0.00204479783337229,
67.3028202161898));
#200414=CARTESIAN_POINT('Ctrl Pts',(-6.76699969105987,0.00204479721659033,
67.3028202162187));
#200415=CARTESIAN_POINT('Ctrl Pts',(-6.76705546570766,-0.182534397879825,
67.3114649101052));
#200416=CARTESIAN_POINT('Ctrl Pts',(-6.75955491081402,-0.367004244749094,
67.3201096039916));
#200417=CARTESIAN_POINT('Ctrl Pts',(-6.74455107192691,-0.550744803125321,
67.3287542978781));
#200418=CARTESIAN_POINT('Ctrl Pts',(-6.72953240757911,-0.734666917598438,
67.3374075336831));
#200419=CARTESIAN_POINT('Ctrl Pts',(-6.70699568187137,-0.917858008923771,
67.3460607694881));
#200420=CARTESIAN_POINT('Ctrl Pts',(-6.67704556877224,-1.09970517528065,
67.3547140052931));
#200421=CARTESIAN_POINT('Ctrl Pts',(-6.64704417399101,-1.28186370702515,
67.3633820574858));
#200422=CARTESIAN_POINT('Ctrl Pts',(-6.60960406084239,-1.46267341902971,
67.3720501096786));
#200423=CARTESIAN_POINT('Ctrl Pts',(-6.56488105234982,-1.64153153137497,
67.3807181618713));
#200424=CARTESIAN_POINT('Ctrl Pts',(-6.52011863950898,-1.82054723122584,
67.3893938512726));
#200425=CARTESIAN_POINT('Ctrl Pts',(-6.46806060170046,-1.99760761274257,
67.398069540674));
#200426=CARTESIAN_POINT('Ctrl Pts',(-6.40891241259666,-2.17212584526415,
67.4067452300754));
#200427=CARTESIAN_POINT('Ctrl Pts',(-6.34967138021081,-2.34691801424483,
67.4154345374672));
#200428=CARTESIAN_POINT('Ctrl Pts',(-6.28331804893838,-2.51915977717957,
67.4241238448591));
#200429=CARTESIAN_POINT('Ctrl Pts',(-6.21010645343616,-2.68828325088532,
67.432813152251));
#200430=CARTESIAN_POINT('Ctrl Pts',(-6.16483447225615,-2.79286442639696,
67.4381863743207));
#200431=CARTESIAN_POINT('Ctrl Pts',(-6.11694093386495,-2.89625366352979,
67.4435595963905));
#200432=CARTESIAN_POINT('Ctrl Pts',(-6.06649463752745,-2.99832149924766,
67.4489328184602));
#200433=CARTESIAN_POINT('Ctrl Pts',(-5.98715960250811,-3.15883983079871,
67.4573830872018));
#200434=CARTESIAN_POINT('Ctrl Pts',(-5.90138241536787,-3.31634371716938,
67.4658333559433));
#200435=CARTESIAN_POINT('Ctrl Pts',(-5.80941452677204,-3.47030140710141,
67.4742836246849));
#200436=CARTESIAN_POINT('Ctrl Pts',(-5.71752780295919,-3.62412322414689,
67.4827264357775));
#200437=CARTESIAN_POINT('Ctrl Pts',(-5.619461436692,-3.77440479935361,67.4911692468701));
#200438=CARTESIAN_POINT('Ctrl Pts',(-5.51551317961652,-3.92063813243157,
67.4996120579627));
#200439=CARTESIAN_POINT('Ctrl Pts',(-5.41164250758393,-4.06676231967352,
67.5080485674984));
#200440=CARTESIAN_POINT('Ctrl Pts',(-5.30189888770947,-4.2088440186668,
67.516485077034));
#200441=CARTESIAN_POINT('Ctrl Pts',(-5.18662405337289,-4.34640310244849,
67.5249215865697));
#200442=CARTESIAN_POINT('Ctrl Pts',(-5.07143170438705,-4.48386375529909,
67.5333520593285));
#200443=CARTESIAN_POINT('Ctrl Pts',(-4.95071624802827,-4.61680799448141,
67.5417825320874));
#200444=CARTESIAN_POINT('Ctrl Pts',(-4.82486058506799,-4.74478759636903,
67.5502130048462));
#200445=CARTESIAN_POINT('Ctrl Pts',(-4.69905902711864,-4.87271218017009,
67.5586398533675));
#200446=CARTESIAN_POINT('Ctrl Pts',(-4.56812189987031,-4.99567614546197,
67.5670667018888));
#200447=CARTESIAN_POINT('Ctrl Pts',(-4.43247039600956,-5.11326658687955,
67.5754935504101));
#200448=CARTESIAN_POINT('Ctrl Pts',(-4.29686076293026,-5.23082073232155,
67.5839177978637));
#200449=CARTESIAN_POINT('Ctrl Pts',(-4.1565399054294,-5.3430044446237,67.5923420453174));
#200450=CARTESIAN_POINT('Ctrl Pts',(-4.0119639385121,-5.44944349049318,
67.6007662927711));
#200451=CARTESIAN_POINT('Ctrl Pts',(-3.97122796450357,-5.47943393979456,
67.6031399232758));
#200452=CARTESIAN_POINT('Ctrl Pts',(-3.93015438138309,-5.50896856644706,
67.6055135537804));
#200453=CARTESIAN_POINT('Ctrl Pts',(-3.88875385622549,-5.53803958505999,
67.607887184285));
#200454=CARTESIAN_POINT('Ctrl Pts',(-3.73842630763758,-5.64359802777051,
67.6165059651739));
#200455=CARTESIAN_POINT('Ctrl Pts',(-3.58385315610053,-5.74299352130163,
67.6251247460627));
#200456=CARTESIAN_POINT('Ctrl Pts',(-3.42556206974887,-5.83590725648531,
67.6337435269516));
#200457=CARTESIAN_POINT('Ctrl Pts',(-3.2671758989147,-5.92887680437854,
67.6423674850892));
#200458=CARTESIAN_POINT('Ctrl Pts',(-3.10506759851736,-6.01535666959871,
67.6509914432267));
#200459=CARTESIAN_POINT('Ctrl Pts',(-2.93978960781891,-6.0950739176617,
67.6596154013643));
#200460=CARTESIAN_POINT('Ctrl Pts',(-2.76854068580091,-6.17767107859849,
67.6685509137598));
#200461=CARTESIAN_POINT('Ctrl Pts',(-2.593889111302,-6.25300774026649,67.6774864261553));
#200462=CARTESIAN_POINT('Ctrl Pts',(-2.41647154396405,-6.32083493513413,
67.6864219385507));
#200463=CARTESIAN_POINT('Ctrl Pts',(-2.24491984835737,-6.38641959206735,
67.6950620203958));
#200464=CARTESIAN_POINT('Ctrl Pts',(-2.07078243740811,-6.44498334513258,
67.7037021022409));
#200465=CARTESIAN_POINT('Ctrl Pts',(-1.89465042004698,-6.49635195981682,
67.712342184086));
#200466=CARTESIAN_POINT('Ctrl Pts',(-1.70948467249197,-6.55035524713152,
67.7214254117567));
#200467=CARTESIAN_POINT('Ctrl Pts',(-1.52211472135507,-6.59640584482545,
67.7305086394273));
#200468=CARTESIAN_POINT('Ctrl Pts',(-1.33324010415943,-6.63436205106874,
67.739591867098));
#200469=CARTESIAN_POINT('Ctrl Pts',(-1.14436548696386,-6.67231825731201,
67.7486750947686));
#200470=CARTESIAN_POINT('Ctrl Pts',(-0.95398659201651,-6.70218004526323,
67.7577583224393));
#200471=CARTESIAN_POINT('Ctrl Pts',(-0.762810281316113,-6.72386863901418,
67.76684155011));
#200472=CARTESIAN_POINT('Ctrl Pts',(-0.572447080124421,-6.74546498701698,
67.7758861450716));
#200473=CARTESIAN_POINT('Ctrl Pts',(-0.38111753514558,-6.75897833174049,
67.7849307400332));
#200474=CARTESIAN_POINT('Ctrl Pts',(-0.189490688569759,-6.76434640441672,
67.7939753349948));
#200475=CARTESIAN_POINT('Ctrl Pts',(0.00196031020367951,-6.76970955104109,
67.8030116301165));
#200476=CARTESIAN_POINT('Ctrl Pts',(0.193707828290141,-6.76694234197754,
67.8120479252382));
#200477=CARTESIAN_POINT('Ctrl Pts',(0.385080243852762,-6.75603450300502,
67.8210842203599));
#200478=CARTESIAN_POINT('Ctrl Pts',(0.576114010867229,-6.74514596631189,
67.8301045250464));
#200479=CARTESIAN_POINT('Ctrl Pts',(0.766773763629801,-6.72614557914719,
67.8391248297328));
#200480=CARTESIAN_POINT('Ctrl Pts',(0.956390590301346,-6.6990750136704,
67.8481451344192));
#200481=CARTESIAN_POINT('Ctrl Pts',(1.14576863137019,-6.67203853831845,
67.8571540797821));
#200482=CARTESIAN_POINT('Ctrl Pts',(1.3341061325675,-6.63695219967758,67.866163025145));
#200483=CARTESIAN_POINT('Ctrl Pts',(1.520739428976,-6.59390935554605,67.8751719705078));
#200484=CARTESIAN_POINT('Ctrl Pts',(1.70694892057874,-6.55096425262442,
67.8841604584582));
#200485=CARTESIAN_POINT('Ctrl Pts',(1.89146170064486,-6.50009876195173,
67.8931489464085));
#200486=CARTESIAN_POINT('Ctrl Pts',(2.07362489293906,-6.44145704040503,
67.9021374343588));
#200487=CARTESIAN_POINT('Ctrl Pts',(2.23344801159656,-6.39000700429728,
67.9100235948841));
#200488=CARTESIAN_POINT('Ctrl Pts',(2.39146249064502,-6.33257186807405,
67.9179097554094));
#200489=CARTESIAN_POINT('Ctrl Pts',(2.54723358303126,-6.26928146389024,
67.9257959159347));
#200490=CARTESIAN_POINT('Ctrl Pts',(2.70765251422937,-6.20410262461569,
67.9339173807286));
#200491=CARTESIAN_POINT('Ctrl Pts',(2.86561976081255,-6.13274155174847,
67.9420388455225));
#200492=CARTESIAN_POINT('Ctrl Pts',(3.02062845100306,-6.05541846291327,
67.9501603103164));
#200493=CARTESIAN_POINT('Ctrl Pts',(3.17562608678761,-5.9781008883548,67.9582811959301));
#200494=CARTESIAN_POINT('Ctrl Pts',(3.32766525875864,-5.8948223081832,67.9664020815438));
#200495=CARTESIAN_POINT('Ctrl Pts',(3.47626203632042,-5.80584974442479,
67.9745229671575));
#200496=CARTESIAN_POINT('Ctrl Pts',(3.62487657544279,-5.71686654590291,
67.9826448234491));
#200497=CARTESIAN_POINT('Ctrl Pts',(3.77004758728321,-5.62218819771634,
67.9907666797406));
#200498=CARTESIAN_POINT('Ctrl Pts',(3.91131860705761,-5.52212601758462,
67.9988885360322));
#200499=CARTESIAN_POINT('Ctrl Pts',(4.05269269641907,-5.42199083332506,
68.0070163179295));
#200500=CARTESIAN_POINT('Ctrl Pts',(4.19016081157461,-5.31646418375312,
68.0151440998269));
#200501=CARTESIAN_POINT('Ctrl Pts',(4.32329767116583,-5.20589917751892,
68.0232718817242));
#200502=CARTESIAN_POINT('Ctrl Pts',(4.45648876576363,-5.09528913121197,
68.0314029745777));
#200503=CARTESIAN_POINT('Ctrl Pts',(4.5853448155403,-4.97963688157713,68.0395340674312));
#200504=CARTESIAN_POINT('Ctrl Pts',(4.70947633867659,-4.8593334538232,68.0476651602847));
#200505=CARTESIAN_POINT('Ctrl Pts',(4.83374334618531,-4.73889871990306,
68.0558051278864));
#200506=CARTESIAN_POINT('Ctrl Pts',(4.95327527488596,-4.61380293270163,
68.0639450954882));
#200507=CARTESIAN_POINT('Ctrl Pts',(5.06772146916316,-4.48447188763435,
68.0720850630899));
#200508=CARTESIAN_POINT('Ctrl Pts',(5.12707821959638,-4.41739520925453,
68.0763068026464));
#200509=CARTESIAN_POINT('Ctrl Pts',(5.18506763295147,-4.34917980776911,
68.0805285422028));
#200510=CARTESIAN_POINT('Ctrl Pts',(5.24164532858782,-4.2798882285982,68.0847502817593));
#200511=CARTESIAN_POINT('Ctrl Pts',(5.3547569012016,-4.1413587356459,68.0931904911922));
#200512=CARTESIAN_POINT('Ctrl Pts',(5.46245722300636,-3.99823976917441,
68.1016307006251));
#200513=CARTESIAN_POINT('Ctrl Pts',(5.56437095760982,-3.85098232222746,
68.1100709100579));
#200514=CARTESIAN_POINT('Ctrl Pts',(5.66620747745769,-3.70383644461725,
68.1185047247815));
#200515=CARTESIAN_POINT('Ctrl Pts',(5.76226596060923,-3.55255861019642,
68.1269385395051));
#200516=CARTESIAN_POINT('Ctrl Pts',(5.85221222128754,-3.39763169237231,
68.1353723542286));
#200517=CARTESIAN_POINT('Ctrl Pts',(5.94210416150533,-3.24279833821013,
68.143801075592));
#200518=CARTESIAN_POINT('Ctrl Pts',(6.02589107136909,-3.08432058183424,
68.1522297969554));
#200519=CARTESIAN_POINT('Ctrl Pts',(6.10328265729014,-2.92270932615979,
68.1606585183188));
#200520=CARTESIAN_POINT('Ctrl Pts',(6.18063938888008,-2.76117085426601,
68.1690834436953));
#200521=CARTESIAN_POINT('Ctrl Pts',(6.25160639556577,-2.59650199714855,
68.1775083690719));
#200522=CARTESIAN_POINT('Ctrl Pts',(6.31593965149612,-2.42923760028925,
68.1859332944484));
#200523=CARTESIAN_POINT('Ctrl Pts',(6.38025380471629,-2.26202286986219,
68.1943557181808));
#200524=CARTESIAN_POINT('Ctrl Pts',(6.43793801577486,-2.09221444756755,
68.2027781419133));
#200525=CARTESIAN_POINT('Ctrl Pts',(6.48879651596112,-1.92036683330318,
68.2112005656458));
#200526=CARTESIAN_POINT('Ctrl Pts',(6.53965581600562,-1.74851651636901,
68.2196231218388));
#200527=CARTESIAN_POINT('Ctrl Pts',(6.5836890897008,-1.57462726119323,68.2280456780318));
#200528=CARTESIAN_POINT('Ctrl Pts',(6.6207503461659,-1.39926904265911,68.2364682342248));
#200529=CARTESIAN_POINT('Ctrl Pts',(6.65781285456765,-1.22390490048931,
68.2448910749334));
#200530=CARTESIAN_POINT('Ctrl Pts',(6.68790280699985,-1.04707202235281,
68.2533139156421));
#200531=CARTESIAN_POINT('Ctrl Pts',(6.71092525262042,-0.869351053223966,
68.2617367563508));
#200532=CARTESIAN_POINT('Ctrl Pts',(6.73395169013205,-0.691599268830729,
68.2701610575064));
#200533=CARTESIAN_POINT('Ctrl Pts',(6.74990813480536,-0.512959417234193,
68.2785853586621));
#200534=CARTESIAN_POINT('Ctrl Pts',(6.75875143026366,-0.334018119132661,
68.2870096598178));
#200535=CARTESIAN_POINT('Ctrl Pts',(6.76759749407248,-0.155020804330292,
68.2954365981599));
#200536=CARTESIAN_POINT('Ctrl Pts',(6.76932595269978,0.0242778120923452,
68.303863536502));
#200537=CARTESIAN_POINT('Ctrl Pts',(6.76394575863086,0.20328987751389,68.312290474844));
#200538=CARTESIAN_POINT('Ctrl Pts',(6.75856072709091,0.382462897293245,
68.3207249900634));
#200539=CARTESIAN_POINT('Ctrl Pts',(6.74605428151076,0.56134851752219,68.3291595052828));
#200540=CARTESIAN_POINT('Ctrl Pts',(6.72648744801321,0.739361624457722,
68.3375940205021));
#200541=CARTESIAN_POINT('Ctrl Pts',(6.70691116356695,0.917460713253555,
68.3460326096648));
#200542=CARTESIAN_POINT('Ctrl Pts',(6.68026773438625,1.09468611783465,68.3544711988275));
#200543=CARTESIAN_POINT('Ctrl Pts',(6.64666964879937,1.27046116813119,68.3629097879902));
#200544=CARTESIAN_POINT('Ctrl Pts',(6.61303400815141,1.44643269518036,68.371357809587));
#200545=CARTESIAN_POINT('Ctrl Pts',(6.57242824847864,1.62095030252979,68.3798058311839));
#200546=CARTESIAN_POINT('Ctrl Pts',(6.52501552695931,1.79344957357042,68.3882538527808));
#200547=CARTESIAN_POINT('Ctrl Pts',(6.49806689520091,1.89149539724183,68.3930555729901));
#200548=CARTESIAN_POINT('Ctrl Pts',(6.46892011363864,1.98888946191966,68.3978572931995));
#200549=CARTESIAN_POINT('Ctrl Pts',(6.43761216901738,2.08553076249653,68.4026590134089));
#200550=CARTESIAN_POINT('Ctrl Pts',(6.38388916882985,2.25136281157614,68.4108985455414));
#200551=CARTESIAN_POINT('Ctrl Pts',(6.32367992429258,2.4153474495578,68.4191380776738));
#200552=CARTESIAN_POINT('Ctrl Pts',(6.25712841355242,2.57694257140414,68.4273776098063));
#200553=CARTESIAN_POINT('Ctrl Pts',(6.19065077035214,2.73835833392454,68.4356079966323));
#200554=CARTESIAN_POINT('Ctrl Pts',(6.11784501206133,2.8973895350872,68.4438383834582));
#200555=CARTESIAN_POINT('Ctrl Pts',(6.03890501359738,3.05350867638336,68.4520687702841));
#200556=CARTESIAN_POINT('Ctrl Pts',(5.96003855086308,3.20948238652685,68.4602914901793));
#200557=CARTESIAN_POINT('Ctrl Pts',(5.87504938770952,3.36254912344422,68.4685142100745));
#200558=CARTESIAN_POINT('Ctrl Pts',(5.78417969659149,3.51220076839847,68.4767369299697));
#200559=CARTESIAN_POINT('Ctrl Pts',(5.69339052261084,3.66171981114062,68.4849523639386));
#200560=CARTESIAN_POINT('Ctrl Pts',(5.59673138984904,3.8078294900049,68.4931677979075));
#200561=CARTESIAN_POINT('Ctrl Pts',(5.49449058491127,3.95004584939484,68.5013832318765));
#200562=CARTESIAN_POINT('Ctrl Pts',(5.39230232383676,4.0921891205795,68.509594443748));
#200563=CARTESIAN_POINT('Ctrl Pts',(5.28453831079439,4.23044276891584,68.5178056556195));
#200564=CARTESIAN_POINT('Ctrl Pts',(5.1715305930025,4.36435107726672,68.526016867491));
#200565=CARTESIAN_POINT('Ctrl Pts',(5.05856077182384,4.49821448008843,68.5342253257708));
#200566=CARTESIAN_POINT('Ctrl Pts',(4.94035097817908,4.62773517407047,68.5424337840505));
#200567=CARTESIAN_POINT('Ctrl Pts',(4.81727410861847,4.75248978562123,68.5506422423303));
#200568=CARTESIAN_POINT('Ctrl Pts',(4.76244070224812,4.80807066232178,68.5542992879647));
#200569=CARTESIAN_POINT('Ctrl Pts',(4.70664175875749,4.8627059701033,68.5579563335992));
#200570=CARTESIAN_POINT('Ctrl Pts',(4.64991270549473,4.91636052698322,68.5616133792336));
#200571=CARTESIAN_POINT('Ctrl Pts',(4.51245672008586,5.04636692693925,68.5704744968172));
#200572=CARTESIAN_POINT('Ctrl Pts',(4.36968067268176,5.1704777176743,68.5793356144008));
#200573=CARTESIAN_POINT('Ctrl Pts',(4.22210643219175,5.28829899639242,68.5881967319845));
#200574=CARTESIAN_POINT('Ctrl Pts',(4.07429896157757,5.4063064828889,68.5970718539061));
#200575=CARTESIAN_POINT('Ctrl Pts',(3.92167835441354,5.51800444251662,68.6059469758278));
#200576=CARTESIAN_POINT('Ctrl Pts',(3.76479554898082,5.62304219034272,68.6148220977495));
#200577=CARTESIAN_POINT('Ctrl Pts',(3.60755963427478,5.72831635542757,68.6237171956516));
#200578=CARTESIAN_POINT('Ctrl Pts',(3.4460425524921,5.82690018600769,68.6326122935537));
#200579=CARTESIAN_POINT('Ctrl Pts',(3.28082209799587,5.91848759070271,68.6415073914558));
#200580=CARTESIAN_POINT('Ctrl Pts',(3.22073033337437,5.95179853142133,68.6447425969941));
#200581=CARTESIAN_POINT('Ctrl Pts',(3.16014888048151,5.98418442393441,68.6479778025323));
#200582=CARTESIAN_POINT('Ctrl Pts',(3.09910619832137,6.01563211736939,68.6512130080706));
#200583=CARTESIAN_POINT('Origin',(0.,0.,4.30282021618968));
#200584=CARTESIAN_POINT('',(3.09910619832143,6.01563211736936,71.0458824924514));
#200585=CARTESIAN_POINT('',(3.0991061983213,6.01563211736942,70.6515955249703));
#200586=CARTESIAN_POINT('',(3.09910619832133,6.0156321173694,4.30282021618968));
#200587=CARTESIAN_POINT('',(-6.76699999999972,1.95537661063743E-6,69.6972235144016));
#200588=CARTESIAN_POINT('Ctrl Pts',(-6.76699999999972,1.95537661063744E-6,
69.6972235144016));
#200589=CARTESIAN_POINT('Ctrl Pts',(-6.7670000509717,-0.176397498243203,
69.7055417487154));
#200590=CARTESIAN_POINT('Ctrl Pts',(-6.76009830406571,-0.352944500227869,
69.7138599830292));
#200591=CARTESIAN_POINT('Ctrl Pts',(-6.74628617363261,-0.52906697444988,
69.7221782173429));
#200592=CARTESIAN_POINT('Ctrl Pts',(-6.73248404601485,-0.705061899877223,
69.730490427549));
#200593=CARTESIAN_POINT('Ctrl Pts',(-6.71178153440809,-0.880632564880317,
69.738802637755));
#200594=CARTESIAN_POINT('Ctrl Pts',(-6.6842221106453,-1.05520793001215,
69.747114847961));
#200595=CARTESIAN_POINT('Ctrl Pts',(-6.6566776101285,-1.22968876373652,
69.7554225571601));
#200596=CARTESIAN_POINT('Ctrl Pts',(-6.62228365146343,-1.40317502912908,
69.7637302663592));
#200597=CARTESIAN_POINT('Ctrl Pts',(-6.58113545826471,-1.5751016094116,
69.7720379755583));
#200598=CARTESIAN_POINT('Ctrl Pts',(-6.5399983857192,-1.74698172505669,
69.7803434395275));
#200599=CARTESIAN_POINT('Ctrl Pts',(-6.49211079391409,-1.91730265716737,
69.7886489034967));
#200600=CARTESIAN_POINT('Ctrl Pts',(-6.43761892794818,-2.08550989892719,
69.796954367466));
#200601=CARTESIAN_POINT('Ctrl Pts',(-6.38313412606942,-2.25369533503596,
69.8052587547512));
#200602=CARTESIAN_POINT('Ctrl Pts',(-6.32204686255277,-2.4197672959954,
69.8135631420363));
#200603=CARTESIAN_POINT('Ctrl Pts',(-6.25455317910352,-2.58318670052439,
69.8218675293215));
#200604=CARTESIAN_POINT('Ctrl Pts',(-6.18705706475731,-2.74661199087429,
69.830172215703));
#200605=CARTESIAN_POINT('Ctrl Pts',(-6.11315420338471,-2.90738421309786,
69.8384769020845));
#200606=CARTESIAN_POINT('Ctrl Pts',(-6.03308875844027,-3.0649843446226,
69.8467815884659));
#200607=CARTESIAN_POINT('Ctrl Pts',(-5.95300716678851,-3.22261625918684,
69.8550879496441));
#200608=CARTESIAN_POINT('Ctrl Pts',(-5.86676067270544,-3.37707449853615,
69.8633943108222));
#200609=CARTESIAN_POINT('Ctrl Pts',(-5.77463944592092,-3.52786454808205,
69.8717006720004));
#200610=CARTESIAN_POINT('Ctrl Pts',(-5.68244049543082,-3.67878182087305,
69.880014041348));
#200611=CARTESIAN_POINT('Ctrl Pts',(-5.58435708959756,-3.82602442268361,
69.8883274106956));
#200612=CARTESIAN_POINT('Ctrl Pts',(-5.48072335517361,-3.96912591184187,
69.8966407800432));
#200613=CARTESIAN_POINT('Ctrl Pts',(-5.3770448097465,-4.11228927777527,
69.9049577440738));
#200614=CARTESIAN_POINT('Ctrl Pts',(-5.26781136237028,-4.25130768522227,
69.9132747081044));
#200615=CARTESIAN_POINT('Ctrl Pts',(-5.15339763823301,-4.38574757393246,
69.921591672135));
#200616=CARTESIAN_POINT('Ctrl Pts',(-5.03884469797823,-4.52035104615927,
69.9299187560656));
#200617=CARTESIAN_POINT('Ctrl Pts',(-4.91909911722505,-4.65036460781145,
69.9382458399962));
#200618=CARTESIAN_POINT('Ctrl Pts',(-4.79457345995464,-4.77539049053568,
69.9465729239267));
#200619=CARTESIAN_POINT('Ctrl Pts',(-4.69010025770259,-4.8802833665815,
69.9535590916187));
#200620=CARTESIAN_POINT('Ctrl Pts',(-4.58226322763573,-4.98166615886119,
69.9605452593107));
#200621=CARTESIAN_POINT('Ctrl Pts',(-4.47132378177533,-5.07932600238756,
69.9675314270027));
#200622=CARTESIAN_POINT('Ctrl Pts',(-4.34047883531328,-5.19450863106032,
69.9757710998309));
#200623=CARTESIAN_POINT('Ctrl Pts',(-4.20499906518267,-5.30479169746879,
69.9840107726591));
#200624=CARTESIAN_POINT('Ctrl Pts',(-4.06528500053261,-5.40978251544779,
69.9922504454873));
#200625=CARTESIAN_POINT('Ctrl Pts',(-3.92572602715796,-5.51465678710836,
70.0004809717677));
#200626=CARTESIAN_POINT('Ctrl Pts',(-3.78194240041995,-5.61425029598904,
70.0087114980482));
#200627=CARTESIAN_POINT('Ctrl Pts',(-3.6343701009482,-5.70820838524083,
70.0169420243286));
#200628=CARTESIAN_POINT('Ctrl Pts',(-3.48693529337704,-5.8020789345118,
70.0251648822952));
#200629=CARTESIAN_POINT('Ctrl Pts',(-3.335719141325,-5.89032433055239,70.0333877402618));
#200630=CARTESIAN_POINT('Ctrl Pts',(-3.18118926543502,-5.97263123401077,
70.0416105982285));
#200631=CARTESIAN_POINT('Ctrl Pts',(-3.02679635783686,-6.05486518435308,
70.0498261678257));
#200632=CARTESIAN_POINT('Ctrl Pts',(-2.86909589330713,-6.13117096632485,
70.0580417374231));
#200633=CARTESIAN_POINT('Ctrl Pts',(-2.70858281339615,-6.20127955691203,
70.0662573070204));
#200634=CARTESIAN_POINT('Ctrl Pts',(-2.54815225129109,-6.27135210553256,
70.0744686530941));
#200635=CARTESIAN_POINT('Ctrl Pts',(-2.38491227884607,-6.3352336656696,
70.0826799991678));
#200636=CARTESIAN_POINT('Ctrl Pts',(-2.21938105490168,-6.39270183358676,
70.0908913452415));
#200637=CARTESIAN_POINT('Ctrl Pts',(-2.05390539096749,-6.4501507125026,
70.0990999352039));
#200638=CARTESIAN_POINT('Ctrl Pts',(-1.88614034339804,-6.50119037084162,
70.1073085251663));
#200639=CARTESIAN_POINT('Ctrl Pts',(-1.71662268952433,-6.54564706822865,
70.1155171151288));
#200640=CARTESIAN_POINT('Ctrl Pts',(-1.64111704977945,-6.56544873077202,
70.1191733410283));
#200641=CARTESIAN_POINT('Ctrl Pts',(-1.56526392684188,-6.58394502631183,
70.1228295669278));
#200642=CARTESIAN_POINT('Ctrl Pts',(-1.48911170966338,-6.60112379191176,
70.1264857928273));
#200643=CARTESIAN_POINT('Ctrl Pts',(-1.30459979446344,-6.64274683401154,
70.1353445925855));
#200644=CARTESIAN_POINT('Ctrl Pts',(-1.11852309617017,-6.6765886904504,
70.1442033923436));
#200645=CARTESIAN_POINT('Ctrl Pts',(-0.931530948320751,-6.70257704859263,
70.1530621921018));
#200646=CARTESIAN_POINT('Ctrl Pts',(-0.744187664709552,-6.72861420793875,
70.1619376270044));
#200647=CARTESIAN_POINT('Ctrl Pts',(-0.555925752958089,-6.74676836154393,
70.170813061907));
#200648=CARTESIAN_POINT('Ctrl Pts',(-0.367398066213739,-6.75701914019358,
70.1796884968097));
#200649=CARTESIAN_POINT('Ctrl Pts',(-0.178332559623217,-6.76729916161544,
70.188589250991));
#200650=CARTESIAN_POINT('Ctrl Pts',(0.0109999786631993,-6.76963067577843,
70.1974900051723));
#200651=CARTESIAN_POINT('Ctrl Pts',(0.199945185758436,-6.76404545539813,
70.2063907593536));
#200652=CARTESIAN_POINT('Ctrl Pts',(0.389147190347937,-6.75845264408381,
70.2153036106471));
#200653=CARTESIAN_POINT('Ctrl Pts',(0.577960553243027,-6.74492161920995,
70.2242164619406));
#200654=CARTESIAN_POINT('Ctrl Pts',(0.765736238075063,-6.72353604985492,
70.2331293132341));
#200655=CARTESIAN_POINT('Ctrl Pts',(0.953928818231158,-6.70210300074299,
70.2420619526383));
#200656=CARTESIAN_POINT('Ctrl Pts',(1.14107885356263,-6.67278055646375,
70.2509945920425));
#200657=CARTESIAN_POINT('Ctrl Pts',(1.32654484722671,-6.63570401451845,
70.2599272314466));
#200658=CARTESIAN_POINT('Ctrl Pts',(1.50311753313202,-6.60040533541278,
70.2684315405151));
#200659=CARTESIAN_POINT('Ctrl Pts',(1.67816371471294,-6.55807880117575,
70.2769358495836));
#200660=CARTESIAN_POINT('Ctrl Pts',(1.85114289571097,-6.50888308234668,
70.2854401586521));
#200661=CARTESIAN_POINT('Ctrl Pts',(2.01839540892856,-6.46131604239289,
70.2936629231298));
#200662=CARTESIAN_POINT('Ctrl Pts',(2.18403584818975,-6.4072349802431,70.3018856876075));
#200663=CARTESIAN_POINT('Ctrl Pts',(2.34752030826476,-6.34676590101483,
70.3101084520851));
#200664=CARTESIAN_POINT('Ctrl Pts',(2.51083172901008,-6.28636082498864,
70.3183225132178));
#200665=CARTESIAN_POINT('Ctrl Pts',(2.67199138108945,-6.21958131934453,
70.3265365743505));
#200666=CARTESIAN_POINT('Ctrl Pts',(2.8304684966601,-6.14660370362485,70.3347506354831));
#200667=CARTESIAN_POINT('Ctrl Pts',(2.98880968970572,-6.07368867928793,
70.3429576515865));
#200668=CARTESIAN_POINT('Ctrl Pts',(3.14447260441048,-5.99458628132299,
70.3511646676898));
#200669=CARTESIAN_POINT('Ctrl Pts',(3.29694442810037,-5.90952167590727,
70.3593716837932));
#200670=CARTESIAN_POINT('Ctrl Pts',(3.44931608228028,-5.82451295543892,
70.367573308128));
#200671=CARTESIAN_POINT('Ctrl Pts',(3.59850050918707,-5.73355000385005,
70.3757749324628));
#200672=CARTESIAN_POINT('Ctrl Pts',(3.74400750141711,-5.63690489802094,
70.3839765567976));
#200673=CARTESIAN_POINT('Ctrl Pts',(3.88944809834842,-5.54030389165792,
70.3921744387054));
#200674=CARTESIAN_POINT('Ctrl Pts',(4.03121430544255,-5.43802609457757,
70.4003723206132));
#200675=CARTESIAN_POINT('Ctrl Pts',(4.16884295742833,-5.33038810935003,
70.408570202521));
#200676=CARTESIAN_POINT('Ctrl Pts',(4.30645946216917,-5.22275962436065,
70.4167673608754));
#200677=CARTESIAN_POINT('Ctrl Pts',(4.43993885156485,-5.10977210763387,
70.4249645192298));
#200678=CARTESIAN_POINT('Ctrl Pts',(4.56884896847381,-4.99178406016084,
70.4331616775842));
#200679=CARTESIAN_POINT('Ctrl Pts',(4.69775764991932,-4.87379732652985,
70.4413587446601));
#200680=CARTESIAN_POINT('Ctrl Pts',(4.82209689480017,-4.75081041453655,
70.4495558117359));
#200681=CARTESIAN_POINT('Ctrl Pts',(4.94146962371839,-4.62322040982997,
70.4577528788118));
#200682=CARTESIAN_POINT('Ctrl Pts',(5.06086272833705,-4.49560862681827,
70.465951345043));
#200683=CARTESIAN_POINT('Ctrl Pts',(5.17528738289712,-4.36339244777921,
70.4741498112742));
#200684=CARTESIAN_POINT('Ctrl Pts',(5.28438516793511,-4.22700395042487,
70.4823482775054));
#200685=CARTESIAN_POINT('Ctrl Pts',(5.39352141177922,-4.09056737382881,
70.4905496338339));
#200686=CARTESIAN_POINT('Ctrl Pts',(5.49732682147636,-3.94995582908396,
70.4987509901625));
#200687=CARTESIAN_POINT('Ctrl Pts',(5.59548484289048,-3.80563245374313,
70.506952346491));
#200688=CARTESIAN_POINT('Ctrl Pts',(5.6937546439409,-3.66114472693949,70.515163042297));
#200689=CARTESIAN_POINT('Ctrl Pts',(5.78636400652852,-3.51293702190165,
70.523373738103));
#200690=CARTESIAN_POINT('Ctrl Pts',(5.87304055902589,-3.36150019961875,
70.531584433909));
#200691=CARTESIAN_POINT('Ctrl Pts',(5.95976818572768,-3.20997414310819,
70.5397999678719));
#200692=CARTESIAN_POINT('Ctrl Pts',(6.04055586799709,-3.05521549406296,
70.5480155018348));
#200693=CARTESIAN_POINT('Ctrl Pts',(6.11517845212588,-2.89773730670247,
70.5562310357977));
#200694=CARTESIAN_POINT('Ctrl Pts',(6.1899168077135,-2.74001480349986,70.5644593155581));
#200695=CARTESIAN_POINT('Ctrl Pts',(6.25847081023811,-2.57956466018399,
70.5726875953185));
#200696=CARTESIAN_POINT('Ctrl Pts',(6.32066399006775,-2.41691864254073,
70.5809158750789));
#200697=CARTESIAN_POINT('Ctrl Pts',(6.37718372406161,-2.26910967574503,
70.5883935468198));
#200698=CARTESIAN_POINT('Ctrl Pts',(6.4284507766546,-2.11948757875861,70.5958712185607));
#200699=CARTESIAN_POINT('Ctrl Pts',(6.47436917792388,-1.96845948598118,
70.6033488903015));
#200700=CARTESIAN_POINT('Ctrl Pts',(6.52392164847197,-1.8054787437859,70.611418359152));
#200701=CARTESIAN_POINT('Ctrl Pts',(6.56740671387244,-1.64032697291816,
70.6194878280025));
#200702=CARTESIAN_POINT('Ctrl Pts',(6.60462488707267,-1.47350571802769,
70.627557296853));
#200703=CARTESIAN_POINT('Ctrl Pts',(6.64179664104419,-1.30689252584746,
70.6356167013052));
#200704=CARTESIAN_POINT('Ctrl Pts',(6.67271697474166,-1.13861435225918,
70.6436761057574));
#200705=CARTESIAN_POINT('Ctrl Pts',(6.6972351109188,-0.969190832125651,
70.6517355102096));
#200706=CARTESIAN_POINT('Ctrl Pts',(6.72172804768124,-0.799941443235838,
70.6597866313129));
#200707=CARTESIAN_POINT('Ctrl Pts',(6.73983182845517,-0.629549416551856,
70.6678377524163));
#200708=CARTESIAN_POINT('Ctrl Pts',(6.75144600718251,-0.458547502554958,
70.6758888735196));
#200709=CARTESIAN_POINT('Ctrl Pts',(6.76305079373281,-0.287683874724291,
70.6839334838264));
#200710=CARTESIAN_POINT('Ctrl Pts',(6.7681763983931,-0.116211711596677,
70.6919780941331));
#200711=CARTESIAN_POINT('Ctrl Pts',(6.76677380928631,0.0553282383315297,
70.7000227044399));
#200712=CARTESIAN_POINT('Ctrl Pts',(6.76537204743504,0.226767012961965,
70.708062569987));
#200713=CARTESIAN_POINT('Ctrl Pts',(6.75744975980007,0.398273122635417,
70.7161024355341));
#200714=CARTESIAN_POINT('Ctrl Pts',(6.74300994095709,0.569303026650945,
70.7241423010811));
#200715=CARTESIAN_POINT('Ctrl Pts',(6.72825891937657,0.744018916959518,
70.7323554394507));
#200716=CARTESIAN_POINT('Ctrl Pts',(6.70670622290195,0.918237444618071,
70.7405685778203));
#200717=CARTESIAN_POINT('Ctrl Pts',(6.67841119570085,1.09138118965717,70.7487817161899));
#200718=CARTESIAN_POINT('Ctrl Pts',(6.65072202773904,1.26081754339706,70.7568189930652));
#200719=CARTESIAN_POINT('Ctrl Pts',(6.61657641809556,1.42922429421833,70.7648562699405));
#200720=CARTESIAN_POINT('Ctrl Pts',(6.57608213318645,1.5960679113327,70.7728935468158));
#200721=CARTESIAN_POINT('Ctrl Pts',(6.53558356602429,1.7629291720872,70.7809316736296));
#200722=CARTESIAN_POINT('Ctrl Pts',(6.4887350748122,1.92822660688197,70.7889698004435));
#200723=CARTESIAN_POINT('Ctrl Pts',(6.43569495932967,2.09143954979786,70.7970079272573));
#200724=CARTESIAN_POINT('Ctrl Pts',(6.38263872636932,2.25470208877821,70.8050484966437));
#200725=CARTESIAN_POINT('Ctrl Pts',(6.32338723949669,2.41587851994996,70.8130890660301));
#200726=CARTESIAN_POINT('Ctrl Pts',(6.25814776127096,2.5744660801998,70.8211296354165));
#200727=CARTESIAN_POINT('Ctrl Pts',(6.19044632037162,2.7390383090039,70.8294736342944));
#200728=CARTESIAN_POINT('Ctrl Pts',(6.11629629914263,2.90082204906028,70.8378176331723));
#200729=CARTESIAN_POINT('Ctrl Pts',(6.03598221320989,3.05928222330237,70.8461616320502));
#200730=CARTESIAN_POINT('Ctrl Pts',(5.95845209476938,3.21224961295032,70.8542163987049));
#200731=CARTESIAN_POINT('Ctrl Pts',(5.87517833461974,3.36211970571117,70.8622711653595));
#200732=CARTESIAN_POINT('Ctrl Pts',(5.78646145606593,3.50844022572187,70.8703259320142));
#200733=CARTESIAN_POINT('Ctrl Pts',(5.6976774256564,3.6548714991158,70.8783867955079));
#200734=CARTESIAN_POINT('Ctrl Pts',(5.60344227763731,3.79774754043969,70.8864476590016));
#200735=CARTESIAN_POINT('Ctrl Pts',(5.50409760496662,3.93664813705781,70.8945085224953));
#200736=CARTESIAN_POINT('Ctrl Pts',(5.40461288606755,4.07574454190754,70.9025807493918));
#200737=CARTESIAN_POINT('Ctrl Pts',(5.30000449801997,4.21085402819647,70.9106529762883));
#200738=CARTESIAN_POINT('Ctrl Pts',(5.1906520976173,4.34159185109576,70.9187252031847));
#200739=CARTESIAN_POINT('Ctrl Pts',(5.17921675375252,4.35526353965021,70.9195693427736));
#200740=CARTESIAN_POINT('Ctrl Pts',(5.16772956208614,4.36888745707087,70.9204134823624));
#200741=CARTESIAN_POINT('Ctrl Pts',(5.15619097792548,4.38246318856872,70.9212576219513));
#200742=CARTESIAN_POINT('Ctrl Pts',(5.04227564832462,4.51649037133375,70.9295914381418));
#200743=CARTESIAN_POINT('Ctrl Pts',(4.9229849074674,4.64624541472378,70.9379252543322));
#200744=CARTESIAN_POINT('Ctrl Pts',(4.79866696305716,4.77127701749372,70.9462590705227));
#200745=CARTESIAN_POINT('Ctrl Pts',(4.67453741010077,4.89611914733169,70.9545802576453));
#200746=CARTESIAN_POINT('Ctrl Pts',(4.54539608396193,5.01625186105031,70.962901444768));
#200747=CARTESIAN_POINT('Ctrl Pts',(4.41163109147194,5.13125716688982,70.9712226318906));
#200748=CARTESIAN_POINT('Ctrl Pts',(4.27798265779982,5.24616226054191,70.9795365681795));
#200749=CARTESIAN_POINT('Ctrl Pts',(4.13971884260089,5.35594861784384,70.9878505044683));
#200750=CARTESIAN_POINT('Ctrl Pts',(3.99726491673493,5.4602346273251,70.9961644407571));
#200751=CARTESIAN_POINT('Ctrl Pts',(3.85493607555099,5.56442906627045,71.0044710768184));
#200752=CARTESIAN_POINT('Ctrl Pts',(3.70842473619227,5.66313257878805,71.0127777128796));
#200753=CARTESIAN_POINT('Ctrl Pts',(3.55818952006788,5.75600350410588,71.0210843489409));
#200754=CARTESIAN_POINT('Ctrl Pts',(3.40868838939289,5.84842063971509,71.0293503967777));
#200755=CARTESIAN_POINT('Ctrl Pts',(3.25549998152355,5.9350618741357,71.0376164446146));
#200756=CARTESIAN_POINT('Ctrl Pts',(3.09910619832143,6.01563211736936,71.0458824924514));
#200757=CARTESIAN_POINT('Ctrl Pts',(3.09910619832131,6.01563211736941,69.0457552630242));
#200758=CARTESIAN_POINT('Ctrl Pts',(2.93375330764821,6.10081787314656,69.0545047109265));
#200759=CARTESIAN_POINT('Ctrl Pts',(2.76488627843062,6.17918207037043,69.0632541588288));
#200760=CARTESIAN_POINT('Ctrl Pts',(2.5930786664669,6.25045854554002,69.0720036067311));
#200761=CARTESIAN_POINT('Ctrl Pts',(2.42127244185368,6.3217344451504,69.0807529839814));
#200762=CARTESIAN_POINT('Ctrl Pts',(2.2465259467246,6.38592262741839,69.0895023612317));
#200763=CARTESIAN_POINT('Ctrl Pts',(2.06943269687121,6.44280508110562,69.098251738482));
#200764=CARTESIAN_POINT('Ctrl Pts',(1.89234081822074,6.49968709436167,69.1070010479874));
#200765=CARTESIAN_POINT('Ctrl Pts',(1.71290249405583,6.54926340459546,69.1157503574927));
#200766=CARTESIAN_POINT('Ctrl Pts',(1.53172716625051,6.59136563150385,69.1244996669981));
#200767=CARTESIAN_POINT('Ctrl Pts',(1.35055318107328,6.63346754640711,69.1332489116653));
#200768=CARTESIAN_POINT('Ctrl Pts',(1.16764249714415,6.66809542395777,69.1419981563325));
#200769=CARTESIAN_POINT('Ctrl Pts',(0.983616340614323,6.69513165624669,
69.1507474009998));
#200770=CARTESIAN_POINT('Ctrl Pts',(0.799591486713716,6.72216769715963,
69.1594965837355));
#200771=CARTESIAN_POINT('Ctrl Pts',(0.614451459526494,6.74161215869373,
69.1682457664712));
#200772=CARTESIAN_POINT('Ctrl Pts',(0.428825047909969,6.75339900185714,
69.1769949492069));
#200773=CARTESIAN_POINT('Ctrl Pts',(0.243199888596737,6.76518576550222,
69.1857440729174));
#200774=CARTESIAN_POINT('Ctrl Pts',(0.0570886373916137,6.76931499599834,
69.194493196628));
#200775=CARTESIAN_POINT('Ctrl Pts',(-0.128876626811447,6.76577266947846,
69.2032423203385));
#200776=CARTESIAN_POINT('Ctrl Pts',(-0.314840698188492,6.76223036567992,
69.21199138793));
#200777=CARTESIAN_POINT('Ctrl Pts',(-0.500658497951622,6.7510166087922,
69.2207404555216));
#200778=CARTESIAN_POINT('Ctrl Pts',(-0.685698951926621,6.73216948296214,
69.2294895231131));
#200779=CARTESIAN_POINT('Ctrl Pts',(-0.870738280460322,6.71332247176287,
69.2382385374916));
#200780=CARTESIAN_POINT('Ctrl Pts',(-1.05499998761304,6.68684221356178,
69.2469875518702));
#200781=CARTESIAN_POINT('Ctrl Pts',(-1.23785829161479,6.65281863948511,
69.2557365662487));
#200782=CARTESIAN_POINT('Ctrl Pts',(-1.43007412917462,6.61705395368849,
69.2649332999479));
#200783=CARTESIAN_POINT('Ctrl Pts',(-1.62073882535849,6.57295372727776,
69.2741300336471));
#200784=CARTESIAN_POINT('Ctrl Pts',(-1.8091369609157,6.52068343478264,69.2833267673463));
#200785=CARTESIAN_POINT('Ctrl Pts',(-1.98838356186171,6.47095219815181,
69.2920767650599));
#200786=CARTESIAN_POINT('Ctrl Pts',(-2.16557827572594,6.4138258685087,69.3008267627736));
#200787=CARTESIAN_POINT('Ctrl Pts',(-2.34011918621764,6.34949849943254,
69.3095767604873));
#200788=CARTESIAN_POINT('Ctrl Pts',(-2.51465655691164,6.28517243495525,
69.3183265807456));
#200789=CARTESIAN_POINT('Ctrl Pts',(-2.68653996295395,6.21364572242345,
69.3270764010039));
#200790=CARTESIAN_POINT('Ctrl Pts',(-2.85518555380057,6.13516132252189,
69.3358262212622));
#200791=CARTESIAN_POINT('Ctrl Pts',(-3.02382794858766,6.05667841000468,
69.3445758756997));
#200792=CARTESIAN_POINT('Ctrl Pts',(-3.18923239109367,5.97123819492035,
69.3533255301373));
#200793=CARTESIAN_POINT('Ctrl Pts',(-3.35083705967792,5.87913088810659,
69.3620751845748));
#200794=CARTESIAN_POINT('Ctrl Pts',(-3.51243888042485,5.78702520443051,
69.3708246848237));
#200795=CARTESIAN_POINT('Ctrl Pts',(-3.67024081223767,5.68825280605734,
69.3795741850726));
#200796=CARTESIAN_POINT('Ctrl Pts',(-3.82370687544469,5.58314917682458,
69.3883236853216));
#200797=CARTESIAN_POINT('Ctrl Pts',(-3.97717043817886,5.4780472600797,69.397073043012));
#200798=CARTESIAN_POINT('Ctrl Pts',(-4.12629803722535,5.36661448084179,
69.4058224007025));
#200799=CARTESIAN_POINT('Ctrl Pts',(-4.27058317206984,5.24922931204514,
69.414571758393));
#200800=CARTESIAN_POINT('Ctrl Pts',(-4.41486614774901,5.13184589986733,
69.4233209851531));
#200801=CARTESIAN_POINT('Ctrl Pts',(-4.5543065819447,5.00851045722983,69.4320702119131));
#200802=CARTESIAN_POINT('Ctrl Pts',(-4.68843089001892,4.87964187103074,
69.4408194386732));
#200803=CARTESIAN_POINT('Ctrl Pts',(-4.82255336917882,4.75077504207914,
69.4495685461291));
#200804=CARTESIAN_POINT('Ctrl Pts',(-4.95135966065179,4.61637541908045,
69.458317653585));
#200805=CARTESIAN_POINT('Ctrl Pts',(-5.07441230869288,4.47689945401795,
69.467066761041));
#200806=CARTESIAN_POINT('Ctrl Pts',(-5.19746344226455,4.3374252055547,69.4758157608173));
#200807=CARTESIAN_POINT('Ctrl Pts',(-5.31476088454799,4.19287495491296,
69.4845647605937));
#200808=CARTESIAN_POINT('Ctrl Pts',(-5.4259062762888,4.0437396158667,69.49331376037));
#200809=CARTESIAN_POINT('Ctrl Pts',(-5.53706380672693,3.89458798906698,
69.5020637156647));
#200810=CARTESIAN_POINT('Ctrl Pts',(-5.64206777071888,3.74085050155248,
69.5108136709594));
#200811=CARTESIAN_POINT('Ctrl Pts',(-5.7405614816403,3.58304938223125,69.5195636262541));
#200812=CARTESIAN_POINT('Ctrl Pts',(-5.83905138951903,3.42525435593249,
69.5283132436952));
#200813=CARTESIAN_POINT('Ctrl Pts',(-5.9310313955767,3.26339625497152,69.5370628611363));
#200814=CARTESIAN_POINT('Ctrl Pts',(-6.01618907820861,3.09802485064976,
69.5458124785775));
#200815=CARTESIAN_POINT('Ctrl Pts',(-6.1013439254499,2.93265895249625,69.5545618046933));
#200816=CARTESIAN_POINT('Ctrl Pts',(-6.17967677261832,2.76378023986033,
69.5633111308092));
#200817=CARTESIAN_POINT('Ctrl Pts',(-6.25092157009219,2.59196229227129,
69.572060456925));
#200818=CARTESIAN_POINT('Ctrl Pts',(-6.32216437407761,2.42014915229073,
69.5808095382275));
#200819=CARTESIAN_POINT('Ctrl Pts',(-6.3863194154894,2.24539720662801,69.58955861953));
#200820=CARTESIAN_POINT('Ctrl Pts',(-6.44316881037564,2.06829994947604,
69.5983077008325));
#200821=CARTESIAN_POINT('Ctrl Pts',(-6.50002334524597,1.89118668024363,
69.6070575731748));
#200822=CARTESIAN_POINT('Ctrl Pts',(-6.5495708241112,1.71172794807611,69.6158074455171));
#200823=CARTESIAN_POINT('Ctrl Pts',(-6.59164294296106,1.53053334250245,
69.6245573178595));
#200824=CARTESIAN_POINT('Ctrl Pts',(-6.63371214082156,1.34935131693493,
69.6333065827144));
#200825=CARTESIAN_POINT('Ctrl Pts',(-6.66830695239711,1.16643393829647,
69.6420558475693));
#200826=CARTESIAN_POINT('Ctrl Pts',(-6.69530988154007,0.982402458339712,
69.6508051124242));
#200827=CARTESIAN_POINT('Ctrl Pts',(-6.72231419690497,0.798361530945886,
69.6595548264312));
#200828=CARTESIAN_POINT('Ctrl Pts',(-6.74172580829287,0.613206671361408,
69.6683045404383));
#200829=CARTESIAN_POINT('Ctrl Pts',(-6.75347878028186,0.427566795112439,
69.6770542544453));
#200830=CARTESIAN_POINT('Ctrl Pts',(-6.76248992368216,0.28523449420484,
69.6837627642335));
#200831=CARTESIAN_POINT('Ctrl Pts',(-6.76699999999996,0.142617266092229,
69.6904712740218));
#200832=CARTESIAN_POINT('Ctrl Pts',(-6.767,2.06659797691628E-12,69.69717978381));
#200833=CARTESIAN_POINT('',(-6.76699385815225,-0.00911722160370732,69.3028202161582));
#200834=CARTESIAN_POINT('Ctrl Pts',(3.09910619832137,6.01563211736939,68.6512130080706));
#200835=CARTESIAN_POINT('Ctrl Pts',(2.93085026217071,6.10231345101066,68.6601304166315));
#200836=CARTESIAN_POINT('Ctrl Pts',(2.75908892941873,6.18186318284619,68.6690478251925));
#200837=CARTESIAN_POINT('Ctrl Pts',(2.58443008893269,6.25403950382626,68.6779652337535));
#200838=CARTESIAN_POINT('Ctrl Pts',(2.40942174209233,6.32636025541599,68.6869004867645));
#200839=CARTESIAN_POINT('Ctrl Pts',(2.23150453288923,6.39127799148669,68.6958357397755));
#200840=CARTESIAN_POINT('Ctrl Pts',(2.05130448005828,6.44859976507248,68.7047709927865));
#200841=CARTESIAN_POINT('Ctrl Pts',(1.94511179249288,6.48237973959225,68.7100365768772));
#200842=CARTESIAN_POINT('Ctrl Pts',(1.8381265741877,6.51352274644971,68.7153021609678));
#200843=CARTESIAN_POINT('Ctrl Pts',(1.73047874464825,6.54199757828759,68.7205677450584));
#200844=CARTESIAN_POINT('Ctrl Pts',(1.56237613924332,6.58646381082468,68.7287904691802));
#200845=CARTESIAN_POINT('Ctrl Pts',(1.39233485484454,6.6245057207038,68.737013193302));
#200846=CARTESIAN_POINT('Ctrl Pts',(1.22088691786,6.65595403633456,68.7452359174238));
#200847=CARTESIAN_POINT('Ctrl Pts',(1.04962045267677,6.68736906499445,68.7534499380722));
#200848=CARTESIAN_POINT('Ctrl Pts',(0.876950649677882,6.71220433284285,
68.7616639587206));
#200849=CARTESIAN_POINT('Ctrl Pts',(0.703423920370135,6.73034054028852,
68.769877979369));
#200850=CARTESIAN_POINT('Ctrl Pts',(0.530046023940738,6.7484611924133,68.7780849548991));
#200851=CARTESIAN_POINT('Ctrl Pts',(0.355813019738684,6.759894190205,68.7862919304292));
#200852=CARTESIAN_POINT('Ctrl Pts',(0.181280812215935,6.76457140306186,
68.7944989059593));
#200853=CARTESIAN_POINT('Ctrl Pts',(0.00686326885021005,6.76924554308376,
68.8027004896712));
#200854=CARTESIAN_POINT('Ctrl Pts',(-0.167852728981888,6.76717272938516,
68.8109020733832));
#200855=CARTESIAN_POINT('Ctrl Pts',(-0.342306770803061,6.75833670918092,
68.8191036570951));
#200856=CARTESIAN_POINT('Ctrl Pts',(-0.516681208078639,6.74950472091178,
68.8273014983695));
#200857=CARTESIAN_POINT('Ctrl Pts',(-0.690793569955339,6.73391569250349,
68.8354993396439));
#200858=CARTESIAN_POINT('Ctrl Pts',(-0.864083972708392,6.71160546278672,
68.8436971809184));
#200859=CARTESIAN_POINT('Ctrl Pts',(-1.03735908312204,6.68929720187837,
68.8518942987588));
#200860=CARTESIAN_POINT('Ctrl Pts',(-1.2098120222788,6.66026895834882,68.8600914165992));
#200861=CARTESIAN_POINT('Ctrl Pts',(-1.38088818471595,6.62460842777231,
68.8682885344396));
#200862=CARTESIAN_POINT('Ctrl Pts',(-1.55196244373833,6.58894829395932,
68.8764855610779));
#200863=CARTESIAN_POINT('Ctrl Pts',(-1.72165960505051,6.54665609224798,
68.8846825877162));
#200864=CARTESIAN_POINT('Ctrl Pts',(-1.88943553250399,6.49787060262909,
68.8928796143544));
#200865=CARTESIAN_POINT('Ctrl Pts',(-2.05724010001063,6.4490767851229,68.9010780402594));
#200866=CARTESIAN_POINT('Ctrl Pts',(-2.22312243568794,6.39378757157837,
68.9092764661645));
#200867=CARTESIAN_POINT('Ctrl Pts',(-2.38655378691528,6.33219156549771,
68.9174748920695));
#200868=CARTESIAN_POINT('Ctrl Pts',(-2.55004275365022,6.27057384458003,
68.9256762082184));
#200869=CARTESIAN_POINT('Ctrl Pts',(-2.71107867914499,6.20264502861652,
68.9338775243674));
#200870=CARTESIAN_POINT('Ctrl Pts',(-2.86915295785607,6.12864179932437,
68.9420788405164));
#200871=CARTESIAN_POINT('Ctrl Pts',(-3.02740725666124,6.05455429276454,
68.950289496589));
#200872=CARTESIAN_POINT('Ctrl Pts',(-3.18269284507116,5.97437870476695,
68.9585001526617));
#200873=CARTESIAN_POINT('Ctrl Pts',(-3.33452496020774,5.88839810897256,
68.9667108087343));
#200874=CARTESIAN_POINT('Ctrl Pts',(-3.4864465463123,5.80236684690689,68.9749263031467));
#200875=CARTESIAN_POINT('Ctrl Pts',(-3.6349102979326,5.71052394677286,68.983141797559));
#200876=CARTESIAN_POINT('Ctrl Pts',(-3.77946072793055,5.61319566789104,
68.9913572919714));
#200877=CARTESIAN_POINT('Ctrl Pts',(-3.92423543050626,5.51571638244359,
68.9995855328703));
#200878=CARTESIAN_POINT('Ctrl Pts',(-4.06508438856073,5.41273492224001,
69.0078137737691));
#200879=CARTESIAN_POINT('Ctrl Pts',(-4.2015844285781,5.30461848670855,69.016042014668));
#200880=CARTESIAN_POINT('Ctrl Pts',(-4.32564111756129,5.20635795129044,
69.0235201686813));
#200881=CARTESIAN_POINT('Ctrl Pts',(-4.44610593272397,5.10385660146879,
69.0309983226946));
#200882=CARTESIAN_POINT('Ctrl Pts',(-4.56268847893731,4.99741561651348,
69.0384764767079));
#200883=CARTESIAN_POINT('Ctrl Pts',(-4.68678626522264,4.88411314515715,
69.0464366936417));
#200884=CARTESIAN_POINT('Ctrl Pts',(-4.80691272293021,4.76595505720867,
69.0543969105755));
#200885=CARTESIAN_POINT('Ctrl Pts',(-4.92264556725855,4.64325851306491,
69.0623571275092));
#200886=CARTESIAN_POINT('Ctrl Pts',(-5.03823363716505,4.52071545448823,
69.0703073867183));
#200887=CARTESIAN_POINT('Ctrl Pts',(-5.14943876600774,4.3936455058644,69.0782576459274));
#200888=CARTESIAN_POINT('Ctrl Pts',(-5.2558708782261,4.26240663374752,69.0862079051364));
#200889=CARTESIAN_POINT('Ctrl Pts',(-5.36219426084468,4.13130183347927,
69.0941500424687));
#200890=CARTESIAN_POINT('Ctrl Pts',(-5.46375408763842,3.99603687626425,
69.102092179801));
#200891=CARTESIAN_POINT('Ctrl Pts',(-5.56019655573902,3.85700703415847,
69.1100343171333));
#200892=CARTESIAN_POINT('Ctrl Pts',(-5.65773929486102,3.71639105982909,
69.118067062926));
#200893=CARTESIAN_POINT('Ctrl Pts',(-5.75004689685807,3.57192403130099,
69.1260998087187));
#200894=CARTESIAN_POINT('Ctrl Pts',(-5.83679413100016,3.42405071112011,
69.1341325545114));
#200895=CARTESIAN_POINT('Ctrl Pts',(-5.92244724556388,3.27804247743251,
69.1420639854377));
#200896=CARTESIAN_POINT('Ctrl Pts',(-6.00267923238474,3.12871371410209,
69.149995416364));
#200897=CARTESIAN_POINT('Ctrl Pts',(-6.07721996602323,2.97652254897702,
69.1579268472902));
#200898=CARTESIAN_POINT('Ctrl Pts',(-6.1517403892892,2.82437285190715,69.165856117112));
#200899=CARTESIAN_POINT('Ctrl Pts',(-6.22057247550348,2.66936264776593,
69.1737853869337));
#200900=CARTESIAN_POINT('Ctrl Pts',(-6.28349206592725,2.51197461321353,
69.1817146567555));
#200901=CARTESIAN_POINT('Ctrl Pts',(-6.34640746558075,2.3545970615186,69.1896433984469));
#200902=CARTESIAN_POINT('Ctrl Pts',(-6.40341101168622,2.19484235030835,
69.1975721401382));
#200903=CARTESIAN_POINT('Ctrl Pts',(-6.45432681739407,2.03321281086555,
69.2055008818296));
#200904=CARTESIAN_POINT('Ctrl Pts',(-6.50640624890183,1.86788940270147,
69.213610826357));
#200905=CARTESIAN_POINT('Ctrl Pts',(-6.55211619024014,1.70060483428536,
69.2217207708844));
#200906=CARTESIAN_POINT('Ctrl Pts',(-6.59132264495505,1.53191213524234,
69.2298307154118));
#200907=CARTESIAN_POINT('Ctrl Pts',(-6.6296864870876,1.36684492572138,69.2377663636058));
#200908=CARTESIAN_POINT('Ctrl Pts',(-6.66182351159207,1.20042988543856,
69.2457020117998));
#200909=CARTESIAN_POINT('Ctrl Pts',(-6.68766023032856,1.03319390420274,
69.2536376599938));
#200910=CARTESIAN_POINT('Ctrl Pts',(-6.71434815464369,0.860448237250684,
69.2618347526879));
#200911=CARTESIAN_POINT('Ctrl Pts',(-6.73431347837947,0.686827057175144,
69.270031845382));
#200912=CARTESIAN_POINT('Ctrl Pts',(-6.74753347295097,0.512914253463772,
69.278228938076));
#200913=CARTESIAN_POINT('Ctrl Pts',(-6.76075346752246,0.339001449752463,
69.2864260307701));
#200914=CARTESIAN_POINT('Ctrl Pts',(-6.7672281747193,0.164797468529505,
69.2946231234641));
#200915=CARTESIAN_POINT('Ctrl Pts',(-6.76699385815225,-0.00911722160361701,
69.3028202161582));
#200916=CARTESIAN_POINT('Ctrl Pts',(-6.76699385815134,-0.00911722227638602,
69.3028202161899));
#200917=CARTESIAN_POINT('Ctrl Pts',(-6.76665361760903,-0.261650898689682,
69.3147228447278));
#200918=CARTESIAN_POINT('Ctrl Pts',(-6.75217477231416,-0.513499531784462,
69.3266254732657));
#200919=CARTESIAN_POINT('Ctrl Pts',(-6.72380134021238,-0.763403259986641,
69.3385281018036));
#200920=CARTESIAN_POINT('Ctrl Pts',(-6.70961211025288,-0.888377265756445,
69.3444804706548));
#200921=CARTESIAN_POINT('Ctrl Pts',(-6.69194860585264,-1.01286553647403,
69.3504328395061));
#200922=CARTESIAN_POINT('Ctrl Pts',(-6.67084484497365,-1.13671370814663,
69.3563852083574));
#200923=CARTESIAN_POINT('Ctrl Pts',(-6.64130098240993,-1.31009291688794,
69.3647181291235));
#200924=CARTESIAN_POINT('Ctrl Pts',(-6.60495559427541,-1.48254225000074,
69.3730510498896));
#200925=CARTESIAN_POINT('Ctrl Pts',(-6.56187774888001,-1.65349611694537,
69.3813839706556));
#200926=CARTESIAN_POINT('Ctrl Pts',(-6.51885081105692,-1.82424795785407,
69.3897070439291));
#200927=CARTESIAN_POINT('Ctrl Pts',(-6.46910734950525,-1.99350751863075,
69.3980301172025));
#200928=CARTESIAN_POINT('Ctrl Pts',(-6.41276783970255,-2.16071692594765,
69.4063531904759));
#200929=CARTESIAN_POINT('Ctrl Pts',(-6.35648456809074,-2.32775942456054,
69.4146679556439));
#200930=CARTESIAN_POINT('Ctrl Pts',(-6.29361847645192,-2.49275551924861,
69.422982720812));
#200931=CARTESIAN_POINT('Ctrl Pts',(-6.22434053338133,-2.65515986797524,
69.43129748598));
#200932=CARTESIAN_POINT('Ctrl Pts',(-6.15511903574275,-2.81743189488023,
69.4396054765458));
#200933=CARTESIAN_POINT('Ctrl Pts',(-6.07949623219774,-2.97711606483858,
69.4479134671115));
#200934=CARTESIAN_POINT('Ctrl Pts',(-5.99769221339464,-3.13368427149024,
69.4562214576773));
#200935=CARTESIAN_POINT('Ctrl Pts',(-5.91593984841844,-3.2901536156757,
69.4645242022965));
#200936=CARTESIAN_POINT('Ctrl Pts',(-5.8280142071297,-3.4435106100762,69.4728269469158));
#200937=CARTESIAN_POINT('Ctrl Pts',(-5.73418268706396,-3.5932489353475,
69.481129691535));
#200938=CARTESIAN_POINT('Ctrl Pts',(-5.64038951279486,-3.7429260675851,
69.4894290431009));
#200939=CARTESIAN_POINT('Ctrl Pts',(-5.54069545335148,-3.88898718300963,
69.4977283946668));
#200940=CARTESIAN_POINT('Ctrl Pts',(-5.43541300878158,-4.03095204932631,
69.5060277462326));
#200941=CARTESIAN_POINT('Ctrl Pts',(-5.33015295590187,-4.17288672225873,
69.5143253326751));
#200942=CARTESIAN_POINT('Ctrl Pts',(-5.2193070928737,-4.3107266024241,69.5226229191175));
#200943=CARTESIAN_POINT('Ctrl Pts',(-5.10323039913294,-4.4440216576166,
69.53092050556));
#200944=CARTESIAN_POINT('Ctrl Pts',(-4.98715910372594,-4.57731051370769,
69.5392177061098));
#200945=CARTESIAN_POINT('Ctrl Pts',(-4.86585769095836,-4.70605470377706,
69.5475149066596));
#200946=CARTESIAN_POINT('Ctrl Pts',(-4.7397205824734,-4.82983827887415,
69.5558121072094));
#200947=CARTESIAN_POINT('Ctrl Pts',(-4.61356838023744,-4.953636666095,69.5641103006144));
#200948=CARTESIAN_POINT('Ctrl Pts',(-4.48257957797818,-5.07247301230305,
69.5724084940193));
#200949=CARTESIAN_POINT('Ctrl Pts',(-4.34718464040284,-5.1859690224919,
69.5807066874243));
#200950=CARTESIAN_POINT('Ctrl Pts',(-4.21169447753411,-5.29954485612957,
69.5890107170734));
#200951=CARTESIAN_POINT('Ctrl Pts',(-4.07179225408218,-5.40777262487352,
69.5973147467224));
#200952=CARTESIAN_POINT('Ctrl Pts',(-3.92794133492156,-5.51031449823099,
69.6056187763714));
#200953=CARTESIAN_POINT('Ctrl Pts',(-3.78403810735694,-5.6128936588145,
69.6139258256087));
#200954=CARTESIAN_POINT('Ctrl Pts',(-3.636183609776,-5.70978260720938,69.6222328748459));
#200955=CARTESIAN_POINT('Ctrl Pts',(-3.48486941236484,-5.80068738847078,
69.6305399240832));
#200956=CARTESIAN_POINT('Ctrl Pts',(-3.33339343391278,-5.89168936266177,
69.6388558549924));
#200957=CARTESIAN_POINT('Ctrl Pts',(-3.17845066714642,-5.97669421330461,
69.6471717859017));
#200958=CARTESIAN_POINT('Ctrl Pts',(-3.02055742531773,-6.0554538921833,
69.6554877168109));
#200959=CARTESIAN_POINT('Ctrl Pts',(-2.90153384758541,-6.11482475981906,
69.6617564578763));
#200960=CARTESIAN_POINT('Ctrl Pts',(-2.7808341726981,-6.17064776489301,
69.6680251989417));
#200961=CARTESIAN_POINT('Ctrl Pts',(-2.65868658361936,-6.2228349367537,
69.674293940007));
#200962=CARTESIAN_POINT('Ctrl Pts',(-2.49403137172798,-6.2931833562808,
69.6827442163997));
#200963=CARTESIAN_POINT('Ctrl Pts',(-2.32644257904295,-6.35705238656149,
69.6911944927923));
#200964=CARTESIAN_POINT('Ctrl Pts',(-2.15645702901611,-6.41420159349603,
69.6996447691849));
#200965=CARTESIAN_POINT('Ctrl Pts',(-1.98662149816884,-6.47130036392502,
69.7080875878641));
#200966=CARTESIAN_POINT('Ctrl Pts',(-1.81439373885687,-6.52169102642675,
69.7165304065432));
#200967=CARTESIAN_POINT('Ctrl Pts',(-1.64033030242613,-6.56518129977708,
69.7249732252224));
#200968=CARTESIAN_POINT('Ctrl Pts',(-1.46639678524654,-6.60863911241158,
69.733409742264));
#200969=CARTESIAN_POINT('Ctrl Pts',(-1.2906306428674,-6.64520672278109,
69.7418462593056));
#200970=CARTESIAN_POINT('Ctrl Pts',(-1.11360371186735,-6.67474162592945,
69.7502827763472));
#200971=CARTESIAN_POINT('Ctrl Pts',(-0.936703456296356,-6.70425539474244,
69.7587132564576));
#200972=CARTESIAN_POINT('Ctrl Pts',(-0.758544537924352,-6.72674643984214,
69.7671437365679));
#200973=CARTESIAN_POINT('Ctrl Pts',(-0.579709319837329,-6.74212326381636,
69.7755742166783));
#200974=CARTESIAN_POINT('Ctrl Pts',(-0.40095098455304,-6.75749347716132,
69.7840010724525));
#200975=CARTESIAN_POINT('Ctrl Pts',(-0.221517258924335,-6.76575553818316,
69.7924279282268));
#200976=CARTESIAN_POINT('Ctrl Pts',(-0.0419966274007469,-6.76686968126969,
69.800854784001));
#200977=CARTESIAN_POINT('Ctrl Pts',(0.137468588909518,-6.76798348043766,
69.8092790385366));
#200978=CARTESIAN_POINT('Ctrl Pts',(0.317020326428212,-6.76195375980029,
69.8177032930721));
#200979=CARTESIAN_POINT('Ctrl Pts',(0.496068720137571,-6.74879284204969,
69.8261275476077));
#200980=CARTESIAN_POINT('Ctrl Pts',(0.546516717905963,-6.74508467167431,
69.8285011336824));
#200981=CARTESIAN_POINT('Ctrl Pts',(0.596924762029775,-6.74081069757095,
69.8308747197571));
#200982=CARTESIAN_POINT('Ctrl Pts',(0.647279686896179,-6.73597194226131,
69.8332483058319));
#200983=CARTESIAN_POINT('Ctrl Pts',(0.83012424644261,-6.71840186176389,
69.841867071554));
#200984=CARTESIAN_POINT('Ctrl Pts',(1.01218623286149,-6.69338904782141,
69.8504858372761));
#200985=CARTESIAN_POINT('Ctrl Pts',(1.19285747028278,-6.66103445836985,
69.8591046029982));
#200986=CARTESIAN_POINT('Ctrl Pts',(1.37363723248664,-6.62866043430969,
69.8677285458016));
#200987=CARTESIAN_POINT('Ctrl Pts',(1.55302427909818,-6.58893588728978,
69.8763524886049));
#200988=CARTESIAN_POINT('Ctrl Pts',(1.73042144915389,-6.54201273373174,
69.8849764314083));
#200989=CARTESIAN_POINT('Ctrl Pts',(1.91422785891201,-6.4933942783904,69.8939119514289));
#200990=CARTESIAN_POINT('Ctrl Pts',(2.09589757769514,-6.43704745443902,
69.9028474714496));
#200991=CARTESIAN_POINT('Ctrl Pts',(2.27478504603368,-6.37319715639973,
69.9117829914703));
#200992=CARTESIAN_POINT('Ctrl Pts',(2.44775758702257,-6.3114580731798,69.9204230578617));
#200993=CARTESIAN_POINT('Ctrl Pts',(2.61812865798086,-6.2427039361286,69.9290631242531));
#200994=CARTESIAN_POINT('Ctrl Pts',(2.78533590748944,-6.16718678835415,
69.9377031906445));
#200995=CARTESIAN_POINT('Ctrl Pts',(2.96111982524427,-6.08779609128523,
69.9467864374799));
#200996=CARTESIAN_POINT('Ctrl Pts',(3.13340647645933,-6.00093053651775,
69.9558696843152));
#200997=CARTESIAN_POINT('Ctrl Pts',(3.30157228940492,-5.90693739748726,
69.9649529311505));
#200998=CARTESIAN_POINT('Ctrl Pts',(3.46973810235057,-5.81294425845674,
69.9740361779858));
#200999=CARTESIAN_POINT('Ctrl Pts',(3.633782764579,-5.71182376729964,69.9831194248212));
#201000=CARTESIAN_POINT('Ctrl Pts',(3.79311806221927,-5.603975764229,69.9922026716565));
#201001=CARTESIAN_POINT('Ctrl Pts',(3.95177566344159,-5.49658646808924,
70.0012472849691));
#201002=CARTESIAN_POINT('Ctrl Pts',(4.10591088612372,-5.38242831851227,
70.0102918982817));
#201003=CARTESIAN_POINT('Ctrl Pts',(4.25497498377582,-5.2618890987403,70.0193365115943));
#201004=CARTESIAN_POINT('Ctrl Pts',(4.40390228927358,-5.14146049460157,
70.028372824906));
#201005=CARTESIAN_POINT('Ctrl Pts',(4.54776757593037,-5.01466266073103,
70.0374091382178));
#201006=CARTESIAN_POINT('Ctrl Pts',(4.6860539502047,-4.88192455654232,70.0464454515295));
#201007=CARTESIAN_POINT('Ctrl Pts',(4.8240956070903,-4.74942135129006,70.0554657738009));
#201008=CARTESIAN_POINT('Ctrl Pts',(4.95657789467508,-4.610999031669,70.0644860960722));
#201009=CARTESIAN_POINT('Ctrl Pts',(5.08301975945316,-4.46712425672365,
70.0735064183435));
#201010=CARTESIAN_POINT('Ctrl Pts',(5.20930238895615,-4.32343067128705,
70.0825153808212));
#201011=CARTESIAN_POINT('Ctrl Pts',(5.32955962012002,-4.17429851201609,
70.0915243432988));
#201012=CARTESIAN_POINT('Ctrl Pts',(5.44334799706848,-4.02023028977329,
70.1005333057765));
#201013=CARTESIAN_POINT('Ctrl Pts',(5.55687797233936,-3.86651194058568,
70.1095218098288));
#201014=CARTESIAN_POINT('Ctrl Pts',(5.66396827503575,-3.70788009414105,
70.1185103138811));
#201015=CARTESIAN_POINT('Ctrl Pts',(5.76421668031801,-3.54486883570375,
70.1274988179333));
#201016=CARTESIAN_POINT('Ctrl Pts',(5.8521697207688,-3.40185074213007,70.135384891116));
#201017=CARTESIAN_POINT('Ctrl Pts',(5.93485673755005,-3.25546220835644,
70.1432709642987));
#201018=CARTESIAN_POINT('Ctrl Pts',(6.01203190609037,-3.10608457066955,
70.1511570374813));
#201019=CARTESIAN_POINT('Ctrl Pts',(6.09151067956367,-2.95224815343529,
70.1592785024024));
#201020=CARTESIAN_POINT('Ctrl Pts',(6.16510661331008,-2.79530964361943,
70.1673999673235));
#201021=CARTESIAN_POINT('Ctrl Pts',(6.23257786278774,-2.63576595779826,
70.1755214322446));
#201022=CARTESIAN_POINT('Ctrl Pts',(6.30004430105979,-2.47623364863726,
70.1836423180444));
#201023=CARTESIAN_POINT('Ctrl Pts',(6.36138678234842,-2.31409687076289,
70.1917632038442));
#201024=CARTESIAN_POINT('Ctrl Pts',(6.41641132721038,-2.14987317766569,
70.199884089644));
#201025=CARTESIAN_POINT('Ctrl Pts',(6.47144244947437,-1.9856298539608,70.2080059461802));
#201026=CARTESIAN_POINT('Ctrl Pts',(6.52015401630036,-1.81929946588932,
70.2161278027164));
#201027=CARTESIAN_POINT('Ctrl Pts',(6.56240171911994,-1.65141535565455,
70.2242496592526));
#201028=CARTESIAN_POINT('Ctrl Pts',(6.6046802457916,-1.4834087574587,70.2323774414816));
#201029=CARTESIAN_POINT('Ctrl Pts',(6.64048539981623,-1.31384652848552,
70.2405052237105));
#201030=CARTESIAN_POINT('Ctrl Pts',(6.66972373877747,-1.14327347926393,
70.2486330059394));
#201031=CARTESIAN_POINT('Ctrl Pts',(6.69897398852963,-0.97263094388149,
70.2567640991743));
#201032=CARTESIAN_POINT('Ctrl Pts',(6.72165204303201,-0.800977130240748,
70.2648951924092));
#201033=CARTESIAN_POINT('Ctrl Pts',(6.7377163131901,-0.628862372043433,
70.2730262856441));
#201034=CARTESIAN_POINT('Ctrl Pts',(6.75379811697253,-0.456559756228839,
70.2811662537008));
#201035=CARTESIAN_POINT('Ctrl Pts',(6.76325169822012,-0.283795556184407,
70.2893062217574));
#201036=CARTESIAN_POINT('Ctrl Pts',(6.7660875743135,-0.111121270333465,
70.2974461898141));
#201037=CARTESIAN_POINT('Ctrl Pts',(6.76755838172983,-0.021564952681512,
70.3016679276447));
#201038=CARTESIAN_POINT('Ctrl Pts',(6.76724994423267,0.0679672234920894,
70.3058896654754));
#201039=CARTESIAN_POINT('Ctrl Pts',(6.76516922120448,0.157398883311155,
70.310111403306));
#201040=CARTESIAN_POINT('Ctrl Pts',(6.76100939962017,0.336192381434253,
70.3185515829519));
#201041=CARTESIAN_POINT('Ctrl Pts',(6.74975428889474,0.514953378025566,
70.3269917625978));
#201042=CARTESIAN_POINT('Ctrl Pts',(6.73141204075728,0.69309518649888,70.3354319422436));
#201043=CARTESIAN_POINT('Ctrl Pts',(6.71308369016171,0.871102020609852,
70.34386572694));
#201044=CARTESIAN_POINT('Ctrl Pts',(6.68767894047735,1.04849027127232,70.3522995116364));
#201045=CARTESIAN_POINT('Ctrl Pts',(6.65525793640312,1.22467579380965,70.3607332963328));
#201046=CARTESIAN_POINT('Ctrl Pts',(6.62285651279589,1.40075491017886,70.3691619874966));
#201047=CARTESIAN_POINT('Ctrl Pts',(6.58344734291239,1.57563241940692,70.3775906786603));
#201048=CARTESIAN_POINT('Ctrl Pts',(6.53714214287557,1.74873142701793,70.3860193698241));
#201049=CARTESIAN_POINT('Ctrl Pts',(6.49085779765335,1.9217524747517,70.394444264896));
#201050=CARTESIAN_POINT('Ctrl Pts',(6.43768370096074,2.09299629634186,70.4028691599679));
#201051=CARTESIAN_POINT('Ctrl Pts',(6.37778228720542,2.26189789712287,70.4112940550398));
#201052=CARTESIAN_POINT('Ctrl Pts',(6.31789866052679,2.43074934440101,70.4197164484303));
#201053=CARTESIAN_POINT('Ctrl Pts',(6.251291811796,2.59725964387249,70.4281388418207));
#201054=CARTESIAN_POINT('Ctrl Pts',(6.1781736163657,2.76088025202882,70.4365612352112));
#201055=CARTESIAN_POINT('Ctrl Pts',(6.10505426995744,2.92450343579186,70.4449837611814));
#201056=CARTESIAN_POINT('Ctrl Pts',(6.0254235020109,3.08523653024769,70.4534062871516));
#201057=CARTESIAN_POINT('Ctrl Pts',(5.93954106611889,3.24255160697364,70.4618288131218));
#201058=CARTESIAN_POINT('Ctrl Pts',(5.85365572792102,3.39987199999579,70.4702516237223));
#201059=CARTESIAN_POINT('Ctrl Pts',(5.76151846022177,3.55377385210287,70.4786744343228));
#201060=CARTESIAN_POINT('Ctrl Pts',(5.66343472902432,3.70375432096694,70.4870972449233));
#201061=CARTESIAN_POINT('Ctrl Pts',(5.56533398886973,3.85376079833756,70.4955215161456));
#201062=CARTESIAN_POINT('Ctrl Pts',(5.46128491189105,3.99984425754618,70.5039457873678));
#201063=CARTESIAN_POINT('Ctrl Pts',(5.35163619679929,4.14153099917261,70.51237005859));
#201064=CARTESIAN_POINT('Ctrl Pts',(5.24195315353632,4.28326209924611,70.5207969672332));
#201065=CARTESIAN_POINT('Ctrl Pts',(5.12666718102087,4.42059347367828,70.5292238758764));
#201066=CARTESIAN_POINT('Ctrl Pts',(5.00616736453775,4.55308437416189,70.5376507845196));
#201067=CARTESIAN_POINT('Ctrl Pts',(4.88555919513755,4.68569440989378,70.5460852706028));
#201068=CARTESIAN_POINT('Ctrl Pts',(4.7597280385235,4.81345502761942,70.5545197566861));
#201069=CARTESIAN_POINT('Ctrl Pts',(4.6291007575472,4.93596142372243,70.5629542427694));
#201070=CARTESIAN_POINT('Ctrl Pts',(4.49841037744726,5.05852699617954,70.5713928031063));
#201071=CARTESIAN_POINT('Ctrl Pts',(4.36291950116576,5.17583306310957,70.5798313634432));
#201072=CARTESIAN_POINT('Ctrl Pts',(4.22308859466462,5.28751470178699,70.5882699237801));
#201073=CARTESIAN_POINT('Ctrl Pts',(4.08310137591308,5.3993211855985,70.5967179172988));
#201074=CARTESIAN_POINT('Ctrl Pts',(3.93876469835609,5.50549047618272,70.6051659108175));
#201075=CARTESIAN_POINT('Ctrl Pts',(3.79056955085271,5.60569990992635,70.6136139043362));
#201076=CARTESIAN_POINT('Ctrl Pts',(3.70633126528106,5.66266176757744,70.6184159812093));
#201077=CARTESIAN_POINT('Ctrl Pts',(3.62084677305327,5.71769874142581,70.6232180580824));
#201078=CARTESIAN_POINT('Ctrl Pts',(3.5342098779379,5.77075814245288,70.6280201349556));
#201079=CARTESIAN_POINT('Ctrl Pts',(3.39243104307275,5.85758835544981,70.6358785982938));
#201080=CARTESIAN_POINT('Ctrl Pts',(3.24726311766159,5.93930530447707,70.643737061632));
#201081=CARTESIAN_POINT('Ctrl Pts',(3.0991061983213,6.01563211736942,70.6515955249703));
#201082=CARTESIAN_POINT('Origin',(0.,0.,4.30282021618968));
#201083=CARTESIAN_POINT('',(3.09910619832135,6.0156321173694,73.0457552630242));
#201084=CARTESIAN_POINT('',(3.09910619832134,6.0156321173694,72.6513713193949));
#201085=CARTESIAN_POINT('',(3.09910619832133,6.0156321173694,4.30282021618968));
#201086=CARTESIAN_POINT('',(-6.76699982792737,0.000627241189940232,71.69717978381));
#201087=CARTESIAN_POINT('Ctrl Pts',(-6.767,2.40452268012357E-12,71.69717978381));
#201088=CARTESIAN_POINT('Ctrl Pts',(-6.76700000000007,-0.186007249524524,
71.7059292956212));
#201089=CARTESIAN_POINT('Ctrl Pts',(-6.75932637294533,-0.372014355747631,
71.7146788074324));
#201090=CARTESIAN_POINT('Ctrl Pts',(-6.74400518264199,-0.557389537485268,
71.7234283192436));
#201091=CARTESIAN_POINT('Ctrl Pts',(-6.72868405705108,-0.742763936249769,
71.7321777940992));
#201092=CARTESIAN_POINT('Ctrl Pts',(-6.70571545645751,-0.927506130240439,
71.7409272689549));
#201093=CARTESIAN_POINT('Ctrl Pts',(-6.67517739404828,-1.11098863989998,
71.7496767438106));
#201094=CARTESIAN_POINT('Ctrl Pts',(-6.64463945808704,-1.29447038981933,
71.7584261824376));
#201095=CARTESIAN_POINT('Ctrl Pts',(-6.60653217008357,-1.47669218313674,
71.7671756210646));
#201096=CARTESIAN_POINT('Ctrl Pts',(-6.56098496092678,-1.6570351059928,
71.7759250596916));
#201097=CARTESIAN_POINT('Ctrl Pts',(-6.51543793658297,-1.83737729708699,
71.7846744628168));
#201098=CARTESIAN_POINT('Ctrl Pts',(-6.4624511216742,-2.01584035510929,
71.793423865942));
#201099=CARTESIAN_POINT('Ctrl Pts',(-6.40220448374251,-2.19181813760798,
71.8021732690671));
#201100=CARTESIAN_POINT('Ctrl Pts',(-6.341958085265,-2.36779522067153,71.8109226374172));
#201101=CARTESIAN_POINT('Ctrl Pts',(-6.27445201433099,-2.54128677684177,
71.8196720057673));
#201102=CARTESIAN_POINT('Ctrl Pts',(-6.19991555071896,-2.71170355384825,
71.8284213741174));
#201103=CARTESIAN_POINT('Ctrl Pts',(-6.12537937716686,-2.8821196676749,
71.8371707084192));
#201104=CARTESIAN_POINT('Ctrl Pts',(-6.04381298052514,-3.04946076371797,
71.845920042721));
#201105=CARTESIAN_POINT('Ctrl Pts',(-5.95549339335826,-3.21315848374558,
71.8546693770228));
#201106=CARTESIAN_POINT('Ctrl Pts',(-5.86717414255411,-3.37685558033488,
71.8634186780029));
#201107=CARTESIAN_POINT('Ctrl Pts',(-5.77210188876609,-3.53690907646737,
71.8721679789831));
#201108=CARTESIAN_POINT('Ctrl Pts',(-5.67059953347017,-3.69277536969254,
71.8809172799633));
#201109=CARTESIAN_POINT('Ctrl Pts',(-5.56909755631399,-3.84864108224901,
71.8896665483486));
#201110=CARTESIAN_POINT('Ctrl Pts',(-5.46116568196859,-4.00031938297506,
71.8984158167339));
#201111=CARTESIAN_POINT('Ctrl Pts',(-5.34717048533604,-4.14729511859852,
71.9071650851192));
#201112=CARTESIAN_POINT('Ctrl Pts',(-5.23317570391827,-4.29427031887929,
71.9159143216362));
#201113=CARTESIAN_POINT('Ctrl Pts',(-5.11311782003492,-4.43654276189573,
71.9246635581533));
#201114=CARTESIAN_POINT('Ctrl Pts',(-4.98740458984718,-4.57362924351891,
71.9334127946703));
#201115=CARTESIAN_POINT('Ctrl Pts',(-4.86169180711711,-4.710715237203,71.9421620000458));
#201116=CARTESIAN_POINT('Ctrl Pts',(-4.73032391204143,-4.84261509523266,
71.9509112054212));
#201117=CARTESIAN_POINT('Ctrl Pts',(-4.59374707013574,-4.96888084538353,
71.9596604107966));
#201118=CARTESIAN_POINT('Ctrl Pts',(-4.45717070301414,-5.09514615659491,
71.9684095857571));
#201119=CARTESIAN_POINT('Ctrl Pts',(-4.31538563571003,-5.21577720459559,
71.9771587607175));
#201120=CARTESIAN_POINT('Ctrl Pts',(-4.16887341029464,-5.33036429232921,
71.985907935678));
#201121=CARTESIAN_POINT('Ctrl Pts',(-4.02236168203657,-5.44495099123652,
71.99465708095));
#201122=CARTESIAN_POINT('Ctrl Pts',(-3.87112305348112,-5.55349359438639,
72.003406226222));
#201123=CARTESIAN_POINT('Ctrl Pts',(-3.71567117017702,-5.65562346298932,
72.0121553714941));
#201124=CARTESIAN_POINT('Ctrl Pts',(-3.5602198014578,-5.75775299351668,
72.0209044878042));
#201125=CARTESIAN_POINT('Ctrl Pts',(-3.4005554453833,-5.85346967463883,
72.0296536041144));
#201126=CARTESIAN_POINT('Ctrl Pts',(-3.23722035986856,-5.942448429869,72.0384027204245));
#201127=CARTESIAN_POINT('Ctrl Pts',(-3.07388580147188,-6.03142689794525,
72.0471518084994));
#201128=CARTESIAN_POINT('Ctrl Pts',(-2.90688078896591,-6.11366734656775,
72.0559008965742));
#201129=CARTESIAN_POINT('Ctrl Pts',(-2.73677250721389,-6.18889046952345,
72.064649984649));
#201130=CARTESIAN_POINT('Ctrl Pts',(-2.56666476031491,-6.26411335596324,
72.0733990452151));
#201131=CARTESIAN_POINT('Ctrl Pts',(-2.39345402575164,-6.33231884500557,
72.0821481057811));
#201132=CARTESIAN_POINT('Ctrl Pts',(-2.21772856065579,-6.39327529762731,
72.0908971663472));
#201133=CARTESIAN_POINT('Ctrl Pts',(-2.04200363348509,-6.45423156365112,
72.0996462001308));
#201134=CARTESIAN_POINT('Ctrl Pts',(-1.86376426189281,-6.50793874375657,
72.1083952339145));
#201135=CARTESIAN_POINT('Ctrl Pts',(-1.68361577753164,-6.55421443909539,
72.1171442676982));
#201136=CARTESIAN_POINT('Ctrl Pts',(-1.50346782967816,-6.60048999661864,
72.1258932754261));
#201137=CARTESIAN_POINT('Ctrl Pts',(-1.32141105795011,-6.63933404237707,
72.1346422831539));
#201138=CARTESIAN_POINT('Ctrl Pts',(-1.13806375487053,-6.67061465607556,
72.1433912908817));
#201139=CARTESIAN_POINT('Ctrl Pts',(-0.954716982603581,-6.70189517921288,
72.1521402732801));
#201140=CARTESIAN_POINT('Ctrl Pts',(-0.770079968902963,-6.72561226592218,
72.1608892556785));
#201141=CARTESIAN_POINT('Ctrl Pts',(-0.584779765559332,-6.74168536983093,
72.1696382380769));
#201142=CARTESIAN_POINT('Ctrl Pts',(-0.391489830652384,-6.75845151013847,
72.1787644570868));
#201143=CARTESIAN_POINT('Ctrl Pts',(-0.197478578239416,-6.76689983031622,
72.1878906760966));
#201144=CARTESIAN_POINT('Ctrl Pts',(-0.0034628764524202,-6.76699911397118,
72.1970168951065));
#201145=CARTESIAN_POINT('Ctrl Pts',(0.1844898346537,-6.76709529501191,72.2058579197723));
#201146=CARTESIAN_POINT('Ctrl Pts',(0.372446404249175,-6.75935639738169,
72.2146989444381));
#201147=CARTESIAN_POINT('Ctrl Pts',(0.559755019488135,-6.74380925873188,
72.2235399691039));
#201148=CARTESIAN_POINT('Ctrl Pts',(0.745134705521623,-6.72842222659807,
72.2322899477137));
#201149=CARTESIAN_POINT('Ctrl Pts',(0.929879431228464,-6.70538706057525,
72.2410399263234));
#201150=CARTESIAN_POINT('Ctrl Pts',(1.1133616362682,-6.67478200894128,72.2497899049331));
#201151=CARTESIAN_POINT('Ctrl Pts',(1.29684196300732,-6.6441772706101,72.2585397939697));
#201152=CARTESIAN_POINT('Ctrl Pts',(1.47905951217543,-6.60600284890583,
72.2672896830062));
#201153=CARTESIAN_POINT('Ctrl Pts',(1.65939532067136,-6.56038841607218,
72.2760395720427));
#201154=CARTESIAN_POINT('Ctrl Pts',(1.83972934300849,-6.51477443503243,
72.2847893744149));
#201155=CARTESIAN_POINT('Ctrl Pts',(2.01818138406308,-6.46172066062127,
72.2935391767871));
#201156=CARTESIAN_POINT('Ctrl Pts',(2.19414528354239,-6.40140730423465,
72.3022889791592));
#201157=CARTESIAN_POINT('Ctrl Pts',(2.37010749864034,-6.34109452518629,
72.3110386977755));
#201158=CARTESIAN_POINT('Ctrl Pts',(2.5435813486649,-6.27352239616492,72.3197884163918));
#201159=CARTESIAN_POINT('Ctrl Pts',(2.71397759435581,-6.19892043966808,
72.3285381350081));
#201160=CARTESIAN_POINT('Ctrl Pts',(2.8843722655814,-6.12431917249507,72.3372877727768));
#201161=CARTESIAN_POINT('Ctrl Pts',(3.05168912680962,-6.04268832278795,
72.3460374105456));
#201162=CARTESIAN_POINT('Ctrl Pts',(3.21535986273852,-5.95430516123335,
72.3547870483143));
#201163=CARTESIAN_POINT('Ctrl Pts',(3.37902914072853,-5.86592278697435,
72.3635366081433));
#201164=CARTESIAN_POINT('Ctrl Pts',(3.53905210621596,-5.77078835741928,
72.3722861679724));
#201165=CARTESIAN_POINT('Ctrl Pts',(3.69488522831733,-5.66922500431606,
72.3810357278015));
#201166=CARTESIAN_POINT('Ctrl Pts',(3.85071701406976,-5.56766252217068,
72.3897852125986));
#201167=CARTESIAN_POINT('Ctrl Pts',(4.00235878822441,-5.45967138329342,
72.3985346973957));
#201168=CARTESIAN_POINT('Ctrl Pts',(4.14929549611363,-5.34561838199578,
72.4072841821929));
#201169=CARTESIAN_POINT('Ctrl Pts',(4.29623099276135,-5.23156632086979,
72.4160335948655));
#201170=CARTESIAN_POINT('Ctrl Pts',(4.43846127436079,-5.1114526730492,72.424783007538));
#201171=CARTESIAN_POINT('Ctrl Pts',(4.57550326054499,-4.98568540049833,
72.4335324202106));
#201172=CARTESIAN_POINT('Ctrl Pts',(4.71254416257839,-4.85991912290304,
72.4422817636659));
#201173=CARTESIAN_POINT('Ctrl Pts',(4.84439664018822,-4.72849950385357,
72.4510311071211));
#201174=CARTESIAN_POINT('Ctrl Pts',(4.97061286794807,-4.59187289861001,
72.4597804505764));
#201175=CARTESIAN_POINT('Ctrl Pts',(5.09682813912745,-4.45524732884616,
72.4685297277212));
#201176=CARTESIAN_POINT('Ctrl Pts',(5.21740705147897,-4.31341506235717,
72.477279004866));
#201177=CARTESIAN_POINT('Ctrl Pts',(5.33194007545752,-4.16685781275652,
72.4860282820109));
#201178=CARTESIAN_POINT('Ctrl Pts',(5.4464722694454,-4.02030162521768,72.494777495752));
#201179=CARTESIAN_POINT('Ctrl Pts',(5.55495848628166,-3.86902074887858,
72.5035267094931));
#201180=CARTESIAN_POINT('Ctrl Pts',(5.65703027291839,-3.71352898080585,
72.5122759232342));
#201181=CARTESIAN_POINT('Ctrl Pts',(5.75910135377053,-3.55803828789498,
72.5210250764781));
#201182=CARTESIAN_POINT('Ctrl Pts',(5.85475793592812,-3.3983370010661,72.529774229722));
#201183=CARTESIAN_POINT('Ctrl Pts',(5.94367514427461,-3.23496750823438,
72.5385233829659));
#201184=CARTESIAN_POINT('Ctrl Pts',(6.03259176732693,-3.07159909077619,
72.5472724786188));
#201185=CARTESIAN_POINT('Ctrl Pts',(6.11476896835969,-2.90456276731339,
72.5560215742717));
#201186=CARTESIAN_POINT('Ctrl Pts',(6.18992765547923,-2.73442583002966,
72.5647706699247));
#201187=CARTESIAN_POINT('Ctrl Pts',(6.26508587283093,-2.56428995616076,
72.5735197108927));
#201188=CARTESIAN_POINT('Ctrl Pts',(6.333225548272,-2.39105376935097,72.5822687518607));
#201189=CARTESIAN_POINT('Ctrl Pts',(6.3941152673307,-2.21530561053964,72.5910177928288));
#201190=CARTESIAN_POINT('Ctrl Pts',(6.45500462602884,-2.03955849184981,
72.5997667820178));
#201191=CARTESIAN_POINT('Ctrl Pts',(6.50864402040774,-1.86129970164427,
72.6085157712068));
#201192=CARTESIAN_POINT('Ctrl Pts',(6.55485128368631,-1.68113463135939,
72.6172647603958));
#201193=CARTESIAN_POINT('Ctrl Pts',(6.60199809554351,-1.49730620116761,
72.6261916458673));
#201194=CARTESIAN_POINT('Ctrl Pts',(6.64140720707892,-1.31149343245602,
72.6351185313387));
#201195=CARTESIAN_POINT('Ctrl Pts',(6.67293928722898,-1.12435326697442,
72.6440454168101));
#201196=CARTESIAN_POINT('Ctrl Pts',(6.70384625876269,-0.940923067005743,
72.6527953309876));
#201197=CARTESIAN_POINT('Ctrl Pts',(6.72718554579806,-0.75621789952081,
72.6615452451651));
#201198=CARTESIAN_POINT('Ctrl Pts',(6.74287786815335,-0.570865181253636,
72.6702951593425));
#201199=CARTESIAN_POINT('Ctrl Pts',(6.7585698819085,-0.385516108073125,
72.679044901447));
#201200=CARTESIAN_POINT('Ctrl Pts',(6.76661520773405,-0.199519795225566,
72.6877946435515));
#201201=CARTESIAN_POINT('Ctrl Pts',(6.76698651789579,-0.0135080204549074,
72.696544385656));
#201202=CARTESIAN_POINT('Ctrl Pts',(6.76735782124901,0.172500343513724,
72.705293967321));
#201203=CARTESIAN_POINT('Ctrl Pts',(6.7600553899518,0.358523882211705,72.7140435489859));
#201204=CARTESIAN_POINT('Ctrl Pts',(6.74510402742355,0.543930748565181,
72.7227931306509));
#201205=CARTESIAN_POINT('Ctrl Pts',(6.73015291918022,0.729334461616064,
72.7315425635076));
#201206=CARTESIAN_POINT('Ctrl Pts',(6.70755316306583,0.914121237635533,
72.7402919963642));
#201207=CARTESIAN_POINT('Ctrl Pts',(6.6773815187456,1.09766345166209,72.7490414292209));
#201208=CARTESIAN_POINT('Ctrl Pts',(6.64721034747552,1.28120278799754,72.7577907248985));
#201209=CARTESIAN_POINT('Ctrl Pts',(6.60946757205121,1.46349731860421,72.766540020576));
#201210=CARTESIAN_POINT('Ctrl Pts',(6.56428138111499,1.64392790278256,72.7752893162535));
#201211=CARTESIAN_POINT('Ctrl Pts',(6.51909583859826,1.82435589779142,72.7840384863791));
#201212=CARTESIAN_POINT('Ctrl Pts',(6.46646716392851,2.00291972192344,72.7927876565047));
#201213=CARTESIAN_POINT('Ctrl Pts',(6.40657409872859,2.17901292274734,72.8015368266303));
#201214=CARTESIAN_POINT('Ctrl Pts',(6.34668181342048,2.35510383059054,72.8102858828294));
#201215=CARTESIAN_POINT('Ctrl Pts',(6.27952541914017,2.52872390822663,72.8190349390286));
#201216=CARTESIAN_POINT('Ctrl Pts',(6.20533299175478,2.69928350890373,72.8277839952277));
#201217=CARTESIAN_POINT('Ctrl Pts',(6.12831602991508,2.87633637965711,72.8368661313858));
#201218=CARTESIAN_POINT('Ctrl Pts',(6.04371690605227,3.05009086601548,72.845948267544));
#201219=CARTESIAN_POINT('Ctrl Pts',(5.95184520316585,3.2199111288282,72.8550304037022));
#201220=CARTESIAN_POINT('Ctrl Pts',(5.86333549509223,3.38351691183107,72.8637801840458));
#201221=CARTESIAN_POINT('Ctrl Pts',(5.76807618099311,3.54347103712097,72.8725299643894));
#201222=CARTESIAN_POINT('Ctrl Pts',(5.66639083308953,3.69923018027792,72.881279744733));
#201223=CARTESIAN_POINT('Ctrl Pts',(5.5647091408213,3.85498372382152,72.8900292105179));
#201224=CARTESIAN_POINT('Ctrl Pts',(5.45660203371988,4.00654234702105,72.8987786763028));
#201225=CARTESIAN_POINT('Ctrl Pts',(5.34243669839129,4.15339127986781,72.9075281420877));
#201226=CARTESIAN_POINT('Ctrl Pts',(5.22827486050502,4.30023571401389,72.9162773398337));
#201227=CARTESIAN_POINT('Ctrl Pts',(5.10805534167019,4.44237052028576,72.9250265375797));
#201228=CARTESIAN_POINT('Ctrl Pts',(4.98218644339857,4.57931296628824,72.9337757353257));
#201229=CARTESIAN_POINT('Ctrl Pts',(4.85632073219489,4.71625194483461,72.9425247115374));
#201230=CARTESIAN_POINT('Ctrl Pts',(4.72480612170219,4.84799861524606,72.951273687749));
#201231=CARTESIAN_POINT('Ctrl Pts',(4.58808925235209,4.9741055489858,72.9600226639606));
#201232=CARTESIAN_POINT('Ctrl Pts',(4.45136349473944,5.10022068121298,72.9687722089623));
#201233=CARTESIAN_POINT('Ctrl Pts',(4.30943501209974,5.22069514871922,72.9775217539641));
#201234=CARTESIAN_POINT('Ctrl Pts',(4.16278587431674,5.33511975166341,72.9862712989658));
#201235=CARTESIAN_POINT('Ctrl Pts',(4.01614535740315,5.44953762807941,72.9950203296195));
#201236=CARTESIAN_POINT('Ctrl Pts',(3.86478496657765,5.55790617532895,73.0037693602732));
#201237=CARTESIAN_POINT('Ctrl Pts',(3.7092187474701,5.65985735539478,73.012518390927));
#201238=CARTESIAN_POINT('Ctrl Pts',(3.55365041605714,5.76180991977161,73.0212675403766));
#201239=CARTESIAN_POINT('Ctrl Pts',(3.39387638174335,5.85734478552922,73.0300166898262));
#201240=CARTESIAN_POINT('Ctrl Pts',(3.23043927904351,5.94613749121334,73.0387658392758));
#201241=CARTESIAN_POINT('Ctrl Pts',(3.18691767070303,5.96978206944215,73.0410956471919));
#201242=CARTESIAN_POINT('Ctrl Pts',(3.14313645919564,5.99294880633459,73.0434254551081));
#201243=CARTESIAN_POINT('Ctrl Pts',(3.09910619832135,6.0156321173694,73.0457552630242));
#201244=CARTESIAN_POINT('Ctrl Pts',(3.09910619832143,6.01563211736936,71.0458824924514));
#201245=CARTESIAN_POINT('Ctrl Pts',(2.94209088868808,6.09652255578414,71.0541813904892));
#201246=CARTESIAN_POINT('Ctrl Pts',(2.78184495475602,6.17129344529748,71.0624802885271));
#201247=CARTESIAN_POINT('Ctrl Pts',(2.61888209128078,6.23969114555912,71.0707791865649));
#201248=CARTESIAN_POINT('Ctrl Pts',(2.45595392010595,6.3080742849968,71.0790763178943));
#201249=CARTESIAN_POINT('Ctrl Pts',(2.2903102923292,6.37008680354989,71.0873734492237));
#201250=CARTESIAN_POINT('Ctrl Pts',(2.12248603660498,6.42552270437331,71.0956705805531));
#201251=CARTESIAN_POINT('Ctrl Pts',(1.95466960589001,6.48095602043069,71.1039673250187));
#201252=CARTESIAN_POINT('Ctrl Pts',(1.78467308026214,6.52981322083523,71.1122640694844));
#201253=CARTESIAN_POINT('Ctrl Pts',(1.61304782859842,6.57193774336412,71.12056081395));
#201254=CARTESIAN_POINT('Ctrl Pts',(1.44140204628814,6.61406730503309,71.1288585509125));
#201255=CARTESIAN_POINT('Ctrl Pts',(1.26812748775522,6.6494625016262,71.137156287875));
#201256=CARTESIAN_POINT('Ctrl Pts',(1.09378731642981,6.67801754313489,71.1454540248375));
#201257=CARTESIAN_POINT('Ctrl Pts',(0.919324345418592,6.70659269790891,
71.1537576064626));
#201258=CARTESIAN_POINT('Ctrl Pts',(0.743794605599573,6.72831801397396,
71.1620611880878));
#201259=CARTESIAN_POINT('Ctrl Pts',(0.567768919042361,6.74313928779241,
71.170364769713));
#201260=CARTESIAN_POINT('Ctrl Pts',(0.391679210801089,6.75796595220428,
71.1786713714047));
#201261=CARTESIAN_POINT('Ctrl Pts',(0.215093543606871,6.76588354772439,
71.1869779730963));
#201262=CARTESIAN_POINT('Ctrl Pts',(0.0385846176868022,6.76688999668814,
71.195284574788));
#201263=CARTESIAN_POINT('Ctrl Pts',(-0.138113486797284,6.76789752434277,
71.2036000793211));
#201264=CARTESIAN_POINT('Ctrl Pts',(-0.314734337484856,6.76197911106946,
71.2119155838542));
#201265=CARTESIAN_POINT('Ctrl Pts',(-0.490707366630687,6.74918478635267,
71.2202310883874));
#201266=CARTESIAN_POINT('Ctrl Pts',(-0.624276972018795,6.73947345211058,
71.2265428434585));
#201267=CARTESIAN_POINT('Ctrl Pts',(-0.75747339057754,6.72580174936138,
71.2328545985296));
#201268=CARTESIAN_POINT('Ctrl Pts',(-0.890050485105451,6.70821132150468,
71.2391663536007));
#201269=CARTESIAN_POINT('Ctrl Pts',(-1.06758137864267,6.68465639004218,
71.2476182775288));
#201270=CARTESIAN_POINT('Ctrl Pts',(-1.24432731076763,6.65402972143532,
71.256070201457));
#201271=CARTESIAN_POINT('Ctrl Pts',(-1.41970372915277,6.61639859148689,
71.2645221253851));
#201272=CARTESIAN_POINT('Ctrl Pts',(-1.59492497311713,6.5788007578553,71.2729665709851));
#201273=CARTESIAN_POINT('Ctrl Pts',(-1.76877879611551,6.53421088507903,
71.2814110165852));
#201274=CARTESIAN_POINT('Ctrl Pts',(-1.940688259322,6.48274772609036,71.2898554621852));
#201275=CARTESIAN_POINT('Ctrl Pts',(-2.1124689467072,6.43132311768781,71.2982935821276));
#201276=CARTESIAN_POINT('Ctrl Pts',(-2.28230786135585,6.37303558151365,
71.3067317020699));
#201277=CARTESIAN_POINT('Ctrl Pts',(-2.44964032459495,6.30805447662894,
71.3151698220122));
#201278=CARTESIAN_POINT('Ctrl Pts',(-2.61685222017403,6.2431201924245,71.3236018620562));
#201279=CARTESIAN_POINT('Ctrl Pts',(-2.78156095851281,6.17150207928877,
71.3320339021001));
#201280=CARTESIAN_POINT('Ctrl Pts',(-2.94321884257679,6.09341873209949,
71.340465942144));
#201281=CARTESIAN_POINT('Ctrl Pts',(-3.10480672631541,6.01536919618852,
71.3488943309863));
#201282=CARTESIAN_POINT('Ctrl Pts',(-3.26334609153346,5.93086015107284,
71.3573227198284));
#201283=CARTESIAN_POINT('Ctrl Pts',(-3.41831037467832,5.84015780457742,
71.3657511086706));
#201284=CARTESIAN_POINT('Ctrl Pts',(-3.57322600690949,5.7494839340117,71.3741768514268));
#201285=CARTESIAN_POINT('Ctrl Pts',(-3.72456850976261,5.65262080686151,
71.3826025941831));
#201286=CARTESIAN_POINT('Ctrl Pts',(-3.87183671278643,5.54988013109466,
71.3910283369393));
#201287=CARTESIAN_POINT('Ctrl Pts',(-3.91315779486081,5.52105275486156,
71.3933924644347));
#201288=CARTESIAN_POINT('Ctrl Pts',(-3.95415828337546,5.49176292349081,
71.3957565919301));
#201289=CARTESIAN_POINT('Ctrl Pts',(-3.9948275075642,5.46201814211638,71.3981207194255));
#201290=CARTESIAN_POINT('Ctrl Pts',(-4.14307559491541,5.35359200330005,
71.4067384736718));
#201291=CARTESIAN_POINT('Ctrl Pts',(-4.28685262780211,5.23916646674295,
71.4153562279182));
#201292=CARTESIAN_POINT('Ctrl Pts',(-4.42568726955956,5.11913871584453,
71.4239739821645));
#201293=CARTESIAN_POINT('Ctrl Pts',(-4.56460539846278,4.99903878717976,
71.4325969186312));
#201294=CARTESIAN_POINT('Ctrl Pts',(-4.69857497469454,4.87333012001369,
71.4412198550979));
#201295=CARTESIAN_POINT('Ctrl Pts',(-4.8271601468813,4.74244809316464,71.4498427915645));
#201296=CARTESIAN_POINT('Ctrl Pts',(-4.96041408538231,4.60681390408956,
71.4587788160383));
#201297=CARTESIAN_POINT('Ctrl Pts',(-5.08788504301749,4.46562390260936,
71.4677148405121));
#201298=CARTESIAN_POINT('Ctrl Pts',(-5.20913259310723,4.31940118852462,
71.4766508649859));
#201299=CARTESIAN_POINT('Ctrl Pts',(-5.32635123376672,4.17803727836012,
71.4852899561754));
#201300=CARTESIAN_POINT('Ctrl Pts',(-5.43775325768484,4.03197000708245,
71.4939290473648));
#201301=CARTESIAN_POINT('Ctrl Pts',(-5.54298386833789,3.88170308438782,
71.5025681385542));
#201302=CARTESIAN_POINT('Ctrl Pts',(-5.65363978417994,3.72368894906779,
71.5116526296702));
#201303=CARTESIAN_POINT('Ctrl Pts',(-5.75747092364945,3.56103102480029,
71.5207371207862));
#201304=CARTESIAN_POINT('Ctrl Pts',(-5.85411822018246,3.3943466034169,71.5298216119022));
#201305=CARTESIAN_POINT('Ctrl Pts',(-5.95076551671542,3.22766218203356,
71.5389061030182));
#201306=CARTESIAN_POINT('Ctrl Pts',(-6.0402288200107,3.05695162330793,71.5479905941342));
#201307=CARTESIAN_POINT('Ctrl Pts',(-6.12220636438889,2.88285938467976,
71.5570750852501));
#201308=CARTESIAN_POINT('Ctrl Pts',(-6.2044003493801,2.70830750028961,71.5661835616275));
#201309=CARTESIAN_POINT('Ctrl Pts',(-6.27914351223528,2.53020004223149,
71.5752920380048));
#201310=CARTESIAN_POINT('Ctrl Pts',(-6.346159090972,2.34916023124721,71.5844005143822));
#201311=CARTESIAN_POINT('Ctrl Pts',(-6.41530684317836,2.16236044192347,
71.5937987868345));
#201312=CARTESIAN_POINT('Ctrl Pts',(-6.47622707583673,1.97243884563274,
71.6031970592868));
#201313=CARTESIAN_POINT('Ctrl Pts',(-6.52866917929949,1.78010329679626,
71.6125953317391));
#201314=CARTESIAN_POINT('Ctrl Pts',(-6.57935300770177,1.5942163603615,71.6216784995909));
#201315=CARTESIAN_POINT('Ctrl Pts',(-6.62211787258374,1.40607494706007,
71.6307616674427));
#201316=CARTESIAN_POINT('Ctrl Pts',(-6.65678721428408,1.21633588442669,
71.6398448352944));
#201317=CARTESIAN_POINT('Ctrl Pts',(-6.69140850982577,1.02685976976572,
71.6489154153293));
#201318=CARTESIAN_POINT('Ctrl Pts',(-6.71795663055262,0.835790645655826,
71.6579859953642));
#201319=CARTESIAN_POINT('Ctrl Pts',(-6.73630570661486,0.643796883363165,
71.6670565753991));
#201320=CARTESIAN_POINT('Ctrl Pts',(-6.75461468962947,0.45222263075211,
71.6761073360602));
#201321=CARTESIAN_POINT('Ctrl Pts',(-6.76476036071652,0.259727996698518,
71.6851580967213));
#201322=CARTESIAN_POINT('Ctrl Pts',(-6.76666842810398,0.0669879399656761,
71.6942088573824));
#201323=CARTESIAN_POINT('Ctrl Pts',(-6.76687720347802,0.0458988643382756,
71.6951991661916));
#201324=CARTESIAN_POINT('Ctrl Pts',(-6.76698740789083,0.0248068593588396,
71.6961894750008));
#201325=CARTESIAN_POINT('Ctrl Pts',(-6.76699898145417,0.00371281540544154,
71.69717978381));
#201326=CARTESIAN_POINT('',(-6.76699597401548,0.00738157559828298,71.3028202162182));
#201327=CARTESIAN_POINT('Ctrl Pts',(3.0991061983213,6.01563211736942,70.6515955249703));
#201328=CARTESIAN_POINT('Ctrl Pts',(2.9439273477698,6.0955764570846,70.6598264419829));
#201329=CARTESIAN_POINT('Ctrl Pts',(2.78546950025012,6.16960710176201,70.6680573589954));
#201330=CARTESIAN_POINT('Ctrl Pts',(2.62422176771963,6.2374473235312,70.676288276008));
#201331=CARTESIAN_POINT('Ctrl Pts',(2.46312559961411,6.30522377904431,70.6845114563896));
#201332=CARTESIAN_POINT('Ctrl Pts',(2.29924509497393,6.36682126235569,70.6927346367712));
#201333=CARTESIAN_POINT('Ctrl Pts',(2.1330936584178,6.42200906604918,70.7009578171528));
#201334=CARTESIAN_POINT('Ctrl Pts',(1.96709140408611,6.47714731832446,70.7091736141957));
#201335=CARTESIAN_POINT('Ctrl Pts',(1.79882261816966,6.52588724955767,70.7173894112385));
#201336=CARTESIAN_POINT('Ctrl Pts',(1.62882023362179,6.56804641020024,70.7256052082814));
#201337=CARTESIAN_POINT('Ctrl Pts',(1.45890650422525,6.6101835851114,70.7338167208389));
#201338=CARTESIAN_POINT('Ctrl Pts',(1.28726132124077,6.64574673866785,70.7420282333963));
#201339=CARTESIAN_POINT('Ctrl Pts',(1.11443272197364,6.67460326223173,70.7502397459538));
#201340=CARTESIAN_POINT('Ctrl Pts',(0.941663085746926,6.70344994096453,
70.7584484570319));
#201341=CARTESIAN_POINT('Ctrl Pts',(0.767711188125084,6.72559448896618,
70.7666571681101));
#201342=CARTESIAN_POINT('Ctrl Pts',(0.593135298543037,6.74095538611718,
70.7748658791882));
#201343=CARTESIAN_POINT('Ctrl Pts',(0.507296674755447,6.74850830923126,
70.7789020863856));
#201344=CARTESIAN_POINT('Ctrl Pts',(0.421307322622372,6.75442195559597,
70.7829382935829));
#201345=CARTESIAN_POINT('Ctrl Pts',(0.335234169516869,6.75869122327602,
70.7869745007803));
#201346=CARTESIAN_POINT('Ctrl Pts',(0.146317993851626,6.76806155181527,
70.7958333005385));
#201347=CARTESIAN_POINT('Ctrl Pts',(-0.0428056339176083,6.76949762802394,
70.8046921002967));
#201348=CARTESIAN_POINT('Ctrl Pts',(-0.231484597436673,6.76303954455019,
70.8135509000549));
#201349=CARTESIAN_POINT('Ctrl Pts',(-0.420517864236536,6.75656933402147,
70.8224263349576));
#201350=CARTESIAN_POINT('Ctrl Pts',(-0.609104538966915,6.74217534833842,
70.8313017698603));
#201351=CARTESIAN_POINT('Ctrl Pts',(-0.796597943978947,6.7199494578195,
70.840177204763));
#201352=CARTESIAN_POINT('Ctrl Pts',(-0.984626218303849,6.69766016268755,
70.8490779589443));
#201353=CARTESIAN_POINT('Ctrl Pts',(-1.17155472263993,6.66749428329949,
70.8579787131257));
#201354=CARTESIAN_POINT('Ctrl Pts',(-1.35674423218656,6.62959531860192,
70.866879467307));
#201355=CARTESIAN_POINT('Ctrl Pts',(-1.54218543481759,6.59164484500764,
70.8757923186005));
#201356=CARTESIAN_POINT('Ctrl Pts',(-1.7258826687811,6.5459403498651,70.884705169894));
#201357=CARTESIAN_POINT('Ctrl Pts',(-1.90721085504091,6.49267554667674,
70.8936180211876));
#201358=CARTESIAN_POINT('Ctrl Pts',(-2.08894162203473,6.43929248617822,
70.9025506605918));
#201359=CARTESIAN_POINT('Ctrl Pts',(-2.26829257115235,6.37831561749839,
70.911483299996));
#201360=CARTESIAN_POINT('Ctrl Pts',(-2.44465490341659,6.3099882252823,70.9204159394002));
#201361=CARTESIAN_POINT('Ctrl Pts',(-2.61256045895414,6.24493721012967,
70.9289202484684));
#201362=CARTESIAN_POINT('Ctrl Pts',(-2.77775712323498,6.1732241478927,70.9374245575367));
#201363=CARTESIAN_POINT('Ctrl Pts',(-2.93973960969522,6.09509803261514,
70.945928866605));
#201364=CARTESIAN_POINT('Ctrl Pts',(-3.09635948615719,6.01955836909586,
70.9541516310826));
#201365=CARTESIAN_POINT('Ctrl Pts',(-3.2502742704664,5.9378775538885,70.9623743955603));
#201366=CARTESIAN_POINT('Ctrl Pts',(-3.40096971677294,5.85027298385242,
70.970597160038));
#201367=CARTESIAN_POINT('Ctrl Pts',(-3.55150566021883,5.76276113844649,
70.9788112211706));
#201368=CARTESIAN_POINT('Ctrl Pts',(-3.6988287435289,5.66933820252418,70.9870252823033));
#201369=CARTESIAN_POINT('Ctrl Pts',(-3.84244629057806,5.57026888974158,
70.995239343436));
#201370=CARTESIAN_POINT('Ctrl Pts',(-3.98594065984513,5.47128454664739,
71.0034463595393));
#201371=CARTESIAN_POINT('Ctrl Pts',(-4.12573552882683,5.36666367404273,
71.0116533756427));
#201372=CARTESIAN_POINT('Ctrl Pts',(-4.26136428589238,5.25671603027222,
71.019860391746));
#201373=CARTESIAN_POINT('Ctrl Pts',(-4.39690393884729,5.14684061887505,
71.0280620160808));
#201374=CARTESIAN_POINT('Ctrl Pts',(-4.52828265402812,5.03164563204686,
71.0362636404155));
#201375=CARTESIAN_POINT('Ctrl Pts',(-4.65506413360352,4.91148316825357,
71.0444652647503));
#201376=CARTESIAN_POINT('Ctrl Pts',(-4.78178776239174,4.79137553496978,
71.0526631466581));
#201377=CARTESIAN_POINT('Ctrl Pts',(-4.90391807495056,4.66630518674944,
71.0608610285659));
#201378=CARTESIAN_POINT('Ctrl Pts',(-5.02105304947212,4.53666345174367,
71.0690589104738));
#201379=CARTESIAN_POINT('Ctrl Pts',(-5.13817768554101,4.40703315905003,
71.0772560688281));
#201380=CARTESIAN_POINT('Ctrl Pts',(-5.25030761510098,4.27283254345412,
71.0854532271825));
#201381=CARTESIAN_POINT('Ctrl Pts',(-5.35707854916275,4.13448889442219,
71.0936503855369));
#201382=CARTESIAN_POINT('Ctrl Pts',(-5.46384829428941,3.99614678589959,
71.1018474526128));
#201383=CARTESIAN_POINT('Ctrl Pts',(-5.56525894268932,3.85366201923922,
71.1100445196887));
#201384=CARTESIAN_POINT('Ctrl Pts',(-5.66098737936329,3.70749388275822,
71.1182415867646));
#201385=CARTESIAN_POINT('Ctrl Pts',(-5.7567321558999,3.56130079687496,71.1264400529958));
#201386=CARTESIAN_POINT('Ctrl Pts',(-5.84679259179066,3.41142338877672,
71.134638519227));
#201387=CARTESIAN_POINT('Ctrl Pts',(-5.9308896591847,3.25834879203808,71.1428369854582));
#201388=CARTESIAN_POINT('Ctrl Pts',(-6.0150163722104,3.10522023392775,71.1510383417867));
#201389=CARTESIAN_POINT('Ctrl Pts',(-6.09317535648685,2.9488925563572,71.1592396981152));
#201390=CARTESIAN_POINT('Ctrl Pts',(-6.16513415501936,2.78987631457271,
71.1674410544438));
#201391=CARTESIAN_POINT('Ctrl Pts',(-6.23717489823892,2.63067898949561,
71.1756517502498));
#201392=CARTESIAN_POINT('Ctrl Pts',(-6.30300120180254,2.46878731080094,
71.1838624460558));
#201393=CARTESIAN_POINT('Ctrl Pts',(-6.36242889037979,2.30473157110771,
71.1920731418618));
#201394=CARTESIAN_POINT('Ctrl Pts',(-6.42189159675405,2.14057916148287,
71.2002886758246));
#201395=CARTESIAN_POINT('Ctrl Pts',(-6.4749480635796,1.97426049028573,71.2085042097875));
#201396=CARTESIAN_POINT('Ctrl Pts',(-6.52146443944355,1.80631961874782,
71.2167197437504));
#201397=CARTESIAN_POINT('Ctrl Pts',(-6.56805298204831,1.63811819928194,
71.2249480235108));
#201398=CARTESIAN_POINT('Ctrl Pts',(-6.60808107478164,1.46828989909528,
71.2331763032712));
#201399=CARTESIAN_POINT('Ctrl Pts',(-6.64146603762873,1.29738886654086,
71.2414045830316));
#201400=CARTESIAN_POINT('Ctrl Pts',(-6.67180552541044,1.14207793171024,
71.2488822547726));
#201401=CARTESIAN_POINT('Ctrl Pts',(-6.69665923944538,0.985881339277095,
71.2563599265136));
#201402=CARTESIAN_POINT('Ctrl Pts',(-6.71600243808305,0.829216649412278,
71.2638375982546));
#201403=CARTESIAN_POINT('Ctrl Pts',(-6.74961577604237,0.556975058692978,
71.276831804233));
#201404=CARTESIAN_POINT('Ctrl Pts',(-6.76669584267219,0.282524382040331,
71.2898260102114));
#201405=CARTESIAN_POINT('Ctrl Pts',(-6.76699597401482,0.00738157620036175,
71.3028202161898));
#201406=CARTESIAN_POINT('Ctrl Pts',(-6.76699597401548,0.00738157559829199,
71.3028202162182));
#201407=CARTESIAN_POINT('Ctrl Pts',(-6.76717949212259,-0.160857071485397,
71.3107656452367));
#201408=CARTESIAN_POINT('Ctrl Pts',(-6.7610850101191,-0.329400696816224,
71.3187110742551));
#201409=CARTESIAN_POINT('Ctrl Pts',(-6.74867107799455,-0.497722494006376,
71.3266565032735));
#201410=CARTESIAN_POINT('Ctrl Pts',(-6.7362701632057,-0.665867787787545,
71.3345936006597));
#201411=CARTESIAN_POINT('Ctrl Pts',(-6.71756300615423,-0.833791337887429,
71.3425306980459));
#201412=CARTESIAN_POINT('Ctrl Pts',(-6.69256010162055,-1.00096367876002,
71.3504677954321));
#201413=CARTESIAN_POINT('Ctrl Pts',(-6.66757768956765,-1.16799900451186,
71.3583983875414));
#201414=CARTESIAN_POINT('Ctrl Pts',(-6.63630985110431,-1.33428396923348,
71.3663289796508));
#201415=CARTESIAN_POINT('Ctrl Pts',(-6.59881906361541,-1.49929182138296,
71.3742595717602));
#201416=CARTESIAN_POINT('Ctrl Pts',(-6.56135044359369,-1.66420210806662,
71.3821854746871));
#201417=CARTESIAN_POINT('Ctrl Pts',(-6.51766628029368,-1.82783641220349,
71.3901113776141));
#201418=CARTESIAN_POINT('Ctrl Pts',(-6.46788050486346,-1.98967604770404,
71.3980372805411));
#201419=CARTESIAN_POINT('Ctrl Pts',(-6.41810573509665,-2.15147990687013,
71.4059614313648));
#201420=CARTESIAN_POINT('Ctrl Pts',(-6.36223214141232,-2.31148951843576,
71.4138855821885));
#201421=CARTESIAN_POINT('Ctrl Pts',(-6.30042409209219,-2.46919931552401,
71.4218097330122));
#201422=CARTESIAN_POINT('Ctrl Pts',(-6.2386211534355,-2.62689607221217,
71.4297332286192));
#201423=CARTESIAN_POINT('Ctrl Pts',(-6.17088487408092,-2.78229303526583,
71.4376567242262));
#201424=CARTESIAN_POINT('Ctrl Pts',(-6.09742840847457,-2.93490303136702,
71.4455802198332));
#201425=CARTESIAN_POINT('Ctrl Pts',(-6.02396286604566,-3.08753188508468,
71.4535046945257));
#201426=CARTESIAN_POINT('Ctrl Pts',(-5.94477589758388,-3.23737274119463,
71.4614291692182));
#201427=CARTESIAN_POINT('Ctrl Pts',(-5.86012727107888,-3.38396178565267,
71.4693536439107));
#201428=CARTESIAN_POINT('Ctrl Pts',(-5.77545071334609,-3.53059919961369,
71.477280733416));
#201429=CARTESIAN_POINT('Ctrl Pts',(-5.68530910465292,-3.6739823359453,
71.4852078229213));
#201430=CARTESIAN_POINT('Ctrl Pts',(-5.59000613642062,-3.81367544434235,
71.4931349124265));
#201431=CARTESIAN_POINT('Ctrl Pts',(-5.49459454317271,-3.95352777302772,
71.5010710371197));
#201432=CARTESIAN_POINT('Ctrl Pts',(-5.39401006165389,-4.08968136020956,
71.5090071618128));
#201433=CARTESIAN_POINT('Ctrl Pts',(-5.28859776599477,-4.22173218827475,
71.5169432865059));
#201434=CARTESIAN_POINT('Ctrl Pts',(-5.18312107389773,-4.35386368627413,
71.5248842593827));
#201435=CARTESIAN_POINT('Ctrl Pts',(-5.07281094777323,-4.4818871483275,
71.5328252322594));
#201436=CARTESIAN_POINT('Ctrl Pts',(-4.95804951925956,-4.60543526331335,
71.5407662051361));
#201437=CARTESIAN_POINT('Ctrl Pts',(-4.84310963577557,-4.72917549663965,
71.5487195262913));
#201438=CARTESIAN_POINT('Ctrl Pts',(-4.72370490072325,-4.84842621974421,
71.5566728474464));
#201439=CARTESIAN_POINT('Ctrl Pts',(-4.60025136267833,-4.96285969982793,
71.5646261686016));
#201440=CARTESIAN_POINT('Ctrl Pts',(-4.51167015056788,-5.0449687793437,
71.5703328890358));
#201441=CARTESIAN_POINT('Ctrl Pts',(-4.42100511994707,-5.12459858535971,
71.57603960947));
#201442=CARTESIAN_POINT('Ctrl Pts',(-4.32841875408156,-5.20164205701575,
71.5817463299042));
#201443=CARTESIAN_POINT('Ctrl Pts',(-4.193232474238,-5.31413400139708,71.59007876955));
#201444=CARTESIAN_POINT('Ctrl Pts',(-4.05348439408398,-5.42149710211226,
71.5984112091959));
#201445=CARTESIAN_POINT('Ctrl Pts',(-3.90959473330228,-5.523346632372,71.6067436488417));
#201446=CARTESIAN_POINT('Ctrl Pts',(-3.76587510147774,-5.62507581090303,
71.6150662423595));
#201447=CARTESIAN_POINT('Ctrl Pts',(-3.61802391975303,-5.72130419835902,
71.6233888358773));
#201448=CARTESIAN_POINT('Ctrl Pts',(-3.46649544371141,-5.81168635928747,
71.6317114293951));
#201449=CARTESIAN_POINT('Ctrl Pts',(-3.31511819536944,-5.90197831745903,
71.6400257168393));
#201450=CARTESIAN_POINT('Ctrl Pts',(-3.16007126151928,-5.98643549636477,
71.6483400042835));
#201451=CARTESIAN_POINT('Ctrl Pts',(-3.00183910827763,-6.0647548151607,
71.6566542917277));
#201452=CARTESIAN_POINT('Ctrl Pts',(-2.84373583348108,-6.14301034368507,
71.6649618072712));
#201453=CARTESIAN_POINT('Ctrl Pts',(-2.68245281923756,-6.21513781974245,
71.6732693228146));
#201454=CARTESIAN_POINT('Ctrl Pts',(-2.5185006408941,-6.28087919974712,
71.6815768383581));
#201455=CARTESIAN_POINT('Ctrl Pts',(-2.35465192683352,-6.34657909274743,
71.6898791113293));
#201456=CARTESIAN_POINT('Ctrl Pts',(-2.18813772759051,-6.40590079190939,
71.6981813843006));
#201457=CARTESIAN_POINT('Ctrl Pts',(-2.0194903885204,-6.45863356838532,
71.7064836572718));
#201458=CARTESIAN_POINT('Ctrl Pts',(-1.85091183091813,-6.5113448382203,
71.7147825442274));
#201459=CARTESIAN_POINT('Ctrl Pts',(-1.68020219858506,-6.55747243617869,
71.723081431183));
#201460=CARTESIAN_POINT('Ctrl Pts',(-1.5079111359526,-6.59685478133862,
71.7313803181387));
#201461=CARTESIAN_POINT('Ctrl Pts',(-1.33565662207888,-6.6362287721718,
71.7396774446198));
#201462=CARTESIAN_POINT('Ctrl Pts',(-1.16182168525784,-6.6688602833746,
71.7479745711009));
#201463=CARTESIAN_POINT('Ctrl Pts',(-0.986968600323926,-6.69463830105665,
71.7562716975821));
#201464=CARTESIAN_POINT('Ctrl Pts',(-0.812123536843244,-6.72041513616211,
71.7645684434293));
#201465=CARTESIAN_POINT('Ctrl Pts',(-0.636260762562076,-6.73933905368834,
71.7728651892766));
#201466=CARTESIAN_POINT('Ctrl Pts',(-0.459950349535424,-6.7513505816216,
71.7811619351239));
#201467=CARTESIAN_POINT('Ctrl Pts',(-0.283618713020177,-6.76336355545088,
71.7894596796977));
#201468=CARTESIAN_POINT('Ctrl Pts',(-0.106839677556948,-6.76846245861269,
71.7977574242715));
#201469=CARTESIAN_POINT('Ctrl Pts',(0.0698137925328148,-6.76663986291366,
71.8060551688453));
#201470=CARTESIAN_POINT('Ctrl Pts',(0.246591760216356,-6.76481598272937,
71.8143587613044));
#201471=CARTESIAN_POINT('Ctrl Pts',(0.423243637336409,-6.75606086014889,
71.8226623537635));
#201472=CARTESIAN_POINT('Ctrl Pts',(0.599197782242467,-6.74041920193067,
71.8309659462226));
#201473=CARTESIAN_POINT('Ctrl Pts',(0.775216041911384,-6.72477184415245,
71.8392725643727));
#201474=CARTESIAN_POINT('Ctrl Pts',(0.950535716746082,-6.70223298749084,
71.8475791825227));
#201475=CARTESIAN_POINT('Ctrl Pts',(1.12459227441324,-6.67289901139902,
71.8558858006728));
#201476=CARTESIAN_POINT('Ctrl Pts',(1.29883522503714,-6.64353362226188,
71.8642013141793));
#201477=CARTESIAN_POINT('Ctrl Pts',(1.47181201382979,-6.60735863986934,
71.8725168276857));
#201478=CARTESIAN_POINT('Ctrl Pts',(1.64296916808702,-6.56452140774295,
71.8808323411922));
#201479=CARTESIAN_POINT('Ctrl Pts',(1.77211105250717,-6.53219976215265,
71.8871065813127));
#201480=CARTESIAN_POINT('Ctrl Pts',(1.900217244485,-6.49608632537552,71.8933808214331));
#201481=CARTESIAN_POINT('Ctrl Pts',(2.02705658233125,-6.45626289830484,
71.8996550615536));
#201482=CARTESIAN_POINT('Ctrl Pts',(2.19791973292639,-6.40261742575404,
71.9081069854818));
#201483=CARTESIAN_POINT('Ctrl Pts',(2.36679702980146,-6.34213952935364,
71.9165589094099));
#201484=CARTESIAN_POINT('Ctrl Pts',(2.53312411224464,-6.27499571569294,
71.9250108333381));
#201485=CARTESIAN_POINT('Ctrl Pts',(2.69930402719014,-6.20791131140141,
71.9334552789382));
#201486=CARTESIAN_POINT('Ctrl Pts',(2.86293791938998,-6.13417286926218,
71.9418997245382));
#201487=CARTESIAN_POINT('Ctrl Pts',(3.02347775513098,-6.05399630527044,
71.9503441701383));
#201488=CARTESIAN_POINT('Ctrl Pts',(3.18389733193687,-5.97387980081571,
71.9587822900807));
#201489=CARTESIAN_POINT('Ctrl Pts',(3.34122717708123,-5.88733493597742,
71.9672204100231));
#201490=CARTESIAN_POINT('Ctrl Pts',(3.49494001234784,-5.79462538134175,
71.9756585299656));
#201491=CARTESIAN_POINT('Ctrl Pts',(3.64854209327107,-5.70198262650086,
71.9840905700095));
#201492=CARTESIAN_POINT('Ctrl Pts',(3.79853207968093,-5.60318421259049,
71.9925226100535));
#201493=CARTESIAN_POINT('Ctrl Pts',(3.94440786547106,-5.49853940522481,
72.0009546500974));
#201494=CARTESIAN_POINT('Ctrl Pts',(4.09022048482257,-5.39393991065567,
72.0093830389395));
#201495=CARTESIAN_POINT('Ctrl Pts',(4.23192218629874,-5.28349926221459,
72.0178114277816));
#201496=CARTESIAN_POINT('Ctrl Pts',(4.36903984800602,-5.16757000983398,
72.0262398166237));
#201497=CARTESIAN_POINT('Ctrl Pts',(4.50611446173429,-5.05167715334841,
72.03466555938));
#201498=CARTESIAN_POINT('Ctrl Pts',(4.63860765299018,-4.93029934301154,
72.0430913021362));
#201499=CARTESIAN_POINT('Ctrl Pts',(4.76607911837203,-4.80382960120549,
72.0515170448924));
#201500=CARTESIAN_POINT('Ctrl Pts',(4.80184555521866,-4.76834423183466,
72.0538811723878));
#201501=CARTESIAN_POINT('Ctrl Pts',(4.83721685378571,-4.73245822456643,
72.0562452998831));
#201502=CARTESIAN_POINT('Ctrl Pts',(4.87218378815524,-4.69618080299697,
72.0586094273784));
#201503=CARTESIAN_POINT('Ctrl Pts',(4.99964580014173,-4.56394178272546,
72.0672271816248));
#201504=CARTESIAN_POINT('Ctrl Pts',(5.12167431490016,-4.42655881366438,
72.0758449358711));
#201505=CARTESIAN_POINT('Ctrl Pts',(5.23787307658841,-4.28450401254921,
72.0844626901175));
#201506=CARTESIAN_POINT('Ctrl Pts',(5.35414171350818,-4.14236378787211,
72.0930856265841));
#201507=CARTESIAN_POINT('Ctrl Pts',(5.46457340843163,-3.99554636005134,
72.1017085630506));
#201508=CARTESIAN_POINT('Ctrl Pts',(5.56881341428031,-3.84455539132053,
72.1103314995172));
#201509=CARTESIAN_POINT('Ctrl Pts',(5.67683824399188,-3.68808212990486,
72.119267523991));
#201510=CARTESIAN_POINT('Ctrl Pts',(5.7782131351049,-3.52712687832724,72.1282035484649));
#201511=CARTESIAN_POINT('Ctrl Pts',(5.87259387358752,-3.36228050523783,
72.1371395729387));
#201512=CARTESIAN_POINT('Ctrl Pts',(5.96383845429135,-3.20291177773142,
72.1457786641281));
#201513=CARTESIAN_POINT('Ctrl Pts',(6.04854611952049,-3.03990665473596,
72.1544177553175));
#201514=CARTESIAN_POINT('Ctrl Pts',(6.1264536926981,-2.87382221983647,72.1630568465069));
#201515=CARTESIAN_POINT('Ctrl Pts',(6.20837789524314,-2.69917507926562,
72.1721413376229));
#201516=CARTESIAN_POINT('Ctrl Pts',(6.28278216656654,-2.5211230917456,72.181225828739));
#201517=CARTESIAN_POINT('Ctrl Pts',(6.34941859802417,-2.34033597311686,
72.1903103198551));
#201518=CARTESIAN_POINT('Ctrl Pts',(6.41605502948179,-2.15954885448812,
72.1993948109711));
#201519=CARTESIAN_POINT('Ctrl Pts',(6.47492353468485,-1.97602698496696,
72.2084793020871));
#201520=CARTESIAN_POINT('Ctrl Pts',(6.52583731511666,-1.79045701892869,
72.2175637932032));
#201521=CARTESIAN_POINT('Ctrl Pts',(6.57649029466412,-1.6058376169782,72.2266017498978));
#201522=CARTESIAN_POINT('Ctrl Pts',(6.61931794910389,-1.41901897994379,
72.2356397065923));
#201523=CARTESIAN_POINT('Ctrl Pts',(6.6541555407529,-1.23065146953451,72.2446776632869));
#201524=CARTESIAN_POINT('Ctrl Pts',(6.68896102508442,-1.04245756399213,
72.253707290343));
#201525=CARTESIAN_POINT('Ctrl Pts',(6.71579110493589,-0.852717869978947,
72.2627369173991));
#201526=CARTESIAN_POINT('Ctrl Pts',(6.73453201061368,-0.662093345397558,
72.2717665444551));
#201527=CARTESIAN_POINT('Ctrl Pts',(6.75323990762897,-0.471804570896919,
72.280780267482));
#201528=CARTESIAN_POINT('Ctrl Pts',(6.76388705756375,-0.280634315568752,
72.2897939905088));
#201529=CARTESIAN_POINT('Ctrl Pts',(6.76641142943289,-0.0892489083408666,
72.2988077135356));
#201530=CARTESIAN_POINT('Ctrl Pts',(6.76893264769673,0.101897408109752,
72.3078101760485));
#201531=CARTESIAN_POINT('Ctrl Pts',(6.76335133547306,0.293258101645628,
72.3168126385614));
#201532=CARTESIAN_POINT('Ctrl Pts',(6.74965733845046,0.484164035737715,
72.3258151010743));
#201533=CARTESIAN_POINT('Ctrl Pts',(6.73599407242338,0.674641553685474,
72.334797360966));
#201534=CARTESIAN_POINT('Ctrl Pts',(6.7142544792872,0.864666111181729,72.3437796208576));
#201535=CARTESIAN_POINT('Ctrl Pts',(6.68448026343205,1.05357135865941,72.3527618807493));
#201536=CARTESIAN_POINT('Ctrl Pts',(6.65823131769849,1.22011020602814,72.3606806401755));
#201537=CARTESIAN_POINT('Ctrl Pts',(6.62573845447481,1.38577897350931,72.3685993996017));
#201538=CARTESIAN_POINT('Ctrl Pts',(6.58706384370005,1.55012222712261,72.3765181590279));
#201539=CARTESIAN_POINT('Ctrl Pts',(6.54734312603064,1.71891079013266,72.3846511124348));
#201540=CARTESIAN_POINT('Ctrl Pts',(6.50111849405804,1.88622290372998,72.3927840658416));
#201541=CARTESIAN_POINT('Ctrl Pts',(6.44853036231096,2.05152264583009,72.4009170192485));
#201542=CARTESIAN_POINT('Ctrl Pts',(6.39594542355418,2.21681235143613,72.4090494788474));
#201543=CARTESIAN_POINT('Ctrl Pts',(6.33699786538176,2.38008958109444,72.4171819384462));
#201544=CARTESIAN_POINT('Ctrl Pts',(6.27187786437763,2.54083392891583,72.4253143980451));
#201545=CARTESIAN_POINT('Ctrl Pts',(6.20674947342521,2.70159898676096,72.433447905416));
#201546=CARTESIAN_POINT('Ctrl Pts',(6.13544719416951,2.85983017505991,72.4415814127868));
#201547=CARTESIAN_POINT('Ctrl Pts',(6.05820918349794,3.01502744415058,72.4497149201577));
#201548=CARTESIAN_POINT('Ctrl Pts',(5.98091415083708,3.1703392896906,72.4578544321986));
#201549=CARTESIAN_POINT('Ctrl Pts',(5.89767479720669,3.32261241532188,72.4659939442396));
#201550=CARTESIAN_POINT('Ctrl Pts',(5.80877536252484,3.47137116824525,72.4741334562806));
#201551=CARTESIAN_POINT('Ctrl Pts',(5.71983918507499,3.62019140421818,72.4822763324397));
#201552=CARTESIAN_POINT('Ctrl Pts',(5.62523846237361,3.76549406637753,72.4904192085988));
#201553=CARTESIAN_POINT('Ctrl Pts',(5.52530040407406,3.90683304541402,72.4985620847579));
#201554=CARTESIAN_POINT('Ctrl Pts',(5.42525311104038,4.04832651140034,72.5067138612791));
#201555=CARTESIAN_POINT('Ctrl Pts',(5.3198570518838,4.1858473514988,72.5148656378004));
#201556=CARTESIAN_POINT('Ctrl Pts',(5.20947977010969,4.31898246405538,72.5230174143216));
#201557=CARTESIAN_POINT('Ctrl Pts',(5.1532645700232,4.38678823776724,72.527169117832));
#201558=CARTESIAN_POINT('Ctrl Pts',(5.09575791151799,4.45345698846682,72.5313208213423));
#201559=CARTESIAN_POINT('Ctrl Pts',(5.03701193096813,4.51893790699593,72.5354725248527));
#201560=CARTESIAN_POINT('Ctrl Pts',(4.9177793359016,4.65183993315137,72.5438989461814));
#201561=CARTESIAN_POINT('Ctrl Pts',(4.79319172920386,4.78012248674441,72.5523253675102));
#201562=CARTESIAN_POINT('Ctrl Pts',(4.66363485474412,4.90334568856978,72.5607517888389));
#201563=CARTESIAN_POINT('Ctrl Pts',(4.53420009938071,5.0264527413593,72.5691702675019));
#201564=CARTESIAN_POINT('Ctrl Pts',(4.39980566021988,5.14450972332865,72.5775887461648));
#201565=CARTESIAN_POINT('Ctrl Pts',(4.26087500532992,5.25711262852098,72.5860072248278));
#201566=CARTESIAN_POINT('Ctrl Pts',(4.12202222607367,5.36965241573113,72.5944209846303));
#201567=CARTESIAN_POINT('Ctrl Pts',(3.9786385581983,5.4767440083115,72.6028347444329));
#201568=CARTESIAN_POINT('Ctrl Pts',(3.8311820745088,5.57802231189177,72.6112485042355));
#201569=CARTESIAN_POINT('Ctrl Pts',(3.68379394012754,5.6792536707612,72.6196583640762));
#201570=CARTESIAN_POINT('Ctrl Pts',(3.53233702992624,5.77467692376878,72.6280682239169));
#201571=CARTESIAN_POINT('Ctrl Pts',(3.37730026173126,5.86396895814686,72.6364780837576));
#201572=CARTESIAN_POINT('Ctrl Pts',(3.28578073723264,5.91667880641666,72.6414424956367));
#201573=CARTESIAN_POINT('Ctrl Pts',(3.19301433768587,5.96725294605387,72.6464069075158));
#201574=CARTESIAN_POINT('Ctrl Pts',(3.09910619832134,6.0156321173694,72.6513713193949));
#201575=CARTESIAN_POINT('Origin',(0.,0.,4.30282021618968));
#201576=CARTESIAN_POINT('',(3.09910619832135,6.0156321173694,75.0457552630242));
#201577=CARTESIAN_POINT('',(3.09910619832131,6.01563211736941,74.651395695404));
#201578=CARTESIAN_POINT('',(3.09910619832133,6.0156321173694,4.30282021618968));
#201579=CARTESIAN_POINT('',(-6.767,-9.23806438532518E-10,73.6971797838536));
#201580=CARTESIAN_POINT('Ctrl Pts',(-6.767,-9.23711102397149E-10,73.6971797838536));
#201581=CARTESIAN_POINT('Ctrl Pts',(-6.76699999997461,-0.18600725045061,
73.7059292956648));
#201582=CARTESIAN_POINT('Ctrl Pts',(-6.75932637289442,-0.372014356672636,
73.7146788074759));
#201583=CARTESIAN_POINT('Ctrl Pts',(-6.74400518256571,-0.557389538408147,
73.7234283192871));
#201584=CARTESIAN_POINT('Ctrl Pts',(-6.72868405694944,-0.742763937170584,
73.7321777941428));
#201585=CARTESIAN_POINT('Ctrl Pts',(-6.70571545633057,-0.927506131158146,
73.7409272689985));
#201586=CARTESIAN_POINT('Ctrl Pts',(-6.67517739389623,-1.11098864081354,
73.7496767438542));
#201587=CARTESIAN_POINT('Ctrl Pts',(-6.64463945790987,-1.29447039072881,
73.7584261824812));
#201588=CARTESIAN_POINT('Ctrl Pts',(-6.60653216988143,-1.47669218404109,
73.7671756211082));
#201589=CARTESIAN_POINT('Ctrl Pts',(-6.56098496069993,-1.65703510689102,
73.7759250597352));
#201590=CARTESIAN_POINT('Ctrl Pts',(-6.51543793633142,-1.837377297979,73.7846744628604));
#201591=CARTESIAN_POINT('Ctrl Pts',(-6.4624511213982,-2.01584035599409,
73.7934238659855));
#201592=CARTESIAN_POINT('Ctrl Pts',(-6.40220448344241,-2.19181813848456,
73.8021732691107));
#201593=CARTESIAN_POINT('Ctrl Pts',(-6.34195808494076,-2.36779522154001,
73.8109226374608));
#201594=CARTESIAN_POINT('Ctrl Pts',(-6.27445201398293,-2.54128677770116,
73.8196720058109));
#201595=CARTESIAN_POINT('Ctrl Pts',(-6.19991555034748,-2.71170355469758,
73.8284213741611));
#201596=CARTESIAN_POINT('Ctrl Pts',(-6.12537937677203,-2.88211966851404,
73.8371707084628));
#201597=CARTESIAN_POINT('Ctrl Pts',(-6.04381298010737,-3.04946076454597,
73.8459200427646));
#201598=CARTESIAN_POINT('Ctrl Pts',(-5.95549339291804,-3.2131584845615,
73.8546693770664));
#201599=CARTESIAN_POINT('Ctrl Pts',(-5.86717414209145,-3.37685558113873,
73.8634186780466));
#201600=CARTESIAN_POINT('Ctrl Pts',(-5.77210188828149,-3.53690907725823,
73.8721679790267));
#201601=CARTESIAN_POINT('Ctrl Pts',(-5.67059953296419,-3.69277537046952,
73.8809172800069));
#201602=CARTESIAN_POINT('Ctrl Pts',(-5.56909755578688,-3.84864108301174,
73.8896665483922));
#201603=CARTESIAN_POINT('Ctrl Pts',(-5.46116568142095,-4.00031938372266,
73.8984158167775));
#201604=CARTESIAN_POINT('Ctrl Pts',(-5.34717048476855,-4.1472951193302,
73.9071650851627));
#201605=CARTESIAN_POINT('Ctrl Pts',(-5.23317570333084,-4.29427031959514,
73.9159143216798));
#201606=CARTESIAN_POINT('Ctrl Pts',(-5.11311781942821,-4.43654276259495,
73.9246635581968));
#201607=CARTESIAN_POINT('Ctrl Pts',(-4.98740458922192,-4.57362924420073,
73.9334127947139));
#201608=CARTESIAN_POINT('Ctrl Pts',(-4.86169180647313,-4.71071523786761,
73.9421620000893));
#201609=CARTESIAN_POINT('Ctrl Pts',(-4.73032391137944,-4.84261509587929,
73.9509112054647));
#201610=CARTESIAN_POINT('Ctrl Pts',(-4.59374706945652,-4.96888084601147,
73.9596604108402));
#201611=CARTESIAN_POINT('Ctrl Pts',(-4.45717070231763,-5.09514615720421,
73.9684095858006));
#201612=CARTESIAN_POINT('Ctrl Pts',(-4.31538563499701,-5.21577720518553,
73.977158760761));
#201613=CARTESIAN_POINT('Ctrl Pts',(-4.16887340956593,-5.33036429289914,
73.9859079357215));
#201614=CARTESIAN_POINT('Ctrl Pts',(-4.02236168129221,-5.4449509917864,
73.9946570809935));
#201615=CARTESIAN_POINT('Ctrl Pts',(-3.87112305272195,-5.55349359491558,
74.0034062262656));
#201616=CARTESIAN_POINT('Ctrl Pts',(-3.71567116940392,-5.65562346349724,
74.0121553715376));
#201617=CARTESIAN_POINT('Ctrl Pts',(-3.56021980067038,-5.75775299400358,
74.0209044878477));
#201618=CARTESIAN_POINT('Ctrl Pts',(-3.40055544458243,-5.85346967510411,
74.0296536041579));
#201619=CARTESIAN_POINT('Ctrl Pts',(-3.23722035905514,-5.94244843031212,
74.0384027204681));
#201620=CARTESIAN_POINT('Ctrl Pts',(-3.07388580064597,-6.03142689836618,
74.047151808543));
#201621=CARTESIAN_POINT('Ctrl Pts',(-2.90688078812843,-6.11366734696596,
74.0559008966178));
#201622=CARTESIAN_POINT('Ctrl Pts',(-2.73677250636577,-6.1888904698985,
74.0646499846927));
#201623=CARTESIAN_POINT('Ctrl Pts',(-2.56666475945633,-6.26411335631504,
74.0733990452587));
#201624=CARTESIAN_POINT('Ctrl Pts',(-2.39345402488356,-6.33231884533368,
74.0821481058248));
#201625=CARTESIAN_POINT('Ctrl Pts',(-2.2177285597792,-6.39327529793139,
74.0908971663908));
#201626=CARTESIAN_POINT('Ctrl Pts',(-2.04200363259986,-6.4542315639312,
74.0996462001745));
#201627=CARTESIAN_POINT('Ctrl Pts',(-1.86376426099994,-6.50793874401228,
74.1083952339582));
#201628=CARTESIAN_POINT('Ctrl Pts',(-1.68361577663215,-6.55421443932645,
74.1171442677419));
#201629=CARTESIAN_POINT('Ctrl Pts',(-1.50346782877241,-6.60048999682495,
74.1258932754697));
#201630=CARTESIAN_POINT('Ctrl Pts',(-1.32141105703911,-6.63933404255839,
74.1346422831975));
#201631=CARTESIAN_POINT('Ctrl Pts',(-1.13806375395533,-6.6706146562317,
74.1433912909254));
#201632=CARTESIAN_POINT('Ctrl Pts',(-0.954716981684124,-6.70189517934386,
74.1521402733238));
#201633=CARTESIAN_POINT('Ctrl Pts',(-0.770079967980283,-6.72561226602783,
74.1608892557222));
#201634=CARTESIAN_POINT('Ctrl Pts',(-0.584779764634478,-6.74168536991115,
74.1696382381205));
#201635=CARTESIAN_POINT('Ctrl Pts',(-0.391489829734905,-6.75845151019133,
74.17876445713));
#201636=CARTESIAN_POINT('Ctrl Pts',(-0.197478577330526,-6.76689983034247,
74.1878906761394));
#201637=CARTESIAN_POINT('Ctrl Pts',(-0.00346287555322934,-6.76699911397164,
74.1970168951488));
#201638=CARTESIAN_POINT('Ctrl Pts',(0.184489835543577,-6.7670952949874,
74.2058579198142));
#201639=CARTESIAN_POINT('Ctrl Pts',(0.372446405128696,-6.75935639733297,
74.2146989444795));
#201640=CARTESIAN_POINT('Ctrl Pts',(0.55975502035636,-6.74380925865982,
74.2235399691449));
#201641=CARTESIAN_POINT('Ctrl Pts',(0.745134706387836,-6.72842222650215,
74.2322899477546));
#201642=CARTESIAN_POINT('Ctrl Pts',(0.929879432091684,-6.70538706045554,
74.2410399263644));
#201643=CARTESIAN_POINT('Ctrl Pts',(1.11336163712745,-6.67478200879796,
74.2497899049741));
#201644=CARTESIAN_POINT('Ctrl Pts',(1.29684196386254,-6.64417727044318,
74.2585397940106));
#201645=CARTESIAN_POINT('Ctrl Pts',(1.47905951302564,-6.60600284871547,
74.2672896830472));
#201646=CARTESIAN_POINT('Ctrl Pts',(1.65939532151561,-6.56038841585863,
74.2760395720837));
#201647=CARTESIAN_POINT('Ctrl Pts',(1.83972934384697,-6.51477443479565,
74.2847893744559));
#201648=CARTESIAN_POINT('Ctrl Pts',(2.01818138489482,-6.4617206603615,74.293539176828));
#201649=CARTESIAN_POINT('Ctrl Pts',(2.19414528436645,-6.40140730395219,
74.3022889792002));
#201650=CARTESIAN_POINT('Ctrl Pts',(2.37010749945662,-6.34109452488119,
74.3110386978165));
#201651=CARTESIAN_POINT('Ctrl Pts',(2.54358134947245,-6.2735223958375,74.3197884164328));
#201652=CARTESIAN_POINT('Ctrl Pts',(2.71397759515373,-6.19892043931874,
74.3285381350491));
#201653=CARTESIAN_POINT('Ctrl Pts',(2.88437226636986,-6.12431917212373,
74.3372877728178));
#201654=CARTESIAN_POINT('Ctrl Pts',(3.05168912758772,-6.042688322395,74.3460374105866));
#201655=CARTESIAN_POINT('Ctrl Pts',(3.21535986350538,-5.95430516081924,
74.3547870483553));
#201656=CARTESIAN_POINT('Ctrl Pts',(3.37902914148398,-5.86592278653917,
74.3635366081844));
#201657=CARTESIAN_POINT('Ctrl Pts',(3.53905210695913,-5.77078835696351,
74.3722861680134));
#201658=CARTESIAN_POINT('Ctrl Pts',(3.6948852290474,-5.66922500384024,74.3810357278425));
#201659=CARTESIAN_POINT('Ctrl Pts',(3.85071701478684,-5.56766252167474,
74.3897852126396));
#201660=CARTESIAN_POINT('Ctrl Pts',(4.00235878892765,-5.4596713827779,74.3985346974367));
#201661=CARTESIAN_POINT('Ctrl Pts',(4.14929549680226,-5.34561838146126,
74.4072841822339));
#201662=CARTESIAN_POINT('Ctrl Pts',(4.29623099343515,-5.23156632031645,
74.4160335949065));
#201663=CARTESIAN_POINT('Ctrl Pts',(4.43846127501901,-5.11145267247764,
74.424783007579));
#201664=CARTESIAN_POINT('Ctrl Pts',(4.5755032611869,-4.98568539990923,74.4335324202516));
#201665=CARTESIAN_POINT('Ctrl Pts',(4.71254416320399,-4.8599191222964,74.4422817637069));
#201666=CARTESIAN_POINT('Ctrl Pts',(4.84439664079679,-4.72849950323008,
74.4510311071621));
#201667=CARTESIAN_POINT('Ctrl Pts',(4.97061286853895,-4.59187289797039,
74.4597804506173));
#201668=CARTESIAN_POINT('Ctrl Pts',(5.09682813970068,-4.45524732819037,
74.4685297277622));
#201669=CARTESIAN_POINT('Ctrl Pts',(5.2174070520339,-4.31341506168594,74.477279004907));
#201670=CARTESIAN_POINT('Ctrl Pts',(5.33194007599354,-4.16685781207063,
74.4860282820518));
#201671=CARTESIAN_POINT('Ctrl Pts',(5.44647226996243,-4.02030162451723,
74.4947774957929));
#201672=CARTESIAN_POINT('Ctrl Pts',(5.55495848677911,-3.86902074816436,
74.503526709534));
#201673=CARTESIAN_POINT('Ctrl Pts',(5.65703027339572,-3.7135289800787,74.5122759232751));
#201674=CARTESIAN_POINT('Ctrl Pts',(5.75910135422783,-3.55803828715479,
74.521025076519));
#201675=CARTESIAN_POINT('Ctrl Pts',(5.85475793636485,-3.39833700031369,
74.5297742297629));
#201676=CARTESIAN_POINT('Ctrl Pts',(5.9436751446903,-3.23496750747063,74.5385233830068));
#201677=CARTESIAN_POINT('Ctrl Pts',(6.03259176772167,-3.07159909000093,
74.5472724786597));
#201678=CARTESIAN_POINT('Ctrl Pts',(6.11476896873301,-2.90456276652748,
74.5560215743127));
#201679=CARTESIAN_POINT('Ctrl Pts',(6.18992765583072,-2.734425829234,74.5647706699656));
#201680=CARTESIAN_POINT('Ctrl Pts',(6.26508587316051,-2.56428995535552,
74.5735197109336));
#201681=CARTESIAN_POINT('Ctrl Pts',(6.33322554857928,-2.39105376853707,
74.5822687519016));
#201682=CARTESIAN_POINT('Ctrl Pts',(6.39411526761537,-2.21530560971801,
74.5910177928697));
#201683=CARTESIAN_POINT('Ctrl Pts',(6.45500462629089,-2.03955849102044,
74.5997667820587));
#201684=CARTESIAN_POINT('Ctrl Pts',(6.50864402064686,-1.86129970080809,
74.6085157712477));
#201685=CARTESIAN_POINT('Ctrl Pts',(6.55485128390227,-1.68113463051737,
74.6172647604367));
#201686=CARTESIAN_POINT('Ctrl Pts',(6.60199809573133,-1.49730620033714,
74.6261916459073));
#201687=CARTESIAN_POINT('Ctrl Pts',(6.64140720723984,-1.31149343163847,
74.6351185313779));
#201688=CARTESIAN_POINT('Ctrl Pts',(6.67293928736435,-1.12435326617099,
74.6440454168485));
#201689=CARTESIAN_POINT('Ctrl Pts',(6.70384625887597,-0.940923066198626,
74.6527953310259));
#201690=CARTESIAN_POINT('Ctrl Pts',(6.7271855458891,-0.756217898710915,
74.6615452452034));
#201691=CARTESIAN_POINT('Ctrl Pts',(6.74287786822208,-0.570865180441881,
74.6702951593809));
#201692=CARTESIAN_POINT('Ctrl Pts',(6.75856988195491,-0.385516107259511,
74.6790449014853));
#201693=CARTESIAN_POINT('Ctrl Pts',(6.76661520775807,-0.199519794411015,
74.6877946435898));
#201694=CARTESIAN_POINT('Ctrl Pts',(6.76698651789742,-0.0135080196403423,
74.6965443856943));
#201695=CARTESIAN_POINT('Ctrl Pts',(6.76735782122824,0.172500344328303,
74.7052939673593));
#201696=CARTESIAN_POINT('Ctrl Pts',(6.76005538990864,0.358523883025376,
74.7140435490242));
#201697=CARTESIAN_POINT('Ctrl Pts',(6.74510402735808,0.543930749377023,
74.7227931306892));
#201698=CARTESIAN_POINT('Ctrl Pts',(6.73015291909244,0.729334462426012,
74.7315425635459));
#201699=CARTESIAN_POINT('Ctrl Pts',(6.70755316295583,0.914121238442667,
74.7402919964026));
#201700=CARTESIAN_POINT('Ctrl Pts',(6.67738151861353,1.0976634524655,74.7490414292593));
#201701=CARTESIAN_POINT('Ctrl Pts',(6.64721034732138,1.28120278879723,74.7577907249368));
#201702=CARTESIAN_POINT('Ctrl Pts',(6.60946757187517,1.46349731939927,74.7665400206143));
#201703=CARTESIAN_POINT('Ctrl Pts',(6.56428138091727,1.64392790357209,74.7752893162918));
#201704=CARTESIAN_POINT('Ctrl Pts',(6.51909583837885,1.82435589857543,74.7840384864174));
#201705=CARTESIAN_POINT('Ctrl Pts',(6.46646716368766,2.00291972270102,74.792787656543));
#201706=CARTESIAN_POINT('Ctrl Pts',(6.4065740984666,2.17901292351763,74.8015368266686));
#201707=CARTESIAN_POINT('Ctrl Pts',(6.34668181313732,2.3551038313536,74.8102858828677));
#201708=CARTESIAN_POINT('Ctrl Pts',(6.27952541883615,2.52872390898159,74.8190349390668));
#201709=CARTESIAN_POINT('Ctrl Pts',(6.20533299143027,2.69928350964975,74.8277839952659));
#201710=CARTESIAN_POINT('Ctrl Pts',(6.1283160295828,2.87633638036279,74.8368661314225));
#201711=CARTESIAN_POINT('Ctrl Pts',(6.04371690571527,3.05009086668109,74.8459482675791));
#201712=CARTESIAN_POINT('Ctrl Pts',(5.95184520282711,3.21991112945433,74.8550304037357));
#201713=CARTESIAN_POINT('Ctrl Pts',(5.8633354947363,3.38351691244787,74.8637801840793));
#201714=CARTESIAN_POINT('Ctrl Pts',(5.76807618062037,3.54347103772773,74.8725299644229));
#201715=CARTESIAN_POINT('Ctrl Pts',(5.66639083270042,3.69923018087395,74.8812797447664));
#201716=CARTESIAN_POINT('Ctrl Pts',(5.56470914041585,3.85498372440678,74.8900292105513));
#201717=CARTESIAN_POINT('Ctrl Pts',(5.45660203329856,4.00654234759486,74.8987786763363));
#201718=CARTESIAN_POINT('Ctrl Pts',(5.34243669795458,4.15339128042954,74.9075281421212));
#201719=CARTESIAN_POINT('Ctrl Pts',(5.22827486005289,4.30023571456359,74.9162773398672));
#201720=CARTESIAN_POINT('Ctrl Pts',(5.10805534120313,4.4423705208228,74.9250265376132));
#201721=CARTESIAN_POINT('Ctrl Pts',(4.98218644291713,4.57931296681202,74.9337757353592));
#201722=CARTESIAN_POINT('Ctrl Pts',(4.85632073169895,4.71625194534528,74.9425247115708));
#201723=CARTESIAN_POINT('Ctrl Pts',(4.72480612119228,4.84799861574302,74.9512736877825));
#201724=CARTESIAN_POINT('Ctrl Pts',(4.58808925182879,4.97410554946848,74.9600226639941));
#201725=CARTESIAN_POINT('Ctrl Pts',(4.45136349420285,5.1002206816813,74.9687722089958));
#201726=CARTESIAN_POINT('Ctrl Pts',(4.30943501155045,5.22069514917263,74.9775217539975));
#201727=CARTESIAN_POINT('Ctrl Pts',(4.16278587375539,5.33511975210141,74.9862712989992));
#201728=CARTESIAN_POINT('Ctrl Pts',(4.01614535682984,5.44953762850192,74.995020329653));
#201729=CARTESIAN_POINT('Ctrl Pts',(3.86478496599301,5.55790617573548,75.0037693603067));
#201730=CARTESIAN_POINT('Ctrl Pts',(3.70921874687482,5.6598573557849,75.0125183909605));
#201731=CARTESIAN_POINT('Ctrl Pts',(3.5536504154511,5.76180992014539,75.0212675404101));
#201732=CARTESIAN_POINT('Ctrl Pts',(3.39387638112723,5.85734478588621,75.0300166898597));
#201733=CARTESIAN_POINT('Ctrl Pts',(3.23043927841802,5.94613749155316,75.0387658393093));
#201734=CARTESIAN_POINT('Ctrl Pts',(3.18691767028355,5.96978206966411,75.0410956472143));
#201735=CARTESIAN_POINT('Ctrl Pts',(3.14313645898471,5.99294880644326,75.0434254551192));
#201736=CARTESIAN_POINT('Ctrl Pts',(3.09910619832135,6.0156321173694,75.0457552630242));
#201737=CARTESIAN_POINT('Ctrl Pts',(3.09910619832135,6.0156321173694,73.0457552630242));
#201738=CARTESIAN_POINT('Ctrl Pts',(2.93375330764824,6.10081787314654,73.0545047109265));
#201739=CARTESIAN_POINT('Ctrl Pts',(2.76488627843065,6.17918207037041,73.0632541588288));
#201740=CARTESIAN_POINT('Ctrl Pts',(2.59307866646694,6.25045854554,73.0720036067311));
#201741=CARTESIAN_POINT('Ctrl Pts',(2.4212724418536,6.32173444515043,73.0807529839814));
#201742=CARTESIAN_POINT('Ctrl Pts',(2.2465259467244,6.38592262741847,73.0895023612317));
#201743=CARTESIAN_POINT('Ctrl Pts',(2.06943269687088,6.44280508110572,73.098251738482));
#201744=CARTESIAN_POINT('Ctrl Pts',(1.89234081822042,6.49968709436177,73.1070010479874));
#201745=CARTESIAN_POINT('Ctrl Pts',(1.7129024940555,6.54926340459555,73.1157503574927));
#201746=CARTESIAN_POINT('Ctrl Pts',(1.53172716625018,6.59136563150393,73.1244996669981));
#201747=CARTESIAN_POINT('Ctrl Pts',(1.35055318107301,6.63346754640716,73.1332489116653));
#201748=CARTESIAN_POINT('Ctrl Pts',(1.16764249714394,6.6680954239578,73.1419981563326));
#201749=CARTESIAN_POINT('Ctrl Pts',(0.983616340614181,6.69513165624671,
73.1507474009998));
#201750=CARTESIAN_POINT('Ctrl Pts',(0.799591486713637,6.72216769715963,
73.1594965837355));
#201751=CARTESIAN_POINT('Ctrl Pts',(0.614451459526477,6.74161215869373,
73.1682457664712));
#201752=CARTESIAN_POINT('Ctrl Pts',(0.428825047910017,6.75339900185714,
73.1769949492069));
#201753=CARTESIAN_POINT('Ctrl Pts',(0.243199888596786,6.76518576550222,
73.1857440729174));
#201754=CARTESIAN_POINT('Ctrl Pts',(0.0570886373916655,6.76931499599834,
73.194493196628));
#201755=CARTESIAN_POINT('Ctrl Pts',(-0.128876626811394,6.76577266947846,
73.2032423203385));
#201756=CARTESIAN_POINT('Ctrl Pts',(-0.314840698188439,6.76223036567992,
73.21199138793));
#201757=CARTESIAN_POINT('Ctrl Pts',(-0.500658497951567,6.75101660879221,
73.2207404555216));
#201758=CARTESIAN_POINT('Ctrl Pts',(-0.685698951926566,6.73216948296215,
73.2294895231131));
#201759=CARTESIAN_POINT('Ctrl Pts',(-0.870738280460138,6.71332247176289,
73.2382385374917));
#201760=CARTESIAN_POINT('Ctrl Pts',(-1.05499998761273,6.68684221356183,
73.2469875518702));
#201761=CARTESIAN_POINT('Ctrl Pts',(-1.23785829161436,6.65281863948519,
73.2557365662487));
#201762=CARTESIAN_POINT('Ctrl Pts',(-1.43007412917419,6.61705395368858,
73.2649332999479));
#201763=CARTESIAN_POINT('Ctrl Pts',(-1.62073882535806,6.57295372727786,
73.2741300336471));
#201764=CARTESIAN_POINT('Ctrl Pts',(-1.80913696091527,6.52068343478276,
73.2833267673463));
#201765=CARTESIAN_POINT('Ctrl Pts',(-1.98838356186122,6.47095219815195,
73.2920767650599));
#201766=CARTESIAN_POINT('Ctrl Pts',(-2.1655782757254,6.41382586850888,73.3008267627736));
#201767=CARTESIAN_POINT('Ctrl Pts',(-2.34011918621703,6.34949849943277,
73.3095767604873));
#201768=CARTESIAN_POINT('Ctrl Pts',(-2.51465655691098,6.28517243495551,
73.3183265807456));
#201769=CARTESIAN_POINT('Ctrl Pts',(-2.68653996295324,6.21364572242376,
73.3270764010039));
#201770=CARTESIAN_POINT('Ctrl Pts',(-2.85518555379981,6.13516132252225,
73.3358262212622));
#201771=CARTESIAN_POINT('Ctrl Pts',(-3.02382794858674,6.05667841000514,
73.3445758756997));
#201772=CARTESIAN_POINT('Ctrl Pts',(-3.18923239109259,5.97123819492092,
73.3533255301372));
#201773=CARTESIAN_POINT('Ctrl Pts',(-3.3508370596767,5.87913088810729,73.3620751845747));
#201774=CARTESIAN_POINT('Ctrl Pts',(-3.51243888042375,5.78702520443118,
73.3708246848237));
#201775=CARTESIAN_POINT('Ctrl Pts',(-3.67024081223669,5.68825280605797,
73.3795741850726));
#201776=CARTESIAN_POINT('Ctrl Pts',(-3.82370687544384,5.58314917682516,
73.3883236853215));
#201777=CARTESIAN_POINT('Ctrl Pts',(-3.97717043817797,5.47804726008034,
73.397073043012));
#201778=CARTESIAN_POINT('Ctrl Pts',(-4.12629803722442,5.3666144808425,73.4058224007025));
#201779=CARTESIAN_POINT('Ctrl Pts',(-4.27058317206889,5.24922931204591,
73.4145717583929));
#201780=CARTESIAN_POINT('Ctrl Pts',(-4.41486614774828,5.13184589986797,
73.423320985153));
#201781=CARTESIAN_POINT('Ctrl Pts',(-4.55430658194418,5.00851045723032,
73.4320702119131));
#201782=CARTESIAN_POINT('Ctrl Pts',(-4.68843089001859,4.87964187103106,
73.4408194386732));
#201783=CARTESIAN_POINT('Ctrl Pts',(-4.82255336917864,4.75077504207933,
73.4495685461291));
#201784=CARTESIAN_POINT('Ctrl Pts',(-4.95135966065174,4.61637541908051,
73.458317653585));
#201785=CARTESIAN_POINT('Ctrl Pts',(-5.07441230869295,4.47689945401787,
73.467066761041));
#201786=CARTESIAN_POINT('Ctrl Pts',(-5.19746344226441,4.33742520555486,
73.4758157608173));
#201787=CARTESIAN_POINT('Ctrl Pts',(-5.31476088454766,4.19287495491336,
73.4845647605937));
#201788=CARTESIAN_POINT('Ctrl Pts',(-5.4259062762883,4.04373961586738,73.49331376037));
#201789=CARTESIAN_POINT('Ctrl Pts',(-5.53706380672648,3.89458798906763,
73.5020637156647));
#201790=CARTESIAN_POINT('Ctrl Pts',(-5.64206777071848,3.74085050155308,
73.5108136709594));
#201791=CARTESIAN_POINT('Ctrl Pts',(-5.74056148163995,3.58304938223181,
73.5195636262541));
#201792=CARTESIAN_POINT('Ctrl Pts',(-5.83905138951866,3.42525435593311,
73.5283132436952));
#201793=CARTESIAN_POINT('Ctrl Pts',(-5.93103139557631,3.26339625497221,
73.5370628611363));
#201794=CARTESIAN_POINT('Ctrl Pts',(-6.01618907820822,3.09802485065052,
73.5458124785774));
#201795=CARTESIAN_POINT('Ctrl Pts',(-6.1013439254495,2.93265895249708,73.5545618046933));
#201796=CARTESIAN_POINT('Ctrl Pts',(-6.17967677261792,2.76378023986123,
73.5633111308091));
#201797=CARTESIAN_POINT('Ctrl Pts',(-6.25092157009179,2.59196229227226,
73.572060456925));
#201798=CARTESIAN_POINT('Ctrl Pts',(-6.32216437407704,2.42014915229219,
73.5808095382274));
#201799=CARTESIAN_POINT('Ctrl Pts',(-6.3863194154887,2.24539720662996,73.5895586195299));
#201800=CARTESIAN_POINT('Ctrl Pts',(-6.44316881037485,2.0682999494785,73.5983077008324));
#201801=CARTESIAN_POINT('Ctrl Pts',(-6.50002334524525,1.89118668024612,
73.6070575731747));
#201802=CARTESIAN_POINT('Ctrl Pts',(-6.54957082411054,1.71172794807862,
73.615807445517));
#201803=CARTESIAN_POINT('Ctrl Pts',(-6.59164294296047,1.53053334250498,
73.6245573178594));
#201804=CARTESIAN_POINT('Ctrl Pts',(-6.633712140821,1.34935131693767,73.6333065827143));
#201805=CARTESIAN_POINT('Ctrl Pts',(-6.66830695239659,1.1664339382994,73.6420558475692));
#201806=CARTESIAN_POINT('Ctrl Pts',(-6.69530988153961,0.982402458342849,
73.6508051124241));
#201807=CARTESIAN_POINT('Ctrl Pts',(-6.7223141969046,0.798361530948973,
73.6595548264311));
#201808=CARTESIAN_POINT('Ctrl Pts',(-6.7417258082926,0.613206671364441,
73.6683045404382));
#201809=CARTESIAN_POINT('Ctrl Pts',(-6.75347878028167,0.427566795115414,
73.6770542544452));
#201810=CARTESIAN_POINT('Ctrl Pts',(-6.76248992368209,0.285234494206924,
73.6837627642335));
#201811=CARTESIAN_POINT('Ctrl Pts',(-6.76699999999995,0.142617266093417,
73.6904712740217));
#201812=CARTESIAN_POINT('Ctrl Pts',(-6.767,2.35809769017265E-12,73.69717978381));
#201813=CARTESIAN_POINT('',(-6.767,2.50669764893102E-12,73.3028202161898));
#201814=CARTESIAN_POINT('Ctrl Pts',(3.09910619832134,6.0156321173694,72.6513713193949));
#201815=CARTESIAN_POINT('Ctrl Pts',(2.93988645429697,6.09765822634244,72.6597884001077));
#201816=CARTESIAN_POINT('Ctrl Pts',(2.77738341495137,6.17337193593024,72.6682054808205));
#201817=CARTESIAN_POINT('Ctrl Pts',(2.61212887414432,6.24252126507083,72.6766225615333));
#201818=CARTESIAN_POINT('Ctrl Pts',(2.44706009708545,6.31159286298236,72.6850301805487));
#201819=CARTESIAN_POINT('Ctrl Pts',(2.27924631418403,6.37411470828925,72.6934377995641));
#201820=CARTESIAN_POINT('Ctrl Pts',(2.10923781216841,6.42988373547446,72.7018454185794));
#201821=CARTESIAN_POINT('Ctrl Pts',(1.9392079965238,6.4856597543121,72.7102540916413));
#201822=CARTESIAN_POINT('Ctrl Pts',(1.7669832318752,6.53468116261311,72.7186627647033));
#201823=CARTESIAN_POINT('Ctrl Pts',(1.59312956559307,6.57679459822437,72.7270714377652));
#201824=CARTESIAN_POINT('Ctrl Pts',(1.41922918817829,6.6189193489049,72.7354823700756));
#201825=CARTESIAN_POINT('Ctrl Pts',(1.24369936248274,6.65413234769309,72.7438933023861));
#201826=CARTESIAN_POINT('Ctrl Pts',(1.06711727979176,6.68233115844836,72.7523042346965));
#201827=CARTESIAN_POINT('Ctrl Pts',(0.89028005608688,6.71057071327607,72.760727319847));
#201828=CARTESIAN_POINT('Ctrl Pts',(0.712387866442494,6.73177575353592,
72.7691504049975));
#201829=CARTESIAN_POINT('Ctrl Pts',(0.534026146759807,6.74589542422478,
72.7775734901479));
#201830=CARTESIAN_POINT('Ctrl Pts',(0.355678451507069,6.76001398469599,
72.7859959129984));
#201831=CARTESIAN_POINT('Ctrl Pts',(0.176861636599639,6.76704829543591,
72.7944183358488));
#201832=CARTESIAN_POINT('Ctrl Pts',(-0.00183830437997168,6.76699975030567,
72.8028407586993));
#201833=CARTESIAN_POINT('Ctrl Pts',(-0.180763637529803,6.76695114394602,
72.8112738046543));
#201834=CARTESIAN_POINT('Ctrl Pts',(-0.359571466234763,6.75980183235657,
72.8197068506094));
#201835=CARTESIAN_POINT('Ctrl Pts',(-0.537677928093749,6.74560534315793,
72.8281398965644));
#201836=CARTESIAN_POINT('Ctrl Pts',(-0.715377632129388,6.73144127576468,
72.8365536832103));
#201837=CARTESIAN_POINT('Ctrl Pts',(-0.892378847347759,6.71026227561055,
72.8449674698562));
#201838=CARTESIAN_POINT('Ctrl Pts',(-1.06811095478611,6.68217240036995,
72.853381256502));
#201839=CARTESIAN_POINT('Ctrl Pts',(-1.24105052271581,6.65452889823411,
72.8616613405937));
#201840=CARTESIAN_POINT('Ctrl Pts',(-1.41315275857235,6.6201296392588,72.8699414246853));
#201841=CARTESIAN_POINT('Ctrl Pts',(-1.58385521493082,6.57903424965522,
72.878221508777));
#201842=CARTESIAN_POINT('Ctrl Pts',(-1.75435970041444,6.53798652011703,
72.8864919901041));
#201843=CARTESIAN_POINT('Ctrl Pts',(-1.92346730065479,6.49025820684884,
72.8947624714312));
#201844=CARTESIAN_POINT('Ctrl Pts',(-2.09062233285272,6.43596047699001,
72.9030329527583));
#201845=CARTESIAN_POINT('Ctrl Pts',(-2.25761228179066,6.38171637187784,
72.911295266111));
#201846=CARTESIAN_POINT('Ctrl Pts',(-2.42265317135319,6.32091588086906,
72.9195575794638));
#201847=CARTESIAN_POINT('Ctrl Pts',(-2.58520099042713,6.25372087953201,
72.9278198928165));
#201848=CARTESIAN_POINT('Ctrl Pts',(-2.74758855745376,6.18659212415626,
72.9360740605501));
#201849=CARTESIAN_POINT('Ctrl Pts',(-2.9074876300941,6.11308155919282,72.9443282282837));
#201850=CARTESIAN_POINT('Ctrl Pts',(-3.06437093980389,6.03340034667727,
72.9525823960172));
#201851=CARTESIAN_POINT('Ctrl Pts',(-3.22116441104271,5.95376476322394,
72.9608318370414));
#201852=CARTESIAN_POINT('Ctrl Pts',(-3.37494524653128,5.86796572892841,
72.9690812780657));
#201853=CARTESIAN_POINT('Ctrl Pts',(-3.52520718160036,5.7762620548927,72.9773307190899));
#201854=CARTESIAN_POINT('Ctrl Pts',(-3.67540325881703,5.68459857338498,
72.9855765444914));
#201855=CARTESIAN_POINT('Ctrl Pts',(-3.82208320952256,5.58703579223704,
72.9938223698928));
#201856=CARTESIAN_POINT('Ctrl Pts',(-3.96476629094543,5.48387793975968,
73.0020681952943));
#201857=CARTESIAN_POINT('Ctrl Pts',(-4.02398769717215,5.44106169955715,
73.0054906709719));
#201858=CARTESIAN_POINT('Ctrl Pts',(-4.08252088026485,5.39728211963936,
73.0089131466495));
#201859=CARTESIAN_POINT('Ctrl Pts',(-4.14033291405278,5.35256315804038,
73.0123356223271));
#201860=CARTESIAN_POINT('Ctrl Pts',(-4.28903258164251,5.23754048388367,
73.0211386510782));
#201861=CARTESIAN_POINT('Ctrl Pts',(-4.43279665683033,5.11642600515404,
73.0299416798293));
#201862=CARTESIAN_POINT('Ctrl Pts',(-4.57116043698929,4.98966744977097,
73.0387447085803));
#201863=CARTESIAN_POINT('Ctrl Pts',(-4.70976229709573,4.86269078333185,
73.047562884537));
#201864=CARTESIAN_POINT('Ctrl Pts',(-4.84294509763682,4.73005081790123,
73.0563810604937));
#201865=CARTESIAN_POINT('Ctrl Pts',(-4.97028196065051,4.59223107341433,
73.0651992364503));
#201866=CARTESIAN_POINT('Ctrl Pts',(-5.09796456485835,4.45403712493097,
73.0740413552513));
#201867=CARTESIAN_POINT('Ctrl Pts',(-5.21976928819236,4.31063545580153,
73.0828834740522));
#201868=CARTESIAN_POINT('Ctrl Pts',(-5.33530858817898,4.16254384588362,
73.0917255928532));
#201869=CARTESIAN_POINT('Ctrl Pts',(-5.45099905431521,4.01425847991506,
73.1005792802638));
#201870=CARTESIAN_POINT('Ctrl Pts',(-5.56040756458574,3.86127113423292,
73.1094329676743));
#201871=CARTESIAN_POINT('Ctrl Pts',(-5.66319003382627,3.70412845899961,
73.1182866550849));
#201872=CARTESIAN_POINT('Ctrl Pts',(-5.76620337901913,3.54663280076187,
73.1271602301623));
#201873=CARTESIAN_POINT('Ctrl Pts',(-5.86256076602242,3.38496337047203,
73.1360338052398));
#201874=CARTESIAN_POINT('Ctrl Pts',(-5.95196277818806,3.21969378777918,
73.1449073803172));
#201875=CARTESIAN_POINT('Ctrl Pts',(-6.04056510611099,3.055902510528,73.1537015829288));
#201876=CARTESIAN_POINT('Ctrl Pts',(-6.12233592568479,2.88857547846388,
73.1624957855403));
#201877=CARTESIAN_POINT('Ctrl Pts',(-6.19703066141498,2.71828990019141,
73.1712899881518));
#201878=CARTESIAN_POINT('Ctrl Pts',(-6.27195892853884,2.54747192792858,
73.1801116856379));
#201879=CARTESIAN_POINT('Ctrl Pts',(-6.33989644591468,2.37338102034605,
73.1889333831241));
#201880=CARTESIAN_POINT('Ctrl Pts',(-6.40056814536355,2.19659200047652,
73.1977550806102));
#201881=CARTESIAN_POINT('Ctrl Pts',(-6.46106297879402,2.02031834395308,
73.2065510616828));
#201882=CARTESIAN_POINT('Ctrl Pts',(-6.51433416114382,1.84136252602717,
73.2153470427554));
#201883=CARTESIAN_POINT('Ctrl Pts',(-6.56015486384009,1.66031839188609,
73.2241430238281));
#201884=CARTESIAN_POINT('Ctrl Pts',(-6.60589579977616,1.47958942759585,
73.2329236924574));
#201885=CARTESIAN_POINT('Ctrl Pts',(-6.64421205068951,1.29677966067728,
73.2417043610867));
#201886=CARTESIAN_POINT('Ctrl Pts',(-6.67492564861701,1.11250015075723,
73.250485029716));
#201887=CARTESIAN_POINT('Ctrl Pts',(-6.70555455524957,0.928728782877719,
73.2592414860665));
#201888=CARTESIAN_POINT('Ctrl Pts',(-6.72862258426218,0.74349602688161,
73.267997942417));
#201889=CARTESIAN_POINT('Ctrl Pts',(-6.74400230942963,0.557424300159112,
73.2767543987675));
#201890=CARTESIAN_POINT('Ctrl Pts',(-6.75926286279254,0.372794374457539,
73.2854430045749));
#201891=CARTESIAN_POINT('Ctrl Pts',(-6.76695376716036,0.187338701658777,
73.2941316103824));
#201892=CARTESIAN_POINT('Ctrl Pts',(-6.76699979207347,0.00167752126097696,
73.3028202161898));
#201893=CARTESIAN_POINT('Ctrl Pts',(-6.767,2.50669783734745E-12,73.3028202161898));
#201894=CARTESIAN_POINT('Ctrl Pts',(-6.76700000000007,-0.18600724952452,
73.311569728001));
#201895=CARTESIAN_POINT('Ctrl Pts',(-6.75932637294533,-0.372014355747722,
73.3203192398122));
#201896=CARTESIAN_POINT('Ctrl Pts',(-6.74400518264197,-0.557389537485457,
73.3290687516234));
#201897=CARTESIAN_POINT('Ctrl Pts',(-6.72868405705108,-0.742763936249799,
73.337818226479));
#201898=CARTESIAN_POINT('Ctrl Pts',(-6.70571545645752,-0.927506130240312,
73.3465677013347));
#201899=CARTESIAN_POINT('Ctrl Pts',(-6.67517739404833,-1.1109886398997,
73.3553171761904));
#201900=CARTESIAN_POINT('Ctrl Pts',(-6.64463945808708,-1.29447038981914,
73.3640666148174));
#201901=CARTESIAN_POINT('Ctrl Pts',(-6.60653217008359,-1.47669218313665,
73.3728160534444));
#201902=CARTESIAN_POINT('Ctrl Pts',(-6.56098496092678,-1.65703510599281,
73.3815654920714));
#201903=CARTESIAN_POINT('Ctrl Pts',(-6.51543793658299,-1.8373772970869,
73.3903148951966));
#201904=CARTESIAN_POINT('Ctrl Pts',(-6.46245112167425,-2.01584035510912,
73.3990642983218));
#201905=CARTESIAN_POINT('Ctrl Pts',(-6.4022044837426,-2.19181813760772,
73.4078137014469));
#201906=CARTESIAN_POINT('Ctrl Pts',(-6.34195808526509,-2.3677952206713,
73.416563069797));
#201907=CARTESIAN_POINT('Ctrl Pts',(-6.27445201433107,-2.54128677684158,
73.4253124381471));
#201908=CARTESIAN_POINT('Ctrl Pts',(-6.19991555071903,-2.71170355384809,
73.4340618064972));
#201909=CARTESIAN_POINT('Ctrl Pts',(-6.12537937716695,-2.88211966767471,
73.442811140799));
#201910=CARTESIAN_POINT('Ctrl Pts',(-6.04381298052524,-3.04946076371776,
73.4515604751008));
#201911=CARTESIAN_POINT('Ctrl Pts',(-5.95549339335838,-3.21315848374535,
73.4603098094026));
#201912=CARTESIAN_POINT('Ctrl Pts',(-5.86717414255423,-3.37685558033468,
73.4690591103828));
#201913=CARTESIAN_POINT('Ctrl Pts',(-5.7721018887662,-3.5369090764672,73.4778084113629));
#201914=CARTESIAN_POINT('Ctrl Pts',(-5.67059953347026,-3.6927753696924,
73.4865577123431));
#201915=CARTESIAN_POINT('Ctrl Pts',(-5.56909755631424,-3.84864108224864,
73.4953069807284));
#201916=CARTESIAN_POINT('Ctrl Pts',(-5.46116568196902,-4.00031938297446,
73.5040562491137));
#201917=CARTESIAN_POINT('Ctrl Pts',(-5.34717048533667,-4.14729511859772,
73.5128055174989));
#201918=CARTESIAN_POINT('Ctrl Pts',(-5.23317570391897,-4.29427031887843,
73.521554754016));
#201919=CARTESIAN_POINT('Ctrl Pts',(-5.11311782003571,-4.43654276189482,
73.530303990533));
#201920=CARTESIAN_POINT('Ctrl Pts',(-4.98740458984806,-4.57362924351795,
73.5390532270501));
#201921=CARTESIAN_POINT('Ctrl Pts',(-4.86169180711799,-4.71071523720209,
73.5478024324255));
#201922=CARTESIAN_POINT('Ctrl Pts',(-4.73032391204231,-4.84261509523179,
73.556551637801));
#201923=CARTESIAN_POINT('Ctrl Pts',(-4.59374707013663,-4.96888084538271,
73.5653008431764));
#201924=CARTESIAN_POINT('Ctrl Pts',(-4.45717070301521,-5.09514615659397,
73.5740500181368));
#201925=CARTESIAN_POINT('Ctrl Pts',(-4.3153856357113,-5.21577720459453,
73.5827991930973));
#201926=CARTESIAN_POINT('Ctrl Pts',(-4.16887341029612,-5.33036429232806,
73.5915483680577));
#201927=CARTESIAN_POINT('Ctrl Pts',(-4.0223616820382,-5.44495099123531,
73.6002975133297));
#201928=CARTESIAN_POINT('Ctrl Pts',(-3.87112305348291,-5.55349359438513,
73.6090466586018));
#201929=CARTESIAN_POINT('Ctrl Pts',(-3.71567117017898,-5.65562346298803,
73.6177958038738));
#201930=CARTESIAN_POINT('Ctrl Pts',(-3.56021980145966,-5.75775299351553,
73.6265449201839));
#201931=CARTESIAN_POINT('Ctrl Pts',(-3.40055544538506,-5.85346967463782,
73.6352940364941));
#201932=CARTESIAN_POINT('Ctrl Pts',(-3.23722035987019,-5.94244842986811,
73.6440431528043));
#201933=CARTESIAN_POINT('Ctrl Pts',(-3.07388580147368,-6.03142689794433,
73.6527922408791));
#201934=CARTESIAN_POINT('Ctrl Pts',(-2.90688078896788,-6.11366734656681,
73.6615413289539));
#201935=CARTESIAN_POINT('Ctrl Pts',(-2.73677250721603,-6.18889046952251,
73.6702904170288));
#201936=CARTESIAN_POINT('Ctrl Pts',(-2.5666647603171,-6.26411335596234,
73.6790394775948));
#201937=CARTESIAN_POINT('Ctrl Pts',(-2.39345402575388,-6.33231884500472,
73.6877885381608));
#201938=CARTESIAN_POINT('Ctrl Pts',(-2.21772856065808,-6.39327529762652,
73.6965375987268));
#201939=CARTESIAN_POINT('Ctrl Pts',(-2.04200363348718,-6.45423156365047,
73.7052866325105));
#201940=CARTESIAN_POINT('Ctrl Pts',(-1.86376426189471,-6.50793874375603,
73.7140356662942));
#201941=CARTESIAN_POINT('Ctrl Pts',(-1.68361577753334,-6.55421443909496,
73.7227847000779));
#201942=CARTESIAN_POINT('Ctrl Pts',(-1.50346782968002,-6.60048999661821,
73.7315337078058));
#201943=CARTESIAN_POINT('Ctrl Pts',(-1.32141105795213,-6.63933404237667,
73.7402827155336));
#201944=CARTESIAN_POINT('Ctrl Pts',(-1.13806375487272,-6.67061465607518,
73.7490317232614));
#201945=CARTESIAN_POINT('Ctrl Pts',(-0.954716982605621,-6.70189517921259,
73.7577807056598));
#201946=CARTESIAN_POINT('Ctrl Pts',(-0.770079968904851,-6.72561226592197,
73.7665296880582));
#201947=CARTESIAN_POINT('Ctrl Pts',(-0.584779765561063,-6.74168536983078,
73.7752786704566));
#201948=CARTESIAN_POINT('Ctrl Pts',(-0.391489830654086,-6.75845151013837,
73.7844048894665));
#201949=CARTESIAN_POINT('Ctrl Pts',(-0.197478578241089,-6.76689983031617,
73.7935311084764));
#201950=CARTESIAN_POINT('Ctrl Pts',(-0.00346287645406101,-6.76699911397118,
73.8026573274862));
#201951=CARTESIAN_POINT('Ctrl Pts',(0.184489834652092,-6.76709529501196,
73.811498352152));
#201952=CARTESIAN_POINT('Ctrl Pts',(0.372446404247607,-6.75935639738178,
73.8203393768178));
#201953=CARTESIAN_POINT('Ctrl Pts',(0.559755019486604,-6.74380925873201,
73.8291804014837));
#201954=CARTESIAN_POINT('Ctrl Pts',(0.745134705520065,-6.72842222659825,
73.8379303800934));
#201955=CARTESIAN_POINT('Ctrl Pts',(0.92987943122688,-6.70538706057547,
73.8466803587031));
#201956=CARTESIAN_POINT('Ctrl Pts',(1.11336163626659,-6.67478200894155,
73.8554303373129));
#201957=CARTESIAN_POINT('Ctrl Pts',(1.2968419630057,-6.64417727061042,73.8641802263494));
#201958=CARTESIAN_POINT('Ctrl Pts',(1.47905951217378,-6.6060028489062,73.872930115386));
#201959=CARTESIAN_POINT('Ctrl Pts',(1.65939532066969,-6.5603884160726,73.8816800044225));
#201960=CARTESIAN_POINT('Ctrl Pts',(1.83972934300687,-6.51477443503289,
73.8904298067946));
#201961=CARTESIAN_POINT('Ctrl Pts',(2.0181813840615,-6.46172066062177,73.8991796091668));
#201962=CARTESIAN_POINT('Ctrl Pts',(2.19414528354085,-6.40140730423517,
73.907929411539));
#201963=CARTESIAN_POINT('Ctrl Pts',(2.37010749863886,-6.34109452518685,
73.9166791301553));
#201964=CARTESIAN_POINT('Ctrl Pts',(2.54358134866346,-6.2735223961655,73.9254288487716));
#201965=CARTESIAN_POINT('Ctrl Pts',(2.71397759435442,-6.19892043966869,
73.9341785673879));
#201966=CARTESIAN_POINT('Ctrl Pts',(2.88437226558005,-6.12431917249571,
73.9429282051566));
#201967=CARTESIAN_POINT('Ctrl Pts',(3.05168912680833,-6.0426883227886,73.9516778429253));
#201968=CARTESIAN_POINT('Ctrl Pts',(3.21535986273728,-5.95430516123402,
73.960427480694));
#201969=CARTESIAN_POINT('Ctrl Pts',(3.37902914072727,-5.86592278697507,
73.9691770405231));
#201970=CARTESIAN_POINT('Ctrl Pts',(3.5390521062147,-5.77078835742004,73.9779266003522));
#201971=CARTESIAN_POINT('Ctrl Pts',(3.69488522831607,-5.66922500431688,
73.9866761601812));
#201972=CARTESIAN_POINT('Ctrl Pts',(3.85071701406866,-5.56766252217145,
73.9954256449784));
#201973=CARTESIAN_POINT('Ctrl Pts',(4.00235878822346,-5.45967138329413,
74.0041751297755));
#201974=CARTESIAN_POINT('Ctrl Pts',(4.14929549611283,-5.3456183819964,74.0129246145726));
#201975=CARTESIAN_POINT('Ctrl Pts',(4.29623099276058,-5.23156632087042,
74.0216740272452));
#201976=CARTESIAN_POINT('Ctrl Pts',(4.43846127436007,-5.11145267304983,
74.0304234399178));
#201977=CARTESIAN_POINT('Ctrl Pts',(4.57550326054431,-4.98568540049895,
74.0391728525904));
#201978=CARTESIAN_POINT('Ctrl Pts',(4.71254416257766,-4.85991912290374,
74.0479221960457));
#201979=CARTESIAN_POINT('Ctrl Pts',(4.84439664018744,-4.72849950385436,
74.0566715395009));
#201980=CARTESIAN_POINT('Ctrl Pts',(4.97061286794725,-4.59187289861089,
74.0654208829561));
#201981=CARTESIAN_POINT('Ctrl Pts',(5.09682813912663,-4.45524732884709,
74.0741701601009));
#201982=CARTESIAN_POINT('Ctrl Pts',(5.21740705147816,-4.31341506235815,
74.0829194372458));
#201983=CARTESIAN_POINT('Ctrl Pts',(5.33194007545673,-4.16685781275754,
74.0916687143906));
#201984=CARTESIAN_POINT('Ctrl Pts',(5.44647226944465,-4.02030162521869,
74.1004179281317));
#201985=CARTESIAN_POINT('Ctrl Pts',(5.55495848628096,-3.86902074887959,
74.1091671418728));
#201986=CARTESIAN_POINT('Ctrl Pts',(5.65703027291773,-3.71352898080685,
74.117916355614));
#201987=CARTESIAN_POINT('Ctrl Pts',(5.75910135376982,-3.55803828789613,
74.1266655088579));
#201988=CARTESIAN_POINT('Ctrl Pts',(5.85475793592736,-3.3983370010674,74.1354146621017));
#201989=CARTESIAN_POINT('Ctrl Pts',(5.94367514427382,-3.23496750823584,
74.1441638153456));
#201990=CARTESIAN_POINT('Ctrl Pts',(6.03259176732619,-3.07159909077765,
74.1529129109985));
#201991=CARTESIAN_POINT('Ctrl Pts',(6.114768968359,-2.90456276731484,74.1616620066515));
#201992=CARTESIAN_POINT('Ctrl Pts',(6.1899276554786,-2.73442583003109,74.1704111023044));
#201993=CARTESIAN_POINT('Ctrl Pts',(6.2650858728303,-2.5642899561623,74.1791601432724));
#201994=CARTESIAN_POINT('Ctrl Pts',(6.33322554827137,-2.39105376935261,
74.1879091842405));
#201995=CARTESIAN_POINT('Ctrl Pts',(6.3941152673301,-2.21530561054139,74.1966582252085));
#201996=CARTESIAN_POINT('Ctrl Pts',(6.45500462602821,-2.03955849185179,
74.2054072143975));
#201997=CARTESIAN_POINT('Ctrl Pts',(6.5086440204071,-1.86129970164647,74.2141562035865));
#201998=CARTESIAN_POINT('Ctrl Pts',(6.55485128368569,-1.68113463136183,
74.2229051927756));
#201999=CARTESIAN_POINT('Ctrl Pts',(6.60199809554296,-1.49730620117003,
74.231832078247));
#202000=CARTESIAN_POINT('Ctrl Pts',(6.64140720707845,-1.31149343245843,
74.2407589637184));
#202001=CARTESIAN_POINT('Ctrl Pts',(6.67293928722858,-1.1243532669768,74.2496858491898));
#202002=CARTESIAN_POINT('Ctrl Pts',(6.70384625876233,-0.940923067008231,
74.2584357633673));
#202003=CARTESIAN_POINT('Ctrl Pts',(6.72718554579776,-0.756217899523402,
74.2671856775448));
#202004=CARTESIAN_POINT('Ctrl Pts',(6.74287786815312,-0.570865181256328,
74.2759355917222));
#202005=CARTESIAN_POINT('Ctrl Pts',(6.75856988190835,-0.385516108075853,
74.2846853338267));
#202006=CARTESIAN_POINT('Ctrl Pts',(6.76661520773397,-0.199519795228328,
74.2934350759312));
#202007=CARTESIAN_POINT('Ctrl Pts',(6.76698651789579,-0.0135080204576999,
74.3021848180357));
#202008=CARTESIAN_POINT('Ctrl Pts',(6.76735782124908,0.172500343510837,
74.3109343997006));
#202009=CARTESIAN_POINT('Ctrl Pts',(6.76005538995195,0.358523882208727,
74.3196839813656));
#202010=CARTESIAN_POINT('Ctrl Pts',(6.74510402742379,0.543930748562116,
74.3284335630306));
#202011=CARTESIAN_POINT('Ctrl Pts',(6.73015291918055,0.729334461612975,
74.3371829958872));
#202012=CARTESIAN_POINT('Ctrl Pts',(6.70755316306626,0.914121237632424,
74.3459324287439));
#202013=CARTESIAN_POINT('Ctrl Pts',(6.67738151874611,1.09766345165897,74.3546818616006));
#202014=CARTESIAN_POINT('Ctrl Pts',(6.64721034747613,1.28120278799434,74.3634311572781));
#202015=CARTESIAN_POINT('Ctrl Pts',(6.60946757205194,1.46349731860093,74.3721804529556));
#202016=CARTESIAN_POINT('Ctrl Pts',(6.56428138111583,1.64392790277922,74.3809297486332));
#202017=CARTESIAN_POINT('Ctrl Pts',(6.51909583859919,1.82435589778807,74.3896789187588));
#202018=CARTESIAN_POINT('Ctrl Pts',(6.46646716392955,2.00291972192008,74.3984280888844));
#202019=CARTESIAN_POINT('Ctrl Pts',(6.40657409872973,2.17901292274399,74.40717725901));
#202020=CARTESIAN_POINT('Ctrl Pts',(6.34668181342172,2.35510383058719,74.4159263152091));
#202021=CARTESIAN_POINT('Ctrl Pts',(6.27952541914152,2.52872390822329,74.4246753714082));
#202022=CARTESIAN_POINT('Ctrl Pts',(6.20533299175623,2.69928350890041,74.4334244276073));
#202023=CARTESIAN_POINT('Ctrl Pts',(6.12831602991656,2.87633637965397,74.4425065637655));
#202024=CARTESIAN_POINT('Ctrl Pts',(6.04371690605376,3.05009086601253,74.4515886999237));
#202025=CARTESIAN_POINT('Ctrl Pts',(5.95184520316735,3.21991112882543,74.4606708360819));
#202026=CARTESIAN_POINT('Ctrl Pts',(5.86333549509379,3.38351691182837,74.4694206164255));
#202027=CARTESIAN_POINT('Ctrl Pts',(5.76807618099473,3.54347103711835,74.478170396769));
#202028=CARTESIAN_POINT('Ctrl Pts',(5.66639083309119,3.69923018027537,74.4869201771126));
#202029=CARTESIAN_POINT('Ctrl Pts',(5.56470914082305,3.85498372381899,74.4956696428975));
#202030=CARTESIAN_POINT('Ctrl Pts',(5.45660203372172,4.00654234701855,74.5044191086824));
#202031=CARTESIAN_POINT('Ctrl Pts',(5.34243669839322,4.15339127986533,74.5131685744674));
#202032=CARTESIAN_POINT('Ctrl Pts',(5.22827486050695,4.30023571401154,74.5219177722134));
#202033=CARTESIAN_POINT('Ctrl Pts',(5.10805534167212,4.44237052028354,74.5306669699594));
#202034=CARTESIAN_POINT('Ctrl Pts',(4.98218644340049,4.57931296628614,74.5394161677054));
#202035=CARTESIAN_POINT('Ctrl Pts',(4.85632073219707,4.71625194483236,74.548165143917));
#202036=CARTESIAN_POINT('Ctrl Pts',(4.72480612170463,4.84799861524367,74.5569141201287));
#202037=CARTESIAN_POINT('Ctrl Pts',(4.58808925235481,4.97410554898329,74.5656630963403));
#202038=CARTESIAN_POINT('Ctrl Pts',(4.45136349474225,5.10022068121052,74.574412641342));
#202039=CARTESIAN_POINT('Ctrl Pts',(4.30943501210264,5.22069514871682,74.5831621863437));
#202040=CARTESIAN_POINT('Ctrl Pts',(4.16278587431974,5.33511975166107,74.5919117313454));
#202041=CARTESIAN_POINT('Ctrl Pts',(4.01614535740639,5.44953762807702,74.6006607619991));
#202042=CARTESIAN_POINT('Ctrl Pts',(3.86478496658113,5.55790617532652,74.6094097926528));
#202043=CARTESIAN_POINT('Ctrl Pts',(3.70921874747383,5.65985735539233,74.6181588233066));
#202044=CARTESIAN_POINT('Ctrl Pts',(3.55365041606096,5.76180991976925,74.6269079727562));
#202045=CARTESIAN_POINT('Ctrl Pts',(3.39387638174726,5.85734478552695,74.6356571222058));
#202046=CARTESIAN_POINT('Ctrl Pts',(3.23043927904751,5.94613749121117,74.6444062716554));
#202047=CARTESIAN_POINT('Ctrl Pts',(3.1869176707057,5.96978206944073,74.6467360795716));
#202048=CARTESIAN_POINT('Ctrl Pts',(3.14313645919697,5.99294880633391,74.6490658874878));
#202049=CARTESIAN_POINT('Ctrl Pts',(3.09910619832131,6.01563211736942,74.651395695404));
#202050=CARTESIAN_POINT('Origin',(0.,0.,4.30282021618968));
#202051=CARTESIAN_POINT('',(3.09910619832125,6.01563211736945,77.0457552630242));
#202052=CARTESIAN_POINT('',(3.09910619832139,6.01563211736937,76.6513581962709));
#202053=CARTESIAN_POINT('',(3.09910619832133,6.0156321173694,4.30282021618968));
#202054=CARTESIAN_POINT('',(-6.767,6.79793587124441E-10,75.6971797837782));
#202055=CARTESIAN_POINT('Ctrl Pts',(-6.767,2.69602239337994E-12,75.69717978381));
#202056=CARTESIAN_POINT('Ctrl Pts',(-6.76700000000007,-0.186007249524269,
75.7059292956212));
#202057=CARTESIAN_POINT('Ctrl Pts',(-6.75932637294534,-0.372014355747412,
75.7146788074323));
#202058=CARTESIAN_POINT('Ctrl Pts',(-6.744005182642,-0.557389537485085,
75.7234283192435));
#202059=CARTESIAN_POINT('Ctrl Pts',(-6.72868405705111,-0.742763936249558,
75.7321777940992));
#202060=CARTESIAN_POINT('Ctrl Pts',(-6.70571545645754,-0.927506130240202,
75.7409272689549));
#202061=CARTESIAN_POINT('Ctrl Pts',(-6.67517739404833,-1.11098863989971,
75.7496767438106));
#202062=CARTESIAN_POINT('Ctrl Pts',(-6.64463945808705,-1.29447038981935,
75.7584261824376));
#202063=CARTESIAN_POINT('Ctrl Pts',(-6.60653217008351,-1.47669218313704,
75.7671756210647));
#202064=CARTESIAN_POINT('Ctrl Pts',(-6.56098496092664,-1.65703510599339,
75.7759250596917));
#202065=CARTESIAN_POINT('Ctrl Pts',(-6.5154379365828,-1.8373772970876,75.7846744628168));
#202066=CARTESIAN_POINT('Ctrl Pts',(-6.462451121674,-2.01584035510994,75.793423865942));
#202067=CARTESIAN_POINT('Ctrl Pts',(-6.40220448374228,-2.19181813760866,
75.8021732690672));
#202068=CARTESIAN_POINT('Ctrl Pts',(-6.34195808526476,-2.36779522067217,
75.8109226374173));
#202069=CARTESIAN_POINT('Ctrl Pts',(-6.27445201433075,-2.54128677684238,
75.8196720057674));
#202070=CARTESIAN_POINT('Ctrl Pts',(-6.19991555071871,-2.71170355384883,
75.8284213741175));
#202071=CARTESIAN_POINT('Ctrl Pts',(-6.12537937716666,-2.88211966767532,
75.8371707084193));
#202072=CARTESIAN_POINT('Ctrl Pts',(-6.043812980525,-3.04946076371825,75.845920042721));
#202073=CARTESIAN_POINT('Ctrl Pts',(-5.95549339335818,-3.21315848374571,
75.8546693770228));
#202074=CARTESIAN_POINT('Ctrl Pts',(-5.86717414255396,-3.37685558033516,
75.863418678003));
#202075=CARTESIAN_POINT('Ctrl Pts',(-5.77210188876585,-3.53690907646778,
75.8721679789832));
#202076=CARTESIAN_POINT('Ctrl Pts',(-5.67059953346982,-3.69277536969308,
75.8809172799633));
#202077=CARTESIAN_POINT('Ctrl Pts',(-5.56909755631364,-3.84864108224952,
75.8896665483486));
#202078=CARTESIAN_POINT('Ctrl Pts',(-5.46116568196824,-4.00031938297553,
75.8984158167339));
#202079=CARTESIAN_POINT('Ctrl Pts',(-5.3471704853357,-4.14729511859896,
75.9071650851192));
#202080=CARTESIAN_POINT('Ctrl Pts',(-5.23317570391805,-4.29427031887955,
75.9159143216363));
#202081=CARTESIAN_POINT('Ctrl Pts',(-5.11311782003484,-4.43654276189582,
75.9246635581533));
#202082=CARTESIAN_POINT('Ctrl Pts',(-4.98740458984725,-4.57362924351883,
75.9334127946703));
#202083=CARTESIAN_POINT('Ctrl Pts',(-4.86169180711724,-4.71071523720286,
75.9421620000458));
#202084=CARTESIAN_POINT('Ctrl Pts',(-4.73032391204163,-4.84261509523246,
75.9509112054212));
#202085=CARTESIAN_POINT('Ctrl Pts',(-4.59374707013602,-4.96888084538327,
75.9596604107966));
#202086=CARTESIAN_POINT('Ctrl Pts',(-4.45717070301449,-5.0951461565946,
75.9684095857571));
#202087=CARTESIAN_POINT('Ctrl Pts',(-4.31538563571046,-5.21577720459523,
75.9771587607175));
#202088=CARTESIAN_POINT('Ctrl Pts',(-4.16887341029516,-5.33036429232881,
75.985907935678));
#202089=CARTESIAN_POINT('Ctrl Pts',(-4.02236168203702,-5.44495099123619,
75.99465708095));
#202090=CARTESIAN_POINT('Ctrl Pts',(-3.8711230534815,-5.55349359438613,
76.003406226222));
#202091=CARTESIAN_POINT('Ctrl Pts',(-3.71567117017732,-5.65562346298912,
76.0121553714941));
#202092=CARTESIAN_POINT('Ctrl Pts',(-3.56021980145791,-5.75775299351661,
76.0209044878042));
#202093=CARTESIAN_POINT('Ctrl Pts',(-3.40055544538322,-5.85346967463889,
76.0296536041144));
#202094=CARTESIAN_POINT('Ctrl Pts',(-3.23722035986827,-5.94244842986915,
76.0384027204246));
#202095=CARTESIAN_POINT('Ctrl Pts',(-3.07388580147139,-6.03142689794551,
76.0471518084994));
#202096=CARTESIAN_POINT('Ctrl Pts',(-2.90688078896521,-6.11366734656809,
76.0559008965743));
#202097=CARTESIAN_POINT('Ctrl Pts',(-2.73677250721297,-6.18889046952386,
76.0646499846491));
#202098=CARTESIAN_POINT('Ctrl Pts',(-2.56666476031406,-6.26411335596358,
76.0733990452152));
#202099=CARTESIAN_POINT('Ctrl Pts',(-2.39345402575087,-6.33231884500586,
76.0821481057812));
#202100=CARTESIAN_POINT('Ctrl Pts',(-2.2177285606551,-6.39327529762755,
76.0908971663472));
#202101=CARTESIAN_POINT('Ctrl Pts',(-2.04200363348435,-6.45423156365136,
76.0996462001309));
#202102=CARTESIAN_POINT('Ctrl Pts',(-1.86376426189204,-6.5079387437568,
76.1083952339146));
#202103=CARTESIAN_POINT('Ctrl Pts',(-1.68361577753084,-6.5542144390956,
76.1171442676983));
#202104=CARTESIAN_POINT('Ctrl Pts',(-1.5034678296775,-6.60048999661879,
76.1258932754261));
#202105=CARTESIAN_POINT('Ctrl Pts',(-1.32141105794959,-6.63933404237717,
76.1346422831539));
#202106=CARTESIAN_POINT('Ctrl Pts',(-1.13806375487016,-6.67061465607562,
76.1433912908817));
#202107=CARTESIAN_POINT('Ctrl Pts',(-0.954716982603054,-6.70189517921296,
76.1521402732801));
#202108=CARTESIAN_POINT('Ctrl Pts',(-0.770079968902272,-6.72561226592226,
76.1608892556785));
#202109=CARTESIAN_POINT('Ctrl Pts',(-0.584779765558476,-6.741685369831,
76.1696382380769));
#202110=CARTESIAN_POINT('Ctrl Pts',(-0.391489830651555,-6.75845151013851,
76.1787644570868));
#202111=CARTESIAN_POINT('Ctrl Pts',(-0.197478578238618,-6.76689983031624,
76.1878906760966));
#202112=CARTESIAN_POINT('Ctrl Pts',(-0.00346287645165238,-6.76699911397118,
76.1970168951065));
#202113=CARTESIAN_POINT('Ctrl Pts',(0.184489834654503,-6.76709529501189,
76.2058579197723));
#202114=CARTESIAN_POINT('Ctrl Pts',(0.372446404250014,-6.75935639738165,
76.2146989444381));
#202115=CARTESIAN_POINT('Ctrl Pts',(0.559755019489007,-6.74380925873181,
76.2235399691039));
#202116=CARTESIAN_POINT('Ctrl Pts',(0.745134705522528,-6.72842222659797,
76.2322899477137));
#202117=CARTESIAN_POINT('Ctrl Pts',(0.929879431229403,-6.70538706057512,
76.2410399263234));
#202118=CARTESIAN_POINT('Ctrl Pts',(1.11336163626917,-6.67478200894112,
76.2497899049332));
#202119=CARTESIAN_POINT('Ctrl Pts',(1.29684196300826,-6.64417727060992,
76.2585397939697));
#202120=CARTESIAN_POINT('Ctrl Pts',(1.47905951217633,-6.60600284890563,
76.2672896830063));
#202121=CARTESIAN_POINT('Ctrl Pts',(1.65939532067223,-6.56038841607196,
76.2760395720428));
#202122=CARTESIAN_POINT('Ctrl Pts',(1.83972934300939,-6.51477443503218,
76.284789374415));
#202123=CARTESIAN_POINT('Ctrl Pts',(2.018181384064,-6.46172066062099,76.2935391767871));
#202124=CARTESIAN_POINT('Ctrl Pts',(2.19414528354333,-6.40140730423432,
76.3022889791593));
#202125=CARTESIAN_POINT('Ctrl Pts',(2.37010749864125,-6.34109452518595,
76.3110386977756));
#202126=CARTESIAN_POINT('Ctrl Pts',(2.54358134866577,-6.27352239616456,
76.3197884163919));
#202127=CARTESIAN_POINT('Ctrl Pts',(2.71397759435665,-6.19892043966771,
76.3285381350082));
#202128=CARTESIAN_POINT('Ctrl Pts',(2.88437226558232,-6.12431917249464,
76.3372877727769));
#202129=CARTESIAN_POINT('Ctrl Pts',(3.05168912681062,-6.04268832278745,
76.3460374105456));
#202130=CARTESIAN_POINT('Ctrl Pts',(3.21535986273959,-5.95430516123277,
76.3547870483143));
#202131=CARTESIAN_POINT('Ctrl Pts',(3.37902914072956,-5.86592278697375,
76.3635366081434));
#202132=CARTESIAN_POINT('Ctrl Pts',(3.53905210621695,-5.77078835741867,
76.3722861679725));
#202133=CARTESIAN_POINT('Ctrl Pts',(3.69488522831828,-5.66922500431544,
76.3810357278016));
#202134=CARTESIAN_POINT('Ctrl Pts',(3.85071701407078,-5.56766252216998,
76.3897852125987));
#202135=CARTESIAN_POINT('Ctrl Pts',(4.00235878822549,-5.45967138329264,
76.3985346973958));
#202136=CARTESIAN_POINT('Ctrl Pts',(4.14929549611476,-5.3456183819949,76.4072841821929));
#202137=CARTESIAN_POINT('Ctrl Pts',(4.29623099276238,-5.23156632086894,
76.4160335948655));
#202138=CARTESIAN_POINT('Ctrl Pts',(4.43846127436172,-5.11145267304839,
76.4247830075381));
#202139=CARTESIAN_POINT('Ctrl Pts',(4.57550326054583,-4.98568540049755,
76.4335324202107));
#202140=CARTESIAN_POINT('Ctrl Pts',(4.71254416257915,-4.8599191229023,76.4422817636659));
#202141=CARTESIAN_POINT('Ctrl Pts',(4.84439664018889,-4.72849950385288,
76.4510311071212));
#202142=CARTESIAN_POINT('Ctrl Pts',(4.97061286794866,-4.59187289860937,
76.4597804505764));
#202143=CARTESIAN_POINT('Ctrl Pts',(5.096828139128,-4.45524732884553,76.4685297277212));
#202144=CARTESIAN_POINT('Ctrl Pts',(5.21740705147949,-4.31341506235654,
76.4772790048661));
#202145=CARTESIAN_POINT('Ctrl Pts',(5.33194007545801,-4.1668578127559,76.4860282820109));
#202146=CARTESIAN_POINT('Ctrl Pts',(5.44647226944581,-4.02030162521712,
76.494777495752));
#202147=CARTESIAN_POINT('Ctrl Pts',(5.554958486282,-3.86902074887809,76.5035267094931));
#202148=CARTESIAN_POINT('Ctrl Pts',(5.65703027291867,-3.71352898080543,
76.5122759232343));
#202149=CARTESIAN_POINT('Ctrl Pts',(5.75910135377071,-3.55803828789468,
76.5210250764781));
#202150=CARTESIAN_POINT('Ctrl Pts',(5.85475793592822,-3.39833700106593,
76.529774229722));
#202151=CARTESIAN_POINT('Ctrl Pts',(5.94367514427463,-3.23496750823435,
76.5385233829659));
#202152=CARTESIAN_POINT('Ctrl Pts',(6.032591767327,-3.07159909077607,76.5472724786188));
#202153=CARTESIAN_POINT('Ctrl Pts',(6.11476896835979,-2.90456276731318,
76.5560215742717));
#202154=CARTESIAN_POINT('Ctrl Pts',(6.18992765547937,-2.73442583002935,
76.5647706699247));
#202155=CARTESIAN_POINT('Ctrl Pts',(6.26508587283102,-2.56428995616053,
76.5735197108927));
#202156=CARTESIAN_POINT('Ctrl Pts',(6.33322554827205,-2.39105376935083,
76.5822687518607));
#202157=CARTESIAN_POINT('Ctrl Pts',(6.39411526733072,-2.21530561053959,
76.5910177928288));
#202158=CARTESIAN_POINT('Ctrl Pts',(6.45500462602877,-2.03955849185003,
76.5997667820178));
#202159=CARTESIAN_POINT('Ctrl Pts',(6.50864402040759,-1.86129970164475,
76.6085157712068));
#202160=CARTESIAN_POINT('Ctrl Pts',(6.55485128368612,-1.68113463136017,
76.6172647603958));
#202161=CARTESIAN_POINT('Ctrl Pts',(6.60199809554333,-1.49730620116842,
76.6261916458672));
#202162=CARTESIAN_POINT('Ctrl Pts',(6.64140720707875,-1.31149343245686,
76.6351185313387));
#202163=CARTESIAN_POINT('Ctrl Pts',(6.67293928722883,-1.12435326697529,
76.6440454168101));
#202164=CARTESIAN_POINT('Ctrl Pts',(6.70384625876256,-0.940923067006646,
76.6527953309876));
#202165=CARTESIAN_POINT('Ctrl Pts',(6.72718554579795,-0.756217899521745,
76.661545245165));
#202166=CARTESIAN_POINT('Ctrl Pts',(6.74287786815327,-0.570865181254601,
76.6702951593425));
#202167=CARTESIAN_POINT('Ctrl Pts',(6.75856988190845,-0.385516108074057,
76.679044901447));
#202168=CARTESIAN_POINT('Ctrl Pts',(6.76661520773403,-0.199519795226464,
76.6877946435515));
#202169=CARTESIAN_POINT('Ctrl Pts',(6.76698651789579,-0.0135080204557706,
76.696544385656));
#202170=CARTESIAN_POINT('Ctrl Pts',(6.76735782124903,0.172500343512832,
76.7052939673209));
#202171=CARTESIAN_POINT('Ctrl Pts',(6.76005538995184,0.358523882210785,
76.7140435489859));
#202172=CARTESIAN_POINT('Ctrl Pts',(6.74510402742362,0.543930748564235,
76.7227931306508));
#202173=CARTESIAN_POINT('Ctrl Pts',(6.73015291918033,0.729334461615028,
76.7315425635075));
#202174=CARTESIAN_POINT('Ctrl Pts',(6.70755316306598,0.914121237634409,
76.7402919963642));
#202175=CARTESIAN_POINT('Ctrl Pts',(6.6773815187458,1.09766345166088,76.7490414292209));
#202176=CARTESIAN_POINT('Ctrl Pts',(6.64721034747576,1.28120278799631,76.7577907248984));
#202177=CARTESIAN_POINT('Ctrl Pts',(6.60946757205149,1.46349731860296,76.7665400205759));
#202178=CARTESIAN_POINT('Ctrl Pts',(6.56428138111531,1.64392790278129,76.7752893162535));
#202179=CARTESIAN_POINT('Ctrl Pts',(6.51909583859862,1.82435589779013,76.7840384863791));
#202180=CARTESIAN_POINT('Ctrl Pts',(6.46646716392891,2.00291972192213,76.7927876565046));
#202181=CARTESIAN_POINT('Ctrl Pts',(6.40657409872904,2.17901292274602,76.8015368266302));
#202182=CARTESIAN_POINT('Ctrl Pts',(6.34668181342102,2.35510383058908,76.8102858828293));
#202183=CARTESIAN_POINT('Ctrl Pts',(6.27952541914081,2.52872390822504,76.8190349390285));
#202184=CARTESIAN_POINT('Ctrl Pts',(6.20533299175553,2.69928350890202,76.8277839952276));
#202185=CARTESIAN_POINT('Ctrl Pts',(6.12831602991583,2.87633637965551,76.8368661313858));
#202186=CARTESIAN_POINT('Ctrl Pts',(6.04371690605302,3.05009086601399,76.845948267544));
#202187=CARTESIAN_POINT('Ctrl Pts',(5.9518452031666,3.21991112882681,76.8550304037022));
#202188=CARTESIAN_POINT('Ctrl Pts',(5.86333549509303,3.38351691182968,76.8637801840457));
#202189=CARTESIAN_POINT('Ctrl Pts',(5.76807618099397,3.54347103711958,76.8725299643893));
#202190=CARTESIAN_POINT('Ctrl Pts',(5.66639083309043,3.69923018027653,76.8812797447329));
#202191=CARTESIAN_POINT('Ctrl Pts',(5.56470914082226,3.85498372382014,76.8900292105178));
#202192=CARTESIAN_POINT('Ctrl Pts',(5.4566020337209,4.00654234701967,76.8987786763027));
#202193=CARTESIAN_POINT('Ctrl Pts',(5.34243669839236,4.15339127986643,76.9075281420876));
#202194=CARTESIAN_POINT('Ctrl Pts',(5.22827486050614,4.30023571401251,76.9162773398336));
#202195=CARTESIAN_POINT('Ctrl Pts',(5.10805534167137,4.4423705202844,76.9250265375796));
#202196=CARTESIAN_POINT('Ctrl Pts',(4.9821864433998,4.57931296628689,76.9337757353256));
#202197=CARTESIAN_POINT('Ctrl Pts',(4.85632073219606,4.71625194483342,76.9425247115373));
#202198=CARTESIAN_POINT('Ctrl Pts',(4.72480612170326,4.84799861524501,76.9512736877489));
#202199=CARTESIAN_POINT('Ctrl Pts',(4.58808925235307,4.97410554898489,76.9600226639606));
#202200=CARTESIAN_POINT('Ctrl Pts',(4.45136349474047,5.10022068121208,76.9687722089623));
#202201=CARTESIAN_POINT('Ctrl Pts',(4.30943501210082,5.22069514871833,76.977521753964));
#202202=CARTESIAN_POINT('Ctrl Pts',(4.16278587431787,5.33511975166253,76.9862712989657));
#202203=CARTESIAN_POINT('Ctrl Pts',(4.01614535740453,5.44953762807839,76.9950203296194));
#202204=CARTESIAN_POINT('Ctrl Pts',(3.86478496657928,5.5579061753278,77.0037693602731));
#202205=CARTESIAN_POINT('Ctrl Pts',(3.70921874747201,5.65985735539353,77.0125183909269));
#202206=CARTESIAN_POINT('Ctrl Pts',(3.55365041605916,5.76180991977037,77.0212675403765));
#202207=CARTESIAN_POINT('Ctrl Pts',(3.39387638174548,5.85734478552798,77.0300166898261));
#202208=CARTESIAN_POINT('Ctrl Pts',(3.23043927904575,5.94613749121212,77.0387658392757));
#202209=CARTESIAN_POINT('Ctrl Pts',(3.1869176707045,5.96978206944137,77.0410956471919));
#202210=CARTESIAN_POINT('Ctrl Pts',(3.14313645919633,5.99294880633424,77.043425455108));
#202211=CARTESIAN_POINT('Ctrl Pts',(3.09910619832125,6.01563211736945,77.0457552630242));
#202212=CARTESIAN_POINT('Ctrl Pts',(3.09910619832135,6.0156321173694,75.0457552630242));
#202213=CARTESIAN_POINT('Ctrl Pts',(2.93375330764827,6.10081787314653,75.0545047109265));
#202214=CARTESIAN_POINT('Ctrl Pts',(2.76488627843071,6.17918207037039,75.0632541588288));
#202215=CARTESIAN_POINT('Ctrl Pts',(2.59307866646703,6.25045854553997,75.0720036067311));
#202216=CARTESIAN_POINT('Ctrl Pts',(2.42127244185378,6.32173444515037,75.0807529839814));
#202217=CARTESIAN_POINT('Ctrl Pts',(2.24652594672467,6.38592262741837,75.0895023612317));
#202218=CARTESIAN_POINT('Ctrl Pts',(2.06943269687124,6.44280508110561,75.098251738482));
#202219=CARTESIAN_POINT('Ctrl Pts',(1.89234081822075,6.49968709436167,75.1070010479874));
#202220=CARTESIAN_POINT('Ctrl Pts',(1.7129024940558,6.54926340459547,75.1157503574927));
#202221=CARTESIAN_POINT('Ctrl Pts',(1.53172716625045,6.59136563150387,75.1244996669981));
#202222=CARTESIAN_POINT('Ctrl Pts',(1.35055318107325,6.63346754640712,75.1332489116653));
#202223=CARTESIAN_POINT('Ctrl Pts',(1.16764249714415,6.66809542395777,75.1419981563325));
#202224=CARTESIAN_POINT('Ctrl Pts',(0.983616340614355,6.69513165624668,
75.1507474009998));
#202225=CARTESIAN_POINT('Ctrl Pts',(0.799591486713841,6.72216769715961,
75.1594965837355));
#202226=CARTESIAN_POINT('Ctrl Pts',(0.614451459526713,6.74161215869371,
75.1682457664712));
#202227=CARTESIAN_POINT('Ctrl Pts',(0.428825047910284,6.75339900185712,
75.1769949492069));
#202228=CARTESIAN_POINT('Ctrl Pts',(0.24319988859702,6.76518576550221,75.1857440729174));
#202229=CARTESIAN_POINT('Ctrl Pts',(0.0570886373918631,6.76931499599834,
75.194493196628));
#202230=CARTESIAN_POINT('Ctrl Pts',(-0.128876626811231,6.76577266947847,
75.2032423203385));
#202231=CARTESIAN_POINT('Ctrl Pts',(-0.314840698188245,6.76223036567993,
75.21199138793));
#202232=CARTESIAN_POINT('Ctrl Pts',(-0.500658497951343,6.75101660879222,
75.2207404555216));
#202233=CARTESIAN_POINT('Ctrl Pts',(-0.685698951926312,6.73216948296217,
75.2294895231131));
#202234=CARTESIAN_POINT('Ctrl Pts',(-0.870738280459918,6.71332247176292,
75.2382385374916));
#202235=CARTESIAN_POINT('Ctrl Pts',(-1.05499998761255,6.68684221356186,
75.2469875518701));
#202236=CARTESIAN_POINT('Ctrl Pts',(-1.23785829161421,6.65281863948522,
75.2557365662487));
#202237=CARTESIAN_POINT('Ctrl Pts',(-1.43007412916014,6.6170539536912,75.2649332999472));
#202238=CARTESIAN_POINT('Ctrl Pts',(-1.62073882533034,6.57295372728428,
75.2741300336457));
#202239=CARTESIAN_POINT('Ctrl Pts',(-1.80913696087426,6.52068343479414,
75.2833267673442));
#202240=CARTESIAN_POINT('Ctrl Pts',(-1.98838356182049,6.47095219816447,
75.2920767650579));
#202241=CARTESIAN_POINT('Ctrl Pts',(-2.165578275685,6.41382586852252,75.3008267627716));
#202242=CARTESIAN_POINT('Ctrl Pts',(-2.34011918617701,6.34949849944751,
75.3095767604853));
#202243=CARTESIAN_POINT('Ctrl Pts',(-2.5146565568714,6.28517243497134,75.3183265807436));
#202244=CARTESIAN_POINT('Ctrl Pts',(-2.68653996291414,6.21364572244067,
75.3270764010019));
#202245=CARTESIAN_POINT('Ctrl Pts',(-2.85518555376123,6.1351613225402,75.3358262212602));
#202246=CARTESIAN_POINT('Ctrl Pts',(-3.02382794854874,6.05667841002411,
75.3445758756977));
#202247=CARTESIAN_POINT('Ctrl Pts',(-3.18923239105522,5.97123819494089,
75.3533255301352));
#202248=CARTESIAN_POINT('Ctrl Pts',(-3.35083705963998,5.87913088812822,
75.3620751845727));
#202249=CARTESIAN_POINT('Ctrl Pts',(-3.51243888038759,5.78702520445313,
75.3708246848217));
#202250=CARTESIAN_POINT('Ctrl Pts',(-3.67024081220112,5.68825280608092,
75.3795741850706));
#202251=CARTESIAN_POINT('Ctrl Pts',(-3.8237068754089,5.58314917684909,75.3883236853195));
#202252=CARTESIAN_POINT('Ctrl Pts',(-3.97717043814377,5.47804726010517,
75.39707304301));
#202253=CARTESIAN_POINT('Ctrl Pts',(-4.12629803719099,5.3666144808682,75.4058224007005));
#202254=CARTESIAN_POINT('Ctrl Pts',(-4.27058317203627,5.24922931207246,
75.414571758391));
#202255=CARTESIAN_POINT('Ctrl Pts',(-4.41486614771621,5.13184589989555,
75.423320985151));
#202256=CARTESIAN_POINT('Ctrl Pts',(-4.55430658191271,5.00851045725891,
75.4320702119111));
#202257=CARTESIAN_POINT('Ctrl Pts',(-4.68843088998778,4.87964187106066,
75.4408194386712));
#202258=CARTESIAN_POINT('Ctrl Pts',(-4.82255336914844,4.75077504210998,
75.4495685461271));
#202259=CARTESIAN_POINT('Ctrl Pts',(-4.9513596606222,4.61637541911219,75.458317653583));
#202260=CARTESIAN_POINT('Ctrl Pts',(-5.07441230866412,4.47689945405055,
75.4670667610389));
#202261=CARTESIAN_POINT('Ctrl Pts',(-5.19746344223641,4.3374252055884,75.4758157608153));
#202262=CARTESIAN_POINT('Ctrl Pts',(-5.31476088452053,4.19287495494774,
75.4845647605916));
#202263=CARTESIAN_POINT('Ctrl Pts',(-5.42590627626208,4.04373961590256,
75.493313760368));
#202264=CARTESIAN_POINT('Ctrl Pts',(-5.53706380670121,3.89458798910355,
75.5020637156627));
#202265=CARTESIAN_POINT('Ctrl Pts',(-5.64206777069419,3.74085050158971,
75.5108136709573));
#202266=CARTESIAN_POINT('Ctrl Pts',(-5.74056148161667,3.5830493822691,75.5195636262521));
#202267=CARTESIAN_POINT('Ctrl Pts',(-5.83905138949643,3.42525435597101,
75.5283132436932));
#202268=CARTESIAN_POINT('Ctrl Pts',(-5.93103139555515,3.26339625501068,
75.5370628611343));
#202269=CARTESIAN_POINT('Ctrl Pts',(-6.01618907818814,3.09802485068951,
75.5458124785754));
#202270=CARTESIAN_POINT('Ctrl Pts',(-6.10134392543066,2.9326589525363,75.5545618046913));
#202271=CARTESIAN_POINT('Ctrl Pts',(-6.1796767726003,2.76378023990064,75.5633111308071));
#202272=CARTESIAN_POINT('Ctrl Pts',(-6.25092157007539,2.59196229231179,
75.572060456923));
#202273=CARTESIAN_POINT('Ctrl Pts',(-6.32216437406182,2.42014915233196,
75.5808095382255));
#202274=CARTESIAN_POINT('Ctrl Pts',(-6.38631941547465,2.24539720666993,
75.5895586195279));
#202275=CARTESIAN_POINT('Ctrl Pts',(-6.44316881036197,2.06829994951861,
75.5983077008304));
#202276=CARTESIAN_POINT('Ctrl Pts',(-6.50002334523345,1.89118668028667,
75.6070575731727));
#202277=CARTESIAN_POINT('Ctrl Pts',(-6.54957082409984,1.71172794811957,
75.6158074455151));
#202278=CARTESIAN_POINT('Ctrl Pts',(-6.59164294295088,1.53053334254628,
75.6245573178574));
#202279=CARTESIAN_POINT('Ctrl Pts',(-6.63371214081254,1.34935131697926,
75.6333065827123));
#202280=CARTESIAN_POINT('Ctrl Pts',(-6.66830695238927,1.16643393834124,
75.6420558475672));
#202281=CARTESIAN_POINT('Ctrl Pts',(-6.69530988153344,0.982402458384889,
75.6508051124221));
#202282=CARTESIAN_POINT('Ctrl Pts',(-6.72231419689959,0.798361530991149,
75.6595548264291));
#202283=CARTESIAN_POINT('Ctrl Pts',(-6.74172580828875,0.61320667140671,
75.6683045404362));
#202284=CARTESIAN_POINT('Ctrl Pts',(-6.75347878027899,0.427566795157723,
75.6770542544432));
#202285=CARTESIAN_POINT('Ctrl Pts',(-6.76248992366693,0.285234494460517,
75.6837627642215));
#202286=CARTESIAN_POINT('Ctrl Pts',(-6.76699999998568,0.142617266559108,
75.6904712739998));
#202287=CARTESIAN_POINT('Ctrl Pts',(-6.767,6.79698250989073E-10,75.6971797837782));
#202288=CARTESIAN_POINT('',(-6.76699840339575,-0.00267271979378576,75.3028202161898));
#202289=CARTESIAN_POINT('Ctrl Pts',(3.09910619832131,6.01563211736942,74.651395695404));
#202290=CARTESIAN_POINT('Ctrl Pts',(2.93375330764829,6.10081787314652,74.6601451433063));
#202291=CARTESIAN_POINT('Ctrl Pts',(2.76488627843079,6.17918207037035,74.6688945912086));
#202292=CARTESIAN_POINT('Ctrl Pts',(2.59307866646717,6.25045854553991,74.6776440391109));
#202293=CARTESIAN_POINT('Ctrl Pts',(2.42127244185392,6.32173444515031,74.6863934163612));
#202294=CARTESIAN_POINT('Ctrl Pts',(2.24652594672481,6.38592262741832,74.6951427936115));
#202295=CARTESIAN_POINT('Ctrl Pts',(2.06943269687138,6.44280508110556,74.7038921708618));
#202296=CARTESIAN_POINT('Ctrl Pts',(1.89234081822095,6.49968709436161,74.7126414803672));
#202297=CARTESIAN_POINT('Ctrl Pts',(1.71290249405607,6.5492634045954,74.7213907898725));
#202298=CARTESIAN_POINT('Ctrl Pts',(1.53172716625078,6.59136563150379,74.7301400993779));
#202299=CARTESIAN_POINT('Ctrl Pts',(1.35055318107365,6.63346754640703,74.7388893440451));
#202300=CARTESIAN_POINT('Ctrl Pts',(1.16764249714461,6.66809542395768,74.7476385887124));
#202301=CARTESIAN_POINT('Ctrl Pts',(0.983616340614882,6.6951316562466,74.7563878333796));
#202302=CARTESIAN_POINT('Ctrl Pts',(0.799591486714308,6.72216769715955,
74.7651370161153));
#202303=CARTESIAN_POINT('Ctrl Pts',(0.614451459527118,6.74161215869367,
74.773886198851));
#202304=CARTESIAN_POINT('Ctrl Pts',(0.428825047910626,6.7533990018571,74.7826353815867));
#202305=CARTESIAN_POINT('Ctrl Pts',(0.243199888597299,6.7651857655022,74.7913845052972));
#202306=CARTESIAN_POINT('Ctrl Pts',(0.0570886373920775,6.76931499599834,
74.8001336290077));
#202307=CARTESIAN_POINT('Ctrl Pts',(-0.12887662681108,6.76577266947847,
74.8088827527183));
#202308=CARTESIAN_POINT('Ctrl Pts',(-0.314840698188095,6.76223036567993,
74.8176318203098));
#202309=CARTESIAN_POINT('Ctrl Pts',(-0.500658497951193,6.75101660879223,
74.8263808879014));
#202310=CARTESIAN_POINT('Ctrl Pts',(-0.685698951926162,6.73216948296219,
74.8351299554929));
#202311=CARTESIAN_POINT('Ctrl Pts',(-0.870738280459833,6.71332247176294,
74.8438789698715));
#202312=CARTESIAN_POINT('Ctrl Pts',(-1.05499998761252,6.68684221356186,
74.85262798425));
#202313=CARTESIAN_POINT('Ctrl Pts',(-1.23785829161425,6.65281863948521,
74.8613769986285));
#202314=CARTESIAN_POINT('Ctrl Pts',(-1.43007412917405,6.61705395368861,
74.8705737323277));
#202315=CARTESIAN_POINT('Ctrl Pts',(-1.62073882535789,6.5729537272779,74.8797704660269));
#202316=CARTESIAN_POINT('Ctrl Pts',(-1.80913696091507,6.52068343478281,
74.8889671997261));
#202317=CARTESIAN_POINT('Ctrl Pts',(-1.98838356186106,6.47095219815201,
74.8977171974397));
#202318=CARTESIAN_POINT('Ctrl Pts',(-2.16557827572526,6.41382586850893,
74.9064671951534));
#202319=CARTESIAN_POINT('Ctrl Pts',(-2.34011918621693,6.3494984994328,74.9152171928671));
#202320=CARTESIAN_POINT('Ctrl Pts',(-2.51465655691097,6.28517243495551,
74.9239670131254));
#202321=CARTESIAN_POINT('Ctrl Pts',(-2.68653996295333,6.21364572242373,
74.9327168333837));
#202322=CARTESIAN_POINT('Ctrl Pts',(-2.85518555379998,6.13516132252217,
74.941466653642));
#202323=CARTESIAN_POINT('Ctrl Pts',(-3.023827948587,6.05667841000501,74.9502163080795));
#202324=CARTESIAN_POINT('Ctrl Pts',(-3.18923239109293,5.97123819492075,
74.958965962517));
#202325=CARTESIAN_POINT('Ctrl Pts',(-3.35083705967711,5.87913088810706,
74.9677156169545));
#202326=CARTESIAN_POINT('Ctrl Pts',(-3.51243888042414,5.78702520443095,
74.9764651172035));
#202327=CARTESIAN_POINT('Ctrl Pts',(-3.67024081223705,5.68825280605774,
74.9852146174524));
#202328=CARTESIAN_POINT('Ctrl Pts',(-3.82370687544417,5.58314917682494,
74.9939641177014));
#202329=CARTESIAN_POINT('Ctrl Pts',(-3.97717043817832,5.47804726008009,
75.0027134753918));
#202330=CARTESIAN_POINT('Ctrl Pts',(-4.12629803722479,5.36661448084222,
75.0114628330823));
#202331=CARTESIAN_POINT('Ctrl Pts',(-4.27058317206927,5.24922931204561,
75.0202121907728));
#202332=CARTESIAN_POINT('Ctrl Pts',(-4.41486614774858,5.13184589986771,
75.0289614175329));
#202333=CARTESIAN_POINT('Ctrl Pts',(-4.5543065819444,5.00851045723011,75.0377106442929));
#202334=CARTESIAN_POINT('Ctrl Pts',(-4.68843089001874,4.87964187103092,
75.046459871053));
#202335=CARTESIAN_POINT('Ctrl Pts',(-4.82255336917867,4.75077504207929,
75.0552089785089));
#202336=CARTESIAN_POINT('Ctrl Pts',(-4.95135966065167,4.61637541908059,
75.0639580859649));
#202337=CARTESIAN_POINT('Ctrl Pts',(-5.07441230869278,4.47689945401807,
75.0727071934208));
#202338=CARTESIAN_POINT('Ctrl Pts',(-5.19746344226443,4.33742520555484,
75.0814561931972));
#202339=CARTESIAN_POINT('Ctrl Pts',(-5.31476088454786,4.19287495491313,
75.0902051929735));
#202340=CARTESIAN_POINT('Ctrl Pts',(-5.42590627628866,4.0437396158669,75.0989541927499));
#202341=CARTESIAN_POINT('Ctrl Pts',(-5.53706380672681,3.89458798906716,
75.1077041480446));
#202342=CARTESIAN_POINT('Ctrl Pts',(-5.64206777071878,3.74085050155263,
75.1164541033393));
#202343=CARTESIAN_POINT('Ctrl Pts',(-5.74056148164022,3.58304938223138,
75.125204058634));
#202344=CARTESIAN_POINT('Ctrl Pts',(-5.83905138951894,3.42525435593264,
75.1339536760751));
#202345=CARTESIAN_POINT('Ctrl Pts',(-5.9310313955766,3.2633962549717,75.1427032935162));
#202346=CARTESIAN_POINT('Ctrl Pts',(-6.0161890782085,3.09802485064997,75.1514529109573));
#202347=CARTESIAN_POINT('Ctrl Pts',(-6.10134392544987,2.93265895249632,
75.1602022370732));
#202348=CARTESIAN_POINT('Ctrl Pts',(-6.17967677261836,2.76378023986026,
75.168951563189));
#202349=CARTESIAN_POINT('Ctrl Pts',(-6.25092157009228,2.59196229227106,
75.1777008893049));
#202350=CARTESIAN_POINT('Ctrl Pts',(-6.32216437407759,2.42014915229077,
75.1864499706074));
#202351=CARTESIAN_POINT('Ctrl Pts',(-6.38631941548928,2.24539720662832,
75.1951990519098));
#202352=CARTESIAN_POINT('Ctrl Pts',(-6.44316881037545,2.06829994947663,
75.2039481332122));
#202353=CARTESIAN_POINT('Ctrl Pts',(-6.50002334524579,1.89118668024426,
75.2126980055546));
#202354=CARTESIAN_POINT('Ctrl Pts',(-6.54957082411103,1.71172794807677,
75.221447877897));
#202355=CARTESIAN_POINT('Ctrl Pts',(-6.5916429429609,1.53053334250314,75.2301977502393));
#202356=CARTESIAN_POINT('Ctrl Pts',(-6.63371214082141,1.34935131693566,
75.2389470150942));
#202357=CARTESIAN_POINT('Ctrl Pts',(-6.66830695239697,1.16643393829723,
75.2476962799491));
#202358=CARTESIAN_POINT('Ctrl Pts',(-6.69530988153995,0.982402458340512,
75.256445544804));
#202359=CARTESIAN_POINT('Ctrl Pts',(-6.72231419690488,0.798361530946657,
75.265195258811));
#202360=CARTESIAN_POINT('Ctrl Pts',(-6.74172580829281,0.613206671362151,
75.2739449728181));
#202361=CARTESIAN_POINT('Ctrl Pts',(-6.75347878028181,0.42756679511315,
75.2826946868251));
#202362=CARTESIAN_POINT('Ctrl Pts',(-6.76248992368213,0.285234494205576,
75.2894031966133));
#202363=CARTESIAN_POINT('Ctrl Pts',(-6.76699999999994,0.142617266092986,
75.2961117064016));
#202364=CARTESIAN_POINT('Ctrl Pts',(-6.767,2.84793741451067E-12,75.3028202161898));
#202365=CARTESIAN_POINT('Ctrl Pts',(-6.76699517037156,-0.00808481094492364,
75.3028202161898));
#202366=CARTESIAN_POINT('Ctrl Pts',(-6.76674412400169,-0.218210883648386,
75.3126841961279));
#202367=CARTESIAN_POINT('Ctrl Pts',(-6.75670250884975,-0.427869699865752,
75.3225481760661));
#202368=CARTESIAN_POINT('Ctrl Pts',(-6.73702211524587,-0.636256252376383,
75.3324121560042));
#202369=CARTESIAN_POINT('Ctrl Pts',(-6.71715949916007,-0.846572274163036,
75.3423674673933));
#202370=CARTESIAN_POINT('Ctrl Pts',(-6.6874788848665,-1.05559238172179,
75.3523227787825));
#202371=CARTESIAN_POINT('Ctrl Pts',(-6.6481840108267,-1.26251271605013,
75.3622780901717));
#202372=CARTESIAN_POINT('Ctrl Pts',(-6.60849008442896,-1.47153439436636,
75.3723345010193));
#202373=CARTESIAN_POINT('Ctrl Pts',(-6.55898568021543,-1.67841345953767,
75.3823909118669));
#202374=CARTESIAN_POINT('Ctrl Pts',(-6.49992815531097,-1.88234507351753,
75.3924473227145));
#202375=CARTESIAN_POINT('Ctrl Pts',(-6.49169906780799,-1.91076094598729,
75.3938485850425));
#202376=CARTESIAN_POINT('Ctrl Pts',(-6.48328457375079,-1.9391196286264,
75.3952498473704));
#202377=CARTESIAN_POINT('Ctrl Pts',(-6.47468544086907,-1.96741897972905,
75.3966511096984));
#202378=CARTESIAN_POINT('Ctrl Pts',(-6.42430666958161,-2.13321320065739,
75.4048605274739));
#202379=CARTESIAN_POINT('Ctrl Pts',(-6.36747888064407,-2.29732383691437,
75.4130699452495));
#202380=CARTESIAN_POINT('Ctrl Pts',(-6.30432968657984,-2.45921048365287,
75.4212793630251));
#202381=CARTESIAN_POINT('Ctrl Pts',(-6.2412567587065,-2.62090161755726,
75.4294788661686));
#202382=CARTESIAN_POINT('Ctrl Pts',(-6.17187775572661,-2.78037377723096,
75.4376783693121));
#202383=CARTESIAN_POINT('Ctrl Pts',(-6.09637055659032,-2.93709976622154,
75.4458778724557));
#202384=CARTESIAN_POINT('Ctrl Pts',(-6.02093917221881,-3.09366839082666,
75.4540691426968));
#202385=CARTESIAN_POINT('Ctrl Pts',(-5.93939199977997,-3.24749601291137,
75.4622604129379));
#202386=CARTESIAN_POINT('Ctrl Pts',(-5.85195570584304,-3.39807348608753,
75.470451683179));
#202387=CARTESIAN_POINT('Ctrl Pts',(-5.76458940576276,-3.5485304200963,
75.4786363962049));
#202388=CARTESIAN_POINT('Ctrl Pts',(-5.67134355334986,-3.69574207647182,
75.4868211092309));
#202389=CARTESIAN_POINT('Ctrl Pts',(-5.57249165080646,-3.83922203078857,
75.4950058222568));
#202390=CARTESIAN_POINT('Ctrl Pts',(-5.47369876359507,-3.98261632648953,
75.5031856489473));
#202391=CARTESIAN_POINT('Ctrl Pts',(-5.36930669694921,-4.1222830617013,
75.5113654756377));
#202392=CARTESIAN_POINT('Ctrl Pts',(-5.25963338298041,-4.25776298972101,
75.5195453023282));
#202393=CARTESIAN_POINT('Ctrl Pts',(-5.14999231549889,-4.3932030835129,
75.5277227239607));
#202394=CARTESIAN_POINT('Ctrl Pts',(-5.03507331681905,-4.5244585393973,
75.5359001455932));
#202395=CARTESIAN_POINT('Ctrl Pts',(-4.91523602282502,-4.65110135773489,
75.5440775672257));
#202396=CARTESIAN_POINT('Ctrl Pts',(-4.79541506395904,-4.77772691327736,
75.5522538741865));
#202397=CARTESIAN_POINT('Ctrl Pts',(-4.67067739207716,-4.89974082083716,
75.5604301811474));
#202398=CARTESIAN_POINT('Ctrl Pts',(-4.54142108047619,-5.01675029972656,
75.5686064881083));
#202399=CARTESIAN_POINT('Ctrl Pts',(-4.4121585599736,-5.13376539923389,
75.5767831878228));
#202400=CARTESIAN_POINT('Ctrl Pts',(-4.27837723475216,-5.24577534900321,
75.5849598875373));
#202401=CARTESIAN_POINT('Ctrl Pts',(-4.14050999471701,-5.35242617731889,
75.5931365872518));
#202402=CARTESIAN_POINT('Ctrl Pts',(-4.00261071665158,-5.45910178949524,
75.601315187094));
#202403=CARTESIAN_POINT('Ctrl Pts',(-3.86062391808235,-5.56041557933863,
75.6094937869362));
#202404=CARTESIAN_POINT('Ctrl Pts',(-3.71501334252604,-5.65605559244722,
75.6176723867783));
#202405=CARTESIAN_POINT('Ctrl Pts',(-3.56926220338754,-5.75178793060015,
75.6258588817427));
#202406=CARTESIAN_POINT('Ctrl Pts',(-3.41988060024241,-5.84183535108088,
75.6340453767071));
#202407=CARTESIAN_POINT('Ctrl Pts',(-3.26735967916884,-5.92593028367207,
75.6422318716715));
#202408=CARTESIAN_POINT('Ctrl Pts',(-3.11476398037107,-6.01006644619835,
75.6504223802981));
#202409=CARTESIAN_POINT('Ctrl Pts',(-2.95902621751108,-6.08824414126907,
75.6586128889247));
#202410=CARTESIAN_POINT('Ctrl Pts',(-2.80065947731021,-6.1602431357985,
75.6668033975513));
#202411=CARTESIAN_POINT('Ctrl Pts',(-2.64206886595309,-6.23234390989435,
75.6750054844843));
#202412=CARTESIAN_POINT('Ctrl Pts',(-2.48084218411102,-6.29824839147717,
75.6832075714173));
#202413=CARTESIAN_POINT('Ctrl Pts',(-2.31751088050882,-6.35778517399914,
75.6914096583503));
#202414=CARTESIAN_POINT('Ctrl Pts',(-2.16384472218788,-6.41379886180526,
75.6991263860162));
#202415=CARTESIAN_POINT('Ctrl Pts',(-2.00831603636468,-6.46417655449741,
75.706843113682));
#202416=CARTESIAN_POINT('Ctrl Pts',(-1.85137628097049,-6.50881670246289,
75.7145598413479));
#202417=CARTESIAN_POINT('Ctrl Pts',(-1.67084417500735,-6.56016748928215,
75.7234366048752));
#202418=CARTESIAN_POINT('Ctrl Pts',(-1.4880440107246,-6.60404021423144,
75.7323133684024));
#202419=CARTESIAN_POINT('Ctrl Pts',(-1.30359371124132,-6.64025093170522,
75.7411901319297));
#202420=CARTESIAN_POINT('Ctrl Pts',(-1.11942465968586,-6.67640643544781,
75.7500533602588));
#202421=CARTESIAN_POINT('Ctrl Pts',(-0.933610755225823,-6.70492318822488,
75.758916588588));
#202422=CARTESIAN_POINT('Ctrl Pts',(-0.746782833147205,-6.72566758025675,
75.7677798169171));
#202423=CARTESIAN_POINT('Ctrl Pts',(-0.56040117232329,-6.74636242178078,
75.7766218743455));
#202424=CARTESIAN_POINT('Ctrl Pts',(-0.373010593702273,-6.7593219234436,
75.7854639317739));
#202425=CARTESIAN_POINT('Ctrl Pts',(-0.185249234690844,-6.76446389014285,
75.7943059892023));
#202426=CARTESIAN_POINT('Ctrl Pts',(0.00223489196362983,-6.76959826465404,
75.8031349912053));
#202427=CARTESIAN_POINT('Ctrl Pts',(0.190088440290167,-6.76693811895071,
75.8119639932082));
#202428=CARTESIAN_POINT('Ctrl Pts',(0.377668239005517,-6.75645289343798,
75.8207929952111));
#202429=CARTESIAN_POINT('Ctrl Pts',(0.564800489672221,-6.74599268470344,
75.829600932032));
#202430=CARTESIAN_POINT('Ctrl Pts',(0.751660027069486,-6.72774466541701,
75.8384088688529));
#202431=CARTESIAN_POINT('Ctrl Pts',(0.937604438106017,-6.70173014360053,
75.8472168056738));
#202432=CARTESIAN_POINT('Ctrl Pts',(1.1226593089935,-6.67584007275025,75.8559826061734));
#202433=CARTESIAN_POINT('Ctrl Pts',(1.30680752142655,-6.64225764464012,
75.864748406673));
#202434=CARTESIAN_POINT('Ctrl Pts',(1.48941603416143,-6.60105513362696,
75.8735142071727));
#202435=CARTESIAN_POINT('Ctrl Pts',(1.66120466573386,-6.56229394512435,
75.8817606183061));
#202436=CARTESIAN_POINT('Ctrl Pts',(1.83145444700487,-6.51682806607553,
75.8900070294395));
#202437=CARTESIAN_POINT('Ctrl Pts',(1.9996179046617,-6.46481378195508,75.8982534405729));
#202438=CARTESIAN_POINT('Ctrl Pts',(2.16783559744715,-6.41278272248148,
75.9065025112922));
#202439=CARTESIAN_POINT('Ctrl Pts',(2.33396528980005,-6.35419915322431,
75.9147515820116));
#202440=CARTESIAN_POINT('Ctrl Pts',(2.49747641154605,-6.28926868354112,
75.9230006527309));
#202441=CARTESIAN_POINT('Ctrl Pts',(2.66106837863366,-6.2243061100723,75.9312538020654));
#202442=CARTESIAN_POINT('Ctrl Pts',(2.82203886860477,-6.15299051241487,
75.9395069513999));
#202443=CARTESIAN_POINT('Ctrl Pts',(2.97987883364944,-6.07557496347202,
75.9477601007344));
#202444=CARTESIAN_POINT('Ctrl Pts',(3.13791136499413,-5.99806496680284,
75.9560233189918));
#202445=CARTESIAN_POINT('Ctrl Pts',(3.292805426646,-5.91444030848025,75.9642865372491));
#202446=CARTESIAN_POINT('Ctrl Pts',(3.44407711282112,-5.8249997288362,75.9725497555064));
#202447=CARTESIAN_POINT('Ctrl Pts',(3.59545431035029,-5.73549676477041,
75.9808187373232));
#202448=CARTESIAN_POINT('Ctrl Pts',(3.74320380036393,-5.6401699817092,75.9890877191399));
#202449=CARTESIAN_POINT('Ctrl Pts',(3.88687203736883,-5.53936050145866,
75.9973567009567));
#202450=CARTESIAN_POINT('Ctrl Pts',(4.03074592888161,-5.43840671704957,
76.0056375194426));
#202451=CARTESIAN_POINT('Ctrl Pts',(4.17052661860345,-5.3319547707308,76.0139183379284));
#202452=CARTESIAN_POINT('Ctrl Pts',(4.30579407760629,-5.22038565254049,
76.0221991564143));
#202453=CARTESIAN_POINT('Ctrl Pts',(4.36171117038323,-5.17426502028438,
76.0256222952753));
#202454=CARTESIAN_POINT('Ctrl Pts',(4.41685746241446,-5.12727037495087,
76.0290454341363));
#202455=CARTESIAN_POINT('Ctrl Pts',(4.47120520070793,-5.07943038668338,
76.0324685729973));
#202456=CARTESIAN_POINT('Ctrl Pts',(4.60511039071803,-4.9615593782442,76.0409027061187));
#202457=CARTESIAN_POINT('Ctrl Pts',(4.73447418182554,-4.83828225145958,
76.0493368392401));
#202458=CARTESIAN_POINT('Ctrl Pts',(4.8588497279284,-4.70997540560565,76.0577709723616));
#202459=CARTESIAN_POINT('Ctrl Pts',(4.98310726230948,-4.58179030162358,
76.0661971028924));
#202460=CARTESIAN_POINT('Ctrl Pts',(5.10238575313522,-4.44858523015409,
76.0746232334233));
#202461=CARTESIAN_POINT('Ctrl Pts',(5.21627314881857,-4.31077527098252,
76.0830493639542));
#202462=CARTESIAN_POINT('Ctrl Pts',(5.33007048663557,-4.17307428674017,
76.0914688314181));
#202463=CARTESIAN_POINT('Ctrl Pts',(5.438485014381,-4.03077593088117,76.0998882988821));
#202464=CARTESIAN_POINT('Ctrl Pts',(5.54114287740415,-3.88433065175885,
76.1083077663461));
#202465=CARTESIAN_POINT('Ctrl Pts',(5.64373576883996,-3.7379780570346,76.1167219051761));
#202466=CARTESIAN_POINT('Ctrl Pts',(5.7405790669913,-3.58748404522176,76.1251360440062));
#202467=CARTESIAN_POINT('Ctrl Pts',(5.83134019552794,-3.43333082064927,
76.1335501828363));
#202468=CARTESIAN_POINT('Ctrl Pts',(5.92205819511733,-3.2792508484305,76.1419603233363));
#202469=CARTESIAN_POINT('Ctrl Pts',(6.00669961796768,-3.1215154188964,76.1503704638363));
#202470=CARTESIAN_POINT('Ctrl Pts',(6.08497590004447,-2.96063461032902,
76.1587806043364));
#202471=CARTESIAN_POINT('Ctrl Pts',(6.16323324838128,-2.79979271617243,
76.1671887105623));
#202472=CARTESIAN_POINT('Ctrl Pts',(6.23512837671761,-2.63580725995374,
76.1755968167882));
#202473=CARTESIAN_POINT('Ctrl Pts',(6.30041904326799,-2.46921219809601,
76.1840049230141));
#202474=CARTESIAN_POINT('Ctrl Pts',(6.36570165658729,-2.30263768478833,
76.1924119921481));
#202475=CARTESIAN_POINT('Ctrl Pts',(6.42438130965619,-2.13345451955307,
76.2008190612821));
#202476=CARTESIAN_POINT('Ctrl Pts',(6.47626410273575,-1.96221616332564,
76.2092261304161));
#202477=CARTESIAN_POINT('Ctrl Pts',(6.5281479297892,-1.79097439448334,76.2176333670949));
#202478=CARTESIAN_POINT('Ctrl Pts',(6.57323452992889,-1.61767767396493,
76.2260406037737));
#202479=CARTESIAN_POINT('Ctrl Pts',(6.61137992921407,-1.44289446307947,
76.2344478404524));
#202480=CARTESIAN_POINT('Ctrl Pts',(6.6495315541235,-1.26808272622187,76.2428564492572));
#202481=CARTESIAN_POINT('Ctrl Pts',(6.68073964883631,-1.0917843429905,76.251265058062));
#202482=CARTESIAN_POINT('Ctrl Pts',(6.70491132087542,-0.914578142750349,
76.2596736668669));
#202483=CARTESIAN_POINT('Ctrl Pts',(6.72909954479188,-0.737250598182512,
76.2680880335796));
#202484=CARTESIAN_POINT('Ctrl Pts',(6.74624167263049,-0.559014326970189,
76.2765024002923));
#202485=CARTESIAN_POINT('Ctrl Pts',(6.75629657398825,-0.380454470751356,
76.2849167670051));
#202486=CARTESIAN_POINT('Ctrl Pts',(6.7663551044929,-0.201830166366891,
76.2933341707414));
#202487=CARTESIAN_POINT('Ctrl Pts',(6.76932129565298,-0.0228823791739918,
76.3017515744777));
#202488=CARTESIAN_POINT('Ctrl Pts',(6.76520616228446,0.155803022397947,
76.3101689782141));
#202489=CARTESIAN_POINT('Ctrl Pts',(6.7610871303496,0.334657705699289,76.3185943563717));
#202490=CARTESIAN_POINT('Ctrl Pts',(6.7498733840753,0.513249171542303,76.3270197345293));
#202491=CARTESIAN_POINT('Ctrl Pts',(6.73162797166826,0.690994827081569,
76.3354451126868));
#202492=CARTESIAN_POINT('Ctrl Pts',(6.72084926653247,0.796000291879156,
76.3404225100069));
#202493=CARTESIAN_POINT('Ctrl Pts',(6.70761749134104,0.900710687160406,
76.345399907327));
#202494=CARTESIAN_POINT('Ctrl Pts',(6.6919540555666,1.00500742195553,76.350377304647));
#202495=CARTESIAN_POINT('Ctrl Pts',(6.66630198399042,1.17581460274618,76.3585288081968));
#202496=CARTESIAN_POINT('Ctrl Pts',(6.6340736292976,1.34585493051098,76.3666803117466));
#202497=CARTESIAN_POINT('Ctrl Pts',(6.59532689361421,1.51457986463876,76.3748318152964));
#202498=CARTESIAN_POINT('Ctrl Pts',(6.55661414630117,1.68315679441345,76.3829761684032));
#202499=CARTESIAN_POINT('Ctrl Pts',(6.51139448118651,1.85042027404336,76.3911205215101));
#202500=CARTESIAN_POINT('Ctrl Pts',(6.45977736301567,2.01582871798928,76.399264874617));
#202501=CARTESIAN_POINT('Ctrl Pts',(6.40819573438519,2.18112343474826,76.4074036280438));
#202502=CARTESIAN_POINT('Ctrl Pts',(6.35022551883061,2.34456530823284,76.4155423814706));
#202503=CARTESIAN_POINT('Ctrl Pts',(6.28602684114741,2.50562478283846,76.4236811348974));
#202504=CARTESIAN_POINT('Ctrl Pts',(6.22185949988904,2.6666056416797,76.4318159156655));
#202505=CARTESIAN_POINT('Ctrl Pts',(6.15146988600607,2.82520607917462,76.4399506964336));
#202506=CARTESIAN_POINT('Ctrl Pts',(6.07506737664011,2.98091351254663,76.4480854772017));
#202507=CARTESIAN_POINT('Ctrl Pts',(5.9986867476782,3.13657635390741,76.4562179283043));
#202508=CARTESIAN_POINT('Ctrl Pts',(5.91629681453725,3.28934751432502,76.4643503794069));
#202509=CARTESIAN_POINT('Ctrl Pts',(5.8281543087654,3.43873615638351,76.4724828305095));
#202510=CARTESIAN_POINT('Ctrl Pts',(5.74000821130039,3.58813088583606,76.480615612999));
#202511=CARTESIAN_POINT('Ctrl Pts',(5.64610925481213,3.73414250504625,76.4887483954885));
#202512=CARTESIAN_POINT('Ctrl Pts',(5.54675927222819,3.87630630574399,76.4968811779779));
#202513=CARTESIAN_POINT('Ctrl Pts',(5.49606091185689,3.94885258519037,76.5010313421425));
#202514=CARTESIAN_POINT('Ctrl Pts',(5.44394377425027,4.02039731685149,76.5051815063071));
#202515=CARTESIAN_POINT('Ctrl Pts',(5.39045223894833,4.09088177042762,76.5093316704717));
#202516=CARTESIAN_POINT('Ctrl Pts',(5.2747518899463,4.24333721654526,76.5183083326585));
#202517=CARTESIAN_POINT('Ctrl Pts',(5.15267820629121,4.39075272790816,76.5272849948453));
#202518=CARTESIAN_POINT('Ctrl Pts',(5.02468706398398,4.53263818421811,76.5362616570321));
#202519=CARTESIAN_POINT('Ctrl Pts',(4.89647541171931,4.67476808834974,76.5452537846907));
#202520=CARTESIAN_POINT('Ctrl Pts',(4.76232608452548,4.81134871614229,76.5542459123493));
#202521=CARTESIAN_POINT('Ctrl Pts',(4.62273175352707,4.94192676341248,76.5632380400078));
#202522=CARTESIAN_POINT('Ctrl Pts',(4.48282650171009,5.07279564937973,76.5722501959847));
#202523=CARTESIAN_POINT('Ctrl Pts',(4.33745215952732,5.19763504337567,76.5812623519615));
#202524=CARTESIAN_POINT('Ctrl Pts',(4.18713634973639,5.31603030359273,76.5902745079383));
#202525=CARTESIAN_POINT('Ctrl Pts',(4.03666276173279,5.43454983678262,76.5992961234781));
#202526=CARTESIAN_POINT('Ctrl Pts',(3.88123753537951,5.54661157850362,76.6083177390179));
#202527=CARTESIAN_POINT('Ctrl Pts',(3.72141859327451,5.65184329698115,76.6173393545577));
#202528=CARTESIAN_POINT('Ctrl Pts',(3.56139431352945,5.75721021866079,76.6263725611969));
#202529=CARTESIAN_POINT('Ctrl Pts',(3.39696523344041,5.85572944270786,76.6354057678361));
#202530=CARTESIAN_POINT('Ctrl Pts',(3.22871696210916,5.94707287483419,76.6444389744753));
#202531=CARTESIAN_POINT('Ctrl Pts',(3.18575890182591,5.97039517486565,76.6467453817405));
#202532=CARTESIAN_POINT('Ctrl Pts',(3.14255198469688,5.99324991326842,76.6490517890057));
#202533=CARTESIAN_POINT('Ctrl Pts',(3.09910619832139,6.01563211736937,76.6513581962709));
#202534=CARTESIAN_POINT('Origin',(0.,0.,4.30282021618968));
#202535=CARTESIAN_POINT('',(3.09910619832139,6.01563211736937,79.0457552630242));
#202536=CARTESIAN_POINT('',(3.09910619832128,6.01563211736943,78.6515182808518));
#202537=CARTESIAN_POINT('',(3.09910619832133,6.0156321173694,4.30282021618968));
#202538=CARTESIAN_POINT('',(-6.767,9.59489064569771E-10,77.697179783765));
#202539=CARTESIAN_POINT('Ctrl Pts',(-6.767,2.64793996645105E-12,77.69717978381));
#202540=CARTESIAN_POINT('Ctrl Pts',(-6.76700000000007,-0.186007249524281,
77.7059292956212));
#202541=CARTESIAN_POINT('Ctrl Pts',(-6.75932637294534,-0.372014355747388,
77.7146788074324));
#202542=CARTESIAN_POINT('Ctrl Pts',(-6.74400518264201,-0.557389537485025,
77.7234283192436));
#202543=CARTESIAN_POINT('Ctrl Pts',(-6.72868405705112,-0.742763936249463,
77.7321777940992));
#202544=CARTESIAN_POINT('Ctrl Pts',(-6.70571545645755,-0.927506130240071,
77.7409272689549));
#202545=CARTESIAN_POINT('Ctrl Pts',(-6.67517739404835,-1.11098863989955,
77.7496767438106));
#202546=CARTESIAN_POINT('Ctrl Pts',(-6.64463945808713,-1.2944703898189,
77.7584261824376));
#202547=CARTESIAN_POINT('Ctrl Pts',(-6.60653217008366,-1.47669218313631,
77.7671756210646));
#202548=CARTESIAN_POINT('Ctrl Pts',(-6.56098496092689,-1.65703510599238,
77.7759250596916));
#202549=CARTESIAN_POINT('Ctrl Pts',(-6.51543793658309,-1.83737729708656,
77.7846744628168));
#202550=CARTESIAN_POINT('Ctrl Pts',(-6.46245112167433,-2.01584035510887,
77.793423865942));
#202551=CARTESIAN_POINT('Ctrl Pts',(-6.40220448374265,-2.19181813760757,
77.8021732690671));
#202552=CARTESIAN_POINT('Ctrl Pts',(-6.3419580852652,-2.367795220671,77.8109226374172));
#202553=CARTESIAN_POINT('Ctrl Pts',(-6.27445201433125,-2.54128677684113,
77.8196720057673));
#202554=CARTESIAN_POINT('Ctrl Pts',(-6.19991555071929,-2.7117035538475,
77.8284213741174));
#202555=CARTESIAN_POINT('Ctrl Pts',(-6.12537937716719,-2.88211966767422,
77.8371707084192));
#202556=CARTESIAN_POINT('Ctrl Pts',(-6.04381298052545,-3.04946076371735,
77.845920042721));
#202557=CARTESIAN_POINT('Ctrl Pts',(-5.95549339335856,-3.21315848374502,
77.8546693770228));
#202558=CARTESIAN_POINT('Ctrl Pts',(-5.8671741425544,-3.37685558033439,
77.8634186780029));
#202559=CARTESIAN_POINT('Ctrl Pts',(-5.77210188876636,-3.53690907646694,
77.8721679789831));
#202560=CARTESIAN_POINT('Ctrl Pts',(-5.67059953347041,-3.69277536969217,
77.8809172799633));
#202561=CARTESIAN_POINT('Ctrl Pts',(-5.56909755631438,-3.84864108224844,
77.8896665483486));
#202562=CARTESIAN_POINT('Ctrl Pts',(-5.46116568196915,-4.00031938297428,
77.8984158167338));
#202563=CARTESIAN_POINT('Ctrl Pts',(-5.34717048533678,-4.14729511859757,
77.9071650851191));
#202564=CARTESIAN_POINT('Ctrl Pts',(-5.23317570391911,-4.29427031887825,
77.9159143216362));
#202565=CARTESIAN_POINT('Ctrl Pts',(-5.11311782003588,-4.43654276189462,
77.9246635581532));
#202566=CARTESIAN_POINT('Ctrl Pts',(-4.98740458984825,-4.57362924351774,
77.9334127946703));
#202567=CARTESIAN_POINT('Ctrl Pts',(-4.86169180711813,-4.71071523720195,
77.9421620000457));
#202568=CARTESIAN_POINT('Ctrl Pts',(-4.73032391204238,-4.84261509523173,
77.9509112054212));
#202569=CARTESIAN_POINT('Ctrl Pts',(-4.59374707013663,-4.96888084538271,
77.9596604107966));
#202570=CARTESIAN_POINT('Ctrl Pts',(-4.45717070301509,-5.09514615659408,
77.968409585757));
#202571=CARTESIAN_POINT('Ctrl Pts',(-4.31538563571106,-5.21577720459474,
77.9771587607175));
#202572=CARTESIAN_POINT('Ctrl Pts',(-4.16887341029574,-5.33036429232835,
77.9859079356779));
#202573=CARTESIAN_POINT('Ctrl Pts',(-4.02236168203749,-5.44495099123585,
77.99465708095));
#202574=CARTESIAN_POINT('Ctrl Pts',(-3.87112305348185,-5.55349359438589,
78.003406226222));
#202575=CARTESIAN_POINT('Ctrl Pts',(-3.71567117017754,-5.65562346298898,
78.0121553714941));
#202576=CARTESIAN_POINT('Ctrl Pts',(-3.56021980145811,-5.75775299351649,
78.0209044878042));
#202577=CARTESIAN_POINT('Ctrl Pts',(-3.4005554453834,-5.85346967463878,
78.0296536041144));
#202578=CARTESIAN_POINT('Ctrl Pts',(-3.23722035986843,-5.94244842986907,
78.0384027204246));
#202579=CARTESIAN_POINT('Ctrl Pts',(-3.07388580147141,-6.0314268979455,
78.0471518084994));
#202580=CARTESIAN_POINT('Ctrl Pts',(-2.90688078896509,-6.11366734656815,
78.0559008965743));
#202581=CARTESIAN_POINT('Ctrl Pts',(-2.7367725072127,-6.18889046952398,
78.0646499846491));
#202582=CARTESIAN_POINT('Ctrl Pts',(-2.56666476031348,-6.26411335596383,
78.0733990452152));
#202583=CARTESIAN_POINT('Ctrl Pts',(-2.39345402574995,-6.33231884500621,
78.0821481057812));
#202584=CARTESIAN_POINT('Ctrl Pts',(-2.21772856065384,-6.39327529762799,
78.0908971663472));
#202585=CARTESIAN_POINT('Ctrl Pts',(-2.04200363348287,-6.45423156365183,
78.0996462001309));
#202586=CARTESIAN_POINT('Ctrl Pts',(-1.86376426189034,-6.50793874375729,
78.1083952339147));
#202587=CARTESIAN_POINT('Ctrl Pts',(-1.6836157775289,-6.5542144390961,78.1171442676984));
#202588=CARTESIAN_POINT('Ctrl Pts',(-1.50346782967559,-6.60048999661922,
78.1258932754262));
#202589=CARTESIAN_POINT('Ctrl Pts',(-1.3214110579477,-6.63933404237755,
78.134642283154));
#202590=CARTESIAN_POINT('Ctrl Pts',(-1.1380637548683,-6.67061465607594,
78.1433912908818));
#202591=CARTESIAN_POINT('Ctrl Pts',(-0.954716982601156,-6.70189517921323,
78.1521402732802));
#202592=CARTESIAN_POINT('Ctrl Pts',(-0.770079968900338,-6.72561226592249,
78.1608892556786));
#202593=CARTESIAN_POINT('Ctrl Pts',(-0.584779765556509,-6.74168536983117,
78.169638238077));
#202594=CARTESIAN_POINT('Ctrl Pts',(-0.391489830649617,-6.75845151013863,
78.1787644570869));
#202595=CARTESIAN_POINT('Ctrl Pts',(-0.197478578236712,-6.7668998303163,
78.1878906760967));
#202596=CARTESIAN_POINT('Ctrl Pts',(-0.00346287644978017,-6.76699911397118,
78.1970168951066));
#202597=CARTESIAN_POINT('Ctrl Pts',(0.18448983465634,-6.76709529501184,
78.2058579197724));
#202598=CARTESIAN_POINT('Ctrl Pts',(0.372446404251812,-6.75935639738155,
78.2146989444382));
#202599=CARTESIAN_POINT('Ctrl Pts',(0.559755019490766,-6.74380925873166,
78.2235399691041));
#202600=CARTESIAN_POINT('Ctrl Pts',(0.745134705524248,-6.72842222659778,
78.2322899477138));
#202601=CARTESIAN_POINT('Ctrl Pts',(0.929879431231083,-6.70538706057489,
78.2410399263235));
#202602=CARTESIAN_POINT('Ctrl Pts',(1.11336163627081,-6.67478200894085,
78.2497899049333));
#202603=CARTESIAN_POINT('Ctrl Pts',(1.29684196300992,-6.6441772706096,78.2585397939698));
#202604=CARTESIAN_POINT('Ctrl Pts',(1.47905951217801,-6.60600284890526,
78.2672896830064));
#202605=CARTESIAN_POINT('Ctrl Pts',(1.65939532067392,-6.56038841607153,
78.2760395720429));
#202606=CARTESIAN_POINT('Ctrl Pts',(1.83972934301116,-6.51477443503168,
78.2847893744151));
#202607=CARTESIAN_POINT('Ctrl Pts',(2.01818138406585,-6.46172066062041,
78.2935391767872));
#202608=CARTESIAN_POINT('Ctrl Pts',(2.19414528354525,-6.40140730423367,
78.3022889791594));
#202609=CARTESIAN_POINT('Ctrl Pts',(2.37010749864318,-6.34109452518523,
78.3110386977757));
#202610=CARTESIAN_POINT('Ctrl Pts',(2.5435813486677,-6.27352239616378,78.319788416392));
#202611=CARTESIAN_POINT('Ctrl Pts',(2.71397759435858,-6.19892043966686,
78.3285381350083));
#202612=CARTESIAN_POINT('Ctrl Pts',(2.88437226558419,-6.12431917249376,
78.337287772777));
#202613=CARTESIAN_POINT('Ctrl Pts',(3.05168912681244,-6.04268832278653,
78.3460374105457));
#202614=CARTESIAN_POINT('Ctrl Pts',(3.21535986274135,-5.95430516123182,
78.3547870483144));
#202615=CARTESIAN_POINT('Ctrl Pts',(3.37902914073126,-5.86592278697277,
78.3635366081435));
#202616=CARTESIAN_POINT('Ctrl Pts',(3.53905210621859,-5.77078835741766,
78.3722861679726));
#202617=CARTESIAN_POINT('Ctrl Pts',(3.69488522831986,-5.66922500431441,
78.3810357278017));
#202618=CARTESIAN_POINT('Ctrl Pts',(3.85071701407236,-5.56766252216889,
78.3897852125988));
#202619=CARTESIAN_POINT('Ctrl Pts',(4.00235878822706,-5.45967138329149,
78.3985346973959));
#202620=CARTESIAN_POINT('Ctrl Pts',(4.14929549611633,-5.34561838199369,
78.407284182193));
#202621=CARTESIAN_POINT('Ctrl Pts',(4.29623099276398,-5.23156632086763,
78.4160335948656));
#202622=CARTESIAN_POINT('Ctrl Pts',(4.43846127436336,-5.11145267304697,
78.4247830075382));
#202623=CARTESIAN_POINT('Ctrl Pts',(4.5755032605475,-4.98568540049603,78.4335324202108));
#202624=CARTESIAN_POINT('Ctrl Pts',(4.7125441625808,-4.85991912290071,78.4422817636661));
#202625=CARTESIAN_POINT('Ctrl Pts',(4.84439664019051,-4.72849950385122,
78.4510311071213));
#202626=CARTESIAN_POINT('Ctrl Pts',(4.97061286795025,-4.59187289860765,
78.4597804505765));
#202627=CARTESIAN_POINT('Ctrl Pts',(5.09682813912948,-4.45524732884383,
78.4685297277214));
#202628=CARTESIAN_POINT('Ctrl Pts',(5.21740705148085,-4.31341506235489,
78.4772790048662));
#202629=CARTESIAN_POINT('Ctrl Pts',(5.33194007545927,-4.16685781275429,
78.486028282011));
#202630=CARTESIAN_POINT('Ctrl Pts',(5.44647226944708,-4.0203016252154,78.4947774957521));
#202631=CARTESIAN_POINT('Ctrl Pts',(5.55495848628328,-3.86902074887626,
78.5035267094932));
#202632=CARTESIAN_POINT('Ctrl Pts',(5.65703027291994,-3.71352898080348,
78.5122759232344));
#202633=CARTESIAN_POINT('Ctrl Pts',(5.75910135377191,-3.55803828789274,
78.5210250764783));
#202634=CARTESIAN_POINT('Ctrl Pts',(5.85475793592935,-3.39833700106398,
78.5297742297221));
#202635=CARTESIAN_POINT('Ctrl Pts',(5.94367514427569,-3.2349675082324,78.538523382966));
#202636=CARTESIAN_POINT('Ctrl Pts',(6.03259176732793,-3.07159909077424,
78.5472724786189));
#202637=CARTESIAN_POINT('Ctrl Pts',(6.1147689683606,-2.90456276731147,78.5560215742719));
#202638=CARTESIAN_POINT('Ctrl Pts',(6.18992765548007,-2.73442583002777,
78.5647706699248));
#202639=CARTESIAN_POINT('Ctrl Pts',(6.26508587283174,-2.56428995615879,
78.5735197108928));
#202640=CARTESIAN_POINT('Ctrl Pts',(6.33322554827277,-2.39105376934892,
78.5822687518609));
#202641=CARTESIAN_POINT('Ctrl Pts',(6.39411526733144,-2.21530561053751,
78.5910177928289));
#202642=CARTESIAN_POINT('Ctrl Pts',(6.45500462602948,-2.03955849184779,
78.5997667820179));
#202643=CARTESIAN_POINT('Ctrl Pts',(6.50864402040829,-1.86129970164234,
78.608515771207));
#202644=CARTESIAN_POINT('Ctrl Pts',(6.55485128368678,-1.68113463135758,
78.617264760396));
#202645=CARTESIAN_POINT('Ctrl Pts',(6.60199809554391,-1.49730620116585,
78.6261916458674));
#202646=CARTESIAN_POINT('Ctrl Pts',(6.64140720707925,-1.31149343245431,
78.6351185313388));
#202647=CARTESIAN_POINT('Ctrl Pts',(6.67293928722926,-1.12435326697276,
78.6440454168102));
#202648=CARTESIAN_POINT('Ctrl Pts',(6.70384625876291,-0.940923067004143,
78.6527953309877));
#202649=CARTESIAN_POINT('Ctrl Pts',(6.72718554579823,-0.756217899519271,
78.6615452451652));
#202650=CARTESIAN_POINT('Ctrl Pts',(6.74287786815348,-0.570865181252157,
78.6702951593426));
#202651=CARTESIAN_POINT('Ctrl Pts',(6.75856988190858,-0.385516108071707,
78.6790449014471));
#202652=CARTESIAN_POINT('Ctrl Pts',(6.76661520773409,-0.199519795224209,
78.6877946435516));
#202653=CARTESIAN_POINT('Ctrl Pts',(6.76698651789579,-0.0135080204536151,
78.6965443856561));
#202654=CARTESIAN_POINT('Ctrl Pts',(6.76735782124898,0.172500343515016,
78.705293967321));
#202655=CARTESIAN_POINT('Ctrl Pts',(6.76005538995173,0.358523882212996,
78.714043548986));
#202656=CARTESIAN_POINT('Ctrl Pts',(6.74510402742344,0.543930748566469,
78.722793130651));
#202657=CARTESIAN_POINT('Ctrl Pts',(6.73015291918008,0.729334461617285,
78.7315425635077));
#202658=CARTESIAN_POINT('Ctrl Pts',(6.70755316306567,0.914121237636686,
78.7402919963643));
#202659=CARTESIAN_POINT('Ctrl Pts',(6.67738151874542,1.09766345166318,78.749041429221));
#202660=CARTESIAN_POINT('Ctrl Pts',(6.64721034747533,1.2812027879985,78.7577907248985));
#202661=CARTESIAN_POINT('Ctrl Pts',(6.60946757205103,1.46349731860504,78.7665400205761));
#202662=CARTESIAN_POINT('Ctrl Pts',(6.56428138111482,1.64392790278326,78.7752893162536));
#202663=CARTESIAN_POINT('Ctrl Pts',(6.51909583859806,1.82435589779211,78.7840384863792));
#202664=CARTESIAN_POINT('Ctrl Pts',(6.4664671639283,2.00291972192412,78.7927876565048));
#202665=CARTESIAN_POINT('Ctrl Pts',(6.40657409872836,2.17901292274802,78.8015368266304));
#202666=CARTESIAN_POINT('Ctrl Pts',(6.34668181342027,2.35510383059109,78.8102858828295));
#202667=CARTESIAN_POINT('Ctrl Pts',(6.27952541914,2.52872390822705,78.8190349390286));
#202668=CARTESIAN_POINT('Ctrl Pts',(6.20533299175465,2.69928350890404,78.8277839952277));
#202669=CARTESIAN_POINT('Ctrl Pts',(6.12831602991494,2.87633637965741,78.8368661313859));
#202670=CARTESIAN_POINT('Ctrl Pts',(6.04371690605212,3.05009086601578,78.8459482675441));
#202671=CARTESIAN_POINT('Ctrl Pts',(5.95184520316569,3.21991112882849,78.8550304037022));
#202672=CARTESIAN_POINT('Ctrl Pts',(5.86333549509206,3.38351691183135,78.8637801840458));
#202673=CARTESIAN_POINT('Ctrl Pts',(5.76807618099294,3.54347103712125,78.8725299643894));
#202674=CARTESIAN_POINT('Ctrl Pts',(5.66639083308935,3.6992301802782,78.881279744733));
#202675=CARTESIAN_POINT('Ctrl Pts',(5.56470914082114,3.85498372382174,78.8900292105179));
#202676=CARTESIAN_POINT('Ctrl Pts',(5.45660203371976,4.00654234702121,78.8987786763028));
#202677=CARTESIAN_POINT('Ctrl Pts',(5.34243669839121,4.15339127986792,78.9075281420877));
#202678=CARTESIAN_POINT('Ctrl Pts',(5.22827486050489,4.30023571401404,78.9162773398337));
#202679=CARTESIAN_POINT('Ctrl Pts',(5.10805534167001,4.44237052028596,78.9250265375797));
#202680=CARTESIAN_POINT('Ctrl Pts',(4.98218644339834,4.57931296628848,78.9337757353258));
#202681=CARTESIAN_POINT('Ctrl Pts',(4.85632073219466,4.71625194483485,78.9425247115374));
#202682=CARTESIAN_POINT('Ctrl Pts',(4.72480612170195,4.84799861524629,78.951273687749));
#202683=CARTESIAN_POINT('Ctrl Pts',(4.58808925235184,4.97410554898602,78.9600226639607));
#202684=CARTESIAN_POINT('Ctrl Pts',(4.45136349473924,5.10022068121315,78.9687722089624));
#202685=CARTESIAN_POINT('Ctrl Pts',(4.30943501209958,5.22069514871934,78.9775217539641));
#202686=CARTESIAN_POINT('Ctrl Pts',(4.16278587431664,5.33511975166349,78.9862712989658));
#202687=CARTESIAN_POINT('Ctrl Pts',(4.01614535740314,5.44953762807941,78.9950203296195));
#202688=CARTESIAN_POINT('Ctrl Pts',(3.86478496657775,5.55790617532888,79.0037693602732));
#202689=CARTESIAN_POINT('Ctrl Pts',(3.70921874747031,5.65985735539464,79.012518390927));
#202690=CARTESIAN_POINT('Ctrl Pts',(3.5536504160574,5.76180991977145,79.0212675403766));
#202691=CARTESIAN_POINT('Ctrl Pts',(3.39387638174367,5.85734478552903,79.0300166898262));
#202692=CARTESIAN_POINT('Ctrl Pts',(3.23043927904389,5.94613749121313,79.0387658392758));
#202693=CARTESIAN_POINT('Ctrl Pts',(3.1869176707033,5.969782069442,79.041095647192));
#202694=CARTESIAN_POINT('Ctrl Pts',(3.14313645919581,5.99294880633451,79.0434254551081));
#202695=CARTESIAN_POINT('Ctrl Pts',(3.09910619832139,6.01563211736937,79.0457552630242));
#202696=CARTESIAN_POINT('Ctrl Pts',(3.09910619832125,6.01563211736945,77.0457552630242));
#202697=CARTESIAN_POINT('Ctrl Pts',(2.93375330764817,6.10081787314658,77.0545047109265));
#202698=CARTESIAN_POINT('Ctrl Pts',(2.7648862784306,6.17918207037043,77.0632541588288));
#202699=CARTESIAN_POINT('Ctrl Pts',(2.59307866646692,6.25045854554001,77.0720036067311));
#202700=CARTESIAN_POINT('Ctrl Pts',(2.42127244185367,6.32173444515041,77.0807529839814));
#202701=CARTESIAN_POINT('Ctrl Pts',(2.24652594672455,6.38592262741841,77.0895023612317));
#202702=CARTESIAN_POINT('Ctrl Pts',(2.06943269687112,6.44280508110565,77.098251738482));
#202703=CARTESIAN_POINT('Ctrl Pts',(1.89234081822075,6.49968709436167,77.1070010479874));
#202704=CARTESIAN_POINT('Ctrl Pts',(1.71290249405593,6.54926340459543,77.1157503574927));
#202705=CARTESIAN_POINT('Ctrl Pts',(1.53172716625069,6.59136563150381,77.124499666998));
#202706=CARTESIAN_POINT('Ctrl Pts',(1.35055318107337,6.6334675464071,77.1332489116653));
#202707=CARTESIAN_POINT('Ctrl Pts',(1.16764249714414,6.66809542395777,77.1419981563325));
#202708=CARTESIAN_POINT('Ctrl Pts',(0.983616340614221,6.6951316562467,77.1507474009998));
#202709=CARTESIAN_POINT('Ctrl Pts',(0.799591486713706,6.72216769715962,
77.1594965837355));
#202710=CARTESIAN_POINT('Ctrl Pts',(0.614451459526574,6.74161215869372,
77.1682457664712));
#202711=CARTESIAN_POINT('Ctrl Pts',(0.428825047910143,6.75339900185713,
77.1769949492069));
#202712=CARTESIAN_POINT('Ctrl Pts',(0.243199888596877,6.76518576550222,
77.1857440729174));
#202713=CARTESIAN_POINT('Ctrl Pts',(0.0570886373917205,6.76931499599834,
77.194493196628));
#202714=CARTESIAN_POINT('Ctrl Pts',(-0.128876626811375,6.76577266947846,
77.2032423203385));
#202715=CARTESIAN_POINT('Ctrl Pts',(-0.314840698188391,6.76223036567992,
77.21199138793));
#202716=CARTESIAN_POINT('Ctrl Pts',(-0.500658497951491,6.75101660879221,
77.2207404555216));
#202717=CARTESIAN_POINT('Ctrl Pts',(-0.685698951926461,6.73216948296216,
77.2294895231131));
#202718=CARTESIAN_POINT('Ctrl Pts',(-0.870738280459878,6.71332247176292,
77.2382385374916));
#202719=CARTESIAN_POINT('Ctrl Pts',(-1.05499998761232,6.68684221356189,
77.2469875518701));
#202720=CARTESIAN_POINT('Ctrl Pts',(-1.23785829161379,6.6528186394853,77.2557365662487));
#202721=CARTESIAN_POINT('Ctrl Pts',(-1.43007412915399,6.61705395369235,
77.2649332999469));
#202722=CARTESIAN_POINT('Ctrl Pts',(-1.62073882531856,6.57295372728701,
77.2741300336452));
#202723=CARTESIAN_POINT('Ctrl Pts',(-1.809136960857,6.52068343479893,77.2833267673434));
#202724=CARTESIAN_POINT('Ctrl Pts',(-1.98838356180342,6.47095219816971,
77.2920767650571));
#202725=CARTESIAN_POINT('Ctrl Pts',(-2.16557827566814,6.41382586852822,
77.3008267627708));
#202726=CARTESIAN_POINT('Ctrl Pts',(-2.34011918616039,6.34949849945364,
77.3095767604844));
#202727=CARTESIAN_POINT('Ctrl Pts',(-2.514656556855,6.28517243497791,77.3183265807427));
#202728=CARTESIAN_POINT('Ctrl Pts',(-2.68653996289799,6.21364572244765,
77.3270764010011));
#202729=CARTESIAN_POINT('Ctrl Pts',(-2.85518555374534,6.13516132254759,
77.3358262212594));
#202730=CARTESIAN_POINT('Ctrl Pts',(-3.023827948533,6.05667841003197,77.3445758756969));
#202731=CARTESIAN_POINT('Ctrl Pts',(-3.18923239103964,5.97123819494921,
77.3533255301344));
#202732=CARTESIAN_POINT('Ctrl Pts',(-3.35083705962459,5.87913088813699,
77.3620751845719));
#202733=CARTESIAN_POINT('Ctrl Pts',(-3.51243888037233,5.78702520446239,
77.3708246848208));
#202734=CARTESIAN_POINT('Ctrl Pts',(-3.67024081218602,5.68825280609066,
77.3795741850698));
#202735=CARTESIAN_POINT('Ctrl Pts',(-3.82370687539398,5.58314917685931,
77.3883236853187));
#202736=CARTESIAN_POINT('Ctrl Pts',(-3.97717043812908,5.47804726011584,
77.3970730430092));
#202737=CARTESIAN_POINT('Ctrl Pts',(-4.12629803717655,5.36661448087931,
77.4058224006996));
#202738=CARTESIAN_POINT('Ctrl Pts',(-4.27058317202209,5.24922931208399,
77.4145717583901));
#202739=CARTESIAN_POINT('Ctrl Pts',(-4.41486614770225,5.13184589990755,
77.4233209851502));
#202740=CARTESIAN_POINT('Ctrl Pts',(-4.554306581899,5.00851045727138,77.4320702119102));
#202741=CARTESIAN_POINT('Ctrl Pts',(-4.68843088997433,4.87964187107359,
77.4408194386703));
#202742=CARTESIAN_POINT('Ctrl Pts',(-4.82255336913539,4.75077504212323,
77.4495685461262));
#202743=CARTESIAN_POINT('Ctrl Pts',(-4.95135966060956,4.61637541912574,
77.4583176535821));
#202744=CARTESIAN_POINT('Ctrl Pts',(-5.07441230865191,4.47689945406439,
77.4670667610381));
#202745=CARTESIAN_POINT('Ctrl Pts',(-5.19746344222487,4.33742520560224,
77.4758157608144));
#202746=CARTESIAN_POINT('Ctrl Pts',(-5.31476088450967,4.19287495496154,
77.4845647605908));
#202747=CARTESIAN_POINT('Ctrl Pts',(-5.42590627625186,4.04373961591627,
77.4933137603671));
#202748=CARTESIAN_POINT('Ctrl Pts',(-5.53706380669141,3.89458798911749,
77.5020637156618));
#202749=CARTESIAN_POINT('Ctrl Pts',(-5.64206777068481,3.74085050160387,
77.5108136709566));
#202750=CARTESIAN_POINT('Ctrl Pts',(-5.74056148160772,3.58304938228345,
77.5195636262513));
#202751=CARTESIAN_POINT('Ctrl Pts',(-5.83905138948787,3.4252543559856,77.5283132436924));
#202752=CARTESIAN_POINT('Ctrl Pts',(-5.931031395547,3.2633962550255,77.5370628611334));
#202753=CARTESIAN_POINT('Ctrl Pts',(-6.0161890781804,3.09802485070454,77.5458124785746));
#202754=CARTESIAN_POINT('Ctrl Pts',(-6.10134392542327,2.93265895255166,
77.5545618046904));
#202755=CARTESIAN_POINT('Ctrl Pts',(-6.17967677259329,2.76378023991631,
77.5633111308063));
#202756=CARTESIAN_POINT('Ctrl Pts',(-6.25092157006877,2.59196229232775,
77.5720604569222));
#202757=CARTESIAN_POINT('Ctrl Pts',(-6.32216437405561,2.42014915234817,
77.5808095382246));
#202758=CARTESIAN_POINT('Ctrl Pts',(-6.38631941546887,2.24539720668636,
77.5895586195271));
#202759=CARTESIAN_POINT('Ctrl Pts',(-6.44316881035664,2.06829994953524,
77.5983077008295));
#202760=CARTESIAN_POINT('Ctrl Pts',(-6.50002334522858,1.89118668030339,
77.6070575731719));
#202761=CARTESIAN_POINT('Ctrl Pts',(-6.54957082409546,1.71172794813635,
77.6158074455142));
#202762=CARTESIAN_POINT('Ctrl Pts',(-6.59164294294697,1.5305333425631,77.6245573178566));
#202763=CARTESIAN_POINT('Ctrl Pts',(-6.63371214080915,1.34935131699594,
77.6333065827115));
#202764=CARTESIAN_POINT('Ctrl Pts',(-6.66830695238639,1.16643393835776,
77.6420558475664));
#202765=CARTESIAN_POINT('Ctrl Pts',(-6.69530988153105,0.982402458401216,
77.6508051124213));
#202766=CARTESIAN_POINT('Ctrl Pts',(-6.72231419689764,0.798361531007603,
77.6595548264283));
#202767=CARTESIAN_POINT('Ctrl Pts',(-6.74172580828725,0.61320667142327,
77.6683045404354));
#202768=CARTESIAN_POINT('Ctrl Pts',(-6.75347878027793,0.427566795174375,
77.6770542544424));
#202769=CARTESIAN_POINT('Ctrl Pts',(-6.76248992366069,0.285234494564716,
77.6837627642166));
#202770=CARTESIAN_POINT('Ctrl Pts',(-6.76699999997978,0.142617266751198,
77.6904712739908));
#202771=CARTESIAN_POINT('Ctrl Pts',(-6.767,9.5948989328826E-10,77.697179783765));
#202772=CARTESIAN_POINT('',(-6.76699925239411,0.00318089572253539,77.3028202162312));
#202773=CARTESIAN_POINT('Ctrl Pts',(3.09910619832139,6.01563211736937,76.6513581962709));
#202774=CARTESIAN_POINT('Ctrl Pts',(2.99281630860975,6.07039006293475,76.6570008096127));
#202775=CARTESIAN_POINT('Ctrl Pts',(2.88509649128983,6.12231922629877,76.6626434229546));
#202776=CARTESIAN_POINT('Ctrl Pts',(2.77609525020218,6.17135189093969,76.6682860362965));
#202777=CARTESIAN_POINT('Ctrl Pts',(2.60895175081397,6.24653902707351,76.67693847117));
#202778=CARTESIAN_POINT('Ctrl Pts',(2.43864473878715,6.31498012337952,76.6855909060436));
#202779=CARTESIAN_POINT('Ctrl Pts',(2.2657338029222,6.37642057382476,76.6942433409172));
#202780=CARTESIAN_POINT('Ctrl Pts',(2.09298300908987,6.43780412099452,76.7028877623097));
#202781=CARTESIAN_POINT('Ctrl Pts',(1.91763338705729,6.492199852584,76.7115321837023));
#202782=CARTESIAN_POINT('Ctrl Pts',(1.7402643927085,6.53940126031971,76.7201766050948));
#202783=CARTESIAN_POINT('Ctrl Pts',(1.55720029904399,6.58811824695285,76.7290985881804));
#202784=CARTESIAN_POINT('Ctrl Pts',(1.37198528946647,6.62917107903984,76.7380205712659));
#202785=CARTESIAN_POINT('Ctrl Pts',(1.18527566951571,6.6623877541955,76.7469425543514));
#202786=CARTESIAN_POINT('Ctrl Pts',(1.00471992640263,6.69450962058919,76.7555704723263));
#202787=CARTESIAN_POINT('Ctrl Pts',(0.822766852872387,6.71930357141152,
76.7641983903011));
#202788=CARTESIAN_POINT('Ctrl Pts',(0.640022910290413,6.7366653230143,76.772826308276));
#202789=CARTESIAN_POINT('Ctrl Pts',(0.447936281930944,6.75491468482993,
76.7818953239169));
#202790=CARTESIAN_POINT('Ctrl Pts',(0.254976129764303,6.76495192010977,
76.7909643395577));
#202791=CARTESIAN_POINT('Ctrl Pts',(0.061856499368857,6.76671728192377,
76.8000333551986));
#202792=CARTESIAN_POINT('Ctrl Pts',(-0.131263131026525,6.76848264373778,
76.8091023708395));
#202793=CARTESIAN_POINT('Ctrl Pts',(-0.32454184880341,6.76197609319795,
76.8181713864804));
#202794=CARTESIAN_POINT('Ctrl Pts',(-0.51726136391349,6.74720161855286,
76.8272404021212));
#202795=CARTESIAN_POINT('Ctrl Pts',(-0.696326350455738,6.73347394233917,
76.8356668614902));
#202796=CARTESIAN_POINT('Ctrl Pts',(-0.874829202650989,6.71261476296558,
76.8440933208592));
#202797=CARTESIAN_POINT('Ctrl Pts',(-1.05218417540381,6.68469875619162,
76.8525197802282));
#202798=CARTESIAN_POINT('Ctrl Pts',(-1.22958109821798,6.65677614639899,
76.8609482327213));
#202799=CARTESIAN_POINT('Ctrl Pts',(-1.40582927286509,6.62179343263393,
76.8693766852145));
#202800=CARTESIAN_POINT('Ctrl Pts',(-1.58035202400563,6.57987663107914,
76.8778051377077));
#202801=CARTESIAN_POINT('Ctrl Pts',(-1.75493964854348,6.53794424825884,
76.8862367232156));
#202802=CARTESIAN_POINT('Ctrl Pts',(-1.92780024864766,6.48907271559709,
76.8946683087235));
#202803=CARTESIAN_POINT('Ctrl Pts',(-2.09837082971887,6.43343833894326,
76.9030998942314));
#202804=CARTESIAN_POINT('Ctrl Pts',(-2.26909933190827,6.37775245374137,
76.9115392860409));
#202805=CARTESIAN_POINT('Ctrl Pts',(-2.43753326381252,6.31529131779788,
76.9199786778504));
#202806=CARTESIAN_POINT('Ctrl Pts',(-2.60312712465974,6.24628034696336,
76.92841806966));
#202807=CARTESIAN_POINT('Ctrl Pts',(-2.76880834318714,6.17723296995842,
76.9368619136013));
#202808=CARTESIAN_POINT('Ctrl Pts',(-2.93164620001799,6.10162900134795,
76.9453057575427));
#202809=CARTESIAN_POINT('Ctrl Pts',(-3.09111792290226,6.01974077404604,
76.953749601484));
#202810=CARTESIAN_POINT('Ctrl Pts',(-3.25075828289685,5.93776595211925,
76.962202374566));
#202811=CARTESIAN_POINT('Ctrl Pts',(-3.40702510742384,5.84949375477547,
76.9706551476479));
#202812=CARTESIAN_POINT('Ctrl Pts',(-3.55942190022044,5.75524150112149,
76.9791079207299));
#202813=CARTESIAN_POINT('Ctrl Pts',(-3.60201197790986,5.72890098087916,
76.9814702031352));
#202814=CARTESIAN_POINT('Ctrl Pts',(-3.64429997750867,5.7020936581561,76.9838324855406));
#202815=CARTESIAN_POINT('Ctrl Pts',(-3.68627549597668,5.67482704298218,
76.9861947679459));
#202816=CARTESIAN_POINT('Ctrl Pts',(-3.83391101635315,5.57892540633714,
76.9945033441093));
#202817=CARTESIAN_POINT('Ctrl Pts',(-3.977946997598,5.47716448481761,77.0028119202726));
#202818=CARTESIAN_POINT('Ctrl Pts',(-4.1178974369687,5.36984261395123,77.011120496436));
#202819=CARTESIAN_POINT('Ctrl Pts',(-4.25772887211959,5.26261200221608,
77.0194220075581));
#202820=CARTESIAN_POINT('Ctrl Pts',(-4.39348141141764,5.14983007320495,
77.0277235186802));
#202821=CARTESIAN_POINT('Ctrl Pts',(-4.5246976870573,5.03183861433754,77.0360250298023));
#202822=CARTESIAN_POINT('Ctrl Pts',(-4.65582664447303,4.91392567320413,
77.0443210166615));
#202823=CARTESIAN_POINT('Ctrl Pts',(-4.78242509459466,4.79081034221048,
77.0526170035207));
#202824=CARTESIAN_POINT('Ctrl Pts',(-4.90406829011053,4.66287499359916,
77.0609129903799));
#202825=CARTESIAN_POINT('Ctrl Pts',(-5.02565301772346,4.5350011372194,77.0692049897662));
#202826=CARTESIAN_POINT('Ctrl Pts',(-5.1422869973124,4.40231213236403,77.0774969891524));
#202827=CARTESIAN_POINT('Ctrl Pts',(-5.25358179426859,4.2652276997752,77.0857889885386));
#202828=CARTESIAN_POINT('Ctrl Pts',(-5.36484365830891,4.12818383143743,
77.0940785342637));
#202829=CARTESIAN_POINT('Ctrl Pts',(-5.47076926924061,3.98674739831546,
77.1023680799888));
#202830=CARTESIAN_POINT('Ctrl Pts',(-5.57100986993585,3.84137189413851,
77.1106576257139));
#202831=CARTESIAN_POINT('Ctrl Pts',(-5.671260739849,3.69598149686717,77.1189480206672));
#202832=CARTESIAN_POINT('Ctrl Pts',(-5.76582523161551,3.54665150508406,
77.1272384156206));
#202833=CARTESIAN_POINT('Ctrl Pts',(-5.85439708039725,3.39386561682046,
77.135528810574));
#202834=CARTESIAN_POINT('Ctrl Pts',(-5.94297809515259,3.24106391730942,
77.1438200634697));
#202835=CARTESIAN_POINT('Ctrl Pts',(-6.02556505536327,3.08480591015634,
77.1521113163654));
#202836=CARTESIAN_POINT('Ctrl Pts',(-6.10189701660318,2.92560110041837,
77.1604025692611));
#202837=CARTESIAN_POINT('Ctrl Pts',(-6.17824966789225,2.76635313765138,
77.1686960695304));
#202838=CARTESIAN_POINT('Ctrl Pts',(-6.24834379031075,2.60415709500604,
77.1769895697996));
#202839=CARTESIAN_POINT('Ctrl Pts',(-6.31196599249762,2.4395438732586,77.1852830700689));
#202840=CARTESIAN_POINT('Ctrl Pts',(-6.37561610182397,2.27485844583481,
77.1935802081857));
#202841=CARTESIAN_POINT('Ctrl Pts',(-6.43278850760393,2.10775405146005,
77.2018773463024));
#202842=CARTESIAN_POINT('Ctrl Pts',(-6.48331916495928,1.93877837961736,
77.2101744844191));
#202843=CARTESIAN_POINT('Ctrl Pts',(-6.53390992209061,1.76960173275166,
77.2184814909241));
#202844=CARTESIAN_POINT('Ctrl Pts',(-6.57784304819629,1.59854969635067,
77.2267884974291));
#202845=CARTESIAN_POINT('Ctrl Pts',(-6.61500499862981,1.42618297146709,
77.235095503934));
#202846=CARTESIAN_POINT('Ctrl Pts',(-6.65219072891959,1.25370594946787,
77.2434078260755));
#202847=CARTESIAN_POINT('Ctrl Pts',(-6.682596583137,1.07991290447914,77.2517201482169));
#202848=CARTESIAN_POINT('Ctrl Pts',(-6.70616071005493,0.905371487796915,
77.2600324703583));
#202849=CARTESIAN_POINT('Ctrl Pts',(-6.72975994054969,0.730570056048034,
77.2683571754003));
#202850=CARTESIAN_POINT('Ctrl Pts',(-6.74649704300768,0.55501837173379,
77.2766818804423));
#202851=CARTESIAN_POINT('Ctrl Pts',(-6.75636219965656,0.379287261916324,
77.2850065854842));
#202852=CARTESIAN_POINT('Ctrl Pts',(-6.76339885567066,0.253941115395554,
77.2909444623861));
#202853=CARTESIAN_POINT('Ctrl Pts',(-6.76694034313661,0.128503706369033,
77.296882339288));
#202854=CARTESIAN_POINT('Ctrl Pts',(-6.7669992523937,0.00318089659341924,
77.3028202161899));
#202855=CARTESIAN_POINT('Ctrl Pts',(-6.76699925239411,0.0031808957225354,
77.3028202162312));
#202856=CARTESIAN_POINT('Ctrl Pts',(-6.7670034961808,-0.00584728497919235,
77.3032479773526));
#202857=CARTESIAN_POINT('Ctrl Pts',(-6.76698967266099,-0.0148756381434245,
77.3036757384741));
#202858=CARTESIAN_POINT('Ctrl Pts',(-6.76695777975772,-0.0239041204926956,
77.3041034995956));
#202859=CARTESIAN_POINT('Ctrl Pts',(-6.76635609879876,-0.194232480717908,
77.3121734993558));
#202860=CARTESIAN_POINT('Ctrl Pts',(-6.75931813085109,-0.364852553213374,
77.3202434991159));
#202861=CARTESIAN_POINT('Ctrl Pts',(-6.74580030092629,-0.535226400715402,
77.328313498876));
#202862=CARTESIAN_POINT('Ctrl Pts',(-6.73229947583749,-0.705385925404503,
77.3363733469311));
#202863=CARTESIAN_POINT('Ctrl Pts',(-6.7123350369203,-0.875299474224632,
77.3444331949862));
#202864=CARTESIAN_POINT('Ctrl Pts',(-6.6859152800386,-1.04442609510985,
77.3524930430413));
#202865=CARTESIAN_POINT('Ctrl Pts',(-6.65952296016933,-1.21337707739172,
77.3605445209152));
#202866=CARTESIAN_POINT('Ctrl Pts',(-6.62668872020822,-1.38154239255614,
77.3685959987892));
#202867=CARTESIAN_POINT('Ctrl Pts',(-6.58747281898622,-1.54838330497255,
77.3766474766631));
#202868=CARTESIAN_POINT('Ctrl Pts',(-6.54828905067751,-1.71508751048173,
77.3846923572785));
#202869=CARTESIAN_POINT('Ctrl Pts',(-6.50273411351098,-1.88046911180129,
77.3927372378938));
#202870=CARTESIAN_POINT('Ctrl Pts',(-6.45091978386893,-2.04399680579214,
77.4007821185092));
#202871=CARTESIAN_POINT('Ctrl Pts',(-6.39913656869029,-2.20742630153382,
77.4088221681802));
#202872=CARTESIAN_POINT('Ctrl Pts',(-6.34110155597938,-2.36900375136368,
77.4168622178512));
#202873=CARTESIAN_POINT('Ctrl Pts',(-6.27697706098986,-2.52821042949497,
77.4249022675222));
#202874=CARTESIAN_POINT('Ctrl Pts',(-6.2114738541361,-2.69084013865428,
77.4331151826773));
#202875=CARTESIAN_POINT('Ctrl Pts',(-6.13961643550004,-2.85099558755428,
77.4413280978324));
#202876=CARTESIAN_POINT('Ctrl Pts',(-6.06163090484721,-3.00814224620467,
77.4495410129875));
#202877=CARTESIAN_POINT('Ctrl Pts',(-5.98531343435147,-3.16192763927256,
77.4575782591893));
#202878=CARTESIAN_POINT('Ctrl Pts',(-5.90312753748605,-3.31283131003964,
77.4656155053911));
#202879=CARTESIAN_POINT('Ctrl Pts',(-5.81533275626469,-3.46037482563882,
77.4736527515929));
#202880=CARTESIAN_POINT('Ctrl Pts',(-5.72752956685935,-3.60793247161122,
77.4816907675289));
#202881=CARTESIAN_POINT('Ctrl Pts',(-5.63411661445339,-3.75212900050376,
77.4897287834649));
#202882=CARTESIAN_POINT('Ctrl Pts',(-5.53539798233441,-3.89251309274203,
77.4977667994009));
#202883=CARTESIAN_POINT('Ctrl Pts',(-5.43665033767426,-4.03293844263521,
77.5058071776393));
#202884=CARTESIAN_POINT('Ctrl Pts',(-5.33259412436941,-4.16954882023107,
77.5138475558778));
#202885=CARTESIAN_POINT('Ctrl Pts',(-5.22357498902705,-4.30192437567318,
77.5218879341162));
#202886=CARTESIAN_POINT('Ctrl Pts',(-5.11044324347957,-4.43929363298708,
77.5302316255436));
#202887=CARTESIAN_POINT('Ctrl Pts',(-4.99196711566391,-4.57210198637334,
77.538575316971));
#202888=CARTESIAN_POINT('Ctrl Pts',(-4.86857559278257,-4.69992135012512,
77.5469190083984));
#202889=CARTESIAN_POINT('Ctrl Pts',(-4.74946264636408,-4.82330860291436,
77.5549733839885));
#202890=CARTESIAN_POINT('Ctrl Pts',(-4.62576979130375,-4.94204685259125,
77.5630277595787));
#202891=CARTESIAN_POINT('Ctrl Pts',(-4.4979170327914,-5.05579186341023,
77.5710821351688));
#202892=CARTESIAN_POINT('Ctrl Pts',(-4.36996859712787,-5.16962199400856,
77.5791425381589));
#202893=CARTESIAN_POINT('Ctrl Pts',(-4.23785434596213,-5.27845120972642,
77.587202941149));
#202894=CARTESIAN_POINT('Ctrl Pts',(-4.10202415288264,-5.38197796810498,
77.5952633441391));
#202895=CARTESIAN_POINT('Ctrl Pts',(-3.96600407471664,-5.48564945268194,
77.6033350152448));
#202896=CARTESIAN_POINT('Ctrl Pts',(-3.82625799285657,-5.58400347747621,
77.6114066863504));
#202897=CARTESIAN_POINT('Ctrl Pts',(-3.68326177367805,-5.67678357052319,
77.6194783574561));
#202898=CARTESIAN_POINT('Ctrl Pts',(-3.66829856193257,-5.68649213614824,
77.6203229820524));
#202899=CARTESIAN_POINT('Ctrl Pts',(-3.65329978129029,-5.69613971216436,
77.6211676066487));
#202900=CARTESIAN_POINT('Ctrl Pts',(-3.63826598985281,-5.70572603505289,
77.622012231245));
#202901=CARTESIAN_POINT('Ctrl Pts',(-3.49178978095392,-5.79912684081984,
77.630241519866));
#202902=CARTESIAN_POINT('Ctrl Pts',(-3.3414993947806,-5.88702079688458,
77.638470808487));
#202903=CARTESIAN_POINT('Ctrl Pts',(-3.1878464031111,-5.96908069221481,
77.646700097108));
#202904=CARTESIAN_POINT('Ctrl Pts',(-3.03437627491775,-6.05104292750244,
77.6549195919963));
#202905=CARTESIAN_POINT('Ctrl Pts',(-2.87755182299575,-6.12718476003757,
77.6631390868847));
#202906=CARTESIAN_POINT('Ctrl Pts',(-2.71785402812939,-6.19722183577293,
77.671358581773));
#202907=CARTESIAN_POINT('Ctrl Pts',(-2.55831422038495,-6.26718962466541,
77.6795699452132));
#202908=CARTESIAN_POINT('Ctrl Pts',(-2.39590705676496,-6.33106454094299,
77.6877813086534));
#202909=CARTESIAN_POINT('Ctrl Pts',(-2.23113866516536,-6.38860777140092,
77.6959926720936));
#202910=CARTESIAN_POINT('Ctrl Pts',(-2.06650020033913,-6.44610562661307,
77.70419756053));
#202911=CARTESIAN_POINT('Ctrl Pts',(-1.89950455311075,-6.49728162276076,
77.7124024489664));
#202912=CARTESIAN_POINT('Ctrl Pts',(-1.73067849209804,-6.54194473814853,
77.7206073374028));
#202913=CARTESIAN_POINT('Ctrl Pts',(-1.56195167504958,-6.58658159843919,
77.7288074026167));
#202914=CARTESIAN_POINT('Ctrl Pts',(-1.3913969335109,-6.62471311340633,
77.7370074678306));
#202915=CARTESIAN_POINT('Ctrl Pts',(-1.2195569702114,-6.65619784835223,
77.7452075330445));
#202916=CARTESIAN_POINT('Ctrl Pts',(-1.04776673447968,-6.68767347215039,
77.7534052252988));
#202917=CARTESIAN_POINT('Ctrl Pts',(-0.874692369420627,-6.71250607877256,
77.761602917553));
#202918=CARTESIAN_POINT('Ctrl Pts',(-0.700887814206145,-6.73060511929628,
77.7698006098073));
#202919=CARTESIAN_POINT('Ctrl Pts',(-0.527106528455025,-6.74870173666741,
77.7779972045305));
#202920=CARTESIAN_POINT('Ctrl Pts',(-0.352595603862347,-6.76006654543032,
77.7861937992537));
#202921=CARTESIAN_POINT('Ctrl Pts',(-0.177915176489748,-6.76466075941541,
77.7943903939769));
#202922=CARTESIAN_POINT('Ctrl Pts',(-0.00322637531430903,-6.76925519363721,
77.8025873816272));
#202923=CARTESIAN_POINT('Ctrl Pts',(0.171631586183683,-6.76707837697295,
77.8107843692774));
#202924=CARTESIAN_POINT('Ctrl Pts',(0.346097434095885,-6.75814364793412,
77.8189813569277));
#202925=CARTESIAN_POINT('Ctrl Pts',(0.520603366968703,-6.74920686606795,
77.8271802279032));
#202926=CARTESIAN_POINT('Ctrl Pts',(0.69471664861912,-6.73350909768876,
77.8353790988787));
#202927=CARTESIAN_POINT('Ctrl Pts',(0.867879937213135,-6.71111566094513,
77.8435779698541));
#202928=CARTESIAN_POINT('Ctrl Pts',(1.04120723211177,-6.68870101494381,
77.8517846061391));
#202929=CARTESIAN_POINT('Ctrl Pts',(1.21358238007501,-6.65957807671737,
77.8599912424241));
#202930=CARTESIAN_POINT('Ctrl Pts',(1.38445612301583,-6.62386369450972,
77.868197878709));
#202931=CARTESIAN_POINT('Ctrl Pts',(1.55541257027319,-6.58813202624326,
77.8764084870744));
#202932=CARTESIAN_POINT('Ctrl Pts',(1.72486581581406,-6.54580264016105,
77.8846190954398));
#202933=CARTESIAN_POINT('Ctrl Pts',(1.8922807084994,-6.49704261339273,77.8928297038051));
#202934=CARTESIAN_POINT('Ctrl Pts',(2.05992648291789,-6.44821534171382,
77.9010516354134));
#202935=CARTESIAN_POINT('Ctrl Pts',(2.22552794612087,-6.39293981922132,
77.9092735670216));
#202936=CARTESIAN_POINT('Ctrl Pts',(2.38856775122155,-6.33143215219309,
77.9174954986298));
#202937=CARTESIAN_POINT('Ctrl Pts',(2.53679907111127,-6.27551106800569,
77.9249706533847));
#202938=CARTESIAN_POINT('Ctrl Pts',(2.68291301063721,-6.21443920689228,
77.9324458081395));
#202939=CARTESIAN_POINT('Ctrl Pts',(2.82653848469758,-6.14841192459675,
77.9399209628944));
#202940=CARTESIAN_POINT('Ctrl Pts',(2.99822540390185,-6.06948427784806,
77.9488566081818));
#202941=CARTESIAN_POINT('Ctrl Pts',(3.16671399792719,-5.98331117677076,
77.9577922534692));
#202942=CARTESIAN_POINT('Ctrl Pts',(3.33140873755182,-5.89016169755665,
77.9667278987566));
#202943=CARTESIAN_POINT('Ctrl Pts',(3.49585590525969,-5.79715224221438,
77.975650111831));
#202944=CARTESIAN_POINT('Ctrl Pts',(3.65652037369879,-5.69718746075504,
77.9845723249053));
#202945=CARTESIAN_POINT('Ctrl Pts',(3.81282991248378,-5.59058289076094,
77.9934945379797));
#202946=CARTESIAN_POINT('Ctrl Pts',(3.96875653449884,-5.48423947359167,
78.0023948940065));
#202947=CARTESIAN_POINT('Ctrl Pts',(4.12034930615262,-5.37128887660934,
78.0112952500334));
#202948=CARTESIAN_POINT('Ctrl Pts',(4.26706426309935,-5.25209021005736,
78.0201956060603));
#202949=CARTESIAN_POINT('Ctrl Pts',(4.41355256407153,-5.13307569030606,
78.0290822121675));
#202950=CARTESIAN_POINT('Ctrl Pts',(4.55517788244426,-5.00783251716709,
78.0379688182747));
#202951=CARTESIAN_POINT('Ctrl Pts',(4.69142623686737,-4.87676212912138,
78.0468554243819));
#202952=CARTESIAN_POINT('Ctrl Pts',(4.82732454476724,-4.74602848447216,
78.0557191992));
#202953=CARTESIAN_POINT('Ctrl Pts',(4.95787326881555,-4.60949767734603,
78.0645829740182));
#202954=CARTESIAN_POINT('Ctrl Pts',(5.08259301445811,-4.46760979153077,
78.0734467488363));
#202955=CARTESIAN_POINT('Ctrl Pts',(5.20185920672812,-4.33192616113814,
78.0819229421307));
#202956=CARTESIAN_POINT('Ctrl Pts',(5.31579507035545,-4.19134408557049,
78.090399135425));
#202957=CARTESIAN_POINT('Ctrl Pts',(5.42401037482033,-4.04628230031488,
78.0988753287194));
#202958=CARTESIAN_POINT('Ctrl Pts',(5.5288150275785,-3.90579246750081,78.1070843754834));
#202959=CARTESIAN_POINT('Ctrl Pts',(5.62815222232991,-3.76123570369797,
78.1152934222473));
#202960=CARTESIAN_POINT('Ctrl Pts',(5.72170744990241,-3.61308079867187,
78.1235024690113));
#202961=CARTESIAN_POINT('Ctrl Pts',(5.81528494302509,-3.46489063371899,
78.1317134694763));
#202962=CARTESIAN_POINT('Ctrl Pts',(5.90307753732829,-3.31310092255337,
78.1399244699413));
#202963=CARTESIAN_POINT('Ctrl Pts',(5.98481544779825,-3.15820725345812,
78.1481354704063));
#202964=CARTESIAN_POINT('Ctrl Pts',(6.06658737979926,-3.00324911342468,
78.156349888512));
#202965=CARTESIAN_POINT('Ctrl Pts',(6.14229944130406,-2.84518475627035,
78.1645643066176));
#202966=CARTESIAN_POINT('Ctrl Pts',(6.21172893037401,-2.68453211855521,
78.1727787247233));
#202967=CARTESIAN_POINT('Ctrl Pts',(6.28123658616688,-2.5236986111493,78.1810023909763));
#202968=CARTESIAN_POINT('Ctrl Pts',(6.34444740071612,-2.36027132994105,
78.1892260572292));
#202969=CARTESIAN_POINT('Ctrl Pts',(6.40118739729601,-2.19478675608787,
78.1974497234822));
#202970=CARTESIAN_POINT('Ctrl Pts',(6.45796377112014,-2.02919608647997,
78.2056786621063));
#202971=CARTESIAN_POINT('Ctrl Pts',(6.50826095498072,-1.86154583509582,
78.2139076007304));
#202972=CARTESIAN_POINT('Ctrl Pts',(6.551955547683,-1.69238515154973,78.2221365393544));
#202973=CARTESIAN_POINT('Ctrl Pts',(6.59571028861772,-1.52299160815792,
78.230376805607));
#202974=CARTESIAN_POINT('Ctrl Pts',(6.63284420883924,-1.3520838265177,78.2386170718595));
#202975=CARTESIAN_POINT('Ctrl Pts',(6.66328527878965,-1.18021959544197,
78.2468573381121));
#202976=CARTESIAN_POINT('Ctrl Pts',(6.67679658451016,-1.10393744858353,
78.2505147902561));
#202977=CARTESIAN_POINT('Ctrl Pts',(6.68899005946708,-1.02746692907892,
78.2541722424001));
#202978=CARTESIAN_POINT('Ctrl Pts',(6.69986269242552,-0.95085693069184,
78.2578296945441));
#202979=CARTESIAN_POINT('Ctrl Pts',(6.72497633512527,-0.773902909151978,
78.2662776893111));
#202980=CARTESIAN_POINT('Ctrl Pts',(6.74309704629527,-0.595799682392562,
78.2747256840781));
#202981=CARTESIAN_POINT('Ctrl Pts',(6.75413168918437,-0.417126030301919,
78.2831736788451));
#202982=CARTESIAN_POINT('Ctrl Pts',(6.76515622657292,-0.238616007130643,
78.291613936958));
#202983=CARTESIAN_POINT('Ctrl Pts',(6.76910761052382,-0.0595369311969636,
78.3000541950708));
#202984=CARTESIAN_POINT('Ctrl Pts',(6.76594432205611,0.119525858443792,
78.3084944531836));
#202985=CARTESIAN_POINT('Ctrl Pts',(6.76278344352315,0.298452230035839,
78.31692828113));
#202986=CARTESIAN_POINT('Ctrl Pts',(6.75251870377821,0.477362007777319,
78.3253621090764));
#202987=CARTESIAN_POINT('Ctrl Pts',(6.73516061201328,0.655668003172985,
78.3337959370228));
#202988=CARTESIAN_POINT('Ctrl Pts',(6.71781307574966,0.833865570223439,
78.3422246363362));
#202989=CARTESIAN_POINT('Ctrl Pts',(6.6933808196366,1.01145975582435,78.3506533356496));
#202990=CARTESIAN_POINT('Ctrl Pts',(6.66192635602018,1.18786624961048,78.3590820349631));
#202991=CARTESIAN_POINT('Ctrl Pts',(6.63048618943762,1.36419256114826,78.36750690317));
#202992=CARTESIAN_POINT('Ctrl Pts',(6.5920302382928,1.53933192953616,78.375931771377));
#202993=CARTESIAN_POINT('Ctrl Pts',(6.54667255803846,1.71270762765458,78.3843566395839));
#202994=CARTESIAN_POINT('Ctrl Pts',(6.50132492192615,1.88604493293353,78.3927796421625));
#202995=CARTESIAN_POINT('Ctrl Pts',(6.44907868569588,2.0576190236097,78.4012026447411));
#202996=CARTESIAN_POINT('Ctrl Pts',(6.39009859827946,2.22686526405773,78.4096256473198));
#202997=CARTESIAN_POINT('Ctrl Pts',(6.33112518559704,2.39609235103065,78.4180476966732));
#202998=CARTESIAN_POINT('Ctrl Pts',(6.265419550659,2.56299179811782,78.4264697460267));
#202999=CARTESIAN_POINT('Ctrl Pts',(6.19319581895587,2.72701568533581,78.4348917953802));
#203000=CARTESIAN_POINT('Ctrl Pts',(6.12097017831694,2.89104390784724,78.4433140673357));
#203001=CARTESIAN_POINT('Ctrl Pts',(6.04222623217052,3.05219611391376,78.4517363392913));
#203002=CARTESIAN_POINT('Ctrl Pts',(5.95722575605389,3.20994552779455,78.4601586112468));
#203003=CARTESIAN_POINT('Ctrl Pts',(5.87221116653224,3.3677211342506,78.4685822816291));
#203004=CARTESIAN_POINT('Ctrl Pts',(5.78093813462091,3.52209252883972,78.4770059520113));
#203005=CARTESIAN_POINT('Ctrl Pts',(5.68371395501394,3.67255832868313,78.4854296223935));
#203006=CARTESIAN_POINT('Ctrl Pts',(5.58642398122583,3.82312595272429,78.4938589932969));
#203007=CARTESIAN_POINT('Ctrl Pts',(5.48317499339245,3.96978242025217,78.5022883642004));
#203008=CARTESIAN_POINT('Ctrl Pts',(5.37431768637092,4.11205525327187,78.5107177351038));
#203009=CARTESIAN_POINT('Ctrl Pts',(5.26542153821299,4.25437885034834,78.5191501136725));
#203010=CARTESIAN_POINT('Ctrl Pts',(5.15091328830068,4.3923154330655,78.5275824922412));
#203011=CARTESIAN_POINT('Ctrl Pts',(5.03118370671966,4.52542589258057,78.53601487081));
#203012=CARTESIAN_POINT('Ctrl Pts',(4.91134334234396,4.65865951588283,78.5444550516482));
#203013=CARTESIAN_POINT('Ctrl Pts',(4.78627222134462,4.78705785004376,78.5528952324864));
#203014=CARTESIAN_POINT('Ctrl Pts',(4.65639849937839,4.91021812295408,78.5613354133247));
#203015=CARTESIAN_POINT('Ctrl Pts',(4.58252279597567,4.98027503404259,78.5661364176143));
#203016=CARTESIAN_POINT('Ctrl Pts',(4.50709378487479,5.04863779999002,78.5709374219039));
#203017=CARTESIAN_POINT('Ctrl Pts',(4.43019502857091,5.11523811848732,78.5757384261936));
#203018=CARTESIAN_POINT('Ctrl Pts',(4.29981660656457,5.22815599711311,78.5838783154898));
#203019=CARTESIAN_POINT('Ctrl Pts',(4.16495145988663,5.33623038679091,78.5920182047859));
#203020=CARTESIAN_POINT('Ctrl Pts',(4.02599897334997,5.43908275967419,78.6001580940821));
#203021=CARTESIAN_POINT('Ctrl Pts',(3.87987442953529,5.54724387605595,78.6087181252104));
#203022=CARTESIAN_POINT('Ctrl Pts',(3.72922967744379,5.64962931001102,78.6172781563387));
#203023=CARTESIAN_POINT('Ctrl Pts',(3.57457188011347,5.74584413936735,78.625838187467));
#203024=CARTESIAN_POINT('Ctrl Pts',(3.42774035267585,5.837190134205,78.6339650486222));
#203025=CARTESIAN_POINT('Ctrl Pts',(3.27729224908201,5.92297436546511,78.6420919097774));
#203026=CARTESIAN_POINT('Ctrl Pts',(3.12369381422815,6.00290146137289,78.6502187709327));
#203027=CARTESIAN_POINT('Ctrl Pts',(3.11550686128119,6.0071616569537,78.6506519409057));
#203028=CARTESIAN_POINT('Ctrl Pts',(3.10731096502865,6.01140522269527,78.6510851108788));
#203029=CARTESIAN_POINT('Ctrl Pts',(3.09910619832128,6.01563211736943,78.6515182808518));
#203030=CARTESIAN_POINT('Origin',(0.,0.,4.30282021618968));
#203031=CARTESIAN_POINT('',(3.09910619832132,6.01563211736941,81.0456744569491));
#203032=CARTESIAN_POINT('',(3.0991061983213,6.01563211736942,80.6514477536361));
#203033=CARTESIAN_POINT('',(3.09910619832133,6.0156321173694,4.30282021618968));
#203034=CARTESIAN_POINT('',(-6.76705444505815,-9.75274733681431E-5,79.6970855167737));
#203035=CARTESIAN_POINT('Ctrl Pts',(-6.7669997635994,-0.00178869944433293,
79.69717978381));
#203036=CARTESIAN_POINT('Ctrl Pts',(-6.76695191418748,-0.182812381294488,
79.7056559560052));
#203037=CARTESIAN_POINT('Ctrl Pts',(-6.75963595610949,-0.363702158404258,
79.7141321282003));
#203038=CARTESIAN_POINT('Ctrl Pts',(-6.74510958551482,-0.543861820130901,
79.7226083003955));
#203039=CARTESIAN_POINT('Ctrl Pts',(-6.73055597313459,-0.7243593412588,
79.731100368238));
#203040=CARTESIAN_POINT('Ctrl Pts',(-6.7087649410064,-0.904123688643009,
79.7395924360806));
#203041=CARTESIAN_POINT('Ctrl Pts',(-6.6798459273942,-1.08256518800263,
79.7480845039232));
#203042=CARTESIAN_POINT('Ctrl Pts',(-6.6508989142315,-1.26117945541856,
79.7565847938333));
#203043=CARTESIAN_POINT('Ctrl Pts',(-6.61481021078436,-1.43846800435146,
79.7650850837434));
#203044=CARTESIAN_POINT('Ctrl Pts',(-6.57173980833,-1.61385404904248,79.7735853736534));
#203045=CARTESIAN_POINT('Ctrl Pts',(-6.52858281749277,-1.7895926883953,
79.7821027524765));
#203046=CARTESIAN_POINT('Ctrl Pts',(-6.47841614982349,-1.96342086604332,
79.7906201312995));
#203047=CARTESIAN_POINT('Ctrl Pts',(-6.42144951339353,-2.13477754038636,
79.7991375101225));
#203048=CARTESIAN_POINT('Ctrl Pts',(-6.3689139499044,-2.29280546705363,
79.8069923761276));
#203049=CARTESIAN_POINT('Ctrl Pts',(-6.31059574714776,-2.44873146061933,
79.8148472421327));
#203050=CARTESIAN_POINT('Ctrl Pts',(-6.24669448988538,-2.60213315378664,
79.8227021081378));
#203051=CARTESIAN_POINT('Ctrl Pts',(-6.17796775742869,-2.76711890800152,
79.8311501308769));
#203052=CARTESIAN_POINT('Ctrl Pts',(-6.10264102872985,-2.92952346695329,
79.8395981536161));
#203053=CARTESIAN_POINT('Ctrl Pts',(-6.02092964377854,-3.08880158389444,
79.8480461763553));
#203054=CARTESIAN_POINT('Ctrl Pts',(-5.93929308438736,-3.24793384509806,
79.8564864629873));
#203055=CARTESIAN_POINT('Ctrl Pts',(-5.85128367428993,-3.40394507573357,
79.8649267496193));
#203056=CARTESIAN_POINT('Ctrl Pts',(-5.7571644884972,-3.55631073619654,
79.8733670362513));
#203057=CARTESIAN_POINT('Ctrl Pts',(-5.66311700133879,-3.70856032670332,
79.881800893195));
#203058=CARTESIAN_POINT('Ctrl Pts',(-5.56296919158213,-3.8571696005349,
79.8902347501387));
#203059=CARTESIAN_POINT('Ctrl Pts',(-5.45702981818307,-4.00163898464877,
79.8986686070824));
#203060=CARTESIAN_POINT('Ctrl Pts',(-5.35115486142754,-4.14602052387062,
79.9070973358029));
#203061=CARTESIAN_POINT('Ctrl Pts',(-5.23949555883428,-4.2862669238484,
79.9155260645234));
#203062=CARTESIAN_POINT('Ctrl Pts',(-5.12240391870074,-4.42190763061366,
79.9239547932438));
#203063=CARTESIAN_POINT('Ctrl Pts',(-5.00536549543674,-4.55748669016151,
79.9323796911993));
#203064=CARTESIAN_POINT('Ctrl Pts',(-4.88289987527993,-4.68846397839237,
79.9408045891548));
#203065=CARTESIAN_POINT('Ctrl Pts',(-4.75539951864566,-4.81440177156671,
79.9492294871103));
#203066=CARTESIAN_POINT('Ctrl Pts',(-4.62792739080197,-4.94031168190461,
79.9576525197794));
#203067=CARTESIAN_POINT('Ctrl Pts',(-4.4954229841731,-5.06118408575414,
79.9660755524485));
#203068=CARTESIAN_POINT('Ctrl Pts',(-4.35831617956601,-5.17661753261077,
79.9744985851175));
#203069=CARTESIAN_POINT('Ctrl Pts',(-4.22122488844035,-5.29203791830211,
79.9829206647299));
#203070=CARTESIAN_POINT('Ctrl Pts',(-4.07953249253786,-5.40202035912182,
79.9913427443423));
#203071=CARTESIAN_POINT('Ctrl Pts',(-3.93370280031777,-5.50620298198061,
79.9997648239546));
#203072=CARTESIAN_POINT('Ctrl Pts',(-3.78786925182711,-5.61038835980909,
80.0081871262776));
#203073=CARTESIAN_POINT('Ctrl Pts',(-3.63789846045687,-5.70877342036208,
80.0166094286006));
#203074=CARTESIAN_POINT('Ctrl Pts',(-3.48428441719833,-5.80103879491155,
80.0250317309236));
#203075=CARTESIAN_POINT('Ctrl Pts',(-3.33064486720266,-5.89331948960107,
80.0334554317219));
#203076=CARTESIAN_POINT('Ctrl Pts',(-3.17336114538983,-5.97947830124503,
80.0418791325202));
#203077=CARTESIAN_POINT('Ctrl Pts',(-3.01295342430362,-6.05924093125344,
80.0503028333185));
#203078=CARTESIAN_POINT('Ctrl Pts',(-2.85243715384369,-6.13905753736398,
80.0587322345123));
#203079=CARTESIAN_POINT('Ctrl Pts',(-2.68879295864841,-6.21246916411479,
80.0671616357061));
#203080=CARTESIAN_POINT('Ctrl Pts',(-2.52256357802893,-6.27924852150334,
80.0755910368999));
#203081=CARTESIAN_POINT('Ctrl Pts',(-2.35627488699592,-6.34605170567442,
80.0840234456924));
#203082=CARTESIAN_POINT('Ctrl Pts',(-2.18739948304234,-6.40621778344014,
80.0924558544848));
#203083=CARTESIAN_POINT('Ctrl Pts',(-2.01649753443931,-6.45956861513215,
80.1008882632773));
#203084=CARTESIAN_POINT('Ctrl Pts',(-1.84543746237381,-6.51296880856813,
80.1093284739801));
#203085=CARTESIAN_POINT('Ctrl Pts',(-1.67234741967609,-6.55954106372498,
80.1177686846829));
#203086=CARTESIAN_POINT('Ctrl Pts',(-1.49780117594638,-6.5991575702762,
80.1262088953857));
#203087=CARTESIAN_POINT('Ctrl Pts',(-1.39852224456197,-6.62169076464089,
80.1310095435196));
#203088=CARTESIAN_POINT('Ctrl Pts',(-1.29877240465794,-6.64197461059254,
80.1358101916534));
#203089=CARTESIAN_POINT('Ctrl Pts',(-1.19865835252534,-6.65999302957002,
80.1406108397873));
#203090=CARTESIAN_POINT('Ctrl Pts',(-1.02891047137568,-6.69054406988795,
80.1487505547574));
#203091=CARTESIAN_POINT('Ctrl Pts',(-0.857776673190221,-6.71464022138195,
80.1568902697276));
#203092=CARTESIAN_POINT('Ctrl Pts',(-0.685793573818161,-6.73215984466425,
80.1650299846978));
#203093=CARTESIAN_POINT('Ctrl Pts',(-0.513960889834913,-6.74966414538893,
80.173162580722));
#203094=CARTESIAN_POINT('Ctrl Pts',(-0.341280745019906,-6.7606033299496,
80.1812951767462));
#203095=CARTESIAN_POINT('Ctrl Pts',(-0.16829978686302,-6.76490681249505,
80.1894277727704));
#203096=CARTESIAN_POINT('Ctrl Pts',(0.00456291223020466,-6.76920735294894,
80.1975548089156));
#203097=CARTESIAN_POINT('Ctrl Pts',(0.177725650628405,-6.76688121430026,
80.2056818450608));
#203098=CARTESIAN_POINT('Ctrl Pts',(0.350636859967422,-6.75790964666088,
80.213808881206));
#203099=CARTESIAN_POINT('Ctrl Pts',(0.523465414621692,-6.74894236759307,
80.221932032481));
#203100=CARTESIAN_POINT('Ctrl Pts',(0.696042314705396,-6.73333600419254,
80.230055183756));
#203101=CARTESIAN_POINT('Ctrl Pts',(0.867816211774448,-6.71112390159662,
80.238178335031));
#203102=CARTESIAN_POINT('Ctrl Pts',(1.03954183910317,-6.68891804076643,
80.2462992036402));
#203103=CARTESIAN_POINT('Ctrl Pts',(1.21046455009964,-6.66011018575533,
80.2544200722494));
#203104=CARTESIAN_POINT('Ctrl Pts',(1.38003837161272,-6.62478551297146,
80.2625409408585));
#203105=CARTESIAN_POINT('Ctrl Pts',(1.54962135755058,-6.58945893110573,
80.2706622483508));
#203106=CARTESIAN_POINT('Ctrl Pts',(1.71785494902696,-6.54761489864508,
80.2787835558431));
#203107=CARTESIAN_POINT('Ctrl Pts',(1.88420342907505,-6.49938969733789,
80.2869048633355));
#203108=CARTESIAN_POINT('Ctrl Pts',(1.97064389023608,-6.47433020392158,
80.2911249774276));
#203109=CARTESIAN_POINT('Ctrl Pts',(2.05657553629773,-6.44754849835256,
80.2953450915198));
#203110=CARTESIAN_POINT('Ctrl Pts',(2.14192478895576,-6.41906902895247,
80.299565205612));
#203111=CARTESIAN_POINT('Ctrl Pts',(2.32362962080415,-6.35843748225097,
80.3085496442289));
#203112=CARTESIAN_POINT('Ctrl Pts',(2.5026037720119,-6.29013824560206,80.3175340828458));
#203113=CARTESIAN_POINT('Ctrl Pts',(2.67823555666833,-6.21444633921619,
80.3265185214627));
#203114=CARTESIAN_POINT('Ctrl Pts',(2.85417047137847,-6.13862379308483,
80.3355184666883));
#203115=CARTESIAN_POINT('Ctrl Pts',(3.02675126992934,-6.05538316938616,
80.3445184119138));
#203116=CARTESIAN_POINT('Ctrl Pts',(3.19538935917925,-5.96504617276715,
80.3535183571394));
#203117=CARTESIAN_POINT('Ctrl Pts',(3.36442484848985,-5.87449629465679,
80.3625395109709));
#203118=CARTESIAN_POINT('Ctrl Pts',(3.52949882702707,-5.77681669733902,
80.3715606648025));
#203119=CARTESIAN_POINT('Ctrl Pts',(3.69004790648951,-5.67237476263799,
80.380581818634));
#203120=CARTESIAN_POINT('Ctrl Pts',(3.85076034593405,-5.56782655742679,
80.3896121515622));
#203121=CARTESIAN_POINT('Ctrl Pts',(4.0069384915457,-5.45650240403707,80.3986424844904));
#203122=CARTESIAN_POINT('Ctrl Pts',(4.15804947416783,-5.33881199990903,
80.4076728174186));
#203123=CARTESIAN_POINT('Ctrl Pts',(4.3093746845413,-5.22095474787759,80.4167159525131));
#203124=CARTESIAN_POINT('Ctrl Pts',(4.45561817943725,-5.09671334563674,
80.4257590876075));
#203125=CARTESIAN_POINT('Ctrl Pts',(4.5962798198103,-4.96653811200565,80.434802222702));
#203126=CARTESIAN_POINT('Ctrl Pts',(4.71925049106152,-4.85273497550414,
80.4427080056136));
#203127=CARTESIAN_POINT('Ctrl Pts',(4.83795553226584,-4.73439739749656,
80.4506137885252));
#203128=CARTESIAN_POINT('Ctrl Pts',(4.95208416706777,-4.61184902206011,
80.4585195714368));
#203129=CARTESIAN_POINT('Ctrl Pts',(5.07700530268695,-4.47771193845811,
80.4671729596158));
#203130=CARTESIAN_POINT('Ctrl Pts',(5.19655298764959,-4.33841063385692,
80.4758263477947));
#203131=CARTESIAN_POINT('Ctrl Pts',(5.31030630322139,-4.19439339666264,
80.4844797359737));
#203132=CARTESIAN_POINT('Ctrl Pts',(5.42395455953369,-4.05050916960719,
80.4931251321345));
#203133=CARTESIAN_POINT('Ctrl Pts',(5.53181893237289,-3.90191793484356,
80.5017705282954));
#203134=CARTESIAN_POINT('Ctrl Pts',(5.63351767492406,-3.74910224004603,
80.5104159244563));
#203135=CARTESIAN_POINT('Ctrl Pts',(5.73846433362059,-3.59140612539331,
80.5193374255234));
#203136=CARTESIAN_POINT('Ctrl Pts',(5.83684479616741,-3.42921148636016,
80.5282589265905));
#203137=CARTESIAN_POINT('Ctrl Pts',(5.92828549141526,-3.26308445068089,
80.5371804276576));
#203138=CARTESIAN_POINT('Ctrl Pts',(6.01672749005155,-3.10240536766239,
80.5458093579503));
#203139=CARTESIAN_POINT('Ctrl Pts',(6.09867748891445,-2.93804799946783,
80.554438288243));
#203140=CARTESIAN_POINT('Ctrl Pts',(6.17384187110355,-2.77055329322657,
80.5630672185357));
#203141=CARTESIAN_POINT('Ctrl Pts',(6.25282901592219,-2.59454002426963,
80.57213500499));
#203142=CARTESIAN_POINT('Ctrl Pts',(6.32432215343465,-2.41506226223281,
80.5812027914443));
#203143=CARTESIAN_POINT('Ctrl Pts',(6.38803548828711,-2.23277665707622,
80.5902705778986));
#203144=CARTESIAN_POINT('Ctrl Pts',(6.45174882313959,-2.05049105191957,
80.5993383643529));
#203145=CARTESIAN_POINT('Ctrl Pts',(6.50768219324855,-1.86539796067073,
80.6084061508072));
#203146=CARTESIAN_POINT('Ctrl Pts',(6.55560873764775,-1.67817850030218,
80.6174739372615));
#203147=CARTESIAN_POINT('Ctrl Pts',(6.600137690445,-1.50423133557365,80.6258988934118));
#203148=CARTESIAN_POINT('Ctrl Pts',(6.63773550657051,-1.32852498474019,
80.6343238495621));
#203149=CARTESIAN_POINT('Ctrl Pts',(6.66828457498004,-1.15163788887098,
80.6427488057124));
#203150=CARTESIAN_POINT('Ctrl Pts',(6.69884073412276,-0.974709735802147,
80.6511757173762));
#203151=CARTESIAN_POINT('Ctrl Pts',(6.7223448270092,-0.796600618026984,
80.65960262904));
#203152=CARTESIAN_POINT('Ctrl Pts',(6.7387307722117,-0.617896900499686,
80.6680295407039));
#203153=CARTESIAN_POINT('Ctrl Pts',(6.75512274316502,-0.439127466649144,
80.6764595512716));
#203154=CARTESIAN_POINT('Ctrl Pts',(6.76439131688234,-0.259763327125723,
80.6848895618393));
#203155=CARTESIAN_POINT('Ctrl Pts',(6.76652242990444,-0.0803940644580883,
80.6933195724071));
#203156=CARTESIAN_POINT('Ctrl Pts',(6.76865550606336,0.0991404294287381,
80.7017573485245));
#203157=CARTESIAN_POINT('Ctrl Pts',(6.76363798155557,0.278679724072522,
80.710195124642));
#203158=CARTESIAN_POINT('Ctrl Pts',(6.75150792001702,0.45763501390017,80.7186329007594));
#203159=CARTESIAN_POINT('Ctrl Pts',(6.73937149109012,0.636684242066582,
80.7270751060875));
#203160=CARTESIAN_POINT('Ctrl Pts',(6.72011510918539,0.815148524095448,
80.7355173114155));
#203161=CARTESIAN_POINT('Ctrl Pts',(6.6938285714976,0.992445492408714,80.7439595167436));
#203162=CARTESIAN_POINT('Ctrl Pts',(6.6675143029586,1.16992949927035,80.7524106281339));
#203163=CARTESIAN_POINT('Ctrl Pts',(6.63415511997451,1.34624340598651,80.7608617395242));
#203164=CARTESIAN_POINT('Ctrl Pts',(6.59389186493309,1.52081526608897,80.7693128509144));
#203165=CARTESIAN_POINT('Ctrl Pts',(6.58259192057082,1.56980912672804,80.771684668305));
#203166=CARTESIAN_POINT('Ctrl Pts',(6.57074847723041,1.61866586484798,80.7740564856957));
#203167=CARTESIAN_POINT('Ctrl Pts',(6.55836535019449,1.66737306364483,80.7764283030862));
#203168=CARTESIAN_POINT('Ctrl Pts',(6.51494345992729,1.83816664714307,80.7847451679758));
#203169=CARTESIAN_POINT('Ctrl Pts',(6.46480354114859,2.00742856727076,80.7930620328654));
#203170=CARTESIAN_POINT('Ctrl Pts',(6.408072719558,2.17460180742512,80.801378897755));
#203171=CARTESIAN_POINT('Ctrl Pts',(6.35139096768909,2.34163044991392,80.8096885689141));
#203172=CARTESIAN_POINT('Ctrl Pts',(6.28812978339475,2.5065736842362,80.8179982400731));
#203173=CARTESIAN_POINT('Ctrl Pts',(6.2184666305487,2.66888773925625,80.8263079112321));
#203174=CARTESIAN_POINT('Ctrl Pts',(6.14885095995114,2.83109116138101,80.8346119185379));
#203175=CARTESIAN_POINT('Ctrl Pts',(6.07284215340048,2.99066865668409,80.8429159258438));
#203176=CARTESIAN_POINT('Ctrl Pts',(5.99066656967292,3.14709438228398,80.8512199331496));
#203177=CARTESIAN_POINT('Ctrl Pts',(5.90853068887912,3.30344453117431,80.8595199283945));
#203178=CARTESIAN_POINT('Ctrl Pts',(5.82023413035652,3.45664563774094,80.8678199236393));
#203179=CARTESIAN_POINT('Ctrl Pts',(5.7260502758238,3.60619428743631,80.8761199188842));
#203180=CARTESIAN_POINT('Ctrl Pts',(5.6318908357205,3.75570417098675,80.8844177625963));
#203181=CARTESIAN_POINT('Ctrl Pts',(5.53184732523244,3.90156318976282,80.8927156063084));
#203182=CARTESIAN_POINT('Ctrl Pts',(5.42623788480702,4.04329462412586,80.9010134500205));
#203183=CARTESIAN_POINT('Ctrl Pts',(5.32063827053594,4.18501287145804,80.9093105216814));
#203184=CARTESIAN_POINT('Ctrl Pts',(5.20947396623572,4.32260402083056,80.9176075933423));
#203185=CARTESIAN_POINT('Ctrl Pts',(5.09310515724321,4.45562216275827,80.9259046650033));
#203186=CARTESIAN_POINT('Ctrl Pts',(4.97672783879117,4.5886500316266,80.9342023433869));
#203187=CARTESIAN_POINT('Ctrl Pts',(4.85514548688546,4.71710396536243,80.9425000217705));
#203188=CARTESIAN_POINT('Ctrl Pts',(4.72875723190401,4.84057269769968,80.9507977001541));
#203189=CARTESIAN_POINT('Ctrl Pts',(4.60228805140475,4.96412048620476,80.9591006914832));
#203190=CARTESIAN_POINT('Ctrl Pts',(4.47100706759699,5.08267645108949,80.9674036828124));
#203191=CARTESIAN_POINT('Ctrl Pts',(4.33534942909444,5.19586704291502,80.9757066741416));
#203192=CARTESIAN_POINT('Ctrl Pts',(4.19964792631716,5.30909423439887,80.9840123502049));
#203193=CARTESIAN_POINT('Ctrl Pts',(4.05956721992392,5.41695237756055,80.9923180262682));
#203194=CARTESIAN_POINT('Ctrl Pts',(3.91557410022157,5.51910939062401,81.0006237023315));
#203195=CARTESIAN_POINT('Ctrl Pts',(3.77143300909909,5.621371383136,81.0089379135435));
#203196=CARTESIAN_POINT('Ctrl Pts',(3.62337175921483,5.71792034346677,81.0172521247555));
#203197=CARTESIAN_POINT('Ctrl Pts',(3.471885496088,5.80846796513967,81.0255663359674));
#203198=CARTESIAN_POINT('Ctrl Pts',(3.3497610985411,5.8814651697565,81.0322690429613));
#203199=CARTESIAN_POINT('Ctrl Pts',(3.22541130420994,5.95056282308713,81.0389717499552));
#203200=CARTESIAN_POINT('Ctrl Pts',(3.09910619832132,6.01563211736941,81.0456744569491));
#203201=CARTESIAN_POINT('Ctrl Pts',(3.09910619832139,6.01563211736937,79.0457552630242));
#203202=CARTESIAN_POINT('Ctrl Pts',(2.93375330764829,6.10081787314652,79.0545047109265));
#203203=CARTESIAN_POINT('Ctrl Pts',(2.7648862784307,6.17918207037039,79.0632541588288));
#203204=CARTESIAN_POINT('Ctrl Pts',(2.59307866646699,6.25045854553998,79.0720036067311));
#203205=CARTESIAN_POINT('Ctrl Pts',(2.42127244185365,6.32173444515041,79.0807529839814));
#203206=CARTESIAN_POINT('Ctrl Pts',(2.24652594672445,6.38592262741845,79.0895023612317));
#203207=CARTESIAN_POINT('Ctrl Pts',(2.06943269687093,6.44280508110571,79.098251738482));
#203208=CARTESIAN_POINT('Ctrl Pts',(1.89234081822047,6.49968709436175,79.1070010479874));
#203209=CARTESIAN_POINT('Ctrl Pts',(1.71290249405556,6.54926340459553,79.1157503574927));
#203210=CARTESIAN_POINT('Ctrl Pts',(1.53172716625023,6.59136563150392,79.1244996669981));
#203211=CARTESIAN_POINT('Ctrl Pts',(1.350553181073,6.63346754640717,79.1332489116653));
#203212=CARTESIAN_POINT('Ctrl Pts',(1.16764249714387,6.66809542395782,79.1419981563326));
#203213=CARTESIAN_POINT('Ctrl Pts',(0.983616340614045,6.69513165624673,
79.1507474009998));
#203214=CARTESIAN_POINT('Ctrl Pts',(0.799591486713628,6.72216769715963,
79.1594965837355));
#203215=CARTESIAN_POINT('Ctrl Pts',(0.614451459526594,6.74161215869372,
79.1682457664712));
#203216=CARTESIAN_POINT('Ctrl Pts',(0.428825047910263,6.75339900185712,
79.1769949492069));
#203217=CARTESIAN_POINT('Ctrl Pts',(0.243199888597033,6.76518576550221,
79.1857440729174));
#203218=CARTESIAN_POINT('Ctrl Pts',(0.0570886373919136,6.76931499599834,
79.194493196628));
#203219=CARTESIAN_POINT('Ctrl Pts',(-0.128876626811146,6.76577266947847,
79.2032423203385));
#203220=CARTESIAN_POINT('Ctrl Pts',(-0.314840698188063,6.76223036567993,
79.21199138793));
#203221=CARTESIAN_POINT('Ctrl Pts',(-0.500658497951067,6.75101660879224,
79.2207404555216));
#203222=CARTESIAN_POINT('Ctrl Pts',(-0.68569895192594,6.73216948296221,
79.2294895231131));
#203223=CARTESIAN_POINT('Ctrl Pts',(-0.870738280459641,6.71332247176296,
79.2382385374917));
#203224=CARTESIAN_POINT('Ctrl Pts',(-1.05499998761236,6.68684221356189,
79.2469875518702));
#203225=CARTESIAN_POINT('Ctrl Pts',(-1.23785829161412,6.65281863948524,
79.2557365662487));
#203226=CARTESIAN_POINT('Ctrl Pts',(-1.43007412917395,6.61705395368863,
79.2649332999479));
#203227=CARTESIAN_POINT('Ctrl Pts',(-1.62073882535782,6.57295372727792,
79.2741300336471));
#203228=CARTESIAN_POINT('Ctrl Pts',(-1.80913696091504,6.52068343478282,
79.2833267673463));
#203229=CARTESIAN_POINT('Ctrl Pts',(-1.98838356186099,6.47095219815203,
79.2920767650599));
#203230=CARTESIAN_POINT('Ctrl Pts',(-2.16557827572516,6.41382586850896,
79.3008267627736));
#203231=CARTESIAN_POINT('Ctrl Pts',(-2.3401191862168,6.34949849943285,79.3095767604873));
#203232=CARTESIAN_POINT('Ctrl Pts',(-2.51465655691069,6.28517243495562,
79.3183265807456));
#203233=CARTESIAN_POINT('Ctrl Pts',(-2.6865399629529,6.21364572242391,79.3270764010039));
#203234=CARTESIAN_POINT('Ctrl Pts',(-2.85518555379941,6.13516132252243,
79.3358262212622));
#203235=CARTESIAN_POINT('Ctrl Pts',(-3.02382794858646,6.05667841000528,
79.3445758756997));
#203236=CARTESIAN_POINT('Ctrl Pts',(-3.18923239109243,5.97123819492101,
79.3533255301372));
#203237=CARTESIAN_POINT('Ctrl Pts',(-3.35083705967665,5.87913088810732,
79.3620751845747));
#203238=CARTESIAN_POINT('Ctrl Pts',(-3.51243888042359,5.78702520443127,
79.3708246848237));
#203239=CARTESIAN_POINT('Ctrl Pts',(-3.67024081223643,5.68825280605813,
79.3795741850726));
#203240=CARTESIAN_POINT('Ctrl Pts',(-3.82370687544348,5.58314917682541,
79.3883236853216));
#203241=CARTESIAN_POINT('Ctrl Pts',(-3.97717043817767,5.47804726008056,
79.397073043012));
#203242=CARTESIAN_POINT('Ctrl Pts',(-4.12629803722418,5.36661448084269,
79.4058224007025));
#203243=CARTESIAN_POINT('Ctrl Pts',(-4.2705831720687,5.24922931204607,79.4145717583929));
#203244=CARTESIAN_POINT('Ctrl Pts',(-4.41486614774809,5.13184589986813,
79.423320985153));
#203245=CARTESIAN_POINT('Ctrl Pts',(-4.55430658194399,5.00851045723048,
79.4320702119131));
#203246=CARTESIAN_POINT('Ctrl Pts',(-4.68843089001841,4.87964187103123,
79.4408194386732));
#203247=CARTESIAN_POINT('Ctrl Pts',(-4.82255336917833,4.75077504207964,
79.4495685461291));
#203248=CARTESIAN_POINT('Ctrl Pts',(-4.95135966065131,4.61637541908097,
79.458317653585));
#203249=CARTESIAN_POINT('Ctrl Pts',(-5.07441230869241,4.47689945401848,
79.467066761041));
#203250=CARTESIAN_POINT('Ctrl Pts',(-5.19746344226413,4.3374252055552,79.4758157608173));
#203251=CARTESIAN_POINT('Ctrl Pts',(-5.31476088454763,4.19287495491341,
79.4845647605937));
#203252=CARTESIAN_POINT('Ctrl Pts',(-5.4259062762885,4.04373961586711,79.4933137603701));
#203253=CARTESIAN_POINT('Ctrl Pts',(-5.53706380672667,3.89458798906735,
79.5020637156648));
#203254=CARTESIAN_POINT('Ctrl Pts',(-5.64206777071866,3.74085050155281,
79.5108136709595));
#203255=CARTESIAN_POINT('Ctrl Pts',(-5.74056148164012,3.58304938223153,
79.5195636262542));
#203256=CARTESIAN_POINT('Ctrl Pts',(-5.83905138951886,3.42525435593277,
79.5283132436953));
#203257=CARTESIAN_POINT('Ctrl Pts',(-5.93103139557654,3.26339625497181,
79.5370628611363));
#203258=CARTESIAN_POINT('Ctrl Pts',(-6.01618907820846,3.09802485065005,
79.5458124785775));
#203259=CARTESIAN_POINT('Ctrl Pts',(-6.10134392544988,2.93265895249632,
79.5545618046933));
#203260=CARTESIAN_POINT('Ctrl Pts',(-6.1796767726184,2.76378023986017,79.5633111308092));
#203261=CARTESIAN_POINT('Ctrl Pts',(-6.25092157009235,2.59196229227089,
79.5720604569251));
#203262=CARTESIAN_POINT('Ctrl Pts',(-6.32216437407757,2.4201491522908,79.5808095382275));
#203263=CARTESIAN_POINT('Ctrl Pts',(-6.38631941548919,2.24539720662856,
79.58955861953));
#203264=CARTESIAN_POINT('Ctrl Pts',(-6.4431688103753,2.06829994947709,79.5983077008324));
#203265=CARTESIAN_POINT('Ctrl Pts',(-6.50002334524564,1.89118668024476,
79.6070575731748));
#203266=CARTESIAN_POINT('Ctrl Pts',(-6.54957082411089,1.71172794807731,
79.6158074455171));
#203267=CARTESIAN_POINT('Ctrl Pts',(-6.59164294296076,1.53053334250371,
79.6245573178595));
#203268=CARTESIAN_POINT('Ctrl Pts',(-6.63371214082133,1.34935131693608,
79.6333065827144));
#203269=CARTESIAN_POINT('Ctrl Pts',(-6.66830695239693,1.16643393829749,
79.6420558475693));
#203270=CARTESIAN_POINT('Ctrl Pts',(-6.69530988153994,0.982402458340616,
79.6508051124242));
#203271=CARTESIAN_POINT('Ctrl Pts',(-6.72231419690488,0.798361530946668,
79.6595548264313));
#203272=CARTESIAN_POINT('Ctrl Pts',(-6.74172580829282,0.613206671362071,
79.6683045404383));
#203273=CARTESIAN_POINT('Ctrl Pts',(-6.75347878028182,0.427566795112976,
79.6770542544453));
#203274=CARTESIAN_POINT('Ctrl Pts',(-6.76248992368213,0.285234494205442,
79.6837627642335));
#203275=CARTESIAN_POINT('Ctrl Pts',(-6.76699999999994,0.142617266092895,
79.6904712740218));
#203276=CARTESIAN_POINT('Ctrl Pts',(-6.767,2.79684983589873E-12,79.69717978381));
#203277=CARTESIAN_POINT('',(-6.76699963750513,0.00221495044038298,79.3028202161514));
#203278=CARTESIAN_POINT('Ctrl Pts',(3.09910619832128,6.01563211736943,78.6515182808518));
#203279=CARTESIAN_POINT('Ctrl Pts',(2.94524964427127,6.09489524234211,78.6596411247725));
#203280=CARTESIAN_POINT('Ctrl Pts',(2.78827182354791,6.16829232074604,78.6677639686933));
#203281=CARTESIAN_POINT('Ctrl Pts',(2.62866640743604,6.23557550819628,78.675886812614));
#203282=CARTESIAN_POINT('Ctrl Pts',(2.46910295246842,6.30284100652542,78.6840075209942));
#203283=CARTESIAN_POINT('Ctrl Pts',(2.30691361570877,6.36399567440877,78.6921282293744));
#203284=CARTESIAN_POINT('Ctrl Pts',(2.14261340044974,6.41883921096433,78.7002489377547));
#203285=CARTESIAN_POINT('Ctrl Pts',(1.97830368986549,6.47368591706666,78.7083701154512));
#203286=CARTESIAN_POINT('Ctrl Pts',(1.8118832036047,6.52222064474138,78.7164912931477));
#203287=CARTESIAN_POINT('Ctrl Pts',(1.64388366608236,6.56429245938872,78.7246124708442));
#203288=CARTESIAN_POINT('Ctrl Pts',(1.57437448245534,6.58169951617574,78.7279725779022));
#203289=CARTESIAN_POINT('Ctrl Pts',(1.50459515420102,6.59800080675089,78.7313326849603));
#203290=CARTESIAN_POINT('Ctrl Pts',(1.43458395721529,6.6131881773998,78.7346927920183));
#203291=CARTESIAN_POINT('Ctrl Pts',(1.2473838437369,6.65379707470939,78.7436772466434));
#203292=CARTESIAN_POINT('Ctrl Pts',(1.05861809858462,6.68641852117337,78.7526617012684));
#203293=CARTESIAN_POINT('Ctrl Pts',(0.868953103732096,6.71097679205601,
78.7616461558935));
#203294=CARTESIAN_POINT('Ctrl Pts',(0.678960741941393,6.73557745118194,
78.7706461179315));
#203295=CARTESIAN_POINT('Ctrl Pts',(0.488066265174348,6.75208708718582,
78.7796460799695));
#203296=CARTESIAN_POINT('Ctrl Pts',(0.296940026432046,6.76048190743105,
78.7886460420075));
#203297=CARTESIAN_POINT('Ctrl Pts',(0.105363375775685,6.76889651107745,
78.7976672135359));
#203298=CARTESIAN_POINT('Ctrl Pts',(-0.0864458899679037,6.7691580253438,
78.8066883850644));
#203299=CARTESIAN_POINT('Ctrl Pts',(-0.277815777047764,6.76129480159114,
78.8157095565928));
#203300=CARTESIAN_POINT('Ctrl Pts',(-0.469380392114852,6.75342357663328,
78.8247399075935));
#203301=CARTESIAN_POINT('Ctrl Pts',(-0.660504497049267,6.73741111340131,
78.8337702585942));
#203302=CARTESIAN_POINT('Ctrl Pts',(-0.850520743133508,6.71333772914037,
78.8428006095949));
#203303=CARTESIAN_POINT('Ctrl Pts',(-1.04080637744029,6.68923021576506,
78.8518437630284));
#203304=CARTESIAN_POINT('Ctrl Pts',(-1.22998077520956,6.65703896072662,
78.8608869164618));
#203305=CARTESIAN_POINT('Ctrl Pts',(-1.41738399877022,6.61689591878474,
78.8699300698952));
#203306=CARTESIAN_POINT('Ctrl Pts',(-1.58121544568112,6.58180211132623,
78.8778357658778));
#203307=CARTESIAN_POINT('Ctrl Pts',(-1.74369331824502,6.54063188396889,
78.8857414618605));
#203308=CARTESIAN_POINT('Ctrl Pts',(-1.90438519169257,6.49350491196103,
78.8936471578431));
#203309=CARTESIAN_POINT('Ctrl Pts',(-2.08027441159858,6.44192093222917,
78.9023005307198));
#203310=CARTESIAN_POINT('Ctrl Pts',(-2.25417886235738,6.38315339922036,
78.9109539035965));
#203311=CARTESIAN_POINT('Ctrl Pts',(-2.42550777024041,6.31737295531168,
78.9196072764732));
#203312=CARTESIAN_POINT('Ctrl Pts',(-2.59667844159213,6.25165326512752,
78.9282526572386));
#203313=CARTESIAN_POINT('Ctrl Pts',(-2.76527803165542,6.17893369116949,
78.936898038004));
#203314=CARTESIAN_POINT('Ctrl Pts',(-2.93073196446853,6.09943433052955,
78.9455434187693));
#203315=CARTESIAN_POINT('Ctrl Pts',(-3.10147039091569,6.01739581075286,
78.9544649275109));
#203316=CARTESIAN_POINT('Ctrl Pts',(-3.26885857849907,5.92813733407461,
78.9633864362524));
#203317=CARTESIAN_POINT('Ctrl Pts',(-3.43228631538297,5.83195504520009,
78.972307944994));
#203318=CARTESIAN_POINT('Ctrl Pts',(-3.59035420242436,5.73892719409548,
78.980936859907));
#203319=CARTESIAN_POINT('Ctrl Pts',(-3.74471699772877,5.63942263458006,
78.98956577482));
#203320=CARTESIAN_POINT('Ctrl Pts',(-3.89484610130794,5.53375666677948,
78.998194689733));
#203321=CARTESIAN_POINT('Ctrl Pts',(-4.05261119092361,5.42271623236701,
79.0072624953888));
#203322=CARTESIAN_POINT('Ctrl Pts',(-4.20570038323733,5.30487142910128,
79.0163303010447));
#203323=CARTESIAN_POINT('Ctrl Pts',(-4.35353273977685,5.18064104949292,
79.0253981067005));
#203324=CARTESIAN_POINT('Ctrl Pts',(-4.50136509631636,5.05641066988457,
79.0344659123563));
#203325=CARTESIAN_POINT('Ctrl Pts',(-4.64394029545781,4.92579493822377,
79.0435337180121));
#203326=CARTESIAN_POINT('Ctrl Pts',(-4.78071558962921,4.78926376921091,
79.0526015236679));
#203327=CARTESIAN_POINT('Ctrl Pts',(-4.90779449631454,4.66241168096109,
79.0610264869316));
#203328=CARTESIAN_POINT('Ctrl Pts',(-5.02981110075196,4.53050898203097,
79.0694514501953));
#203329=CARTESIAN_POINT('Ctrl Pts',(-5.14636901431176,4.39399305513013,
79.077876413459));
#203330=CARTESIAN_POINT('Ctrl Pts',(-5.26295398405147,4.25744543926569,
79.0863033323799));
#203331=CARTESIAN_POINT('Ctrl Pts',(-5.37407752116965,4.11628271249826,
79.0947302513008));
#203332=CARTESIAN_POINT('Ctrl Pts',(-5.47938350389405,3.97097537353907,
79.1031571702217));
#203333=CARTESIAN_POINT('Ctrl Pts',(-5.58472821329221,3.82561459725595,
79.1115871881739));
#203334=CARTESIAN_POINT('Ctrl Pts',(-5.68425090798292,3.67610643805485,
79.1200172061261));
#203335=CARTESIAN_POINT('Ctrl Pts',(-5.77763855521455,3.52295071286816,
79.1284472240783));
#203336=CARTESIAN_POINT('Ctrl Pts',(-5.87111223070906,3.36965390134536,
79.1368850077236));
#203337=CARTESIAN_POINT('Ctrl Pts',(-5.95843939463506,3.21270309393495,
79.1453227913688));
#203338=CARTESIAN_POINT('Ctrl Pts',(-6.03935223600749,3.05262404652643,
79.153760575014));
#203339=CARTESIAN_POINT('Ctrl Pts',(-6.12030755138395,2.89246096798033,
79.1622027879495));
#203340=CARTESIAN_POINT('Ctrl Pts',(-6.19484168647654,2.72916667353424,
79.1706450008849));
#203341=CARTESIAN_POINT('Ctrl Pts',(-6.26273460320383,2.56328778911644,
79.1790872138204));
#203342=CARTESIAN_POINT('Ctrl Pts',(-6.3306991437123,2.39723391040623,79.1875383328869));
#203343=CARTESIAN_POINT('Ctrl Pts',(-6.39200835218371,2.22859030456305,
79.1959894519534));
#203344=CARTESIAN_POINT('Ctrl Pts',(-6.44649140458477,2.057920691041,79.2044405710198));
#203345=CARTESIAN_POINT('Ctrl Pts',(-6.46178185571332,2.01002294541771,
79.2068123438441));
#203346=CARTESIAN_POINT('Ctrl Pts',(-6.47653496985489,1.96196570363734,
79.2091841166684));
#203347=CARTESIAN_POINT('Ctrl Pts',(-6.49074769014697,1.91376158986739,
79.2115558894926));
#203348=CARTESIAN_POINT('Ctrl Pts',(-6.54928341862,1.7152307768398,79.2213241426621));
#203349=CARTESIAN_POINT('Ctrl Pts',(-6.59872468730928,1.51395107279027,
79.2310923958316));
#203350=CARTESIAN_POINT('Ctrl Pts',(-6.63885430811011,1.31068778726586,
79.2408606490011));
#203351=CARTESIAN_POINT('Ctrl Pts',(-6.67885051141634,1.10810028381354,
79.2505964260137));
#203352=CARTESIAN_POINT('Ctrl Pts',(-6.70959683203901,0.903542416313194,
79.2603322030262));
#203353=CARTESIAN_POINT('Ctrl Pts',(-6.73092711602759,0.697788763684628,
79.2700679800387));
#203354=CARTESIAN_POINT('Ctrl Pts',(-6.75211763844694,0.493383262509683,
79.2797399657078));
#203355=CARTESIAN_POINT('Ctrl Pts',(-6.76401506195236,0.287797655196327,
79.2894119513768));
#203356=CARTESIAN_POINT('Ctrl Pts',(-6.76650549202476,0.0818072515051274,
79.2990839370458));
#203357=CARTESIAN_POINT('Ctrl Pts',(-6.76682617563486,0.0552826174535358,
79.3003293634144));
#203358=CARTESIAN_POINT('Ctrl Pts',(-6.76699095172329,0.0287512925092576,
79.3015747897828));
#203359=CARTESIAN_POINT('Ctrl Pts',(-6.76699963750513,0.00221495044041987,
79.3028202161514));
#203360=CARTESIAN_POINT('Ctrl Pts',(-6.7669996375054,0.00221494962268042,
79.3028202161898));
#203361=CARTESIAN_POINT('Ctrl Pts',(-6.76705768574337,-0.175131027606415,
79.3111435697184));
#203362=CARTESIAN_POINT('Ctrl Pts',(-6.7601397171255,-0.352517298753123,
79.319466923247));
#203363=CARTESIAN_POINT('Ctrl Pts',(-6.74626262667905,-0.529367142797431,
79.3277902767756));
#203364=CARTESIAN_POINT('Ctrl Pts',(-6.7322525829915,-0.707911344895013,
79.3361933744575));
#203365=CARTESIAN_POINT('Ctrl Pts',(-6.71114937080536,-0.88590843078606,
79.3445964721395));
#203366=CARTESIAN_POINT('Ctrl Pts',(-6.6830241242902,-1.0627688150088,79.3529995698214));
#203367=CARTESIAN_POINT('Ctrl Pts',(-6.655157240719,-1.23800453188821,79.3613254753246));
#203368=CARTESIAN_POINT('Ctrl Pts',(-6.62039688252329,-1.41212400484039,
79.3696513808278));
#203369=CARTESIAN_POINT('Ctrl Pts',(-6.5788638914875,-1.58456268329212,
79.3779772863311));
#203370=CARTESIAN_POINT('Ctrl Pts',(-6.53731874143279,-1.75705184414598,
79.3863056292904));
#203371=CARTESIAN_POINT('Ctrl Pts',(-6.488997086651,-1.92785889472785,79.3946339722497));
#203372=CARTESIAN_POINT('Ctrl Pts',(-6.43407015601563,-2.09643273859884,
79.402962315209));
#203373=CARTESIAN_POINT('Ctrl Pts',(-6.37911835254023,-2.26508291861684,
79.4112944295341));
#203374=CARTESIAN_POINT('Ctrl Pts',(-6.31755541741858,-2.43149754880781,
79.4196265438591));
#203375=CARTESIAN_POINT('Ctrl Pts',(-6.24960146698585,-2.59514363838466,
79.4279586581841));
#203376=CARTESIAN_POINT('Ctrl Pts',(-6.18061406368497,-2.76127847982298,
79.4364174884306));
#203377=CARTESIAN_POINT('Ctrl Pts',(-6.10503982736518,-2.92455955110825,
79.4448763186771));
#203378=CARTESIAN_POINT('Ctrl Pts',(-6.02315802361306,-3.08445399099835,
79.4533351489236));
#203379=CARTESIAN_POINT('Ctrl Pts',(-5.9423486357773,-3.24225427401333,
79.4616831928443));
#203380=CARTESIAN_POINT('Ctrl Pts',(-5.85539611981876,-3.39675582751105,
79.4700312367649));
#203381=CARTESIAN_POINT('Ctrl Pts',(-5.76261325153627,-3.54747480797519,
79.4783792806856));
#203382=CARTESIAN_POINT('Ctrl Pts',(-5.66798341050639,-3.7011940605217,
79.486893504095));
#203383=CARTESIAN_POINT('Ctrl Pts',(-5.56728888392529,-3.85097825478445,
79.4954077275044));
#203384=CARTESIAN_POINT('Ctrl Pts',(-5.46090525826983,-3.99634867850654,
79.5039219509138));
#203385=CARTESIAN_POINT('Ctrl Pts',(-5.35452163261437,-4.14171910222862,
79.5124361743232));
#203386=CARTESIAN_POINT('Ctrl Pts',(-5.24244918545136,-4.2826754981324,
79.5209503977326));
#203387=CARTESIAN_POINT('Ctrl Pts',(-5.12510375959006,-4.41877816295816,
79.529464621142));
#203388=CARTESIAN_POINT('Ctrl Pts',(-5.01388286691539,-4.54777731027228,
79.5375344672487));
#203389=CARTESIAN_POINT('Ctrl Pts',(-4.8975829761562,-4.67281272641128,
79.5456043133554));
#203390=CARTESIAN_POINT('Ctrl Pts',(-4.77652078403894,-4.79344742326898,
79.5536741594621));
#203391=CARTESIAN_POINT('Ctrl Pts',(-4.6556109035564,-4.91393034633537,
79.5617338526761));
#203392=CARTESIAN_POINT('Ctrl Pts',(-4.52995090422578,-5.03002330656301,
79.5697935458901));
#203393=CARTESIAN_POINT('Ctrl Pts',(-4.39989884924542,-5.14132075603233,
79.577853239104));
#203394=CARTESIAN_POINT('Ctrl Pts',(-4.26998187397997,-5.25250260542331,
79.5859045610464));
#203395=CARTESIAN_POINT('Ctrl Pts',(-4.13568220223781,-5.35889861557442,
79.5939558829889));
#203396=CARTESIAN_POINT('Ctrl Pts',(-3.99739593178139,-5.46013871294289,
79.6020072049313));
#203397=CARTESIAN_POINT('Ctrl Pts',(-3.85922299034842,-5.56129584154424,
79.610051928616));
#203398=CARTESIAN_POINT('Ctrl Pts',(-3.71707025231958,-5.65730524799441,
79.6180966523007));
#203399=CARTESIAN_POINT('Ctrl Pts',(-3.57136811959561,-5.74783600621453,
79.6261413759855));
#203400=CARTESIAN_POINT('Ctrl Pts',(-3.42575349911879,-5.83831238945783,
79.6341812678133));
#203401=CARTESIAN_POINT('Ctrl Pts',(-3.27659404391417,-5.92331647864713,
79.6422211596412));
#203402=CARTESIAN_POINT('Ctrl Pts',(-3.12435037074722,-6.0025597673669,
79.6502610514691));
#203403=CARTESIAN_POINT('Ctrl Pts',(-2.96882847742748,-6.08350937951311,
79.6584740640242));
#203404=CARTESIAN_POINT('Ctrl Pts',(-2.81008835775638,-6.15844704994757,
79.6666870765793));
#203405=CARTESIAN_POINT('Ctrl Pts',(-2.64864941067012,-6.22711372140873,
79.6749000891344));
#203406=CARTESIAN_POINT('Ctrl Pts',(-2.49066854835798,-6.29430952617163,
79.6829371757796));
#203407=CARTESIAN_POINT('Ctrl Pts',(-2.33010367007658,-6.35550012483698,
79.6909742624247));
#203408=CARTESIAN_POINT('Ctrl Pts',(-2.16746305262348,-6.41049084825118,
79.6990113490699));
#203409=CARTESIAN_POINT('Ctrl Pts',(-2.00480686971419,-6.46548683453089,
79.7070492049013));
#203410=CARTESIAN_POINT('Ctrl Pts',(-1.84007490598416,-6.51428164429123,
79.7150870607326));
#203411=CARTESIAN_POINT('Ctrl Pts',(-1.6737916435351,-6.55673017090318,
79.723124916564));
#203412=CARTESIAN_POINT('Ctrl Pts',(-1.50745952074804,-6.59919117050447,
79.7311651342227));
#203413=CARTESIAN_POINT('Ctrl Pts',(-1.33957555373981,-6.63530208281808,
79.7392053518814));
#203414=CARTESIAN_POINT('Ctrl Pts',(-1.17067533445569,-6.66496873670815,
79.7472455695401));
#203415=CARTESIAN_POINT('Ctrl Pts',(-0.995393962881926,-6.69575621469898,
79.7555895514778));
#203416=CARTESIAN_POINT('Ctrl Pts',(-0.819018488221558,-6.71960291021645,
79.7639335334154));
#203417=CARTESIAN_POINT('Ctrl Pts',(-0.64215326736394,-6.73646258664099,
79.772277515353));
#203418=CARTESIAN_POINT('Ctrl Pts',(-0.471430162501238,-6.75273676588449,
79.780331730288));
#203419=CARTESIAN_POINT('Ctrl Pts',(-0.300251127745629,-6.76250112163038,
79.788385945223));
#203420=CARTESIAN_POINT('Ctrl Pts',(-0.1291590707959,-6.76576728349647,
79.7964401601579));
#203421=CARTESIAN_POINT('Ctrl Pts',(0.0420610202531481,-6.76903588954436,
79.8045004023403));
#203422=CARTESIAN_POINT('Ctrl Pts',(0.21319363292898,-6.76579662622857,
79.8125606445227));
#203423=CARTESIAN_POINT('Ctrl Pts',(0.383700933640461,-6.75611297962989,
79.8206208867051));
#203424=CARTESIAN_POINT('Ctrl Pts',(0.55444661522343,-6.74641579463076,
79.8286923976575));
#203425=CARTESIAN_POINT('Ctrl Pts',(0.724564872197164,-6.73025628546016,
79.8367639086099));
#203426=CARTESIAN_POINT('Ctrl Pts',(0.893527435234065,-6.70774908016721,
79.8448354195623));
#203427=CARTESIAN_POINT('Ctrl Pts',(0.911236457571604,-6.70539009250672,
79.8456813973054));
#203428=CARTESIAN_POINT('Ctrl Pts',(0.928932797974419,-6.70296141928674,
79.8465273750486));
#203429=CARTESIAN_POINT('Ctrl Pts',(0.946615858222378,-6.70046322405861,
79.8473733527917));
#203430=CARTESIAN_POINT('Ctrl Pts',(1.11862785791944,-6.67616202557831,
79.8556026027777));
#203431=CARTESIAN_POINT('Ctrl Pts',(1.2899562381074,-6.6451971130301,79.8638318527636));
#203432=CARTESIAN_POINT('Ctrl Pts',(1.46004516960714,-6.60761357092762,
79.8720611027496));
#203433=CARTESIAN_POINT('Ctrl Pts',(1.62993166766089,-6.57007475934273,
79.8802805585918));
#203434=CARTESIAN_POINT('Ctrl Pts',(1.79858130760347,-6.52593308004909,
79.8885000144341));
#203435=CARTESIAN_POINT('Ctrl Pts',(1.96544378896078,-6.47528529969418,
79.8967194702764));
#203436=CARTESIAN_POINT('Ctrl Pts',(2.13214118695583,-6.42468762710348,
79.9049307943002));
#203437=CARTESIAN_POINT('Ctrl Pts',(2.29705460668081,-6.36759677547963,
79.9131421183241));
#203438=CARTESIAN_POINT('Ctrl Pts',(2.45964425939344,-6.30416046093633,
79.9213534423479));
#203439=CARTESIAN_POINT('Ctrl Pts',(2.62210569620719,-6.24077417137282,
79.9295582910378));
#203440=CARTESIAN_POINT('Ctrl Pts',(2.78224668328266,-6.17105251532309,
79.9377631397277));
#203441=CARTESIAN_POINT('Ctrl Pts',(2.93954283066635,-6.09519293760895,
79.9459679884176));
#203442=CARTESIAN_POINT('Ctrl Pts',(3.09674650590379,-6.01937795665121,
79.9541680135948));
#203443=CARTESIAN_POINT('Ctrl Pts',(3.25110835094132,-5.93743239769007,
79.962368038772));
#203444=CARTESIAN_POINT('Ctrl Pts',(3.40212411776653,-5.84960173749558,
79.9705680639492));
#203445=CARTESIAN_POINT('Ctrl Pts',(3.55309617723402,-5.76179649746857,
79.9787657158548));
#203446=CARTESIAN_POINT('Ctrl Pts',(3.70072377584982,-5.66810972558389,
79.9869633677604));
#203447=CARTESIAN_POINT('Ctrl Pts',(3.84452722089665,-5.5688328622598,79.9951610196659));
#203448=CARTESIAN_POINT('Ctrl Pts',(3.98831140979427,-5.46956929270689,
80.0033575738564));
#203449=CARTESIAN_POINT('Ctrl Pts',(4.12827216937939,-5.36471732559827,
80.011554128047));
#203450=CARTESIAN_POINT('Ctrl Pts',(4.26395876097249,-5.25461175394776,
80.0197506822375));
#203451=CARTESIAN_POINT('Ctrl Pts',(4.39965185465598,-5.14450090604725,
80.0279476292062));
#203452=CARTESIAN_POINT('Ctrl Pts',(4.53107009367345,-5.02913617807617,
80.0361445761749));
#203453=CARTESIAN_POINT('Ctrl Pts',(4.65779577200375,-4.90889270063056,
80.0443415231436));
#203454=CARTESIAN_POINT('Ctrl Pts',(4.78455056498328,-4.78862159779195,
80.0525403533237));
#203455=CARTESIAN_POINT('Ctrl Pts',(4.9066103898475,-4.6634697599225,80.0607391835038));
#203456=CARTESIAN_POINT('Ctrl Pts',(5.0235943304235,-4.53384924797207,80.0689380136838));
#203457=CARTESIAN_POINT('Ctrl Pts',(5.14068906973142,-4.40410596884279,
80.0771446092032));
#203458=CARTESIAN_POINT('Ctrl Pts',(5.25269807911143,-4.2698858263462,80.0853512047225));
#203459=CARTESIAN_POINT('Ctrl Pts',(5.35928009382647,-4.13163477039239,
80.0935578002418));
#203460=CARTESIAN_POINT('Ctrl Pts',(5.46591369484532,-3.99331680013794,
80.1017683678002));
#203461=CARTESIAN_POINT('Ctrl Pts',(5.56711485645141,-3.8509643188439,80.1099789353586));
#203462=CARTESIAN_POINT('Ctrl Pts',(5.66258569484486,-3.70505225989302,
80.1181895029171));
#203463=CARTESIAN_POINT('Ctrl Pts',(5.75818820115869,-3.55893896737507,
80.1264113940207));
#203464=CARTESIAN_POINT('Ctrl Pts',(5.84804440549935,-3.40925659385929,
80.1346332851244));
#203465=CARTESIAN_POINT('Ctrl Pts',(5.93190183353251,-3.25650574041159,
80.142855176228));
#203466=CARTESIAN_POINT('Ctrl Pts',(6.00814799222413,-3.1176192268919,80.1503308122991));
#203467=CARTESIAN_POINT('Ctrl Pts',(6.07943540432172,-2.97619644230726,
80.1578064483702));
#203468=CARTESIAN_POINT('Ctrl Pts',(6.14560918025433,-2.83262719106729,
80.1652820844413));
#203469=CARTESIAN_POINT('Ctrl Pts',(6.22470948231096,-2.66101281695794,
80.1742180271611));
#203470=CARTESIAN_POINT('Ctrl Pts',(6.29666781814262,-2.48597403768251,
80.1831539698809));
#203471=CARTESIAN_POINT('Ctrl Pts',(6.36120676037905,-2.30810258691158,
80.1920899126008));
#203472=CARTESIAN_POINT('Ctrl Pts',(6.42564868348748,-2.13049852405331,
80.2010124222314));
#203473=CARTESIAN_POINT('Ctrl Pts',(6.48269337982514,-1.95007052854569,
80.2099349318619));
#203474=CARTESIAN_POINT('Ctrl Pts',(6.53211133643309,-1.76743047626838,
80.2188574414925));
#203475=CARTESIAN_POINT('Ctrl Pts',(6.58140820379596,-1.58523794848564,
80.2277580882209));
#203476=CARTESIAN_POINT('Ctrl Pts',(6.62311556177473,-1.40084443052398,
80.2366587349492));
#203477=CARTESIAN_POINT('Ctrl Pts',(6.65705370659433,-1.21487651533753,
80.2455593816775));
#203478=CARTESIAN_POINT('Ctrl Pts',(6.69093940424708,-1.02919599035258,
80.2544462735672));
#203479=CARTESIAN_POINT('Ctrl Pts',(6.71707979213586,-0.84194617415011,
80.263333165457));
#203480=CARTESIAN_POINT('Ctrl Pts',(6.73534547030215,-0.653766315804292,
80.2722200573467));
#203481=CARTESIAN_POINT('Ctrl Pts',(6.75356419891538,-0.466070149340212,
80.2810841066352));
#203482=CARTESIAN_POINT('Ctrl Pts',(6.76394858228651,-0.277448967141324,
80.2899481559237));
#203483=CARTESIAN_POINT('Ctrl Pts',(6.76642062655753,-0.0885488819625929,
80.2988122052122));
#203484=CARTESIAN_POINT('Ctrl Pts',(6.76878410090522,0.0920548842518706,
80.3072869535635));
#203485=CARTESIAN_POINT('Ctrl Pts',(6.76391525614064,0.272913323144809,
80.3157617019147));
#203486=CARTESIAN_POINT('Ctrl Pts',(6.75178996101479,0.453454873542969,
80.3242364502659));
#203487=CARTESIAN_POINT('Ctrl Pts',(6.74004500892569,0.62833324454433,80.332445364962));
#203488=CARTESIAN_POINT('Ctrl Pts',(6.72150205526021,0.802745656646183,
80.3406542796581));
#203489=CARTESIAN_POINT('Ctrl Pts',(6.69622702346234,0.976131471807344,
80.3488631943541));
#203490=CARTESIAN_POINT('Ctrl Pts',(6.6709459826429,1.14955850864174,80.3570740606815));
#203491=CARTESIAN_POINT('Ctrl Pts',(6.63892972637024,1.32195810991732,80.365284927009));
#203492=CARTESIAN_POINT('Ctrl Pts',(6.60029558116797,1.49277836305817,80.3734957933364));
#203493=CARTESIAN_POINT('Ctrl Pts',(6.56164536418001,1.66366967734154,80.3817100753803));
#203494=CARTESIAN_POINT('Ctrl Pts',(6.5163718521155,1.83297998756787,80.3899243574241));
#203495=CARTESIAN_POINT('Ctrl Pts',(6.46464267260206,2.00017102158102,80.398138639468));
#203496=CARTESIAN_POINT('Ctrl Pts',(6.41285526779065,2.16755024237514,80.4063621673384));
#203497=CARTESIAN_POINT('Ctrl Pts',(6.35459778749166,2.33280508219615,80.4145856952087));
#203498=CARTESIAN_POINT('Ctrl Pts',(6.29008693431294,2.49541486706832,80.4228092230791));
#203499=CARTESIAN_POINT('Ctrl Pts',(6.22553473216907,2.65812887853181,80.4310380219132));
#203500=CARTESIAN_POINT('Ctrl Pts',(6.15472131080019,2.81819413062466,80.4392668207473));
#203501=CARTESIAN_POINT('Ctrl Pts',(6.07791003216543,2.97511321480425,80.4474956195814));
#203502=CARTESIAN_POINT('Ctrl Pts',(6.00099302893615,3.13224828557905,80.4557357447003));
#203503=CARTESIAN_POINT('Ctrl Pts',(5.91806184704512,3.2862282261816,80.4639758698193));
#203504=CARTESIAN_POINT('Ctrl Pts',(5.82942449224626,3.43658247234071,80.4722159949382));
#203505=CARTESIAN_POINT('Ctrl Pts',(5.79007318376855,3.50333352030426,80.4758742686557));
#203506=CARTESIAN_POINT('Ctrl Pts',(5.74959774891652,3.56937035449353,80.4795325423732));
#203507=CARTESIAN_POINT('Ctrl Pts',(5.70802771687682,3.63465384642967,80.4831908160907));
#203508=CARTESIAN_POINT('Ctrl Pts',(5.61203314018049,3.78540814865593,80.4916385949285));
#203509=CARTESIAN_POINT('Ctrl Pts',(5.50997922611138,3.93248806020852,80.5000863737663));
#203510=CARTESIAN_POINT('Ctrl Pts',(5.40217158634465,4.0753933738586,80.5085341526041));
#203511=CARTESIAN_POINT('Ctrl Pts',(5.29445862764512,4.21817318223248,80.5169745122579));
#203512=CARTESIAN_POINT('Ctrl Pts',(5.18100221423595,4.35678543482519,80.5254148719117));
#203513=CARTESIAN_POINT('Ctrl Pts',(5.06215147060626,4.49075845360657,80.5338552315655));
#203514=CARTESIAN_POINT('Ctrl Pts',(4.94338845035151,4.6246325873074,80.5422893614153));
#203515=CARTESIAN_POINT('Ctrl Pts',(4.81923925685959,4.75387406404093,80.5507234912651));
#203516=CARTESIAN_POINT('Ctrl Pts',(4.69009377095809,4.87804360575222,80.5591576211149));
#203517=CARTESIAN_POINT('Ctrl Pts',(4.56103691621416,5.00212793124292,80.5675859627122));
#203518=CARTESIAN_POINT('Ctrl Pts',(4.42699084761324,5.121147033405,80.5760143043094));
#203519=CARTESIAN_POINT('Ctrl Pts',(4.28838298229058,5.23469773694724,80.5844426459066));
#203520=CARTESIAN_POINT('Ctrl Pts',(4.14983311762816,5.34820092503456,80.5928674606523));
#203521=CARTESIAN_POINT('Ctrl Pts',(4.00672551906653,5.45624006508905,80.6012922753979));
#203522=CARTESIAN_POINT('Ctrl Pts',(3.85952187208725,5.55845121584063,80.6097170901435));
#203523=CARTESIAN_POINT('Ctrl Pts',(3.71235445181019,5.66063721250806,80.6181398315488));
#203524=CARTESIAN_POINT('Ctrl Pts',(3.56109326579427,5.75699788833466,80.6265625729541));
#203525=CARTESIAN_POINT('Ctrl Pts',(3.40623060849283,5.84721147571786,80.6349853143594));
#203526=CARTESIAN_POINT('Ctrl Pts',(3.30533641544299,5.90598631052804,80.6404727941183));
#203527=CARTESIAN_POINT('Ctrl Pts',(3.20291415697681,5.96215280184155,80.6459602738772));
#203528=CARTESIAN_POINT('Ctrl Pts',(3.0991061983213,6.01563211736942,80.6514477536361));
#203529=CARTESIAN_POINT('Origin',(0.,0.,4.30282021618968));
#203530=CARTESIAN_POINT('',(3.09910619832137,6.01563211736938,83.0458350405685));
#203531=CARTESIAN_POINT('',(3.09910619832129,6.01563211736943,82.6511646947363));
#203532=CARTESIAN_POINT('',(3.09910619832133,6.0156321173694,4.30282021618968));
#203533=CARTESIAN_POINT('',(-6.76699851999205,-0.00447553632174044,81.6971797837716));
#203534=CARTESIAN_POINT('Ctrl Pts',(-6.76699851999152,-0.00447553713416882,
81.6971797838099));
#203535=CARTESIAN_POINT('Ctrl Pts',(-6.76684449886227,-0.237355015602491,
81.7081713552182));
#203536=CARTESIAN_POINT('Ctrl Pts',(-6.75466803722761,-0.469867458515164,
81.7191629266265));
#203537=CARTESIAN_POINT('Ctrl Pts',(-6.73058789011693,-0.70105324577479,
81.7301544980348));
#203538=CARTESIAN_POINT('Ctrl Pts',(-6.71101117766606,-0.889002997871695,
81.7390904414846));
#203539=CARTESIAN_POINT('Ctrl Pts',(-6.68354502816971,-1.07625201055286,
81.7480263849344));
#203540=CARTESIAN_POINT('Ctrl Pts',(-6.64825291327549,-1.2621498330721,
81.7569623283841));
#203541=CARTESIAN_POINT('Ctrl Pts',(-6.61301385179067,-1.44776820185748,
81.7658848387408));
#203542=CARTESIAN_POINT('Ctrl Pts',(-6.56997234717697,-1.63203918032549,
81.7748073490974));
#203543=CARTESIAN_POINT('Ctrl Pts',(-6.51924335481708,-1.8143194538651,
81.7837298594541));
#203544=CARTESIAN_POINT('Ctrl Pts',(-6.46863866423085,-1.99615308416877,
81.7926305068915));
#203545=CARTESIAN_POINT('Ctrl Pts',(-6.41038414977033,-2.17600549655582,
81.8015311543289));
#203546=CARTESIAN_POINT('Ctrl Pts',(-6.34464511076868,-2.35324614488138,
81.8104318017663));
#203547=CARTESIAN_POINT('Ctrl Pts',(-6.27900766333836,-2.53021288965983,
81.8193186943516));
#203548=CARTESIAN_POINT('Ctrl Pts',(-6.20590885266379,-2.70457568057547,
81.8282055869369));
#203549=CARTESIAN_POINT('Ctrl Pts',(-6.12556369540599,-2.87571876467852,
81.8370924795222));
#203550=CARTESIAN_POINT('Ctrl Pts',(-6.04542505519367,-3.04642194717093,
81.8459565294763));
#203551=CARTESIAN_POINT('Ctrl Pts',(-5.9580773443216,-3.21392170370398,
81.8548205794303));
#203552=CARTESIAN_POINT('Ctrl Pts',(-5.86378328803403,-3.37762261819949,
81.8636846293844));
#203553=CARTESIAN_POINT('Ctrl Pts',(-5.7736305847321,-3.5341338613871,81.8721593742094));
#203554=CARTESIAN_POINT('Ctrl Pts',(-5.67712867345867,-3.68717253080188,
81.8806341190345));
#203555=CARTESIAN_POINT('Ctrl Pts',(-5.57454854344113,-3.83623481252365,
81.8891088638596));
#203556=CARTESIAN_POINT('Ctrl Pts',(-5.47518608158014,-3.98062140357163,
81.897317778289));
#203557=CARTESIAN_POINT('Ctrl Pts',(-5.37021571557012,-4.12113741998357,
81.9055266927183));
#203558=CARTESIAN_POINT('Ctrl Pts',(-5.25998029941111,-4.25733440662195,
81.9137356071477));
#203559=CARTESIAN_POINT('Ctrl Pts',(-5.14971867534191,-4.393563773402,81.9219464732047));
#203560=CARTESIAN_POINT('Ctrl Pts',(-5.03418973133497,-4.52547178789233,
81.9301573392618));
#203561=CARTESIAN_POINT('Ctrl Pts',(-4.91377607024943,-4.65264373571027,
81.9383682053188));
#203562=CARTESIAN_POINT('Ctrl Pts',(-4.79331231718771,-4.77986858694569,
81.9465824870889));
#203563=CARTESIAN_POINT('Ctrl Pts',(-4.66796004342189,-4.90235318810453,
81.9547967688589));
#203564=CARTESIAN_POINT('Ctrl Pts',(-4.53813814433031,-5.01972022955207,
81.963011050629));
#203565=CARTESIAN_POINT('Ctrl Pts',(-4.40817012044269,-5.13721937687014,
81.9712345782216));
#203566=CARTESIAN_POINT('Ctrl Pts',(-4.27372268707219,-5.24958922053345,
81.9794581058142));
#203567=CARTESIAN_POINT('Ctrl Pts',(-4.13524795759656,-5.35649263316898,
81.9876816334069));
#203568=CARTESIAN_POINT('Ctrl Pts',(-3.99668447120583,-5.46346456673359,
81.9959104319608));
#203569=CARTESIAN_POINT('Ctrl Pts',(-3.85408883231614,-5.56496287877393,
82.0041392305148));
#203570=CARTESIAN_POINT('Ctrl Pts',(-3.70794140233327,-5.66069426456356,
82.0123680290687));
#203571=CARTESIAN_POINT('Ctrl Pts',(-3.5615928121081,-5.75655741694507,
82.0206081539054));
#203572=CARTESIAN_POINT('Ctrl Pts',(-3.41168297026833,-5.84663760535682,
82.028848278742));
#203573=CARTESIAN_POINT('Ctrl Pts',(-3.25871692629095,-5.93068739644107,
82.0370884035787));
#203574=CARTESIAN_POINT('Ctrl Pts',(-3.19080631546901,-5.96800203506002,
82.0407466789473));
#203575=CARTESIAN_POINT('Ctrl Pts',(-3.12229359885775,-6.00412872029134,
82.0444049543158));
#203576=CARTESIAN_POINT('Ctrl Pts',(-3.05322414153483,-6.03904887722801,
82.0480632296844));
#203577=CARTESIAN_POINT('Ctrl Pts',(-2.89372265821817,-6.11968968497332,
82.056511252447));
#203578=CARTESIAN_POINT('Ctrl Pts',(-2.73088594234967,-6.19407759388282,
82.0649592752095));
#203579=CARTESIAN_POINT('Ctrl Pts',(-2.56523216055996,-6.26193843489609,
82.0734072979722));
#203580=CARTESIAN_POINT('Ctrl Pts',(-2.39973007288556,-6.32973713371055,
82.081847584628));
#203581=CARTESIAN_POINT('Ctrl Pts',(-2.23141636847651,-6.3910205527999,
82.0902878712839));
#203582=CARTESIAN_POINT('Ctrl Pts',(-2.06083201069516,-6.44556129624831,
82.0987281579397));
#203583=CARTESIAN_POINT('Ctrl Pts',(-1.8903776016018,-6.50006049134993,
82.1071620149077));
#203584=CARTESIAN_POINT('Ctrl Pts',(-1.71765630395417,-6.54782714917387,
82.1155958718757));
#203585=CARTESIAN_POINT('Ctrl Pts',(-1.54322754976388,-6.58868254885981,
82.1240297288437));
#203586=CARTESIAN_POINT('Ctrl Pts',(-1.3689048573118,-6.62951310634169,
82.1324584575887));
#203587=CARTESIAN_POINT('Ctrl Pts',(-1.19287710217506,-6.66344070828384,
82.1408871863339));
#203588=CARTESIAN_POINT('Ctrl Pts',(-1.0157177001322,-6.69033680420038,
82.1493159150789));
#203589=CARTESIAN_POINT('Ctrl Pts',(-0.838638815093584,-6.71722067613647,
82.1577408130593));
#203590=CARTESIAN_POINT('Ctrl Pts',(-0.660429637888545,-6.73707936440374,
82.1661657110397));
#203591=CARTESIAN_POINT('Ctrl Pts',(-0.481672964666132,-6.74983556504229,
82.17459060902));
#203592=CARTESIAN_POINT('Ctrl Pts',(-0.302955868461923,-6.76258894143727,
82.1830136417143));
#203593=CARTESIAN_POINT('Ctrl Pts',(-0.123691850085766,-6.76824293911863,
82.1914366744085));
#203594=CARTESIAN_POINT('Ctrl Pts',(0.0555314560726346,-6.7667721446334,
82.1998597071028));
#203595=CARTESIAN_POINT('Ctrl Pts',(0.234734483317544,-6.76530151656689,
82.2082817867404));
#203596=CARTESIAN_POINT('Ctrl Pts',(0.413896474133007,-6.75670770619259,
82.2167038663781));
#203597=CARTESIAN_POINT('Ctrl Pts',(0.59242975795581,-6.74101742928235,
82.2251259460158));
#203598=CARTESIAN_POINT('Ctrl Pts',(0.770967762853059,-6.72532673746368,
82.2335482483641));
#203599=CARTESIAN_POINT('Ctrl Pts',(0.948876695453036,-6.70253923454659,
82.2419705507124));
#203600=CARTESIAN_POINT('Ctrl Pts',(1.12557359749265,-6.67273355354666,
82.2503928530608));
#203601=CARTESIAN_POINT('Ctrl Pts',(1.30229983904777,-6.64292292348294,
82.2588165538845));
#203602=CARTESIAN_POINT('Ctrl Pts',(1.47781332012457,-6.60609184807301,
82.2672402547082));
#203603=CARTESIAN_POINT('Ctrl Pts',(1.65154050273,-6.56237022483815,82.2756639555319));
#203604=CARTESIAN_POINT('Ctrl Pts',(1.82538524810783,-6.51861901478122,
82.284093356751));
#203605=CARTESIAN_POINT('Ctrl Pts',(1.99744095581411,-6.46796802077563,
82.2925227579701));
#203606=CARTESIAN_POINT('Ctrl Pts',(2.1671475147585,-6.41059752669562,82.3009521591891));
#203607=CARTESIAN_POINT('Ctrl Pts',(2.33691462476739,-6.35320656290303,
82.3093845680068));
#203608=CARTESIAN_POINT('Ctrl Pts',(2.50433060082657,-6.28909143113933,
82.3178169768245));
#203609=CARTESIAN_POINT('Ctrl Pts',(2.66885405457968,-6.21848108748058,
82.3262493856423));
#203610=CARTESIAN_POINT('Ctrl Pts',(2.83352973021915,-6.14780541307741,
82.33468959637));
#203611=CARTESIAN_POINT('Ctrl Pts',(2.99530723229255,-6.0706226569568,82.3431298070977));
#203612=CARTESIAN_POINT('Ctrl Pts',(3.15366756962959,-5.98720885390401,
82.3515700178254));
#203613=CARTESIAN_POINT('Ctrl Pts',(3.24374022720949,-5.93976450612001,
82.3563706656616));
#203614=CARTESIAN_POINT('Ctrl Pts',(3.33270784491619,-5.89030516238423,
82.3611713134978));
#203615=CARTESIAN_POINT('Ctrl Pts',(3.4204789128823,-5.8388879940043,82.365971961334));
#203616=CARTESIAN_POINT('Ctrl Pts',(3.56929871923541,-5.75170786484738,
82.3741116763666));
#203617=CARTESIAN_POINT('Ctrl Pts',(3.71497368254471,-5.65872288260556,
82.3822513913993));
#203618=CARTESIAN_POINT('Ctrl Pts',(3.85701704920413,-5.56018960847098,
82.3903911064319));
#203619=CARTESIAN_POINT('Ctrl Pts',(3.99893618558721,-5.46174251094684,
82.3985237025186));
#203620=CARTESIAN_POINT('Ctrl Pts',(4.13722974863279,-5.35775698770687,
82.4066562986052));
#203621=CARTESIAN_POINT('Ctrl Pts',(4.27143656465306,-5.2485349073951,82.4147888946919));
#203622=CARTESIAN_POINT('Ctrl Pts',(4.40555162969398,-5.13938749715697,
82.4229159308996));
#203623=CARTESIAN_POINT('Ctrl Pts',(4.53558522739118,-5.02501088763539,
82.4310429671073));
#203624=CARTESIAN_POINT('Ctrl Pts',(4.6611061552842,-4.90574952572711,82.439170003315));
#203625=CARTESIAN_POINT('Ctrl Pts',(4.78656708190211,-4.78654517290811,
82.4472931546524));
#203626=CARTESIAN_POINT('Ctrl Pts',(4.90751936936548,-4.66246096916189,
82.4554163059897));
#203627=CARTESIAN_POINT('Ctrl Pts',(5.02356586021245,-4.53388079332793,
82.463539457327));
#203628=CARTESIAN_POINT('Ctrl Pts',(5.13957974113306,-4.40533674947898,
82.4716603259984));
#203629=CARTESIAN_POINT('Ctrl Pts',(5.25069032670882,-4.27229952214212,
82.4797811946698));
#203630=CARTESIAN_POINT('Ctrl Pts',(5.35653824932944,-4.13518886914138,
82.4879020633413));
#203631=CARTESIAN_POINT('Ctrl Pts',(5.46239189237695,-3.99807080615612,
82.4960233708955));
#203632=CARTESIAN_POINT('Ctrl Pts',(5.5629820773229,-3.85687916516457,82.5041446784498));
#203633=CARTESIAN_POINT('Ctrl Pts',(5.65799046218856,-3.71206585741461,
82.512265986004));
#203634=CARTESIAN_POINT('Ctrl Pts',(5.70736012164754,-3.63681582870554,
82.5164860997222));
#203635=CARTESIAN_POINT('Ctrl Pts',(5.75522327816138,-3.5605883772458,82.5207062134404));
#203636=CARTESIAN_POINT('Ctrl Pts',(5.80153993560331,-3.48344992437095,
82.5249263271586));
#203637=CARTESIAN_POINT('Ctrl Pts',(5.90014608446744,-3.31922551381491,
82.5339107656847));
#203638=CARTESIAN_POINT('Ctrl Pts',(5.99169144311935,-3.15095198919124,
82.5428952042108));
#203639=CARTESIAN_POINT('Ctrl Pts',(6.07589018140923,-2.97923606037772,
82.5518796427368));
#203640=CARTESIAN_POINT('Ctrl Pts',(6.16023424169624,-2.80722376011943,
82.5608795878676));
#203641=CARTESIAN_POINT('Ctrl Pts',(6.23720623284492,-2.63175739503266,
82.5698795329984));
#203642=CARTESIAN_POINT('Ctrl Pts',(6.30656822692905,-2.4534641222339,82.5788794781291));
#203643=CARTESIAN_POINT('Ctrl Pts',(6.37609367433266,-2.27475069676127,
82.5879006318616));
#203644=CARTESIAN_POINT('Ctrl Pts',(6.43797315635529,-2.09319725824079,
82.596921785594));
#203645=CARTESIAN_POINT('Ctrl Pts',(6.49201759673769,-1.90944927234219,
82.6059429393265));
#203646=CARTESIAN_POINT('Ctrl Pts',(6.54611702776427,-1.7255143214193,82.614973272154));
#203647=CARTESIAN_POINT('Ctrl Pts',(6.59236542900976,-1.5393805929323,82.6240036049815));
#203648=CARTESIAN_POINT('Ctrl Pts',(6.6306244269346,-1.35170585148481,82.633033937809));
#203649=CARTESIAN_POINT('Ctrl Pts',(6.66893766405852,-1.16376504641265,
82.642077072802));
#203650=CARTESIAN_POINT('Ctrl Pts',(6.69923880258356,-0.974279094345651,
82.6511202077949));
#203651=CARTESIAN_POINT('Ctrl Pts',(6.72144074951205,-0.78391533394807,
82.6601633427879));
#203652=CARTESIAN_POINT('Ctrl Pts',(6.74085036615258,-0.617493550152844,
82.6680691261863));
#203653=CARTESIAN_POINT('Ctrl Pts',(6.75407072242936,-0.450401076252289,
82.6759749095848));
#203654=CARTESIAN_POINT('Ctrl Pts',(6.7610762003542,-0.283085875670381,
82.6838806929833));
#203655=CARTESIAN_POINT('Ctrl Pts',(6.76874414635676,-0.0999486311830835,
82.6925340812115));
#203656=CARTESIAN_POINT('Ctrl Pts',(6.76897170395597,0.0836172998891594,
82.7011874694397));
#203657=CARTESIAN_POINT('Ctrl Pts',(6.76173064094708,0.266997639085809,
82.7098408576679));
#203658=CARTESIAN_POINT('Ctrl Pts',(6.75449626557353,0.450208613531016,
82.7184862538782));
#203659=CARTESIAN_POINT('Ctrl Pts',(6.73980703935953,0.633234035245532,
82.7271316500885));
#203660=CARTESIAN_POINT('Ctrl Pts',(6.71768676693586,0.8154590739791,82.7357770462988));
#203661=CARTESIAN_POINT('Ctrl Pts',(6.69486004752519,1.00350376660773,82.7446985473413));
#203662=CARTESIAN_POINT('Ctrl Pts',(6.66411975782486,1.19069578225963,82.7536200483838));
#203663=CARTESIAN_POINT('Ctrl Pts',(6.62555026623527,1.37636211426706,82.7625415494262));
#203664=CARTESIAN_POINT('Ctrl Pts',(6.58824561820975,1.55593972548965,82.7711704797681));
#203665=CARTESIAN_POINT('Ctrl Pts',(6.54361717444127,1.73408980035634,82.7797994101099));
#203666=CARTESIAN_POINT('Ctrl Pts',(6.4917936668636,1.91021045617222,82.7884283404518));
#203667=CARTESIAN_POINT('Ctrl Pts',(6.4373344838341,2.09528837695898,82.7974961268446));
#203668=CARTESIAN_POINT('Ctrl Pts',(6.37492934271898,2.27812473444926,82.8065639132373));
#203669=CARTESIAN_POINT('Ctrl Pts',(6.3047881599716,2.45803483658835,82.81563169963));
#203670=CARTESIAN_POINT('Ctrl Pts',(6.2346469772242,2.6379449387275,82.8246994860228));
#203671=CARTESIAN_POINT('Ctrl Pts',(6.15676986189347,2.81492840888824,82.8337672724156));
#203672=CARTESIAN_POINT('Ctrl Pts',(6.07142741218859,2.98832029383147,82.8428350588083));
#203673=CARTESIAN_POINT('Ctrl Pts',(5.99213502880834,3.14942014347823,82.8512600149415));
#203674=CARTESIAN_POINT('Ctrl Pts',(5.90643326115009,3.30734900210329,82.8596849710747));
#203675=CARTESIAN_POINT('Ctrl Pts',(5.81460892997491,3.46159096247029,82.8681099272079));
#203676=CARTESIAN_POINT('Ctrl Pts',(5.7227632854908,3.6158687238773,82.8765368388543));
#203677=CARTESIAN_POINT('Ctrl Pts',(5.62479241364502,3.7664575958224,82.8849637505007));
#203678=CARTESIAN_POINT('Ctrl Pts',(5.52102743361863,3.91286916178275,82.8933906621471));
#203679=CARTESIAN_POINT('Ctrl Pts',(5.41722429516715,4.05933456897905,82.9018206726972));
#203680=CARTESIAN_POINT('Ctrl Pts',(5.30762299173378,4.20161933681769,82.9102506832473));
#203681=CARTESIAN_POINT('Ctrl Pts',(5.19259625134287,4.33926643230628,82.9186806937974));
#203682=CARTESIAN_POINT('Ctrl Pts',(5.07746355072462,4.47704032542017,82.9271184698969));
#203683=CARTESIAN_POINT('Ctrl Pts',(4.9568956407762,4.61016775621796,82.9355562459964));
#203684=CARTESIAN_POINT('Ctrl Pts',(4.83130434358136,4.73822618072332,82.9439940220958));
#203685=CARTESIAN_POINT('Ctrl Pts',(4.70564712021333,4.86635182646184,82.9524362274058));
#203686=CARTESIAN_POINT('Ctrl Pts',(4.57496148808737,4.98940292814892,82.9608784327157));
#203687=CARTESIAN_POINT('Ctrl Pts',(4.43969438295703,5.10699547541798,82.9693206380257));
#203688=CARTESIAN_POINT('Ctrl Pts',(4.30428457847358,5.22471207635414,82.9777717493977));
#203689=CARTESIAN_POINT('Ctrl Pts',(4.16428390133668,5.33695840839891,82.9862228607697));
#203690=CARTESIAN_POINT('Ctrl Pts',(4.02017128777912,5.44339157299164,82.9946739721418));
#203691=CARTESIAN_POINT('Ctrl Pts',(3.97972585955839,5.47326220549613,82.9970457896388));
#203692=CARTESIAN_POINT('Ctrl Pts',(3.93895672434481,5.50267522728859,82.9994176071359));
#203693=CARTESIAN_POINT('Ctrl Pts',(3.89787485526619,5.53162368682863,83.0017894246329));
#203694=CARTESIAN_POINT('Ctrl Pts',(3.75383633567919,5.63312085212294,83.0101053335404));
#203695=CARTESIAN_POINT('Ctrl Pts',(3.60569134154582,5.72908693007432,83.0184212424479));
#203696=CARTESIAN_POINT('Ctrl Pts',(3.45389851985335,5.81918155882379,83.0267371513554));
#203697=CARTESIAN_POINT('Ctrl Pts',(3.3376986542595,5.88815045758124,83.0331031144264));
#203698=CARTESIAN_POINT('Ctrl Pts',(3.2193618466181,5.95367935534069,83.0394690774975));
#203699=CARTESIAN_POINT('Ctrl Pts',(3.09910619832137,6.01563211736938,83.0458350405685));
#203700=CARTESIAN_POINT('Ctrl Pts',(3.09910619832132,6.01563211736941,81.0456744569491));
#203701=CARTESIAN_POINT('Ctrl Pts',(2.94210478641535,6.09651539601574,81.0540061427842));
#203702=CARTESIAN_POINT('Ctrl Pts',(2.78208187347672,6.171172809358,81.0623378286193));
#203703=CARTESIAN_POINT('Ctrl Pts',(2.61957258730343,6.23940129017588,81.0706695144544));
#203704=CARTESIAN_POINT('Ctrl Pts',(2.46569449257949,6.30400602065859,81.0785586878816));
#203705=CARTESIAN_POINT('Ctrl Pts',(2.3095875099172,6.36284691913867,81.0864478613087));
#203706=CARTESIAN_POINT('Ctrl Pts',(2.15171708221271,6.41579321659559,81.0943370347359));
#203707=CARTESIAN_POINT('Ctrl Pts',(1.99023121152499,6.46995205475702,81.1024068807382));
#203708=CARTESIAN_POINT('Ctrl Pts',(1.82640100248875,6.51810993784101,81.1104767267405));
#203709=CARTESIAN_POINT('Ctrl Pts',(1.6607218399461,6.56005274142869,81.1185465727428));
#203710=CARTESIAN_POINT('Ctrl Pts',(1.49525112286374,6.60194277563448,81.1266062658523));
#203711=CARTESIAN_POINT('Ctrl Pts',(1.32793643788382,6.63763319832059,81.1346659589618));
#203712=CARTESIAN_POINT('Ctrl Pts',(1.15929269380034,6.66695803572372,81.1427256520714));
#203713=CARTESIAN_POINT('Ctrl Pts',(0.990824113030937,6.69625241462552,
81.1507769739096));
#203714=CARTESIAN_POINT('Ctrl Pts',(0.821029584695862,6.71919430216325,
81.1588282957477));
#203715=CARTESIAN_POINT('Ctrl Pts',(0.650438617202402,6.73566764361573,
81.1668796175859));
#203716=CARTESIAN_POINT('Ctrl Pts',(0.479987453230496,6.75212748475701,
81.1749243411664));
#203717=CARTESIAN_POINT('Ctrl Pts',(0.308741518659208,6.76212929509531,
81.182969064747));
#203718=CARTESIAN_POINT('Ctrl Pts',(0.137239838793602,6.76560819340345,
81.1910137883275));
#203719=CARTESIAN_POINT('Ctrl Pts',(-0.0341588329914937,6.76908500220065,
81.1990536800514));
#203720=CARTESIAN_POINT('Ctrl Pts',(-0.205812572206715,6.76604669058816,
81.2070935717753));
#203721=CARTESIAN_POINT('Ctrl Pts',(-0.377178023321409,6.75648027738729,
81.2151334634992));
#203722=CARTESIAN_POINT('Ctrl Pts',(-0.552233442102512,6.74670787310032,
81.2233464761195));
#203723=CARTESIAN_POINT('Ctrl Pts',(-0.726987619962262,6.73012300380536,
81.2315594887397));
#203724=CARTESIAN_POINT('Ctrl Pts',(-0.900861684984169,6.70676801630469,
81.23977250136));
#203725=CARTESIAN_POINT('Ctrl Pts',(-1.07101129665723,6.68391330215645,
81.2478095879021));
#203726=CARTESIAN_POINT('Ctrl Pts',(-1.24031773478452,6.65457563381443,
81.2558466744441));
#203727=CARTESIAN_POINT('Ctrl Pts',(-1.40824455710652,6.61884704970434,
81.2638837609862));
#203728=CARTESIAN_POINT('Ctrl Pts',(-1.57618745080706,6.58311504620245,
81.2719216167149));
#203729=CARTESIAN_POINT('Ctrl Pts',(-1.74275010031391,6.5409909866855,81.2799594724435));
#203730=CARTESIAN_POINT('Ctrl Pts',(-1.90740742616755,6.4926178010569,81.2879973281722));
#203731=CARTESIAN_POINT('Ctrl Pts',(-2.07211313460704,6.44423040154625,
81.2960375457286));
#203732=CARTESIAN_POINT('Ctrl Pts',(-2.23491204674428,6.38959032622561,
81.3040777632851));
#203733=CARTESIAN_POINT('Ctrl Pts',(-2.39529552841332,6.32888997625675,
81.3121179808415));
#203734=CARTESIAN_POINT('Ctrl Pts',(-2.561738400809,6.26589632816343,81.3204619629702));
#203735=CARTESIAN_POINT('Ctrl Pts',(-2.72557934853586,6.19637569642848,
81.3288059450988));
#203736=CARTESIAN_POINT('Ctrl Pts',(-2.88627507206607,6.12059680165015,
81.3371499272275));
#203737=CARTESIAN_POINT('Ctrl Pts',(-3.04139020298881,6.04744953346841,
81.345204142062));
#203738=CARTESIAN_POINT('Ctrl Pts',(-3.19357460436433,5.96847161385049,
81.3532583568966));
#203739=CARTESIAN_POINT('Ctrl Pts',(-3.34236735467854,5.88395015838673,
81.3613125717311));
#203740=CARTESIAN_POINT('Ctrl Pts',(-3.49127145176187,5.79936545259009,
81.3693728138136));
#203741=CARTESIAN_POINT('Ctrl Pts',(-3.63677852870179,5.70922914630083,
81.3774330558961));
#203742=CARTESIAN_POINT('Ctrl Pts',(-3.77845849628231,5.61387035759395,
81.3854932979786));
#203743=CARTESIAN_POINT('Ctrl Pts',(-3.92033654217598,5.51837825075937,
81.3935648088324));
#203744=CARTESIAN_POINT('Ctrl Pts',(-4.05837650447829,5.41764931211516,
81.4016363196862));
#203745=CARTESIAN_POINT('Ctrl Pts',(-4.19218262275185,5.31205175591291,
81.40970783054));
#203746=CARTESIAN_POINT('Ctrl Pts',(-4.20620690106646,5.30098402943948,
81.4105538091551));
#203747=CARTESIAN_POINT('Ctrl Pts',(-4.22018470439754,5.28986285200514,
81.4113997877703));
#203748=CARTESIAN_POINT('Ctrl Pts',(-4.23411560180295,5.27868866960052,
81.4122457663854));
#203749=CARTESIAN_POINT('Ctrl Pts',(-4.36845503934569,5.17093298555859,
81.4204037685602));
#203750=CARTESIAN_POINT('Ctrl Pts',(-4.4988921346547,5.05787415795229,81.428561770735));
#203751=CARTESIAN_POINT('Ctrl Pts',(-4.62497610536319,4.93982641646643,
81.4367197729098));
#203752=CARTESIAN_POINT('Ctrl Pts',(-4.75090927689525,4.82191986265173,
81.4448680179362));
#203753=CARTESIAN_POINT('Ctrl Pts',(-4.87249942391205,4.69903652038096,
81.4530162629626));
#203754=CARTESIAN_POINT('Ctrl Pts',(-4.98932656618061,4.57153250190835,
81.461164507989));
#203755=CARTESIAN_POINT('Ctrl Pts',(-5.10603856463953,4.44415415028118,
81.4693047221764));
#203756=CARTESIAN_POINT('Ctrl Pts',(-5.21799665939793,4.31216445731424,
81.4774449363638));
#203757=CARTESIAN_POINT('Ctrl Pts',(-5.32481567914318,4.17595821137508,
81.4855851505511));
#203758=CARTESIAN_POINT('Ctrl Pts',(-5.43155188351587,4.03985756433609,
81.4937190537382));
#203759=CARTESIAN_POINT('Ctrl Pts',(-5.53315672209,3.89954716054724,81.5018529569252));
#203760=CARTESIAN_POINT('Ctrl Pts',(-5.62928349726135,3.7554568706698,81.5099868601123));
#203761=CARTESIAN_POINT('Ctrl Pts',(-5.72535678064825,3.61144676289266,
81.5181162370162));
#203762=CARTESIAN_POINT('Ctrl Pts',(-5.81595786936321,3.46366126170424,
81.5262456139202));
#203763=CARTESIAN_POINT('Ctrl Pts',(-5.90078181708742,3.31256138767729,
81.5343749908241));
#203764=CARTESIAN_POINT('Ctrl Pts',(-5.9855811562542,3.16150534973705,81.5425020092875));
#203765=CARTESIAN_POINT('Ctrl Pts',(-6.06460651182814,3.0071371716185,81.5506290277509));
#203766=CARTESIAN_POINT('Ctrl Pts',(-6.1375975210793,2.84994485371932,81.5587560462143));
#203767=CARTESIAN_POINT('Ctrl Pts',(-6.21058124993748,2.69276821476278,
81.5668822540589));
#203768=CARTESIAN_POINT('Ctrl Pts',(-6.27753167707233,2.5327683287134,81.5750084619034));
#203769=CARTESIAN_POINT('Ctrl Pts',(-6.33823548707841,2.37045563348903,
81.5831346697479));
#203770=CARTESIAN_POINT('Ctrl Pts',(-6.39894479854332,2.20812822820593,
81.5912616140536));
#203771=CARTESIAN_POINT('Ctrl Pts',(-6.45340623847369,2.04348793934419,
81.5993885583594));
#203772=CARTESIAN_POINT('Ctrl Pts',(-6.5014555272332,1.87706287252424,81.6075155026651));
#203773=CARTESIAN_POINT('Ctrl Pts',(-6.54953903645635,1.7105192786023,81.6156482349399));
#203774=CARTESIAN_POINT('Ctrl Pts',(-6.5912011704572,1.54218871938156,81.6237809672148));
#203775=CARTESIAN_POINT('Ctrl Pts',(-6.62632804143762,1.3726127229694,81.6319136994897));
#203776=CARTESIAN_POINT('Ctrl Pts',(-6.66146828452887,1.20297217230138,
81.6400495277362));
#203777=CARTESIAN_POINT('Ctrl Pts',(-6.69006824454796,1.03208559991146,
81.6481853559828));
#203778=CARTESIAN_POINT('Ctrl Pts',(-6.71206564568308,0.86050204418177,
81.6563211842293));
#203779=CARTESIAN_POINT('Ctrl Pts',(-6.73408768690814,0.68872629146398,
81.6644661257133));
#203780=CARTESIAN_POINT('Ctrl Pts',(-6.74949236136949,0.516252359863862,
81.6726110671973));
#203781=CARTESIAN_POINT('Ctrl Pts',(-6.75826942861491,0.3436325512072,81.6807560086813));
#203782=CARTESIAN_POINT('Ctrl Pts',(-6.76416890125792,0.227606797918737,
81.686230600378));
#203783=CARTESIAN_POINT('Ctrl Pts',(-6.76707523355838,0.111515163443945,
81.6917051920748));
#203784=CARTESIAN_POINT('Ctrl Pts',(-6.76699851999205,-0.00447553632183878,
81.6971797837716));
#203785=CARTESIAN_POINT('',(-6.76699999999136,-1.0814002431372E-5,81.3028202162286));
#203786=CARTESIAN_POINT('Ctrl Pts',(3.0991061983213,6.01563211736942,80.6514477536361));
#203787=CARTESIAN_POINT('Ctrl Pts',(2.9397834969441,6.09771126744672,80.6598698448734));
#203788=CARTESIAN_POINT('Ctrl Pts',(2.77719573725724,6.1734582995146,80.6682919361106));
#203789=CARTESIAN_POINT('Ctrl Pts',(2.61187701857521,6.24262664587902,80.6767140273478));
#203790=CARTESIAN_POINT('Ctrl Pts',(2.44653889357179,6.31180311173027,80.6851371072317));
#203791=CARTESIAN_POINT('Ctrl Pts',(2.27846947826298,6.37439922403963,80.6935601871156));
#203792=CARTESIAN_POINT('Ctrl Pts',(2.10822248442043,6.43021671144792,80.7019832669995));
#203793=CARTESIAN_POINT('Ctrl Pts',(1.9378637769666,6.48607082548292,80.7104118739865));
#203794=CARTESIAN_POINT('Ctrl Pts',(1.76532495233179,6.53513732031799,80.7188404809734));
#203795=CARTESIAN_POINT('Ctrl Pts',(1.59117553345244,6.57726762582627,80.7272690879603));
#203796=CARTESIAN_POINT('Ctrl Pts',(1.41697174456474,6.61941108455135,80.7357003263855));
#203797=CARTESIAN_POINT('Ctrl Pts',(1.24115668445808,6.65461396335232,80.7441315648106));
#203798=CARTESIAN_POINT('Ctrl Pts',(1.06431026002788,6.68277881351758,80.7525628032357));
#203799=CARTESIAN_POINT('Ctrl Pts',(0.887288511139442,6.71097158614219,
80.7610024003388));
#203800=CARTESIAN_POINT('Ctrl Pts',(0.709233685047566,6.73211233764841,
80.7694419974419));
#203801=CARTESIAN_POINT('Ctrl Pts',(0.530732312228089,6.74615536529934,
80.777881594545));
#203802=CARTESIAN_POINT('Ctrl Pts',(0.36704217122651,6.75903316640507,80.7856209122767));
#203803=CARTESIAN_POINT('Ctrl Pts',(0.202976761306707,6.76594283975284,
80.7933602300084));
#203804=CARTESIAN_POINT('Ctrl Pts',(0.0389883967627574,6.76688768230402,
80.8010995477402));
#203805=CARTESIAN_POINT('Ctrl Pts',(-0.133483982855122,6.76788140672843,
80.8092392627103));
#203806=CARTESIAN_POINT('Ctrl Pts',(-0.30621500353927,6.76227820303757,
80.8173789776805));
#203807=CARTESIAN_POINT('Ctrl Pts',(-0.478655139864533,6.75005024107831,
80.8255186926507));
#203808=CARTESIAN_POINT('Ctrl Pts',(-0.650944461079201,6.73783297362135,
80.8336512886749));
#203809=CARTESIAN_POINT('Ctrl Pts',(-0.822943041537907,6.71900250649092,
80.8417838846991));
#203810=CARTESIAN_POINT('Ctrl Pts',(-0.994100226346764,6.69358302704742,
80.8499164807233));
#203811=CARTESIAN_POINT('Ctrl Pts',(-1.16514039892165,6.66818092572381,
80.8580435168685));
#203812=CARTESIAN_POINT('Ctrl Pts',(-1.33533996033664,6.63619883409692,
80.8661705530137));
#203813=CARTESIAN_POINT('Ctrl Pts',(-1.50415229546543,6.59771285159078,
80.874297589159));
#203814=CARTESIAN_POINT('Ctrl Pts',(-1.6728839352451,6.55924526608028,80.882420740434));
#203815=CARTESIAN_POINT('Ctrl Pts',(-1.84022931293789,6.51428006191169,
80.890543891709));
#203816=CARTESIAN_POINT('Ctrl Pts',(-2.00565096226898,6.46294462436044,
80.898667042984));
#203817=CARTESIAN_POINT('Ctrl Pts',(-2.17102612688705,6.41162361244872,
80.9067879115931));
#203818=CARTESIAN_POINT('Ctrl Pts',(-2.33447829066059,6.35393604184711,
80.9149087802022));
#203819=CARTESIAN_POINT('Ctrl Pts',(-2.49548416997083,6.29005943989602,
80.9230296488113));
#203820=CARTESIAN_POINT('Ctrl Pts',(-2.65649875066311,6.22617938580567,
80.9311509563037));
#203821=CARTESIAN_POINT('Ctrl Pts',(-2.81506644088867,6.15610976349821,
80.939272263796));
#203822=CARTESIAN_POINT('Ctrl Pts',(-2.97068282382818,6.08007669032326,
80.9473935712883));
#203823=CARTESIAN_POINT('Ctrl Pts',(-3.05154651372621,6.0405672586357,80.9516136853805));
#203824=CARTESIAN_POINT('Ctrl Pts',(-3.13161363381079,5.9994483599442,80.9558337994728));
#203825=CARTESIAN_POINT('Ctrl Pts',(-3.21081588728411,5.95675669622018,
80.960053913565));
#203826=CARTESIAN_POINT('Ctrl Pts',(-3.37943402629467,5.86586800842756,
80.9690383521819));
#203827=CARTESIAN_POINT('Ctrl Pts',(-3.54404722440834,5.76789338143807,
80.9780227907987));
#203828=CARTESIAN_POINT('Ctrl Pts',(-3.70410000890383,5.66320864210729,
80.9870072294156));
#203829=CARTESIAN_POINT('Ctrl Pts',(-3.86442903502222,5.558343223119,80.9960071746411));
#203830=CARTESIAN_POINT('Ctrl Pts',(-4.02018171549801,5.44674467480157,
81.0050071198667));
#203831=CARTESIAN_POINT('Ctrl Pts',(-4.17083333289308,5.32883085762984,
81.0140070650922));
#203832=CARTESIAN_POINT('Ctrl Pts',(-4.32183996475892,5.21063917346854,
81.0230282189237));
#203833=CARTESIAN_POINT('Ctrl Pts',(-4.46772129296103,5.08610259167696,
81.0320493727553));
#203834=CARTESIAN_POINT('Ctrl Pts',(-4.60798526343422,4.95567965187148,
81.0410705265868));
#203835=CARTESIAN_POINT('Ctrl Pts',(-4.74839195362789,4.82512400567356,
81.050100859515));
#203836=CARTESIAN_POINT('Ctrl Pts',(-4.88316969675948,4.68867020304724,
81.0591311924432));
#203837=CARTESIAN_POINT('Ctrl Pts',(-5.01186376137092,4.54681323978201,
81.0681615253715));
#203838=CARTESIAN_POINT('Ctrl Pts',(-5.1407402736086,4.40475516804848,81.0772046604659));
#203839=CARTESIAN_POINT('Ctrl Pts',(-5.26351570130875,4.25727879643791,
81.0862477955604));
#203840=CARTESIAN_POINT('Ctrl Pts',(-5.37977452335198,4.10491352867426,
81.0952909306549));
#203841=CARTESIAN_POINT('Ctrl Pts',(-5.48141151086053,3.97171119147293,
81.1031967135665));
#203842=CARTESIAN_POINT('Ctrl Pts',(-5.57806856415838,3.83477294544959,
81.1111024964781));
#203843=CARTESIAN_POINT('Ctrl Pts',(-5.6694950009845,3.69447092745521,81.1190082793898));
#203844=CARTESIAN_POINT('Ctrl Pts',(-5.76956711990332,3.54090133952534,
81.1276616675687));
#203845=CARTESIAN_POINT('Ctrl Pts',(-5.86345990784307,3.38316533597308,
81.1363150557477));
#203846=CARTESIAN_POINT('Ctrl Pts',(-5.95083554270128,3.2217767371007,81.1449684439267));
#203847=CARTESIAN_POINT('Ctrl Pts',(-6.03813047995985,3.06053719205275,
81.1536138400876));
#203848=CARTESIAN_POINT('Ctrl Pts',(-6.11892012502693,2.89565204649202,
81.1622592362485));
#203849=CARTESIAN_POINT('Ctrl Pts',(-6.19291112170672,2.72766215625052,
81.1709046324094));
#203850=CARTESIAN_POINT('Ctrl Pts',(-6.26926514222222,2.55430723333459,
81.1798261334765));
#203851=CARTESIAN_POINT('Ctrl Pts',(-6.33837888946051,2.3776462407962,81.1887476345436));
#203852=CARTESIAN_POINT('Ctrl Pts',(-6.39998139241647,2.19830097500841,
81.1976691356107));
#203853=CARTESIAN_POINT('Ctrl Pts',(-6.45956370932354,2.02483713913816,
81.2062980659034));
#203854=CARTESIAN_POINT('Ctrl Pts',(-6.51211948838974,1.84886260438781,
81.2149269961962));
#203855=CARTESIAN_POINT('Ctrl Pts',(-6.55745221137515,1.67096065050354,
81.2235559264889));
#203856=CARTESIAN_POINT('Ctrl Pts',(-6.60509049763723,1.48401083483837,
81.2326237129432));
#203857=CARTESIAN_POINT('Ctrl Pts',(-6.64475173378035,1.29493275011024,
81.2416914993975));
#203858=CARTESIAN_POINT('Ctrl Pts',(-6.67626694563522,1.10442232439344,
81.2507592858517));
#203859=CARTESIAN_POINT('Ctrl Pts',(-6.70778215749009,0.913911898676632,
81.259827072306));
#203860=CARTESIAN_POINT('Ctrl Pts',(-6.73115124658922,0.721969511502301,
81.2688948587602));
#203861=CARTESIAN_POINT('Ctrl Pts',(-6.74626749550357,0.529305090767147,
81.2779626452145));
#203862=CARTESIAN_POINT('Ctrl Pts',(-6.76008024654131,0.353254425517801,
81.2862485022062));
#203863=CARTESIAN_POINT('Ctrl Pts',(-6.76700028223179,0.176618259281482,
81.294534359198));
#203864=CARTESIAN_POINT('Ctrl Pts',(-6.76699999999136,-1.08131744157636E-5,
81.3028202161898));
#203865=CARTESIAN_POINT('Ctrl Pts',(-6.76699999999136,-1.08140023413723E-5,
81.3028202162286));
#203866=CARTESIAN_POINT('Ctrl Pts',(-6.76699970791981,-0.182778316985658,
81.3113940335024));
#203867=CARTESIAN_POINT('Ctrl Pts',(-6.7595906328111,-0.365468940004556,
81.3199678507761));
#203868=CARTESIAN_POINT('Ctrl Pts',(-6.74481736487667,-0.547473939524143,
81.3285416680498));
#203869=CARTESIAN_POINT('Ctrl Pts',(-6.73003416201002,-0.729601336291533,
81.3371212511632));
#203870=CARTESIAN_POINT('Ctrl Pts',(-6.70787690894711,-0.911041880323436,
81.3457008342765));
#203871=CARTESIAN_POINT('Ctrl Pts',(-6.67844190688181,-1.09119324429949,
81.3542804173899));
#203872=CARTESIAN_POINT('Ctrl Pts',(-6.64897036818727,-1.27156822380576,
81.362870650037));
#203873=CARTESIAN_POINT('Ctrl Pts',(-6.61220307661963,-1.4506505185501,
81.371460882684));
#203874=CARTESIAN_POINT('Ctrl Pts',(-6.56828749042721,-1.62784779481913,
81.3800511153311));
#203875=CARTESIAN_POINT('Ctrl Pts',(-6.52434159461615,-1.80516736894028,
81.388647276777));
#203876=CARTESIAN_POINT('Ctrl Pts',(-6.47323764070425,-1.98059902926588,
81.3972434382229));
#203877=CARTESIAN_POINT('Ctrl Pts',(-6.41517285708126,-2.15356592974719,
81.4058395996688));
#203878=CARTESIAN_POINT('Ctrl Pts',(-6.35703981832765,-2.32673615275291,
81.4144458658991));
#203879=CARTESIAN_POINT('Ctrl Pts',(-6.29192970565408,-2.49743553495125,
81.4230521321295));
#203880=CARTESIAN_POINT('Ctrl Pts',(-6.2200882296409,-2.66510626720264,
81.4316583983598));
#203881=CARTESIAN_POINT('Ctrl Pts',(-6.20545600367273,-2.69925640134103,
81.4334112692529));
#203882=CARTESIAN_POINT('Ctrl Pts',(-6.19054469472299,-2.73328097576781,
81.4351641401461));
#203883=CARTESIAN_POINT('Ctrl Pts',(-6.17535661333137,-2.76717540069012,
81.4369170110392));
#203884=CARTESIAN_POINT('Ctrl Pts',(-6.10329869816184,-2.92798317705082,
81.4452332834416));
#203885=CARTESIAN_POINT('Ctrl Pts',(-6.02488576505313,-3.08613048155137,
81.4535495558439));
#203886=CARTESIAN_POINT('Ctrl Pts',(-5.94033851401064,-3.24109045522674,
81.4618658282463));
#203887=CARTESIAN_POINT('Ctrl Pts',(-5.85586274776895,-3.395919410061,81.4701750692305));
#203888=CARTESIAN_POINT('Ctrl Pts',(-5.76526316296489,-3.54756609939069,
81.4784843102147));
#203889=CARTESIAN_POINT('Ctrl Pts',(-5.66880778399605,-3.69552530881684,
81.4867935511988));
#203890=CARTESIAN_POINT('Ctrl Pts',(-5.57241627341678,-3.84338654634624,
81.4950972901795));
#203891=CARTESIAN_POINT('Ctrl Pts',(-5.47017688428602,-3.98756487879765,
81.5034010291601));
#203892=CARTESIAN_POINT('Ctrl Pts',(-5.36240274750198,-4.1275811044222,
81.5117047681407));
#203893=CARTESIAN_POINT('Ctrl Pts',(-5.25468022266644,-4.26753027768668,
81.5200045305444));
#203894=CARTESIAN_POINT('Ctrl Pts',(-5.14142844419832,-4.4033210411868,
81.528304292948));
#203895=CARTESIAN_POINT('Ctrl Pts',(-5.02300302361465,-4.53450434168477,
81.5366040553517));
#203896=CARTESIAN_POINT('Ctrl Pts',(-4.90461261987558,-4.66564885300029,
81.5449013636244));
#203897=CARTESIAN_POINT('Ctrl Pts',(-4.78105185617886,-4.79218835893123,
81.5531986718971));
#203898=CARTESIAN_POINT('Ctrl Pts',(-4.65271581509934,-4.91370782036585,
81.5614959801698));
#203899=CARTESIAN_POINT('Ctrl Pts',(-4.52436680752477,-5.03523955957903,
81.5697941267651));
#203900=CARTESIAN_POINT('Ctrl Pts',(-4.39124180596366,-5.15174999613048,
81.5780922733604));
#203901=CARTESIAN_POINT('Ctrl Pts',(-4.25377227858367,-5.26286142720413,
81.5863904199557));
#203902=CARTESIAN_POINT('Ctrl Pts',(-4.11628892777808,-5.37398403123103,
81.5946894009819));
#203903=CARTESIAN_POINT('Ctrl Pts',(-3.97446045079063,-5.47970632839051,
81.6029883820081));
#203904=CARTESIAN_POINT('Ctrl Pts',(-3.82875080005061,-5.57969141719431,
81.6112873630342));
#203905=CARTESIAN_POINT('Ctrl Pts',(-3.68300228199366,-5.67970317651797,
81.6195885577718));
#203906=CARTESIAN_POINT('Ctrl Pts',(-3.53337081375088,-5.77397448037678,
81.6278897525095));
#203907=CARTESIAN_POINT('Ctrl Pts',(-3.38034882694759,-5.86221210876526,
81.6361909472471));
#203908=CARTESIAN_POINT('Ctrl Pts',(-3.22726058878378,-5.95048793991827,
81.6444957360137));
#203909=CARTESIAN_POINT('Ctrl Pts',(-3.07077920774856,-6.03272471552547,
81.6528005247802));
#203910=CARTESIAN_POINT('Ctrl Pts',(-2.9114213296124,-6.10867537535577,
81.6611053135468));
#203911=CARTESIAN_POINT('Ctrl Pts',(-2.75187453414262,-6.18471607401132,
81.6694199475658));
#203912=CARTESIAN_POINT('Ctrl Pts',(-2.58944474282217,-6.25445561775319,
81.6777345815849));
#203913=CARTESIAN_POINT('Ctrl Pts',(-2.42466927924726,-6.31769482376876,
81.686049215604));
#203914=CARTESIAN_POINT('Ctrl Pts',(-2.25978962668599,-6.38097401649491,
81.6943691070398));
#203915=CARTESIAN_POINT('Ctrl Pts',(-2.09256167309976,-6.43774456298398,
81.7026889984757));
#203916=CARTESIAN_POINT('Ctrl Pts',(-1.92353762137143,-6.48785727487657,
81.7110088899116));
#203917=CARTESIAN_POINT('Ctrl Pts',(-1.75426082387943,-6.53804492152256,
81.7193412222829));
#203918=CARTESIAN_POINT('Ctrl Pts',(-1.58318289791363,-6.5815547516397,
81.7276735546541));
#203919=CARTESIAN_POINT('Ctrl Pts',(-1.41086728702232,-6.6182884870947,
81.7360058870254));
#203920=CARTESIAN_POINT('Ctrl Pts',(-1.28113350697068,-6.645944753009,81.7422791722466));
#203921=CARTESIAN_POINT('Ctrl Pts',(-1.15069837691565,-6.66976114965995,
81.7485524574677));
#203922=CARTESIAN_POINT('Ctrl Pts',(-1.01980382054277,-6.68971517836196,
81.7548257426889));
#203923=CARTESIAN_POINT('Ctrl Pts',(-0.851423318902484,-6.71538369702073,
81.7628955886912));
#203924=CARTESIAN_POINT('Ctrl Pts',(-0.681762116722721,-6.73473816862062,
81.7709654346935));
#203925=CARTESIAN_POINT('Ctrl Pts',(-0.511344976443914,-6.74765257812416,
81.7790352806958));
#203926=CARTESIAN_POINT('Ctrl Pts',(-0.34114224260392,-6.76055073965788,
81.7870949738053));
#203927=CARTESIAN_POINT('Ctrl Pts',(-0.170185830310789,-6.7670249328393,
81.7951546669149));
#203928=CARTESIAN_POINT('Ctrl Pts',(0.000988519058528649,-6.76699992779888,
81.8032143600244));
#203929=CARTESIAN_POINT('Ctrl Pts',(0.171985076677993,-6.76697494873017,
81.8112656818626));
#203930=CARTESIAN_POINT('Ctrl Pts',(0.34319875099108,-6.76046420495569,
81.8193170037007));
#203931=CARTESIAN_POINT('Ctrl Pts',(0.514087976305923,-6.7474441496479,
81.8273683255389));
#203932=CARTESIAN_POINT('Ctrl Pts',(0.684837153669671,-6.7344347645978,
81.8354130491194));
#203933=CARTESIAN_POINT('Ctrl Pts',(0.855262041130861,-6.71492671366791,
81.8434577727));
#203934=CARTESIAN_POINT('Ctrl Pts',(1.02482047121684,-6.68894849746766,
81.8515024962805));
#203935=CARTESIAN_POINT('Ctrl Pts',(1.19427706038546,-6.66298588441595,
81.8595423880044));
#203936=CARTESIAN_POINT('Ctrl Pts',(1.36286786030057,-6.6305608985558,81.8675822797283));
#203937=CARTESIAN_POINT('Ctrl Pts',(1.53005533614705,-6.59175391442429,
81.8756221714522));
#203938=CARTESIAN_POINT('Ctrl Pts',(1.70084281640561,-6.55211130960179,
81.8838351840725));
#203939=CARTESIAN_POINT('Ctrl Pts',(1.87016545477484,-6.50580877506365,
81.8920481966927));
#203940=CARTESIAN_POINT('Ctrl Pts',(2.03746021251925,-6.45298728360757,
81.900261209313));
#203941=CARTESIAN_POINT('Ctrl Pts',(2.20117144835849,-6.40129725003008,
81.908298295855));
#203942=CARTESIAN_POINT('Ctrl Pts',(2.36294043284138,-6.34336483738883,
81.9163353823971));
#203943=CARTESIAN_POINT('Ctrl Pts',(2.5222544486576,-6.27937269926121,81.9243724689392));
#203944=CARTESIAN_POINT('Ctrl Pts',(2.6815837115667,-6.21537443678809,81.9324103246678));
#203945=CARTESIAN_POINT('Ctrl Pts',(2.83845719122023,-6.14531543321051,
81.9404481803965));
#203946=CARTESIAN_POINT('Ctrl Pts',(2.99238209066652,-6.06942653167977,
81.9484860361251));
#203947=CARTESIAN_POINT('Ctrl Pts',(3.1463522191037,-5.99351533110288,81.9565262536816));
#203948=CARTESIAN_POINT('Ctrl Pts',(3.29737170786323,-5.91177098794107,
81.964566471238));
#203949=CARTESIAN_POINT('Ctrl Pts',(3.44497244406968,-5.82447026429019,
81.9726066887945));
#203950=CARTESIAN_POINT('Ctrl Pts',(3.59814963068672,-5.73387126334909,
81.9809506709231));
#203951=CARTESIAN_POINT('Ctrl Pts',(3.74764431061086,-5.63728806054833,
81.9892946530517));
#203952=CARTESIAN_POINT('Ctrl Pts',(3.8929673046525,-5.5350785509247,81.9976386351804));
#203953=CARTESIAN_POINT('Ctrl Pts',(4.0332435655986,-5.43641854231636,82.0056928500149));
#203954=CARTESIAN_POINT('Ctrl Pts',(4.16963277697767,-5.33251672891265,
82.0137470648495));
#203955=CARTESIAN_POINT('Ctrl Pts',(4.30173007168806,-5.22373500383917,
82.021801279684));
#203956=CARTESIAN_POINT('Ctrl Pts',(4.43392621937963,-5.11487187363287,
82.0298615217665));
#203957=CARTESIAN_POINT('Ctrl Pts',(4.56182377806979,-5.00112180711831,
82.037921763849));
#203958=CARTESIAN_POINT('Ctrl Pts',(4.6850554580905,-4.88288279140677,82.0459820059314));
#203959=CARTESIAN_POINT('Ctrl Pts',(4.80845942445318,-4.76447846944046,
82.0540535167853));
#203960=CARTESIAN_POINT('Ctrl Pts',(4.92718424009014,-4.6415729430195,82.0621250276391));
#203961=CARTESIAN_POINT('Ctrl Pts',(5.04090313915448,-4.51459683046698,
82.0701965384929));
#203962=CARTESIAN_POINT('Ctrl Pts',(5.05282206715812,-4.50128840806624,
82.0710425171081));
#203963=CARTESIAN_POINT('Ctrl Pts',(5.06468604374235,-4.48793529482951,
82.0718884957232));
#203964=CARTESIAN_POINT('Ctrl Pts',(5.07649472081613,-4.47453800403192,
82.0727344743383));
#203965=CARTESIAN_POINT('Ctrl Pts',(5.19136352595938,-4.34421597249018,
82.080963724075));
#203966=CARTESIAN_POINT('Ctrl Pts',(5.30137952524032,-4.20927629108711,
82.0891929738116));
#203967=CARTESIAN_POINT('Ctrl Pts',(5.40614979156494,-4.07011467051757,
82.0974222235483));
#203968=CARTESIAN_POINT('Ctrl Pts',(5.51079536422877,-3.93111867491511,
82.105641679139));
#203969=CARTESIAN_POINT('Ctrl Pts',(5.61020742200935,-3.78791102924984,
82.1138611347297));
#203970=CARTESIAN_POINT('Ctrl Pts',(5.70403084721884,-3.64092311014335,
82.1220805903205));
#203971=CARTESIAN_POINT('Ctrl Pts',(5.79776144934126,-3.49408061178211,
82.1302919140908));
#203972=CARTESIAN_POINT('Ctrl Pts',(5.88591423820863,-3.34346558824972,
82.1385032378611));
#203973=CARTESIAN_POINT('Ctrl Pts',(5.96817521452784,-3.18954128499626,
82.1467145616315));
#203974=CARTESIAN_POINT('Ctrl Pts',(6.05037132098683,-3.03573836430453,
82.1549194100662));
#203975=CARTESIAN_POINT('Ctrl Pts',(6.12668470074347,-2.87863167657969,
82.163124258501));
#203976=CARTESIAN_POINT('Ctrl Pts',(6.19684539157228,-2.7187122306249,82.1713291069358));
#203977=CARTESIAN_POINT('Ctrl Pts',(6.26696483592478,-2.55888679904712,
82.1795291318564));
#203978=CARTESIAN_POINT('Ctrl Pts',(6.33093865322651,-2.39625223088614,
82.187729156777));
#203979=CARTESIAN_POINT('Ctrl Pts',(6.38854341812386,-2.23132292480185,
82.1959291816976));
#203980=CARTESIAN_POINT('Ctrl Pts',(6.44613151089718,-2.06644135299531,
82.2041268333452));
#203981=CARTESIAN_POINT('Ctrl Pts',(6.49735410112811,-1.8992667030229,82.2123244849928));
#203982=CARTESIAN_POINT('Ctrl Pts',(6.54203630798522,-1.73033232212865,
82.2205221366405));
#203983=CARTESIAN_POINT('Ctrl Pts',(6.58671253162069,-1.56142056258448,
82.2287186905722));
#203984=CARTESIAN_POINT('Ctrl Pts',(6.6248500236285,-1.39074988791779,82.236915244504));
#203985=CARTESIAN_POINT('Ctrl Pts',(6.65632409129223,-1.21886774987393,
82.2451117984358));
#203986=CARTESIAN_POINT('Ctrl Pts',(6.68779966718853,-1.04697737526393,
82.2533087451452));
#203987=CARTESIAN_POINT('Ctrl Pts',(6.71261111791783,-0.873875774517605,
82.2615056918546));
#203988=CARTESIAN_POINT('Ctrl Pts',(6.73068507658497,-0.700119561101074,
82.269702638564));
#203989=CARTESIAN_POINT('Ctrl Pts',(6.74876318766153,-0.526323427988551,
82.2779014684844));
#203990=CARTESIAN_POINT('Ctrl Pts',(6.76010068660101,-0.351872739416242,
82.2861002984048));
#203991=CARTESIAN_POINT('Ctrl Pts',(6.76467617079343,-0.177328238866729,
82.2942991283253));
#203992=CARTESIAN_POINT('Ctrl Pts',(6.7692559885543,-0.00261842236166177,
82.3025057235858));
#203993=CARTESIAN_POINT('Ctrl Pts',(6.7670609865657,0.172185024544171,82.3107123188463));
#203994=CARTESIAN_POINT('Ctrl Pts',(6.75812192251174,0.346521399723311,
82.3189189141068));
#203995=CARTESIAN_POINT('Ctrl Pts',(6.74917853189954,0.520942154707554,
82.3271294814065));
#203996=CARTESIAN_POINT('Ctrl Pts',(6.73348460347278,0.694895030160229,
82.3353400487061));
#203997=CARTESIAN_POINT('Ctrl Pts',(6.71112269830597,0.867825517187885,
82.3435506160058));
#203998=CARTESIAN_POINT('Ctrl Pts',(6.68872995287063,1.04099450011368,82.3517725068532));
#203999=CARTESIAN_POINT('Ctrl Pts',(6.6596509120071,1.21313792285201,82.3599943977005));
#204000=CARTESIAN_POINT('Ctrl Pts',(6.62401932489763,1.38371130781775,82.3682162885479));
#204001=CARTESIAN_POINT('Ctrl Pts',(6.59162180316011,1.53880277007267,82.3756919276945));
#204002=CARTESIAN_POINT('Ctrl Pts',(6.55380790922888,1.69259623300692,82.3831675668412));
#204003=CARTESIAN_POINT('Ctrl Pts',(6.51071347235611,1.84469484763215,82.3906432059878));
#204004=CARTESIAN_POINT('Ctrl Pts',(6.45920089351945,2.02650466916343,82.3995791494376));
#204005=CARTESIAN_POINT('Ctrl Pts',(6.40003585945146,2.20627140930722,82.4085150928874));
#204006=CARTESIAN_POINT('Ctrl Pts',(6.33339242783275,2.3833651325533,82.4174510363371));
#204007=CARTESIAN_POINT('Ctrl Pts',(6.26684917896782,2.56019263696217,82.4263735466938));
#204008=CARTESIAN_POINT('Ctrl Pts',(6.19285005496423,2.73435490116357,82.4352960570504));
#204009=CARTESIAN_POINT('Ctrl Pts',(6.11161861126517,2.90523784748119,82.4442185674071));
#204010=CARTESIAN_POINT('Ctrl Pts',(6.03058620981137,3.07570207755101,82.4531192148445));
#204011=CARTESIAN_POINT('Ctrl Pts',(5.94235696813749,3.24290279408672,82.4620198622819));
#204012=CARTESIAN_POINT('Ctrl Pts',(5.84720185082691,3.40624713074174,82.4709205097193));
#204013=CARTESIAN_POINT('Ctrl Pts',(5.7521937840059,3.56933903888475,82.4798074023046));
#204014=CARTESIAN_POINT('Ctrl Pts',(5.65028132072025,3.72858623291068,82.4886942948899));
#204015=CARTESIAN_POINT('Ctrl Pts',(5.54178187019136,3.88341894510731,82.4975811874752));
#204016=CARTESIAN_POINT('Ctrl Pts',(5.43356130375142,4.03785367943704,82.5064452374293));
#204017=CARTESIAN_POINT('Ctrl Pts',(5.31878768247145,4.18789636300229,82.5153092873833));
#204018=CARTESIAN_POINT('Ctrl Pts',(5.19782193069723,4.33300544388799,82.5241733373373));
#204019=CARTESIAN_POINT('Ctrl Pts',(5.0821689409042,4.4717413985231,82.5326480821624));
#204020=CARTESIAN_POINT('Ctrl Pts',(4.96085617335053,4.6059675719914,82.5411228269875));
#204021=CARTESIAN_POINT('Ctrl Pts',(4.83423698792294,4.73523407495319,82.5495975718126));
#204022=CARTESIAN_POINT('Ctrl Pts',(4.70777943043633,4.86433557070347,82.5580614987229));
#204023=CARTESIAN_POINT('Ctrl Pts',(4.57615374704214,4.98836079582789,82.5665254256332));
#204024=CARTESIAN_POINT('Ctrl Pts',(4.4398150550172,5.10689056836375,82.5749893525435));
#204025=CARTESIAN_POINT('Ctrl Pts',(4.3075405445235,5.22188703347757,82.583200974441));
#204026=CARTESIAN_POINT('Ctrl Pts',(4.17083028506245,5.33171077287963,82.5914125963386));
#204027=CARTESIAN_POINT('Ctrl Pts',(4.03013340544854,5.43602002703152,82.5996242182362));
#204028=CARTESIAN_POINT('Ctrl Pts',(3.88295208309319,5.54513668976138,82.6082142976528));
#204029=CARTESIAN_POINT('Ctrl Pts',(3.73140830947619,5.64821825406331,82.6168043770695));
#204030=CARTESIAN_POINT('Ctrl Pts',(3.5760496501881,5.74492453382894,82.6253944564862));
#204031=CARTESIAN_POINT('Ctrl Pts',(3.42069099090001,5.84163081359456,82.6339845359029));
#204032=CARTESIAN_POINT('Ctrl Pts',(3.26151784721451,5.93196161725502,82.6425746153196));
#204033=CARTESIAN_POINT('Ctrl Pts',(3.09910619832129,6.01563211736943,82.6511646947363));
#204034=CARTESIAN_POINT('Origin',(0.,0.,4.30282021618968));
#204035=CARTESIAN_POINT('',(3.09910619832135,6.0156321173694,85.0458695769521));
#204036=CARTESIAN_POINT('',(3.09910619832134,6.0156321173694,84.651395695404));
#204037=CARTESIAN_POINT('',(3.09910619832133,6.0156321173694,4.30282021618968));
#204038=CARTESIAN_POINT('',(-6.76699823995479,0.00488061971302377,83.6971797838462));
#204039=CARTESIAN_POINT('Ctrl Pts',(-6.76699823995479,0.00488061971293362,
83.6971797838461));
#204040=CARTESIAN_POINT('Ctrl Pts',(-6.76712107896984,-0.165436153062113,
83.7052188399697));
#204041=CARTESIAN_POINT('Ctrl Pts',(-6.76080980226119,-0.336005823343854,
83.7132578960933));
#204042=CARTESIAN_POINT('Ctrl Pts',(-6.74803370927081,-0.50629048830176,
83.7212969522169));
#204043=CARTESIAN_POINT('Ctrl Pts',(-6.73526962568816,-0.67641508726984,
83.729328451703));
#204044=CARTESIAN_POINT('Ctrl Pts',(-6.71605284687801,-0.846254842235936,
83.7373599511891));
#204045=CARTESIAN_POINT('Ctrl Pts',(-6.69040469136798,-1.01527043969643,
83.7453914506752));
#204046=CARTESIAN_POINT('Ctrl Pts',(-6.6647749659965,-1.18416458667371,
83.7534171789218));
#204047=CARTESIAN_POINT('Ctrl Pts',(-6.63272311857364,-1.35223538512838,
83.7614429071684));
#204048=CARTESIAN_POINT('Ctrl Pts',(-6.59432239577663,-1.51894737912768,
83.7694686354151));
#204049=CARTESIAN_POINT('Ctrl Pts',(-6.55593841162304,-1.6855867043744,
83.7774908652951));
#204050=CARTESIAN_POINT('Ctrl Pts',(-6.51121114226346,-1.85086803825692,
83.7855130951752));
#204051=CARTESIAN_POINT('Ctrl Pts',(-6.46026515247052,-2.01426491797257,
83.7935353250553));
#204052=CARTESIAN_POINT('Ctrl Pts',(-6.40933009653302,-2.17762673000443,
83.8015558332316));
#204053=CARTESIAN_POINT('Ctrl Pts',(-6.35217908691007,-2.33910453390513,
83.8095763414079));
#204054=CARTESIAN_POINT('Ctrl Pts',(-6.28898685641384,-2.49818600585585,
83.8175968495842));
#204055=CARTESIAN_POINT('Ctrl Pts',(-6.22579554048134,-2.6572651754643,
83.8256172416819));
#204056=CARTESIAN_POINT('Ctrl Pts',(-6.15656331650125,-2.81394773292535,
83.8336376337797));
#204057=CARTESIAN_POINT('Ctrl Pts',(-6.08151339503498,-2.96774052538462,
83.8416580258774));
#204058=CARTESIAN_POINT('Ctrl Pts',(-6.00644953686954,-3.12156187701944,
83.8496799073543));
#204059=CARTESIAN_POINT('Ctrl Pts',(-5.92556599674474,-3.2724920584335,
83.8577017888312));
#204060=CARTESIAN_POINT('Ctrl Pts',(-5.83913225538147,-3.42006191525296,
83.8657236703081));
#204061=CARTESIAN_POINT('Ctrl Pts',(-5.75262086069104,-3.56776435097263,
83.8737527587597));
#204062=CARTESIAN_POINT('Ctrl Pts',(-5.6605494967974,-3.71210010851727,
83.8817818472114));
#204063=CARTESIAN_POINT('Ctrl Pts',(-5.56323170656305,-3.85262793156718,
83.889810935663));
#204064=CARTESIAN_POINT('Ctrl Pts',(-5.46586746257829,-3.99322283427849,
83.897843856726));
#204065=CARTESIAN_POINT('Ctrl Pts',(-5.36325202968282,-4.13000588231652,
83.905876777789));
#204066=CARTESIAN_POINT('Ctrl Pts',(-5.25573932231426,-4.26256884705451,
83.913909698852));
#204067=CARTESIAN_POINT('Ctrl Pts',(-5.14808399478493,-4.39530766218087,
83.9219532759251));
#204068=CARTESIAN_POINT('Ctrl Pts',(-5.03551866539925,-4.52381493162073,
83.9299968529981));
#204069=CARTESIAN_POINT('Ctrl Pts',(-4.9184347670821,-4.64771862766649,
83.9380404300712));
#204070=CARTESIAN_POINT('Ctrl Pts',(-4.83364399579953,-4.7374482156242,
83.9438654932413));
#204071=CARTESIAN_POINT('Ctrl Pts',(-4.74648423770331,-4.82476424712684,
83.9496905564114));
#204072=CARTESIAN_POINT('Ctrl Pts',(-4.65711466349154,-4.90953887968026,
83.9555156195815));
#204073=CARTESIAN_POINT('Ctrl Pts',(-4.52001718694038,-5.0395874818039,
83.9644515630322));
#204074=CARTESIAN_POINT('Ctrl Pts',(-4.37738205023,-5.1639731719019,83.9733875064829));
#204075=CARTESIAN_POINT('Ctrl Pts',(-4.22968046560856,-5.28224309918139,
83.9823234499336));
#204076=CARTESIAN_POINT('Ctrl Pts',(-4.08220091564451,-5.40033523539078,
83.9912459602912));
#204077=CARTESIAN_POINT('Ctrl Pts',(-3.92967031582237,-5.51232979217855,
84.0001684706487));
#204078=CARTESIAN_POINT('Ctrl Pts',(-3.77259434826907,-5.61781282025383,
84.0090909810063));
#204079=CARTESIAN_POINT('Ctrl Pts',(-3.615903265581,-5.72303738217621,84.0179916284446));
#204080=CARTESIAN_POINT('Ctrl Pts',(-3.45468925772409,-5.82178211557599,
84.0268922758829));
#204081=CARTESIAN_POINT('Ctrl Pts',(-3.28948794808252,-5.91367551015609,
84.0357929233213));
#204082=CARTESIAN_POINT('Ctrl Pts',(-3.12454193667582,-6.00542689483636,
84.0446798159075));
#204083=CARTESIAN_POINT('Ctrl Pts',(-2.95562113934356,-6.09034793589034,
84.0535667084936));
#204084=CARTESIAN_POINT('Ctrl Pts',(-2.78328932799944,-6.16811069263875,
84.0624536010799));
#204085=CARTESIAN_POINT('Ctrl Pts',(-2.61140047374007,-6.24567357007432,
84.0713176510347));
#204086=CARTESIAN_POINT('Ctrl Pts',(-2.43611833521379,-6.31611477217599,
84.0801817009897));
#204087=CARTESIAN_POINT('Ctrl Pts',(-2.25802970177353,-6.37915283293233,
84.0890457509446));
#204088=CARTESIAN_POINT('Ctrl Pts',(-2.08776264196135,-6.43942229007791,
84.0975204957651));
#204089=CARTESIAN_POINT('Ctrl Pts',(-1.91493053823632,-6.49292478630404,
84.1059952405857));
#204090=CARTESIAN_POINT('Ctrl Pts',(-1.74006688801186,-6.5394538170435,
84.1144699854062));
#204091=CARTESIAN_POINT('Ctrl Pts',(-1.57068824926195,-6.58452335481699,
84.1226788998353));
#204092=CARTESIAN_POINT('Ctrl Pts',(-1.39956653595643,-6.62300566039124,
84.1308878142645));
#204093=CARTESIAN_POINT('Ctrl Pts',(-1.22725383853958,-6.65478301793453,
84.1390967286936));
#204094=CARTESIAN_POINT('Ctrl Pts',(-1.05490017465371,-6.68656793038326,
84.1473075947505));
#204095=CARTESIAN_POINT('Ctrl Pts',(-0.881355312725267,-6.71164465439116,
84.1555184608073));
#204096=CARTESIAN_POINT('Ctrl Pts',(-0.707179597201149,-6.72994695501402,
84.1637293268642));
#204097=CARTESIAN_POINT('Ctrl Pts',(-0.532931424732736,-6.74825686937782,
84.1719436086341));
#204098=CARTESIAN_POINT('Ctrl Pts',(-0.358052229684333,-6.75978670881848,
84.180157890404));
#204099=CARTESIAN_POINT('Ctrl Pts',(-0.183105602099797,-6.76452225500661,
84.1883721721739));
#204100=CARTESIAN_POINT('Ctrl Pts',(-0.00796205827666974,-6.76926313142577,
84.1965956997663));
#204101=CARTESIAN_POINT('Ctrl Pts',(0.167248713592808,-6.76719443034825,
84.2048192273588));
#204102=CARTESIAN_POINT('Ctrl Pts',(0.341964019730027,-6.75835406065782,
84.2130427549512));
#204103=CARTESIAN_POINT('Ctrl Pts',(0.516791311582013,-6.74950802463431,
84.2212715535049));
#204104=CARTESIAN_POINT('Ctrl Pts',(0.691122150898044,-6.73388169943994,
84.2295003520586));
#204105=CARTESIAN_POINT('Ctrl Pts',(0.864400883076171,-6.71156465463435,
84.2377291506124));
#204106=CARTESIAN_POINT('Ctrl Pts',(1.03791811956269,-6.68921689220249,
84.2459692754488));
#204107=CARTESIAN_POINT('Ctrl Pts',(1.21038000627911,-6.66016007453195,
84.2542094002852));
#204108=CARTESIAN_POINT('Ctrl Pts',(1.38124196449292,-6.62453467313167,
84.2624495251216));
#204109=CARTESIAN_POINT('Ctrl Pts',(1.45709762272291,-6.60871846511687,
84.2661078004914));
#204110=CARTESIAN_POINT('Ctrl Pts',(1.53263814352889,-6.59160825051821,
84.2697660758612));
#204111=CARTESIAN_POINT('Ctrl Pts',(1.60781698502866,-6.57321941993825,
84.2734243512309));
#204112=CARTESIAN_POINT('Ctrl Pts',(1.78142681481329,-6.53075425709142,
84.2818723739935));
#204113=CARTESIAN_POINT('Ctrl Pts',(1.95350399173718,-6.48137002673282,
84.290320396756));
#204114=CARTESIAN_POINT('Ctrl Pts',(2.12347658587396,-6.42519542031564,
84.2987684195186));
#204115=CARTESIAN_POINT('Ctrl Pts',(2.29329353102955,-6.36907225466338,
84.3072087061743));
#204116=CARTESIAN_POINT('Ctrl Pts',(2.4610094197909,-6.30617121171915,84.3156489928301));
#204117=CARTESIAN_POINT('Ctrl Pts',(2.62606542132665,-6.23667133997876,
84.3240892794859));
#204118=CARTESIAN_POINT('Ctrl Pts',(2.79099568559647,-6.16722441223177,
84.3325231364538));
#204119=CARTESIAN_POINT('Ctrl Pts',(2.95326979570846,-6.09118880578558,
84.3409569934217));
#204120=CARTESIAN_POINT('Ctrl Pts',(3.11234654466722,-6.00879255640416,
84.3493908503896));
#204121=CARTESIAN_POINT('Ctrl Pts',(3.27132656670402,-5.92644640822003,
84.3578195791346));
#204122=CARTESIAN_POINT('Ctrl Pts',(3.42711280831388,-5.83774748107507,
84.3662483078796));
#204123=CARTESIAN_POINT('Ctrl Pts',(3.57918606578331,-5.74297101738313,
84.3746770366247));
#204124=CARTESIAN_POINT('Ctrl Pts',(3.73119020762479,-5.64823762855466,
84.3831019346049));
#204125=CARTESIAN_POINT('Ctrl Pts',(3.87948444766638,-5.54743238707693,
84.3915268325852));
#204126=CARTESIAN_POINT('Ctrl Pts',(4.02357578236501,-5.44087556589616,
84.3999517305654));
#204127=CARTESIAN_POINT('Ctrl Pts',(4.16763521500838,-5.33434233656845,
84.4083747632596));
#204128=CARTESIAN_POINT('Ctrl Pts',(4.30749332813591,-5.22206026246067,
84.4167977959537));
#204129=CARTESIAN_POINT('Ctrl Pts',(4.44268718767619,-5.10439218246971,
84.4252208286479));
#204130=CARTESIAN_POINT('Ctrl Pts',(4.57786575018514,-4.98673741648807,
84.4336429082855));
#204131=CARTESIAN_POINT('Ctrl Pts',(4.70838085972113,-4.86369807842071,
84.4420649879231));
#204132=CARTESIAN_POINT('Ctrl Pts',(4.83380345490516,-4.73567663162795,
84.4504870675607));
#204133=CARTESIAN_POINT('Ctrl Pts',(4.95922936672243,-4.60765179947876,
84.458909369909));
#204134=CARTESIAN_POINT('Ctrl Pts',(5.07956226260474,-4.47464483441219,
84.4673316722572));
#204135=CARTESIAN_POINT('Ctrl Pts',(5.19441042327864,-4.33709457523516,
84.4757539746055));
#204136=CARTESIAN_POINT('Ctrl Pts',(5.30927765383616,-4.19952147662023,
84.4841776754291));
#204137=CARTESIAN_POINT('Ctrl Pts',(5.41865812026474,-4.05740383619905,
84.4926013762528));
#204138=CARTESIAN_POINT('Ctrl Pts',(5.52220059741159,-3.9112133107192,84.5010250770764));
#204139=CARTESIAN_POINT('Ctrl Pts',(5.62581314269915,-3.76492385677452,
84.5094544782954));
#204140=CARTESIAN_POINT('Ctrl Pts',(5.72357961147391,-3.61455628270737,
84.5178838795144));
#204141=CARTESIAN_POINT('Ctrl Pts',(5.81519174534528,-3.4606117905463,84.5263132807334));
#204142=CARTESIAN_POINT('Ctrl Pts',(5.90683656629883,-3.30661237120416,
84.534745689551));
#204143=CARTESIAN_POINT('Ctrl Pts',(5.99232250868261,-3.14903377870128,
84.5431780983686));
#204144=CARTESIAN_POINT('Ctrl Pts',(6.07138718921519,-2.98840201422662,
84.5516105071863));
#204145=CARTESIAN_POINT('Ctrl Pts',(6.15052502269068,-2.82762162856968,
84.5600507179139));
#204146=CARTESIAN_POINT('Ctrl Pts',(6.22322958216186,-2.6637827288813,84.5684909286415));
#204147=CARTESIAN_POINT('Ctrl Pts',(6.28928611455797,-2.49743251545028,
84.5769311393692));
#204148=CARTESIAN_POINT('Ctrl Pts',(6.32685794298873,-2.4028153526696,84.5817317872063));
#204149=CARTESIAN_POINT('Ctrl Pts',(6.36227993459848,-2.30738607939501,
84.5865324350435));
#204150=CARTESIAN_POINT('Ctrl Pts',(6.39551975129777,-2.21124763668844,
84.5913330828807));
#204151=CARTESIAN_POINT('Ctrl Pts',(6.45187936042859,-2.04824056891767,
84.5994727979135));
#204152=CARTESIAN_POINT('Ctrl Pts',(6.50207497499668,-1.88286885991759,
84.6076125129464));
#204153=CARTESIAN_POINT('Ctrl Pts',(6.54590366792075,-1.71564395207796,
84.6157522279793));
#204154=CARTESIAN_POINT('Ctrl Pts',(6.58969402853302,-1.54856529813915,
84.6238848240663));
#204155=CARTESIAN_POINT('Ctrl Pts',(6.62712845929958,-1.37963702336426,
84.6320174201532));
#204156=CARTESIAN_POINT('Ctrl Pts',(6.65805292930488,-1.20938835391066,
84.6401500162402));
#204157=CARTESIAN_POINT('Ctrl Pts',(6.68895625768357,-1.0392560755803,84.6482770524482));
#204158=CARTESIAN_POINT('Ctrl Pts',(6.71335842095531,-0.867805558621238,
84.6564040886562));
#204159=CARTESIAN_POINT('Ctrl Pts',(6.7311558454839,-0.695578883957801,
84.6645311248642));
#204160=CARTESIAN_POINT('Ctrl Pts',(6.74894476252135,-0.52343453676293,
84.6726542762018));
#204161=CARTESIAN_POINT('Ctrl Pts',(6.76013519024366,-0.350515134175944,
84.6807774275394));
#204162=CARTESIAN_POINT('Ctrl Pts',(6.76467506093265,-0.177370572519474,
84.6889005788769));
#204163=CARTESIAN_POINT('Ctrl Pts',(6.76921365588425,-0.00427466577078583,
84.6970214475487));
#204164=CARTESIAN_POINT('Ctrl Pts',(6.76710540739535,0.169045908238103,
84.7051423162204));
#204165=CARTESIAN_POINT('Ctrl Pts',(6.75835028798784,0.34203857217374,84.7132631848921));
#204166=CARTESIAN_POINT('Ctrl Pts',(6.74959469542019,0.515040585294734,
84.7213844924466));
#204167=CARTESIAN_POINT('Ctrl Pts',(6.73419152881631,0.687714286980306,
84.7295058000011));
#204168=CARTESIAN_POINT('Ctrl Pts',(6.7121928362885,0.859509353339107,84.7376271075556));
#204169=CARTESIAN_POINT('Ctrl Pts',(6.70076155093691,0.948780041724772,
84.7418472212722));
#204170=CARTESIAN_POINT('Ctrl Pts',(6.68755019439306,1.03781355316633,84.7460673349888));
#204171=CARTESIAN_POINT('Ctrl Pts',(6.67257157733132,1.12653341956206,84.7502874487054));
#204172=CARTESIAN_POINT('Ctrl Pts',(6.64068275318351,1.31541415576423,84.7592718872312));
#204173=CARTESIAN_POINT('Ctrl Pts',(6.60079688724046,1.50277917244423,84.7682563257569));
#204174=CARTESIAN_POINT('Ctrl Pts',(6.55309139297731,1.68798169281742,84.7772407642827));
#204175=CARTESIAN_POINT('Ctrl Pts',(6.50530356187837,1.8735038616869,84.7862407094131));
#204176=CARTESIAN_POINT('Ctrl Pts',(6.44966918678762,2.05685584286998,84.7952406545436));
#204177=CARTESIAN_POINT('Ctrl Pts',(6.38641536804921,2.23740647776504,84.804240599674));
#204178=CARTESIAN_POINT('Ctrl Pts',(6.32301249006314,2.41838258486618,84.8132617534062));
#204179=CARTESIAN_POINT('Ctrl Pts',(6.25195432189093,2.5965439108255,84.8222829071383));
#204180=CARTESIAN_POINT('Ctrl Pts',(6.17351698119904,2.77127715734951,84.8313040608705));
#204181=CARTESIAN_POINT('Ctrl Pts',(6.09499982989494,2.94618819632867,84.8403343936977));
#204182=CARTESIAN_POINT('Ctrl Pts',(6.0090886094478,3.11766397215953,84.8493647265248));
#204183=CARTESIAN_POINT('Ctrl Pts',(5.91610595291568,3.285114815935,84.858395059352));
#204184=CARTESIAN_POINT('Ctrl Pts',(5.82299147628616,3.45280305222386,84.8674381943446));
#204185=CARTESIAN_POINT('Ctrl Pts',(5.72278563427439,3.61645473798033,84.8764813293372));
#204186=CARTESIAN_POINT('Ctrl Pts',(5.61585624227032,3.77550627944829,84.8855244643298));
#204187=CARTESIAN_POINT('Ctrl Pts',(5.52237531856668,3.91455397002478,84.8934302477299));
#204188=CARTESIAN_POINT('Ctrl Pts',(5.42375645092302,4.05008622305118,84.90133603113));
#204189=CARTESIAN_POINT('Ctrl Pts',(5.32027149338863,4.18174607510264,84.9092418145301));
#204190=CARTESIAN_POINT('Ctrl Pts',(5.20699117754997,4.32586817728066,84.9178959190671));
#204191=CARTESIAN_POINT('Ctrl Pts',(5.08777886983725,4.46547663036308,84.9265500236042));
#204192=CARTESIAN_POINT('Ctrl Pts',(4.9630126903714,4.6000863073656,84.9352041281412));
#204193=CARTESIAN_POINT('Ctrl Pts',(4.83836199103351,4.73457139337084,84.9438502226782));
#204194=CARTESIAN_POINT('Ctrl Pts',(4.70816787888502,4.86406670915905,84.9524963172153));
#204195=CARTESIAN_POINT('Ctrl Pts',(4.57284837415254,4.98812056259775,84.9611424117523));
#204196=CARTESIAN_POINT('Ctrl Pts',(4.43768172844762,5.11203428286467,84.9697787395258));
#204197=CARTESIAN_POINT('Ctrl Pts',(4.29740146827764,5.23051860308039,84.9784150672993));
#204198=CARTESIAN_POINT('Ctrl Pts',(4.1524621651814,5.34315889401925,84.9870513950728));
#204199=CARTESIAN_POINT('Ctrl Pts',(4.00762643038123,5.45571869634839,84.995681551644));
#204200=CARTESIAN_POINT('Ctrl Pts',(3.85813853101576,5.56244261091302,85.0043117082153));
#204201=CARTESIAN_POINT('Ctrl Pts',(3.70448679699984,5.6629556391388,85.0129418647865));
#204202=CARTESIAN_POINT('Ctrl Pts',(3.55096226977574,5.76338545359587,85.0215648765342));
#204203=CARTESIAN_POINT('Ctrl Pts',(3.39328104032662,5.85761447586562,85.0301878882819));
#204204=CARTESIAN_POINT('Ctrl Pts',(3.23196143974569,5.94531027382062,85.0388109000296));
#204205=CARTESIAN_POINT('Ctrl Pts',(3.18794344947024,5.96923912541509,85.0411637923371));
#204206=CARTESIAN_POINT('Ctrl Pts',(3.14365473671839,5.99268180246005,85.0435166846446));
#204207=CARTESIAN_POINT('Ctrl Pts',(3.09910619832135,6.0156321173694,85.0458695769521));
#204208=CARTESIAN_POINT('Ctrl Pts',(3.09910619832137,6.01563211736938,83.0458350405685));
#204209=CARTESIAN_POINT('Ctrl Pts',(2.94222343601837,6.09645427064887,83.0541399300722));
#204210=CARTESIAN_POINT('Ctrl Pts',(2.78207422307906,6.17118846651213,83.0624448195759));
#204211=CARTESIAN_POINT('Ctrl Pts',(2.6191668397426,6.23957162516729,83.0707497090796));
#204212=CARTESIAN_POINT('Ctrl Pts',(2.45634445559085,6.30791910396183,83.0790502653921));
#204213=CARTESIAN_POINT('Ctrl Pts',(2.29076708901272,6.36992201488416,83.0873508217047));
#204214=CARTESIAN_POINT('Ctrl Pts',(2.12296520258661,6.42536440589998,83.0956513780172));
#204215=CARTESIAN_POINT('Ctrl Pts',(1.95522012516891,6.48078802700013,83.1039491241922));
#204216=CARTESIAN_POINT('Ctrl Pts',(1.78525235890356,6.52965544612152,83.1122468703673));
#204217=CARTESIAN_POINT('Ctrl Pts',(1.61361002882069,6.5717997287569,83.1205446165423));
#204218=CARTESIAN_POINT('Ctrl Pts',(1.44195933667373,6.61394606457574,83.1288427669666));
#204219=CARTESIAN_POINT('Ctrl Pts',(1.26863425343041,6.64936851793706,83.1371409173909));
#204220=CARTESIAN_POINT('Ctrl Pts',(1.09419623148279,6.67795055439982,83.1454390678152));
#204221=CARTESIAN_POINT('Ctrl Pts',(0.919747450146447,6.70653435381104,
83.1537377300718));
#204222=CARTESIAN_POINT('Ctrl Pts',(0.744185936702099,6.72827683829004,
83.1620363923285));
#204223=CARTESIAN_POINT('Ctrl Pts',(0.568081393202253,6.7431129703348,83.1703350545852));
#204224=CARTESIAN_POINT('Ctrl Pts',(0.391936721418534,6.7579524830335,83.178635607827));
#204225=CARTESIAN_POINT('Ctrl Pts',(0.215249119809965,6.76588247737562,
83.1869361610688));
#204226=CARTESIAN_POINT('Ctrl Pts',(0.0385916370279971,6.76688995666041,
83.1952367143106));
#204227=CARTESIAN_POINT('Ctrl Pts',(-0.138135460949674,6.76789783296132,
83.2035405385411));
#204228=CARTESIAN_POINT('Ctrl Pts',(-0.31483206857426,6.76197775539134,
83.2118443627717));
#204229=CARTESIAN_POINT('Ctrl Pts',(-0.490926723087211,6.74916883420165,
83.2201481870023));
#204230=CARTESIAN_POINT('Ctrl Pts',(-0.667228372344878,6.736344856454,83.228461772165));
#204231=CARTESIAN_POINT('Ctrl Pts',(-0.842926306957382,6.71661587932008,
83.2367753573277));
#204232=CARTESIAN_POINT('Ctrl Pts',(-1.01745452551502,6.69007289112077,
83.2450889424904));
#204233=CARTESIAN_POINT('Ctrl Pts',(-1.19208697913823,6.66351405041269,
83.2534074928507));
#204234=CARTESIAN_POINT('Ctrl Pts',(-1.36554798195602,6.63013314811858,
83.2617260432111));
#204235=CARTESIAN_POINT('Ctrl Pts',(-1.53728312963927,6.59007204659604,
83.2700445935714));
#204236=CARTESIAN_POINT('Ctrl Pts',(-1.70928687689542,6.54994828815728,
83.2783761544255));
#204237=CARTESIAN_POINT('Ctrl Pts',(-1.87955903735623,6.50312353745619,
83.2867077152797));
#204238=CARTESIAN_POINT('Ctrl Pts',(-2.04756025847315,6.4497896080354,83.2950392761338));
#204239=CARTESIAN_POINT('Ctrl Pts',(-2.21330439089012,6.39717221751008,
83.30325890285));
#204240=CARTESIAN_POINT('Ctrl Pts',(-2.37683794933173,6.33821963469623,
83.3114785295662));
#204241=CARTESIAN_POINT('Ctrl Pts',(-2.53766439000712,6.27316096108571,
83.3196981562824));
#204242=CARTESIAN_POINT('Ctrl Pts',(-2.69556019893281,6.2092878078018,83.3277680022852));
#204243=CARTESIAN_POINT('Ctrl Pts',(-2.8513344453291,6.13933136950248,83.3358378482879));
#204244=CARTESIAN_POINT('Ctrl Pts',(-3.00447155353015,6.06345113644269,
83.3439076942907));
#204245=CARTESIAN_POINT('Ctrl Pts',(-3.15741599577087,5.98766637036764,
83.3519673874007));
#204246=CARTESIAN_POINT('Ctrl Pts',(-3.30772957139011,5.90597280226232,
83.3600270805108));
#204247=CARTESIAN_POINT('Ctrl Pts',(-3.45491318585497,5.81857919755377,
83.3680867736208));
#204248=CARTESIAN_POINT('Ctrl Pts',(-3.60194392675879,5.73127636498458,
83.3761380954595));
#204249=CARTESIAN_POINT('Ctrl Pts',(-3.74585085788079,5.63828546631741,
83.3841894172981));
#204250=CARTESIAN_POINT('Ctrl Pts',(-3.8861562566868,5.53986268319117,83.3922407391367));
#204251=CARTESIAN_POINT('Ctrl Pts',(-4.02634667174486,5.44152055997241,
83.4002854627177));
#204252=CARTESIAN_POINT('Ctrl Pts',(-4.16294112513135,5.33775562550626,
83.4083301862988));
#204253=CARTESIAN_POINT('Ctrl Pts',(-4.29548794327362,5.22886912526896,
83.4163749098798));
#204254=CARTESIAN_POINT('Ctrl Pts',(-4.42795515057297,5.12004802491216,
83.4244148016042));
#204255=CARTESIAN_POINT('Ctrl Pts',(-4.55637927464699,5.0061117186563,83.4324546933286));
#204256=CARTESIAN_POINT('Ctrl Pts',(-4.68033910352281,4.88740369480927,
83.4404945850529));
#204257=CARTESIAN_POINT('Ctrl Pts',(-4.80696812712494,4.76613956198648,
83.4487075976729));
#204258=CARTESIAN_POINT('Ctrl Pts',(-4.92893809121434,4.63989611294284,
83.4569206102929));
#204259=CARTESIAN_POINT('Ctrl Pts',(-5.0458367834887,4.5090819635922,83.4651336229128));
#204260=CARTESIAN_POINT('Ctrl Pts',(-5.16023145813442,4.38106990663177,
83.4731707094554));
#204261=CARTESIAN_POINT('Ctrl Pts',(-5.26976966830451,4.24868127686682,
83.481207795998));
#204262=CARTESIAN_POINT('Ctrl Pts',(-5.37410374915295,4.11233484693796,
83.4892448825405));
#204263=CARTESIAN_POINT('Ctrl Pts',(-5.47844781525869,3.97597536802094,
83.4972827382697));
#204264=CARTESIAN_POINT('Ctrl Pts',(-5.57758653316142,3.83565763137752,
83.5053205939988));
#204265=CARTESIAN_POINT('Ctrl Pts',(-5.67121396523096,3.69183168096399,
83.513358449728));
#204266=CARTESIAN_POINT('Ctrl Pts',(-5.76486890860173,3.54796346901492,
83.521398667285));
#204267=CARTESIAN_POINT('Ctrl Pts',(-5.85300913900852,3.40058530437991,
83.5294388848419));
#204268=CARTESIAN_POINT('Ctrl Pts',(-5.93537338346487,3.25017411823687,
83.5374791023989));
#204269=CARTESIAN_POINT('Ctrl Pts',(-6.02084940184901,3.09408030111023,
83.5458230845266));
#204270=CARTESIAN_POINT('Ctrl Pts',(-6.10010425481225,2.93472019737296,
83.5541670666544));
#204271=CARTESIAN_POINT('Ctrl Pts',(-6.17289996649483,2.77265125893036,
83.5625110487821));
#204272=CARTESIAN_POINT('Ctrl Pts',(-6.24316765067548,2.61621060166151,
83.5705652636172));
#204273=CARTESIAN_POINT('Ctrl Pts',(-6.30741721867655,2.45724646474984,
83.5786194784523));
#204274=CARTESIAN_POINT('Ctrl Pts',(-6.36548523708809,2.2962767029288,83.5866736932873));
#204275=CARTESIAN_POINT('Ctrl Pts',(-6.4235967098092,2.13518648185925,83.5947339353703));
#204276=CARTESIAN_POINT('Ctrl Pts',(-6.47551730969434,1.97208800099019,
83.6027941774533));
#204277=CARTESIAN_POINT('Ctrl Pts',(-6.52113434031348,1.80751097246582,
83.6108544195363));
#204278=CARTESIAN_POINT('Ctrl Pts',(-6.5668151466706,1.64270385396613,83.6189259303907));
#204279=CARTESIAN_POINT('Ctrl Pts',(-6.60617471542386,1.47641442368363,
83.626997441245));
#204280=CARTESIAN_POINT('Ctrl Pts',(-6.6391518532878,1.30917976954475,83.6350689520994));
#204281=CARTESIAN_POINT('Ctrl Pts',(-6.64260820164493,1.29165183172083,
83.6359149307103));
#204282=CARTESIAN_POINT('Ctrl Pts',(-6.64599448470253,1.27411351203699,
83.6367609093211));
#204283=CARTESIAN_POINT('Ctrl Pts',(-6.64931066511964,1.25656542954444,
83.637606887932));
#204284=CARTESIAN_POINT('Ctrl Pts',(-6.70553663204556,0.959037013795542,
83.6519504879214));
#204285=CARTESIAN_POINT('Ctrl Pts',(-6.74178309739482,0.657773115918566,
83.6662940879108));
#204286=CARTESIAN_POINT('Ctrl Pts',(-6.75768976121672,0.354849392202926,
83.6806376879002));
#204287=CARTESIAN_POINT('Ctrl Pts',(-6.76380467329694,0.238398076058037,
83.6861517198701));
#204288=CARTESIAN_POINT('Ctrl Pts',(-6.76691398399781,0.12170181386997,
83.6916657518401));
#204289=CARTESIAN_POINT('Ctrl Pts',(-6.76699823995424,0.0048806204788414,
83.69717978381));
#204290=CARTESIAN_POINT('',(-6.767,3.23694968940892E-12,83.3028202161898));
#204291=CARTESIAN_POINT('Ctrl Pts',(3.09910619832129,6.01563211736943,82.6511646947363));
#204292=CARTESIAN_POINT('Ctrl Pts',(2.94351145532274,6.09579071467805,82.6593942226567));
#204293=CARTESIAN_POINT('Ctrl Pts',(2.78494486261122,6.1698366203801,82.6676237505772));
#204294=CARTESIAN_POINT('Ctrl Pts',(2.62393210008548,6.23756918471779,82.6758532784977));
#204295=CARTESIAN_POINT('Ctrl Pts',(2.46270285731928,6.30539281489142,82.6840938709459));
#204296=CARTESIAN_POINT('Ctrl Pts',(2.29902120868915,6.36688602715692,82.6923344633941));
#204297=CARTESIAN_POINT('Ctrl Pts',(2.13342861867361,6.42189779808309,82.7005750558424));
#204298=CARTESIAN_POINT('Ctrl Pts',(2.07999748796384,6.43964823681139,82.7032340164407));
#204299=CARTESIAN_POINT('Ctrl Pts',(2.0263674867545,6.45672426696228,82.7058929770391));
#204300=CARTESIAN_POINT('Ctrl Pts',(1.97255701528041,6.47312195323617,82.7085519376374));
#204301=CARTESIAN_POINT('Ctrl Pts',(1.80159092869621,6.52522051648016,82.7169999604));
#204302=CARTESIAN_POINT('Ctrl Pts',(1.62841111951404,6.57058692165375,82.7254479831626));
#204303=CARTESIAN_POINT('Ctrl Pts',(1.45357508981669,6.60903990442367,82.7338960059252));
#204304=CARTESIAN_POINT('Ctrl Pts',(1.27889916269323,6.64745767464886,82.742336292581));
#204305=CARTESIAN_POINT('Ctrl Pts',(1.10257036235085,6.67897457038737,82.7507765792369));
#204306=CARTESIAN_POINT('Ctrl Pts',(0.925160630309959,6.70345931651148,
82.7592168658927));
#204307=CARTESIAN_POINT('Ctrl Pts',(0.747886046428055,6.72792541051135,
82.7676507228607));
#204308=CARTESIAN_POINT('Ctrl Pts',(0.5695325015942,6.74536998863663,82.7760845798287));
#204309=CARTESIAN_POINT('Ctrl Pts',(0.39068178667714,6.75571289662007,82.7845184367967));
#204310=CARTESIAN_POINT('Ctrl Pts',(0.21193982227986,6.7660495155785,82.7929471655418));
#204311=CARTESIAN_POINT('Ctrl Pts',(0.0327016226476002,6.76929305449129,
82.8013758942868));
#204312=CARTESIAN_POINT('Ctrl Pts',(-0.146445846855666,6.76541518415084,
82.8098046230319));
#204313=CARTESIAN_POINT('Ctrl Pts',(-0.325511895799725,6.76153907625991,
82.8182295210123));
#204314=CARTESIAN_POINT('Ctrl Pts',(-0.504486963965482,6.75054802012883,
82.8266544189926));
#204315=CARTESIAN_POINT('Ctrl Pts',(-0.682783631235683,6.73246578252847,
82.835079316973));
#204316=CARTESIAN_POINT('Ctrl Pts',(-0.861040823333554,6.71438754836494,
82.8435023496672));
#204317=CARTESIAN_POINT('Ctrl Pts',(-1.03861958224152,6.68922129399911,
82.8519253823615));
#204318=CARTESIAN_POINT('Ctrl Pts',(-1.2149366183719,6.6570427378333,82.8603484150557));
#204319=CARTESIAN_POINT('Ctrl Pts',(-1.39123370443,6.62486782263455,82.8687704946934));
#204320=CARTESIAN_POINT('Ctrl Pts',(-1.56626902432563,6.58568224724365,
82.877192574331));
#204321=CARTESIAN_POINT('Ctrl Pts',(-1.73946819088527,6.53961309351695,
82.8856146539687));
#204322=CARTESIAN_POINT('Ctrl Pts',(-1.91267193746574,6.49354272155296,
82.894036956317));
#204323=CARTESIAN_POINT('Ctrl Pts',(-2.08403911173682,6.44058849442824,
82.9024592586653));
#204324=CARTESIAN_POINT('Ctrl Pts',(-2.25300887074723,6.38092783444025,
82.9108815610136));
#204325=CARTESIAN_POINT('Ctrl Pts',(-2.42200668622488,6.32125726813906,
82.9193052618373));
#204326=CARTESIAN_POINT('Ctrl Pts',(-2.58860597858924,6.25487816043816,
82.927728962661));
#204327=CARTESIAN_POINT('Ctrl Pts',(-2.75226397544351,6.18201682377813,
82.9361526634848));
#204328=CARTESIAN_POINT('Ctrl Pts',(-2.91603272116038,6.10910618118551,
82.9445820647038));
#204329=CARTESIAN_POINT('Ctrl Pts',(-3.07685588910995,6.0297046799482,82.9530114659229));
#204330=CARTESIAN_POINT('Ctrl Pts',(-3.23421257418138,5.94408597052626,
82.9614408671419));
#204331=CARTESIAN_POINT('Ctrl Pts',(-3.39162540389929,5.85843671246782,
82.9698732759596));
#204332=CARTESIAN_POINT('Ctrl Pts',(-3.5455689945942,5.76656598783355,82.9783056847773));
#204333=CARTESIAN_POINT('Ctrl Pts',(-3.69554923193981,5.6687921883157,82.986738093595));
#204334=CARTESIAN_POINT('Ctrl Pts',(-3.84566823536477,5.57092792563375,
82.9951783043227));
#204335=CARTESIAN_POINT('Ctrl Pts',(-3.99181628267492,5.46714986298643,
83.0036185150504));
#204336=CARTESIAN_POINT('Ctrl Pts',(-4.1335293971468,5.35781893338355,83.0120587257781));
#204337=CARTESIAN_POINT('Ctrl Pts',(-4.21413339843345,5.29563336627339,
83.0168593736144));
#204338=CARTESIAN_POINT('Ctrl Pts',(-4.29330323395663,5.23165211256194,
83.0216600214506));
#204339=CARTESIAN_POINT('Ctrl Pts',(-4.37095855156853,5.16594718715455,
83.0264606692868));
#204340=CARTESIAN_POINT('Ctrl Pts',(-4.50262664672873,5.05454152123131,
83.0346003843194));
#204341=CARTESIAN_POINT('Ctrl Pts',(-4.63020117296965,4.93795617861826,
83.0427400993521));
#204342=CARTESIAN_POINT('Ctrl Pts',(-4.75324657479831,4.81652737967596,
83.0508798143848));
#204343=CARTESIAN_POINT('Ctrl Pts',(-4.87618436185678,4.69520478163266,
83.0590124104715));
#204344=CARTESIAN_POINT('Ctrl Pts',(-4.99460065026711,4.5690474145762,83.0671450065582));
#204345=CARTESIAN_POINT('Ctrl Pts',(-5.10809285403984,4.4384317494479,83.0752776026449));
#204346=CARTESIAN_POINT('Ctrl Pts',(-5.22150746845331,4.3079053801957,83.0834046388527));
#204347=CARTESIAN_POINT('Ctrl Pts',(-5.33000446128772,4.17292705644808,
83.0915316750604));
#204348=CARTESIAN_POINT('Ctrl Pts',(-5.43321807438887,4.03391005801246,
83.0996587112681));
#204349=CARTESIAN_POINT('Ctrl Pts',(-5.53638234951505,3.89495951221795,
83.1077818626055));
#204350=CARTESIAN_POINT('Ctrl Pts',(-5.63426805627028,3.75197442951678,
83.1159050139428));
#204351=CARTESIAN_POINT('Ctrl Pts',(-5.72654973831429,3.60540110037878,
83.1240281652802));
#204352=CARTESIAN_POINT('Ctrl Pts',(-5.81880548851989,3.45886895943548,
83.1321490339516));
#204353=CARTESIAN_POINT('Ctrl Pts',(-5.9054601563769,3.30875089049244,83.1402699026231));
#204354=CARTESIAN_POINT('Ctrl Pts',(-5.98623166756643,3.15552205224822,
83.1483907712945));
#204355=CARTESIAN_POINT('Ctrl Pts',(-6.06700754395764,3.002284932931,83.1565120788488));
#204356=CARTESIAN_POINT('Ctrl Pts',(-6.1418994541896,2.84593703056162,83.1646333864031));
#204357=CARTESIAN_POINT('Ctrl Pts',(-6.21067125504395,2.68697814687258,
83.1727546939574));
#204358=CARTESIAN_POINT('Ctrl Pts',(-6.24640747341314,2.6043775851792,83.1769748076754));
#204359=CARTESIAN_POINT('Ctrl Pts',(-6.28049190995254,2.52107237950219,
83.1811949213935));
#204360=CARTESIAN_POINT('Ctrl Pts',(-6.31289654940185,2.43713482527131,
83.1854150351116));
#204361=CARTESIAN_POINT('Ctrl Pts',(-6.38012902587568,2.26298292184015,
83.1941708398695));
#204362=CARTESIAN_POINT('Ctrl Pts',(-6.44010519243268,2.08616622098546,
83.2029266446274));
#204363=CARTESIAN_POINT('Ctrl Pts',(-6.49265040050596,1.90729645750466,
83.2116824493853));
#204364=CARTESIAN_POINT('Ctrl Pts',(-6.54529416165284,1.72809120834186,
83.2204546764108));
#204365=CARTESIAN_POINT('Ctrl Pts',(-6.59047901362006,1.54682546602365,
83.2292269034364));
#204366=CARTESIAN_POINT('Ctrl Pts',(-6.6280807354594,1.36412417478471,83.2379991304619));
#204367=CARTESIAN_POINT('Ctrl Pts',(-6.66571845078739,1.18124799642541,
83.2467797545246));
#204368=CARTESIAN_POINT('Ctrl Pts',(-6.69575849200273,0.996933801297433,
83.2555603785872));
#204369=CARTESIAN_POINT('Ctrl Pts',(-6.71812825172542,0.81181389084494,
83.2643410026499));
#204370=CARTESIAN_POINT('Ctrl Pts',(-6.74053178465382,0.626414491792852,
83.2731348834407));
#204371=CARTESIAN_POINT('Ctrl Pts',(-6.75524185616454,0.440207224918582,
83.2819287642314));
#204372=CARTESIAN_POINT('Ctrl Pts',(-6.76223779849073,0.253828597016198,
83.2907226450222));
#204373=CARTESIAN_POINT('Ctrl Pts',(-6.76541320615378,0.169232684746745,
83.2947141239609));
#204374=CARTESIAN_POINT('Ctrl Pts',(-6.76700007130205,0.0846014611602841,
83.2987056028995));
#204375=CARTESIAN_POINT('Ctrl Pts',(-6.7669999999976,-5.7030305532282E-6,
83.3026970818381));
#204376=CARTESIAN_POINT('Ctrl Pts',(-6.767,3.23694969632991E-12,83.3028202161898));
#204377=CARTESIAN_POINT('Ctrl Pts',(-6.76700000000009,-0.186007249523727,
83.311569728001));
#204378=CARTESIAN_POINT('Ctrl Pts',(-6.75932637294537,-0.372014355746867,
83.3203192398122));
#204379=CARTESIAN_POINT('Ctrl Pts',(-6.74400518264205,-0.55738953748454,
83.3290687516234));
#204380=CARTESIAN_POINT('Ctrl Pts',(-6.72868405705117,-0.742763936248949,
83.337818226479));
#204381=CARTESIAN_POINT('Ctrl Pts',(-6.70571545645763,-0.927506130239531,
83.3465677013347));
#204382=CARTESIAN_POINT('Ctrl Pts',(-6.67517739404845,-1.11098863989898,
83.3553171761904));
#204383=CARTESIAN_POINT('Ctrl Pts',(-6.64463945808724,-1.29447038981831,
83.3640666148174));
#204384=CARTESIAN_POINT('Ctrl Pts',(-6.6065321700838,-1.47669218313569,
83.3728160534444));
#204385=CARTESIAN_POINT('Ctrl Pts',(-6.56098496092705,-1.65703510599173,
83.3815654920714));
#204386=CARTESIAN_POINT('Ctrl Pts',(-6.51543793658328,-1.8373772970859,
83.3903148951966));
#204387=CARTESIAN_POINT('Ctrl Pts',(-6.46245112167454,-2.01584035510819,
83.3990642983218));
#204388=CARTESIAN_POINT('Ctrl Pts',(-6.40220448374289,-2.19181813760686,
83.4078137014469));
#204389=CARTESIAN_POINT('Ctrl Pts',(-6.34195808526534,-2.36779522067063,
83.416563069797));
#204390=CARTESIAN_POINT('Ctrl Pts',(-6.27445201433127,-2.5412867768411,
83.4253124381471));
#204391=CARTESIAN_POINT('Ctrl Pts',(-6.19991555071916,-2.71170355384779,
83.4340618064973));
#204392=CARTESIAN_POINT('Ctrl Pts',(-6.12537937716709,-2.88211966767442,
83.442811140799));
#204393=CARTESIAN_POINT('Ctrl Pts',(-6.04381298052539,-3.04946076371747,
83.4515604751008));
#204394=CARTESIAN_POINT('Ctrl Pts',(-5.95549339335854,-3.21315848374505,
83.4603098094026));
#204395=CARTESIAN_POINT('Ctrl Pts',(-5.86717414255433,-3.37685558033451,
83.4690591103828));
#204396=CARTESIAN_POINT('Ctrl Pts',(-5.77210188876624,-3.53690907646714,
83.477808411363));
#204397=CARTESIAN_POINT('Ctrl Pts',(-5.67059953347023,-3.69277536969245,
83.4865577123431));
#204398=CARTESIAN_POINT('Ctrl Pts',(-5.5690975563141,-3.84864108224885,
83.4953069807284));
#204399=CARTESIAN_POINT('Ctrl Pts',(-5.46116568196876,-4.00031938297482,
83.5040562491137));
#204400=CARTESIAN_POINT('Ctrl Pts',(-5.34717048533628,-4.14729511859822,
83.512805517499));
#204401=CARTESIAN_POINT('Ctrl Pts',(-5.23317570391869,-4.29427031887876,
83.521554754016));
#204402=CARTESIAN_POINT('Ctrl Pts',(-5.11311782003554,-4.436542761895,83.5303039905331));
#204403=CARTESIAN_POINT('Ctrl Pts',(-4.98740458984802,-4.57362924351799,
83.5390532270501));
#204404=CARTESIAN_POINT('Ctrl Pts',(-4.86169180711786,-4.71071523720223,
83.5478024324256));
#204405=CARTESIAN_POINT('Ctrl Pts',(-4.73032391204209,-4.84261509523202,
83.556551637801));
#204406=CARTESIAN_POINT('Ctrl Pts',(-4.59374707013629,-4.96888084538302,
83.5653008431765));
#204407=CARTESIAN_POINT('Ctrl Pts',(-4.45717070301487,-5.09514615659427,
83.5740500181369));
#204408=CARTESIAN_POINT('Ctrl Pts',(-4.31538563571095,-5.21577720459482,
83.5827991930973));
#204409=CARTESIAN_POINT('Ctrl Pts',(-4.16887341029576,-5.33036429232834,
83.5915483680577));
#204410=CARTESIAN_POINT('Ctrl Pts',(-4.02236168203758,-5.44495099123578,
83.6002975133298));
#204411=CARTESIAN_POINT('Ctrl Pts',(-3.87112305348201,-5.55349359438577,
83.6090466586018));
#204412=CARTESIAN_POINT('Ctrl Pts',(-3.7156711701778,-5.65562346298881,
83.6177958038739));
#204413=CARTESIAN_POINT('Ctrl Pts',(-3.56021980145802,-5.75775299351656,
83.626544920184));
#204414=CARTESIAN_POINT('Ctrl Pts',(-3.40055544538295,-5.85346967463906,
83.6352940364942));
#204415=CARTESIAN_POINT('Ctrl Pts',(-3.2372203598676,-5.94244842986952,
83.6440431528044));
#204416=CARTESIAN_POINT('Ctrl Pts',(-3.0738858014707,-6.03142689794585,
83.6527922408793));
#204417=CARTESIAN_POINT('Ctrl Pts',(-2.90688078896451,-6.11366734656842,
83.6615413289541));
#204418=CARTESIAN_POINT('Ctrl Pts',(-2.73677250721226,-6.18889046952417,
83.670290417029));
#204419=CARTESIAN_POINT('Ctrl Pts',(-2.56666476031311,-6.26411335596398,
83.679039477595));
#204420=CARTESIAN_POINT('Ctrl Pts',(-2.39345402574968,-6.33231884500632,
83.6877885381611));
#204421=CARTESIAN_POINT('Ctrl Pts',(-2.21772856065365,-6.39327529762806,
83.6965375987271));
#204422=CARTESIAN_POINT('Ctrl Pts',(-2.04200363348295,-6.4542315636518,
83.7052866325108));
#204423=CARTESIAN_POINT('Ctrl Pts',(-1.86376426189069,-6.50793874375718,
83.7140356662945));
#204424=CARTESIAN_POINT('Ctrl Pts',(-1.68361577752954,-6.55421443909593,
83.7227847000782));
#204425=CARTESIAN_POINT('Ctrl Pts',(-1.50346782967588,-6.60048999661917,
83.731533707806));
#204426=CARTESIAN_POINT('Ctrl Pts',(-1.32141105794765,-6.63933404237757,
83.7402827155339));
#204427=CARTESIAN_POINT('Ctrl Pts',(-1.1380637548679,-6.670614656076,83.7490317232617));
#204428=CARTESIAN_POINT('Ctrl Pts',(-0.954716982600968,-6.70189517921325,
83.7577807056601));
#204429=CARTESIAN_POINT('Ctrl Pts',(-0.770079968900371,-6.72561226592248,
83.7665296880584));
#204430=CARTESIAN_POINT('Ctrl Pts',(-0.584779765556764,-6.74168536983115,
83.7752786704568));
#204431=CARTESIAN_POINT('Ctrl Pts',(-0.391489830649839,-6.75845151013861,
83.7844048894667));
#204432=CARTESIAN_POINT('Ctrl Pts',(-0.1974785782369,-6.76689983031629,
83.7935311084766));
#204433=CARTESIAN_POINT('Ctrl Pts',(-0.00346287644993494,-6.76699911397118,
83.8026573274864));
#204434=CARTESIAN_POINT('Ctrl Pts',(0.184489834656155,-6.76709529501185,
83.8114983521522));
#204435=CARTESIAN_POINT('Ctrl Pts',(0.372446404251599,-6.75935639738156,
83.820339376818));
#204436=CARTESIAN_POINT('Ctrl Pts',(0.559755019490524,-6.74380925873168,
83.8291804014839));
#204437=CARTESIAN_POINT('Ctrl Pts',(0.745134705523977,-6.72842222659781,
83.8379303800936));
#204438=CARTESIAN_POINT('Ctrl Pts',(0.929879431230782,-6.70538706057493,
83.8466803587034));
#204439=CARTESIAN_POINT('Ctrl Pts',(1.11336163627048,-6.6747820089409,83.8554303373131));
#204440=CARTESIAN_POINT('Ctrl Pts',(1.29684196300956,-6.64417727060967,
83.8641802263496));
#204441=CARTESIAN_POINT('Ctrl Pts',(1.47905951217763,-6.60600284890534,
83.8729301153862));
#204442=CARTESIAN_POINT('Ctrl Pts',(1.65939532067351,-6.56038841607163,
83.8816800044227));
#204443=CARTESIAN_POINT('Ctrl Pts',(1.83972934301073,-6.5147744350318,83.8904298067949));
#204444=CARTESIAN_POINT('Ctrl Pts',(2.01818138406539,-6.46172066062056,
83.899179609167));
#204445=CARTESIAN_POINT('Ctrl Pts',(2.19414528354477,-6.40140730423383,
83.9079294115392));
#204446=CARTESIAN_POINT('Ctrl Pts',(2.37010749864279,-6.34109452518538,
83.9166791301555));
#204447=CARTESIAN_POINT('Ctrl Pts',(2.54358134866741,-6.2735223961639,83.9254288487718));
#204448=CARTESIAN_POINT('Ctrl Pts',(2.71397759435839,-6.19892043966695,
83.9341785673881));
#204449=CARTESIAN_POINT('Ctrl Pts',(2.88437226558397,-6.12431917249386,
83.9429282051568));
#204450=CARTESIAN_POINT('Ctrl Pts',(3.0516891268122,-6.04268832278665,83.9516778429255));
#204451=CARTESIAN_POINT('Ctrl Pts',(3.21535986274109,-5.95430516123197,
83.9604274806942));
#204452=CARTESIAN_POINT('Ctrl Pts',(3.37902914073103,-5.8659227869729,83.9691770405233));
#204453=CARTESIAN_POINT('Ctrl Pts',(3.53905210621839,-5.77078835741778,
83.9779266003524));
#204454=CARTESIAN_POINT('Ctrl Pts',(3.6948852283197,-5.66922500431451,83.9866761601815));
#204455=CARTESIAN_POINT('Ctrl Pts',(3.85071701407212,-5.56766252216905,
83.9954256449786));
#204456=CARTESIAN_POINT('Ctrl Pts',(4.00235878822675,-5.45967138329171,
84.0041751297757));
#204457=CARTESIAN_POINT('Ctrl Pts',(4.14929549611595,-5.34561838199398,
84.0129246145728));
#204458=CARTESIAN_POINT('Ctrl Pts',(4.29623099276359,-5.23156632086795,
84.0216740272454));
#204459=CARTESIAN_POINT('Ctrl Pts',(4.43846127436296,-5.11145267304732,
84.030423439918));
#204460=CARTESIAN_POINT('Ctrl Pts',(4.57550326054708,-4.98568540049641,
84.0391728525906));
#204461=CARTESIAN_POINT('Ctrl Pts',(4.71254416258032,-4.85991912290116,
84.0479221960458));
#204462=CARTESIAN_POINT('Ctrl Pts',(4.84439664018998,-4.72849950385176,
84.0566715395011));
#204463=CARTESIAN_POINT('Ctrl Pts',(4.97061286794968,-4.59187289860827,
84.0654208829563));
#204464=CARTESIAN_POINT('Ctrl Pts',(5.09682813912903,-4.45524732884435,
84.0741701601011));
#204465=CARTESIAN_POINT('Ctrl Pts',(5.21740705148052,-4.31341506235529,
84.082919437246));
#204466=CARTESIAN_POINT('Ctrl Pts',(5.33194007545904,-4.16685781275457,
84.0916687143908));
#204467=CARTESIAN_POINT('Ctrl Pts',(5.44647226944677,-4.02030162521581,
84.1004179281319));
#204468=CARTESIAN_POINT('Ctrl Pts',(5.55495848628289,-3.86902074887681,
84.1091671418731));
#204469=CARTESIAN_POINT('Ctrl Pts',(5.65703027291949,-3.71352898080418,
84.1179163556142));
#204470=CARTESIAN_POINT('Ctrl Pts',(5.7591013537715,-3.55803828789341,84.1266655088581));
#204471=CARTESIAN_POINT('Ctrl Pts',(5.85475793592897,-3.39833700106464,
84.1354146621019));
#204472=CARTESIAN_POINT('Ctrl Pts',(5.94367514427535,-3.23496750823304,
84.1441638153458));
#204473=CARTESIAN_POINT('Ctrl Pts',(6.03259176732768,-3.07159909077474,
84.1529129109987));
#204474=CARTESIAN_POINT('Ctrl Pts',(6.11476896836043,-2.90456276731183,
84.1616620066516));
#204475=CARTESIAN_POINT('Ctrl Pts',(6.18992765547997,-2.73442583002799,
84.1704111023046));
#204476=CARTESIAN_POINT('Ctrl Pts',(6.26508587283153,-2.56428995615927,
84.1791601432726));
#204477=CARTESIAN_POINT('Ctrl Pts',(6.33322554827248,-2.39105376934968,
84.1879091842406));
#204478=CARTESIAN_POINT('Ctrl Pts',(6.39411526733108,-2.21530561053855,
84.1966582252087));
#204479=CARTESIAN_POINT('Ctrl Pts',(6.45500462602914,-2.03955849184886,
84.2054072143977));
#204480=CARTESIAN_POINT('Ctrl Pts',(6.50864402040797,-1.86129970164345,
84.2141562035867));
#204481=CARTESIAN_POINT('Ctrl Pts',(6.55485128368649,-1.68113463135873,
84.2229051927757));
#204482=CARTESIAN_POINT('Ctrl Pts',(6.60199809554365,-1.49730620116697,
84.2318320782472));
#204483=CARTESIAN_POINT('Ctrl Pts',(6.64140720707904,-1.31149343245541,
84.2407589637186));
#204484=CARTESIAN_POINT('Ctrl Pts',(6.67293928722908,-1.12435326697383,
84.24968584919));
#204485=CARTESIAN_POINT('Ctrl Pts',(6.70384625876276,-0.940923067005181,
84.2584357633675));
#204486=CARTESIAN_POINT('Ctrl Pts',(6.72718554579811,-0.756217899520276,
84.2671856775449));
#204487=CARTESIAN_POINT('Ctrl Pts',(6.74287786815339,-0.57086518125313,
84.2759355917224));
#204488=CARTESIAN_POINT('Ctrl Pts',(6.75856988190853,-0.385516108072647,
84.2846853338269));
#204489=CARTESIAN_POINT('Ctrl Pts',(6.76661520773406,-0.199519795225118,
84.2934350759314));
#204490=CARTESIAN_POINT('Ctrl Pts',(6.76698651789579,-0.0135080204544889,
84.3021848180358));
#204491=CARTESIAN_POINT('Ctrl Pts',(6.767357821249,0.172500343514049,84.3109343997008));
#204492=CARTESIAN_POINT('Ctrl Pts',(6.76005538995178,0.358523882211937,
84.3196839813658));
#204493=CARTESIAN_POINT('Ctrl Pts',(6.74510402742353,0.54393074856532,84.3284335630308));
#204494=CARTESIAN_POINT('Ctrl Pts',(6.73015291918021,0.729334461616109,
84.3371829958874));
#204495=CARTESIAN_POINT('Ctrl Pts',(6.70755316306584,0.914121237635484,
84.3459324287441));
#204496=CARTESIAN_POINT('Ctrl Pts',(6.67738151874562,1.09766345166195,84.3546818616008));
#204497=CARTESIAN_POINT('Ctrl Pts',(6.64721034747555,1.28120278799737,84.3634311572783));
#204498=CARTESIAN_POINT('Ctrl Pts',(6.60946757205126,1.46349731860402,84.3721804529558));
#204499=CARTESIAN_POINT('Ctrl Pts',(6.56428138111505,1.64392790278234,84.3809297486334));
#204500=CARTESIAN_POINT('Ctrl Pts',(6.51909583859829,1.8243558977913,84.389678918759));
#204501=CARTESIAN_POINT('Ctrl Pts',(6.46646716392852,2.00291972192341,84.3984280888846));
#204502=CARTESIAN_POINT('Ctrl Pts',(6.40657409872857,2.1790129227474,84.4071772590102));
#204503=CARTESIAN_POINT('Ctrl Pts',(6.34668181342049,2.35510383059051,84.4159263152093));
#204504=CARTESIAN_POINT('Ctrl Pts',(6.27952541914021,2.52872390822651,84.4246753714084));
#204505=CARTESIAN_POINT('Ctrl Pts',(6.20533299175487,2.69928350890354,84.4334244276075));
#204506=CARTESIAN_POINT('Ctrl Pts',(6.12831602991515,2.87633637965694,84.4425065637657));
#204507=CARTESIAN_POINT('Ctrl Pts',(6.04371690605233,3.05009086601535,84.4515886999239));
#204508=CARTESIAN_POINT('Ctrl Pts',(5.9518452031659,3.2199111288281,84.460670836082));
#204509=CARTESIAN_POINT('Ctrl Pts',(5.8633354950923,3.38351691183094,84.4694206164256));
#204510=CARTESIAN_POINT('Ctrl Pts',(5.7680761809932,3.54347103712082,84.4781703967692));
#204511=CARTESIAN_POINT('Ctrl Pts',(5.66639083308964,3.69923018027775,84.4869201771128));
#204512=CARTESIAN_POINT('Ctrl Pts',(5.56470914082143,3.85498372382133,84.4956696428977));
#204513=CARTESIAN_POINT('Ctrl Pts',(5.45660203372004,4.00654234702084,84.5044191086826));
#204514=CARTESIAN_POINT('Ctrl Pts',(5.34243669839147,4.15339127986758,84.5131685744675));
#204515=CARTESIAN_POINT('Ctrl Pts',(5.22827486050518,4.30023571401369,84.5219177722135));
#204516=CARTESIAN_POINT('Ctrl Pts',(5.10805534167033,4.44237052028559,84.5306669699595));
#204517=CARTESIAN_POINT('Ctrl Pts',(4.98218644339869,4.5793129662881,84.5394161677056));
#204518=CARTESIAN_POINT('Ctrl Pts',(4.85632073219513,4.71625194483436,84.5481651439172));
#204519=CARTESIAN_POINT('Ctrl Pts',(4.72480612170254,4.84799861524571,84.5569141201288));
#204520=CARTESIAN_POINT('Ctrl Pts',(4.58808925235257,4.97410554898535,84.5656630963404));
#204521=CARTESIAN_POINT('Ctrl Pts',(4.45136349473991,5.10022068121257,84.5744126413421));
#204522=CARTESIAN_POINT('Ctrl Pts',(4.3094350121002,5.22069514871884,84.5831621863439));
#204523=CARTESIAN_POINT('Ctrl Pts',(4.16278587431718,5.33511975166306,84.5919117313456));
#204524=CARTESIAN_POINT('Ctrl Pts',(4.01614535740373,5.44953762807898,84.6006607619993));
#204525=CARTESIAN_POINT('Ctrl Pts',(3.86478496657836,5.55790617532845,84.609409792653));
#204526=CARTESIAN_POINT('Ctrl Pts',(3.70921874747096,5.65985735539421,84.6181588233068));
#204527=CARTESIAN_POINT('Ctrl Pts',(3.55365041605799,5.76180991977109,84.6269079727564));
#204528=CARTESIAN_POINT('Ctrl Pts',(3.39387638174418,5.85734478552874,84.635657122206));
#204529=CARTESIAN_POINT('Ctrl Pts',(3.23043927904432,5.9461374912129,84.6444062716556));
#204530=CARTESIAN_POINT('Ctrl Pts',(3.18691767070357,5.96978206944186,84.6467360795718));
#204531=CARTESIAN_POINT('Ctrl Pts',(3.14313645919591,5.99294880633446,84.6490658874879));
#204532=CARTESIAN_POINT('Ctrl Pts',(3.09910619832133,6.0156321173694,84.651395695404));
#204533=CARTESIAN_POINT('Origin',(0.,0.,4.30282021618968));
#204534=CARTESIAN_POINT('',(3.09910619832123,6.01563211736946,87.0457552630241));
#204535=CARTESIAN_POINT('',(3.09910619832139,6.01563211736938,86.6514537215909));
#204536=CARTESIAN_POINT('',(3.09910619832133,6.0156321173694,4.30282021618968));
#204537=CARTESIAN_POINT('',(-6.767,3.23394441651206E-12,85.6971797838099));
#204538=CARTESIAN_POINT('Ctrl Pts',(-6.767,3.23394454464685E-12,85.6971797838099));
#204539=CARTESIAN_POINT('Ctrl Pts',(-6.76700000000009,-0.186007249523693,
85.7059292956211));
#204540=CARTESIAN_POINT('Ctrl Pts',(-6.75932637294538,-0.372014355746796,
85.7146788074323));
#204541=CARTESIAN_POINT('Ctrl Pts',(-6.74400518264206,-0.557389537484432,
85.7234283192435));
#204542=CARTESIAN_POINT('Ctrl Pts',(-6.72868405705119,-0.742763936248805,
85.7321777940991));
#204543=CARTESIAN_POINT('Ctrl Pts',(-6.70571545645765,-0.927506130239353,
85.7409272689548));
#204544=CARTESIAN_POINT('Ctrl Pts',(-6.67517739404848,-1.11098863989877,
85.7496767438105));
#204545=CARTESIAN_POINT('Ctrl Pts',(-6.64463945808725,-1.29447038981831,
85.7584261824375));
#204546=CARTESIAN_POINT('Ctrl Pts',(-6.60653217008376,-1.47669218313591,
85.7671756210645));
#204547=CARTESIAN_POINT('Ctrl Pts',(-6.56098496092695,-1.65703510599216,
85.7759250596916));
#204548=CARTESIAN_POINT('Ctrl Pts',(-6.51543793658314,-1.83737729708641,
85.7846744628167));
#204549=CARTESIAN_POINT('Ctrl Pts',(-6.46245112167436,-2.01584035510878,
85.7934238659419));
#204550=CARTESIAN_POINT('Ctrl Pts',(-6.40220448374266,-2.19181813760754,
85.8021732690671));
#204551=CARTESIAN_POINT('Ctrl Pts',(-6.34195808526511,-2.36779522067127,
85.8109226374172));
#204552=CARTESIAN_POINT('Ctrl Pts',(-6.27445201433103,-2.54128677684169,
85.8196720057673));
#204553=CARTESIAN_POINT('Ctrl Pts',(-6.19991555071892,-2.71170355384834,
85.8284213741174));
#204554=CARTESIAN_POINT('Ctrl Pts',(-6.12537937716685,-2.88211966767492,
85.8371707084192));
#204555=CARTESIAN_POINT('Ctrl Pts',(-6.04381298052516,-3.04946076371794,
85.8459200427209));
#204556=CARTESIAN_POINT('Ctrl Pts',(-5.95549339335831,-3.21315848374548,
85.8546693770227));
#204557=CARTESIAN_POINT('Ctrl Pts',(-5.86717414255401,-3.37685558033507,
85.8634186780029));
#204558=CARTESIAN_POINT('Ctrl Pts',(-5.77210188876583,-3.53690907646783,
85.8721679789831));
#204559=CARTESIAN_POINT('Ctrl Pts',(-5.67059953346971,-3.69277536969325,
85.8809172799633));
#204560=CARTESIAN_POINT('Ctrl Pts',(-5.56909755631362,-3.84864108224955,
85.8896665483486));
#204561=CARTESIAN_POINT('Ctrl Pts',(-5.46116568196832,-4.00031938297542,
85.8984158167339));
#204562=CARTESIAN_POINT('Ctrl Pts',(-5.34717048533588,-4.14729511859873,
85.9071650851191));
#204563=CARTESIAN_POINT('Ctrl Pts',(-5.2331757039183,-4.29427031887923,
85.9159143216362));
#204564=CARTESIAN_POINT('Ctrl Pts',(-5.11311782003516,-4.43654276189544,
85.9246635581532));
#204565=CARTESIAN_POINT('Ctrl Pts',(-4.98740458984765,-4.57362924351839,
85.9334127946702));
#204566=CARTESIAN_POINT('Ctrl Pts',(-4.86169180711756,-4.71071523720254,
85.9421620000457));
#204567=CARTESIAN_POINT('Ctrl Pts',(-4.73032391204184,-4.84261509523225,
85.9509112054211));
#204568=CARTESIAN_POINT('Ctrl Pts',(-4.59374707013612,-4.96888084538318,
85.9596604107966));
#204569=CARTESIAN_POINT('Ctrl Pts',(-4.45717070301458,-5.09514615659453,
85.968409585757));
#204570=CARTESIAN_POINT('Ctrl Pts',(-4.31538563571053,-5.21577720459517,
85.9771587607174));
#204571=CARTESIAN_POINT('Ctrl Pts',(-4.16887341029521,-5.33036429232877,
85.9859079356779));
#204572=CARTESIAN_POINT('Ctrl Pts',(-4.02236168203715,-5.44495099123609,
85.9946570809499));
#204573=CARTESIAN_POINT('Ctrl Pts',(-3.87112305348171,-5.55349359438598,
86.0034062262219));
#204574=CARTESIAN_POINT('Ctrl Pts',(-3.71567117017763,-5.65562346298892,
86.012155371494));
#204575=CARTESIAN_POINT('Ctrl Pts',(-3.56021980145826,-5.7577529935164,
86.0209044878041));
#204576=CARTESIAN_POINT('Ctrl Pts',(-3.4005554453836,-5.85346967463866,
86.0296536041143));
#204577=CARTESIAN_POINT('Ctrl Pts',(-3.2372203598687,-5.94244842986892,
86.0384027204245));
#204578=CARTESIAN_POINT('Ctrl Pts',(-3.07388580147185,-6.03142689794527,
86.0471518084993));
#204579=CARTESIAN_POINT('Ctrl Pts',(-2.90688078896572,-6.11366734656785,
86.0559008965742));
#204580=CARTESIAN_POINT('Ctrl Pts',(-2.73677250721351,-6.18889046952362,
86.064649984649));
#204581=CARTESIAN_POINT('Ctrl Pts',(-2.56666476031465,-6.26411335596334,
86.073399045215));
#204582=CARTESIAN_POINT('Ctrl Pts',(-2.3934540257515,-6.33231884500562,
86.0821481057811));
#204583=CARTESIAN_POINT('Ctrl Pts',(-2.21772856065578,-6.39327529762732,
86.0908971663471));
#204584=CARTESIAN_POINT('Ctrl Pts',(-2.04200363348489,-6.45423156365119,
86.0996462001308));
#204585=CARTESIAN_POINT('Ctrl Pts',(-1.86376426189243,-6.50793874375669,
86.1083952339145));
#204586=CARTESIAN_POINT('Ctrl Pts',(-1.68361577753108,-6.55421443909554,
86.1171442676982));
#204587=CARTESIAN_POINT('Ctrl Pts',(-1.50346782967784,-6.60048999661871,
86.125893275426));
#204588=CARTESIAN_POINT('Ctrl Pts',(-1.32141105795003,-6.63933404237708,
86.1346422831538));
#204589=CARTESIAN_POINT('Ctrl Pts',(-1.13806375487071,-6.67061465607553,
86.1433912908816));
#204590=CARTESIAN_POINT('Ctrl Pts',(-0.954716982604021,-6.70189517921281,
86.15214027328));
#204591=CARTESIAN_POINT('Ctrl Pts',(-0.770079968903664,-6.72561226592209,
86.1608892556784));
#204592=CARTESIAN_POINT('Ctrl Pts',(-0.584779765560293,-6.74168536983085,
86.1696382380768));
#204593=CARTESIAN_POINT('Ctrl Pts',(-0.391489830653286,-6.75845151013842,
86.1787644570866));
#204594=CARTESIAN_POINT('Ctrl Pts',(-0.197478578240259,-6.7668998303162,
86.1878906760965));
#204595=CARTESIAN_POINT('Ctrl Pts',(-0.00346287645320154,-6.76699911397118,
86.1970168951064));
#204596=CARTESIAN_POINT('Ctrl Pts',(0.184489834652916,-6.76709529501194,
86.2058579197722));
#204597=CARTESIAN_POINT('Ctrl Pts',(0.372446404248391,-6.75935639738173,
86.214698944438));
#204598=CARTESIAN_POINT('Ctrl Pts',(0.559755019487351,-6.74380925873195,
86.2235399691038));
#204599=CARTESIAN_POINT('Ctrl Pts',(0.745134705520902,-6.72842222659816,
86.2322899477135));
#204600=CARTESIAN_POINT('Ctrl Pts',(0.929879431227806,-6.70538706057534,
86.2410399263233));
#204601=CARTESIAN_POINT('Ctrl Pts',(1.11336163626761,-6.67478200894138,
86.249789904933));
#204602=CARTESIAN_POINT('Ctrl Pts',(1.29684196300673,-6.64417727061022,
86.2585397939696));
#204603=CARTESIAN_POINT('Ctrl Pts',(1.47905951217484,-6.60600284890597,
86.2672896830061));
#204604=CARTESIAN_POINT('Ctrl Pts',(1.65939532067077,-6.56038841607233,
86.2760395720427));
#204605=CARTESIAN_POINT('Ctrl Pts',(1.83972934300797,-6.51477443503258,
86.2847893744148));
#204606=CARTESIAN_POINT('Ctrl Pts',(2.01818138406261,-6.46172066062142,
86.293539176787));
#204607=CARTESIAN_POINT('Ctrl Pts',(2.19414528354198,-6.40140730423479,
86.3022889791592));
#204608=CARTESIAN_POINT('Ctrl Pts',(2.37010749864,-6.34109452518642,86.3110386977755));
#204609=CARTESIAN_POINT('Ctrl Pts',(2.54358134866462,-6.27352239616503,
86.3197884163918));
#204610=CARTESIAN_POINT('Ctrl Pts',(2.71397759435559,-6.19892043966817,
86.3285381350081));
#204611=CARTESIAN_POINT('Ctrl Pts',(2.88437226558136,-6.1243191724951,86.3372877727768));
#204612=CARTESIAN_POINT('Ctrl Pts',(3.05168912680975,-6.04268832278789,
86.3460374105455));
#204613=CARTESIAN_POINT('Ctrl Pts',(3.21535986273881,-5.9543051612332,86.3547870483143));
#204614=CARTESIAN_POINT('Ctrl Pts',(3.37902914072875,-5.86592278697421,
86.3635366081433));
#204615=CARTESIAN_POINT('Ctrl Pts',(3.53905210621612,-5.77078835741917,
86.3722861679724));
#204616=CARTESIAN_POINT('Ctrl Pts',(3.69488522831744,-5.66922500431599,
86.3810357278015));
#204617=CARTESIAN_POINT('Ctrl Pts',(3.85071701406992,-5.56766252217057,
86.3897852125986));
#204618=CARTESIAN_POINT('Ctrl Pts',(4.00235878822462,-5.45967138329328,
86.3985346973957));
#204619=CARTESIAN_POINT('Ctrl Pts',(4.14929549611388,-5.34561838199558,
86.4072841821928));
#204620=CARTESIAN_POINT('Ctrl Pts',(4.29623099276148,-5.23156632086967,
86.4160335948654));
#204621=CARTESIAN_POINT('Ctrl Pts',(4.43846127436082,-5.11145267304917,
86.424783007538));
#204622=CARTESIAN_POINT('Ctrl Pts',(4.57550326054493,-4.98568540049838,
86.4335324202106));
#204623=CARTESIAN_POINT('Ctrl Pts',(4.71254416257829,-4.85991912290314,
86.4422817636658));
#204624=CARTESIAN_POINT('Ctrl Pts',(4.84439664018807,-4.72849950385372,
86.4510311071211));
#204625=CARTESIAN_POINT('Ctrl Pts',(4.97061286794788,-4.59187289861021,
86.4597804505763));
#204626=CARTESIAN_POINT('Ctrl Pts',(5.09682813912722,-4.45524732884642,
86.4685297277211));
#204627=CARTESIAN_POINT('Ctrl Pts',(5.2174070514787,-4.31341506235749,86.477279004866));
#204628=CARTESIAN_POINT('Ctrl Pts',(5.33194007545723,-4.1668578127569,86.4860282820108));
#204629=CARTESIAN_POINT('Ctrl Pts',(5.44647226944507,-4.02030162521812,
86.4947774957519));
#204630=CARTESIAN_POINT('Ctrl Pts',(5.55495848628131,-3.86902074887908,
86.503526709493));
#204631=CARTESIAN_POINT('Ctrl Pts',(5.65703027291801,-3.71352898080642,
86.5122759232341));
#204632=CARTESIAN_POINT('Ctrl Pts',(5.75910135377003,-3.55803828789578,
86.521025076478));
#204633=CARTESIAN_POINT('Ctrl Pts',(5.85475793592752,-3.39833700106713,
86.5297742297219));
#204634=CARTESIAN_POINT('Ctrl Pts',(5.94367514427392,-3.23496750823566,
86.5385233829658));
#204635=CARTESIAN_POINT('Ctrl Pts',(6.03259176732633,-3.07159909077738,
86.5472724786187));
#204636=CARTESIAN_POINT('Ctrl Pts',(6.11476896835918,-2.90456276731448,
86.5560215742716));
#204637=CARTESIAN_POINT('Ctrl Pts',(6.1899276554788,-2.73442583003065,86.5647706699245));
#204638=CARTESIAN_POINT('Ctrl Pts',(6.26508587283052,-2.56428995616176,
86.5735197108926));
#204639=CARTESIAN_POINT('Ctrl Pts',(6.33322554827161,-2.39105376935199,
86.5822687518606));
#204640=CARTESIAN_POINT('Ctrl Pts',(6.39411526733035,-2.21530561054067,
86.5910177928287));
#204641=CARTESIAN_POINT('Ctrl Pts',(6.45500462602845,-2.03955849185104,
86.5997667820177));
#204642=CARTESIAN_POINT('Ctrl Pts',(6.50864402040733,-1.86129970164568,
86.6085157712067));
#204643=CARTESIAN_POINT('Ctrl Pts',(6.5548512836859,-1.68113463136101,86.6172647603957));
#204644=CARTESIAN_POINT('Ctrl Pts',(6.60199809554315,-1.49730620116918,
86.6261916458672));
#204645=CARTESIAN_POINT('Ctrl Pts',(6.64140720707862,-1.31149343245754,
86.6351185313386));
#204646=CARTESIAN_POINT('Ctrl Pts',(6.67293928722873,-1.12435326697588,
86.64404541681));
#204647=CARTESIAN_POINT('Ctrl Pts',(6.70384625876248,-0.940923067007218,
86.6527953309875));
#204648=CARTESIAN_POINT('Ctrl Pts',(6.72718554579789,-0.756217899522293,
86.661545245165));
#204649=CARTESIAN_POINT('Ctrl Pts',(6.74287786815322,-0.570865181255125,
86.6702951593424));
#204650=CARTESIAN_POINT('Ctrl Pts',(6.75856988190842,-0.38551610807462,
86.6790449014469));
#204651=CARTESIAN_POINT('Ctrl Pts',(6.76661520773401,-0.199519795227065,
86.6877946435514));
#204652=CARTESIAN_POINT('Ctrl Pts',(6.76698651789579,-0.0135080204564092,
86.6965443856559));
#204653=CARTESIAN_POINT('Ctrl Pts',(6.76735782124905,0.172500343512155,
86.7052939673208));
#204654=CARTESIAN_POINT('Ctrl Pts',(6.76005538995188,0.358523882210071,
86.7140435489858));
#204655=CARTESIAN_POINT('Ctrl Pts',(6.74510402742368,0.543930748563485,
86.7227931306508));
#204656=CARTESIAN_POINT('Ctrl Pts',(6.7301529191804,0.729334461614369,86.7315425635075));
#204657=CARTESIAN_POINT('Ctrl Pts',(6.70755316306606,0.914121237633841,
86.7402919963641));
#204658=CARTESIAN_POINT('Ctrl Pts',(6.67738151874588,1.0976634516604,86.7490414292208));
#204659=CARTESIAN_POINT('Ctrl Pts',(6.64721034747584,1.28120278799586,86.7577907248984));
#204660=CARTESIAN_POINT('Ctrl Pts',(6.60946757205158,1.46349731860254,86.7665400205759));
#204661=CARTESIAN_POINT('Ctrl Pts',(6.56428138111541,1.6439279027809,86.7752893162534));
#204662=CARTESIAN_POINT('Ctrl Pts',(6.5190958385987,1.82435589778983,86.784038486379));
#204663=CARTESIAN_POINT('Ctrl Pts',(6.46646716392898,2.00291972192192,86.7927876565046));
#204664=CARTESIAN_POINT('Ctrl Pts',(6.40657409872909,2.17901292274589,86.8015368266302));
#204665=CARTESIAN_POINT('Ctrl Pts',(6.34668181342099,2.35510383058916,86.8102858828293));
#204666=CARTESIAN_POINT('Ctrl Pts',(6.2795254191407,2.52872390822532,86.8190349390284));
#204667=CARTESIAN_POINT('Ctrl Pts',(6.20533299175532,2.6992835089025,86.8277839952275));
#204668=CARTESIAN_POINT('Ctrl Pts',(6.1283160299156,2.876336379656,86.8368661313857));
#204669=CARTESIAN_POINT('Ctrl Pts',(6.04371690605276,3.05009086601451,86.845948267544));
#204670=CARTESIAN_POINT('Ctrl Pts',(5.95184520316631,3.21991112882734,86.8550304037022));
#204671=CARTESIAN_POINT('Ctrl Pts',(5.86333549509272,3.38351691183022,86.8637801840457));
#204672=CARTESIAN_POINT('Ctrl Pts',(5.76807618099362,3.54347103712014,86.8725299643893));
#204673=CARTESIAN_POINT('Ctrl Pts',(5.66639083309006,3.6992301802771,86.8812797447329));
#204674=CARTESIAN_POINT('Ctrl Pts',(5.56470914082193,3.85498372382061,86.8900292105178));
#204675=CARTESIAN_POINT('Ctrl Pts',(5.45660203372061,4.00654234702005,86.8987786763027));
#204676=CARTESIAN_POINT('Ctrl Pts',(5.34243669839213,4.15339127986673,86.9075281420876));
#204677=CARTESIAN_POINT('Ctrl Pts',(5.22827486050581,4.30023571401293,86.9162773398336));
#204678=CARTESIAN_POINT('Ctrl Pts',(5.10805534167092,4.44237052028491,86.9250265375796));
#204679=CARTESIAN_POINT('Ctrl Pts',(4.98218644339924,4.5793129662875,86.9337757353256));
#204680=CARTESIAN_POINT('Ctrl Pts',(4.85632073219563,4.71625194483385,86.9425247115373));
#204681=CARTESIAN_POINT('Ctrl Pts',(4.72480612170299,4.84799861524527,86.9512736877489));
#204682=CARTESIAN_POINT('Ctrl Pts',(4.58808925235296,4.97410554898499,86.9600226639605));
#204683=CARTESIAN_POINT('Ctrl Pts',(4.45136349474034,5.10022068121219,86.9687722089622));
#204684=CARTESIAN_POINT('Ctrl Pts',(4.30943501210067,5.22069514871845,86.9775217539639));
#204685=CARTESIAN_POINT('Ctrl Pts',(4.16278587431769,5.33511975166267,86.9862712989656));
#204686=CARTESIAN_POINT('Ctrl Pts',(4.01614535740428,5.44953762807857,86.9950203296194));
#204687=CARTESIAN_POINT('Ctrl Pts',(3.86478496657895,5.55790617532803,87.0037693602731));
#204688=CARTESIAN_POINT('Ctrl Pts',(3.7092187474716,5.6598573553938,87.0125183909269));
#204689=CARTESIAN_POINT('Ctrl Pts',(3.55365041605866,5.76180991977067,87.0212675403765));
#204690=CARTESIAN_POINT('Ctrl Pts',(3.3938763817449,5.85734478552832,87.0300166898261));
#204691=CARTESIAN_POINT('Ctrl Pts',(3.23043927904508,5.94613749121249,87.0387658392757));
#204692=CARTESIAN_POINT('Ctrl Pts',(3.18691767070404,5.96978206944161,87.0410956471919));
#204693=CARTESIAN_POINT('Ctrl Pts',(3.1431364591961,5.99294880633436,87.043425455108));
#204694=CARTESIAN_POINT('Ctrl Pts',(3.09910619832123,6.01563211736946,87.0457552630241));
#204695=CARTESIAN_POINT('Ctrl Pts',(3.09910619832135,6.0156321173694,85.0458695769521));
#204696=CARTESIAN_POINT('Ctrl Pts',(2.95819911900836,6.08822399040388,85.0533117780863));
#204697=CARTESIAN_POINT('Ctrl Pts',(2.81469155616859,6.15588807595813,85.0607539792206));
#204698=CARTESIAN_POINT('Ctrl Pts',(2.66893775428139,6.21844516449019,85.0681961803548));
#204699=CARTESIAN_POINT('Ctrl Pts',(2.50393692119552,6.28926302028242,85.076621136488));
#204700=CARTESIAN_POINT('Ctrl Pts',(2.33612920776672,6.35350388484595,85.0850460926212));
#204701=CARTESIAN_POINT('Ctrl Pts',(2.16606800253779,6.41096236210929,85.0934710487543));
#204702=CARTESIAN_POINT('Ctrl Pts',(1.99596732446964,6.46843417603711,85.1018979604007));
#204703=CARTESIAN_POINT('Ctrl Pts',(1.82361242586232,6.5191203576838,85.1103248720472));
#204704=CARTESIAN_POINT('Ctrl Pts',(1.64957246988648,6.56286520253103,85.1187517836936));
#204705=CARTESIAN_POINT('Ctrl Pts',(1.47546851264278,6.60662613406086,85.1271817942435));
#204706=CARTESIAN_POINT('Ctrl Pts',(1.29967858393249,6.64344055835283,85.1356118047934));
#204707=CARTESIAN_POINT('Ctrl Pts',(1.12278304682798,6.67320367063345,85.1440418153433));
#204708=CARTESIAN_POINT('Ctrl Pts',(0.945724557251994,6.70299420007101,
85.1524795914428));
#204709=CARTESIAN_POINT('Ctrl Pts',(0.767558751721852,6.72572038496047,
85.1609173675422));
#204710=CARTESIAN_POINT('Ctrl Pts',(0.58887326327967,6.74132904402347,85.1693551436416));
#204711=CARTESIAN_POINT('Ctrl Pts',(0.410093978127306,6.75694589648193,
85.1777973489516));
#204712=CARTESIAN_POINT('Ctrl Pts',(0.230794796639656,6.76543775071114,
85.1862395542615));
#204713=CARTESIAN_POINT('Ctrl Pts',(0.0515649678104242,6.76680353299065,
85.1946817595714));
#204714=CARTESIAN_POINT('Ctrl Pts',(-0.127853938626412,6.76817075609531,
85.2031328709434));
#204715=CARTESIAN_POINT('Ctrl Pts',(-0.307203014981049,6.76239689544306,
85.2115839823154));
#204716=CARTESIAN_POINT('Ctrl Pts',(-0.48589543792917,6.74953291890629,
85.2200350936874));
#204717=CARTESIAN_POINT('Ctrl Pts',(-0.536045743225493,6.74592262396484,
85.2224069111848));
#204718=CARTESIAN_POINT('Ctrl Pts',(-0.586144369622427,6.74175418650349,
85.2247787286822));
#204719=CARTESIAN_POINT('Ctrl Pts',(-0.636178460520079,6.73702946159287,
85.2271505461796));
#204720=CARTESIAN_POINT('Ctrl Pts',(-0.811612333427688,6.72046322096327,
85.2354668185837));
#204721=CARTESIAN_POINT('Ctrl Pts',(-0.986568801570855,6.69702410260573,
85.2437830909879));
#204722=CARTESIAN_POINT('Ctrl Pts',(-1.16047802969381,6.66675181348443,
85.252099363392));
#204723=CARTESIAN_POINT('Ctrl Pts',(-1.33424021735945,6.63650511961927,
85.260408604378));
#204724=CARTESIAN_POINT('Ctrl Pts',(-1.50695658807425,6.5994368251738,85.2687178453639));
#204725=CARTESIAN_POINT('Ctrl Pts',(-1.67806259715569,6.55563840674782,
85.2770270863499));
#204726=CARTESIAN_POINT('Ctrl Pts',(-1.84905530757672,6.51186898965361,
85.2853308253324));
#204727=CARTESIAN_POINT('Ctrl Pts',(-2.01843944515858,6.46137841441279,
85.2936345643148));
#204728=CARTESIAN_POINT('Ctrl Pts',(-2.18566060489128,6.40430923052801,
85.3019383032972));
#204729=CARTESIAN_POINT('Ctrl Pts',(-2.35280168409568,6.34726737650031,
85.3102380657028));
#204730=CARTESIAN_POINT('Ctrl Pts',(-2.51778152113153,6.2836533044426,85.3185378281083));
#204731=CARTESIAN_POINT('Ctrl Pts',(-2.68006061094702,6.21365947905502,
85.3268375905138));
#204732=CARTESIAN_POINT('Ctrl Pts',(-2.84229171696341,6.14368634992387,
85.3351348987884));
#204733=CARTESIAN_POINT('Ctrl Pts',(-3.00182334843409,6.06733736524985,
85.3434322070629));
#204734=CARTESIAN_POINT('Ctrl Pts',(-3.15813552791922,5.98485329705703,
85.3517295153375));
#204735=CARTESIAN_POINT('Ctrl Pts',(-3.31446350048274,5.90236089504557,
85.3600276619348));
#204736=CARTESIAN_POINT('Ctrl Pts',(-3.46757105987245,5.81373232664027,
85.368325808532));
#204737=CARTESIAN_POINT('Ctrl Pts',(-3.61696189367654,5.71925481681764,
85.3766239551292));
#204738=CARTESIAN_POINT('Ctrl Pts',(-3.76636774966895,5.62476780668695,
85.3849229361573));
#204739=CARTESIAN_POINT('Ctrl Pts',(-3.91205584060509,5.5244308684518,85.3932219171854));
#204740=CARTESIAN_POINT('Ctrl Pts',(-4.05355805395681,5.41857509897223,
85.4015208982135));
#204741=CARTESIAN_POINT('Ctrl Pts',(-4.19509801231297,5.31269109299801,
85.4098220929531));
#204742=CARTESIAN_POINT('Ctrl Pts',(-4.33244958896701,5.20128553019176,
85.4181232876927));
#204743=CARTESIAN_POINT('Ctrl Pts',(-4.46517688560014,5.08473051206278,
85.4264244824323));
#204744=CARTESIAN_POINT('Ctrl Pts',(-4.59796164694242,4.96812503106455,
85.4347292712007));
#204745=CARTESIAN_POINT('Ctrl Pts',(-4.72611787672735,4.84636588087864,
85.4430340599692));
#204746=CARTESIAN_POINT('Ctrl Pts',(-4.84924560815635,4.71986292510454,
85.4513388487377));
#204747=CARTESIAN_POINT('Ctrl Pts',(-4.97251930640533,4.5932100012123,85.4596534827587));
#204748=CARTESIAN_POINT('Ctrl Pts',(-5.09075235283867,4.46180228524923,
85.4679681167797));
#204749=CARTESIAN_POINT('Ctrl Pts',(-5.20358347502239,4.32608460602355,
85.4762827508007));
#204750=CARTESIAN_POINT('Ctrl Pts',(-5.31648594132527,4.19028111130573,
85.4846026422385));
#204751=CARTESIAN_POINT('Ctrl Pts',(-5.42397946013126,4.05016249427654,
85.4929225336763));
#204752=CARTESIAN_POINT('Ctrl Pts',(-5.52574532132024,3.90620373814621,
85.5012424251142));
#204753=CARTESIAN_POINT('Ctrl Pts',(-5.6276633554689,3.76202971699739,85.5095747574874));
#204754=CARTESIAN_POINT('Ctrl Pts',(-5.72383642602608,3.6140043726023,85.5179070898606));
#204755=CARTESIAN_POINT('Ctrl Pts',(-5.81399042155263,3.46262969115876,
85.5262394222338));
#204756=CARTESIAN_POINT('Ctrl Pts',(-5.88186598152559,3.34866201608571,
85.5325127074322));
#204757=CARTESIAN_POINT('Ctrl Pts',(-5.94633065287796,3.23279636145966,
85.5387859926306));
#204758=CARTESIAN_POINT('Ctrl Pts',(-6.0072853954291,3.11525459278439,85.545059277829));
#204759=CARTESIAN_POINT('Ctrl Pts',(-6.09005780069759,2.95564084485329,
85.5535779735543));
#204760=CARTESIAN_POINT('Ctrl Pts',(-6.16659053788697,2.79248414834737,
85.5620966692796));
#204761=CARTESIAN_POINT('Ctrl Pts',(-6.23657570988366,2.62629252271889,
85.5706153650049));
#204762=CARTESIAN_POINT('Ctrl Pts',(-6.30643161256696,2.46040786893491,
85.5791183258836));
#204763=CARTESIAN_POINT('Ctrl Pts',(-6.36976392634525,2.29149974865825,
85.5876212867623));
#204764=CARTESIAN_POINT('Ctrl Pts',(-6.42630967810643,2.12010210156863,
85.5961242476409));
#204765=CARTESIAN_POINT('Ctrl Pts',(-6.48271542230086,1.94912883591822,
85.6046061551455));
#204766=CARTESIAN_POINT('Ctrl Pts',(-6.53236801268392,1.77567863702722,
85.6130880626501));
#204767=CARTESIAN_POINT('Ctrl Pts',(-6.57505205867814,1.60030604125346,
85.6215699701548));
#204768=CARTESIAN_POINT('Ctrl Pts',(-6.61767563375348,1.42518189760665,
85.6300398612554));
#204769=CARTESIAN_POINT('Ctrl Pts',(-6.65335025806408,1.24814109133454,
85.638509752356));
#204770=CARTESIAN_POINT('Ctrl Pts',(-6.68190923369001,1.06975604355769,
85.6469796434566));
#204771=CARTESIAN_POINT('Ctrl Pts',(-6.71041353818299,0.891712482562082,
85.6554333204413));
#204772=CARTESIAN_POINT('Ctrl Pts',(-6.73182930768125,0.712330125957433,
85.6638869974259));
#204773=CARTESIAN_POINT('Ctrl Pts',(-6.74604022591236,0.53219382782244,
85.6723406744106));
#204774=CARTESIAN_POINT('Ctrl Pts',(-6.7599586881881,0.355764674596114,
85.6806203775437));
#204775=CARTESIAN_POINT('Ctrl Pts',(-6.76696587699467,0.178612617432928,
85.6889000806768));
#204776=CARTESIAN_POINT('Ctrl Pts',(-6.76699987560668,0.00129751271649814,
85.6971797838099));
#204777=CARTESIAN_POINT('',(-6.767,3.38585957231421E-12,85.3028202161898));
#204778=CARTESIAN_POINT('Ctrl Pts',(3.09910619832133,6.0156321173694,84.651395695404));
#204779=CARTESIAN_POINT('Ctrl Pts',(2.93375330764826,6.10081787314653,84.6601451433063));
#204780=CARTESIAN_POINT('Ctrl Pts',(2.76488627843069,6.17918207037039,84.6688945912086));
#204781=CARTESIAN_POINT('Ctrl Pts',(2.59307866646701,6.25045854553998,84.6776440391109));
#204782=CARTESIAN_POINT('Ctrl Pts',(2.4212724418537,6.3217344451504,84.6863934163612));
#204783=CARTESIAN_POINT('Ctrl Pts',(2.24652594672453,6.38592262741842,84.6951427936115));
#204784=CARTESIAN_POINT('Ctrl Pts',(2.06943269687104,6.44280508110567,84.7038921708618));
#204785=CARTESIAN_POINT('Ctrl Pts',(1.8923408182206,6.49968709436171,84.7126414803672));
#204786=CARTESIAN_POINT('Ctrl Pts',(1.71290249405572,6.54926340459549,84.7213907898726));
#204787=CARTESIAN_POINT('Ctrl Pts',(1.53172716625042,6.59136563150387,84.7301400993779));
#204788=CARTESIAN_POINT('Ctrl Pts',(1.35055318107316,6.63346754640714,84.7388893440452));
#204789=CARTESIAN_POINT('Ctrl Pts',(1.167642497144,6.66809542395779,84.7476385887124));
#204790=CARTESIAN_POINT('Ctrl Pts',(0.983616340614138,6.69513165624671,
84.7563878333796));
#204791=CARTESIAN_POINT('Ctrl Pts',(0.799591486713623,6.72216769715963,
84.7651370161153));
#204792=CARTESIAN_POINT('Ctrl Pts',(0.614451459526492,6.74161215869373,
84.773886198851));
#204793=CARTESIAN_POINT('Ctrl Pts',(0.428825047910062,6.75339900185713,
84.7826353815867));
#204794=CARTESIAN_POINT('Ctrl Pts',(0.243199888596733,6.76518576550222,
84.7913845052973));
#204795=CARTESIAN_POINT('Ctrl Pts',(0.0570886373915132,6.76931499599835,
84.8001336290078));
#204796=CARTESIAN_POINT('Ctrl Pts',(-0.128876626811645,6.76577266947846,
84.8088827527183));
#204797=CARTESIAN_POINT('Ctrl Pts',(-0.314840698188532,6.76223036567991,
84.8176318203099));
#204798=CARTESIAN_POINT('Ctrl Pts',(-0.500658497951505,6.75101660879221,
84.8263808879014));
#204799=CARTESIAN_POINT('Ctrl Pts',(-0.685698951926348,6.73216948296217,
84.835129955493));
#204800=CARTESIAN_POINT('Ctrl Pts',(-0.870738280460146,6.7133224717629,
84.8438789698715));
#204801=CARTESIAN_POINT('Ctrl Pts',(-1.05499998761296,6.6868422135618,84.85262798425));
#204802=CARTESIAN_POINT('Ctrl Pts',(-1.23785829161481,6.65281863948511,
84.8613769986285));
#204803=CARTESIAN_POINT('Ctrl Pts',(-1.43007412917461,6.61705395368849,
84.8705737323277));
#204804=CARTESIAN_POINT('Ctrl Pts',(-1.62073882535845,6.57295372727777,
84.8797704660269));
#204805=CARTESIAN_POINT('Ctrl Pts',(-1.80913696091563,6.52068343478266,
84.8889671997261));
#204806=CARTESIAN_POINT('Ctrl Pts',(-1.98838356186154,6.47095219815185,
84.8977171974398));
#204807=CARTESIAN_POINT('Ctrl Pts',(-2.16557827572569,6.41382586850878,
84.9064671951535));
#204808=CARTESIAN_POINT('Ctrl Pts',(-2.3401191862173,6.34949849943267,84.9152171928671));
#204809=CARTESIAN_POINT('Ctrl Pts',(-2.51465655691127,6.28517243495539,
84.9239670131254));
#204810=CARTESIAN_POINT('Ctrl Pts',(-2.68653996295356,6.21364572242362,
84.9327168333838));
#204811=CARTESIAN_POINT('Ctrl Pts',(-2.85518555380015,6.13516132252208,
84.9414666536421));
#204812=CARTESIAN_POINT('Ctrl Pts',(-3.02382794858705,6.05667841000498,
84.9502163080796));
#204813=CARTESIAN_POINT('Ctrl Pts',(-3.18923239109288,5.97123819492077,
84.9589659625171));
#204814=CARTESIAN_POINT('Ctrl Pts',(-3.35083705967695,5.87913088810715,
84.9677156169546));
#204815=CARTESIAN_POINT('Ctrl Pts',(-3.51243888042392,5.78702520443108,
84.9764651172035));
#204816=CARTESIAN_POINT('Ctrl Pts',(-3.67024081223678,5.68825280605791,
84.9852146174524));
#204817=CARTESIAN_POINT('Ctrl Pts',(-3.82370687544385,5.58314917682516,
84.9939641177014));
#204818=CARTESIAN_POINT('Ctrl Pts',(-3.97717043817796,5.47804726008035,
85.0027134753918));
#204819=CARTESIAN_POINT('Ctrl Pts',(-4.12629803722439,5.36661448084252,
85.0114628330823));
#204820=CARTESIAN_POINT('Ctrl Pts',(-4.27058317206883,5.24922931204596,
85.0202121907728));
#204821=CARTESIAN_POINT('Ctrl Pts',(-4.4148661477481,5.13184589986812,85.0289614175328));
#204822=CARTESIAN_POINT('Ctrl Pts',(-4.55430658194388,5.00851045723057,
85.0377106442929));
#204823=CARTESIAN_POINT('Ctrl Pts',(-4.6884308900182,4.87964187103144,85.046459871053));
#204824=CARTESIAN_POINT('Ctrl Pts',(-4.82255336917833,4.75077504207965,
85.0552089785089));
#204825=CARTESIAN_POINT('Ctrl Pts',(-4.95135966065151,4.61637541908077,
85.0639580859649));
#204826=CARTESIAN_POINT('Ctrl Pts',(-5.07441230869279,4.47689945401805,
85.0727071934208));
#204827=CARTESIAN_POINT('Ctrl Pts',(-5.19746344226474,4.33742520555449,
85.0814561931972));
#204828=CARTESIAN_POINT('Ctrl Pts',(-5.31476088454844,4.19287495491241,
85.0902051929736));
#204829=CARTESIAN_POINT('Ctrl Pts',(-5.42590627628947,4.0437396158658,85.0989541927499));
#204830=CARTESIAN_POINT('Ctrl Pts',(-5.53706380672759,3.89458798906604,
85.1077041480446));
#204831=CARTESIAN_POINT('Ctrl Pts',(-5.64206777071953,3.74085050155149,
85.1164541033393));
#204832=CARTESIAN_POINT('Ctrl Pts',(-5.74056148164094,3.58304938223022,
85.125204058634));
#204833=CARTESIAN_POINT('Ctrl Pts',(-5.8390513895197,3.42525435593135,85.1339536760752));
#204834=CARTESIAN_POINT('Ctrl Pts',(-5.93103139557738,3.26339625497028,
85.1427032935163));
#204835=CARTESIAN_POINT('Ctrl Pts',(-6.0161890782093,3.09802485064841,85.1514529109574));
#204836=CARTESIAN_POINT('Ctrl Pts',(-6.10134392545072,2.93265895249457,
85.1602022370733));
#204837=CARTESIAN_POINT('Ctrl Pts',(-6.17967677261924,2.76378023985831,
85.1689515631891));
#204838=CARTESIAN_POINT('Ctrl Pts',(-6.25092157009318,2.59196229226891,
85.177700889305));
#204839=CARTESIAN_POINT('Ctrl Pts',(-6.32216437407842,2.42014915228859,
85.1864499706075));
#204840=CARTESIAN_POINT('Ctrl Pts',(-6.38631941549005,2.24539720662612,
85.1951990519099));
#204841=CARTESIAN_POINT('Ctrl Pts',(-6.44316881037616,2.0682999494744,85.2039481332124));
#204842=CARTESIAN_POINT('Ctrl Pts',(-6.50002334524642,1.89118668024207,
85.2126980055547));
#204843=CARTESIAN_POINT('Ctrl Pts',(-6.54957082411158,1.71172794807464,
85.2214478778971));
#204844=CARTESIAN_POINT('Ctrl Pts',(-6.59164294296138,1.53053334250105,
85.2301977502394));
#204845=CARTESIAN_POINT('Ctrl Pts',(-6.63371214082185,1.3493513169335,85.2389470150943));
#204846=CARTESIAN_POINT('Ctrl Pts',(-6.66830695239737,1.16643393829499,
85.2476962799492));
#204847=CARTESIAN_POINT('Ctrl Pts',(-6.69530988154029,0.982402458338193,
85.2564455448041));
#204848=CARTESIAN_POINT('Ctrl Pts',(-6.72231419690515,0.798361530944327,
85.2651952588112));
#204849=CARTESIAN_POINT('Ctrl Pts',(-6.74172580829302,0.613206671359816,
85.2739449728182));
#204850=CARTESIAN_POINT('Ctrl Pts',(-6.75347878028196,0.427566795110811,
85.2826946868252));
#204851=CARTESIAN_POINT('Ctrl Pts',(-6.76248992368217,0.285234494204192,
85.2894031966134));
#204852=CARTESIAN_POINT('Ctrl Pts',(-6.76699999999993,0.142617266092563,
85.2961117064016));
#204853=CARTESIAN_POINT('Ctrl Pts',(-6.767,3.38585956577759E-12,85.3028202161898));
#204854=CARTESIAN_POINT('Ctrl Pts',(-6.76699999999426,8.81760040218907E-6,
85.3030125520247));
#204855=CARTESIAN_POINT('Ctrl Pts',(-6.76700021690518,-0.166457813100077,
85.310839071891));
#204856=CARTESIAN_POINT('Ctrl Pts',(-6.76085354170972,-0.333110924625458,
85.3186655917572));
#204857=CARTESIAN_POINT('Ctrl Pts',(-6.74854471695431,-0.49943288164484,
85.3264921116235));
#204858=CARTESIAN_POINT('Ctrl Pts',(-6.73624143578192,-0.665679931466091,
85.3343151066234));
#204859=CARTESIAN_POINT('Ctrl Pts',(-6.71778154932752,-0.831595732536135,
85.3421381016233));
#204860=CARTESIAN_POINT('Ctrl Pts',(-6.69320189408862,-0.996663135150782,
85.3499610966232));
#204861=CARTESIAN_POINT('Ctrl Pts',(-6.66862904033346,-1.16168486164644,
85.3577819269071));
#204862=CARTESIAN_POINT('Ctrl Pts',(-6.63793984559386,-1.3258582686396,
85.365602757191));
#204863=CARTESIAN_POINT('Ctrl Pts',(-6.60122290099131,-1.48867229819993,
85.3734235874748));
#204864=CARTESIAN_POINT('Ctrl Pts',(-6.56450073493061,-1.65150948128383,
85.3812455299465));
#204865=CARTESIAN_POINT('Ctrl Pts',(-6.52174918981563,-1.81298651663494,
85.3890674724182));
#204866=CARTESIAN_POINT('Ctrl Pts',(-6.47310775543939,-1.9726036060168,
85.3968894148899));
#204867=CARTESIAN_POINT('Ctrl Pts',(-6.44432244876842,-2.06706272151583,
85.4015183288127));
#204868=CARTESIAN_POINT('Ctrl Pts',(-6.41347540245782,-2.16087071110073,
85.4061472427355));
#204869=CARTESIAN_POINT('Ctrl Pts',(-6.38060368627069,-2.25392670660535,
85.4107761566583));
#204870=CARTESIAN_POINT('Ctrl Pts',(-6.31680169767356,-2.43454269666451,
85.4197605951841));
#204871=CARTESIAN_POINT('Ctrl Pts',(-6.24538097869586,-2.61229424427641,
85.4287450337099));
#204872=CARTESIAN_POINT('Ctrl Pts',(-6.16662721156435,-2.78657456989654,
85.4377294722357));
#204873=CARTESIAN_POINT('Ctrl Pts',(-6.08773752013061,-2.96115569295806,
85.4467294173662));
#204874=CARTESIAN_POINT('Ctrl Pts',(-6.00148958222123,-3.13225340160032,
85.4557293624967));
#204875=CARTESIAN_POINT('Ctrl Pts',(-5.90821535324118,-3.29928482246155,
85.4647293076272));
#204876=CARTESIAN_POINT('Ctrl Pts',(-5.81472132114677,-3.46670985715271,
85.4737504613594));
#204877=CARTESIAN_POINT('Ctrl Pts',(-5.71416798582239,-3.63004922193328,
85.4827716150916));
#204878=CARTESIAN_POINT('Ctrl Pts',(-5.60693253178595,-3.78874604374592,
85.4917927688238));
#204879=CARTESIAN_POINT('Ctrl Pts',(-5.49958796482978,-3.94760434082565,
85.500823101651));
#204880=CARTESIAN_POINT('Ctrl Pts',(-5.38554783485579,-4.10181046343896,
85.5098534344783));
#204881=CARTESIAN_POINT('Ctrl Pts',(-5.26523110145149,-4.25083879349804,
85.5188837673055));
#204882=CARTESIAN_POINT('Ctrl Pts',(-5.14474379684518,-4.40007839875279,
85.5279269022981));
#204883=CARTESIAN_POINT('Ctrl Pts',(-5.01796224673951,-4.54412534796465,
85.5369700372908));
#204884=CARTESIAN_POINT('Ctrl Pts',(-4.88534545312323,-4.68248745899529,
85.5460131722834));
#204885=CARTESIAN_POINT('Ctrl Pts',(-4.76940782238251,-4.80344782079978,
85.5539189556833));
#204886=CARTESIAN_POINT('Ctrl Pts',(-4.64901108990684,-4.92006385517504,
85.5618247390832));
#204887=CARTESIAN_POINT('Ctrl Pts',(-4.52448428868203,-5.03203049687395,
85.569730522483));
#204888=CARTESIAN_POINT('Ctrl Pts',(-4.38818169837358,-5.1545851850342,
85.5783839107113));
#204889=CARTESIAN_POINT('Ctrl Pts',(-4.2468097099974,-5.27167687447455,
85.5870372989395));
#204890=CARTESIAN_POINT('Ctrl Pts',(-4.10082390915043,-5.38289255569347,
85.5956906871678));
#204891=CARTESIAN_POINT('Ctrl Pts',(-3.95497293654614,-5.49400552134164,
85.6043360833782));
#204892=CARTESIAN_POINT('Ctrl Pts',(-3.80451689149178,-5.59925311926044,
85.6129814795886));
#204893=CARTESIAN_POINT('Ctrl Pts',(-3.64994492812084,-5.69826210538661,
85.621626875799));
#204894=CARTESIAN_POINT('Ctrl Pts',(-3.49043645693213,-5.8004331050072,
85.6305483768414));
#204895=CARTESIAN_POINT('Ctrl Pts',(-3.32654505478421,-5.89596019245491,
85.6394698778838));
#204896=CARTESIAN_POINT('Ctrl Pts',(-3.15884329998869,-5.98447976069069,
85.6483913789262));
#204897=CARTESIAN_POINT('Ctrl Pts',(-2.99664113765321,-6.07009642817492,
85.6570203092681));
#204898=CARTESIAN_POINT('Ctrl Pts',(-2.83087485950027,-6.14915772209436,
85.6656492396101));
#204899=CARTESIAN_POINT('Ctrl Pts',(-2.66209046795408,-6.22137953676096,
85.6742781699521));
#204900=CARTESIAN_POINT('Ctrl Pts',(-2.48472192419546,-6.29727445795405,
85.6833459563447));
#204901=CARTESIAN_POINT('Ctrl Pts',(-2.30402055860341,-6.36561589289683,
85.6924137427373));
#204902=CARTESIAN_POINT('Ctrl Pts',(-2.12064792181933,-6.42612958099067,
85.7014815291299));
#204903=CARTESIAN_POINT('Ctrl Pts',(-1.93727528503519,-6.48664326908454,
85.7105493155225));
#204904=CARTESIAN_POINT('Ctrl Pts',(-1.75123173686825,-6.53932905451853,
85.7196171019152));
#204905=CARTESIAN_POINT('Ctrl Pts',(-1.56320225990795,-6.58397203021236,
85.7286848883078));
#204906=CARTESIAN_POINT('Ctrl Pts',(-1.3885025011636,-6.62545019209115,
85.737109844441));
#204907=CARTESIAN_POINT('Ctrl Pts',(-1.21216511647651,-6.65996749395453,
85.7455348005742));
#204908=CARTESIAN_POINT('Ctrl Pts',(-1.03477051646232,-6.6874164651426,
85.7539597567074));
#204909=CARTESIAN_POINT('Ctrl Pts',(-0.857334741458616,-6.71487180750037,
85.7623866683537));
#204910=CARTESIAN_POINT('Ctrl Pts',(-0.678841589563437,-6.7352554973071,
85.7708135800001));
#204911=CARTESIAN_POINT('Ctrl Pts',(-0.499878492326469,-6.74851172429221,
85.7792404916465));
#204912=CARTESIAN_POINT('Ctrl Pts',(-0.320849583386895,-6.7617728261084,
85.7876705021966));
#204913=CARTESIAN_POINT('Ctrl Pts',(-0.141350715065076,-6.76790121450158,
85.7961005127466));
#204914=CARTESIAN_POINT('Ctrl Pts',(0.03802837429104,-6.76689314550989,
85.8045305232967));
#204915=CARTESIAN_POINT('Ctrl Pts',(0.217572703912353,-6.76588414790614,
85.8129682993962));
#204916=CARTESIAN_POINT('Ctrl Pts',(0.396996702288371,-6.75772556060025,
85.8214060754956));
#204917=CARTESIAN_POINT('Ctrl Pts',(0.575712320100965,-6.74246574514724,
85.8298438515951));
#204918=CARTESIAN_POINT('Ctrl Pts',(0.754521750438224,-6.72719791941606,
85.838286056905));
#204919=CARTESIAN_POINT('Ctrl Pts',(0.932621729260149,-6.70482146719918,
85.8467282622149));
#204920=CARTESIAN_POINT('Ctrl Pts',(1.10943154956437,-6.6754363630276,85.8551704675248));
#204921=CARTESIAN_POINT('Ctrl Pts',(1.28642789450093,-6.6460202591879,85.8636215788968));
#204922=CARTESIAN_POINT('Ctrl Pts',(1.46213103664878,-6.60958079575246,
85.8720726902688));
#204923=CARTESIAN_POINT('Ctrl Pts',(1.63597158178026,-6.56626880226567,
85.8805238016408));
#204924=CARTESIAN_POINT('Ctrl Pts',(1.68476020004871,-6.55411322420374,
85.8828956191381));
#204925=CARTESIAN_POINT('Ctrl Pts',(1.73340220587232,-6.54141662990167,
85.8852674366353));
#204926=CARTESIAN_POINT('Ctrl Pts',(1.78188525111196,-6.52818305134512,
85.8876392541326));
#204927=CARTESIAN_POINT('Ctrl Pts',(1.95188071309984,-6.48178232941534,
85.8959555265367));
#204928=CARTESIAN_POINT('Ctrl Pts',(2.12022741980042,-6.42869236466029,
85.9042717989408));
#204929=CARTESIAN_POINT('Ctrl Pts',(2.28637078269115,-6.36904997971097,
85.9125880713449));
#204930=CARTESIAN_POINT('Ctrl Pts',(2.45237367117229,-6.30945802246857,
85.9208973123309));
#204931=CARTESIAN_POINT('Ctrl Pts',(2.61617660165709,-6.24332479987565,
85.9292065533169));
#204932=CARTESIAN_POINT('Ctrl Pts',(2.77723907424595,-6.17083723043166,
85.9375157943029));
#204933=CARTESIAN_POINT('Ctrl Pts',(2.93819489855025,-6.09839765897758,
85.9458195332853));
#204934=CARTESIAN_POINT('Ctrl Pts',(3.09641356454046,-6.01961226702696,
85.9541232722678));
#204935=CARTESIAN_POINT('Ctrl Pts',(3.25137331876829,-5.93471655110854,
85.9624270112502));
#204936=CARTESIAN_POINT('Ctrl Pts',(3.40625886433244,-5.84986149089239,
85.9707267736558));
#204937=CARTESIAN_POINT('Ctrl Pts',(3.55788830384298,-5.75890210508579,
85.9790265360614));
#204938=CARTESIAN_POINT('Ctrl Pts',(3.70576312159477,-5.66212051148933,
85.9873262984669));
#204939=CARTESIAN_POINT('Ctrl Pts',(3.85359421470125,-5.56536753494151,
85.9956236067416));
#204940=CARTESIAN_POINT('Ctrl Pts',(3.99767260818949,-5.46279597245703,
86.0039209150161));
#204941=CARTESIAN_POINT('Ctrl Pts',(4.13752730753579,-5.35473218559021,
86.0122182232907));
#204942=CARTESIAN_POINT('Ctrl Pts',(4.27739613717027,-5.24665748044564,
86.020516369888));
#204943=CARTESIAN_POINT('Ctrl Pts',(4.41304014003943,-5.13308964888474,
86.0288145164852));
#204944=CARTESIAN_POINT('Ctrl Pts',(4.54401960099712,-5.01439675990582,
86.0371126630825));
#204945=CARTESIAN_POINT('Ctrl Pts',(4.67501223276379,-4.89569193561004,
86.0454116441105));
#204946=CARTESIAN_POINT('Ctrl Pts',(4.80133912936477,-4.77186126004794,
86.0537106251386));
#204947=CARTESIAN_POINT('Ctrl Pts',(4.92259588018237,-4.64331118927125,
86.0620096061667));
#204948=CARTESIAN_POINT('Ctrl Pts',(5.0438849756283,-4.51472682840981,86.0703108009062));
#204949=CARTESIAN_POINT('Ctrl Pts',(5.16010099092831,-4.38142081646386,
86.0786119956458));
#204950=CARTESIAN_POINT('Ctrl Pts',(5.27087828325675,-4.24383448347039,
86.0869131903853));
#204951=CARTESIAN_POINT('Ctrl Pts',(5.38170353696998,-4.10618858203179,
86.0952179791538));
#204952=CARTESIAN_POINT('Ctrl Pts',(5.48708515662819,-3.96425893704951,
86.1035227679222));
#204953=CARTESIAN_POINT('Ctrl Pts',(5.58669937349187,-3.81851792063696,
86.1118275566907));
#204954=CARTESIAN_POINT('Ctrl Pts',(5.68643168211522,-3.67260412955802,
86.1201421907117));
#204955=CARTESIAN_POINT('Ctrl Pts',(5.78038273072586,-3.52287022708953,
86.1284568247327));
#204956=CARTESIAN_POINT('Ctrl Pts',(5.86827286704844,-3.36981639824236,
86.1367714587537));
#204957=CARTESIAN_POINT('Ctrl Pts',(5.95621857708335,-3.2166657921024,86.1450913501915));
#204958=CARTESIAN_POINT('Ctrl Pts',(6.03809557102104,-3.06019138113712,
86.1534112416293));
#204959=CARTESIAN_POINT('Ctrl Pts',(6.11367129886114,-2.90091576049384,
86.1617311330671));
#204960=CARTESIAN_POINT('Ctrl Pts',(6.18936003691977,-2.7414019711526,86.1700634654403));
#204961=CARTESIAN_POINT('Ctrl Pts',(6.25872854155942,-2.57907892088648,
86.1783957978135));
#204962=CARTESIAN_POINT('Ctrl Pts',(6.32159283092554,-2.41448816107904,
86.1867281301867));
#204963=CARTESIAN_POINT('Ctrl Pts',(6.36892238984446,-2.29057030338326,
86.1930014153852));
#204964=CARTESIAN_POINT('Ctrl Pts',(6.41256614476117,-2.16536740233288,
86.1992747005836));
#204965=CARTESIAN_POINT('Ctrl Pts',(6.45246456311795,-2.03911501924414,
86.205547985782));
#204966=CARTESIAN_POINT('Ctrl Pts',(6.50378920111996,-1.87670612872185,
86.2136178317848));
#204967=CARTESIAN_POINT('Ctrl Pts',(6.54907277841643,-1.71205827198792,
86.2216876777875));
#204968=CARTESIAN_POINT('Ctrl Pts',(6.58810987231774,-1.54567050507847,
86.2297575237903));
#204969=CARTESIAN_POINT('Ctrl Pts',(6.62709785258962,-1.37949207514341,
86.2378172169003));
#204970=CARTESIAN_POINT('Ctrl Pts',(6.65985490231959,-1.21157844919782,
86.2458769100104));
#204971=CARTESIAN_POINT('Ctrl Pts',(6.68622408375805,-1.04244736163216,
86.2539366031204));
#204972=CARTESIAN_POINT('Ctrl Pts',(6.71256587661338,-0.873491943563923,
86.2619879249591));
#204973=CARTESIAN_POINT('Ctrl Pts',(6.73253294754114,-0.703321945801222,
86.2700392467977));
#204974=CARTESIAN_POINT('Ctrl Pts',(6.74601852567449,-0.532468826558542,
86.2780905686363));
#204975=CARTESIAN_POINT('Ctrl Pts',(6.75949305204262,-0.361755725677831,
86.2861352922173));
#204976=CARTESIAN_POINT('Ctrl Pts',(6.76649662848728,-0.190360987609441,
86.2941800157983));
#204977=CARTESIAN_POINT('Ctrl Pts',(6.76697381633973,-0.0188246905025418,
86.3022247393793));
#204978=CARTESIAN_POINT('Ctrl Pts',(6.76745071758155,0.152608577733117,
86.3102646311037));
#204979=CARTESIAN_POINT('Ctrl Pts',(6.76140903252064,0.324182863595643,
86.3183045228282));
#204980=CARTESIAN_POINT('Ctrl Pts',(6.74884529036586,0.495354667593435,
86.3263444145526));
#204981=CARTESIAN_POINT('Ctrl Pts',(6.73601101642186,0.670212269487086,
86.3345574271725));
#204982=CARTESIAN_POINT('Ctrl Pts',(6.71637059217592,0.844649462487381,
86.3427704397925));
#204983=CARTESIAN_POINT('Ctrl Pts',(6.68997648786138,1.01808820436242,86.3509834524125));
#204984=CARTESIAN_POINT('Ctrl Pts',(6.66414775601771,1.18781181770462,86.359020538955));
#204985=CARTESIAN_POINT('Ctrl Pts',(6.63185181772796,1.35657893875707,86.3670576254976));
#204986=CARTESIAN_POINT('Ctrl Pts',(6.59319008474597,1.52385481802155,86.3750947120402));
#204987=CARTESIAN_POINT('Ctrl Pts',(6.55452465165618,1.69114670636625,86.3831325677693));
#204988=CARTESIAN_POINT('Ctrl Pts',(6.50949229479818,1.85694670467716,86.3911704234985));
#204989=CARTESIAN_POINT('Ctrl Pts',(6.4582451107684,2.02073231508681,86.3992082792277));
#204990=CARTESIAN_POINT('Ctrl Pts',(6.40698286836635,2.18456605193971,86.4072484967846));
#204991=CARTESIAN_POINT('Ctrl Pts',(6.34950227540817,2.34638386635018,86.4152887143416));
#204992=CARTESIAN_POINT('Ctrl Pts',(6.28600460439041,2.50568056894382,86.4233289318985));
#204993=CARTESIAN_POINT('Ctrl Pts',(6.22010795067768,2.67099560302524,86.4316729140263));
#204994=CARTESIAN_POINT('Ctrl Pts',(6.14773084491761,2.83359489251654,86.440016896154));
#204995=CARTESIAN_POINT('Ctrl Pts',(6.06915147397983,2.9929399235348,86.4483608782818));
#204996=CARTESIAN_POINT('Ctrl Pts',(5.99330098371672,3.1467512684143,86.4564150931168));
#204997=CARTESIAN_POINT('Ctrl Pts',(5.91167202087316,3.29753029957398,86.4644693079519));
#204998=CARTESIAN_POINT('Ctrl Pts',(5.82455972292786,3.44482119043159,86.4725235227869));
#204999=CARTESIAN_POINT('Ctrl Pts',(5.73738223583291,3.5922223041642,86.4805837648699));
#205000=CARTESIAN_POINT('Ctrl Pts',(5.64471344418015,3.73612976820829,86.4886440069529));
#205001=CARTESIAN_POINT('Ctrl Pts',(5.54688994195431,3.87611931857704,86.4967042490358));
#205002=CARTESIAN_POINT('Ctrl Pts',(5.44892967576163,4.01630458394055,86.5047757598902));
#205003=CARTESIAN_POINT('Ctrl Pts',(5.34580054384363,4.15256071197133,86.5128472707445));
#205004=CARTESIAN_POINT('Ctrl Pts',(5.23787762964169,4.28449844636443,86.5209187815989));
#205005=CARTESIAN_POINT('Ctrl Pts',(5.22656618142751,4.29832689846952,86.5217647602097));
#205006=CARTESIAN_POINT('Ctrl Pts',(5.21520210372238,4.31210794734796,86.5226107388206));
#205007=CARTESIAN_POINT('Ctrl Pts',(5.20378584998983,4.32584116992818,86.5234567174315));
#205008=CARTESIAN_POINT('Ctrl Pts',(5.09271791362746,4.4594507346177,86.5316871843359));
#205009=CARTESIAN_POINT('Ctrl Pts',(4.97633771015214,4.58897633015651,86.5399176512402));
#205010=CARTESIAN_POINT('Ctrl Pts',(4.85497578109233,4.71396851548745,86.5481481181446));
#205011=CARTESIAN_POINT('Ctrl Pts',(4.72803515647347,4.84470626991591,86.5567569184318));
#205012=CARTESIAN_POINT('Ctrl Pts',(4.59564415093411,4.97048364059416,86.565365718719));
#205013=CARTESIAN_POINT('Ctrl Pts',(4.45823065755993,5.09082197724422,86.5739745190062));
#205014=CARTESIAN_POINT('Ctrl Pts',(4.32717392744067,5.20559344925974,86.5821850752491));
#205015=CARTESIAN_POINT('Ctrl Pts',(4.19154920801982,5.31541745721965,86.5903956314921));
#205016=CARTESIAN_POINT('Ctrl Pts',(4.0517674352365,5.41991417374454,86.598606187735));
#205017=CARTESIAN_POINT('Ctrl Pts',(3.91208318633185,5.52433798430395,86.6068110155824));
#205018=CARTESIAN_POINT('Ctrl Pts',(3.76824794408863,5.62344168917379,86.6150158434298));
#205019=CARTESIAN_POINT('Ctrl Pts',(3.62070678920349,5.71688475890635,86.6232206712771));
#205020=CARTESIAN_POINT('Ctrl Pts',(3.47325584970364,5.81027069202138,86.6314204822076));
#205021=CARTESIAN_POINT('Ctrl Pts',(3.32210381493285,5.89800269529541,86.6396202931382));
#205022=CARTESIAN_POINT('Ctrl Pts',(3.16772581273165,5.97978278663645,86.6478201040687));
#205023=CARTESIAN_POINT('Ctrl Pts',(3.14492241646647,5.99186264129749,86.6490313099094));
#205024=CARTESIAN_POINT('Ctrl Pts',(3.1220486842215,6.00381271105085,86.6502425157501));
#205025=CARTESIAN_POINT('Ctrl Pts',(3.09910619832139,6.01563211736938,86.6514537215909));
#205026=CARTESIAN_POINT('Origin',(0.,0.,4.30282021618968));
#205027=CARTESIAN_POINT('',(3.09910619832144,6.01563211736935,89.0458803684832));
#205028=CARTESIAN_POINT('',(3.09910619832125,6.01563211736945,88.6513956954041));
#205029=CARTESIAN_POINT('',(3.09910619832133,6.0156321173694,4.30282021618968));
#205030=CARTESIAN_POINT('',(-6.76699899245737,-0.00240081800135623,87.6971797838099));
#205031=CARTESIAN_POINT('Ctrl Pts',(-6.76699761639396,-0.00567976394980745,
87.6971797838099));
#205032=CARTESIAN_POINT('Ctrl Pts',(-6.76677386767964,-0.272258979179347,
87.7097537505765));
#205033=CARTESIAN_POINT('Ctrl Pts',(-6.75079460165027,-0.538161101664258,
87.7223277173431));
#205034=CARTESIAN_POINT('Ctrl Pts',(-6.71931721421665,-0.801913445910326,
87.7349016841098));
#205035=CARTESIAN_POINT('Ctrl Pts',(-6.68967829484414,-1.05026107266005,
87.7467412558651));
#205036=CARTESIAN_POINT('Ctrl Pts',(-6.64629915915566,-1.29670433671583,
87.7585808276203));
#205037=CARTESIAN_POINT('Ctrl Pts',(-6.58942873953572,-1.54003827438822,
87.7704203993756));
#205038=CARTESIAN_POINT('Ctrl Pts',(-6.55066589085075,-1.70589456081885,
87.7784902453784));
#205039=CARTESIAN_POINT('Ctrl Pts',(-6.50556537859396,-1.87059265702531,
87.7865600913812));
#205040=CARTESIAN_POINT('Ctrl Pts',(-6.45420528747431,-2.03359856096002,
87.7946299373839));
#205041=CARTESIAN_POINT('Ctrl Pts',(-6.40290981388201,-2.19639938273411,
87.802689630494));
#205042=CARTESIAN_POINT('Ctrl Pts',(-6.345370541888,-2.35751189703273,87.810749323604));
#205043=CARTESIAN_POINT('Ctrl Pts',(-6.28171678335449,-2.51641078795225,
87.8188090167141));
#205044=CARTESIAN_POINT('Ctrl Pts',(-6.2181291393595,-2.67514463713527,
87.8268603385527));
#205045=CARTESIAN_POINT('Ctrl Pts',(-6.1484397846706,-2.83166909497776,
87.8349116603913));
#205046=CARTESIAN_POINT('Ctrl Pts',(-6.07282817571208,-2.98547265073346,
87.8429629822299));
#205047=CARTESIAN_POINT('Ctrl Pts',(-5.9972785323391,-3.13915016066734,
87.8510077058109));
#205048=CARTESIAN_POINT('Ctrl Pts',(-5.91581645835378,-3.29011087351234,
87.859052429392));
#205049=CARTESIAN_POINT('Ctrl Pts',(-5.82866995165558,-3.43786206742903,
87.867097152973));
#205050=CARTESIAN_POINT('Ctrl Pts',(-5.74157578726874,-3.58552451838527,
87.8751370446974));
#205051=CARTESIAN_POINT('Ctrl Pts',(-5.64880417587126,-3.72998096734556,
87.8831769364218));
#205052=CARTESIAN_POINT('Ctrl Pts',(-5.55062954996713,-3.87076227622309,
87.8912168281462));
#205053=CARTESIAN_POINT('Ctrl Pts',(-5.45034095540003,-4.01457499237677,
87.8994298407661));
#205054=CARTESIAN_POINT('Ctrl Pts',(-5.34441419912616,-4.15455214362565,
87.9076428533861));
#205055=CARTESIAN_POINT('Ctrl Pts',(-5.23318945006422,-4.29022344170284,
87.9158558660061));
#205056=CARTESIAN_POINT('Ctrl Pts',(-5.1243471804551,-4.42298860528448,
87.9238929525486));
#205057=CARTESIAN_POINT('Ctrl Pts',(-5.01043184572974,-4.55163022099534,
87.9319300390912));
#205058=CARTESIAN_POINT('Ctrl Pts',(-4.89180360283301,-4.67574020998921,
87.9399671256338));
#205059=CARTESIAN_POINT('Ctrl Pts',(-4.77316400666122,-4.79986207688677,
87.9480049813629));
#205060=CARTESIAN_POINT('Ctrl Pts',(-4.6498108622847,-4.91945118331582,
87.9560428370921));
#205061=CARTESIAN_POINT('Ctrl Pts',(-4.52214165802727,-5.03413585680148,
87.9640806928213));
#205062=CARTESIAN_POINT('Ctrl Pts',(-4.3944349397009,-5.14885422900698,
87.9721209103782));
#205063=CARTESIAN_POINT('Ctrl Pts',(-4.26240991493434,-5.25866505025289,
87.9801611279351));
#205064=CARTESIAN_POINT('Ctrl Pts',(-4.12649752469757,-5.36323663273073,
87.9882013454921));
#205065=CARTESIAN_POINT('Ctrl Pts',(-3.98545027727593,-5.47175899659563,
87.9965453276199));
#205066=CARTESIAN_POINT('Ctrl Pts',(-3.84021654539729,-5.57463823408338,
88.0048893097476));
#205067=CARTESIAN_POINT('Ctrl Pts',(-3.69131042004525,-5.67155326016298,
88.0132332918754));
#205068=CARTESIAN_POINT('Ctrl Pts',(-3.54757546166741,-5.7651026504705,
88.0212875067105));
#205069=CARTESIAN_POINT('Ctrl Pts',(-3.4004192511565,-5.85309499968583,
88.0293417215455));
#205070=CARTESIAN_POINT('Ctrl Pts',(-3.25032824980126,-5.93528897936267,
88.0373959363806));
#205071=CARTESIAN_POINT('Ctrl Pts',(-3.10012493015034,-6.01754446764181,
88.0454561784636));
#205072=CARTESIAN_POINT('Ctrl Pts',(-2.94698277869687,-6.09399278091668,
88.0535164205466));
#205073=CARTESIAN_POINT('Ctrl Pts',(-2.79140779562201,-6.16444089261473,
88.0615766626296));
#205074=CARTESIAN_POINT('Ctrl Pts',(-2.63561530804912,-6.23498749560533,
88.069648173484));
#205075=CARTESIAN_POINT('Ctrl Pts',(-2.47738354540936,-6.29951702038352,
88.0777196843383));
#205076=CARTESIAN_POINT('Ctrl Pts',(-2.31723373688198,-6.35788619028809,
88.0857911951927));
#205077=CARTESIAN_POINT('Ctrl Pts',(-2.30044836484954,-6.36400388871734,
88.0866371738036));
#205078=CARTESIAN_POINT('Ctrl Pts',(-2.28364193153735,-6.3700539605859,
88.0874831524145));
#205079=CARTESIAN_POINT('Ctrl Pts',(-2.2668150428355,-6.37603627354603,
88.0883291310254));
#205080=CARTESIAN_POINT('Ctrl Pts',(-2.10313162623069,-6.43422917193996,
88.0965583807613));
#205081=CARTESIAN_POINT('Ctrl Pts',(-1.93696538622776,-6.48620049473463,
88.1047876304973));
#205082=CARTESIAN_POINT('Ctrl Pts',(-1.76882973990278,-6.53173256886988,
88.1130168802333));
#205083=CARTESIAN_POINT('Ctrl Pts',(-1.600894202349,-6.57721045242981,88.1212363358233));
#205084=CARTESIAN_POINT('Ctrl Pts',(-1.43099426845363,-6.61626425463261,
88.1294557914134));
#205085=CARTESIAN_POINT('Ctrl Pts',(-1.25966241056945,-6.64872466051937,
88.1376752470035));
#205086=CARTESIAN_POINT('Ctrl Pts',(-1.08850005781628,-6.68115295209054,
88.1458865707731));
#205087=CARTESIAN_POINT('Ctrl Pts',(-0.915908952253664,-6.70700077162168,
88.1540978945428));
#205088=CARTESIAN_POINT('Ctrl Pts',(-0.742435866460153,-6.72614882263198,
88.1623092183124));
#205089=CARTESIAN_POINT('Ctrl Pts',(-0.569099579126017,-6.74528177375594,
88.1705140667465));
#205090=CARTESIAN_POINT('Ctrl Pts',(-0.394883051739474,-6.75772544035168,
88.1787189151806));
#205091=CARTESIAN_POINT('Ctrl Pts',(-0.220342460866645,-6.76341172781454,
88.1869237636147));
#205092=CARTESIAN_POINT('Ctrl Pts',(-0.0459044799351441,-6.76909467238954,
88.1951237885347));
#205093=CARTESIAN_POINT('Ctrl Pts',(0.128856827466691,-6.76802813993521,
88.2033238134546));
#205094=CARTESIAN_POINT('Ctrl Pts',(0.303380870132504,-6.76019593263669,
88.2115238383745));
#205095=CARTESIAN_POINT('Ctrl Pts',(0.477854401586501,-6.75236599215641,
88.2197214900214));
#205096=CARTESIAN_POINT('Ctrl Pts',(0.652090447071619,-6.73777428929547,
88.2279191416683));
#205097=CARTESIAN_POINT('Ctrl Pts',(0.825528870059933,-6.71645673586137,
88.2361167933152));
#205098=CARTESIAN_POINT('Ctrl Pts',(0.998944068579247,-6.69514203697848,
88.2443133472463));
#205099=CARTESIAN_POINT('Ctrl Pts',(1.17156150126438,-6.66710332416293,
88.2525099011774));
#205100=CARTESIAN_POINT('Ctrl Pts',(1.34282659419896,-6.63242834397116,
88.2607064551085));
#205101=CARTESIAN_POINT('Ctrl Pts',(1.51409989413084,-6.5977517021596,88.2689034018172));
#205102=CARTESIAN_POINT('Ctrl Pts',(1.6840203735552,-6.5564382305585,88.2771003485259));
#205103=CARTESIAN_POINT('Ctrl Pts',(1.85204403267246,-6.50862672927572,
88.2852972952346));
#205104=CARTESIAN_POINT('Ctrl Pts',(2.02010629445776,-6.46080424351895,
88.2934961251543));
#205105=CARTESIAN_POINT('Ctrl Pts',(2.18627052300146,-6.40648085285346,
88.3016949550741));
#205106=CARTESIAN_POINT('Ctrl Pts',(2.35000820109461,-6.34584513321812,
88.3098937849938));
#205107=CARTESIAN_POINT('Ctrl Pts',(2.513900959701,-6.28515198380467,88.3181003802536));
#205108=CARTESIAN_POINT('Ctrl Pts',(2.67536223929557,-6.21813468550847,
88.3263069755135));
#205109=CARTESIAN_POINT('Ctrl Pts',(2.83388295057802,-6.145030221441,88.3345135707733));
#205110=CARTESIAN_POINT('Ctrl Pts',(2.99248038679347,-6.07189037439384,
88.3427241380723));
#205111=CARTESIAN_POINT('Ctrl Pts',(3.14813409755171,-5.99265765015605,
88.3509347053712));
#205112=CARTESIAN_POINT('Ctrl Pts',(3.30035999983158,-5.90761482084874,
88.3591452726702));
#205113=CARTESIAN_POINT('Ctrl Pts',(3.45279584342336,-5.82245470530509,
88.3673671635169));
#205114=CARTESIAN_POINT('Ctrl Pts',(3.60179412446357,-5.73146865773804,
88.3755890543636));
#205115=CARTESIAN_POINT('Ctrl Pts',(3.74689910053372,-5.63498324136103,
88.3838109452103));
#205116=CARTESIAN_POINT('Ctrl Pts',(3.87883376871325,-5.54725522721139,
88.3912865843652));
#205117=CARTESIAN_POINT('Ctrl Pts',(4.00755002574031,-5.45498147662335,
88.39876222352));
#205118=CARTESIAN_POINT('Ctrl Pts',(4.13272995211434,-5.35843560592987,
88.4062378626748));
#205119=CARTESIAN_POINT('Ctrl Pts',(4.28236274204428,-5.24303029769447,
88.4151738061255));
#205120=CARTESIAN_POINT('Ctrl Pts',(4.42725421261317,-5.12128037415425,
88.4241097495762));
#205121=CARTESIAN_POINT('Ctrl Pts',(4.56688427115261,-4.99358158578579,
88.433045693027));
#205122=CARTESIAN_POINT('Ctrl Pts',(4.7063044286795,-4.86607476256624,88.4419682033846));
#205123=CARTESIAN_POINT('Ctrl Pts',(4.84047876584189,-4.73263709217481,
88.4508907137422));
#205124=CARTESIAN_POINT('Ctrl Pts',(4.96892031122625,-4.59370438107234,
88.4598132240998));
#205125=CARTESIAN_POINT('Ctrl Pts',(5.09704713496527,-4.45511209822695,
88.4687138715382));
#205126=CARTESIAN_POINT('Ctrl Pts',(5.21946902751944,-4.31105183678416,
88.4776145189764));
#205127=CARTESIAN_POINT('Ctrl Pts',(5.33573633219791,-4.161995530183,88.4865151664148));
#205128=CARTESIAN_POINT('Ctrl Pts',(5.45182396010673,-4.01316957170713,
88.495402059001));
#205129=CARTESIAN_POINT('Ctrl Pts',(5.56177581438848,-3.85936317156363,
88.5042889515872));
#205130=CARTESIAN_POINT('Ctrl Pts',(5.6651809466036,-3.70108279321601,88.5131758441734));
#205131=CARTESIAN_POINT('Ctrl Pts',(5.76832028902891,-3.54320925452507,
88.5220398941283));
#205132=CARTESIAN_POINT('Ctrl Pts',(5.86494634674065,-3.38088490018784,
88.5309039440832));
#205133=CARTESIAN_POINT('Ctrl Pts',(5.95469054103665,-3.21464610190433,
88.5397679940381));
#205134=CARTESIAN_POINT('Ctrl Pts',(6.04049321020595,-3.05570843775663,
88.5482427388586));
#205135=CARTESIAN_POINT('Ctrl Pts',(6.12000535808697,-2.89319298766221,
88.5567174836791));
#205136=CARTESIAN_POINT('Ctrl Pts',(6.19294068818319,-2.7275950272438,88.5651922284996));
#205137=CARTESIAN_POINT('Ctrl Pts',(6.26358822935403,-2.56719143805004,
88.5734011429287));
#205138=CARTESIAN_POINT('Ctrl Pts',(6.32799608660961,-2.40404991503855,
88.5816100573578));
#205139=CARTESIAN_POINT('Ctrl Pts',(6.38596282342662,-2.23869779510616,
88.5898189717869));
#205140=CARTESIAN_POINT('Ctrl Pts',(6.44394334154081,-2.07330636354732,
88.5980298378437));
#205141=CARTESIAN_POINT('Ctrl Pts',(6.49547957054619,-1.90570362404628,
88.6062407039005));
#205142=CARTESIAN_POINT('Ctrl Pts',(6.54041966642451,-1.73643300678358,
88.6144515699573));
#205143=CARTESIAN_POINT('Ctrl Pts',(6.58537845734285,-1.56709197309426,
88.6226658517271));
#205144=CARTESIAN_POINT('Ctrl Pts',(6.62373555724049,-1.39608202325226,
88.6308801334969));
#205145=CARTESIAN_POINT('Ctrl Pts',(6.65539001618576,-1.22395781481834,
88.6390944152667));
#205146=CARTESIAN_POINT('Ctrl Pts',(6.68708010472354,-1.05163986699947,
88.6473179428591));
#205147=CARTESIAN_POINT('Ctrl Pts',(6.71205241932193,-0.878205505909337,
88.6555414704515));
#205148=CARTESIAN_POINT('Ctrl Pts',(6.73025765205767,-0.704216541213815,
88.6637649980439));
#205149=CARTESIAN_POINT('Ctrl Pts',(6.74847455363942,-0.530116056360071,
88.6719937965976));
#205150=CARTESIAN_POINT('Ctrl Pts',(6.7599157037378,-0.355460613673461,
88.6802225951513));
#205151=CARTESIAN_POINT('Ctrl Pts',(6.76458392267415,-0.180813033541366,
88.688451393705));
#205152=CARTESIAN_POINT('Ctrl Pts',(6.7692585670403,-0.00592506499107798,
88.6966915185414));
#205153=CARTESIAN_POINT('Ctrl Pts',(6.76714166390616,0.168954664377458,
88.7049316433779));
#205154=CARTESIAN_POINT('Ctrl Pts',(6.75828803461468,0.343266428862604,
88.7131717682143));
#205155=CARTESIAN_POINT('Ctrl Pts',(6.75435738858502,0.420653658713603,
88.7168300435843));
#205156=CARTESIAN_POINT('Ctrl Pts',(6.74909961933731,0.497929046713516,
88.7204883189543));
#205157=CARTESIAN_POINT('Ctrl Pts',(6.74252275698131,0.575044234463026,
88.7241465943243));
#205158=CARTESIAN_POINT('Ctrl Pts',(6.72733486726004,0.753125651402736,
88.7325946170868));
#205159=CARTESIAN_POINT('Ctrl Pts',(6.70507433255718,0.93075961668229,88.7410426398493));
#205160=CARTESIAN_POINT('Ctrl Pts',(6.67578011767778,1.10736119690823,88.7494906626119));
#205161=CARTESIAN_POINT('Ctrl Pts',(6.64651272838582,1.28380105779292,88.7579309492676));
#205162=CARTESIAN_POINT('Ctrl Pts',(6.61022455195311,1.45921009062143,88.7663712359234));
#205163=CARTESIAN_POINT('Ctrl Pts',(6.56700632778351,1.63300853973619,88.7748115225792));
#205164=CARTESIAN_POINT('Ctrl Pts',(6.52382102662986,1.80667459171475,88.7832453795471));
#205165=CARTESIAN_POINT('Ctrl Pts',(6.4737162820617,1.97873218332865,88.791679236515));
#205166=CARTESIAN_POINT('Ctrl Pts',(6.41683395237216,2.14861141849424,88.8001130934829));
#205167=CARTESIAN_POINT('Ctrl Pts',(6.35998621009213,2.31838735826556,88.808541822228));
#205168=CARTESIAN_POINT('Ctrl Pts',(6.29636920474078,2.48598726692218,88.816970550973));
#205169=CARTESIAN_POINT('Ctrl Pts',(6.22617482945705,2.65085570958427,88.825399279718));
#205170=CARTESIAN_POINT('Ctrl Pts',(6.1560123567467,2.81564922134812,88.8338241776983));
#205171=CARTESIAN_POINT('Ctrl Pts',(6.07927860530176,2.97771343617818,88.8422490756786));
#205172=CARTESIAN_POINT('Ctrl Pts',(5.99621400014499,3.13651186263742,88.8506739736589));
#205173=CARTESIAN_POINT('Ctrl Pts',(5.91316778562696,3.29527513086665,88.8590970063531));
#205174=CARTESIAN_POINT('Ctrl Pts',(5.82379366413594,3.45077375588089,88.8675200390473));
#205175=CARTESIAN_POINT('Ctrl Pts',(5.72837875409058,3.60249439273453,88.8759430717414));
#205176=CARTESIAN_POINT('Ctrl Pts',(5.63297464013393,3.7541978625704,88.884365151379));
#205177=CARTESIAN_POINT('Ctrl Pts',(5.53153127772242,3.90212391420367,88.8927872310166));
#205178=CARTESIAN_POINT('Ctrl Pts',(5.42438015879135,4.04578656047384,88.9012093106542));
#205179=CARTESIAN_POINT('Ctrl Pts',(5.31722620639194,4.18945300571098,88.9096316130024));
#205180=CARTESIAN_POINT('Ctrl Pts',(5.20436439622973,4.32885555373081,88.9180539153507));
#205181=CARTESIAN_POINT('Ctrl Pts',(5.08616791855498,4.46353950405528,88.926476217699));
#205182=CARTESIAN_POINT('Ctrl Pts',(4.96795181502739,4.59824581788366,88.9348999185226));
#205183=CARTESIAN_POINT('Ctrl Pts',(4.84439949836761,4.72823172174645,88.9433236193463));
#205184=CARTESIAN_POINT('Ctrl Pts',(4.71592282819866,4.85307746470987,88.9517473201699));
#205185=CARTESIAN_POINT('Ctrl Pts',(4.58735921669263,4.97800769192873,88.9601767213889));
#205186=CARTESIAN_POINT('Ctrl Pts',(4.45386483222662,5.09779057494462,88.9686061226079));
#205187=CARTESIAN_POINT('Ctrl Pts',(4.31588735153932,5.21204426005986,88.9770355238269));
#205188=CARTESIAN_POINT('Ctrl Pts',(4.17786064067857,5.32633871073124,88.9854679326445));
#205189=CARTESIAN_POINT('Ctrl Pts',(4.03534790489707,5.43509982189,88.9939003414622));
#205190=CARTESIAN_POINT('Ctrl Pts',(3.88882839713545,5.53798724245849,89.0023327502798));
#205191=CARTESIAN_POINT('Ctrl Pts',(3.74217332526218,5.64096985746205,89.0107729610074));
#205192=CARTESIAN_POINT('Ctrl Pts',(3.59150435104617,5.73806773708686,89.0192131717351));
#205193=CARTESIAN_POINT('Ctrl Pts',(3.43732901724787,5.82898432209127,89.0276533824627));
#205194=CARTESIAN_POINT('Ctrl Pts',(3.34963671825044,5.88069612422988,89.0324540302998));
#205195=CARTESIAN_POINT('Ctrl Pts',(3.26081053119302,5.93040902174888,89.0372546781368));
#205196=CARTESIAN_POINT('Ctrl Pts',(3.17094717973204,5.97807519050651,89.0420553259739));
#205197=CARTESIAN_POINT('Ctrl Pts',(3.14708018295447,5.99073494865754,89.0433303401437));
#205198=CARTESIAN_POINT('Ctrl Pts',(3.1231325977284,6.0032543053834,89.0446053543134));
#205199=CARTESIAN_POINT('Ctrl Pts',(3.09910619832144,6.01563211736935,89.0458803684832));
#205200=CARTESIAN_POINT('Ctrl Pts',(3.09910619832123,6.01563211736946,87.0457552630241));
#205201=CARTESIAN_POINT('Ctrl Pts',(2.93375330764813,6.1008178731466,87.0545047109265));
#205202=CARTESIAN_POINT('Ctrl Pts',(2.76488627843054,6.17918207037046,87.0632541588287));
#205203=CARTESIAN_POINT('Ctrl Pts',(2.59307866646683,6.25045854554005,87.072003606731));
#205204=CARTESIAN_POINT('Ctrl Pts',(2.42127244185361,6.32173444515043,87.0807529839813));
#205205=CARTESIAN_POINT('Ctrl Pts',(2.24652594672453,6.38592262741842,87.0895023612317));
#205206=CARTESIAN_POINT('Ctrl Pts',(2.06943269687114,6.44280508110564,87.098251738482));
#205207=CARTESIAN_POINT('Ctrl Pts',(1.89234081822068,6.49968709436169,87.1070010479873));
#205208=CARTESIAN_POINT('Ctrl Pts',(1.71290249405577,6.54926340459548,87.1157503574927));
#205209=CARTESIAN_POINT('Ctrl Pts',(1.53172716625045,6.59136563150387,87.124499666998));
#205210=CARTESIAN_POINT('Ctrl Pts',(1.35055318107335,6.63346754640709,87.1332489116653));
#205211=CARTESIAN_POINT('Ctrl Pts',(1.16764249714435,6.66809542395773,87.1419981563325));
#205212=CARTESIAN_POINT('Ctrl Pts',(0.983616340614653,6.69513165624664,
87.1507474009997));
#205213=CARTESIAN_POINT('Ctrl Pts',(0.799591486714114,6.72216769715958,
87.1594965837354));
#205214=CARTESIAN_POINT('Ctrl Pts',(0.614451459526959,6.74161215869369,
87.1682457664711));
#205215=CARTESIAN_POINT('Ctrl Pts',(0.428825047910503,6.75339900185711,
87.1769949492068));
#205216=CARTESIAN_POINT('Ctrl Pts',(0.243199888597404,6.76518576550219,
87.1857440729174));
#205217=CARTESIAN_POINT('Ctrl Pts',(0.0570886373924126,6.76931499599833,
87.1944931966279));
#205218=CARTESIAN_POINT('Ctrl Pts',(-0.128876626810517,6.76577266947848,
87.2032423203384));
#205219=CARTESIAN_POINT('Ctrl Pts',(-0.314840698187495,6.76223036567996,
87.2119913879299));
#205220=CARTESIAN_POINT('Ctrl Pts',(-0.500658497950559,6.75101660879228,
87.2207404555215));
#205221=CARTESIAN_POINT('Ctrl Pts',(-0.685698951925494,6.73216948296226,
87.229489523113));
#205222=CARTESIAN_POINT('Ctrl Pts',(-0.870738280459194,6.71332247176302,
87.2382385374916));
#205223=CARTESIAN_POINT('Ctrl Pts',(-1.05499998761191,6.68684221356196,
87.2469875518701));
#205224=CARTESIAN_POINT('Ctrl Pts',(-1.23785829161367,6.65281863948532,
87.2557365662486));
#205225=CARTESIAN_POINT('Ctrl Pts',(-1.4300741291735,6.61705395368873,87.2649332999478));
#205226=CARTESIAN_POINT('Ctrl Pts',(-1.62073882535738,6.57295372727803,
87.274130033647));
#205227=CARTESIAN_POINT('Ctrl Pts',(-1.80913696091459,6.52068343478295,
87.2833267673462));
#205228=CARTESIAN_POINT('Ctrl Pts',(-1.98838356186048,6.47095219815218,
87.2920767650598));
#205229=CARTESIAN_POINT('Ctrl Pts',(-2.1655782757246,6.41382586850915,87.3008267627735));
#205230=CARTESIAN_POINT('Ctrl Pts',(-2.34011918621618,6.34949849943308,
87.3095767604872));
#205231=CARTESIAN_POINT('Ctrl Pts',(-2.51465655691013,6.28517243495584,
87.3183265807455));
#205232=CARTESIAN_POINT('Ctrl Pts',(-2.6865399629524,6.21364572242412,87.3270764010038));
#205233=CARTESIAN_POINT('Ctrl Pts',(-2.85518555379898,6.13516132252263,
87.3358262212621));
#205234=CARTESIAN_POINT('Ctrl Pts',(-3.02382794858592,6.05667841000555,
87.3445758756996));
#205235=CARTESIAN_POINT('Ctrl Pts',(-3.18923239109178,5.97123819492136,
87.3533255301371));
#205236=CARTESIAN_POINT('Ctrl Pts',(-3.35083705967589,5.87913088810775,
87.3620751845746));
#205237=CARTESIAN_POINT('Ctrl Pts',(-3.51243888042279,5.78702520443176,
87.3708246848236));
#205238=CARTESIAN_POINT('Ctrl Pts',(-3.67024081223559,5.68825280605868,
87.3795741850725));
#205239=CARTESIAN_POINT('Ctrl Pts',(-3.8237068754426,5.58314917682601,87.3883236853214));
#205240=CARTESIAN_POINT('Ctrl Pts',(-3.97717043817686,5.47804726008115,
87.3970730430119));
#205241=CARTESIAN_POINT('Ctrl Pts',(-4.12629803722343,5.36661448084326,
87.4058224007024));
#205242=CARTESIAN_POINT('Ctrl Pts',(-4.27058317206802,5.24922931204663,
87.4145717583928));
#205243=CARTESIAN_POINT('Ctrl Pts',(-4.41486614774747,5.13184589986867,
87.4233209851529));
#205244=CARTESIAN_POINT('Ctrl Pts',(-4.55430658194343,5.00851045723099,
87.432070211913));
#205245=CARTESIAN_POINT('Ctrl Pts',(-4.68843089001791,4.87964187103171,
87.4408194386731));
#205246=CARTESIAN_POINT('Ctrl Pts',(-4.82255336917802,4.75077504207996,
87.449568546129));
#205247=CARTESIAN_POINT('Ctrl Pts',(-4.95135966065118,4.61637541908112,
87.458317653585));
#205248=CARTESIAN_POINT('Ctrl Pts',(-5.07441230869245,4.47689945401844,
87.4670667610409));
#205249=CARTESIAN_POINT('Ctrl Pts',(-5.19746344226383,4.33742520555554,
87.4758157608173));
#205250=CARTESIAN_POINT('Ctrl Pts',(-5.31476088454702,4.19287495491417,
87.4845647605936));
#205251=CARTESIAN_POINT('Ctrl Pts',(-5.42590627628761,4.04373961586831,
87.4933137603699));
#205252=CARTESIAN_POINT('Ctrl Pts',(-5.53706380672581,3.89458798906857,
87.5020637156646));
#205253=CARTESIAN_POINT('Ctrl Pts',(-5.64206777071784,3.74085050155405,
87.5108136709593));
#205254=CARTESIAN_POINT('Ctrl Pts',(-5.74056148163933,3.5830493822328,87.519563626254));
#205255=CARTESIAN_POINT('Ctrl Pts',(-5.83905138951811,3.42525435593406,
87.5283132436951));
#205256=CARTESIAN_POINT('Ctrl Pts',(-5.93103139557581,3.26339625497312,
87.5370628611362));
#205257=CARTESIAN_POINT('Ctrl Pts',(-6.01618907820777,3.09802485065139,
87.5458124785773));
#205258=CARTESIAN_POINT('Ctrl Pts',(-6.1013439254492,2.93265895249773,87.5545618046932));
#205259=CARTESIAN_POINT('Ctrl Pts',(-6.17967677261773,2.76378023986166,
87.5633111308091));
#205260=CARTESIAN_POINT('Ctrl Pts',(-6.2509215700917,2.59196229227245,87.572060456925));
#205261=CARTESIAN_POINT('Ctrl Pts',(-6.32216437407696,2.42014915229239,
87.5808095382274));
#205262=CARTESIAN_POINT('Ctrl Pts',(-6.38631941548862,2.24539720663018,
87.5895586195299));
#205263=CARTESIAN_POINT('Ctrl Pts',(-6.44316881037478,2.06829994947872,
87.5983077008323));
#205264=CARTESIAN_POINT('Ctrl Pts',(-6.50002334524512,1.89118668024652,
87.6070575731746));
#205265=CARTESIAN_POINT('Ctrl Pts',(-6.54957082411038,1.71172794807922,
87.615807445517));
#205266=CARTESIAN_POINT('Ctrl Pts',(-6.59164294296029,1.53053334250576,
87.6245573178593));
#205267=CARTESIAN_POINT('Ctrl Pts',(-6.63371214082084,1.34935131693846,
87.6333065827142));
#205268=CARTESIAN_POINT('Ctrl Pts',(-6.66830695239645,1.1664339383002,87.6420558475691));
#205269=CARTESIAN_POINT('Ctrl Pts',(-6.69530988153949,0.982402458343655,
87.650805112424));
#205270=CARTESIAN_POINT('Ctrl Pts',(-6.72231419690451,0.798361530949721,
87.6595548264311));
#205271=CARTESIAN_POINT('Ctrl Pts',(-6.74172580829254,0.613206671365132,
87.6683045404381));
#205272=CARTESIAN_POINT('Ctrl Pts',(-6.75347878028163,0.427566795116044,
87.6770542544451));
#205273=CARTESIAN_POINT('Ctrl Pts',(-6.76248992368205,0.285234494207813,
87.6837627642334));
#205274=CARTESIAN_POINT('Ctrl Pts',(-6.76699999999992,0.142617266094565,
87.6904712740216));
#205275=CARTESIAN_POINT('Ctrl Pts',(-6.767,3.76450867784256E-12,87.6971797838099));
#205276=CARTESIAN_POINT('',(-6.767,3.91310898614772E-12,87.3028202161898));
#205277=CARTESIAN_POINT('Ctrl Pts',(3.09910619832139,6.01563211736938,86.6514537215909));
#205278=CARTESIAN_POINT('Ctrl Pts',(2.94383374465635,6.09562467911404,86.6596510417769));
#205279=CARTESIAN_POINT('Ctrl Pts',(2.78541012641986,6.16962848848196,86.6678483619629));
#205280=CARTESIAN_POINT('Ctrl Pts',(2.62433993952006,6.23739760491824,86.6760456821488));
#205281=CARTESIAN_POINT('Ctrl Pts',(2.46328560259829,6.30516005259089,86.6842421956843));
#205282=CARTESIAN_POINT('Ctrl Pts',(2.29958554603934,6.36668888949535,86.6924387092198));
#205283=CARTESIAN_POINT('Ctrl Pts',(2.13376513616885,6.42178599329426,86.7006352227552));
#205284=CARTESIAN_POINT('Ctrl Pts',(1.96793089327903,6.47688769338684,86.7088324200578));
#205285=CARTESIAN_POINT('Ctrl Pts',(1.79997628520236,6.5255564784604,86.7170296173603));
#205286=CARTESIAN_POINT('Ctrl Pts',(1.63044270444559,6.56764383835788,86.7252268146628));
#205287=CARTESIAN_POINT('Ctrl Pts',(1.46086415536567,6.60974236181358,86.7334261862497));
#205288=CARTESIAN_POINT('Ctrl Pts',(1.28970614750773,6.64525589676282,86.7416255578366));
#205289=CARTESIAN_POINT('Ctrl Pts',(1.11752120001407,6.67408685645603,86.7498249294235));
#205290=CARTESIAN_POINT('Ctrl Pts',(0.945170491246863,6.70294557151733,
86.7580321944895));
#205291=CARTESIAN_POINT('Ctrl Pts',(0.771791222117369,6.72510880078116,
86.7662394595554));
#205292=CARTESIAN_POINT('Ctrl Pts',(0.597942898001018,6.74053063866118,
86.7744467246214));
#205293=CARTESIAN_POINT('Ctrl Pts',(0.424004893424784,6.75596043196741,
86.7826582234429));
#205294=CARTESIAN_POINT('Ctrl Pts',(0.249597709372894,6.76464188321101,
86.7908697222644));
#205295=CARTESIAN_POINT('Ctrl Pts',(0.0752817218204754,6.76658123887978,
86.7990812210859));
#205296=CARTESIAN_POINT('Ctrl Pts',(-0.0992660794267649,6.76852317359599,
86.8073036399493));
#205297=CARTESIAN_POINT('Ctrl Pts',(-0.27372208355303,6.76370510835888,
86.8155260588126));
#205298=CARTESIAN_POINT('Ctrl Pts',(-0.447529064371234,6.7521853304351,
86.823748477676));
#205299=CARTESIAN_POINT('Ctrl Pts',(-0.57165930965902,6.74395808402298,
86.8296208014777));
#205300=CARTESIAN_POINT('Ctrl Pts',(-0.695458615619168,6.73231365799035,
86.8354931252795));
#205301=CARTESIAN_POINT('Ctrl Pts',(-0.818727194630302,6.71728924349494,
86.8413654490812));
#205302=CARTESIAN_POINT('Ctrl Pts',(-1.00630558582367,6.69442651949601,
86.850301392532));
#205303=CARTESIAN_POINT('Ctrl Pts',(-1.19304528443073,6.66368782905504,
86.8592373359827));
#205304=CARTESIAN_POINT('Ctrl Pts',(-1.37829705002254,6.62514801660304,
86.8681732794335));
#205305=CARTESIAN_POINT('Ctrl Pts',(-1.56327033307593,6.58666613971115,
86.8770957897911));
#205306=CARTESIAN_POINT('Ctrl Pts',(-1.7467598940025,6.54040659298026,86.8860183001487));
#205307=CARTESIAN_POINT('Ctrl Pts',(-1.92812452835058,6.48649557181479,
86.8949408105064));
#205308=CARTESIAN_POINT('Ctrl Pts',(-2.10904476306238,6.43271664938115,
86.9038414579448));
#205309=CARTESIAN_POINT('Ctrl Pts',(-2.28785021585018,6.37132374460046,
86.9127421053832));
#205310=CARTESIAN_POINT('Ctrl Pts',(-2.46391332976258,6.30249316567803,
86.9216427528216));
#205311=CARTESIAN_POINT('Ctrl Pts',(-2.63970435986028,6.23376895592098,
86.9305296454077));
#205312=CARTESIAN_POINT('Ctrl Pts',(-2.81276126539432,6.15763009309876,
86.9394165379939));
#205313=CARTESIAN_POINT('Ctrl Pts',(-2.98247215036693,6.07430233625934,
86.9483034305801));
#205314=CARTESIAN_POINT('Ctrl Pts',(-3.15174681501544,5.9911887628596,86.9571674805351));
#205315=CARTESIAN_POINT('Ctrl Pts',(-3.31769238976927,5.90092328075294,
86.96603153049));
#205316=CARTESIAN_POINT('Ctrl Pts',(-3.47971814726007,5.80377899438193,
86.974895580445));
#205317=CARTESIAN_POINT('Ctrl Pts',(-3.63462780549006,5.71090124189506,
86.9833703252653));
#205318=CARTESIAN_POINT('Ctrl Pts',(-3.78595431431762,5.61173602165759,
86.9918450700856));
#205319=CARTESIAN_POINT('Ctrl Pts',(-3.93319867912149,5.50656309784579,
87.0003198149059));
#205320=CARTESIAN_POINT('Ctrl Pts',(-4.07582437658705,5.40468917123996,
87.008528729335));
#205321=CARTESIAN_POINT('Ctrl Pts',(-4.21448195710526,5.29727593196517,
87.0167376437641));
#205322=CARTESIAN_POINT('Ctrl Pts',(-4.34872903395071,5.18467402922056,
87.0249465581932));
#205323=CARTESIAN_POINT('Ctrl Pts',(-4.48300802735684,5.07204535594547,
87.03315742425));
#205324=CARTESIAN_POINT('Ctrl Pts',(-4.6128741552097,4.95422579040202,87.0413682903068));
#205325=CARTESIAN_POINT('Ctrl Pts',(-4.7379194619536,4.83160513411861,87.0495791563636));
#205326=CARTESIAN_POINT('Ctrl Pts',(-4.8630167874318,4.70893346775331,87.0577934381333));
#205327=CARTESIAN_POINT('Ctrl Pts',(-4.98328904247643,4.58145698081226,
87.0660077199029));
#205328=CARTESIAN_POINT('Ctrl Pts',(-5.09836630564968,4.44960110722479,
87.0742220016726));
#205329=CARTESIAN_POINT('Ctrl Pts',(-5.21357309736919,4.31759681944019,
87.082445529265));
#205330=CARTESIAN_POINT('Ctrl Pts',(-5.32357298385505,4.18120356786216,
87.0906690568573));
#205331=CARTESIAN_POINT('Ctrl Pts',(-5.42803680107344,4.04087929616716,
87.0988925844497));
#205332=CARTESIAN_POINT('Ctrl Pts',(-5.53256757553528,3.90046508207229,
87.1071213830034));
#205333=CARTESIAN_POINT('Ctrl Pts',(-5.63155500635019,3.75611511803967,
87.1153501815571));
#205334=CARTESIAN_POINT('Ctrl Pts',(-5.72471423974431,3.60831482457791,
87.1235789801108));
#205335=CARTESIAN_POINT('Ctrl Pts',(-5.81800169936844,3.46031109583945,
87.1318191049472));
#205336=CARTESIAN_POINT('Ctrl Pts',(-5.905444760755,3.30884785924964,87.1400592297836));
#205337=CARTESIAN_POINT('Ctrl Pts',(-5.98680486650131,3.15443441688621,
87.14829935462));
#205338=CARTESIAN_POINT('Ctrl Pts',(-6.0229253958474,3.08588122087992,87.1519576299902));
#205339=CARTESIAN_POINT('Ctrl Pts',(-6.05784761721732,3.01674679976217,
87.1556159053605));
#205340=CARTESIAN_POINT('Ctrl Pts',(-6.0915537524103,2.94707683671396,87.1592741807307));
#205341=CARTESIAN_POINT('Ctrl Pts',(-6.1759339152134,2.77266458829585,87.1684323315999));
#205342=CARTESIAN_POINT('Ctrl Pts',(-6.25285077445145,2.59456200883916,
87.1775904824692));
#205343=CARTESIAN_POINT('Ctrl Pts',(-6.32201145009694,2.41339185066229,
87.1867486333385));
#205344=CARTESIAN_POINT('Ctrl Pts',(-6.39107338526958,2.2324803485341,87.1958937091454));
#205345=CARTESIAN_POINT('Ctrl Pts',(-6.45240116500455,2.04851021229947,
87.2050387849522));
#205346=CARTESIAN_POINT('Ctrl Pts',(-6.50574998604927,1.86212408797588,
87.2141838607591));
#205347=CARTESIAN_POINT('Ctrl Pts',(-6.55895794440002,1.67623009920609,
87.2233047898278));
#205348=CARTESIAN_POINT('Ctrl Pts',(-6.60422893723639,1.48793306383961,
87.2324257188965));
#205349=CARTESIAN_POINT('Ctrl Pts',(-6.64136810965814,1.29789006931091,
87.2415466479652));
#205350=CARTESIAN_POINT('Ctrl Pts',(-6.67843688274809,1.10820731166839,
87.2506502878142));
#205351=CARTESIAN_POINT('Ctrl Pts',(-6.70740454900505,0.916785410033402,
87.2597539276632));
#205352=CARTESIAN_POINT('Ctrl Pts',(-6.72812655419379,0.724294187987466,
87.2688575675122));
#205353=CARTESIAN_POINT('Ctrl Pts',(-6.74878566459043,0.532387209371671,
87.2779335762738));
#205354=CARTESIAN_POINT('Ctrl Pts',(-6.76124902294262,0.339417601311186,
87.2870095850354));
#205355=CARTESIAN_POINT('Ctrl Pts',(-6.76542347337597,0.146062404106671,
87.2960855937971));
#205356=CARTESIAN_POINT('Ctrl Pts',(-6.76645598844231,0.0982376287365919,
87.298330467928));
#205357=CARTESIAN_POINT('Ctrl Pts',(-6.76698164913032,0.0503893190892879,
87.3005753420589));
#205358=CARTESIAN_POINT('Ctrl Pts',(-6.76699952786402,0.00252782281982319,
87.3028202161898));
#205359=CARTESIAN_POINT('Ctrl Pts',(-6.767,3.91310882501737E-12,87.3028202161898));
#205360=CARTESIAN_POINT('Ctrl Pts',(-6.76700000000011,-0.186007249523053,
87.311569728001));
#205361=CARTESIAN_POINT('Ctrl Pts',(-6.75932637294541,-0.372014355746198,
87.3203192398122));
#205362=CARTESIAN_POINT('Ctrl Pts',(-6.7440051826421,-0.557389537483875,
87.3290687516234));
#205363=CARTESIAN_POINT('Ctrl Pts',(-6.72868405705124,-0.742763936248352,
87.337818226479));
#205364=CARTESIAN_POINT('Ctrl Pts',(-6.7057154564577,-0.927506130239004,
87.3465677013347));
#205365=CARTESIAN_POINT('Ctrl Pts',(-6.67517739404852,-1.11098863989852,
87.3553171761904));
#205366=CARTESIAN_POINT('Ctrl Pts',(-6.6446394580873,-1.29447038981804,
87.3640666148174));
#205367=CARTESIAN_POINT('Ctrl Pts',(-6.60653217008382,-1.47669218313562,
87.3728160534445));
#205368=CARTESIAN_POINT('Ctrl Pts',(-6.56098496092703,-1.65703510599185,
87.3815654920715));
#205369=CARTESIAN_POINT('Ctrl Pts',(-6.51543793658326,-1.83737729708595,
87.3903148951966));
#205370=CARTESIAN_POINT('Ctrl Pts',(-6.46245112167454,-2.01584035510818,
87.3990642983218));
#205371=CARTESIAN_POINT('Ctrl Pts',(-6.40220448374292,-2.1918181376068,
87.407813701447));
#205372=CARTESIAN_POINT('Ctrl Pts',(-6.34195808526543,-2.36779522067039,
87.4165630697971));
#205373=CARTESIAN_POINT('Ctrl Pts',(-6.27445201433143,-2.54128677684068,
87.4253124381472));
#205374=CARTESIAN_POINT('Ctrl Pts',(-6.19991555071942,-2.71170355384721,
87.4340618064973));
#205375=CARTESIAN_POINT('Ctrl Pts',(-6.12537937716736,-2.88211966767384,
87.442811140799));
#205376=CARTESIAN_POINT('Ctrl Pts',(-6.04381298052568,-3.0494607637169,
87.4515604751008));
#205377=CARTESIAN_POINT('Ctrl Pts',(-5.95549339335884,-3.2131584837445,
87.4603098094026));
#205378=CARTESIAN_POINT('Ctrl Pts',(-5.86717414255468,-3.37685558033391,
87.4690591103828));
#205379=CARTESIAN_POINT('Ctrl Pts',(-5.77210188876663,-3.5369090764665,
87.477808411363));
#205380=CARTESIAN_POINT('Ctrl Pts',(-5.67059953347068,-3.69277536969176,
87.4865577123431));
#205381=CARTESIAN_POINT('Ctrl Pts',(-5.56909755631467,-3.84864108224802,
87.4953069807284));
#205382=CARTESIAN_POINT('Ctrl Pts',(-5.46116568196946,-4.00031938297385,
87.5040562491137));
#205383=CARTESIAN_POINT('Ctrl Pts',(-5.34717048533713,-4.14729511859712,
87.512805517499));
#205384=CARTESIAN_POINT('Ctrl Pts',(-5.23317570391972,-4.29427031887749,
87.521554754016));
#205385=CARTESIAN_POINT('Ctrl Pts',(-5.11311782003678,-4.43654276189357,
87.530303990533));
#205386=CARTESIAN_POINT('Ctrl Pts',(-4.98740458984947,-4.57362924351641,
87.5390532270501));
#205387=CARTESIAN_POINT('Ctrl Pts',(-4.86169180711949,-4.71071523720054,
87.5478024324255));
#205388=CARTESIAN_POINT('Ctrl Pts',(-4.73032391204389,-4.84261509523025,
87.5565516378009));
#205389=CARTESIAN_POINT('Ctrl Pts',(-4.59374707013829,-4.96888084538117,
87.5653008431764));
#205390=CARTESIAN_POINT('Ctrl Pts',(-4.45717070301705,-5.09514615659235,
87.5740500181368));
#205391=CARTESIAN_POINT('Ctrl Pts',(-4.31538563571333,-5.21577720459284,
87.5827991930972));
#205392=CARTESIAN_POINT('Ctrl Pts',(-4.16887341029835,-5.33036429232631,
87.5915483680576));
#205393=CARTESIAN_POINT('Ctrl Pts',(-4.02236168204043,-5.44495099123367,
87.6002975133297));
#205394=CARTESIAN_POINT('Ctrl Pts',(-3.87112305348512,-5.5534935943836,
87.6090466586017));
#205395=CARTESIAN_POINT('Ctrl Pts',(-3.71567117018118,-5.65562346298659,
87.6177958038737));
#205396=CARTESIAN_POINT('Ctrl Pts',(-3.56021980146173,-5.75775299351426,
87.6265449201839));
#205397=CARTESIAN_POINT('Ctrl Pts',(-3.40055544538699,-5.8534696746367,
87.635294036494));
#205398=CARTESIAN_POINT('Ctrl Pts',(-3.23722035987199,-5.94244842986713,
87.6440431528042));
#205399=CARTESIAN_POINT('Ctrl Pts',(-3.07388580147527,-6.03142689794352,
87.6527922408791));
#205400=CARTESIAN_POINT('Ctrl Pts',(-2.90688078896926,-6.11366734656616,
87.6615413289539));
#205401=CARTESIAN_POINT('Ctrl Pts',(-2.73677250721718,-6.188890469522,87.6702904170288));
#205402=CARTESIAN_POINT('Ctrl Pts',(-2.56666476031827,-6.26411335596186,
87.6790394775948));
#205403=CARTESIAN_POINT('Ctrl Pts',(-2.39345402575506,-6.33231884500427,
87.6877885381608));
#205404=CARTESIAN_POINT('Ctrl Pts',(-2.21772856065927,-6.39327529762611,
87.6965375987268));
#205405=CARTESIAN_POINT('Ctrl Pts',(-2.04200363348862,-6.45423156365,87.7052866325105));
#205406=CARTESIAN_POINT('Ctrl Pts',(-1.8637642618964,-6.50793874375554,
87.7140356662942));
#205407=CARTESIAN_POINT('Ctrl Pts',(-1.68361577753529,-6.55421443909446,
87.7227847000779));
#205408=CARTESIAN_POINT('Ctrl Pts',(-1.50346782968192,-6.60048999661778,
87.7315337078057));
#205409=CARTESIAN_POINT('Ctrl Pts',(-1.32141105795398,-6.6393340423763,
87.7402827155336));
#205410=CARTESIAN_POINT('Ctrl Pts',(-1.13806375487451,-6.67061465607488,
87.7490317232614));
#205411=CARTESIAN_POINT('Ctrl Pts',(-0.954716982608237,-6.70189517921219,
87.7577807056598));
#205412=CARTESIAN_POINT('Ctrl Pts',(-0.770079968908298,-6.72561226592155,
87.7665296880581));
#205413=CARTESIAN_POINT('Ctrl Pts',(-0.584779765565347,-6.74168536983041,
87.7752786704565));
#205414=CARTESIAN_POINT('Ctrl Pts',(-0.391489830658313,-6.75845151013813,
87.7844048894664));
#205415=CARTESIAN_POINT('Ctrl Pts',(-0.197478578245256,-6.76689983031605,
87.7935311084762));
#205416=CARTESIAN_POINT('Ctrl Pts',(-0.00346287645816003,-6.76699911397117,
87.8026573274861));
#205417=CARTESIAN_POINT('Ctrl Pts',(0.184489834648061,-6.76709529501207,
87.8114983521519));
#205418=CARTESIAN_POINT('Ctrl Pts',(0.372446404243646,-6.759356397382,87.8203393768177));
#205419=CARTESIAN_POINT('Ctrl Pts',(0.559755019482719,-6.74380925873233,
87.8291804014835));
#205420=CARTESIAN_POINT('Ctrl Pts',(0.745134705516256,-6.72842222659867,
87.8379303800933));
#205421=CARTESIAN_POINT('Ctrl Pts',(0.929879431223152,-6.70538706057599,
87.846680358703));
#205422=CARTESIAN_POINT('Ctrl Pts',(1.11336163626295,-6.67478200894216,
87.8554303373128));
#205423=CARTESIAN_POINT('Ctrl Pts',(1.29684196300207,-6.64417727061113,
87.8641802263493));
#205424=CARTESIAN_POINT('Ctrl Pts',(1.47905951217019,-6.60600284890701,
87.8729301153858));
#205425=CARTESIAN_POINT('Ctrl Pts',(1.65939532066612,-6.5603884160735,87.8816800044224));
#205426=CARTESIAN_POINT('Ctrl Pts',(1.83972934300345,-6.51477443503386,
87.8904298067945));
#205427=CARTESIAN_POINT('Ctrl Pts',(2.01818138405824,-6.46172066062279,
87.8991796091667));
#205428=CARTESIAN_POINT('Ctrl Pts',(2.19414528353774,-6.40140730423624,
87.9079294115389));
#205429=CARTESIAN_POINT('Ctrl Pts',(2.37010749863578,-6.341094525188,87.9166791301552));
#205430=CARTESIAN_POINT('Ctrl Pts',(2.54358134866041,-6.27352239616673,
87.9254288487715));
#205431=CARTESIAN_POINT('Ctrl Pts',(2.71397759435142,-6.19892043967,87.9341785673878));
#205432=CARTESIAN_POINT('Ctrl Pts',(2.88437226557709,-6.1243191724971,87.9429282051565));
#205433=CARTESIAN_POINT('Ctrl Pts',(3.05168912680541,-6.04268832279008,
87.9516778429252));
#205434=CARTESIAN_POINT('Ctrl Pts',(3.2153598627344,-5.95430516123558,87.9604274806939));
#205435=CARTESIAN_POINT('Ctrl Pts',(3.3790291407245,-5.86592278697667,87.969177040523));
#205436=CARTESIAN_POINT('Ctrl Pts',(3.53905210621203,-5.77078835742169,
87.9779266003521));
#205437=CARTESIAN_POINT('Ctrl Pts',(3.6948852283135,-5.66922500431856,87.9866761601812));
#205438=CARTESIAN_POINT('Ctrl Pts',(3.85071701406603,-5.56766252217326,
87.9954256449783));
#205439=CARTESIAN_POINT('Ctrl Pts',(4.00235878822078,-5.45967138329609,
88.0041751297754));
#205440=CARTESIAN_POINT('Ctrl Pts',(4.14929549611011,-5.34561838199851,
88.0129246145725));
#205441=CARTESIAN_POINT('Ctrl Pts',(4.29623099275787,-5.23156632087264,
88.0216740272451));
#205442=CARTESIAN_POINT('Ctrl Pts',(4.43846127435738,-5.11145267305216,
88.0304234399177));
#205443=CARTESIAN_POINT('Ctrl Pts',(4.57550326054164,-4.9856854005014,88.0391728525903));
#205444=CARTESIAN_POINT('Ctrl Pts',(4.71254416257516,-4.85991912290617,
88.0479221960455));
#205445=CARTESIAN_POINT('Ctrl Pts',(4.8443966401851,-4.72849950385677,88.0566715395008));
#205446=CARTESIAN_POINT('Ctrl Pts',(4.97061286794506,-4.59187289861326,
88.065420882956));
#205447=CARTESIAN_POINT('Ctrl Pts',(5.09682813912455,-4.45524732884947,
88.0741701601009));
#205448=CARTESIAN_POINT('Ctrl Pts',(5.21740705147619,-4.31341506236053,
88.0829194372457));
#205449=CARTESIAN_POINT('Ctrl Pts',(5.33194007545486,-4.16685781275992,
88.0916687143905));
#205450=CARTESIAN_POINT('Ctrl Pts',(5.44647226944278,-4.02030162522122,
88.1004179281316));
#205451=CARTESIAN_POINT('Ctrl Pts',(5.55495848627908,-3.86902074888228,
88.1091671418728));
#205452=CARTESIAN_POINT('Ctrl Pts',(5.65703027291587,-3.71352898080969,
88.1179163556139));
#205453=CARTESIAN_POINT('Ctrl Pts',(5.75910135376803,-3.55803828789902,
88.1266655088578));
#205454=CARTESIAN_POINT('Ctrl Pts',(5.85475793592566,-3.39833700107034,
88.1354146621017));
#205455=CARTESIAN_POINT('Ctrl Pts',(5.9436751442722,-3.23496750823882,88.1441638153455));
#205456=CARTESIAN_POINT('Ctrl Pts',(6.03259176732475,-3.0715990907805,88.1529129109985));
#205457=CARTESIAN_POINT('Ctrl Pts',(6.11476896835772,-2.90456276731755,
88.1616620066514));
#205458=CARTESIAN_POINT('Ctrl Pts',(6.18992765547747,-2.73442583003366,
88.1704111023043));
#205459=CARTESIAN_POINT('Ctrl Pts',(6.26508587282926,-2.56428995616483,
88.1791601432724));
#205460=CARTESIAN_POINT('Ctrl Pts',(6.33322554827043,-2.39105376935511,
88.1879091842404));
#205461=CARTESIAN_POINT('Ctrl Pts',(6.39411526732925,-2.21530561054385,
88.1966582252084));
#205462=CARTESIAN_POINT('Ctrl Pts',(6.45500462602747,-2.03955849185415,
88.2054072143975));
#205463=CARTESIAN_POINT('Ctrl Pts',(6.50864402040646,-1.86129970164872,
88.2141562035865));
#205464=CARTESIAN_POINT('Ctrl Pts',(6.55485128368514,-1.68113463136397,
88.2229051927755));
#205465=CARTESIAN_POINT('Ctrl Pts',(6.60199809554247,-1.49730620117218,
88.231832078247));
#205466=CARTESIAN_POINT('Ctrl Pts',(6.64140720707802,-1.31149343246059,
88.2407589637184));
#205467=CARTESIAN_POINT('Ctrl Pts',(6.67293928722821,-1.12435326697897,
88.2496858491898));
#205468=CARTESIAN_POINT('Ctrl Pts',(6.70384625876204,-0.940923067010339,
88.2584357633673));
#205469=CARTESIAN_POINT('Ctrl Pts',(6.72718554579753,-0.75621789952545,
88.2671856775447));
#205470=CARTESIAN_POINT('Ctrl Pts',(6.74287786815295,-0.570865181258313,
88.2759355917222));
#205471=CARTESIAN_POINT('Ctrl Pts',(6.75856988190823,-0.38551610807784,
88.2846853338267));
#205472=CARTESIAN_POINT('Ctrl Pts',(6.76661520773391,-0.199519795230314,
88.2934350759312));
#205473=CARTESIAN_POINT('Ctrl Pts',(6.76698651789578,-0.0135080204596825,
88.3021848180356));
#205474=CARTESIAN_POINT('Ctrl Pts',(6.76735782124913,0.172500343508857,
88.3109343997006));
#205475=CARTESIAN_POINT('Ctrl Pts',(6.76005538995206,0.358523882206753,
88.3196839813656));
#205476=CARTESIAN_POINT('Ctrl Pts',(6.74510402742395,0.543930748560149,
88.3284335630305));
#205477=CARTESIAN_POINT('Ctrl Pts',(6.73015291918077,0.729334461610889,
88.3371829958872));
#205478=CARTESIAN_POINT('Ctrl Pts',(6.70755316306655,0.914121237630222,
88.3459324287439));
#205479=CARTESIAN_POINT('Ctrl Pts',(6.67738151874649,1.09766345165665,88.3546818616006));
#205480=CARTESIAN_POINT('Ctrl Pts',(6.64721034747657,1.2812027879921,88.3634311572781));
#205481=CARTESIAN_POINT('Ctrl Pts',(6.60946757205242,1.46349731859877,88.3721804529556));
#205482=CARTESIAN_POINT('Ctrl Pts',(6.56428138111635,1.64392790277714,88.3809297486332));
#205483=CARTESIAN_POINT('Ctrl Pts',(6.51909583859976,1.82435589778607,88.3896789187587));
#205484=CARTESIAN_POINT('Ctrl Pts',(6.46646716393014,2.00291972191816,88.3984280888844));
#205485=CARTESIAN_POINT('Ctrl Pts',(6.40657409873036,2.17901292274215,88.40717725901));
#205486=CARTESIAN_POINT('Ctrl Pts',(6.34668181342242,2.35510383058531,88.4159263152091));
#205487=CARTESIAN_POINT('Ctrl Pts',(6.27952541914228,2.52872390822137,88.4246753714082));
#205488=CARTESIAN_POINT('Ctrl Pts',(6.20533299175708,2.69928350889846,88.4334244276073));
#205489=CARTESIAN_POINT('Ctrl Pts',(6.12831602991743,2.8763363796521,88.4425065637655));
#205490=CARTESIAN_POINT('Ctrl Pts',(6.04371690605466,3.05009086601076,88.4515886999237));
#205491=CARTESIAN_POINT('Ctrl Pts',(5.95184520316826,3.21991112882374,88.4606708360819));
#205492=CARTESIAN_POINT('Ctrl Pts',(5.86333549509478,3.38351691182665,88.4694206164255));
#205493=CARTESIAN_POINT('Ctrl Pts',(5.7680761809958,3.54347103711661,88.478170396769));
#205494=CARTESIAN_POINT('Ctrl Pts',(5.66639083309234,3.69923018027361,88.4869201771126));
#205495=CARTESIAN_POINT('Ctrl Pts',(5.56470914082432,3.85498372381716,88.4956696428975));
#205496=CARTESIAN_POINT('Ctrl Pts',(5.45660203372311,4.00654234701665,88.5044191086824));
#205497=CARTESIAN_POINT('Ctrl Pts',(5.34243669839474,4.15339127986338,88.5131685744673));
#205498=CARTESIAN_POINT('Ctrl Pts',(5.2282748605086,4.30023571400953,88.5219177722133));
#205499=CARTESIAN_POINT('Ctrl Pts',(5.10805534167391,4.44237052028148,88.5306669699593));
#205500=CARTESIAN_POINT('Ctrl Pts',(4.98218644340242,4.57931296628404,88.5394161677053));
#205501=CARTESIAN_POINT('Ctrl Pts',(4.85632073219883,4.71625194483055,88.548165143917));
#205502=CARTESIAN_POINT('Ctrl Pts',(4.72480612170621,4.84799861524214,88.5569141201286));
#205503=CARTESIAN_POINT('Ctrl Pts',(4.58808925235619,4.97410554898201,88.5656630963402));
#205504=CARTESIAN_POINT('Ctrl Pts',(4.45136349474367,5.10022068120928,88.574412641342));
#205505=CARTESIAN_POINT('Ctrl Pts',(4.30943501210409,5.22069514871562,88.5831621863436));
#205506=CARTESIAN_POINT('Ctrl Pts',(4.16278587432121,5.33511975165992,88.5919117313453));
#205507=CARTESIAN_POINT('Ctrl Pts',(4.01614535740789,5.44953762807591,88.6006607619991));
#205508=CARTESIAN_POINT('Ctrl Pts',(3.86478496658266,5.55790617532546,88.6094097926528));
#205509=CARTESIAN_POINT('Ctrl Pts',(3.70921874747539,5.65985735539131,88.6181588233065));
#205510=CARTESIAN_POINT('Ctrl Pts',(3.55365041606255,5.76180991976828,88.6269079727562));
#205511=CARTESIAN_POINT('Ctrl Pts',(3.39387638174887,5.85734478552602,88.6356571222058));
#205512=CARTESIAN_POINT('Ctrl Pts',(3.23043927904913,5.94613749121029,88.6444062716554));
#205513=CARTESIAN_POINT('Ctrl Pts',(3.18691767070677,5.96978206944017,88.6467360795716));
#205514=CARTESIAN_POINT('Ctrl Pts',(3.14313645919747,5.99294880633365,88.6490658874879));
#205515=CARTESIAN_POINT('Ctrl Pts',(3.09910619832125,6.01563211736945,88.6513956954041));
#205516=CARTESIAN_POINT('Origin',(0.,0.,4.30282021618968));
#205517=CARTESIAN_POINT('',(3.09910619832119,6.01563211736948,91.0458502363996));
#205518=CARTESIAN_POINT('',(3.09910619832126,6.01563211736944,90.6515218032501));
#205519=CARTESIAN_POINT('',(3.09910619832133,6.0156321173694,4.30282021618968));
#205520=CARTESIAN_POINT('',(-6.76699986371212,0.00135813113412233,89.6971797838355));
#205521=CARTESIAN_POINT('Ctrl Pts',(-6.76699986371212,0.00135813113412683,
89.6971797838355));
#205522=CARTESIAN_POINT('Ctrl Pts',(-6.76703500186648,-0.173720607425384,
89.7054399898427));
#205523=CARTESIAN_POINT('Ctrl Pts',(-6.7602712822433,-0.348979168962801,
89.71370019585));
#205524=CARTESIAN_POINT('Ctrl Pts',(-6.74669303449373,-0.523853126662233,
89.7219604018572));
#205525=CARTESIAN_POINT('Ctrl Pts',(-6.7331260173862,-0.698582445166926,
89.7302137758035));
#205526=CARTESIAN_POINT('Ctrl Pts',(-6.71275572688528,-0.872927442307335,
89.7384671497498));
#205527=CARTESIAN_POINT('Ctrl Pts',(-6.68561853810828,-1.04632392828553,
89.746720523696));
#205528=CARTESIAN_POINT('Ctrl Pts',(-6.65849853992186,-1.21961057281989,
89.7549686693788));
#205529=CARTESIAN_POINT('Ctrl Pts',(-6.62462023809079,-1.39194955459326,
89.7632168150617));
#205530=CARTESIAN_POINT('Ctrl Pts',(-6.58407182212003,-1.56278189174469,
89.7714649607445));
#205531=CARTESIAN_POINT('Ctrl Pts',(-6.54354124270484,-1.73353908266899,
89.7797094782089));
#205532=CARTESIAN_POINT('Ctrl Pts',(-6.49634647718534,-1.90279060574003,
89.7879539956732));
#205533=CARTESIAN_POINT('Ctrl Pts',(-6.44262681568658,-2.06998761199101,
89.7961985131377));
#205534=CARTESIAN_POINT('Ctrl Pts',(-6.3884416573607,-2.23863342997576,
89.8045144717954));
#205535=CARTESIAN_POINT('Ctrl Pts',(-6.32761805760378,-2.40518859796871,
89.812830430453));
#205536=CARTESIAN_POINT('Ctrl Pts',(-6.26035054698763,-2.5691049081016,
89.8211463891107));
#205537=CARTESIAN_POINT('Ctrl Pts',(-6.19366655536911,-2.73159930920131,
89.8293902101226));
#205538=CARTESIAN_POINT('Ctrl Pts',(-6.12065017010656,-2.89150013206863,
89.8376340311344));
#205539=CARTESIAN_POINT('Ctrl Pts',(-6.0415394290993,-3.04829301850045,
89.8458778521462));
#205540=CARTESIAN_POINT('Ctrl Pts',(-5.9624154888514,-3.20511206505934,
89.8541230485993));
#205541=CARTESIAN_POINT('Ctrl Pts',(-5.87719532613465,-3.35882182562928,
89.8623682450523));
#205542=CARTESIAN_POINT('Ctrl Pts',(-5.78616317349773,-3.50893213523127,
89.8706134415054));
#205543=CARTESIAN_POINT('Ctrl Pts',(-5.69509985964289,-3.65909382909624,
89.8788614603719));
#205544=CARTESIAN_POINT('Ctrl Pts',(-5.59822077542912,-3.80565331434493,
89.8871094792383));
#205545=CARTESIAN_POINT('Ctrl Pts',(-5.49585379998729,-3.94814893452176,
89.8953574981047));
#205546=CARTESIAN_POINT('Ctrl Pts',(-5.39198942920089,-4.09272894057942,
89.9037261666729));
#205547=CARTESIAN_POINT('Ctrl Pts',(-5.28247558541717,-4.23312495718327,
89.912094835241));
#205548=CARTESIAN_POINT('Ctrl Pts',(-5.16769692743683,-4.36888972922869,
89.9204635038092));
#205549=CARTESIAN_POINT('Ctrl Pts',(-5.05437929604085,-4.50292634078969,
89.9287256469355));
#205550=CARTESIAN_POINT('Ctrl Pts',(-4.93593037606399,-4.63244869562128,
89.9369877900618));
#205551=CARTESIAN_POINT('Ctrl Pts',(-4.81275718074231,-4.75706393894525,
89.9452499331881));
#205552=CARTESIAN_POINT('Ctrl Pts',(-4.68720184094805,-4.88408921565603,
89.9536718644772));
#205553=CARTESIAN_POINT('Ctrl Pts',(-4.5567379217822,-5.00601537902839,
89.9620937957663));
#205554=CARTESIAN_POINT('Ctrl Pts',(-4.42183123249962,-5.12246986826579,
89.9705157270554));
#205555=CARTESIAN_POINT('Ctrl Pts',(-4.28692454321713,-5.2389243575031,
89.9789376583444));
#205556=CARTESIAN_POINT('Ctrl Pts',(-4.14757542056657,-5.34990697991828,
89.9873595896335));
#205557=CARTESIAN_POINT('Ctrl Pts',(-4.00427986530766,-5.45509227788969,
89.9957815209225));
#205558=CARTESIAN_POINT('Ctrl Pts',(-3.8669748904592,-5.55588022393795,
90.0038513669253));
#205559=CARTESIAN_POINT('Ctrl Pts',(-3.72560857413471,-5.65166688119633,
90.0119212129281));
#205560=CARTESIAN_POINT('Ctrl Pts',(-3.58058750187815,-5.74209736432551,
90.0199910589308));
#205561=CARTESIAN_POINT('Ctrl Pts',(-3.43574888457639,-5.83241407440466,
90.0280507520409));
#205562=CARTESIAN_POINT('Ctrl Pts',(-3.28726497294158,-5.91738782370924,
90.0361104451509));
#205563=CARTESIAN_POINT('Ctrl Pts',(-3.13557561949261,-5.99670363903733,
90.044170138261));
#205564=CARTESIAN_POINT('Ctrl Pts',(-2.98404381953061,-6.07593707229316,
90.0522214600996));
#205565=CARTESIAN_POINT('Ctrl Pts',(-2.82931353102591,-6.14952409478376,
90.0602727819382));
#205566=CARTESIAN_POINT('Ctrl Pts',(-2.67185372211453,-6.21719283017849,
90.0683241037768));
#205567=CARTESIAN_POINT('Ctrl Pts',(-2.5145229554147,-6.28480610936931,
90.0763688273578));
#205568=CARTESIAN_POINT('Ctrl Pts',(-2.3544674615105,-6.34651060832816,
90.0844135509388));
#205569=CARTESIAN_POINT('Ctrl Pts',(-2.19218086535646,-6.40208029109016,
90.0924582745199));
#205570=CARTESIAN_POINT('Ctrl Pts',(-2.02999174247932,-6.45761659734908,
90.1004981662442));
#205571=CARTESIAN_POINT('Ctrl Pts',(-1.86557453707419,-6.50702530198869,
90.1085380579686));
#205572=CARTESIAN_POINT('Ctrl Pts',(-1.69944281225294,-6.5501284817843,
90.116577949693));
#205573=CARTESIAN_POINT('Ctrl Pts',(-1.52973381624805,-6.59415979112994,
90.1247909623129));
#205574=CARTESIAN_POINT('Ctrl Pts',(-1.35823599277948,-6.63161078727063,
90.1330039749329));
#205575=CARTESIAN_POINT('Ctrl Pts',(-1.18551359082838,-6.66234542229395,
90.1412169875528));
#205576=CARTESIAN_POINT('Ctrl Pts',(-1.01649097311715,-6.69242170890971,
90.1492540740954));
#205577=CARTESIAN_POINT('Ctrl Pts',(-0.84629609241444,-6.71606639881895,
90.157291160638));
#205578=CARTESIAN_POINT('Ctrl Pts',(-0.675467926551339,-6.73320370107726,
90.1653282471806));
#205579=CARTESIAN_POINT('Ctrl Pts',(-0.50462341163754,-6.75034264345517,
90.1733661029097));
#205580=CARTESIAN_POINT('Ctrl Pts',(-0.333145862640353,-6.76097292068633,
90.1814039586389));
#205581=CARTESIAN_POINT('Ctrl Pts',(-0.161578941431658,-6.7650706755869,
90.189441814368));
#205582=CARTESIAN_POINT('Ctrl Pts',(0.01003839266516,-6.76916963456375,
90.197482031925));
#205583=CARTESIAN_POINT('Ctrl Pts',(0.181744777936125,-6.76673224159009,
90.2055222494819));
#205584=CARTESIAN_POINT('Ctrl Pts',(0.352997142022572,-6.75778676918145,
90.2135624670388));
#205585=CARTESIAN_POINT('Ctrl Pts',(0.530719530148687,-6.7485033310937,
90.2219064491666));
#205586=CARTESIAN_POINT('Ctrl Pts',(0.707952476140451,-6.73221047264373,
90.2302504312944));
#205587=CARTESIAN_POINT('Ctrl Pts',(0.884096636273593,-6.70899859425606,
90.2385944134221));
#205588=CARTESIAN_POINT('Ctrl Pts',(1.05412371518278,-6.68659281097452,
90.2466486282572));
#205589=CARTESIAN_POINT('Ctrl Pts',(1.22313601107666,-6.65774064209402,
90.2547028430922));
#205590=CARTESIAN_POINT('Ctrl Pts',(1.39060703617396,-6.62257510874309,
90.2627570579273));
#205591=CARTESIAN_POINT('Ctrl Pts',(1.55820338564052,-6.58738325980541,
90.2708173000103));
#205592=CARTESIAN_POINT('Ctrl Pts',(1.72425580781475,-6.54586872928396,
90.2788775420933));
#205593=CARTESIAN_POINT('Ctrl Pts',(1.88825438303719,-6.49821393807105,
90.2869377841763));
#205594=CARTESIAN_POINT('Ctrl Pts',(2.05248223951706,-6.4504925221912,90.2950092950307));
#205595=CARTESIAN_POINT('Ctrl Pts',(2.21465016887878,-6.39661383472942,
90.303080805885));
#205596=CARTESIAN_POINT('Ctrl Pts',(2.37426903535021,-6.33680799360192,
90.3111523167393));
#205597=CARTESIAN_POINT('Ctrl Pts',(2.39099875911102,-6.33053971702871,
90.3119982953502));
#205598=CARTESIAN_POINT('Ctrl Pts',(2.40770050421689,-6.32420637030809,
90.312844273961));
#205599=CARTESIAN_POINT('Ctrl Pts',(2.42437372432497,-6.31780824691623,
90.3136902525719));
#205600=CARTESIAN_POINT('Ctrl Pts',(2.58656233099902,-6.25557055608454,
90.3219195023079));
#205601=CARTESIAN_POINT('Ctrl Pts',(2.74659110609951,-6.1869919234823,90.3301487520439));
#205602=CARTESIAN_POINT('Ctrl Pts',(2.9039284677193,-6.11224087012034,90.3383780017798));
#205603=CARTESIAN_POINT('Ctrl Pts',(3.0610785722831,-6.03757878267239,90.3465974573699));
#205604=CARTESIAN_POINT('Ctrl Pts',(3.21554332089398,-5.95675905463117,
90.3548169129599));
#205605=CARTESIAN_POINT('Ctrl Pts',(3.3668081037196,-5.86999933498532,90.36303636855));
#205606=CARTESIAN_POINT('Ctrl Pts',(3.51792323453601,-5.78332545003357,
90.3712476923197));
#205607=CARTESIAN_POINT('Ctrl Pts',(3.66584439531142,-5.69072345389549,
90.3794590160893));
#205608=CARTESIAN_POINT('Ctrl Pts',(3.81007864031179,-5.59245829261514,
90.387670339859));
#205609=CARTESIAN_POINT('Ctrl Pts',(3.95419914419499,-5.49427062187266,
90.3958751882931));
#205610=CARTESIAN_POINT('Ctrl Pts',(4.09463822819254,-5.3904288820048,90.4040800367272));
#205611=CARTESIAN_POINT('Ctrl Pts',(4.23092909976346,-5.28124303102734,
90.4122848851613));
#205612=CARTESIAN_POINT('Ctrl Pts',(4.36713984786098,-5.17212136886549,
90.4204849100811));
#205613=CARTESIAN_POINT('Ctrl Pts',(4.49920696246336,-5.0576620778637,90.428684935001));
#205614=CARTESIAN_POINT('Ctrl Pts',(4.62669404638303,-4.93821741128961,
90.4368849599209));
#205615=CARTESIAN_POINT('Ctrl Pts',(4.75414423265293,-4.81880731470754,
90.4450826115679));
#205616=CARTESIAN_POINT('Ctrl Pts',(4.87701676449178,-4.69441495859912,
90.4532802632148));
#205617=CARTESIAN_POINT('Ctrl Pts',(4.99490947754159,-4.56543188659793,
90.4614779148617));
#205618=CARTESIAN_POINT('Ctrl Pts',(5.11278640403386,-4.43646608622139,
90.4696744687928));
#205619=CARTESIAN_POINT('Ctrl Pts',(5.2256845972344,-4.30291105840411,90.4778710227239));
#205620=CARTESIAN_POINT('Ctrl Pts',(5.33323982719857,-4.16519410659131,
90.486067576655));
#205621=CARTESIAN_POINT('Ctrl Pts',(5.44080021119289,-4.02747055540326,
90.4942645233637));
#205622=CARTESIAN_POINT('Ctrl Pts',(5.54301690099167,-3.88558496561313,
90.5024614700724));
#205623=CARTESIAN_POINT('Ctrl Pts',(5.63956690012634,-3.73999654799299,
90.5106584167811));
#205624=CARTESIAN_POINT('Ctrl Pts',(5.73613908118205,-3.59437468209926,
90.5188572467008));
#205625=CARTESIAN_POINT('Ctrl Pts',(5.82704178035555,-3.4450485929394,90.5270560766206));
#205626=CARTESIAN_POINT('Ctrl Pts',(5.91199613255347,-3.29250523593705,
90.5352549065403));
#205627=CARTESIAN_POINT('Ctrl Pts',(5.99703094738359,-3.13981740087427,
90.5434615018002));
#205628=CARTESIAN_POINT('Ctrl Pts',(6.07610598455327,-2.98390652384556,
90.55166809706));
#205629=CARTESIAN_POINT('Ctrl Pts',(6.14898861742622,-2.82528369951812,
90.5598746923198));
#205630=CARTESIAN_POINT('Ctrl Pts',(6.22190652591139,-2.66658410083417,
90.5680852596188));
#205631=CARTESIAN_POINT('Ctrl Pts',(6.28862591752067,-2.5051702691891,90.5762958269178));
#205632=CARTESIAN_POINT('Ctrl Pts',(6.34896293916979,-2.34157182188556,
90.5845063942168));
#205633=CARTESIAN_POINT('Ctrl Pts',(6.40938317420954,-2.17774774890267,
90.5927282850635));
#205634=CARTESIAN_POINT('Ctrl Pts',(6.46340333699398,-2.01173338019453,
90.6009501759102));
#205635=CARTESIAN_POINT('Ctrl Pts',(6.5108895817058,-1.84407316959898,90.6091720667569));
#205636=CARTESIAN_POINT('Ctrl Pts',(6.55406578495451,-1.69163047017469,
90.6166477059118));
#205637=CARTESIAN_POINT('Ctrl Pts',(6.59184092278741,-1.53782748310096,
90.6241233450666));
#205638=CARTESIAN_POINT('Ctrl Pts',(6.62415141723914,-1.38307881246466,
90.6315989842215));
#205639=CARTESIAN_POINT('Ctrl Pts',(6.66277349961948,-1.19810126857434,
90.6405349276722));
#205640=CARTESIAN_POINT('Ctrl Pts',(6.69366778144579,-1.01138724800797,
90.649470871123));
#205641=CARTESIAN_POINT('Ctrl Pts',(6.71669652522179,-0.823575611631092,
90.6584068145737));
#205642=CARTESIAN_POINT('Ctrl Pts',(6.73969065068789,-0.636046305957762,
90.6673293249313));
#205643=CARTESIAN_POINT('Ctrl Pts',(6.75484279967089,-0.447422932502711,
90.6762518352889));
#205644=CARTESIAN_POINT('Ctrl Pts',(6.76206644467396,-0.258353242314716,
90.6851743456465));
#205645=CARTESIAN_POINT('Ctrl Pts',(6.76927238950509,-0.0697468315408935,
90.6940749930848));
#205646=CARTESIAN_POINT('Ctrl Pts',(6.76858859394774,0.119303455756674,
90.7029756405231));
#205647=CARTESIAN_POINT('Ctrl Pts',(6.75998037107751,0.308146690144195,
90.7118762879614));
#205648=CARTESIAN_POINT('Ctrl Pts',(6.75138545115332,0.496698090619526,
90.7207631805476));
#205649=CARTESIAN_POINT('Ctrl Pts',(6.73489054362257,0.685042819801436,
90.7296500731339));
#205650=CARTESIAN_POINT('Ctrl Pts',(6.7105128222379,0.872528889252838,90.7385369657201));
#205651=CARTESIAN_POINT('Ctrl Pts',(6.68619776069702,1.05953304952001,90.747401015675));
#205652=CARTESIAN_POINT('Ctrl Pts',(6.65404034946211,1.24568269884231,90.7562650656299));
#205653=CARTESIAN_POINT('Ctrl Pts',(6.61410939888276,1.43033068190916,90.7651291155848));
#205654=CARTESIAN_POINT('Ctrl Pts',(6.5759321979058,1.60686900762538,90.7736038604053));
#205655=CARTESIAN_POINT('Ctrl Pts',(6.53064961384517,1.78203447442935,90.7820786052257));
#205656=CARTESIAN_POINT('Ctrl Pts',(6.47836623906234,1.95526465537975,90.7905533500462));
#205657=CARTESIAN_POINT('Ctrl Pts',(6.42772285583972,2.12306106247923,90.7987622644753));
#205658=CARTESIAN_POINT('Ctrl Pts',(6.37055887359042,2.28887966137623,90.8069711789044));
#205659=CARTESIAN_POINT('Ctrl Pts',(6.3070641999167,2.45218885449901,90.8151800933335));
#205660=CARTESIAN_POINT('Ctrl Pts',(6.24355443070684,2.6155368735529,90.8233909593904));
#205661=CARTESIAN_POINT('Ctrl Pts',(6.17371110054856,2.77637396635425,90.8316018254472));
#205662=CARTESIAN_POINT('Ctrl Pts',(6.09777225654522,2.93418856028501,90.839812691504));
#205663=CARTESIAN_POINT('Ctrl Pts',(6.02180182205004,3.09206880494707,90.8480269732738));
#205664=CARTESIAN_POINT('Ctrl Pts',(5.93973097627568,3.24692372521614,90.8562412550436));
#205665=CARTESIAN_POINT('Ctrl Pts',(5.85184373025022,3.39826631633414,90.8644555368135));
#205666=CARTESIAN_POINT('Ctrl Pts',(5.76385756019135,3.54977925548576,90.8726790644059));
#205667=CARTESIAN_POINT('Ctrl Pts',(5.67004209261495,3.69777166119129,90.8809025919983));
#205668=CARTESIAN_POINT('Ctrl Pts',(5.5707252204531,3.84178467879289,90.8891261195907));
#205669=CARTESIAN_POINT('Ctrl Pts',(5.4713446900399,3.98589000313626,90.8973549181444));
#205670=CARTESIAN_POINT('Ctrl Pts',(5.36645593864416,4.1260105705275,90.905583716698));
#205671=CARTESIAN_POINT('Ctrl Pts',(5.25642711667533,4.26172065803007,90.9138125152517));
#205672=CARTESIAN_POINT('Ctrl Pts',(5.14624684883752,4.39761753960863,90.9220526400881));
#205673=CARTESIAN_POINT('Ctrl Pts',(5.03091261310206,4.52909154878991,90.9302927649246));
#205674=CARTESIAN_POINT('Ctrl Pts',(4.91083005091975,4.65575313037359,90.938532889761));
#205675=CARTESIAN_POINT('Ctrl Pts',(4.85751834893465,4.71198564546683,90.942191165131));
#205676=CARTESIAN_POINT('Ctrl Pts',(4.80327120491539,4.76727015589958,90.945849440501));
#205677=CARTESIAN_POINT('Ctrl Pts',(4.74812616705041,4.82157514737365,90.949507715871));
#205678=CARTESIAN_POINT('Ctrl Pts',(4.6207926986536,4.94696889417971,90.957954910927));
#205679=CARTESIAN_POINT('Ctrl Pts',(4.48837834219849,5.0674242804353,90.9664021059829));
#205680=CARTESIAN_POINT('Ctrl Pts',(4.35129296385923,5.18252241120762,90.9748493010389));
#205681=CARTESIAN_POINT('Ctrl Pts',(4.21431818108728,5.29752768493548,90.9832896812008));
#205682=CARTESIAN_POINT('Ctrl Pts',(4.07268013894871,5.40718410131449,90.9917300613627));
#205683=CARTESIAN_POINT('Ctrl Pts',(3.9268248019547,5.51111023068433,91.0001704415246));
#205684=CARTESIAN_POINT('Ctrl Pts',(3.78109282050226,5.6149484656772,91.0086036833281));
#205685=CARTESIAN_POINT('Ctrl Pts',(3.63115092728356,5.71306588493759,91.0170369251317));
#205686=CARTESIAN_POINT('Ctrl Pts',(3.47747738834778,5.80512187757759,91.0254701669352));
#205687=CARTESIAN_POINT('Ctrl Pts',(3.3536864243144,5.87927713002294,91.0322635234234));
#205688=CARTESIAN_POINT('Ctrl Pts',(3.22747467812902,5.94949982342603,91.0390568799115));
#205689=CARTESIAN_POINT('Ctrl Pts',(3.09910619832119,6.01563211736948,91.0458502363996));
#205690=CARTESIAN_POINT('Ctrl Pts',(3.09910619832144,6.01563211736935,89.0458803684832));
#205691=CARTESIAN_POINT('Ctrl Pts',(2.94574414940646,6.09464048541888,89.0540188657321));
#205692=CARTESIAN_POINT('Ctrl Pts',(2.7891686254625,6.16787827641324,89.062157362981));
#205693=CARTESIAN_POINT('Ctrl Pts',(2.62985788981656,6.23507309334619,89.0702958602299));
#205694=CARTESIAN_POINT('Ctrl Pts',(2.47068172296856,6.30221115123082,89.0784274829403));
#205695=CARTESIAN_POINT('Ctrl Pts',(2.30877527871085,6.36331625436805,89.0865591056507));
#205696=CARTESIAN_POINT('Ctrl Pts',(2.14464122207223,6.41816196652816,89.094690728361));
#205697=CARTESIAN_POINT('Ctrl Pts',(1.98061446992856,6.47297182268394,89.1028170349311));
#205698=CARTESIAN_POINT('Ctrl Pts',(1.8143633510293,6.52153031983798,89.1109433415012));
#205699=CARTESIAN_POINT('Ctrl Pts',(1.64641026628949,6.56365921076472,89.1190696480713));
#205700=CARTESIAN_POINT('Ctrl Pts',(1.47853167663572,6.60576941554849,89.1271923502426));
#205701=CARTESIAN_POINT('Ctrl Pts',(1.30895297895508,6.64145560418459,89.1353150524138));
#205702=CARTESIAN_POINT('Ctrl Pts',(1.13821147157311,6.67058945266304,89.143437754585));
#205703=CARTESIAN_POINT('Ctrl Pts',(0.967513373666449,6.6997158941255,89.1515583916331));
#205704=CARTESIAN_POINT('Ctrl Pts',(0.795653415853312,6.72229325329825,
89.1596790286812));
#205705=CARTESIAN_POINT('Ctrl Pts',(0.623178770462661,6.73824437224153,
89.1677996657292));
#205706=CARTESIAN_POINT('Ctrl Pts',(0.450693819226889,6.75419644430903,
89.1759207880082));
#205707=CARTESIAN_POINT('Ctrl Pts',(0.277594471498387,6.76352144946732,
89.1840419102872));
#205708=CARTESIAN_POINT('Ctrl Pts',(0.104432856585541,6.76619411327117,
89.1921630325662));
#205709=CARTESIAN_POINT('Ctrl Pts',(0.0415555946075978,6.76716459268289,
89.195111918977));
#205710=CARTESIAN_POINT('Ctrl Pts',(-0.0213298580456094,6.76725845031424,
89.1980608053878));
#205711=CARTESIAN_POINT('Ctrl Pts',(-0.0841970533259905,6.76647617717015,
89.2010096917986));
#205712=CARTESIAN_POINT('Ctrl Pts',(-0.27573595059093,6.76409280799471,
89.2099941303244));
#205713=CARTESIAN_POINT('Ctrl Pts',(-0.467010343119068,6.75357432232411,
89.2189785688502));
#205714=CARTESIAN_POINT('Ctrl Pts',(-0.657353833176219,6.7349962834443,
89.227963007376));
#205715=CARTESIAN_POINT('Ctrl Pts',(-0.848025844737191,6.71638617997815,
89.2369629525065));
#205716=CARTESIAN_POINT('Ctrl Pts',(-1.03776350463907,6.68968874356541,
89.245962897637));
#205717=CARTESIAN_POINT('Ctrl Pts',(-1.22590818518116,6.65503103835781,
89.2549628427675));
#205718=CARTESIAN_POINT('Ctrl Pts',(-1.41449623349204,6.62029166137833,
89.2639839964997));
#205719=CARTESIAN_POINT('Ctrl Pts',(-1.6014835555457,6.57755452620292,89.2730051502319));
#205720=CARTESIAN_POINT('Ctrl Pts',(-1.78622161222539,6.5269978820296,89.2820263039641));
#205721=CARTESIAN_POINT('Ctrl Pts',(-1.97114764133391,6.47638979607234,
89.2910566367913));
#205722=CARTESIAN_POINT('Ctrl Pts',(-2.15381960422244,6.41794637496796,
89.3000869696185));
#205723=CARTESIAN_POINT('Ctrl Pts',(-2.33360513622278,6.35189547050286,
89.3091173024458));
#205724=CARTESIAN_POINT('Ctrl Pts',(-2.5136455474358,6.28575092667567,89.3181604374384));
#205725=CARTESIAN_POINT('Ctrl Pts',(-2.69079112119019,6.21197741704217,
89.327203572431));
#205726=CARTESIAN_POINT('Ctrl Pts',(-2.86442828932985,6.13085145597958,
89.3362467074237));
#205727=CARTESIAN_POINT('Ctrl Pts',(-3.01622717794516,6.05992867568379,
89.3441524908236));
#205728=CARTESIAN_POINT('Ctrl Pts',(-3.16534490603844,5.98338734153934,
89.3520582742235));
#205729=CARTESIAN_POINT('Ctrl Pts',(-3.31138686120792,5.90144101516058,
89.3599640576234));
#205730=CARTESIAN_POINT('Ctrl Pts',(-3.47123917081076,5.81174549225478,
89.3686174458516));
#205731=CARTESIAN_POINT('Ctrl Pts',(-3.6275470699987,5.71549403260485,89.3772708340798));
#205732=CARTESIAN_POINT('Ctrl Pts',(-3.77977306256917,5.61298535500285,
89.3859242223081));
#205733=CARTESIAN_POINT('Ctrl Pts',(-3.93185846363741,5.51057135143603,
89.3945696185184));
#205734=CARTESIAN_POINT('Ctrl Pts',(-4.07986922599621,5.40191182545246,
89.4032150147288));
#205735=CARTESIAN_POINT('Ctrl Pts',(-4.22329472397144,5.28735006165423,
89.4118604109392));
#205736=CARTESIAN_POINT('Ctrl Pts',(-4.37130074920802,5.16912958103372,
89.4207819119816));
#205737=CARTESIAN_POINT('Ctrl Pts',(-4.51442349841515,5.04462377878463,
89.4297034130241));
#205738=CARTESIAN_POINT('Ctrl Pts',(-4.65213466616417,4.91425803635438,
89.4386249140665));
#205739=CARTESIAN_POINT('Ctrl Pts',(-4.78532974938659,4.78816749340004,
89.4472538444085));
#205740=CARTESIAN_POINT('Ctrl Pts',(-4.91346229956792,4.65659547223805,
89.4558827747504));
#205741=CARTESIAN_POINT('Ctrl Pts',(-5.03608783609214,4.51996773297828,
89.4645117050923));
#205742=CARTESIAN_POINT('Ctrl Pts',(-5.16494994615941,4.37639128655632,
89.473579491485));
#205743=CARTESIAN_POINT('Ctrl Pts',(-5.28773002020762,4.22723167850583,
89.4826472778776));
#205744=CARTESIAN_POINT('Ctrl Pts',(-5.40395577284719,4.07302725317564,
89.4917150642702));
#205745=CARTESIAN_POINT('Ctrl Pts',(-5.52018152548685,3.91882282784535,
89.5007828506629));
#205746=CARTESIAN_POINT('Ctrl Pts',(-5.62985269355601,3.75957387589938,
89.5098506370555));
#205747=CARTESIAN_POINT('Ctrl Pts',(-5.7325456686147,3.59586000245377,89.5189184234482));
#205748=CARTESIAN_POINT('Ctrl Pts',(-5.82795857013114,3.44375207418494,
89.5273433795813));
#205749=CARTESIAN_POINT('Ctrl Pts',(-5.91730593764035,3.28785670772003,
89.5357683357145));
#205750=CARTESIAN_POINT('Ctrl Pts',(-6.00029950281174,3.12868900285043,
89.5441932918476));
#205751=CARTESIAN_POINT('Ctrl Pts',(-6.08331233158658,2.96948435362806,
89.552620203494));
#205752=CARTESIAN_POINT('Ctrl Pts',(-6.1599682642167,2.80700614562378,89.5610471151404));
#205753=CARTESIAN_POINT('Ctrl Pts',(-6.23002569731353,2.64179272669396,
89.5694740267868));
#205754=CARTESIAN_POINT('Ctrl Pts',(-6.3001088932571,2.47651855235525,89.5779040373368));
#205755=CARTESIAN_POINT('Ctrl Pts',(-6.36358862201089,2.30850746667938,
89.5863340478868));
#205756=CARTESIAN_POINT('Ctrl Pts',(-6.42027184426169,2.13831673186659,
89.5947640584368));
#205757=CARTESIAN_POINT('Ctrl Pts',(-6.47700728191154,1.96796922090771,
89.6032018345362));
#205758=CARTESIAN_POINT('Ctrl Pts',(-6.52693359967498,1.79543836414719,
89.6116396106356));
#205759=CARTESIAN_POINT('Ctrl Pts',(-6.569907643377,1.62129656679353,89.6200773867351));
#205760=CARTESIAN_POINT('Ctrl Pts',(-6.61290424528407,1.4470633578334,89.628519592045));
#205761=CARTESIAN_POINT('Ctrl Pts',(-6.64894122299971,1.27121784521705,
89.6369617973549));
#205762=CARTESIAN_POINT('Ctrl Pts',(-6.67792665757091,1.09434206539997,
89.6454040026647));
#205763=CARTESIAN_POINT('Ctrl Pts',(-6.70694267018077,0.917279691367016,
89.6538551140367));
#205764=CARTESIAN_POINT('Ctrl Pts',(-6.72889223375355,0.739185207131805,
89.6623062254088));
#205765=CARTESIAN_POINT('Ctrl Pts',(-6.7437352225717,0.56064627693926,89.6707573367808));
#205766=CARTESIAN_POINT('Ctrl Pts',(-6.74790093037528,0.510539049624142,
89.6731291542781));
#205767=CARTESIAN_POINT('Ctrl Pts',(-6.75150720210199,0.460396821494576,
89.6755009717754));
#205768=CARTESIAN_POINT('Ctrl Pts',(-6.7545538882394,0.410232581434043,
89.6778727892727));
#205769=CARTESIAN_POINT('Ctrl Pts',(-6.76282073461048,0.274117455950735,
89.6843084541184));
#205770=CARTESIAN_POINT('Ctrl Pts',(-6.76697248697646,0.137764909183088,
89.6907441189641));
#205771=CARTESIAN_POINT('Ctrl Pts',(-6.76699986371201,0.00135813167870539,
89.6971797838098));
#205772=CARTESIAN_POINT('',(-6.76699948056331,-0.00136021873801901,89.3028202161898));
#205773=CARTESIAN_POINT('Ctrl Pts',(3.09910619832125,6.01563211736945,88.6513956954041));
#205774=CARTESIAN_POINT('Ctrl Pts',(2.93375330764816,6.10081787314658,88.6601451433064));
#205775=CARTESIAN_POINT('Ctrl Pts',(2.7648862784306,6.17918207037044,88.6688945912087));
#205776=CARTESIAN_POINT('Ctrl Pts',(2.59307866646691,6.25045854554002,88.677644039111));
#205777=CARTESIAN_POINT('Ctrl Pts',(2.4212724418536,6.32173444515044,88.6863934163613));
#205778=CARTESIAN_POINT('Ctrl Pts',(2.24652594672442,6.38592262741846,88.6951427936116));
#205779=CARTESIAN_POINT('Ctrl Pts',(2.06943269687093,6.44280508110571,88.7038921708619));
#205780=CARTESIAN_POINT('Ctrl Pts',(1.89234081822049,6.49968709436174,88.7126414803672));
#205781=CARTESIAN_POINT('Ctrl Pts',(1.7129024940556,6.54926340459552,88.7213907898726));
#205782=CARTESIAN_POINT('Ctrl Pts',(1.5317271662503,6.5913656315039,88.730140099378));
#205783=CARTESIAN_POINT('Ctrl Pts',(1.3505531810731,6.63346754640715,88.7388893440452));
#205784=CARTESIAN_POINT('Ctrl Pts',(1.167642497144,6.66809542395779,88.7476385887124));
#205785=CARTESIAN_POINT('Ctrl Pts',(0.983616340614198,6.6951316562467,88.7563878333797));
#205786=CARTESIAN_POINT('Ctrl Pts',(0.799591486713808,6.72216769715961,
88.7651370161154));
#205787=CARTESIAN_POINT('Ctrl Pts',(0.614451459526804,6.7416121586937,88.773886198851));
#205788=CARTESIAN_POINT('Ctrl Pts',(0.4288250479105,6.75339900185711,88.7826353815867));
#205789=CARTESIAN_POINT('Ctrl Pts',(0.243199888597169,6.76518576550221,
88.7913845052973));
#205790=CARTESIAN_POINT('Ctrl Pts',(0.0570886373919456,6.76931499599834,
88.8001336290078));
#205791=CARTESIAN_POINT('Ctrl Pts',(-0.128876626811216,6.76577266947847,
88.8088827527183));
#205792=CARTESIAN_POINT('Ctrl Pts',(-0.314840698188169,6.76223036567993,
88.8176318203099));
#205793=CARTESIAN_POINT('Ctrl Pts',(-0.500658497951208,6.75101660879223,
88.8263808879014));
#205794=CARTESIAN_POINT('Ctrl Pts',(-0.685698951926118,6.73216948296219,
88.835129955493));
#205795=CARTESIAN_POINT('Ctrl Pts',(-0.870738280460047,6.71332247176291,
88.8438789698715));
#205796=CARTESIAN_POINT('Ctrl Pts',(-1.05499998761299,6.6868422135618,88.85262798425));
#205797=CARTESIAN_POINT('Ctrl Pts',(-1.23785829161497,6.65281863948508,
88.8613769986286));
#205798=CARTESIAN_POINT('Ctrl Pts',(-1.43007412917477,6.61705395368845,
88.8705737323278));
#205799=CARTESIAN_POINT('Ctrl Pts',(-1.62073882535861,6.57295372727773,
88.879770466027));
#205800=CARTESIAN_POINT('Ctrl Pts',(-1.80913696091579,6.52068343478261,
88.8889671997262));
#205801=CARTESIAN_POINT('Ctrl Pts',(-1.98838356186177,6.47095219815179,
88.8977171974399));
#205802=CARTESIAN_POINT('Ctrl Pts',(-2.16557827572598,6.41382586850869,
88.9064671951535));
#205803=CARTESIAN_POINT('Ctrl Pts',(-2.34011918621764,6.34949849943254,
88.9152171928672));
#205804=CARTESIAN_POINT('Ctrl Pts',(-2.51465655691168,6.28517243495523,
88.9239670131255));
#205805=CARTESIAN_POINT('Ctrl Pts',(-2.68653996295402,6.21364572242343,
88.9327168333838));
#205806=CARTESIAN_POINT('Ctrl Pts',(-2.85518555380067,6.13516132252184,
88.9414666536421));
#205807=CARTESIAN_POINT('Ctrl Pts',(-3.02382794858768,6.05667841000467,
88.9502163080796));
#205808=CARTESIAN_POINT('Ctrl Pts',(-3.18923239109361,5.97123819492038,
88.9589659625171));
#205809=CARTESIAN_POINT('Ctrl Pts',(-3.35083705967778,5.87913088810667,
88.9677156169546));
#205810=CARTESIAN_POINT('Ctrl Pts',(-3.51243888042463,5.78702520443064,
88.9764651172036));
#205811=CARTESIAN_POINT('Ctrl Pts',(-3.67024081223738,5.68825280605752,
88.9852146174525));
#205812=CARTESIAN_POINT('Ctrl Pts',(-3.82370687544434,5.58314917682482,
88.9939641177014));
#205813=CARTESIAN_POINT('Ctrl Pts',(-3.97717043817854,5.47804726007993,
89.0027134753919));
#205814=CARTESIAN_POINT('Ctrl Pts',(-4.12629803722506,5.36661448084201,
89.0114628330824));
#205815=CARTESIAN_POINT('Ctrl Pts',(-4.27058317206959,5.24922931204535,
89.0202121907728));
#205816=CARTESIAN_POINT('Ctrl Pts',(-4.41486614774869,5.13184589986761,
89.0289614175329));
#205817=CARTESIAN_POINT('Ctrl Pts',(-4.55430658194432,5.00851045723017,
89.037710644293));
#205818=CARTESIAN_POINT('Ctrl Pts',(-4.68843089001849,4.87964187103116,
89.046459871053));
#205819=CARTESIAN_POINT('Ctrl Pts',(-4.82255336917847,4.7507750420795,89.055208978509));
#205820=CARTESIAN_POINT('Ctrl Pts',(-4.95135966065152,4.61637541908075,
89.0639580859649));
#205821=CARTESIAN_POINT('Ctrl Pts',(-5.07441230869268,4.47689945401818,
89.0727071934208));
#205822=CARTESIAN_POINT('Ctrl Pts',(-5.19746344226446,4.33742520555481,
89.0814561931972));
#205823=CARTESIAN_POINT('Ctrl Pts',(-5.31476088454801,4.19287495491294,
89.0902051929736));
#205824=CARTESIAN_POINT('Ctrl Pts',(-5.42590627628892,4.04373961586655,
89.0989541927499));
#205825=CARTESIAN_POINT('Ctrl Pts',(-5.53706380672706,3.8945879890668,89.1077041480446));
#205826=CARTESIAN_POINT('Ctrl Pts',(-5.64206777071902,3.74085050155226,
89.1164541033393));
#205827=CARTESIAN_POINT('Ctrl Pts',(-5.74056148164046,3.583049382231,89.125204058634));
#205828=CARTESIAN_POINT('Ctrl Pts',(-5.83905138951924,3.42525435593214,
89.1339536760752));
#205829=CARTESIAN_POINT('Ctrl Pts',(-5.93103139557694,3.26339625497108,
89.1427032935163));
#205830=CARTESIAN_POINT('Ctrl Pts',(-6.01618907820889,3.09802485064922,
89.1514529109574));
#205831=CARTESIAN_POINT('Ctrl Pts',(-6.10134392545018,2.93265895249567,
89.1602022370732));
#205832=CARTESIAN_POINT('Ctrl Pts',(-6.1796767726186,2.76378023985972,89.1689515631891));
#205833=CARTESIAN_POINT('Ctrl Pts',(-6.25092157009246,2.59196229227063,
89.177700889305));
#205834=CARTESIAN_POINT('Ctrl Pts',(-6.32216437407776,2.42014915229033,
89.1864499706074));
#205835=CARTESIAN_POINT('Ctrl Pts',(-6.38631941548944,2.24539720662787,
89.1951990519099));
#205836=CARTESIAN_POINT('Ctrl Pts',(-6.4431688103756,2.06829994947617,89.2039481332123));
#205837=CARTESIAN_POINT('Ctrl Pts',(-6.5000233452459,1.89118668024385,89.2126980055547));
#205838=CARTESIAN_POINT('Ctrl Pts',(-6.54957082411112,1.71172794807643,
89.221447877897));
#205839=CARTESIAN_POINT('Ctrl Pts',(-6.59164294296096,1.53053334250286,
89.2301977502394));
#205840=CARTESIAN_POINT('Ctrl Pts',(-6.63371214082145,1.34935131693543,
89.2389470150943));
#205841=CARTESIAN_POINT('Ctrl Pts',(-6.668306952397,1.16643393829706,89.2476962799492));
#205842=CARTESIAN_POINT('Ctrl Pts',(-6.69530988153997,0.982402458340396,
89.2564455448041));
#205843=CARTESIAN_POINT('Ctrl Pts',(-6.7223141969049,0.798361530946474,
89.2651952588111));
#205844=CARTESIAN_POINT('Ctrl Pts',(-6.74172580829283,0.613206671361901,
89.2739449728181));
#205845=CARTESIAN_POINT('Ctrl Pts',(-6.75347878028183,0.427566795112832,
89.2826946868252));
#205846=CARTESIAN_POINT('Ctrl Pts',(-6.76248992368212,0.285234494205639,
89.2894031966134));
#205847=CARTESIAN_POINT('Ctrl Pts',(-6.76699999999992,0.142617266093434,
89.2961117064016));
#205848=CARTESIAN_POINT('Ctrl Pts',(-6.767,3.67735927903396E-12,89.3028202161898));
#205849=CARTESIAN_POINT('Ctrl Pts',(-6.76699802633313,-0.00516832696203806,
89.3028202161898));
#205850=CARTESIAN_POINT('Ctrl Pts',(-6.76684902442674,-0.20025962320532,
89.311976675311));
#205851=CARTESIAN_POINT('Ctrl Pts',(-6.75825935055282,-0.395062537055501,
89.3211331344321));
#205852=CARTESIAN_POINT('Ctrl Pts',(-6.74132778610909,-0.588887663509377,
89.3302895935532));
#205853=CARTESIAN_POINT('Ctrl Pts',(-6.72431072437874,-0.78369152541593,
89.3394922889458));
#205854=CARTESIAN_POINT('Ctrl Pts',(-6.69886739001077,-0.977507505031502,
89.3486949843384));
#205855=CARTESIAN_POINT('Ctrl Pts',(-6.66514850928785,-1.16965137931693,
89.357897679731));
#205856=CARTESIAN_POINT('Ctrl Pts',(-6.6324927612709,-1.35573709174684,
89.3668102205798));
#205857=CARTESIAN_POINT('Ctrl Pts',(-6.59207542885528,-1.54025441184314,
89.3757227614285));
#205858=CARTESIAN_POINT('Ctrl Pts',(-6.54407704261772,-1.72259822950209,
89.3846353022773));
#205859=CARTESIAN_POINT('Ctrl Pts',(-6.49858031319104,-1.89543835986806,
89.3930833250398));
#205860=CARTESIAN_POINT('Ctrl Pts',(-6.44619239626076,-2.06662499248261,
89.4015313478023));
#205861=CARTESIAN_POINT('Ctrl Pts',(-6.38705197200869,-2.23558853702105,
89.4099793705649));
#205862=CARTESIAN_POINT('Ctrl Pts',(-6.32796570440939,-2.40439735659551,
89.4184196572206));
#205863=CARTESIAN_POINT('Ctrl Pts',(-6.26213936463124,-2.57098683266773,
89.4268599438764));
#205864=CARTESIAN_POINT('Ctrl Pts',(-6.1897617529613,-2.73480135322066,
89.4353002305322));
#205865=CARTESIAN_POINT('Ctrl Pts',(-6.1174392775055,-2.89849108224927,
89.4437340875001));
#205866=CARTESIAN_POINT('Ctrl Pts',(-6.0385756133742,-3.0594097658754,89.452167944468));
#205867=CARTESIAN_POINT('Ctrl Pts',(-5.9534082322147,-3.21702027046742,
89.4606018014359));
#205868=CARTESIAN_POINT('Ctrl Pts',(-5.86829263724442,-3.37453493969028,
89.4690305301809));
#205869=CARTESIAN_POINT('Ctrl Pts',(-5.77688112535556,-3.5287451476719,
89.4774592589259));
#205870=CARTESIAN_POINT('Ctrl Pts',(-5.67945798257234,-3.67913658678165,
89.485887987671));
#205871=CARTESIAN_POINT('Ctrl Pts',(-5.58207911753852,-3.82945967463254,
89.4943128856513));
#205872=CARTESIAN_POINT('Ctrl Pts',(-5.47869425069848,-3.97596717494488,
89.5027377836316));
#205873=CARTESIAN_POINT('Ctrl Pts',(-5.369632233226,-4.11817176425417,89.5111626816119));
#205874=CARTESIAN_POINT('Ctrl Pts',(-5.26059436226174,-4.26034486923589,
89.519585714306));
#205875=CARTESIAN_POINT('Ctrl Pts',(-5.14588204741826,-4.3982166966584,
89.5280087470002));
#205876=CARTESIAN_POINT('Ctrl Pts',(-5.02586617310408,-4.53133073280336,
89.5364317796943));
#205877=CARTESIAN_POINT('Ctrl Pts',(-4.90586387844969,-4.66442970724639,
89.5448538593319));
#205878=CARTESIAN_POINT('Ctrl Pts',(-4.78055944389228,-4.79277171599418,
89.5532759389695));
#205879=CARTESIAN_POINT('Ctrl Pts',(-4.65036277948422,-4.91593480623857,
89.5616980186071));
#205880=CARTESIAN_POINT('Ctrl Pts',(-4.5201626721991,-5.03910115336652,
89.5701203209553));
#205881=CARTESIAN_POINT('Ctrl Pts',(-4.38507031965246,-5.15708808006154,
89.5785426233036));
#205882=CARTESIAN_POINT('Ctrl Pts',(-4.24553134830853,-5.26951160645174,
89.5869649256518));
#205883=CARTESIAN_POINT('Ctrl Pts',(-4.10596920731208,-5.38195380012905,
89.5953886264755));
#205884=CARTESIAN_POINT('Ctrl Pts',(-3.9619592355185,-5.48883054305774,
89.6038123272991));
#205885=CARTESIAN_POINT('Ctrl Pts',(-3.81397916368428,-5.58979891758033,
89.6122360281228));
#205886=CARTESIAN_POINT('Ctrl Pts',(-3.6658989523829,-5.69083561832481,
89.6206654293418));
#205887=CARTESIAN_POINT('Ctrl Pts',(-3.51384354830047,-5.78595577306,89.6290948305607));
#205888=CARTESIAN_POINT('Ctrl Pts',(-3.35831947105741,-5.87485994133619,
89.6375242317797));
#205889=CARTESIAN_POINT('Ctrl Pts',(-3.20273990303963,-5.96379583049613,
89.6459566405973));
#205890=CARTESIAN_POINT('Ctrl Pts',(-3.04368948665119,-6.04651115076413,
89.654389049415));
#205891=CARTESIAN_POINT('Ctrl Pts',(-2.88169873408829,-6.12275276374557,
89.6628214582326));
#205892=CARTESIAN_POINT('Ctrl Pts',(-2.7195581029678,-6.19906491768568,
89.6712616689602));
#205893=CARTESIAN_POINT('Ctrl Pts',(-2.55447200463676,-6.26889126054263,
89.6797018796879));
#205894=CARTESIAN_POINT('Ctrl Pts',(-2.38699131364464,-6.33202664781072,
89.6881420904155));
#205895=CARTESIAN_POINT('Ctrl Pts',(-2.29173115451881,-6.36793697873903,
89.6929427382526));
#205896=CARTESIAN_POINT('Ctrl Pts',(-2.19569663012468,-6.40168359059077,
89.6977433860897));
#205897=CARTESIAN_POINT('Ctrl Pts',(-2.09899123165856,-6.43323595163589,
89.7025440339268));
#205898=CARTESIAN_POINT('Ctrl Pts',(-1.93502286481216,-6.48673440356076,
89.7106837489597));
#205899=CARTESIAN_POINT('Ctrl Pts',(-1.76879808507651,-6.534028424973,89.7188234639926));
#205900=CARTESIAN_POINT('Ctrl Pts',(-1.60083180762972,-6.57492406980347,
89.7269631790255));
#205901=CARTESIAN_POINT('Ctrl Pts',(-1.43301243248145,-6.61578394754832,
89.7350957751124));
#205902=CARTESIAN_POINT('Ctrl Pts',(-1.26345494472767,-6.65025650143955,
89.7432283711994));
#205903=CARTESIAN_POINT('Ctrl Pts',(-1.09269118493701,-6.67819698529184,
89.7513609672863));
#205904=CARTESIAN_POINT('Ctrl Pts',(-0.922044168413402,-6.70611836753046,
89.7594880034943));
#205905=CARTESIAN_POINT('Ctrl Pts',(-0.75019288165403,-6.72751651176724,
89.7676150397023));
#205906=CARTESIAN_POINT('Ctrl Pts',(-0.577681135053577,-6.74229734632071,
89.7757420759102));
#205907=CARTESIAN_POINT('Ctrl Pts',(-0.40525185219047,-6.75707111536772,
89.7838652272478));
#205908=CARTESIAN_POINT('Ctrl Pts',(-0.232163102268462,-6.76523384249223,
89.7919883785854));
#205909=CARTESIAN_POINT('Ctrl Pts',(-0.0589656085607672,-6.76674309080868,
89.8001115299229));
#205910=CARTESIAN_POINT('Ctrl Pts',(0.11418321536401,-6.76825191501514,
89.8082323985946));
#205911=CARTESIAN_POINT('Ctrl Pts',(0.287440356326177,-6.76311098204415,
89.8163532672663));
#205912=CARTESIAN_POINT('Ctrl Pts',(0.460253321125572,-6.75132993419762,
89.8244741359379));
#205913=CARTESIAN_POINT('Ctrl Pts',(0.633075625399209,-6.73954824965817,
89.8325954434925));
#205914=CARTESIAN_POINT('Ctrl Pts',(0.805453339905235,-6.72112575425677,
89.840716751047));
#205915=CARTESIAN_POINT('Ctrl Pts',(0.976837135832493,-6.69612411847769,
89.8488380586015));
#205916=CARTESIAN_POINT('Ctrl Pts',(1.06589411380776,-6.68313239942469,
89.8530581723182));
#205917=CARTESIAN_POINT('Ctrl Pts',(1.1546828009662,-6.66836503221109,89.8572782860349));
#205918=CARTESIAN_POINT('Ctrl Pts',(1.24312696509458,-6.65183616369606,
89.8614983997516));
#205919=CARTESIAN_POINT('Ctrl Pts',(1.43142074315825,-6.61664692164167,
89.8704828382773));
#205920=CARTESIAN_POINT('Ctrl Pts',(1.6180590903051,-6.57348838654307,89.8794672768031));
#205921=CARTESIAN_POINT('Ctrl Pts',(1.80239843341973,-6.52254926291907,
89.8884517153289));
#205922=CARTESIAN_POINT('Ctrl Pts',(1.98705593523852,-6.47152222140794,
89.8974516604593));
#205923=CARTESIAN_POINT('Ctrl Pts',(2.16940627181495,-6.41268781441574,
89.9064516055897));
#205924=CARTESIAN_POINT('Ctrl Pts',(2.3488223553158,-6.34628415241303,89.9154515507202));
#205925=CARTESIAN_POINT('Ctrl Pts',(2.52866123742258,-6.27972400847639,
89.9244727044523));
#205926=CARTESIAN_POINT('Ctrl Pts',(2.70555180636407,-6.20555900358184,
89.9334938581845));
#205927=CARTESIAN_POINT('Ctrl Pts',(2.8788856896544,-6.12407594547154,89.9425150119166));
#205928=CARTESIAN_POINT('Ctrl Pts',(3.05239594153723,-6.04250997770734,
89.9515453447438));
#205929=CARTESIAN_POINT('Ctrl Pts',(3.22234206447384,-5.9536111880958,89.960575677571));
#205930=CARTESIAN_POINT('Ctrl Pts',(3.38814012573824,-5.85771247914768,
89.9696060103982));
#205931=CARTESIAN_POINT('Ctrl Pts',(3.55417323639093,-5.76167781605931,
89.9786491453908));
#205932=CARTESIAN_POINT('Ctrl Pts',(3.71604631992265,-5.65862351070531,
89.9876922803834));
#205933=CARTESIAN_POINT('Ctrl Pts',(3.87320230542965,-5.54892718471007,
89.996735415376));
#205934=CARTESIAN_POINT('Ctrl Pts',(4.01059284338607,-5.45302732323355,
90.004641198776));
#205935=CARTESIAN_POINT('Ctrl Pts',(4.14437857112505,-5.352051822645,90.0125469821761));
#205936=CARTESIAN_POINT('Ctrl Pts',(4.27420733716696,-5.24627874201402,
90.0204527655762));
#205937=CARTESIAN_POINT('Ctrl Pts',(4.41631326885093,-5.13050330465603,
90.0291061538045));
#205938=CARTESIAN_POINT('Ctrl Pts',(4.55380320092629,-5.0088767392532,90.0377595420328));
#205939=CARTESIAN_POINT('Ctrl Pts',(4.68619881506422,-4.88178549976243,
90.0464129302611));
#205940=CARTESIAN_POINT('Ctrl Pts',(4.8184721524608,-4.75481163804676,90.0550583264716));
#205941=CARTESIAN_POINT('Ctrl Pts',(4.94566033750963,-4.6223833784292,90.063703722682));
#205942=CARTESIAN_POINT('Ctrl Pts',(5.06731916572162,-4.48492647350103,
90.0723491188924));
#205943=CARTESIAN_POINT('Ctrl Pts',(5.19286336708493,-4.34307965806887,
90.0812706199348));
#205944=CARTESIAN_POINT('Ctrl Pts',(5.31251892980312,-4.19587788347152,
90.0901921209772));
#205945=CARTESIAN_POINT('Ctrl Pts',(5.42583830773499,-4.04383081474924,
90.0991136220195));
#205946=CARTESIAN_POINT('Ctrl Pts',(5.53544150274975,-3.89676996047409,
90.1077425523615));
#205947=CARTESIAN_POINT('Ctrl Pts',(5.63911728330392,-3.74517682179181,
90.1163714827035));
#205948=CARTESIAN_POINT('Ctrl Pts',(5.73650075164642,-3.58954706423527,
90.1250004130455));
#205949=CARTESIAN_POINT('Ctrl Pts',(5.8388370151344,-3.42600218185482,90.1340681994381));
#205950=CARTESIAN_POINT('Ctrl Pts',(5.93422402424429,-3.25799964095291,
90.1431359858307));
#205951=CARTESIAN_POINT('Ctrl Pts',(6.0222887918476,-3.08615079145313,90.1522037722233));
#205952=CARTESIAN_POINT('Ctrl Pts',(6.11035355945096,-2.91430194195324,
90.1612715586158));
#205953=CARTESIAN_POINT('Ctrl Pts',(6.19109587612012,-2.7386071153367,90.1703393450084));
#205954=CARTESIAN_POINT('Ctrl Pts',(6.26419778537867,-2.55970996514391,
90.179407131401));
#205955=CARTESIAN_POINT('Ctrl Pts',(6.33211738031526,-2.3934951275337,90.1878320875342));
#205956=CARTESIAN_POINT('Ctrl Pts',(6.39341187239156,-2.22458893283593,
90.1962570436673));
#205957=CARTESIAN_POINT('Ctrl Pts',(6.44788558095911,-2.05354827916454,
90.2046819998005));
#205958=CARTESIAN_POINT('Ctrl Pts',(6.5023719333974,-1.88246792531532,90.2131089114469));
#205959=CARTESIAN_POINT('Ctrl Pts',(6.55003424509045,-1.70925244065029,
90.2215358230933));
#205960=CARTESIAN_POINT('Ctrl Pts',(6.59072679538052,-1.534473625923,90.2299627347397));
#205961=CARTESIAN_POINT('Ctrl Pts',(6.6314343099064,-1.35963053821748,90.2383927452897));
#205962=CARTESIAN_POINT('Ctrl Pts',(6.66516687738618,-1.18322329697116,
90.2468227558397));
#205963=CARTESIAN_POINT('Ctrl Pts',(6.69182986510452,-1.00583401040893,
90.2552527663898));
#205964=CARTESIAN_POINT('Ctrl Pts',(6.7185174142095,-0.828281316545892,
90.2636905424892));
#205965=CARTESIAN_POINT('Ctrl Pts',(6.73812232313079,-0.6497450981302,90.2721283185887));
#205966=CARTESIAN_POINT('Ctrl Pts',(6.75060170196344,-0.470813828862723,
90.2805660946882));
#205967=CARTESIAN_POINT('Ctrl Pts',(6.76308763155006,-0.291788633868696,
90.2890082999981));
#205968=CARTESIAN_POINT('Ctrl Pts',(6.7684405560547,-0.112368305394942,
90.297450505308));
#205969=CARTESIAN_POINT('Ctrl Pts',(6.76666971342945,0.0668579790049228,
90.3058927106179));
#205970=CARTESIAN_POINT('Ctrl Pts',(6.76489700266267,0.246273337273407,
90.31434382199));
#205971=CARTESIAN_POINT('Ctrl Pts',(6.75598552361211,0.425493911419589,
90.322794933362));
#205972=CARTESIAN_POINT('Ctrl Pts',(6.73999650540597,0.60393385988483,90.331246044734));
#205973=CARTESIAN_POINT('Ctrl Pts',(6.73550916267943,0.65401330782504,90.3336178622313));
#205974=CARTESIAN_POINT('Ctrl Pts',(6.73046466724945,0.704031317616007,
90.3359896797286));
#205975=CARTESIAN_POINT('Ctrl Pts',(6.72486509888547,0.75397506708915,90.3383614972259));
#205976=CARTESIAN_POINT('Ctrl Pts',(6.70523127933225,0.929093308572983,
90.3466778233656));
#205977=CARTESIAN_POINT('Ctrl Pts',(6.6787339000174,1.10361393938351,90.3549941495051));
#205978=CARTESIAN_POINT('Ctrl Pts',(6.64542263473519,1.27696789534791,90.3633104756447));
#205979=CARTESIAN_POINT('Ctrl Pts',(6.61213959741287,1.45017495120281,90.3716197545311));
#205980=CARTESIAN_POINT('Ctrl Pts',(6.57205424364966,1.62221696198514,90.3799290334175));
#205981=CARTESIAN_POINT('Ctrl Pts',(6.52526791707303,1.79253106260878,90.3882383123039));
#205982=CARTESIAN_POINT('Ctrl Pts',(6.47851265905959,1.96273206577888,90.3965420733953));
#205983=CARTESIAN_POINT('Ctrl Pts',(6.42506538689996,2.1312071107869,90.4048458344868));
#205984=CARTESIAN_POINT('Ctrl Pts',(6.36507833186934,2.29740436779586,90.4131495955782));
#205985=CARTESIAN_POINT('Ctrl Pts',(6.30512011780479,2.46352171940775,90.4214493643334));
#205986=CARTESIAN_POINT('Ctrl Pts',(6.23862850497366,2.62736313892462,90.4297491330887));
#205987=CARTESIAN_POINT('Ctrl Pts',(6.16580537077836,2.78839257094132,90.4380489018439));
#205988=CARTESIAN_POINT('Ctrl Pts',(6.0930039075049,2.94937408334741,90.4463462007296));
#205989=CARTESIAN_POINT('Ctrl Pts',(6.01387482180807,3.10754495961661,90.4546434996153));
#205990=CARTESIAN_POINT('Ctrl Pts',(5.92866794794776,3.26238951735946,90.4629407985011));
#205991=CARTESIAN_POINT('Ctrl Pts',(5.84345361350842,3.41724763304674,90.4712388238851));
#205992=CARTESIAN_POINT('Ctrl Pts',(5.75216058895213,3.56877853995535,90.4795368492692));
#205993=CARTESIAN_POINT('Ctrl Pts',(5.65508472775332,3.71649104962345,90.4878348746533));
#205994=CARTESIAN_POINT('Ctrl Pts',(5.55799936493663,3.86421801713724,90.4961337122338));
#205995=CARTESIAN_POINT('Ctrl Pts',(5.45513022814476,4.00812555134536,90.5044325498142));
#205996=CARTESIAN_POINT('Ctrl Pts',(5.34681653722777,4.14775142905498,90.5127313873947));
#205997=CARTESIAN_POINT('Ctrl Pts',(5.23847424448607,4.28741417703322,90.5210324164054));
#205998=CARTESIAN_POINT('Ctrl Pts',(5.12468474555575,4.42279274016383,90.5293334454162));
#205999=CARTESIAN_POINT('Ctrl Pts',(5.00582768909733,4.55345782313469,90.5376344744269));
#206000=CARTESIAN_POINT('Ctrl Pts',(4.88691949199242,4.68417912739366,90.5459390751228));
#206001=CARTESIAN_POINT('Ctrl Pts',(4.76293962589371,4.81018265238984,90.5542436758187));
#206002=CARTESIAN_POINT('Ctrl Pts',(4.63430486078077,4.93107568967906,90.5625482765147));
#206003=CARTESIAN_POINT('Ctrl Pts',(4.50552329878613,5.05210668905711,90.5708623543491));
#206004=CARTESIAN_POINT('Ctrl Pts',(4.37207647916042,5.16801531114477,90.5791764321836));
#206005=CARTESIAN_POINT('Ctrl Pts',(4.23441539124735,5.2784481899861,90.587490510018));
#206006=CARTESIAN_POINT('Ctrl Pts',(4.09666738435227,5.38895079596351,90.5958098373474));
#206007=CARTESIAN_POINT('Ctrl Pts',(3.95470008203291,5.493970557266,90.6041291646767));
#206008=CARTESIAN_POINT('Ctrl Pts',(3.80899387004078,5.59319718032467,90.6124484920061));
#206009=CARTESIAN_POINT('Ctrl Pts',(3.66308419770517,5.6925623608445,90.6207794362265));
#206010=CARTESIAN_POINT('Ctrl Pts',(3.51342547851905,5.78611805558909,90.629110380447));
#206011=CARTESIAN_POINT('Ctrl Pts',(3.36052415939679,5.87359909885843,90.6374413246674));
#206012=CARTESIAN_POINT('Ctrl Pts',(3.27438251317608,5.92288422683237,90.6421348175283));
#206013=CARTESIAN_POINT('Ctrl Pts',(3.18721208119283,5.97024212636128,90.6468283103892));
#206014=CARTESIAN_POINT('Ctrl Pts',(3.09910619832126,6.01563211736944,90.6515218032501));
#206015=CARTESIAN_POINT('Origin',(0.,0.,4.30282021618968));
#206016=CARTESIAN_POINT('',(3.09910619832149,6.01563211736932,93.0457552630241));
#206017=CARTESIAN_POINT('',(3.09910619832136,6.01563211736939,92.6514522942042));
#206018=CARTESIAN_POINT('',(3.09910619832133,6.0156321173694,4.30282021618968));
#206019=CARTESIAN_POINT('',(-6.76729221817928,0.000612721246602595,91.6966736401472));
#206020=CARTESIAN_POINT('Ctrl Pts',(-6.767,3.66969153868988E-12,91.6971797838099));
#206021=CARTESIAN_POINT('Ctrl Pts',(-6.7670000000001,-0.186007249523421,
91.7059292956211));
#206022=CARTESIAN_POINT('Ctrl Pts',(-6.75932637294539,-0.372014355746692,
91.7146788074323));
#206023=CARTESIAN_POINT('Ctrl Pts',(-6.74400518264205,-0.557389537484492,
91.7234283192435));
#206024=CARTESIAN_POINT('Ctrl Pts',(-6.72868405705117,-0.742763936248965,
91.7321777940992));
#206025=CARTESIAN_POINT('Ctrl Pts',(-6.70571545645762,-0.927506130239609,
91.7409272689548));
#206026=CARTESIAN_POINT('Ctrl Pts',(-6.67517739404842,-1.11098863989912,
91.7496767438105));
#206027=CARTESIAN_POINT('Ctrl Pts',(-6.64463945808718,-1.29447038981863,
91.7584261824375));
#206028=CARTESIAN_POINT('Ctrl Pts',(-6.60653217008369,-1.47669218313621,
91.7671756210645));
#206029=CARTESIAN_POINT('Ctrl Pts',(-6.56098496092688,-1.65703510599243,
91.7759250596916));
#206030=CARTESIAN_POINT('Ctrl Pts',(-6.51543793658307,-1.83737729708665,
91.7846744628167));
#206031=CARTESIAN_POINT('Ctrl Pts',(-6.46245112167429,-2.01584035510899,
91.7934238659419));
#206032=CARTESIAN_POINT('Ctrl Pts',(-6.4022044837426,-2.19181813760771,
91.8021732690671));
#206033=CARTESIAN_POINT('Ctrl Pts',(-6.34195808526513,-2.36779522067117,
91.8109226374172));
#206034=CARTESIAN_POINT('Ctrl Pts',(-6.27445201433117,-2.54128677684134,
91.8196720057673));
#206035=CARTESIAN_POINT('Ctrl Pts',(-6.19991555071918,-2.71170355384774,
91.8284213741174));
#206036=CARTESIAN_POINT('Ctrl Pts',(-6.12537937716706,-2.88211966767448,
91.8371707084192));
#206037=CARTESIAN_POINT('Ctrl Pts',(-6.04381298052531,-3.04946076371764,
91.8459200427209));
#206038=CARTESIAN_POINT('Ctrl Pts',(-5.95549339335839,-3.21315848374533,
91.8546693770227));
#206039=CARTESIAN_POINT('Ctrl Pts',(-5.86717414255426,-3.37685558033461,
91.8634186780029));
#206040=CARTESIAN_POINT('Ctrl Pts',(-5.77210188876627,-3.53690907646709,
91.8721679789831));
#206041=CARTESIAN_POINT('Ctrl Pts',(-5.67059953347037,-3.69277536969223,
91.8809172799633));
#206042=CARTESIAN_POINT('Ctrl Pts',(-5.56909755631429,-3.84864108224858,
91.8896665483485));
#206043=CARTESIAN_POINT('Ctrl Pts',(-5.46116568196899,-4.0003193829745,
91.8984158167338));
#206044=CARTESIAN_POINT('Ctrl Pts',(-5.34717048533656,-4.14729511859786,
91.9071650851191));
#206045=CARTESIAN_POINT('Ctrl Pts',(-5.23317570391898,-4.29427031887841,
91.9159143216361));
#206046=CARTESIAN_POINT('Ctrl Pts',(-5.11311782003584,-4.43654276189466,
91.9246635581532));
#206047=CARTESIAN_POINT('Ctrl Pts',(-4.98740458984832,-4.57362924351766,
91.9334127946702));
#206048=CARTESIAN_POINT('Ctrl Pts',(-4.86169180711831,-4.71071523720176,
91.9421620000456));
#206049=CARTESIAN_POINT('Ctrl Pts',(-4.73032391204268,-4.84261509523143,
91.9509112054211));
#206050=CARTESIAN_POINT('Ctrl Pts',(-4.59374707013705,-4.96888084538231,
91.9596604107965));
#206051=CARTESIAN_POINT('Ctrl Pts',(-4.45717070301551,-5.09514615659371,
91.968409585757));
#206052=CARTESIAN_POINT('Ctrl Pts',(-4.31538563571146,-5.21577720459441,
91.9771587607174));
#206053=CARTESIAN_POINT('Ctrl Pts',(-4.16887341029613,-5.33036429232806,
91.9859079356779));
#206054=CARTESIAN_POINT('Ctrl Pts',(-4.02236168203806,-5.44495099123543,
91.9946570809499));
#206055=CARTESIAN_POINT('Ctrl Pts',(-3.87112305348261,-5.55349359438535,
92.0034062262219));
#206056=CARTESIAN_POINT('Ctrl Pts',(-3.71567117017851,-5.65562346298834,
92.0121553714939));
#206057=CARTESIAN_POINT('Ctrl Pts',(-3.56021980145912,-5.75775299351586,
92.0209044878041));
#206058=CARTESIAN_POINT('Ctrl Pts',(-3.40055544538445,-5.85346967463817,
92.0296536041143));
#206059=CARTESIAN_POINT('Ctrl Pts',(-3.23722035986952,-5.94244842986847,
92.0384027204244));
#206060=CARTESIAN_POINT('Ctrl Pts',(-3.07388580147277,-6.03142689794479,
92.0471518084993));
#206061=CARTESIAN_POINT('Ctrl Pts',(-2.90688078896673,-6.11366734656736,
92.0559008965741));
#206062=CARTESIAN_POINT('Ctrl Pts',(-2.73677250721463,-6.18889046952313,
92.064649984649));
#206063=CARTESIAN_POINT('Ctrl Pts',(-2.56666476031568,-6.26411335596292,
92.073399045215));
#206064=CARTESIAN_POINT('Ctrl Pts',(-2.39345402575245,-6.33231884500526,
92.082148105781));
#206065=CARTESIAN_POINT('Ctrl Pts',(-2.21772856065664,-6.39327529762702,
92.0908971663471));
#206066=CARTESIAN_POINT('Ctrl Pts',(-2.0420036334856,-6.45423156365097,
92.0996462001308));
#206067=CARTESIAN_POINT('Ctrl Pts',(-1.86376426189299,-6.50793874375653,
92.1083952339145));
#206068=CARTESIAN_POINT('Ctrl Pts',(-1.68361577753148,-6.55421443909543,
92.1171442676982));
#206069=CARTESIAN_POINT('Ctrl Pts',(-1.50346782967784,-6.60048999661872,
92.125893275426));
#206070=CARTESIAN_POINT('Ctrl Pts',(-1.32141105794962,-6.63933404237718,
92.1346422831539));
#206071=CARTESIAN_POINT('Ctrl Pts',(-1.13806375486988,-6.67061465607567,
92.1433912908817));
#206072=CARTESIAN_POINT('Ctrl Pts',(-0.954716982602583,-6.70189517921303,
92.1521402732801));
#206073=CARTESIAN_POINT('Ctrl Pts',(-0.770079968901612,-6.72561226592234,
92.1608892556785));
#206074=CARTESIAN_POINT('Ctrl Pts',(-0.584779765557624,-6.74168536983108,
92.1696382380769));
#206075=CARTESIAN_POINT('Ctrl Pts',(-0.391489830650703,-6.75845151013856,
92.1787644570868));
#206076=CARTESIAN_POINT('Ctrl Pts',(-0.197478578237765,-6.76689983031627,
92.1878906760966));
#206077=CARTESIAN_POINT('Ctrl Pts',(-0.00346287645080042,-6.76699911397118,
92.1970168951065));
#206078=CARTESIAN_POINT('Ctrl Pts',(0.184489834655289,-6.76709529501187,
92.2058579197723));
#206079=CARTESIAN_POINT('Ctrl Pts',(0.372446404250735,-6.75935639738161,
92.2146989444381));
#206080=CARTESIAN_POINT('Ctrl Pts',(0.559755019489661,-6.74380925873175,
92.2235399691039));
#206081=CARTESIAN_POINT('Ctrl Pts',(0.745134705523179,-6.7284222265979,
92.2322899477137));
#206082=CARTESIAN_POINT('Ctrl Pts',(0.929879431230048,-6.70538706057503,
92.2410399263234));
#206083=CARTESIAN_POINT('Ctrl Pts',(1.11336163626981,-6.67478200894101,
92.2497899049332));
#206084=CARTESIAN_POINT('Ctrl Pts',(1.2968419630089,-6.6441772706098,92.2585397939697));
#206085=CARTESIAN_POINT('Ctrl Pts',(1.47905951217697,-6.60600284890549,
92.2672896830062));
#206086=CARTESIAN_POINT('Ctrl Pts',(1.65939532067285,-6.5603884160718,92.2760395720428));
#206087=CARTESIAN_POINT('Ctrl Pts',(1.83972934301001,-6.514774435032,92.2847893744149));
#206088=CARTESIAN_POINT('Ctrl Pts',(2.01818138406461,-6.4617206606208,92.2935391767871));
#206089=CARTESIAN_POINT('Ctrl Pts',(2.19414528354394,-6.40140730423412,
92.3022889791592));
#206090=CARTESIAN_POINT('Ctrl Pts',(2.37010749864179,-6.34109452518575,
92.3110386977756));
#206091=CARTESIAN_POINT('Ctrl Pts',(2.54358134866624,-6.27352239616437,
92.3197884163919));
#206092=CARTESIAN_POINT('Ctrl Pts',(2.71397759435706,-6.19892043966753,
92.3285381350082));
#206093=CARTESIAN_POINT('Ctrl Pts',(2.88437226558266,-6.12431917249448,
92.3372877727769));
#206094=CARTESIAN_POINT('Ctrl Pts',(3.0516891268109,-6.04268832278731,92.3460374105456));
#206095=CARTESIAN_POINT('Ctrl Pts',(3.21535986273981,-5.95430516123266,
92.3547870483143));
#206096=CARTESIAN_POINT('Ctrl Pts',(3.37902914072971,-5.86592278697366,
92.3635366081434));
#206097=CARTESIAN_POINT('Ctrl Pts',(3.53905210621704,-5.77078835741861,
92.3722861679724));
#206098=CARTESIAN_POINT('Ctrl Pts',(3.69488522831831,-5.66922500431542,
92.3810357278015));
#206099=CARTESIAN_POINT('Ctrl Pts',(3.85071701407076,-5.56766252216999,
92.3897852125986));
#206100=CARTESIAN_POINT('Ctrl Pts',(4.00235878822542,-5.45967138329269,
92.3985346973957));
#206101=CARTESIAN_POINT('Ctrl Pts',(4.14929549611464,-5.34561838199499,
92.4072841821929));
#206102=CARTESIAN_POINT('Ctrl Pts',(4.29623099276231,-5.231566320869,92.4160335948655));
#206103=CARTESIAN_POINT('Ctrl Pts',(4.43846127436171,-5.1114526730484,92.424783007538));
#206104=CARTESIAN_POINT('Ctrl Pts',(4.57550326054586,-4.98568540049753,
92.4335324202106));
#206105=CARTESIAN_POINT('Ctrl Pts',(4.71254416257918,-4.85991912290227,
92.4422817636659));
#206106=CARTESIAN_POINT('Ctrl Pts',(4.84439664018891,-4.72849950385285,
92.4510311071211));
#206107=CARTESIAN_POINT('Ctrl Pts',(4.97061286794868,-4.59187289860934,
92.4597804505764));
#206108=CARTESIAN_POINT('Ctrl Pts',(5.09682813912806,-4.45524732884546,
92.4685297277212));
#206109=CARTESIAN_POINT('Ctrl Pts',(5.21740705147959,-4.31341506235642,
92.477279004866));
#206110=CARTESIAN_POINT('Ctrl Pts',(5.33194007545814,-4.16685781275573,
92.4860282820109));
#206111=CARTESIAN_POINT('Ctrl Pts',(5.44647226944594,-4.02030162521694,
92.494777495752));
#206112=CARTESIAN_POINT('Ctrl Pts',(5.55495848628212,-3.86902074887791,
92.5035267094931));
#206113=CARTESIAN_POINT('Ctrl Pts',(5.65703027291878,-3.71352898080525,
92.5122759232342));
#206114=CARTESIAN_POINT('Ctrl Pts',(5.75910135377082,-3.5580382878945,92.5210250764781));
#206115=CARTESIAN_POINT('Ctrl Pts',(5.85475793592832,-3.39833700106574,
92.529774229722));
#206116=CARTESIAN_POINT('Ctrl Pts',(5.94367514427473,-3.23496750823416,
92.5385233829659));
#206117=CARTESIAN_POINT('Ctrl Pts',(6.03259176732709,-3.07159909077588,
92.5472724786188));
#206118=CARTESIAN_POINT('Ctrl Pts',(6.11476896835988,-2.90456276731299,
92.5560215742717));
#206119=CARTESIAN_POINT('Ctrl Pts',(6.18992765547945,-2.73442583002917,
92.5647706699247));
#206120=CARTESIAN_POINT('Ctrl Pts',(6.26508587283112,-2.56428995616029,
92.5735197108927));
#206121=CARTESIAN_POINT('Ctrl Pts',(6.33322554827217,-2.39105376935052,
92.5822687518607));
#206122=CARTESIAN_POINT('Ctrl Pts',(6.39411526733085,-2.21530561053922,
92.5910177928288));
#206123=CARTESIAN_POINT('Ctrl Pts',(6.45500462602899,-2.03955849184935,
92.5997667820178));
#206124=CARTESIAN_POINT('Ctrl Pts',(6.50864402040788,-1.86129970164377,
92.6085157712068));
#206125=CARTESIAN_POINT('Ctrl Pts',(6.55485128368645,-1.68113463135886,
92.6172647603958));
#206126=CARTESIAN_POINT('Ctrl Pts',(6.60199809554361,-1.49730620116717,
92.6261916458673));
#206127=CARTESIAN_POINT('Ctrl Pts',(6.64140720707899,-1.31149343245567,
92.6351185313387));
#206128=CARTESIAN_POINT('Ctrl Pts',(6.67293928722902,-1.12435326697415,
92.6440454168101));
#206129=CARTESIAN_POINT('Ctrl Pts',(6.70384625876272,-0.940923067005509,
92.6527953309876));
#206130=CARTESIAN_POINT('Ctrl Pts',(6.72718554579808,-0.756217899520606,
92.661545245165));
#206131=CARTESIAN_POINT('Ctrl Pts',(6.74287786815337,-0.570865181253461,
92.6702951593425));
#206132=CARTESIAN_POINT('Ctrl Pts',(6.75856988190851,-0.38551610807298,
92.679044901447));
#206133=CARTESIAN_POINT('Ctrl Pts',(6.76661520773405,-0.199519795225453,
92.6877946435514));
#206134=CARTESIAN_POINT('Ctrl Pts',(6.76698651789579,-0.0135080204548247,
92.6965443856559));
#206135=CARTESIAN_POINT('Ctrl Pts',(6.76735782124901,0.172500343513712,
92.7052939673209));
#206136=CARTESIAN_POINT('Ctrl Pts',(6.7600553899518,0.358523882211601,92.7140435489859));
#206137=CARTESIAN_POINT('Ctrl Pts',(6.74510402742356,0.543930748564983,
92.7227931306508));
#206138=CARTESIAN_POINT('Ctrl Pts',(6.73015291918024,0.729334461615836,
92.7315425635075));
#206139=CARTESIAN_POINT('Ctrl Pts',(6.70755316306587,0.914121237635275,
92.7402919963642));
#206140=CARTESIAN_POINT('Ctrl Pts',(6.67738151874565,1.09766345166181,92.7490414292209));
#206141=CARTESIAN_POINT('Ctrl Pts',(6.64721034747558,1.28120278799723,92.7577907248984));
#206142=CARTESIAN_POINT('Ctrl Pts',(6.60946757205129,1.46349731860387,92.766540020576));
#206143=CARTESIAN_POINT('Ctrl Pts',(6.56428138111508,1.64392790278219,92.7752893162535));
#206144=CARTESIAN_POINT('Ctrl Pts',(6.51909583859835,1.82435589779109,92.7840384863791));
#206145=CARTESIAN_POINT('Ctrl Pts',(6.4664671639286,2.00291972192314,92.7927876565047));
#206146=CARTESIAN_POINT('Ctrl Pts',(6.40657409872868,2.17901292274708,92.8015368266303));
#206147=CARTESIAN_POINT('Ctrl Pts',(6.34668181342061,2.35510383059019,92.8102858828294));
#206148=CARTESIAN_POINT('Ctrl Pts',(6.27952541914034,2.52872390822619,92.8190349390285));
#206149=CARTESIAN_POINT('Ctrl Pts',(6.20533299175501,2.69928350890322,92.8277839952276));
#206150=CARTESIAN_POINT('Ctrl Pts',(6.12831602991533,2.87633637965657,92.8368661313858));
#206151=CARTESIAN_POINT('Ctrl Pts',(6.04371690605255,3.05009086601493,92.845948267544));
#206152=CARTESIAN_POINT('Ctrl Pts',(5.95184520316616,3.21991112882762,92.8550304037022));
#206153=CARTESIAN_POINT('Ctrl Pts',(5.86333549509257,3.38351691183047,92.8637801840457));
#206154=CARTESIAN_POINT('Ctrl Pts',(5.76807618099349,3.54347103712036,92.8725299643893));
#206155=CARTESIAN_POINT('Ctrl Pts',(5.66639083308994,3.69923018027729,92.8812797447329));
#206156=CARTESIAN_POINT('Ctrl Pts',(5.56470914082181,3.85498372382078,92.8900292105178));
#206157=CARTESIAN_POINT('Ctrl Pts',(5.45660203372051,4.00654234702019,92.8987786763027));
#206158=CARTESIAN_POINT('Ctrl Pts',(5.34243669839204,4.15339127986684,92.9075281420876));
#206159=CARTESIAN_POINT('Ctrl Pts',(5.22827486050581,4.30023571401292,92.9162773398336));
#206160=CARTESIAN_POINT('Ctrl Pts',(5.10805534167103,4.44237052028479,92.9250265375796));
#206161=CARTESIAN_POINT('Ctrl Pts',(4.98218644339946,4.57931296628727,92.9337757353256));
#206162=CARTESIAN_POINT('Ctrl Pts',(4.85632073219587,4.7162519448336,92.9425247115373));
#206163=CARTESIAN_POINT('Ctrl Pts',(4.72480612170326,4.84799861524501,92.9512736877489));
#206164=CARTESIAN_POINT('Ctrl Pts',(4.58808925235326,4.97410554898472,92.9600226639605));
#206165=CARTESIAN_POINT('Ctrl Pts',(4.45136349474066,5.10022068121191,92.9687722089622));
#206166=CARTESIAN_POINT('Ctrl Pts',(4.30943501210102,5.22069514871816,92.9775217539639));
#206167=CARTESIAN_POINT('Ctrl Pts',(4.16278587431808,5.33511975166237,92.9862712989656));
#206168=CARTESIAN_POINT('Ctrl Pts',(4.01614535740469,5.44953762807827,92.9950203296194));
#206169=CARTESIAN_POINT('Ctrl Pts',(3.8647849665794,5.55790617532772,93.0037693602731));
#206170=CARTESIAN_POINT('Ctrl Pts',(3.70921874747207,5.65985735539349,93.0125183909268));
#206171=CARTESIAN_POINT('Ctrl Pts',(3.55365041605906,5.76180991977043,93.0212675403765));
#206172=CARTESIAN_POINT('Ctrl Pts',(3.39387638174522,5.85734478552814,93.0300166898261));
#206173=CARTESIAN_POINT('Ctrl Pts',(3.23043927904532,5.94613749121236,93.0387658392757));
#206174=CARTESIAN_POINT('Ctrl Pts',(3.18691767070429,5.96978206944148,93.0410956471919));
#206175=CARTESIAN_POINT('Ctrl Pts',(3.14313645919635,5.99294880633423,93.043425455108));
#206176=CARTESIAN_POINT('Ctrl Pts',(3.09910619832149,6.01563211736932,93.0457552630241));
#206177=CARTESIAN_POINT('Ctrl Pts',(3.09910619832119,6.01563211736948,91.0458502363996));
#206178=CARTESIAN_POINT('Ctrl Pts',(2.9398956747614,6.09765347618519,91.0542757770372));
#206179=CARTESIAN_POINT('Ctrl Pts',(2.77736701447553,6.17338133629389,91.0627013176748));
#206180=CARTESIAN_POINT('Ctrl Pts',(2.61204730635548,6.24255539577833,91.0711268583124));
#206181=CARTESIAN_POINT('Ctrl Pts',(2.44677049905691,6.31171150444485,91.079550212504));
#206182=CARTESIAN_POINT('Ctrl Pts',(2.27870439445777,6.374317072692,91.0879735666956));
#206183=CARTESIAN_POINT('Ctrl Pts',(2.10839732830607,6.43015938418262,91.0963969208872));
#206184=CARTESIAN_POINT('Ctrl Pts',(1.93811414965261,6.4859938631555,91.1048190936078));
#206185=CARTESIAN_POINT('Ctrl Pts',(1.76559095281422,6.5350668725321,91.1132412663284));
#206186=CARTESIAN_POINT('Ctrl Pts',(1.59139286804078,6.5772150443443,91.121663439049));
#206187=CARTESIAN_POINT('Ctrl Pts',(1.4171948994209,6.61936318805251,91.1300856061537));
#206188=CARTESIAN_POINT('Ctrl Pts',(1.24132236927861,6.65458642527241,91.1385077732585));
#206189=CARTESIAN_POINT('Ctrl Pts',(1.06435263838302,6.6827720641338,91.1469299403633));
#206190=CARTESIAN_POINT('Ctrl Pts',(0.887358321108872,6.71096161882183,
91.1553532775585));
#206191=CARTESIAN_POINT('Ctrl Pts',(0.709266828560109,6.73211157397049,
91.1637766147537));
#206192=CARTESIAN_POINT('Ctrl Pts',(0.530663084433825,6.74616081121842,
91.1721999519489));
#206193=CARTESIAN_POINT('Ctrl Pts',(0.351940488742354,6.76021939750797,
91.1806288944399));
#206194=CARTESIAN_POINT('Ctrl Pts',(0.172705293067564,6.76716779651611,
91.1890578369308));
#206195=CARTESIAN_POINT('Ctrl Pts',(-0.00645406409859743,6.76699692219943,
91.1974867794218));
#206196=CARTESIAN_POINT('Ctrl Pts',(-0.185672892685407,6.76682599116153,
91.2059185198754));
#206197=CARTESIAN_POINT('Ctrl Pts',(-0.364815499032925,6.75953108099326,
91.2143502603289));
#206198=CARTESIAN_POINT('Ctrl Pts',(-0.543295520171679,6.74515522265881,
91.2227820007825));
#206199=CARTESIAN_POINT('Ctrl Pts',(-0.721947152431176,6.73076554172873,
91.2312218484764));
#206200=CARTESIAN_POINT('Ctrl Pts',(-0.89993459407557,6.7092813395262,91.2396616961704));
#206201=CARTESIAN_POINT('Ctrl Pts',(-1.07667744414064,6.68079745848344,
91.2481015438643));
#206202=CARTESIAN_POINT('Ctrl Pts',(-1.21150496096729,6.65906865333423,
91.254539845083));
#206203=CARTESIAN_POINT('Ctrl Pts',(-1.34560832735392,6.63326756376359,
91.2609781463017));
#206204=CARTESIAN_POINT('Ctrl Pts',(-1.47873466302166,6.6034561251195,91.2674164475204));
#206205=CARTESIAN_POINT('Ctrl Pts',(-1.64704155002527,6.56576658450292,
91.2755561625533));
#206206=CARTESIAN_POINT('Ctrl Pts',(-1.81412186111606,6.52158998995999,
91.2836958775862));
#206207=CARTESIAN_POINT('Ctrl Pts',(-1.97943381462411,6.47102239012682,
91.2918355926191));
#206208=CARTESIAN_POINT('Ctrl Pts',(-2.14460118729004,6.4204990164129,91.2999681887061));
#206209=CARTESIAN_POINT('Ctrl Pts',(-2.30800293306743,6.36359586973028,
91.3081007847931));
#206210=CARTESIAN_POINT('Ctrl Pts',(-2.4691078287673,6.30045994590237,91.31623338088));
#206211=CARTESIAN_POINT('Ctrl Pts',(-2.63010258451681,6.23736718517938,
91.324360417088));
#206212=CARTESIAN_POINT('Ctrl Pts',(-2.78880327691345,6.16805026393771,
91.332487453296));
#206213=CARTESIAN_POINT('Ctrl Pts',(-2.94469425532868,6.0927058637878,91.3406144895039));
#206214=CARTESIAN_POINT('Ctrl Pts',(-3.10051071503471,6.01739747962485,
91.3487376408415));
#206215=CARTESIAN_POINT('Ctrl Pts',(-3.25351980628306,5.93606751307471,
91.3568607921791));
#206216=CARTESIAN_POINT('Ctrl Pts',(-3.4032262897393,5.84896057610472,91.3649839435167));
#206217=CARTESIAN_POINT('Ctrl Pts',(-3.55289070456197,5.76187811683088,
91.3731048121884));
#206218=CARTESIAN_POINT('Ctrl Pts',(-3.69925404424552,5.66902210526866,
91.3812256808601));
#206219=CARTESIAN_POINT('Ctrl Pts',(-3.84184613011026,5.57068284077965,
91.3893465495319));
#206220=CARTESIAN_POINT('Ctrl Pts',(-3.98444592219597,5.47233826166117,
91.3974678570864));
#206221=CARTESIAN_POINT('Ctrl Pts',(-4.12327374954491,5.36851004223815,
91.4055891646408));
#206222=CARTESIAN_POINT('Ctrl Pts',(-4.25788871121837,5.25953160679534,
91.4137104721953));
#206223=CARTESIAN_POINT('Ctrl Pts',(-4.32783932476428,5.20290262345106,
91.417930585912));
#206224=CARTESIAN_POINT('Ctrl Pts',(-4.39665288973983,5.14488366640152,
91.4221506996287));
#206225=CARTESIAN_POINT('Ctrl Pts',(-4.46427107342832,5.08552581184593,
91.4263708133454));
#206226=CARTESIAN_POINT('Ctrl Pts',(-4.60822724507752,4.95915552159235,
91.4353552518713));
#206227=CARTESIAN_POINT('Ctrl Pts',(-4.74669213064618,4.82677724828876,
91.4443396903972));
#206228=CARTESIAN_POINT('Ctrl Pts',(-4.87920862823121,4.68888176031281,
91.4533241289231));
#206229=CARTESIAN_POINT('Ctrl Pts',(-5.01195384138075,4.55074827295602,
91.4623240740535));
#206230=CARTESIAN_POINT('Ctrl Pts',(-5.13872998085703,4.40707871057319,
91.471324019184));
#206231=CARTESIAN_POINT('Ctrl Pts',(-5.25911933895199,4.25839791220375,
91.4803239643144));
#206232=CARTESIAN_POINT('Ctrl Pts',(-5.37979239766028,4.10936674371559,
91.4893451180467));
#206233=CARTESIAN_POINT('Ctrl Pts',(-5.49404841016782,3.95530089760421,
91.4983662717789));
#206234=CARTESIAN_POINT('Ctrl Pts',(-5.60151061891099,3.7967575358755,91.5073874255112));
#206235=CARTESIAN_POINT('Ctrl Pts',(-5.70908217129881,3.63805285502625,
91.5164177583384));
#206236=CARTESIAN_POINT('Ctrl Pts',(-5.80984598096192,3.47486175796944,
91.5254480911657));
#206237=CARTESIAN_POINT('Ctrl Pts',(-5.90346983463317,3.30776856983317,
91.534478423993));
#206238=CARTESIAN_POINT('Ctrl Pts',(-5.99722641741692,3.14043849622708,
91.5435215589857));
#206239=CARTESIAN_POINT('Ctrl Pts',(-6.08382268774475,2.96919547887985,
91.5525646939784));
#206240=CARTESIAN_POINT('Ctrl Pts',(-6.16297235725555,2.79464858680014,
91.5616078289711));
#206241=CARTESIAN_POINT('Ctrl Pts',(-6.23216740342193,2.64205438987798,
91.5695136123708));
#206242=CARTESIAN_POINT('Ctrl Pts',(-6.29567185242913,2.48693553989782,
91.5774193957705));
#206243=CARTESIAN_POINT('Ctrl Pts',(-6.35332481091421,2.3297108934419,91.5853251791702));
#206244=CARTESIAN_POINT('Ctrl Pts',(-6.42129982523422,2.14433710040292,
91.5946463962235));
#206245=CARTESIAN_POINT('Ctrl Pts',(-6.48119410585874,1.9558845786944,91.6039676132768));
#206246=CARTESIAN_POINT('Ctrl Pts',(-6.53275243902799,1.76505936737944,
91.61328883033));
#206247=CARTESIAN_POINT('Ctrl Pts',(-6.58166644677203,1.58402120554867,
91.6221319805078));
#206248=CARTESIAN_POINT('Ctrl Pts',(-6.62307798233069,1.40084792773441,
91.6309751306855));
#206249=CARTESIAN_POINT('Ctrl Pts',(-6.65681923776214,1.21616061264945,
91.6398182808632));
#206250=CARTESIAN_POINT('Ctrl Pts',(-6.69052569194362,1.03166378690272,
91.6486523100798));
#206251=CARTESIAN_POINT('Ctrl Pts',(-6.71657759937819,0.845656305320527,
91.6574863392965));
#206252=CARTESIAN_POINT('Ctrl Pts',(-6.73485780107018,0.658771128210807,
91.6663203685131));
#206253=CARTESIAN_POINT('Ctrl Pts',(-6.75311200586027,0.472151726922313,
91.6751418345537));
#206254=CARTESIAN_POINT('Ctrl Pts',(-6.7636165360224,0.284657390739837,
91.6839633005943));
#206255=CARTESIAN_POINT('Ctrl Pts',(-6.76630578097467,0.0969282123470912,
91.6927847666349));
#206256=CARTESIAN_POINT('Ctrl Pts',(-6.76675239146241,0.0657514986545169,
91.6942497723599));
#206257=CARTESIAN_POINT('Ctrl Pts',(-6.76698357027965,0.0345683247144677,
91.6957147780849));
#206258=CARTESIAN_POINT('Ctrl Pts',(-6.76699915505439,0.00338164061046775,
91.6971797838099));
#206259=CARTESIAN_POINT('',(-6.7669999994732,-8.44378501004791E-5,91.3028202161459));
#206260=CARTESIAN_POINT('Ctrl Pts',(3.09910619832126,6.01563211736944,90.6515218032501));
#206261=CARTESIAN_POINT('Ctrl Pts',(3.06939383950441,6.03093919625649,90.6531046117919));
#206262=CARTESIAN_POINT('Ctrl Pts',(3.03957510944118,6.04602251175088,90.6546874203336));
#206263=CARTESIAN_POINT('Ctrl Pts',(3.00965363156952,6.06088063056685,90.6562702288754));
#206264=CARTESIAN_POINT('Ctrl Pts',(2.85710093032343,6.13663377920923,90.6643400748781));
#206265=CARTESIAN_POINT('Ctrl Pts',(2.70140454992178,6.20676334665172,90.6724099208809));
#206266=CARTESIAN_POINT('Ctrl Pts',(2.54302590332117,6.27098941595643,90.6804797668836));
#206267=CARTESIAN_POINT('Ctrl Pts',(2.38484651720289,6.33513468069675,90.6885394599937));
#206268=CARTESIAN_POINT('Ctrl Pts',(2.22399192081392,6.39339108726076,90.6965991531037));
#206269=CARTESIAN_POINT('Ctrl Pts',(2.06094945812464,6.44552374373532,90.7046588462138));
#206270=CARTESIAN_POINT('Ctrl Pts',(1.89807634092915,6.49760225216582,90.7127101680524));
#206271=CARTESIAN_POINT('Ctrl Pts',(1.73302023197066,6.54356955527737,90.720761489891));
#206272=CARTESIAN_POINT('Ctrl Pts',(1.56628977029931,6.58323821196345,90.7288128117296));
#206273=CARTESIAN_POINT('Ctrl Pts',(1.39969594836909,6.6228743592033,90.7368575353107));
#206274=CARTESIAN_POINT('Ctrl Pts',(1.23143086590423,6.6562220479362,90.7449022588917));
#206275=CARTESIAN_POINT('Ctrl Pts',(1.0620195938675,6.68314322622533,90.7529469824727));
#206276=CARTESIAN_POINT('Ctrl Pts',(0.892710074361159,6.71004823500001,
90.7609868741971));
#206277=CARTESIAN_POINT('Ctrl Pts',(0.7222561032782,6.73053435882903,90.7690267659215));
#206278=CARTESIAN_POINT('Ctrl Pts',(0.551194145090353,6.74451436460907,
90.7770666576459));
#206279=CARTESIAN_POINT('Ctrl Pts',(0.376448754287485,6.75879539821432,
90.7852796702659));
#206280=CARTESIAN_POINT('Ctrl Pts',(0.201069283828813,6.76628685388274,
90.7934926828858));
#206281=CARTESIAN_POINT('Ctrl Pts',(0.0256349535357023,6.76695144427365,
90.8017056955058));
#206282=CARTESIAN_POINT('Ctrl Pts',(-0.146041501907251,6.76760179886755,
90.8097427820483));
#206283=CARTESIAN_POINT('Ctrl Pts',(-0.317770101994881,6.7617148055548,
90.8177798685909));
#206284=CARTESIAN_POINT('Ctrl Pts',(-0.489006855450561,6.74930820864793,
90.8258169551335));
#206285=CARTESIAN_POINT('Ctrl Pts',(-0.660259997060672,6.73690042437198,
90.8338548108626));
#206286=CARTESIAN_POINT('Ctrl Pts',(-0.831020825641169,6.71797182097387,
90.8418926665918));
#206287=CARTESIAN_POINT('Ctrl Pts',(-1.0007496397776,6.69259211057159,90.849930522321));
#206288=CARTESIAN_POINT('Ctrl Pts',(-1.1705283266965,6.66720494264488,90.8579707398779));
#206289=CARTESIAN_POINT('Ctrl Pts',(-1.33927402626337,6.63536294985121,
90.8660109574349));
#206290=CARTESIAN_POINT('Ctrl Pts',(-1.5064565559803,6.59718710095022,90.8740511749918));
#206291=CARTESIAN_POINT('Ctrl Pts',(-1.67995534878654,6.55756894401786,
90.8823951571196));
#206292=CARTESIAN_POINT('Ctrl Pts',(-1.85177011566018,6.51112908758498,
90.8907391392473));
#206293=CARTESIAN_POINT('Ctrl Pts',(-2.02132588847267,6.45805935653972,
90.8990831213751));
#206294=CARTESIAN_POINT('Ctrl Pts',(-2.18499337958725,6.40683261509513,
90.9071373362101));
#206295=CARTESIAN_POINT('Ctrl Pts',(-2.34655582124598,6.34942894572099,
90.9151915510452));
#206296=CARTESIAN_POINT('Ctrl Pts',(-2.50551733007726,6.28606967100131,
90.9232457658803));
#206297=CARTESIAN_POINT('Ctrl Pts',(-2.66459779531212,6.22266298234156,
90.9313060079633));
#206298=CARTESIAN_POINT('Ctrl Pts',(-2.82107311305556,6.15329196468001,
90.9393662500463));
#206299=CARTESIAN_POINT('Ctrl Pts',(-2.97447219276308,6.07822376804928,
90.9474264921293));
#206300=CARTESIAN_POINT('Ctrl Pts',(-3.12808573490635,6.00305062093041,
90.9554980029836));
#206301=CARTESIAN_POINT('Ctrl Pts',(-3.27861413220835,5.92216457836578,
90.963569513838));
#206302=CARTESIAN_POINT('Ctrl Pts',(-3.4256149483357,5.83587621747917,90.9716410246923));
#206303=CARTESIAN_POINT('Ctrl Pts',(-3.44102216867744,5.82683229633553,
90.9724870033032));
#206304=CARTESIAN_POINT('Ctrl Pts',(-3.45639066779913,5.81772906586434,
90.973332981914));
#206305=CARTESIAN_POINT('Ctrl Pts',(-3.47171995776792,5.80856690887141,
90.9741789605249));
#206306=CARTESIAN_POINT('Ctrl Pts',(-3.62083549545187,5.71944210471361,
90.9824082102609));
#206307=CARTESIAN_POINT('Ctrl Pts',(-3.76673597130493,5.62444058443306,
90.9906374599968));
#206308=CARTESIAN_POINT('Ctrl Pts',(-3.90892657006052,5.5238195182206,90.9988667097328));
#206309=CARTESIAN_POINT('Ctrl Pts',(-4.05094793887191,5.42331820744605,
91.0070861653229));
#206310=CARTESIAN_POINT('Ctrl Pts',(-4.18926793260898,5.3172108734082,91.0153056209129));
#206311=CARTESIAN_POINT('Ctrl Pts',(-4.32341688020288,5.20580017672373,
91.0235250765029));
#206312=CARTESIAN_POINT('Ctrl Pts',(-4.45743310913498,5.09449970288364,
91.0317364002726));
#206313=CARTESIAN_POINT('Ctrl Pts',(-4.58728623588905,4.97790654285264,
91.0399477240422));
#206314=CARTESIAN_POINT('Ctrl Pts',(-4.71253604220504,4.85636623937266,
91.0481590478119));
#206315=CARTESIAN_POINT('Ctrl Pts',(-4.8376870782683,4.73492178088313,91.056363896246));
#206316=CARTESIAN_POINT('Ctrl Pts',(-4.95824176799382,4.60853819793749,
91.0645687446801));
#206317=CARTESIAN_POINT('Ctrl Pts',(-5.07379337674746,4.47760089446052,
91.0727735931142));
#206318=CARTESIAN_POINT('Ctrl Pts',(-5.18927705434655,4.34674056717016,
91.0809736180341));
#206319=CARTESIAN_POINT('Ctrl Pts',(-5.29976327354346,4.21133212052189,
91.089173642954));
#206320=CARTESIAN_POINT('Ctrl Pts',(-5.40488249686137,4.07179741577618,
91.0973736678739));
#206321=CARTESIAN_POINT('Ctrl Pts',(-5.5099712962948,3.9323030955349,91.1055713195208));
#206322=CARTESIAN_POINT('Ctrl Pts',(-5.60969597518714,3.78868517966619,
91.1137689711678));
#206323=CARTESIAN_POINT('Ctrl Pts',(-5.70372745865022,3.64139836840733,
91.1219666228147));
#206324=CARTESIAN_POINT('Ctrl Pts',(-5.79774635072071,3.49413127975619,
91.1301631767458));
#206325=CARTESIAN_POINT('Ctrl Pts',(-5.88607337199358,3.34319657600585,
91.1383597306769));
#206326=CARTESIAN_POINT('Ctrl Pts',(-5.96842295158974,3.18907768342773,
91.1465562846079));
#206327=CARTESIAN_POINT('Ctrl Pts',(-6.05077647736528,3.03495140549564,
91.1547532313166));
#206328=CARTESIAN_POINT('Ctrl Pts',(-6.12715182167917,2.87764095115629,
91.1629501780253));
#206329=CARTESIAN_POINT('Ctrl Pts',(-6.19730950732372,2.7176541116255,91.171147124734));
#206330=CARTESIAN_POINT('Ctrl Pts',(-6.26748331137602,2.55763051584927,
91.1793459546538));
#206331=CARTESIAN_POINT('Ctrl Pts',(-6.33143646761472,2.39492963869119,
91.1875447845735));
#206332=CARTESIAN_POINT('Ctrl Pts',(-6.38897773375776,2.23007903840818,
91.1957436144933));
#206333=CARTESIAN_POINT('Ctrl Pts',(-6.44657349883587,2.06507230353235,
91.2039502097531));
#206334=CARTESIAN_POINT('Ctrl Pts',(-6.49774512238016,1.89791211681596,
91.2121568050129));
#206335=CARTESIAN_POINT('Ctrl Pts',(-6.54235105473117,1.72914189026173,
91.2203634002727));
#206336=CARTESIAN_POINT('Ctrl Pts',(-6.58697857660921,1.56028997795012,
91.2285739675717));
#206337=CARTESIAN_POINT('Ctrl Pts',(-6.62503399333639,1.38982682204616,
91.2367845348707));
#206338=CARTESIAN_POINT('Ctrl Pts',(-6.65642698240801,1.21830572019939,
91.2449951021697));
#206339=CARTESIAN_POINT('Ctrl Pts',(-6.68786326690575,1.04654806619846,
91.2532169930164));
#206340=CARTESIAN_POINT('Ctrl Pts',(-6.7126187097016,0.873729905530169,
91.2614388838631));
#206341=CARTESIAN_POINT('Ctrl Pts',(-6.73065479887372,0.700410578445401,
91.2696607747098));
#206342=CARTESIAN_POINT('Ctrl Pts',(-6.74705386046797,0.542822406574355,
91.2771364138647));
#206343=CARTESIAN_POINT('Ctrl Pts',(-6.75789860586077,0.384820155424103,
91.2846120530196));
#206344=CARTESIAN_POINT('Ctrl Pts',(-6.76319748642094,0.226823190325659,
91.2920876921745));
#206345=CARTESIAN_POINT('Ctrl Pts',(-6.76573329468454,0.151212878832433,
91.295665200165));
#206346=CARTESIAN_POINT('Ctrl Pts',(-6.76700094344126,0.0755668471369315,
91.2992427081555));
#206347=CARTESIAN_POINT('Ctrl Pts',(-6.7669999994732,-8.44378502934827E-5,
91.302820216146));
#206348=CARTESIAN_POINT('Ctrl Pts',(-6.76699999947319,-8.44387777600782E-5,
91.3028202161898));
#206349=CARTESIAN_POINT('Ctrl Pts',(-6.76699768248362,-0.185770078054274,
91.3116011887582));
#206350=CARTESIAN_POINT('Ctrl Pts',(-6.75934825938162,-0.371614094343413,
91.3203821613265));
#206351=CARTESIAN_POINT('Ctrl Pts',(-6.74403856800726,-0.556985451542986,
91.3291631338949));
#206352=CARTESIAN_POINT('Ctrl Pts',(-6.72875226280503,-0.742073646504984,
91.3379306931729));
#206353=CARTESIAN_POINT('Ctrl Pts',(-6.70582905174118,-0.926690340762121,
91.3466982524509));
#206354=CARTESIAN_POINT('Ctrl Pts',(-6.67530773716562,-1.11020521262372,
91.3554658117289));
#206355=CARTESIAN_POINT('Ctrl Pts',(-6.64485355501386,-1.2933164387602,
91.3642140865326));
#206356=CARTESIAN_POINT('Ctrl Pts',(-6.60683466384861,-1.47533039936832,
91.3729623613364));
#206357=CARTESIAN_POINT('Ctrl Pts',(-6.56134143433908,-1.65562301929674,
91.3817106361401));
#206358=CARTESIAN_POINT('Ctrl Pts',(-6.51590982674312,-1.83567142758392,
91.390447061149));
#206359=CARTESIAN_POINT('Ctrl Pts',(-6.4630241384197,-2.01400287093144,
91.399183486158));
#206360=CARTESIAN_POINT('Ctrl Pts',(-6.40282590211974,-2.19000216144748,
91.4079199111669));
#206361=CARTESIAN_POINT('Ctrl Pts',(-6.3427454549406,-2.36565707639755,
91.4166392417246));
#206362=CARTESIAN_POINT('Ctrl Pts',(-6.27538109980184,-2.53898867583702,
91.4253585722821));
#206363=CARTESIAN_POINT('Ctrl Pts',(-6.20092433901847,-2.70939593669297,
91.4340779028398));
#206364=CARTESIAN_POINT('Ctrl Pts',(-6.15263714409944,-2.81990958963724,
91.4397326212262));
#206365=CARTESIAN_POINT('Ctrl Pts',(-6.10136800821583,-2.92919352916704,
91.4453873396127));
#206366=CARTESIAN_POINT('Ctrl Pts',(-6.04718044105795,-3.03708704407466,
91.4510420579992));
#206367=CARTESIAN_POINT('Ctrl Pts',(-5.96851673554355,-3.19371529163704,
91.4592509724283));
#206368=CARTESIAN_POINT('Ctrl Pts',(-5.88376810752466,-3.34727700123832,
91.4674598868574));
#206369=CARTESIAN_POINT('Ctrl Pts',(-5.79321279975888,-3.49728100911406,
91.4756688012865));
#206370=CARTESIAN_POINT('Ctrl Pts',(-5.70263596292875,-3.64732067968058,
91.4838796673433));
#206371=CARTESIAN_POINT('Ctrl Pts',(-5.60624988002251,-3.79380065855253,
91.4920905334001));
#206372=CARTESIAN_POINT('Ctrl Pts',(-5.50437678694001,-3.93625776434878,
91.5003013994569));
#206373=CARTESIAN_POINT('Ctrl Pts',(-5.4024613147416,-4.07877413217403,
91.5085156812267));
#206374=CARTESIAN_POINT('Ctrl Pts',(-5.29505449192088,-4.2172640035322,
91.5167299629964));
#206375=CARTESIAN_POINT('Ctrl Pts',(-5.18251962523664,-4.35129628203333,
91.5249442447662));
#206376=CARTESIAN_POINT('Ctrl Pts',(-5.06985809167539,-4.48547942444569,
91.5331677723586));
#206377=CARTESIAN_POINT('Ctrl Pts',(-4.95205721468211,-4.61519467984284,
91.541391299951));
#206378=CARTESIAN_POINT('Ctrl Pts',(-4.82951870647705,-4.74004620903513,
91.5496148275435));
#206379=CARTESIAN_POINT('Ctrl Pts',(-4.70690165585513,-4.86497776320074,
91.5578436260971));
#206380=CARTESIAN_POINT('Ctrl Pts',(-4.57954117910739,-4.98503913308348,
91.5660724246508));
#206381=CARTESIAN_POINT('Ctrl Pts',(-4.44787296901597,-5.09987402310067,
91.5743012232045));
#206382=CARTESIAN_POINT('Ctrl Pts',(-4.31602352816969,-5.21486697415469,
91.5825413480409));
#206383=CARTESIAN_POINT('Ctrl Pts',(-4.17985478727197,-5.32461885352455,
91.5907814728773));
#206384=CARTESIAN_POINT('Ctrl Pts',(-4.03983317364497,-5.42881542595782,
91.5990215977137));
#206385=CARTESIAN_POINT('Ctrl Pts',(-3.97766935567199,-5.47507440408533,
91.6026798730838));
#206386=CARTESIAN_POINT('Ctrl Pts',(-3.91474649289734,-5.52023902595243,
91.6063381484538));
#206387=CARTESIAN_POINT('Ctrl Pts',(-3.85110698089105,-5.5642846819454,
91.6099964238239));
#206388=CARTESIAN_POINT('Ctrl Pts',(-3.70414482204787,-5.66599892343348,
91.6184444465864));
#206389=CARTESIAN_POINT('Ctrl Pts',(-3.553022930525,-5.76197564419767,91.6268924693489));
#206390=CARTESIAN_POINT('Ctrl Pts',(-3.39821706777274,-5.85187232945986,
91.6353404921115));
#206391=CARTESIAN_POINT('Ctrl Pts',(-3.24355296537231,-5.94168669364259,
91.6437807787672));
#206392=CARTESIAN_POINT('Ctrl Pts',(-3.08521190319609,-6.02543195366043,
91.652221065423));
#206393=CARTESIAN_POINT('Ctrl Pts',(-2.92369862713102,-6.10280880723886,
91.6606613520788));
#206394=CARTESIAN_POINT('Ctrl Pts',(-2.7623083895356,-6.18012671625321,
91.6690952090467));
#206395=CARTESIAN_POINT('Ctrl Pts',(-2.59775105516567,-6.25108574644093,
91.6775290660146));
#206396=CARTESIAN_POINT('Ctrl Pts',(-2.43055632733157,-6.31543228446545,
91.6859629229825));
#206397=CARTESIAN_POINT('Ctrl Pts',(-2.26346326257204,-6.37973969645425,
91.6943916517275));
#206398=CARTESIAN_POINT('Ctrl Pts',(-2.09373631212831,-6.43744251306235,
91.7028203804725));
#206399=CARTESIAN_POINT('Ctrl Pts',(-1.92192589874289,-6.48833490502312,
91.7112491092175));
#206400=CARTESIAN_POINT('Ctrl Pts',(-1.75019357130512,-6.53920416695017,
91.7196740071978));
#206401=CARTESIAN_POINT('Ctrl Pts',(-1.57637998831376,-6.58326908164322,
91.728098905178));
#206402=CARTESIAN_POINT('Ctrl Pts',(-1.40105187917827,-6.62037330003762,
91.7365238031583));
#206403=CARTESIAN_POINT('Ctrl Pts',(-1.22576258797132,-6.65746930349772,
91.7449468358525));
#206404=CARTESIAN_POINT('Ctrl Pts',(-1.04895976461049,-6.6876076117648,
91.7533698685466));
#206405=CARTESIAN_POINT('Ctrl Pts',(-0.871222033941675,-6.71068261561926,
91.7617929012408));
#206406=CARTESIAN_POINT('Ctrl Pts',(-0.693504414095105,-6.73375500856325,
91.7702149808784));
#206407=CARTESIAN_POINT('Ctrl Pts',(-0.514852428456964,-6.74976564742314,
91.778637060516));
#206408=CARTESIAN_POINT('Ctrl Pts',(-0.33585187311627,-6.75866055659879,
91.7870591401536));
#206409=CARTESIAN_POINT('Ctrl Pts',(-0.156846584344886,-6.76755570098844,
91.7954814425018));
#206410=CARTESIAN_POINT('Ctrl Pts',(0.0225069594262393,-6.76933472437189,
91.80390374485));
#206411=CARTESIAN_POINT('Ctrl Pts',(0.201620523660513,-6.76399572475019,
91.8123260471983));
#206412=CARTESIAN_POINT('Ctrl Pts',(0.380763828683505,-6.75865583861797,
91.8207497480219));
#206413=CARTESIAN_POINT('Ctrl Pts',(0.559666741463216,-6.74619558364666,
91.8291734488456));
#206414=CARTESIAN_POINT('Ctrl Pts',(0.73774334201908,-6.72666512926774,
91.8375971496692));
#206415=CARTESIAN_POINT('Ctrl Pts',(0.91594044863803,-6.70712145845184,
91.8460265508882));
#206416=CARTESIAN_POINT('Ctrl Pts',(1.09330979384886,-6.68049806409771,
91.8544559521072));
#206417=CARTESIAN_POINT('Ctrl Pts',(1.26927186134911,-6.64689686560483,
91.8628853533262));
#206418=CARTESIAN_POINT('Ctrl Pts',(1.44529671187075,-6.61328367825098,
91.8713177621438));
#206419=CARTESIAN_POINT('Ctrl Pts',(1.61991295711736,-6.57268779106609,
91.8797501709614));
#206420=CARTESIAN_POINT('Ctrl Pts',(1.79255296508185,-6.52526190029,91.8881825797791));
#206421=CARTESIAN_POINT('Ctrl Pts',(1.96535270460476,-6.47779212969989,
91.8966227905067));
#206422=CARTESIAN_POINT('Ctrl Pts',(2.13617223350927,-6.42347982387776,
91.9050630012343));
#206423=CARTESIAN_POINT('Ctrl Pts',(2.30445966206695,-6.36252738036594,
91.9135032119619));
#206424=CARTESIAN_POINT('Ctrl Pts',(2.4001786797552,-6.32785867059568,91.9183038597991));
#206425=CARTESIAN_POINT('Ctrl Pts',(2.49507886966456,-6.29104267349489,
91.9231045076362));
#206426=CARTESIAN_POINT('Ctrl Pts',(2.58906175767578,-6.25212349645629,
91.9279051554734));
#206427=CARTESIAN_POINT('Ctrl Pts',(2.74841398519276,-6.18613427559421,
91.9360448705063));
#206428=CARTESIAN_POINT('Ctrl Pts',(2.90544553379042,-6.11396437463473,
91.9441845855391));
#206429=CARTESIAN_POINT('Ctrl Pts',(3.05963911340726,-6.03580131347184,
91.952324300572));
#206430=CARTESIAN_POINT('Ctrl Pts',(3.21369783624446,-5.9577066132533,91.960456896659));
#206431=CARTESIAN_POINT('Ctrl Pts',(3.36492320624515,-5.87362935061182,
91.9685894927459));
#206432=CARTESIAN_POINT('Ctrl Pts',(3.51281707085037,-5.78380542780808,
91.9767220888329));
#206433=CARTESIAN_POINT('Ctrl Pts',(3.66060982727565,-5.69404291345678,
91.9848491250408));
#206434=CARTESIAN_POINT('Ctrl Pts',(3.80507530116462,-5.5985417501571,91.9929761612488));
#206435=CARTESIAN_POINT('Ctrl Pts',(3.94573920100857,-5.49758412010442,
92.0011031974568));
#206436=CARTESIAN_POINT('Ctrl Pts',(4.08633586096258,-5.39667474962609,
92.0092263487944));
#206437=CARTESIAN_POINT('Ctrl Pts',(4.2231342686755,-5.29031431943281,92.0173495001319));
#206438=CARTESIAN_POINT('Ctrl Pts',(4.35568845978136,-5.17882873257337,
92.0254726514695));
#206439=CARTESIAN_POINT('Ctrl Pts',(4.48820540217429,-5.06737447399248,
92.0335935201412));
#206440=CARTESIAN_POINT('Ctrl Pts',(4.61648022398761,-4.95079816347045,
92.0417143888128));
#206441=CARTESIAN_POINT('Ctrl Pts',(4.74009948392975,-4.82946641798542,
92.0498352574845));
#206442=CARTESIAN_POINT('Ctrl Pts',(4.86372542472989,-4.70812811526843,
92.0579565650389));
#206443=CARTESIAN_POINT('Ctrl Pts',(4.98269503684909,-4.58203411784084,
92.0660778725935));
#206444=CARTESIAN_POINT('Ctrl Pts',(5.09663111734629,-4.45158850902658,
92.074199180148));
#206445=CARTESIAN_POINT('Ctrl Pts',(5.15583626539749,-4.38380443616069,
92.0784192938647));
#206446=CARTESIAN_POINT('Ctrl Pts',(5.21368287901529,-4.31484593128487,
92.0826394075814));
#206447=CARTESIAN_POINT('Ctrl Pts',(5.27012224682327,-4.24477331591906,
92.0868595212981));
#206448=CARTESIAN_POINT('Ctrl Pts',(5.39027920574609,-4.0955917659986,92.0958439598239));
#206449=CARTESIAN_POINT('Ctrl Pts',(5.50399607223322,-3.94143273754319,
92.1048283983497));
#206450=CARTESIAN_POINT('Ctrl Pts',(5.6109066604396,-3.78285810569662,92.1138128368755));
#206451=CARTESIAN_POINT('Ctrl Pts',(5.7180017699404,-3.62400978349979,92.122812782006));
#206452=CARTESIAN_POINT('Ctrl Pts',(5.81826698801442,-3.46073082361633,
92.1318127271365));
#206453=CARTESIAN_POINT('Ctrl Pts',(5.91138078136888,-3.29360991279518,
92.140812672267));
#206454=CARTESIAN_POINT('Ctrl Pts',(6.00471399976738,-3.12609517725809,
92.1498338259992));
#206455=CARTESIAN_POINT('Ctrl Pts',(6.0908619575219,-2.95472058548155,92.1588549797314));
#206456=CARTESIAN_POINT('Ctrl Pts',(6.16954900714058,-2.78009964722323,
92.1678761334636));
#206457=CARTESIAN_POINT('Ctrl Pts',(6.24831612145253,-2.60530103078371,
92.1769064662908));
#206458=CARTESIAN_POINT('Ctrl Pts',(6.31960706899713,-2.42724968904704,
92.1859367991181));
#206459=CARTESIAN_POINT('Ctrl Pts',(6.38319474430584,-2.24657825509514,
92.1949671319453));
#206460=CARTESIAN_POINT('Ctrl Pts',(6.44687256689409,-2.06565068600097,
92.204010266938));
#206461=CARTESIAN_POINT('Ctrl Pts',(6.50282520144573,-1.88209582305477,
92.2130534019306));
#206462=CARTESIAN_POINT('Ctrl Pts',(6.55087502987781,-1.69656280252853,
92.2220965369233));
#206463=CARTESIAN_POINT('Ctrl Pts',(6.59288164995984,-1.53436419828303,
92.2300023203232));
#206464=CARTESIAN_POINT('Ctrl Pts',(6.62884906818787,-1.37065403521884,
92.2379081037231));
#206465=CARTESIAN_POINT('Ctrl Pts',(6.6586905907916,-1.20587255383952,92.245813887123));
#206466=CARTESIAN_POINT('Ctrl Pts',(6.69135405592223,-1.02550862795411,
92.2544672753513));
#206467=CARTESIAN_POINT('Ctrl Pts',(6.71670584184189,-0.843701615481007,
92.2631206635796));
#206468=CARTESIAN_POINT('Ctrl Pts',(6.73463390008914,-0.661056148727285,
92.2717740518079));
#206469=CARTESIAN_POINT('Ctrl Pts',(6.75254540050286,-0.478579368018239,
92.2804194480183));
#206470=CARTESIAN_POINT('Ctrl Pts',(6.76304681876529,-0.295265979047824,
92.2890648442287));
#206471=CARTESIAN_POINT('Ctrl Pts',(6.7660775779376,-0.111728283483179,
92.2977102404392));
#206472=CARTESIAN_POINT('Ctrl Pts',(6.76920512934841,0.0776709878100624,
92.3066317414816));
#206473=CARTESIAN_POINT('Ctrl Pts',(6.76437688126879,0.267308811449076,
92.315553242524));
#206474=CARTESIAN_POINT('Ctrl Pts',(6.75158428734202,0.456506966996586,
92.3244747435664));
#206475=CARTESIAN_POINT('Ctrl Pts',(6.73921121229972,0.639500579539438,
92.3331036739083));
#206476=CARTESIAN_POINT('Ctrl Pts',(6.71938787487004,0.822082567868297,
92.3417326042503));
#206477=CARTESIAN_POINT('Ctrl Pts',(6.69215941006571,1.00363909363324,92.3503615345923));
#206478=CARTESIAN_POINT('Ctrl Pts',(6.66354614134544,1.19442934556127,92.3594293209849));
#206479=CARTESIAN_POINT('Ctrl Pts',(6.62675488043951,1.38408676929546,92.3684971073775));
#206480=CARTESIAN_POINT('Ctrl Pts',(6.58189984786576,1.57190438407198,92.3775648937701));
#206481=CARTESIAN_POINT('Ctrl Pts',(6.53704481529201,1.7597219988485,92.3866326801627));
#206482=CARTESIAN_POINT('Ctrl Pts',(6.48412606752052,1.94569941665851,92.3957004665552));
#206483=CARTESIAN_POINT('Ctrl Pts',(6.42332063750698,2.12914090369261,92.4047682529478));
#206484=CARTESIAN_POINT('Ctrl Pts',(6.36682580422096,2.29957792264669,92.413193209081));
#206485=CARTESIAN_POINT('Ctrl Pts',(6.30354787053495,2.46775110860223,92.4216181652141));
#206486=CARTESIAN_POINT('Ctrl Pts',(6.23370034057328,2.63311015036146,92.4300431213473));
#206487=CARTESIAN_POINT('Ctrl Pts',(6.16383659832928,2.79850757354195,92.4384700329937));
#206488=CARTESIAN_POINT('Ctrl Pts',(6.08740034848315,2.96108924468914,92.44689694464));
#206489=CARTESIAN_POINT('Ctrl Pts',(6.00465273953959,3.12032602103366,92.4553238562864));
#206490=CARTESIAN_POINT('Ctrl Pts',(5.92187470107723,3.27962135494305,92.4637538668364));
#206491=CARTESIAN_POINT('Ctrl Pts',(5.83278082863023,3.43556904734347,92.4721838773864));
#206492=CARTESIAN_POINT('Ctrl Pts',(5.73767778366786,3.58766534821801,92.4806138879364));
#206493=CARTESIAN_POINT('Ctrl Pts',(5.64248713176929,3.73990175702425,92.4890516640358));
#206494=CARTESIAN_POINT('Ctrl Pts',(5.54127642379871,3.8882794047072,92.4974894401353));
#206495=CARTESIAN_POINT('Ctrl Pts',(5.4343957681525,4.03232335448018,92.5059272162347));
#206496=CARTESIAN_POINT('Ctrl Pts',(5.32745900804079,4.17644291670857,92.5143694215446));
#206497=CARTESIAN_POINT('Ctrl Pts',(5.21484656800135,4.31622398273164,92.5228116268544));
#206498=CARTESIAN_POINT('Ctrl Pts',(5.09694861405359,4.45122498035061,92.5312538321643));
#206499=CARTESIAN_POINT('Ctrl Pts',(4.97892628425141,4.58636839659401,92.5397049435363));
#206500=CARTESIAN_POINT('Ctrl Pts',(4.85560752589527,4.71672142683671,92.5481560549083));
#206501=CARTESIAN_POINT('Ctrl Pts',(4.72741983164075,4.84187884352859,92.5566071662803));
#206502=CARTESIAN_POINT('Ctrl Pts',(4.69144375668446,4.877004466393,92.5589789837777));
#206503=CARTESIAN_POINT('Ctrl Pts',(4.65508438413134,4.9117210944733,92.5613508012751));
#206504=CARTESIAN_POINT('Ctrl Pts',(4.61835163230548,4.94602033966514,92.5637226187725));
#206505=CARTESIAN_POINT('Ctrl Pts',(4.48956147683812,5.06627828117774,92.572038542003));
#206506=CARTESIAN_POINT('Ctrl Pts',(4.35594639022535,5.18161926967145,92.5803544652335));
#206507=CARTESIAN_POINT('Ctrl Pts',(4.21791411620621,5.29164336556314,92.588670388464));
#206508=CARTESIAN_POINT('Ctrl Pts',(4.07998670130477,5.40158387933824,92.5969799943286));
#206509=CARTESIAN_POINT('Ctrl Pts',(3.93764905253301,5.50621532877486,92.6052896001932));
#206510=CARTESIAN_POINT('Ctrl Pts',(3.79134424574178,5.60517598388139,92.6135992060579));
#206511=CARTESIAN_POINT('Ctrl Pts',(3.64514512056804,5.70406515588133,92.621902809573));
#206512=CARTESIAN_POINT('Ctrl Pts',(3.49498483646513,5.79729150392402,92.6302064130881));
#206513=CARTESIAN_POINT('Ctrl Pts',(3.34133787182237,5.88453483516969,92.6385100166033));
#206514=CARTESIAN_POINT('Ctrl Pts',(3.26151141794891,5.9298616385572,92.6428241091369));
#206515=CARTESIAN_POINT('Ctrl Pts',(3.18074432323989,5.97357415670657,92.6471382016706));
#206516=CARTESIAN_POINT('Ctrl Pts',(3.09910619832136,6.01563211736939,92.6514522942042));
#206517=CARTESIAN_POINT('Origin',(0.,0.,4.30282021618968));
#206518=CARTESIAN_POINT('',(3.09910619832144,6.01563211736935,95.0455663730808));
#206519=CARTESIAN_POINT('',(3.09910619832124,6.01563211736945,94.6514100603466));
#206520=CARTESIAN_POINT('',(3.09910619832133,6.0156321173694,4.30282021618968));
#206521=CARTESIAN_POINT('',(-6.76699933137488,-0.00202679626836213,93.6971797838099));
#206522=CARTESIAN_POINT('Ctrl Pts',(-6.7669985271066,-0.00446476618441742,
93.6971797838099));
#206523=CARTESIAN_POINT('Ctrl Pts',(-6.76686577009316,-0.205677209860647,
93.7066386602188));
#206524=CARTESIAN_POINT('Ctrl Pts',(-6.75775404271323,-0.406695906542261,
93.7160975366277));
#206525=CARTESIAN_POINT('Ctrl Pts',(-6.73974217978172,-0.606765481937798,
93.7255564130366));
#206526=CARTESIAN_POINT('Ctrl Pts',(-6.7220965388771,-0.802767189078906,
93.734822969034));
#206527=CARTESIAN_POINT('Ctrl Pts',(-6.69590926045183,-0.99785783025461,
93.7440895250314));
#206528=CARTESIAN_POINT('Ctrl Pts',(-6.66130632404342,-1.19133834709506,
93.7533560810288));
#206529=CARTESIAN_POINT('Ctrl Pts',(-6.62562615069218,-1.39084217819991,
93.7629111176435));
#206530=CARTESIAN_POINT('Ctrl Pts',(-6.58099798383396,-1.58863380155292,
93.7724661542581));
#206531=CARTESIAN_POINT('Ctrl Pts',(-6.5276158027552,-1.78396214411084,
93.7820211908727));
#206532=CARTESIAN_POINT('Ctrl Pts',(-6.47423362167641,-1.97929048666888,
93.7915762274874));
#206533=CARTESIAN_POINT('Ctrl Pts',(-6.41209751328803,-2.17215534877263,
93.801131264102));
#206534=CARTESIAN_POINT('Ctrl Pts',(-6.34145688008581,-2.3618242182712,
93.8106863007167));
#206535=CARTESIAN_POINT('Ctrl Pts',(-6.27748215676012,-2.5335952358799,
93.819339688945));
#206536=CARTESIAN_POINT('Ctrl Pts',(-6.20648337750343,-2.70287511116803,
93.8279930771732));
#206537=CARTESIAN_POINT('Ctrl Pts',(-6.12867281049903,-2.8690867156379,
93.8366464654015));
#206538=CARTESIAN_POINT('Ctrl Pts',(-6.05093410707278,-3.03514481190078,
93.8452918616119));
#206539=CARTESIAN_POINT('Ctrl Pts',(-5.96639629222485,-3.19814001496491,
93.8539372578223));
#206540=CARTESIAN_POINT('Ctrl Pts',(-5.87531981022229,-3.35751487377338,
93.8625826540327));
#206541=CARTESIAN_POINT('Ctrl Pts',(-5.78133465218575,-3.52197962870041,
93.8715041550751));
#206542=CARTESIAN_POINT('Ctrl Pts',(-5.68038637326566,-3.68258866056744,
93.8804256561175));
#206543=CARTESIAN_POINT('Ctrl Pts',(-5.57281380666296,-3.8387543912403,
93.8893471571598));
#206544=CARTESIAN_POINT('Ctrl Pts',(-5.46876896269455,-3.98979884052895,
93.8979760875018));
#206545=CARTESIAN_POINT('Ctrl Pts',(-5.35852758771888,-4.13668650649272,
93.9066050178438));
#206546=CARTESIAN_POINT('Ctrl Pts',(-5.24244181427066,-4.27891257494081,
93.9152339481857));
#206547=CARTESIAN_POINT('Ctrl Pts',(-5.12045207103073,-4.42837207421136,
93.9243017345784));
#206548=CARTESIAN_POINT('Ctrl Pts',(-4.99200812919201,-4.57268315854584,
93.933369520971));
#206549=CARTESIAN_POINT('Ctrl Pts',(-4.85756907180305,-4.71129618180204,
93.9424373073636));
#206550=CARTESIAN_POINT('Ctrl Pts',(-4.72313001441418,-4.84990920505814,
93.9515050937562));
#206551=CARTESIAN_POINT('Ctrl Pts',(-4.58269608808526,-4.982823862403,93.9605728801488));
#206552=CARTESIAN_POINT('Ctrl Pts',(-4.43677464882927,-5.10953224038228,
93.9696406665414));
#206553=CARTESIAN_POINT('Ctrl Pts',(-4.30119781988855,-5.22725805349268,
93.9780656226746));
#206554=CARTESIAN_POINT('Ctrl Pts',(-4.16094358476472,-5.33957486833351,
93.9864905788078));
#206555=CARTESIAN_POINT('Ctrl Pts',(-4.01647643407986,-5.44611843926307,
93.994915534941));
#206556=CARTESIAN_POINT('Ctrl Pts',(-3.87197575118233,-5.55268673997833,
94.0033424465874));
#206557=CARTESIAN_POINT('Ctrl Pts',(-3.72326046989799,-5.65347892814872,
94.0117693582337));
#206558=CARTESIAN_POINT('Ctrl Pts',(-3.57082524629212,-5.74817328030765,
94.0201962698801));
#206559=CARTESIAN_POINT('Ctrl Pts',(-3.4183339663168,-5.84290245526845,
94.0286262804302));
#206560=CARTESIAN_POINT('Ctrl Pts',(-3.26212029796605,-5.9315291481623,
94.0370562909802));
#206561=CARTESIAN_POINT('Ctrl Pts',(-3.10270507368833,-6.01377670234843,
94.0454863015303));
#206562=CARTESIAN_POINT('Ctrl Pts',(-2.9431429994403,-6.09610002126119,
94.0539240776297));
#206563=CARTESIAN_POINT('Ctrl Pts',(-2.78037377191445,-6.17203230892936,
94.0623618537292));
#206564=CARTESIAN_POINT('Ctrl Pts',(-2.61494087740784,-6.24134386231535,
94.0707996298286));
#206565=CARTESIAN_POINT('Ctrl Pts',(-2.44942114282594,-6.31069179915781,
94.0792418351385));
#206566=CARTESIAN_POINT('Ctrl Pts',(-2.28123526116274,-6.37341194966489,
94.0876840404485));
#206567=CARTESIAN_POINT('Ctrl Pts',(-2.11094413489262,-6.42932374821508,
94.0961262457584));
#206568=CARTESIAN_POINT('Ctrl Pts',(-1.94047336085457,-6.4852945306362,
94.1045773571304));
#206569=CARTESIAN_POINT('Ctrl Pts',(-1.76789322286463,-6.53444251764913,
94.1130284685024));
#206570=CARTESIAN_POINT('Ctrl Pts',(-1.59377817003713,-6.57663744969366,
94.1214795798744));
#206571=CARTESIAN_POINT('Ctrl Pts',(-1.54491251075818,-6.58847952273159,
94.1238513973717));
#206572=CARTESIAN_POINT('Ctrl Pts',(-1.49592600811817,-6.59977424701124,
94.1262232148689));
#206573=CARTESIAN_POINT('Ctrl Pts',(-1.44683147260946,-6.61051947201328,
94.1285950323662));
#206574=CARTESIAN_POINT('Ctrl Pts',(-1.27469195035897,-6.64819531269818,
94.1369113047703));
#206575=CARTESIAN_POINT('Ctrl Pts',(-1.10091298009481,-6.67917962337993,
94.1452275771744));
#206576=CARTESIAN_POINT('Ctrl Pts',(-0.926049399486271,-6.70333659528679,
94.1535438495785));
#206577=CARTESIAN_POINT('Ctrl Pts',(-0.751333666241069,-6.72747314244546,
94.1618530905645));
#206578=CARTESIAN_POINT('Ctrl Pts',(-0.575535492661531,-6.74479380444557,
94.1701623315505));
#206579=CARTESIAN_POINT('Ctrl Pts',(-0.399220451517156,-6.75521369248157,
94.1784715725366));
#206580=CARTESIAN_POINT('Ctrl Pts',(-0.223022158218122,-6.76562668093901,
94.186775311519));
#206581=CARTESIAN_POINT('Ctrl Pts',(-0.0463080254900932,-6.76914797997407,
94.1950790505015));
#206582=CARTESIAN_POINT('Ctrl Pts',(0.130350469610198,-6.76574443465554,
94.203382789484));
#206583=CARTESIAN_POINT('Ctrl Pts',(0.306924364736936,-6.76234251926057,
94.2116825518895));
#206584=CARTESIAN_POINT('Ctrl Pts',(0.48344232817631,-6.75202237510446,
94.219982314295));
#206585=CARTESIAN_POINT('Ctrl Pts',(0.659331865264326,-6.73480292892428,
94.2282820767005));
#206586=CARTESIAN_POINT('Ctrl Pts',(0.835169394121983,-6.71758857430861,
94.2365793849751));
#206587=CARTESIAN_POINT('Ctrl Pts',(1.01037852113831,-6.69347901789371,
94.2448766932496));
#206588=CARTESIAN_POINT('Ctrl Pts',(1.18439063156209,-6.66254514670392,
94.2531740015242));
#206589=CARTESIAN_POINT('Ctrl Pts',(1.35842032338573,-6.63160815009512,
94.2614721481214));
#206590=CARTESIAN_POINT('Ctrl Pts',(1.53125241308379,-6.59384551445604,
94.2697702947187));
#206591=CARTESIAN_POINT('Ctrl Pts',(1.70232667151901,-6.54937958156611,
94.2780684413159));
#206592=CARTESIAN_POINT('Ctrl Pts',(1.87341813254701,-6.50490917734692,
94.286367422344));
#206593=CARTESIAN_POINT('Ctrl Pts',(2.04275107291088,-6.45373421938314,
94.294666403372));
#206594=CARTESIAN_POINT('Ctrl Pts',(2.20977875475255,-6.39602742763384,
94.3029653844001));
#206595=CARTESIAN_POINT('Ctrl Pts',(2.37685099038889,-6.33830524288786,
94.3112665791396));
#206596=CARTESIAN_POINT('Ctrl Pts',(2.54161641293948,-6.2740478653736,94.3195677738792));
#206597=CARTESIAN_POINT('Ctrl Pts',(2.70354647290647,-6.20347688549212,
94.3278689686187));
#206598=CARTESIAN_POINT('Ctrl Pts',(2.86554664101356,-6.132875351678,94.3361737573872));
#206599=CARTESIAN_POINT('Ctrl Pts',(3.02470868112125,-6.05595490657058,
94.3444785461557));
#206600=CARTESIAN_POINT('Ctrl Pts',(3.18052676064206,-5.97298405529763,
94.3527833349242));
#206601=CARTESIAN_POINT('Ctrl Pts',(3.33652956109664,-5.88991484282572,
94.3610979689452));
#206602=CARTESIAN_POINT('Ctrl Pts',(3.48918017297209,-5.80078105698932,
94.3694126029662));
#206603=CARTESIAN_POINT('Ctrl Pts',(3.63799896426392,-5.70589629558886,
94.3777272369872));
#206604=CARTESIAN_POINT('Ctrl Pts',(3.78691185499685,-5.61095153771256,
94.386047128425));
#206605=CARTESIAN_POINT('Ctrl Pts',(3.93198780781265,-5.51024875057221,
94.3943670198628));
#206606=CARTESIAN_POINT('Ctrl Pts',(4.07277854115722,-5.40414322114887,
94.4026869113006));
#206607=CARTESIAN_POINT('Ctrl Pts',(4.21377980229941,-5.29787902955442,
94.4110192436738));
#206608=CARTESIAN_POINT('Ctrl Pts',(4.35048276869771,-5.18619617025387,
94.419351576047));
#206609=CARTESIAN_POINT('Ctrl Pts',(4.48247340901378,-5.06948923832415,
94.4276839084202));
#206610=CARTESIAN_POINT('Ctrl Pts',(4.58184713693827,-4.98162237994152,
94.4339571936187));
#206611=CARTESIAN_POINT('Ctrl Pts',(4.67855047776066,-4.89090850201358,
94.4402304788172));
#206612=CARTESIAN_POINT('Ctrl Pts',(4.77242149879349,-4.79752874278558,
94.4465037640157));
#206613=CARTESIAN_POINT('Ctrl Pts',(4.89317556303413,-4.67740662926717,
94.4545736100184));
#206614=CARTESIAN_POINT('Ctrl Pts',(5.00961438061434,-4.55250058113334,
94.4626434560212));
#206615=CARTESIAN_POINT('Ctrl Pts',(5.12132461771142,-4.42315760063137,
94.4707133020239));
#206616=CARTESIAN_POINT('Ctrl Pts',(5.2328943091212,-4.29397735005069,94.478772995134));
#206617=CARTESIAN_POINT('Ctrl Pts',(5.33974701646822,-4.16037155295409,
94.486832688244));
#206618=CARTESIAN_POINT('Ctrl Pts',(5.4415037112129,-4.022726234888,94.494892381354));
#206619=CARTESIAN_POINT('Ctrl Pts',(5.54315471546799,-3.88522388334705,
94.5029437031927));
#206620=CARTESIAN_POINT('Ctrl Pts',(5.63972002037714,-3.74369065775069,
94.5109950250313));
#206621=CARTESIAN_POINT('Ctrl Pts',(5.73085868944113,-3.59854799629755,
94.5190463468699));
#206622=CARTESIAN_POINT('Ctrl Pts',(5.82192266810941,-3.45352428284892,
94.527091070451));
#206623=CARTESIAN_POINT('Ctrl Pts',(5.9075686650232,-3.30489733531461,94.535135794032));
#206624=CARTESIAN_POINT('Ctrl Pts',(5.98749723392353,-3.15312002209845,
94.543180517613));
#206625=CARTESIAN_POINT('Ctrl Pts',(6.06737779578135,-3.00143387002813,
94.5512204093374));
#206626=CARTESIAN_POINT('Ctrl Pts',(6.1415475923023,-2.84660144832157,94.5592603010618));
#206627=CARTESIAN_POINT('Ctrl Pts',(6.20975164025075,-2.68910274374244,
94.5673001927862));
#206628=CARTESIAN_POINT('Ctrl Pts',(6.27942430820883,-2.5282126605576,94.5755132054062));
#206629=CARTESIAN_POINT('Ctrl Pts',(6.34287118327832,-2.36454050467807,
94.5837262180261));
#206630=CARTESIAN_POINT('Ctrl Pts',(6.39987084133188,-2.19862279945196,
94.5919392306461));
#206631=CARTESIAN_POINT('Ctrl Pts',(6.45564954348077,-2.0362591190885,94.5999763171886));
#206632=CARTESIAN_POINT('Ctrl Pts',(6.50525432077201,-1.87174548789571,
94.6080134037312));
#206633=CARTESIAN_POINT('Ctrl Pts',(6.54852718205247,-1.70560275149872,
94.6160504902738));
#206634=CARTESIAN_POINT('Ctrl Pts',(6.59180418474718,-1.53944411446844,
94.624088346003));
#206635=CARTESIAN_POINT('Ctrl Pts',(6.62874797049889,-1.37165642332735,
94.6321262017322));
#206636=CARTESIAN_POINT('Ctrl Pts',(6.65925113857969,-1.20277315954635,
94.6401640574613));
#206637=CARTESIAN_POINT('Ctrl Pts',(6.68976326965166,-1.03384027143787,
94.6482042750183));
#206638=CARTESIAN_POINT('Ctrl Pts',(6.7138309497305,-0.863811537386868,
94.6562444925752));
#206639=CARTESIAN_POINT('Ctrl Pts',(6.73139837525425,-0.693227894436233,
94.6642847101322));
#206640=CARTESIAN_POINT('Ctrl Pts',(6.74962950937001,-0.516199492159291,
94.6726286922599));
#206641=CARTESIAN_POINT('Ctrl Pts',(6.76085958200391,-0.338573875059958,
94.6809726743877));
#206642=CARTESIAN_POINT('Ctrl Pts',(6.76508549784856,-0.160957158272201,
94.6893166565154));
#206643=CARTESIAN_POINT('Ctrl Pts',(6.76916465736336,0.0104913387888412,
94.6973708713505));
#206644=CARTESIAN_POINT('Ctrl Pts',(6.76671805279467,0.181931176453537,
94.7054250861855));
#206645=CARTESIAN_POINT('Ctrl Pts',(6.75779593370413,0.352821652413778,
94.7134793010206));
#206646=CARTESIAN_POINT('Ctrl Pts',(6.74886713788282,0.523840011636674,
94.7215395431036));
#206647=CARTESIAN_POINT('Ctrl Pts',(6.73345321223899,0.694307821062776,
94.7295997851866));
#206648=CARTESIAN_POINT('Ctrl Pts',(6.71165577000229,0.863693131265336,
94.7376600272696));
#206649=CARTESIAN_POINT('Ctrl Pts',(6.68982785344615,1.03331525375057,94.745731538124));
#206650=CARTESIAN_POINT('Ctrl Pts',(6.66159867532509,1.20185149252047,94.7538030489783));
#206651=CARTESIAN_POINT('Ctrl Pts',(6.62712018020191,1.36878307892839,94.7618745598326));
#206652=CARTESIAN_POINT('Ctrl Pts',(6.62350647392875,1.38627925208894,94.7627205384435));
#206653=CARTESIAN_POINT('Ctrl Pts',(6.61982416158567,1.40375781456,94.7635665170543));
#206654=CARTESIAN_POINT('Ctrl Pts',(6.61607344889682,1.42121818128059,94.7644124956652));
#206655=CARTESIAN_POINT('Ctrl Pts',(6.57958530667037,1.5910782577725,94.7726424483258));
#206656=CARTESIAN_POINT('Ctrl Pts',(6.53649789669645,1.75978186392105,94.7808724009865));
#206657=CARTESIAN_POINT('Ctrl Pts',(6.48689578226858,1.92677764933739,94.7891023536471));
#206658=CARTESIAN_POINT('Ctrl Pts',(6.43735351517776,2.0935719463057,94.797322376474));
#206659=CARTESIAN_POINT('Ctrl Pts',(6.38131229709004,2.25866218522143,94.8055423993008));
#206660=CARTESIAN_POINT('Ctrl Pts',(6.31890785907017,2.42150623963295,94.8137624221277));
#206661=CARTESIAN_POINT('Ctrl Pts',(6.25656618174205,2.58418652034779,94.8219741780054));
#206662=CARTESIAN_POINT('Ctrl Pts',(6.18787415730906,2.74462478290262,94.8301859338831));
#206663=CARTESIAN_POINT('Ctrl Pts',(6.11301759282562,2.90229304340627,94.8383976897607));
#206664=CARTESIAN_POINT('Ctrl Pts',(6.03432991560557,3.0680306681019,94.8470297182324));
#206665=CARTESIAN_POINT('Ctrl Pts',(5.94883021529023,3.23070692169701,94.8556617467041));
#206666=CARTESIAN_POINT('Ctrl Pts',(5.85679275852635,3.38972972133078,94.8642937751757));
#206667=CARTESIAN_POINT('Ctrl Pts',(5.76936430980571,3.54078905273825,94.8724935330257));
#206668=CARTESIAN_POINT('Ctrl Pts',(5.67603708184902,3.68855153338375,94.8806932908757));
#206669=CARTESIAN_POINT('Ctrl Pts',(5.57709418534632,3.83253303283563,94.8888930487256));
#206670=CARTESIAN_POINT('Ctrl Pts',(5.47818390360759,3.97646707135008,94.8970901036714));
#206671=CARTESIAN_POINT('Ctrl Pts',(5.37366184258913,4.11662231548417,94.9052871586173));
#206672=CARTESIAN_POINT('Ctrl Pts',(5.26385501927317,4.25254269068197,94.9134842135631));
#206673=CARTESIAN_POINT('Ctrl Pts',(5.1540644262943,4.3884429757484,94.9216800569178));
#206674=CARTESIAN_POINT('Ctrl Pts',(5.03899085257448,4.52010936008753,94.9298759002725));
#206675=CARTESIAN_POINT('Ctrl Pts',(4.91900229758501,4.6471179666922,94.9380717436273));
#206676=CARTESIAN_POINT('Ctrl Pts',(4.79900966164792,4.77413089300445,94.946267865732));
#206677=CARTESIAN_POINT('Ctrl Pts',(4.67410195871594,4.89648546630697,94.9544639878367));
#206678=CARTESIAN_POINT('Ctrl Pts',(4.54468484794874,5.01379383629055,94.9626601099415));
#206679=CARTESIAN_POINT('Ctrl Pts',(4.41519628569744,5.13116697249464,94.9708607571441));
#206680=CARTESIAN_POINT('Ctrl Pts',(4.28119360827926,5.24348809903702,94.9790614043466));
#206681=CARTESIAN_POINT('Ctrl Pts',(4.14311689527926,5.35040852571573,94.9872620515492));
#206682=CARTESIAN_POINT('Ctrl Pts',(4.00499597758547,5.45736318253085,94.9954653241553));
#206683=CARTESIAN_POINT('Ctrl Pts',(3.86279871414833,5.55891348177531,95.0036685967615));
#206684=CARTESIAN_POINT('Ctrl Pts',(3.71699506866281,5.65475345700733,95.0118718693676));
#206685=CARTESIAN_POINT('Ctrl Pts',(3.57106337376203,5.75067760196464,95.0200823463496));
#206686=CARTESIAN_POINT('Ctrl Pts',(3.42151927671942,5.84088121963626,95.0282928233316));
#206687=CARTESIAN_POINT('Ctrl Pts',(3.26885886520031,5.92510343533354,95.0365033003136));
#206688=CARTESIAN_POINT('Ctrl Pts',(3.21268785259049,5.95609278675008,95.0395243245694));
#206689=CARTESIAN_POINT('Ctrl Pts',(3.15609515520393,5.98627280382349,95.0425453488251));
#206690=CARTESIAN_POINT('Ctrl Pts',(3.09910619832144,6.01563211736935,95.0455663730808));
#206691=CARTESIAN_POINT('Ctrl Pts',(3.09910619832149,6.01563211736932,93.0457552630241));
#206692=CARTESIAN_POINT('Ctrl Pts',(2.93375330764842,6.10081787314646,93.0545047109265));
#206693=CARTESIAN_POINT('Ctrl Pts',(2.76488627843086,6.17918207037032,93.0632541588287));
#206694=CARTESIAN_POINT('Ctrl Pts',(2.59307866646717,6.25045854553991,93.072003606731));
#206695=CARTESIAN_POINT('Ctrl Pts',(2.42127244185387,6.32173444515033,93.0807529839814));
#206696=CARTESIAN_POINT('Ctrl Pts',(2.2465259467247,6.38592262741836,93.0895023612317));
#206697=CARTESIAN_POINT('Ctrl Pts',(2.06943269687121,6.44280508110562,93.098251738482));
#206698=CARTESIAN_POINT('Ctrl Pts',(1.89234081822077,6.49968709436166,93.1070010479873));
#206699=CARTESIAN_POINT('Ctrl Pts',(1.7129024940559,6.54926340459544,93.1157503574927));
#206700=CARTESIAN_POINT('Ctrl Pts',(1.5317271662506,6.59136563150383,93.124499666998));
#206701=CARTESIAN_POINT('Ctrl Pts',(1.3505531810734,6.63346754640709,93.1332489116653));
#206702=CARTESIAN_POINT('Ctrl Pts',(1.1676424971443,6.66809542395774,93.1419981563325));
#206703=CARTESIAN_POINT('Ctrl Pts',(0.983616340614511,6.69513165624666,
93.1507474009997));
#206704=CARTESIAN_POINT('Ctrl Pts',(0.799591486713998,6.72216769715959,
93.1594965837354));
#206705=CARTESIAN_POINT('Ctrl Pts',(0.614451459526872,6.7416121586937,93.1682457664711));
#206706=CARTESIAN_POINT('Ctrl Pts',(0.428825047910443,6.75339900185711,
93.1769949492068));
#206707=CARTESIAN_POINT('Ctrl Pts',(0.243199888597115,6.76518576550221,
93.1857440729174));
#206708=CARTESIAN_POINT('Ctrl Pts',(0.0570886373918941,6.76931499599834,
93.1944931966279));
#206709=CARTESIAN_POINT('Ctrl Pts',(-0.128876626811264,6.76577266947847,
93.2032423203385));
#206710=CARTESIAN_POINT('Ctrl Pts',(-0.314840698188214,6.76223036567993,
93.21199138793));
#206711=CARTESIAN_POINT('Ctrl Pts',(-0.500658497951248,6.75101660879223,
93.2207404555215));
#206712=CARTESIAN_POINT('Ctrl Pts',(-0.685698951926153,6.73216948296219,
93.2294895231131));
#206713=CARTESIAN_POINT('Ctrl Pts',(-0.870738280459569,6.71332247176296,
93.2382385374916));
#206714=CARTESIAN_POINT('Ctrl Pts',(-1.05499998761201,6.68684221356194,
93.2469875518701));
#206715=CARTESIAN_POINT('Ctrl Pts',(-1.23785829161348,6.65281863948535,
93.2557365662486));
#206716=CARTESIAN_POINT('Ctrl Pts',(-1.43007412917329,6.61705395368877,
93.2649332999478));
#206717=CARTESIAN_POINT('Ctrl Pts',(-1.62073882535714,6.57295372727809,
93.274130033647));
#206718=CARTESIAN_POINT('Ctrl Pts',(-1.80913696091433,6.52068343478302,
93.2833267673462));
#206719=CARTESIAN_POINT('Ctrl Pts',(-1.98838356186031,6.47095219815223,
93.2920767650599));
#206720=CARTESIAN_POINT('Ctrl Pts',(-2.16557827572453,6.41382586850918,
93.3008267627735));
#206721=CARTESIAN_POINT('Ctrl Pts',(-2.3401191862162,6.34949849943307,93.3095767604872));
#206722=CARTESIAN_POINT('Ctrl Pts',(-2.51465655691025,6.2851724349558,93.3183265807455));
#206723=CARTESIAN_POINT('Ctrl Pts',(-2.68653996295261,6.21364572242404,
93.3270764010038));
#206724=CARTESIAN_POINT('Ctrl Pts',(-2.85518555379927,6.13516132252249,
93.3358262212621));
#206725=CARTESIAN_POINT('Ctrl Pts',(-3.0238279485863,6.05667841000536,93.3445758756996));
#206726=CARTESIAN_POINT('Ctrl Pts',(-3.18923239109224,5.97123819492111,
93.3533255301371));
#206727=CARTESIAN_POINT('Ctrl Pts',(-3.35083705967644,5.87913088810744,
93.3620751845746));
#206728=CARTESIAN_POINT('Ctrl Pts',(-3.5124388804233,5.78702520443145,93.3708246848236));
#206729=CARTESIAN_POINT('Ctrl Pts',(-3.67024081223607,5.68825280605837,
93.3795741850725));
#206730=CARTESIAN_POINT('Ctrl Pts',(-3.82370687544305,5.58314917682571,
93.3883236853214));
#206731=CARTESIAN_POINT('Ctrl Pts',(-3.97717043817728,5.47804726008085,
93.3970730430119));
#206732=CARTESIAN_POINT('Ctrl Pts',(-4.12629803722381,5.36661448084297,
93.4058224007024));
#206733=CARTESIAN_POINT('Ctrl Pts',(-4.27058317206837,5.24922931204634,
93.4145717583928));
#206734=CARTESIAN_POINT('Ctrl Pts',(-4.4148661477477,5.13184589986847,93.4233209851529));
#206735=CARTESIAN_POINT('Ctrl Pts',(-4.55430658194353,5.00851045723089,
93.432070211913));
#206736=CARTESIAN_POINT('Ctrl Pts',(-4.6884308900179,4.87964187103172,93.4408194386731));
#206737=CARTESIAN_POINT('Ctrl Pts',(-4.82255336917762,4.75077504208035,
93.449568546129));
#206738=CARTESIAN_POINT('Ctrl Pts',(-4.95135966065043,4.6163754190819,93.4583176535849));
#206739=CARTESIAN_POINT('Ctrl Pts',(-5.07441230869137,4.47689945401966,
93.4670667610408));
#206740=CARTESIAN_POINT('Ctrl Pts',(-5.19746344226328,4.33742520555623,
93.4758157608172));
#206741=CARTESIAN_POINT('Ctrl Pts',(-5.31476088454695,4.19287495491429,
93.4845647605936));
#206742=CARTESIAN_POINT('Ctrl Pts',(-5.42590627628796,4.04373961586783,
93.4933137603699));
#206743=CARTESIAN_POINT('Ctrl Pts',(-5.53706380672614,3.89458798906811,
93.5020637156646));
#206744=CARTESIAN_POINT('Ctrl Pts',(-5.64206777071813,3.7408505015536,93.5108136709593));
#206745=CARTESIAN_POINT('Ctrl Pts',(-5.7405614816396,3.58304938223237,93.519563626254));
#206746=CARTESIAN_POINT('Ctrl Pts',(-5.83905138951835,3.42525435593364,
93.5283132436952));
#206747=CARTESIAN_POINT('Ctrl Pts',(-5.93103139557603,3.26339625497273,
93.5370628611363));
#206748=CARTESIAN_POINT('Ctrl Pts',(-6.01618907820797,3.09802485065101,
93.5458124785774));
#206749=CARTESIAN_POINT('Ctrl Pts',(-6.10134392544937,2.93265895249737,
93.5545618046932));
#206750=CARTESIAN_POINT('Ctrl Pts',(-6.17967677261788,2.76378023986132,
93.5633111308091));
#206751=CARTESIAN_POINT('Ctrl Pts',(-6.25092157009184,2.59196229227214,
93.572060456925));
#206752=CARTESIAN_POINT('Ctrl Pts',(-6.32216437407717,2.42014915229186,
93.5808095382274));
#206753=CARTESIAN_POINT('Ctrl Pts',(-6.38631941548889,2.24539720662942,
93.5895586195299));
#206754=CARTESIAN_POINT('Ctrl Pts',(-6.4431688103751,2.06829994947774,93.5983077008324));
#206755=CARTESIAN_POINT('Ctrl Pts',(-6.50002334524544,1.89118668024543,
93.6070575731747));
#206756=CARTESIAN_POINT('Ctrl Pts',(-6.5495708241107,1.71172794807803,93.615807445517));
#206757=CARTESIAN_POINT('Ctrl Pts',(-6.59164294296059,1.53053334250447,
93.6245573178594));
#206758=CARTESIAN_POINT('Ctrl Pts',(-6.6337121408211,1.34935131693718,93.6333065827143));
#206759=CARTESIAN_POINT('Ctrl Pts',(-6.66830695239667,1.16643393829894,
93.6420558475692));
#206760=CARTESIAN_POINT('Ctrl Pts',(-6.69530988153967,0.982402458342421,
93.6508051124241));
#206761=CARTESIAN_POINT('Ctrl Pts',(-6.72231419690466,0.79836153094851,
93.6595548264311));
#206762=CARTESIAN_POINT('Ctrl Pts',(-6.74172580829264,0.613206671363948,
93.6683045404381));
#206763=CARTESIAN_POINT('Ctrl Pts',(-6.7534787802817,0.427566795114886,
93.6770542544452));
#206764=CARTESIAN_POINT('Ctrl Pts',(-6.76248992368207,0.285234494207059,
93.6837627642334));
#206765=CARTESIAN_POINT('Ctrl Pts',(-6.76699999999992,0.142617266094214,
93.6904712740216));
#206766=CARTESIAN_POINT('Ctrl Pts',(-6.767,3.81860140813756E-12,93.6971797838099));
#206767=CARTESIAN_POINT('',(-6.76699756073415,0.00574569560949348,93.3028202161555));
#206768=CARTESIAN_POINT('Ctrl Pts',(3.09910619832136,6.01563211736939,92.6514522942042));
#206769=CARTESIAN_POINT('Ctrl Pts',(2.94207261405183,6.09653197042874,92.6597505912818));
#206770=CARTESIAN_POINT('Ctrl Pts',(2.78181483905431,6.17130714984468,92.6680488883594));
#206771=CARTESIAN_POINT('Ctrl Pts',(2.61884743168782,6.23970569254209,92.6763471854369));
#206772=CARTESIAN_POINT('Ctrl Pts',(2.4508680467396,6.3102077967317,92.6849006923113));
#206773=CARTESIAN_POINT('Ctrl Pts',(2.28001003531816,6.37393458933078,92.6934541991857));
#206774=CARTESIAN_POINT('Ctrl Pts',(2.10686043388856,6.43066311604915,92.7020077060601));
#206775=CARTESIAN_POINT('Ctrl Pts',(1.93887427303521,6.48569995896189,92.7103061414581));
#206776=CARTESIAN_POINT('Ctrl Pts',(1.76873158870496,6.53414984324859,92.7186045768561));
#206777=CARTESIAN_POINT('Ctrl Pts',(1.59698493863653,6.57585949559205,92.7269030122542));
#206778=CARTESIAN_POINT('Ctrl Pts',(1.42520530402759,6.61757715841907,92.7352030413955));
#206779=CARTESIAN_POINT('Ctrl Pts',(1.25182142793851,6.65255192688433,92.7435030705369));
#206780=CARTESIAN_POINT('Ctrl Pts',(1.07739734666933,6.68068139918301,92.7518030996783));
#206781=CARTESIAN_POINT('Ctrl Pts',(0.902910777742995,6.70882094890225,
92.760106102316));
#206782=CARTESIAN_POINT('Ctrl Pts',(0.727383604427435,6.73011025950068,
92.7684091049538));
#206783=CARTESIAN_POINT('Ctrl Pts',(0.551386481042489,6.74449864322943,
92.7767121075915));
#206784=CARTESIAN_POINT('Ctrl Pts',(0.366057091468037,6.75964997253599,
92.7854553778274));
#206785=CARTESIAN_POINT('Ctrl Pts',(0.180207001970892,6.76714860824585,
92.7941986480633));
#206786=CARTESIAN_POINT('Ctrl Pts',(-0.00549659759097798,6.76699776765258,
92.8029419182992));
#206787=CARTESIAN_POINT('Ctrl Pts',(-0.182160250272311,6.76685426989462,
92.8112595710528));
#206788=CARTESIAN_POINT('Ctrl Pts',(-0.358690993949632,6.75978841471152,
92.8195772238063));
#206789=CARTESIAN_POINT('Ctrl Pts',(-0.534519146364061,6.7458563787091,
92.82789487656));
#206790=CARTESIAN_POINT('Ctrl Pts',(-0.710474373024073,6.73191427376755,
92.8362185406345));
#206791=CARTESIAN_POINT('Ctrl Pts',(-0.885725651466783,6.71109613397475,
92.844542204709));
#206792=CARTESIAN_POINT('Ctrl Pts',(-1.05971193905513,6.68350952765267,
92.8528658687835));
#206793=CARTESIAN_POINT('Ctrl Pts',(-1.23392922408229,6.65588629525221,
92.861200583988));
#206794=CARTESIAN_POINT('Ctrl Pts',(-1.40687782424718,6.62147671746085,
92.8695352991925));
#206795=CARTESIAN_POINT('Ctrl Pts',(-1.57800942395164,6.58043883475257,
92.877870014397));
#206796=CARTESIAN_POINT('Ctrl Pts',(-1.60375249315826,6.57426556776695,
92.879123793072));
#206797=CARTESIAN_POINT('Ctrl Pts',(-1.62945447887022,6.56794240090994,
92.880377571747));
#206798=CARTESIAN_POINT('Ctrl Pts',(-1.65511355105345,6.56146996740206,
92.881631350422));
#206799=CARTESIAN_POINT('Ctrl Pts',(-1.82026611364065,6.51981066762819,
92.8897011964247));
#206800=CARTESIAN_POINT('Ctrl Pts',(-1.98414975799722,6.47183494238821,
92.8977710424275));
#206801=CARTESIAN_POINT('Ctrl Pts',(-2.14623193028149,6.41763020915355,
92.9058408884303));
#206802=CARTESIAN_POINT('Ctrl Pts',(-2.30811018257692,6.36349367236789,
92.9139005815403));
#206803=CARTESIAN_POINT('Ctrl Pts',(-2.46819112315017,6.30314383765067,
92.9219602746503));
#206804=CARTESIAN_POINT('Ctrl Pts',(-2.62595177941827,6.23671918977999,
92.9300199677604));
#206805=CARTESIAN_POINT('Ctrl Pts',(-2.78354857618758,6.17036353445642,
92.938071289599));
#206806=CARTESIAN_POINT('Ctrl Pts',(-2.93882954361198,6.09794576581048,
92.9461226114376));
#206807=CARTESIAN_POINT('Ctrl Pts',(-3.09128638965204,6.01965426392182,
92.9541739332763));
#206808=CARTESIAN_POINT('Ctrl Pts',(-3.24361829353213,5.94142692385735,
92.9622186568573));
#206809=CARTESIAN_POINT('Ctrl Pts',(-3.39313035230538,5.85733560086816,
92.9702633804384));
#206810=CARTESIAN_POINT('Ctrl Pts',(-3.53933390940917,5.76761688028135,
92.9783081040194));
#206811=CARTESIAN_POINT('Ctrl Pts',(-3.68544965310094,5.67795204694007,
92.9863479957438));
#206812=CARTESIAN_POINT('Ctrl Pts',(-3.8282605337627,5.58266673908945,92.9943878874682));
#206813=CARTESIAN_POINT('Ctrl Pts',(-3.96730228755121,5.48204355684912,
93.0024277791926));
#206814=CARTESIAN_POINT('Ctrl Pts',(-4.10933799122855,5.37925368181994,
93.0106407918125));
#206815=CARTESIAN_POINT('Ctrl Pts',(-4.24744005283929,5.27089362854747,
93.0188538044325));
#206816=CARTESIAN_POINT('Ctrl Pts',(-4.38114420888447,5.1573117436275,93.0270668170525));
#206817=CARTESIAN_POINT('Ctrl Pts',(-4.51198436741841,5.04616282897079,
93.035103903595));
#206818=CARTESIAN_POINT('Ctrl Pts',(-4.63861283387288,4.93001378566132,
93.0431409901376));
#206819=CARTESIAN_POINT('Ctrl Pts',(-4.76062789442236,4.80923185663238,
93.0511780766801));
#206820=CARTESIAN_POINT('Ctrl Pts',(-4.88265463238121,4.6884383682105,93.0592159324093));
#206821=CARTESIAN_POINT('Ctrl Pts',(-5.00006681965695,4.56301137397376,
93.0672537881385));
#206822=CARTESIAN_POINT('Ctrl Pts',(-5.1124997964976,4.43335480542805,93.0752916438677));
#206823=CARTESIAN_POINT('Ctrl Pts',(-5.22496581042372,4.30366013885046,
93.0833318614246));
#206824=CARTESIAN_POINT('Ctrl Pts',(-5.33244945706255,4.16973370631207,
93.0913720789815));
#206825=CARTESIAN_POINT('Ctrl Pts',(-5.43462664060732,4.03201218713451,
93.0994122965384));
#206826=CARTESIAN_POINT('Ctrl Pts',(-5.54066414361326,3.88908746072163,
93.1077562786662));
#206827=CARTESIAN_POINT('Ctrl Pts',(-5.64098612335692,3.74207564227954,
93.116100260794));
#206828=CARTESIAN_POINT('Ctrl Pts',(-5.73528054026139,3.59149636286869,
93.1244442429217));
#206829=CARTESIAN_POINT('Ctrl Pts',(-5.82630032911838,3.44614635522084,
93.1324984577568));
#206830=CARTESIAN_POINT('Ctrl Pts',(-5.91170405792819,3.29747286424898,
93.1405526725918));
#206831=CARTESIAN_POINT('Ctrl Pts',(-5.99125894798247,3.14596649985659,
93.1486068874269));
#206832=CARTESIAN_POINT('Ctrl Pts',(-6.07087337171676,2.99434675800357,
93.1566671295099));
#206833=CARTESIAN_POINT('Ctrl Pts',(-6.14463008186374,2.83989025648101,
93.1647273715929));
#206834=CARTESIAN_POINT('Ctrl Pts',(-6.21234493611154,2.68310629583871,
93.1727876136759));
#206835=CARTESIAN_POINT('Ctrl Pts',(-6.2801544603705,2.52610314046481,93.1808591245303));
#206836=CARTESIAN_POINT('Ctrl Pts',(-6.34190514192247,2.36676637884349,
93.1889306353846));
#206837=CARTESIAN_POINT('Ctrl Pts',(-6.39746284724739,2.20561966759669,
93.1970021462389));
#206838=CARTESIAN_POINT('Ctrl Pts',(-6.40328587483431,2.1887298097517,93.1978481248498));
#206839=CARTESIAN_POINT('Ctrl Pts',(-6.40904091765605,2.17182007727671,
93.1986941034606));
#206840=CARTESIAN_POINT('Ctrl Pts',(-6.41472785398784,2.15489107828506,
93.1995400820715));
#206841=CARTESIAN_POINT('Ctrl Pts',(-6.48413205695589,1.94828709794964,
93.2098645288014));
#206842=CARTESIAN_POINT('Ctrl Pts',(-6.54357511398344,1.73825647702735,
93.2201889755314));
#206843=CARTESIAN_POINT('Ctrl Pts',(-6.592774769044,1.52565062994672,93.2305134222613));
#206844=CARTESIAN_POINT('Ctrl Pts',(-6.64160012784474,1.31466222455912,
93.2407593236887));
#206845=CARTESIAN_POINT('Ctrl Pts',(-6.68033733735106,1.10113750658047,
93.251005225116));
#206846=CARTESIAN_POINT('Ctrl Pts',(-6.70875668730291,0.885930420839292,
93.2612511265434));
#206847=CARTESIAN_POINT('Ctrl Pts',(-6.7367317048082,0.674088066912383,
93.2713368347764));
#206848=CARTESIAN_POINT('Ctrl Pts',(-6.75470895760259,0.460615460068659,
93.2814225430094));
#206849=CARTESIAN_POINT('Ctrl Pts',(-6.76251438321489,0.246349785491624,
93.2915082512425));
#206850=CARTESIAN_POINT('Ctrl Pts',(-6.76543252899164,0.166244163527138,
93.2952789062135));
#206851=CARTESIAN_POINT('Ctrl Pts',(-6.76692939501214,0.0860279287729566,
93.2990495611845));
#206852=CARTESIAN_POINT('Ctrl Pts',(-6.76699756073415,0.00574569560929515,
93.3028202161555));
#206853=CARTESIAN_POINT('Ctrl Pts',(-6.76699756073477,0.00574569487926894,
93.3028202161898));
#206854=CARTESIAN_POINT('Ctrl Pts',(-6.7671436277408,-0.166284859165535,
93.3109000594902));
#206855=CARTESIAN_POINT('Ctrl Pts',(-6.76072543132084,-0.338454857998046,
93.3189799027906));
#206856=CARTESIAN_POINT('Ctrl Pts',(-6.74773793184909,-0.51021740766559,
93.327059746091));
#206857=CARTESIAN_POINT('Ctrl Pts',(-6.73475543507659,-0.68191379553035,
93.335136477089));
#206858=CARTESIAN_POINT('Ctrl Pts',(-6.71520869785343,-0.853202677750636,
93.3432132080871));
#206859=CARTESIAN_POINT('Ctrl Pts',(-6.68914476403856,-1.02353862933231,
93.3512899390851));
#206860=CARTESIAN_POINT('Ctrl Pts',(-6.66308569624209,-1.19384277996337,
93.359365162194));
#206861=CARTESIAN_POINT('Ctrl Pts',(-6.6305119087998,-1.36319398784643,
93.3674403853029));
#206862=CARTESIAN_POINT('Ctrl Pts',(-6.59152214198045,-1.53105351042396,
93.3755156084118));
#206863=CARTESIAN_POINT('Ctrl Pts',(-6.55253204053807,-1.6989144736272,
93.383590900825));
#206864=CARTESIAN_POINT('Ctrl Pts',(-6.50712593385131,-1.86528336504561,
93.3916661932381));
#206865=CARTESIAN_POINT('Ctrl Pts',(-6.45545333513781,-2.02963327669265,
93.3997414856512));
#206866=CARTESIAN_POINT('Ctrl Pts',(-6.40377020156673,-2.19401669551671,
93.4078184244312));
#206867=CARTESIAN_POINT('Ctrl Pts',(-6.34581814429612,-2.35637996189023,
93.4158953632113));
#206868=CARTESIAN_POINT('Ctrl Pts',(-6.28179599943399,-2.51621303181888,
93.4239723019913));
#206869=CARTESIAN_POINT('Ctrl Pts',(-6.21771389257149,-2.67619579855353,
93.4320568054883));
#206870=CARTESIAN_POINT('Ctrl Pts',(-6.14755048035773,-2.83364329106876,
93.4401413089853));
#206871=CARTESIAN_POINT('Ctrl Pts',(-6.07155237022323,-2.98806640080783,
93.4482258124823));
#206872=CARTESIAN_POINT('Ctrl Pts',(-5.99551744981171,-3.14256430658379,
93.4563142317716));
#206873=CARTESIAN_POINT('Ctrl Pts',(-5.91364237693362,-3.29403458549646,
93.4644026510609));
#206874=CARTESIAN_POINT('Ctrl Pts',(-5.82621866723013,-3.44201467771698,
93.4724910703501));
#206875=CARTESIAN_POINT('Ctrl Pts',(-5.73867350453855,-3.59020035060252,
93.4805907264389));
#206876=CARTESIAN_POINT('Ctrl Pts',(-5.64556450551341,-3.73488583879291,
93.4886903825276));
#206877=CARTESIAN_POINT('Ctrl Pts',(-5.54722586563247,-3.87563855327843,
93.4967900386163));
#206878=CARTESIAN_POINT('Ctrl Pts',(-5.46361919463534,-3.99530530793551,
93.5036762969846));
#206879=CARTESIAN_POINT('Ctrl Pts',(-5.37623319098954,-4.11212980405513,
93.5105625553527));
#206880=CARTESIAN_POINT('Ctrl Pts',(-5.28529476372309,-4.2258665691857,
93.5174488137209));
#206881=CARTESIAN_POINT('Ctrl Pts',(-5.16728864195111,-4.37345692190449,
93.5263847571717));
#206882=CARTESIAN_POINT('Ctrl Pts',(-5.04302184668053,-4.51619565427602,
93.5353207006224));
#206883=CARTESIAN_POINT('Ctrl Pts',(-4.91289916910149,-4.65356967867054,
93.5442566440732));
#206884=CARTESIAN_POINT('Ctrl Pts',(-4.78297210041976,-4.79073719347021,
93.5531791544308));
#206885=CARTESIAN_POINT('Ctrl Pts',(-4.64720689148205,-4.92255590486862,
93.5621016647885));
#206886=CARTESIAN_POINT('Ctrl Pts',(-4.50604780372686,-5.04854654237517,
93.5710241751461));
#206887=CARTESIAN_POINT('Ctrl Pts',(-4.36523459954218,-5.17422846372152,
93.5799248225845));
#206888=CARTESIAN_POINT('Ctrl Pts',(-4.21905408696584,-5.29411064107391,
93.5888254700228));
#206889=CARTESIAN_POINT('Ctrl Pts',(-4.06798599589699,-5.40775174515121,
93.5977261174611));
#206890=CARTESIAN_POINT('Ctrl Pts',(-3.91715136191804,-5.52121723092777,
93.6066130100474));
#206891=CARTESIAN_POINT('Ctrl Pts',(-3.76144442130983,-5.62846072784876,
93.6154999026337));
#206892=CARTESIAN_POINT('Ctrl Pts',(-3.60137875133706,-5.72908021321206,
93.6243867952199));
#206893=CARTESIAN_POINT('Ctrl Pts',(-3.44172450988688,-5.82944106893782,
93.6332508451749));
#206894=CARTESIAN_POINT('Ctrl Pts',(-3.27773411294933,-5.92321175066983,
93.6421148951298));
#206895=CARTESIAN_POINT('Ctrl Pts',(-3.10995030000059,-6.01003312233188,
93.6509789450847));
#206896=CARTESIAN_POINT('Ctrl Pts',(-2.94953547754915,-6.09304133793616,
93.6594536899051));
#206897=CARTESIAN_POINT('Ctrl Pts',(-2.78565349739834,-6.16969738636362,
93.6679284347254));
#206898=CARTESIAN_POINT('Ctrl Pts',(-2.6188045693501,-6.23972368198713,
93.6764031795457));
#206899=CARTESIAN_POINT('Ctrl Pts',(-2.4571892520777,-6.30755343742514,
93.6846120939748));
#206900=CARTESIAN_POINT('Ctrl Pts',(-2.29294561100739,-6.36909655218897,
93.6928210084039));
#206901=CARTESIAN_POINT('Ctrl Pts',(-2.12660442730655,-6.42416084868368,
93.701029922833));
#206902=CARTESIAN_POINT('Ctrl Pts',(-1.96022369683498,-6.47923823643493,
93.7092407888898));
#206903=CARTESIAN_POINT('Ctrl Pts',(-1.79174476827033,-6.52783362528962,
93.7174516549466));
#206904=CARTESIAN_POINT('Ctrl Pts',(-1.62171364575998,-6.56980470418687,
93.7256625210034));
#206905=CARTESIAN_POINT('Ctrl Pts',(-1.45161179045112,-6.61179324301629,
93.7338768027733));
#206906=CARTESIAN_POINT('Ctrl Pts',(-1.27995680022436,-6.64715189667427,
93.7420910845432));
#206907=CARTESIAN_POINT('Ctrl Pts',(-1.10730501427173,-6.67578943686578,
93.7503053663131));
#206908=CARTESIAN_POINT('Ctrl Pts',(-0.934458895105898,-6.70445921086925,
93.7585288939055));
#206909=CARTESIAN_POINT('Ctrl Pts',(-0.760614090683128,-6.72639270303103,
93.766752421498));
#206910=CARTESIAN_POINT('Ctrl Pts',(-0.586333187500856,-6.74155044431436,
93.7749759490904));
#206911=CARTESIAN_POINT('Ctrl Pts',(-0.411940577039404,-6.75671790112019,
93.7832047476441));
#206912=CARTESIAN_POINT('Ctrl Pts',(-0.237111665358444,-6.76510093255562,
93.7914335461977));
#206913=CARTESIAN_POINT('Ctrl Pts',(-0.0624091373087647,-6.76671220753332,
93.7996623447514));
#206914=CARTESIAN_POINT('Ctrl Pts',(0.112533854790776,-6.76832570030208,
93.8079024695878));
#206915=CARTESIAN_POINT('Ctrl Pts',(0.287349760914585,-6.76314882971623,
93.8161425944243));
#206916=CARTESIAN_POINT('Ctrl Pts',(0.461479900410779,-6.75124620359211,
93.8243827192607));
#206917=CARTESIAN_POINT('Ctrl Pts',(0.538786496261446,-6.74596192879625,
93.8280409946307));
#206918=CARTESIAN_POINT('Ctrl Pts',(0.615958043517288,-6.739352691166,93.8316992700007));
#206919=CARTESIAN_POINT('Ctrl Pts',(0.6929463317061,-6.73142736582481,93.8353575453706));
#206920=CARTESIAN_POINT('Ctrl Pts',(0.870734700620672,-6.71312548252962,
93.8438055681332));
#206921=CARTESIAN_POINT('Ctrl Pts',(1.04795191929681,-6.68775986739998,
93.8522535908957));
#206922=CARTESIAN_POINT('Ctrl Pts',(1.22401382577075,-6.65537971526209,
93.8607016136583));
#206923=CARTESIAN_POINT('Ctrl Pts',(1.39991450709895,-6.62302921459652,
93.869141900314));
#206924=CARTESIAN_POINT('Ctrl Pts',(1.57466165860447,-6.58367704073766,
93.8775821869698));
#206925=CARTESIAN_POINT('Ctrl Pts',(1.74767720129136,-6.53742406457516,
93.8860224736256));
#206926=CARTESIAN_POINT('Ctrl Pts',(1.92056094324894,-6.4912063232586,93.8944563305936));
#206927=CARTESIAN_POINT('Ctrl Pts',(2.09171538498122,-6.4380983451796,93.9028901875615));
#206928=CARTESIAN_POINT('Ctrl Pts',(2.26057320010668,-6.37825193975273,
93.9113240445294));
#206929=CARTESIAN_POINT('Ctrl Pts',(2.42932834091417,-6.31844192404733,
93.9197527732745));
#206930=CARTESIAN_POINT('Ctrl Pts',(2.59578932572333,-6.25190176107784,
93.9281815020195));
#206931=CARTESIAN_POINT('Ctrl Pts',(2.75940416272226,-6.17883303438045,
93.9366102307645));
#206932=CARTESIAN_POINT('Ctrl Pts',(2.92294463857237,-6.10579751661789,
93.9450351287448));
#206933=CARTESIAN_POINT('Ctrl Pts',(3.08364124193321,-6.02623948743528,
93.9534600267251));
#206934=CARTESIAN_POINT('Ctrl Pts',(3.24096177081412,-5.94040872332211,
93.9618849247053));
#206935=CARTESIAN_POINT('Ctrl Pts',(3.39824746867427,-5.8545969622796,93.9703079573995));
#206936=CARTESIAN_POINT('Ctrl Pts',(3.55215828860114,-5.76251539255458,
93.9787309900937));
#206937=CARTESIAN_POINT('Ctrl Pts',(3.70218598865787,-5.66446007183256,
93.9871540227878));
#206938=CARTESIAN_POINT('Ctrl Pts',(3.85219671325051,-5.56641584595887,
93.9955761024254));
#206939=CARTESIAN_POINT('Ctrl Pts',(3.99832491479458,-5.46239939897792,
94.003998182063));
#206940=CARTESIAN_POINT('Ctrl Pts',(4.14009048145941,-5.35275067655212,
94.0124202617006));
#206941=CARTESIAN_POINT('Ctrl Pts',(4.28185979692558,-5.2430990546121,94.0208425640488));
#206942=CARTESIAN_POINT('Ctrl Pts',(4.41926598396192,-5.12781506460663,
94.0292648663971));
#206943=CARTESIAN_POINT('Ctrl Pts',(4.55186094232517,-5.00727979662957,
94.0376871687453));
#206944=CARTESIAN_POINT('Ctrl Pts',(4.6844779173268,-4.88672451445709,94.0461108695689));
#206945=CARTESIAN_POINT('Ctrl Pts',(4.81228182461522,-4.76091644064371,
94.0545345703925));
#206946=CARTESIAN_POINT('Ctrl Pts',(4.93486018483085,-4.63027471713842,
94.0629582712162));
#206947=CARTESIAN_POINT('Ctrl Pts',(5.05752149494364,-4.49954458718429,
94.0713876724352));
#206948=CARTESIAN_POINT('Ctrl Pts',(5.17494996344339,-4.36397451477395,
94.0798170736541));
#206949=CARTESIAN_POINT('Ctrl Pts',(5.28677162918184,-4.22401879030835,
94.0882464748731));
#206950=CARTESIAN_POINT('Ctrl Pts',(5.39863319273521,-4.08401312983478,
94.0966788836907));
#206951=CARTESIAN_POINT('Ctrl Pts',(5.50488376129901,-3.93961896153071,
94.1051112925084));
#206952=CARTESIAN_POINT('Ctrl Pts',(5.60519142255469,-3.79132142089264,
94.113543701326));
#206953=CARTESIAN_POINT('Ctrl Pts',(5.70559189137714,-3.64288667105506,
94.1219839120536));
#206954=CARTESIAN_POINT('Ctrl Pts',(5.80003828501711,-3.49054161288996,
94.1304241227813));
#206955=CARTESIAN_POINT('Ctrl Pts',(5.88824297134146,-3.33479890105054,
94.1388643335089));
#206956=CARTESIAN_POINT('Ctrl Pts',(5.93841229178721,-3.24621510416893,
94.143664981346));
#206957=CARTESIAN_POINT('Ctrl Pts',(5.98656317132938,-3.15653257250145,
94.148465629183));
#206958=CARTESIAN_POINT('Ctrl Pts',(6.03264948575596,-3.06584885178777,
94.1532662770201));
#206959=CARTESIAN_POINT('Ctrl Pts',(6.11079091147118,-2.9120905112935,94.161405992053));
#206960=CARTESIAN_POINT('Ctrl Pts',(6.18315003011602,-2.75514606313375,
94.1695457070858));
#206961=CARTESIAN_POINT('Ctrl Pts',(6.24945581875254,-2.59549435935816,
94.1776854221186));
#206962=CARTESIAN_POINT('Ctrl Pts',(6.31570361674432,-2.43598228600438,
94.1858180182056));
#206963=CARTESIAN_POINT('Ctrl Pts',(6.37590848331387,-2.27376800591042,
94.1939506142925));
#206964=CARTESIAN_POINT('Ctrl Pts',(6.42984539723636,-2.1093546803794,94.2020832103794));
#206965=CARTESIAN_POINT('Ctrl Pts',(6.48374543699039,-1.94505375661961,
94.2102102465873));
#206966=CARTESIAN_POINT('Ctrl Pts',(6.53138594184629,-1.77855712712222,
94.2183372827952));
#206967=CARTESIAN_POINT('Ctrl Pts',(6.5725901133903,-1.61038759352028,94.2264643190031));
#206968=CARTESIAN_POINT('Ctrl Pts',(6.61377458859492,-1.44229844799767,
94.2345874703406));
#206969=CARTESIAN_POINT('Ctrl Pts',(6.64852877021056,-1.27253834572459,
94.2427106216782));
#206970=CARTESIAN_POINT('Ctrl Pts',(6.67672581118828,-1.10164488026417,
94.2508337730157));
#206971=CARTESIAN_POINT('Ctrl Pts',(6.70491492858801,-0.930799437137095,
94.2589546416874));
#206972=CARTESIAN_POINT('Ctrl Pts',(6.72655051667087,-0.75882162631679,
94.2670755103591));
#206973=CARTESIAN_POINT('Ctrl Pts',(6.74155691183685,-0.586258820372734,
94.2751963790307));
#206974=CARTESIAN_POINT('Ctrl Pts',(6.7565641180058,-0.413686688474876,
94.2833176865852));
#206975=CARTESIAN_POINT('Ctrl Pts',(6.76494137982004,-0.240529862795474,
94.2914389941397));
#206976=CARTESIAN_POINT('Ctrl Pts',(6.76666492757033,-0.0673406117405915,
94.2995603016942));
#206977=CARTESIAN_POINT('Ctrl Pts',(6.76756054289508,0.0226545434845253,
94.3037804154111));
#206978=CARTESIAN_POINT('Ctrl Pts',(6.76666037691786,0.112658408977732,
94.308000529128));
#206979=CARTESIAN_POINT('Ctrl Pts',(6.76396665283788,0.202593482859393,
94.3122206428449));
#206980=CARTESIAN_POINT('Ctrl Pts',(6.7582318314502,0.394061342924849,94.3212050813707));
#206981=CARTESIAN_POINT('Ctrl Pts',(6.74436776794409,0.585122379039508,
94.3301895198965));
#206982=CARTESIAN_POINT('Ctrl Pts',(6.72246167560015,0.775111617824945,
94.3391739584224));
#206983=CARTESIAN_POINT('Ctrl Pts',(6.70051777464833,0.965428766696629,
94.3481739035528));
#206984=CARTESIAN_POINT('Ctrl Pts',(6.67050412973394,1.1546701834502,94.3571738486833));
#206985=CARTESIAN_POINT('Ctrl Pts',(6.63255931114618,1.34217956478561,94.3661737938138));
#206986=CARTESIAN_POINT('Ctrl Pts',(6.59452507461947,1.53013081679105,94.375194947546));
#206987=CARTESIAN_POINT('Ctrl Pts',(6.54852231632505,1.71634163162484,94.3842161012782));
#206988=CARTESIAN_POINT('Ctrl Pts',(6.49474060721642,1.90016668873393,94.3932372550104));
#206989=CARTESIAN_POINT('Ctrl Pts',(6.44090417479457,2.08417878928858,94.4022675878376));
#206990=CARTESIAN_POINT('Ctrl Pts',(6.37927305184458,2.26580005505941,94.4112979206649));
#206991=CARTESIAN_POINT('Ctrl Pts',(6.31008612126959,2.44440220548111,94.4203282534922));
#206992=CARTESIAN_POINT('Ctrl Pts',(6.24080110543641,2.62325755745248,94.4293713884848));
#206993=CARTESIAN_POINT('Ctrl Pts',(6.16393894993225,2.79908501286153,94.4384145234775));
#206994=CARTESIAN_POINT('Ctrl Pts',(6.07978686387173,2.9712759363433,94.4474576584701));
#206995=CARTESIAN_POINT('Ctrl Pts',(6.00621855314991,3.1218104739313,94.4553634418699));
#206996=CARTESIAN_POINT('Ctrl Pts',(5.92707946764804,3.26956594019165,94.4632692252698));
#206997=CARTESIAN_POINT('Ctrl Pts',(5.84259004176172,3.4141515203498,94.4711750086696));
#206998=CARTESIAN_POINT('Ctrl Pts',(5.75011093293703,3.57240973386773,94.4798283968978));
#206999=CARTESIAN_POINT('Ctrl Pts',(5.6511389163362,3.72700935470634,94.4884817851261));
#207000=CARTESIAN_POINT('Ctrl Pts',(5.5459820708745,3.87741819636967,94.4971351733544));
#207001=CARTESIAN_POINT('Ctrl Pts',(5.44092234521913,4.02768812479813,94.5057805695647));
#207002=CARTESIAN_POINT('Ctrl Pts',(5.32968935726328,4.17377474551138,94.5144259657751));
#207003=CARTESIAN_POINT('Ctrl Pts',(5.21263527468974,4.31517351830263,94.5230713619855));
#207004=CARTESIAN_POINT('Ctrl Pts',(5.09184287902795,4.46108809157999,94.5319928630279));
#207005=CARTESIAN_POINT('Ctrl Pts',(4.96485157862196,4.60201014718321,94.5409143640703));
#207006=CARTESIAN_POINT('Ctrl Pts',(4.8320959348139,4.73741890450433,94.5498358651127));
#207007=CARTESIAN_POINT('Ctrl Pts',(4.70369386463786,4.86838708228767,94.5584647954546));
#207008=CARTESIAN_POINT('Ctrl Pts',(4.56989974694032,4.99419757961759,94.5670937257966));
#207009=CARTESIAN_POINT('Ctrl Pts',(4.43114705478339,5.11441343448929,94.5757226561386));
#207010=CARTESIAN_POINT('Ctrl Pts',(4.28533758315489,5.24074330966307,94.5847904425312));
#207011=CARTESIAN_POINT('Ctrl Pts',(4.1340522368523,5.36089437811868,94.5938582289238));
#207012=CARTESIAN_POINT('Ctrl Pts',(3.97783754250411,5.47440384749288,94.6029260153164));
#207013=CARTESIAN_POINT('Ctrl Pts',(3.82162284815593,5.58791331686708,94.611993801709));
#207014=CARTESIAN_POINT('Ctrl Pts',(3.66047910098683,5.6947809291248,94.6210615881017));
#207015=CARTESIAN_POINT('Ctrl Pts',(3.49499323025666,5.7945932834376,94.6301293744943));
#207016=CARTESIAN_POINT('Ctrl Pts',(3.36553668759303,5.87267464619951,94.6372229364451));
#207017=CARTESIAN_POINT('Ctrl Pts',(3.23347124895921,5.94641053713559,94.6443164983958));
#207018=CARTESIAN_POINT('Ctrl Pts',(3.09910619832125,6.01563211736945,94.6514100603466));
#207019=CARTESIAN_POINT('Origin',(0.,0.,4.30282021618968));
#207020=CARTESIAN_POINT('',(3.09910619832136,6.01563211736939,97.0457552630242));
#207021=CARTESIAN_POINT('',(3.09910619832137,6.01563211736939,96.6512761190133));
#207022=CARTESIAN_POINT('',(3.09910619832133,6.0156321173694,4.30282021618968));
#207023=CARTESIAN_POINT('',(-6.767,3.9611911840931E-12,95.6971797838099));
#207024=CARTESIAN_POINT('Ctrl Pts',(-6.767,4.34585066737734E-12,95.6971797838099));
#207025=CARTESIAN_POINT('Ctrl Pts',(-6.76700000000012,-0.186007249522647,
95.7059292956211));
#207026=CARTESIAN_POINT('Ctrl Pts',(-6.75932637294543,-0.37201435574582,
95.7146788074323));
#207027=CARTESIAN_POINT('Ctrl Pts',(-6.74400518264213,-0.557389537483525,
95.7234283192435));
#207028=CARTESIAN_POINT('Ctrl Pts',(-6.72868405705128,-0.742763936248029,
95.7321777940992));
#207029=CARTESIAN_POINT('Ctrl Pts',(-6.70571545645775,-0.927506130238709,
95.7409272689549));
#207030=CARTESIAN_POINT('Ctrl Pts',(-6.67517739404857,-1.11098863989826,
95.7496767438105));
#207031=CARTESIAN_POINT('Ctrl Pts',(-6.64463945808734,-1.2944703898178,
95.7584261824376));
#207032=CARTESIAN_POINT('Ctrl Pts',(-6.60653217008387,-1.47669218313541,
95.7671756210646));
#207033=CARTESIAN_POINT('Ctrl Pts',(-6.56098496092707,-1.65703510599166,
95.7759250596916));
#207034=CARTESIAN_POINT('Ctrl Pts',(-6.51543793658327,-1.83737729708592,
95.7846744628168));
#207035=CARTESIAN_POINT('Ctrl Pts',(-6.46245112167451,-2.0158403551083,
95.7934238659419));
#207036=CARTESIAN_POINT('Ctrl Pts',(-6.40220448374283,-2.19181813760706,
95.8021732690671));
#207037=CARTESIAN_POINT('Ctrl Pts',(-6.34195808526528,-2.36779522067079,
95.8109226374172));
#207038=CARTESIAN_POINT('Ctrl Pts',(-6.27445201433122,-2.54128677684122,
95.8196720057673));
#207039=CARTESIAN_POINT('Ctrl Pts',(-6.19991555071912,-2.71170355384789,
95.8284213741174));
#207040=CARTESIAN_POINT('Ctrl Pts',(-6.12537937716708,-2.88211966767442,
95.8371707084192));
#207041=CARTESIAN_POINT('Ctrl Pts',(-6.04381298052543,-3.04946076371738,
95.845920042721));
#207042=CARTESIAN_POINT('Ctrl Pts',(-5.95549339335863,-3.21315848374488,
95.8546693770228));
#207043=CARTESIAN_POINT('Ctrl Pts',(-5.86717414255438,-3.37685558033442,
95.8634186780029));
#207044=CARTESIAN_POINT('Ctrl Pts',(-5.77210188876624,-3.53690907646714,
95.8721679789831));
#207045=CARTESIAN_POINT('Ctrl Pts',(-5.67059953347018,-3.69277536969252,
95.8809172799633));
#207046=CARTESIAN_POINT('Ctrl Pts',(-5.569097556314,-3.848641082249,95.8896665483486));
#207047=CARTESIAN_POINT('Ctrl Pts',(-5.4611656819686,-4.00031938297504,
95.8984158167339));
#207048=CARTESIAN_POINT('Ctrl Pts',(-5.34717048533606,-4.14729511859851,
95.9071650851192));
#207049=CARTESIAN_POINT('Ctrl Pts',(-5.23317570391852,-4.29427031887897,
95.9159143216362));
#207050=CARTESIAN_POINT('Ctrl Pts',(-5.11311782003543,-4.43654276189513,
95.9246635581532));
#207051=CARTESIAN_POINT('Ctrl Pts',(-4.98740458984797,-4.57362924351804,
95.9334127946703));
#207052=CARTESIAN_POINT('Ctrl Pts',(-4.86169180711801,-4.71071523720206,
95.9421620000457));
#207053=CARTESIAN_POINT('Ctrl Pts',(-4.73032391204244,-4.84261509523166,
95.9509112054211));
#207054=CARTESIAN_POINT('Ctrl Pts',(-4.59374707013688,-4.96888084538247,
95.9596604107966));
#207055=CARTESIAN_POINT('Ctrl Pts',(-4.45717070301531,-5.09514615659389,
95.968409585757));
#207056=CARTESIAN_POINT('Ctrl Pts',(-4.31538563571123,-5.2157772045946,
95.9771587607175));
#207057=CARTESIAN_POINT('Ctrl Pts',(-4.16887341029587,-5.33036429232826,
95.9859079356779));
#207058=CARTESIAN_POINT('Ctrl Pts',(-4.02236168203777,-5.44495099123564,
95.99465708095));
#207059=CARTESIAN_POINT('Ctrl Pts',(-3.87112305348229,-5.55349359438558,
96.003406226222));
#207060=CARTESIAN_POINT('Ctrl Pts',(-3.71567117017816,-5.65562346298857,
96.012155371494));
#207061=CARTESIAN_POINT('Ctrl Pts',(-3.56021980145874,-5.7577529935161,
96.0209044878042));
#207062=CARTESIAN_POINT('Ctrl Pts',(-3.40055544538404,-5.85346967463841,
96.0296536041143));
#207063=CARTESIAN_POINT('Ctrl Pts',(-3.23722035986908,-5.94244842986871,
96.0384027204245));
#207064=CARTESIAN_POINT('Ctrl Pts',(-3.0738858014723,-6.03142689794504,
96.0471518084994));
#207065=CARTESIAN_POINT('Ctrl Pts',(-2.90688078896622,-6.11366734656761,
96.0559008965742));
#207066=CARTESIAN_POINT('Ctrl Pts',(-2.73677250721408,-6.18889046952337,
96.064649984649));
#207067=CARTESIAN_POINT('Ctrl Pts',(-2.56666476031511,-6.26411335596316,
96.0733990452151));
#207068=CARTESIAN_POINT('Ctrl Pts',(-2.39345402575184,-6.33231884500549,
96.0821481057811));
#207069=CARTESIAN_POINT('Ctrl Pts',(-2.21772856065599,-6.39327529762724,
96.0908971663472));
#207070=CARTESIAN_POINT('Ctrl Pts',(-2.04200363348504,-6.45423156365115,
96.0996462001309));
#207071=CARTESIAN_POINT('Ctrl Pts',(-1.86376426189252,-6.50793874375666,
96.1083952339145));
#207072=CARTESIAN_POINT('Ctrl Pts',(-1.6836157775311,-6.55421443909553,
96.1171442676983));
#207073=CARTESIAN_POINT('Ctrl Pts',(-1.50346782967756,-6.60048999661878,
96.1258932754261));
#207074=CARTESIAN_POINT('Ctrl Pts',(-1.32141105794943,-6.63933404237721,
96.1346422831539));
#207075=CARTESIAN_POINT('Ctrl Pts',(-1.13806375486979,-6.67061465607568,
96.1433912908817));
#207076=CARTESIAN_POINT('Ctrl Pts',(-0.954716982602963,-6.70189517921296,
96.1521402732801));
#207077=CARTESIAN_POINT('Ctrl Pts',(-0.770079968902468,-6.72561226592223,
96.1608892556785));
#207078=CARTESIAN_POINT('Ctrl Pts',(-0.584779765558964,-6.74168536983096,
96.1696382380769));
#207079=CARTESIAN_POINT('Ctrl Pts',(-0.391489830652015,-6.75845151013849,
96.1787644570868));
#207080=CARTESIAN_POINT('Ctrl Pts',(-0.197478578239049,-6.76689983031623,
96.1878906760966));
#207081=CARTESIAN_POINT('Ctrl Pts',(-0.00346287645205357,-6.76699911397118,
96.1970168951065));
#207082=CARTESIAN_POINT('Ctrl Pts',(0.184489834654066,-6.76709529501191,
96.2058579197723));
#207083=CARTESIAN_POINT('Ctrl Pts',(0.372446404249543,-6.75935639738167,
96.2146989444381));
#207084=CARTESIAN_POINT('Ctrl Pts',(0.559755019488502,-6.74380925873185,
96.2235399691039));
#207085=CARTESIAN_POINT('Ctrl Pts',(0.745134705521925,-6.72842222659804,
96.2322899477137));
#207086=CARTESIAN_POINT('Ctrl Pts',(0.929879431228705,-6.70538706057522,
96.2410399263234));
#207087=CARTESIAN_POINT('Ctrl Pts',(1.11336163626838,-6.67478200894125,
96.2497899049332));
#207088=CARTESIAN_POINT('Ctrl Pts',(1.2968419630075,-6.64417727061007,96.2585397939697));
#207089=CARTESIAN_POINT('Ctrl Pts',(1.4790595121756,-6.6060028489058,96.2672896830062));
#207090=CARTESIAN_POINT('Ctrl Pts',(1.65939532067153,-6.56038841607213,
96.2760395720427));
#207091=CARTESIAN_POINT('Ctrl Pts',(1.8397293430086,-6.5147744350324,96.2847893744149));
#207092=CARTESIAN_POINT('Ctrl Pts',(2.01818138406312,-6.46172066062126,
96.2935391767871));
#207093=CARTESIAN_POINT('Ctrl Pts',(2.19414528354237,-6.40140730423466,
96.3022889791592));
#207094=CARTESIAN_POINT('Ctrl Pts',(2.37010749864039,-6.34109452518628,
96.3110386977755));
#207095=CARTESIAN_POINT('Ctrl Pts',(2.543581348665,-6.27352239616488,96.3197884163918));
#207096=CARTESIAN_POINT('Ctrl Pts',(2.71397759435597,-6.19892043966801,
96.3285381350082));
#207097=CARTESIAN_POINT('Ctrl Pts',(2.88437226558162,-6.12431917249497,
96.3372877727769));
#207098=CARTESIAN_POINT('Ctrl Pts',(3.05168912680989,-6.04268832278782,
96.3460374105456));
#207099=CARTESIAN_POINT('Ctrl Pts',(3.21535986273884,-5.95430516123318,
96.3547870483143));
#207100=CARTESIAN_POINT('Ctrl Pts',(3.37902914072867,-5.86592278697426,
96.3635366081434));
#207101=CARTESIAN_POINT('Ctrl Pts',(3.53905210621594,-5.77078835741928,
96.3722861679724));
#207102=CARTESIAN_POINT('Ctrl Pts',(3.69488522831715,-5.66922500431617,
96.3810357278015));
#207103=CARTESIAN_POINT('Ctrl Pts',(3.85071701406964,-5.56766252217076,
96.3897852125986));
#207104=CARTESIAN_POINT('Ctrl Pts',(4.00235878822435,-5.45967138329347,
96.3985346973957));
#207105=CARTESIAN_POINT('Ctrl Pts',(4.14929549611362,-5.34561838199579,
96.4072841821929));
#207106=CARTESIAN_POINT('Ctrl Pts',(4.29623099276123,-5.23156632086988,
96.4160335948654));
#207107=CARTESIAN_POINT('Ctrl Pts',(4.43846127436058,-5.11145267304938,
96.424783007538));
#207108=CARTESIAN_POINT('Ctrl Pts',(4.57550326054469,-4.9856854004986,96.4335324202106));
#207109=CARTESIAN_POINT('Ctrl Pts',(4.71254416257796,-4.85991912290345,
96.4422817636658));
#207110=CARTESIAN_POINT('Ctrl Pts',(4.84439664018766,-4.72849950385413,
96.4510311071211));
#207111=CARTESIAN_POINT('Ctrl Pts',(4.97061286794741,-4.59187289861073,
96.4597804505763));
#207112=CARTESIAN_POINT('Ctrl Pts',(5.09682813912685,-4.45524732884685,
96.4685297277212));
#207113=CARTESIAN_POINT('Ctrl Pts',(5.21740705147843,-4.31341506235783,
96.477279004866));
#207114=CARTESIAN_POINT('Ctrl Pts',(5.33194007545704,-4.16685781275714,
96.4860282820108));
#207115=CARTESIAN_POINT('Ctrl Pts',(5.44647226944489,-4.02030162521836,
96.4947774957519));
#207116=CARTESIAN_POINT('Ctrl Pts',(5.55495848628114,-3.86902074887933,
96.5035267094931));
#207117=CARTESIAN_POINT('Ctrl Pts',(5.65703027291785,-3.71352898080667,
96.5122759232342));
#207118=CARTESIAN_POINT('Ctrl Pts',(5.75910135376988,-3.55803828789603,
96.5210250764781));
#207119=CARTESIAN_POINT('Ctrl Pts',(5.85475793592737,-3.39833700106738,
96.5297742297219));
#207120=CARTESIAN_POINT('Ctrl Pts',(5.94367514427378,-3.23496750823592,
96.5385233829658));
#207121=CARTESIAN_POINT('Ctrl Pts',(6.0325917673262,-3.07159909077764,96.5472724786187));
#207122=CARTESIAN_POINT('Ctrl Pts',(6.11476896835905,-2.90456276731474,
96.5560215742717));
#207123=CARTESIAN_POINT('Ctrl Pts',(6.18992765547868,-2.73442583003091,
96.5647706699246));
#207124=CARTESIAN_POINT('Ctrl Pts',(6.26508587283041,-2.56428995616202,
96.5735197108926));
#207125=CARTESIAN_POINT('Ctrl Pts',(6.33322554827152,-2.39105376935225,
96.5822687518607));
#207126=CARTESIAN_POINT('Ctrl Pts',(6.39411526733026,-2.21530561054093,
96.5910177928287));
#207127=CARTESIAN_POINT('Ctrl Pts',(6.45500462602837,-2.0395584918513,96.5997667820177));
#207128=CARTESIAN_POINT('Ctrl Pts',(6.50864402040725,-1.86129970164594,
96.6085157712068));
#207129=CARTESIAN_POINT('Ctrl Pts',(6.55485128368583,-1.68113463136127,
96.6172647603958));
#207130=CARTESIAN_POINT('Ctrl Pts',(6.6019980955431,-1.49730620116944,96.6261916458672));
#207131=CARTESIAN_POINT('Ctrl Pts',(6.64140720707857,-1.3114934324578,96.6351185313386));
#207132=CARTESIAN_POINT('Ctrl Pts',(6.67293928722869,-1.12435326697614,
96.6440454168101));
#207133=CARTESIAN_POINT('Ctrl Pts',(6.70384625876244,-0.940923067007474,
96.6527953309875));
#207134=CARTESIAN_POINT('Ctrl Pts',(6.72718554579786,-0.756217899522548,
96.661545245165));
#207135=CARTESIAN_POINT('Ctrl Pts',(6.7428778681532,-0.570865181255377,
96.6702951593425));
#207136=CARTESIAN_POINT('Ctrl Pts',(6.7585698819084,-0.38551610807487,96.6790449014469));
#207137=CARTESIAN_POINT('Ctrl Pts',(6.766615207734,-0.199519795227315,96.6877946435514));
#207138=CARTESIAN_POINT('Ctrl Pts',(6.76698651789579,-0.0135080204566571,
96.6965443856559));
#207139=CARTESIAN_POINT('Ctrl Pts',(6.76735782124905,0.17250034351191,96.7052939673209));
#207140=CARTESIAN_POINT('Ctrl Pts',(6.76005538995189,0.35852388220983,96.7140435489858));
#207141=CARTESIAN_POINT('Ctrl Pts',(6.7451040274237,0.543930748563247,96.7227931306508));
#207142=CARTESIAN_POINT('Ctrl Pts',(6.73015291918043,0.729334461614134,
96.7315425635075));
#207143=CARTESIAN_POINT('Ctrl Pts',(6.70755316306609,0.914121237633609,
96.7402919963642));
#207144=CARTESIAN_POINT('Ctrl Pts',(6.67738151874591,1.09766345166018,96.7490414292209));
#207145=CARTESIAN_POINT('Ctrl Pts',(6.64721034747589,1.28120278799564,96.7577907248984));
#207146=CARTESIAN_POINT('Ctrl Pts',(6.60946757205163,1.46349731860232,96.7665400205759));
#207147=CARTESIAN_POINT('Ctrl Pts',(6.56428138111546,1.64392790278068,96.7752893162534));
#207148=CARTESIAN_POINT('Ctrl Pts',(6.51909583859876,1.82435589778962,96.784038486379));
#207149=CARTESIAN_POINT('Ctrl Pts',(6.46646716392905,2.00291972192171,96.7927876565046));
#207150=CARTESIAN_POINT('Ctrl Pts',(6.40657409872916,2.17901292274569,96.8015368266302));
#207151=CARTESIAN_POINT('Ctrl Pts',(6.34668181342111,2.35510383058884,96.8102858828293));
#207152=CARTESIAN_POINT('Ctrl Pts',(6.27952541914087,2.52872390822489,96.8190349390285));
#207153=CARTESIAN_POINT('Ctrl Pts',(6.20533299175556,2.69928350890195,96.8277839952276));
#207154=CARTESIAN_POINT('Ctrl Pts',(6.12831602991585,2.87633637965547,96.8368661313858));
#207155=CARTESIAN_POINT('Ctrl Pts',(6.04371690605303,3.05009086601398,96.845948267544));
#207156=CARTESIAN_POINT('Ctrl Pts',(5.95184520316659,3.21991112882683,96.8550304037022));
#207157=CARTESIAN_POINT('Ctrl Pts',(5.86333549509301,3.38351691182972,96.8637801840457));
#207158=CARTESIAN_POINT('Ctrl Pts',(5.76807618099393,3.54347103711965,96.8725299643893));
#207159=CARTESIAN_POINT('Ctrl Pts',(5.66639083309038,3.69923018027662,96.8812797447329));
#207160=CARTESIAN_POINT('Ctrl Pts',(5.56470914082218,3.85498372382024,96.8900292105178));
#207161=CARTESIAN_POINT('Ctrl Pts',(5.4566020337208,4.0065423470198,96.8987786763027));
#207162=CARTESIAN_POINT('Ctrl Pts',(5.34243669839225,4.15339127986658,96.9075281420876));
#207163=CARTESIAN_POINT('Ctrl Pts',(5.22827486050601,4.30023571401268,96.9162773398336));
#207164=CARTESIAN_POINT('Ctrl Pts',(5.10805534167121,4.44237052028458,96.9250265375796));
#207165=CARTESIAN_POINT('Ctrl Pts',(4.98218644339962,4.57931296628709,96.9337757353256));
#207166=CARTESIAN_POINT('Ctrl Pts',(4.85632073219602,4.71625194483345,96.9425247115373));
#207167=CARTESIAN_POINT('Ctrl Pts',(4.72480612170339,4.84799861524488,96.9512736877489));
#207168=CARTESIAN_POINT('Ctrl Pts',(4.58808925235337,4.97410554898461,96.9600226639605));
#207169=CARTESIAN_POINT('Ctrl Pts',(4.45136349474075,5.10022068121183,96.9687722089622));
#207170=CARTESIAN_POINT('Ctrl Pts',(4.30943501210109,5.2206951487181,96.977521753964));
#207171=CARTESIAN_POINT('Ctrl Pts',(4.16278587431812,5.33511975166233,96.9862712989657));
#207172=CARTESIAN_POINT('Ctrl Pts',(4.01614535740482,5.44953762807817,96.9950203296194));
#207173=CARTESIAN_POINT('Ctrl Pts',(3.86478496657961,5.55790617532758,97.0037693602731));
#207174=CARTESIAN_POINT('Ctrl Pts',(3.70921874747237,5.65985735539329,97.0125183909268));
#207175=CARTESIAN_POINT('Ctrl Pts',(3.55365041605945,5.76180991977019,97.0212675403764));
#207176=CARTESIAN_POINT('Ctrl Pts',(3.39387638174569,5.85734478552786,97.0300166898261));
#207177=CARTESIAN_POINT('Ctrl Pts',(3.23043927904589,5.94613749121205,97.0387658392757));
#207178=CARTESIAN_POINT('Ctrl Pts',(3.18691767070463,5.9697820694413,97.0410956471919));
#207179=CARTESIAN_POINT('Ctrl Pts',(3.14313645919646,5.99294880633418,97.043425455108));
#207180=CARTESIAN_POINT('Ctrl Pts',(3.09910619832136,6.01563211736939,97.0457552630242));
#207181=CARTESIAN_POINT('Ctrl Pts',(3.09910619832144,6.01563211736935,95.0455663730808));
#207182=CARTESIAN_POINT('Ctrl Pts',(2.94398460122206,6.09554696150953,95.0537894768725));
#207183=CARTESIAN_POINT('Ctrl Pts',(2.78592596187934,6.1693775730439,95.0620125806642));
#207184=CARTESIAN_POINT('Ctrl Pts',(2.62545481752041,6.23692841077712,95.0702356844558));
#207185=CARTESIAN_POINT('Ctrl Pts',(2.54683969676187,6.27002169547297,95.0742641987422));
#207186=CARTESIAN_POINT('Ctrl Pts',(2.46764580997816,6.30160856605184,95.0782927130285));
#207187=CARTESIAN_POINT('Ctrl Pts',(2.38793604010017,6.331670432705,95.0823212273148));
#207188=CARTESIAN_POINT('Ctrl Pts',(2.21112594449757,6.39835286730585,95.0912571707656));
#207189=CARTESIAN_POINT('Ctrl Pts',(2.03140856638816,6.45766767263564,95.1001931142163));
#207190=CARTESIAN_POINT('Ctrl Pts',(1.84939388817998,6.50938025055862,95.109129057667));
#207191=CARTESIAN_POINT('Ctrl Pts',(1.66765282630942,6.56101509076109,95.1180515680247));
#207192=CARTESIAN_POINT('Ctrl Pts',(1.48362160296594,6.60507043626395,95.1269740783823));
#207193=CARTESIAN_POINT('Ctrl Pts',(1.2979268806446,6.64136091569342,95.13589658874));
#207194=CARTESIAN_POINT('Ctrl Pts',(1.11268716801945,6.6775624721863,95.1447972361783));
#207195=CARTESIAN_POINT('Ctrl Pts',(0.925792344517236,6.7060370863505,95.1536978836166));
#207196=CARTESIAN_POINT('Ctrl Pts',(0.737880206460599,6.72665011732539,
95.162598531055));
#207197=CARTESIAN_POINT('Ctrl Pts',(0.550258463421176,6.74723129340497,
95.1714854236412));
#207198=CARTESIAN_POINT('Ctrl Pts',(0.361622797206337,6.75997509256352,
95.1803723162275));
#207199=CARTESIAN_POINT('Ctrl Pts',(0.172620047030761,6.76479795111156,
95.1892592088138));
#207200=CARTESIAN_POINT('Ctrl Pts',(-0.0158968955242036,6.7696084131128,
95.1981232587687));
#207201=CARTESIAN_POINT('Ctrl Pts',(-0.204778781918719,6.76653855445609,
95.2069873087236));
#207202=CARTESIAN_POINT('Ctrl Pts',(-0.393375586261886,6.75555657574808,
95.2158513586785));
#207203=CARTESIAN_POINT('Ctrl Pts',(-0.573689302776424,6.7450569206642,
95.2243261034989));
#207204=CARTESIAN_POINT('Ctrl Pts',(-0.753742179121024,6.7273251723314,
95.2328008483192));
#207205=CARTESIAN_POINT('Ctrl Pts',(-0.9329623871501,6.70237794996397,95.2412755931395));
#207206=CARTESIAN_POINT('Ctrl Pts',(-1.10656092998103,6.67821325615911,
95.2494845075686));
#207207=CARTESIAN_POINT('Ctrl Pts',(-1.27921074848217,6.64730098063199,
95.2576934219978));
#207208=CARTESIAN_POINT('Ctrl Pts',(-1.45035732016783,6.6097467912043,95.2659023364269));
#207209=CARTESIAN_POINT('Ctrl Pts',(-1.62154458108142,6.57218367345887,
95.2741132024837));
#207210=CARTESIAN_POINT('Ctrl Pts',(-1.79122753534553,6.52797557215911,
95.2823240685405));
#207211=CARTESIAN_POINT('Ctrl Pts',(-1.95886402317029,6.47727880662313,
95.2905349345973));
#207212=CARTESIAN_POINT('Ctrl Pts',(-2.12657024762539,6.42656095127762,
95.2987492163671));
#207213=CARTESIAN_POINT('Ctrl Pts',(-2.29222796905997,6.36934915715565,
95.3069634981369));
#207214=CARTESIAN_POINT('Ctrl Pts',(-2.45531221441518,6.30584894599796,
95.3151777799067));
#207215=CARTESIAN_POINT('Ctrl Pts',(-2.618580023963,6.24227726033969,95.3234013074991));
#207216=CARTESIAN_POINT('Ctrl Pts',(-2.77926823992194,6.17240314957602,
95.3316248350915));
#207217=CARTESIAN_POINT('Ctrl Pts',(-2.9368729363965,6.09647983310548,95.3398483626839));
#207218=CARTESIAN_POINT('Ctrl Pts',(-3.09457865135069,6.02050785274249,
95.3480771612376));
#207219=CARTESIAN_POINT('Ctrl Pts',(-3.24919659322046,5.9384791039557,95.3563059597913));
#207220=CARTESIAN_POINT('Ctrl Pts',(-3.40024936417954,5.85069169085132,
95.364534758345));
#207221=CARTESIAN_POINT('Ctrl Pts',(-3.55151004719001,5.76278344539789,
95.3727748831814));
#207222=CARTESIAN_POINT('Ctrl Pts',(-3.69919545785659,5.66910089366582,
95.3810150080178));
#207223=CARTESIAN_POINT('Ctrl Pts',(-3.84285815269377,5.5699847592498,95.3892551328542));
#207224=CARTESIAN_POINT('Ctrl Pts',(-3.90663846046189,5.52598128594028,
95.3929134082243));
#207225=CARTESIAN_POINT('Ctrl Pts',(-3.96962633961643,5.48090738209684,
95.3965716835943));
#207226=CARTESIAN_POINT('Ctrl Pts',(-4.03178486307862,5.43479528757525,
95.4002299589643));
#207227=CARTESIAN_POINT('Ctrl Pts',(-4.17399707305187,5.32929563116208,
95.4085997109481));
#207228=CARTESIAN_POINT('Ctrl Pts',(-4.31220732511742,5.21810561209049,
95.416969462932));
#207229=CARTESIAN_POINT('Ctrl Pts',(-4.44594362259907,5.10155606699276,
95.4253392149158));
#207230=CARTESIAN_POINT('Ctrl Pts',(-4.57955297740067,4.98511715088576,
95.4337010223194));
#207231=CARTESIAN_POINT('Ctrl Pts',(-4.70869658297601,4.86332907027042,
95.442062829723));
#207232=CARTESIAN_POINT('Ctrl Pts',(-4.83293364915331,4.73656429734482,
95.4504246371266));
#207233=CARTESIAN_POINT('Ctrl Pts',(-4.95707439156866,4.60989780796848,
95.4587799614349));
#207234=CARTESIAN_POINT('Ctrl Pts',(-5.07631593703795,4.47826256013943,
95.4671352857431));
#207235=CARTESIAN_POINT('Ctrl Pts',(-5.19025245315042,4.34206960706137,
95.4754906100514));
#207236=CARTESIAN_POINT('Ctrl Pts',(-5.30412042747101,4.20595858477569,
95.4838409079737));
#207237=CARTESIAN_POINT('Ctrl Pts',(-5.41268951421426,4.06529558465423,
95.4921912058961));
#207238=CARTESIAN_POINT('Ctrl Pts',(-5.51559228467209,3.92052684588,95.5005415038184));
#207239=CARTESIAN_POINT('Ctrl Pts',(-5.61845546337996,3.77581380675001,
95.508888588971));
#207240=CARTESIAN_POINT('Ctrl Pts',(-5.71565647205855,3.62699845604368,
95.5172356741236));
#207241=CARTESIAN_POINT('Ctrl Pts',(-5.80686935428632,3.47455857660371,
95.5255827592762));
#207242=CARTESIAN_POINT('Ctrl Pts',(-5.8980635146385,3.32214998617016,95.5339281311501));
#207243=CARTESIAN_POINT('Ctrl Pts',(-5.9832718217372,3.16611864344385,95.542273503024));
#207244=CARTESIAN_POINT('Ctrl Pts',(-6.0622125463111,3.00696991061571,95.5506188748979));
#207245=CARTESIAN_POINT('Ctrl Pts',(-6.14114950608394,2.84782876782837,
95.5589638487685));
#207246=CARTESIAN_POINT('Ctrl Pts',(-6.21381932690151,2.68557083841541,
95.5673088226391));
#207247=CARTESIAN_POINT('Ctrl Pts',(-6.27998689226227,2.52072482294559,
95.5756537965098));
#207248=CARTESIAN_POINT('Ctrl Pts',(-6.34616172701123,2.35586069694572,
95.5839996871869));
#207249=CARTESIAN_POINT('Ctrl Pts',(-6.40583275540286,2.18840823654171,
95.592345577864));
#207250=CARTESIAN_POINT('Ctrl Pts',(-6.45881344340899,2.01891503120842,
95.6006914685412));
#207251=CARTESIAN_POINT('Ctrl Pts',(-6.5118302066246,1.84930641584334,95.6090430420391));
#207252=CARTESIAN_POINT('Ctrl Pts',(-6.55814742301891,1.67765460618518,
95.617394615537));
#207253=CARTESIAN_POINT('Ctrl Pts',(-6.59762851793987,1.50452216310249,
95.6257461890349));
#207254=CARTESIAN_POINT('Ctrl Pts',(-6.63712300236069,1.33133100440341,
95.6341005948603));
#207255=CARTESIAN_POINT('Ctrl Pts',(-6.669776674115,1.15665854709362,95.6424550006858));
#207256=CARTESIAN_POINT('Ctrl Pts',(-6.69550426880555,0.981076748479276,
95.6508094065112));
#207257=CARTESIAN_POINT('Ctrl Pts',(-6.72125887753533,0.805310588534168,
95.6591725844838));
#207258=CARTESIAN_POINT('Ctrl Pts',(-6.74007283333838,0.628633519789852,
95.6675357624564));
#207259=CARTESIAN_POINT('Ctrl Pts',(-6.75191274003437,0.451623018635648,
95.6758989404291));
#207260=CARTESIAN_POINT('Ctrl Pts',(-6.76195530203917,0.301483412050447,
95.6829925548893));
#207261=CARTESIAN_POINT('Ctrl Pts',(-6.76698136676099,0.151104096454122,
95.6900861693496));
#207262=CARTESIAN_POINT('Ctrl Pts',(-6.7669999482633,0.000836782275842868,
95.6971797838099));
#207263=CARTESIAN_POINT('',(-6.76699802674232,-0.00516779117013347,95.3028202162247));
#207264=CARTESIAN_POINT('Ctrl Pts',(3.09910619832125,6.01563211736945,94.6514100603466));
#207265=CARTESIAN_POINT('Ctrl Pts',(2.93949235646195,6.09786125588604,94.6598365869624));
#207266=CARTESIAN_POINT('Ctrl Pts',(2.77663313941226,6.17371884275999,94.6682631135781));
#207267=CARTESIAN_POINT('Ctrl Pts',(2.61106778260609,6.24296516365713,94.6766896401939));
#207268=CARTESIAN_POINT('Ctrl Pts',(2.44544509023424,6.3122354646734,94.6851190849302));
#207269=CARTESIAN_POINT('Ctrl Pts',(2.27711469535598,6.37488980680728,94.6935485296666));
#207270=CARTESIAN_POINT('Ctrl Pts',(2.10663459586528,6.4307371023471,94.7019779744029));
#207271=CARTESIAN_POINT('Ctrl Pts',(1.93599819608286,6.48663560004254,94.7104151474587));
#207272=CARTESIAN_POINT('Ctrl Pts',(1.76320846910119,6.53571447812687,94.7188523205145));
#207273=CARTESIAN_POINT('Ctrl Pts',(1.58883842969782,6.57783257952917,94.7272894935703));
#207274=CARTESIAN_POINT('Ctrl Pts',(1.41438029856451,6.61997195899293,94.7357309290852));
#207275=CARTESIAN_POINT('Ctrl Pts',(1.23834058661119,6.65514347807464,94.7441723646001));
#207276=CARTESIAN_POINT('Ctrl Pts',(1.06130178350248,6.68325725408909,94.7526138001151));
#207277=CARTESIAN_POINT('Ctrl Pts',(0.884070075688366,6.71140166338611,
94.761064433572));
#207278=CARTESIAN_POINT('Ctrl Pts',(0.705837430278023,6.7324729208087,94.7695150670289));
#207279=CARTESIAN_POINT('Ctrl Pts',(0.527191902262931,6.74643296106827,
94.7779657004857));
#207280=CARTESIAN_POINT('Ctrl Pts',(0.44884716015256,6.7525551168599,94.7816717137636));
#207281=CARTESIAN_POINT('Ctrl Pts',(0.370423027894518,6.75731028461828,
94.7853777270414));
#207282=CARTESIAN_POINT('Ctrl Pts',(0.291969074682313,6.76069841506254,
94.7890837403192));
#207283=CARTESIAN_POINT('Ctrl Pts',(0.115918856514544,6.76830136022299,
94.7974000127233));
#207284=CARTESIAN_POINT('Ctrl Pts',(-0.0605992048154732,6.76903077016871,
94.8057162851275));
#207285=CARTESIAN_POINT('Ctrl Pts',(-0.237015202430699,6.76284797949923,
94.8140325575316));
#207286=CARTESIAN_POINT('Ctrl Pts',(-0.413282040112049,6.75667041638654,
94.8223417985176));
#207287=CARTESIAN_POINT('Ctrl Pts',(-0.589446640035441,6.74359230872918,
94.8306510395036));
#207288=CARTESIAN_POINT('Ctrl Pts',(-0.764937249910979,6.72362699766269,
94.8389602804896));
#207289=CARTESIAN_POINT('Ctrl Pts',(-0.940311657841507,6.70367490672223,
94.8472640194721));
#207290=CARTESIAN_POINT('Ctrl Pts',(-1.11501262044503,6.67684473866661,
94.8555677584545));
#207291=CARTESIAN_POINT('Ctrl Pts',(-1.28847143884538,6.6432018147336,94.8638714974369));
#207292=CARTESIAN_POINT('Ctrl Pts',(-1.46184718956637,6.60957500205768,
94.8721712598425));
#207293=CARTESIAN_POINT('Ctrl Pts',(-1.63398164068556,6.56914200154682,
94.880471022248));
#207294=CARTESIAN_POINT('Ctrl Pts',(-1.80431402068705,6.52201961931671,
94.8887707846536));
#207295=CARTESIAN_POINT('Ctrl Pts',(-1.97459603563731,6.47491117055713,
94.8970680929282));
#207296=CARTESIAN_POINT('Ctrl Pts',(-2.14307670663951,6.42111737538106,
94.9053654012028));
#207297=CARTESIAN_POINT('Ctrl Pts',(-2.30920799371961,6.36080556547215,
94.9136627094774));
#207298=CARTESIAN_POINT('Ctrl Pts',(-2.47535606595535,6.3004876619301,94.9219608560746));
#207299=CARTESIAN_POINT('Ctrl Pts',(-2.63915395035085,6.23365053940582,
94.9302590026719));
#207300=CARTESIAN_POINT('Ctrl Pts',(-2.80007069077254,6.16051078455972,
94.9385571492691));
#207301=CARTESIAN_POINT('Ctrl Pts',(-2.96100361238503,6.08736367505105,
94.9468561302972));
#207302=CARTESIAN_POINT('Ctrl Pts',(-3.11905449539384,6.00791281353841,
94.9551551113253));
#207303=CARTESIAN_POINT('Ctrl Pts',(-3.27371431297307,5.92242210561146,
94.9634540923533));
#207304=CARTESIAN_POINT('Ctrl Pts',(-3.42841538528168,5.83690859346765,
94.9717552870929));
#207305=CARTESIAN_POINT('Ctrl Pts',(-3.57972328468885,5.74535219221408,
94.9800564818325));
#207306=CARTESIAN_POINT('Ctrl Pts',(-3.72715528268313,5.64806183560053,
94.988357676572));
#207307=CARTESIAN_POINT('Ctrl Pts',(-3.87465111183475,5.55072935681443,
94.9966624653405));
#207308=CARTESIAN_POINT('Ctrl Pts',(-4.01826740484435,5.44765816651817,
95.004967254109));
#207309=CARTESIAN_POINT('Ctrl Pts',(-4.15755185767649,5.33919952340524,
95.0132720428776));
#207310=CARTESIAN_POINT('Ctrl Pts',(-4.29700143097627,5.23061230354519,
95.0215866768986));
#207311=CARTESIAN_POINT('Ctrl Pts',(-4.43210862885219,5.11662508423684,
95.0299013109196));
#207312=CARTESIAN_POINT('Ctrl Pts',(-4.5624546914198,4.99762905673695,95.0382159449406));
#207313=CARTESIAN_POINT('Ctrl Pts',(-4.69288317295837,4.8785577869939,95.0465358363784));
#207314=CARTESIAN_POINT('Ctrl Pts',(-4.81854426821285,4.75447163723195,
95.0548557278162));
#207315=CARTESIAN_POINT('Ctrl Pts',(-4.93905725149254,4.62579749518707,
95.063175619254));
#207316=CARTESIAN_POINT('Ctrl Pts',(-5.05975044075847,4.49693094357734,
95.0715079516272));
#207317=CARTESIAN_POINT('Ctrl Pts',(-5.17527990584107,4.36346295197853,
95.0798402840004));
#207318=CARTESIAN_POINT('Ctrl Pts',(-5.285305403807,4.22585326158973,95.0881726163736));
#207319=CARTESIAN_POINT('Ctrl Pts',(-5.36814191307135,4.12224903708273,
95.094445901572));
#207320=CARTESIAN_POINT('Ctrl Pts',(-5.44785943194402,4.01629781736874,
95.1007191867703));
#207321=CARTESIAN_POINT('Ctrl Pts',(-5.52432948364893,3.9082058231479,95.1069924719686));
#207322=CARTESIAN_POINT('Ctrl Pts',(-5.62379197454233,3.76761354223343,
95.1151519613111));
#207323=CARTESIAN_POINT('Ctrl Pts',(-5.71806758277806,3.62296217473682,
95.1233114506537));
#207324=CARTESIAN_POINT('Ctrl Pts',(-5.80680017721763,3.47467418643322,
95.1314709399962));
#207325=CARTESIAN_POINT('Ctrl Pts',(-5.89508512257271,3.32713429957558,
95.1395892653454));
#207326=CARTESIAN_POINT('Ctrl Pts',(-5.97788261509272,3.17599468398584,
95.1477075906945));
#207327=CARTESIAN_POINT('Ctrl Pts',(-6.05488091884273,3.02170581934017,
95.1558259160436));
#207328=CARTESIAN_POINT('Ctrl Pts',(-6.13179484964074,2.86758602084709,
95.1639353455205));
#207329=CARTESIAN_POINT('Ctrl Pts',(-6.20292207562393,2.71032416579163,
95.1720447749973));
#207330=CARTESIAN_POINT('Ctrl Pts',(-6.26799429392437,2.55039928860787,
95.1801542044741));
#207331=CARTESIAN_POINT('Ctrl Pts',(-6.33300770738426,2.3906189332669,95.1882563055746));
#207332=CARTESIAN_POINT('Ctrl Pts',(-6.39197686717571,2.22818068358095,
95.1963584066751));
#207333=CARTESIAN_POINT('Ctrl Pts',(-6.44467957671181,2.06358768980473,
95.2044605077756));
#207334=CARTESIAN_POINT('Ctrl Pts',(-6.49799726017764,1.89707410406887,
95.2126571501435));
#207335=CARTESIAN_POINT('Ctrl Pts',(-6.54490113992903,1.72835550117301,
95.2208537925113));
#207336=CARTESIAN_POINT('Ctrl Pts',(-6.5852111044506,1.55797423272034,95.2290504348791));
#207337=CARTESIAN_POINT('Ctrl Pts',(-6.6250059872246,1.38977010043113,95.2371423403432));
#207338=CARTESIAN_POINT('Ctrl Pts',(-6.65837438342804,1.21994591049759,
95.2452342458073));
#207339=CARTESIAN_POINT('Ctrl Pts',(-6.68519307302459,1.04903888220792,
95.2533261512713));
#207340=CARTESIAN_POINT('Ctrl Pts',(-6.71253245083062,0.874813672609407,
95.261575162091));
#207341=CARTESIAN_POINT('Ctrl Pts',(-6.73306507342869,0.699463520814487,
95.2698241729108));
#207342=CARTESIAN_POINT('Ctrl Pts',(-6.74671515434204,0.523568167645297,
95.2780731837305));
#207343=CARTESIAN_POINT('Ctrl Pts',(-6.7603652352554,0.347672814475979,
95.2863221945502));
#207344=CARTESIAN_POINT('Ctrl Pts',(-6.7671327394428,0.171232663151217,
95.29457120537));
#207345=CARTESIAN_POINT('Ctrl Pts',(-6.76699802674289,-0.0051677904223947,
95.3028202161897));
#207346=CARTESIAN_POINT('Ctrl Pts',(-6.76699802674232,-0.0051677911699413,
95.3028202162247));
#207347=CARTESIAN_POINT('Ctrl Pts',(-6.76685125828067,-0.197354715467158,
95.3118074494536));
#207348=CARTESIAN_POINT('Ctrl Pts',(-6.75851323921425,-0.389205863367142,
95.3207946826824));
#207349=CARTESIAN_POINT('Ctrl Pts',(-6.74209344069607,-0.5800560636034,
95.3297819159113));
#207350=CARTESIAN_POINT('Ctrl Pts',(-6.72557542582627,-0.772047849733753,
95.338822907002));
#207351=CARTESIAN_POINT('Ctrl Pts',(-6.7008787490104,-0.963026460833392,
95.3478638980926));
#207352=CARTESIAN_POINT('Ctrl Pts',(-6.66816458479939,-1.15233244770216,
95.3569048891833));
#207353=CARTESIAN_POINT('Ctrl Pts',(-6.63534812016205,-1.34223041311084,
95.3659741523471));
#207354=CARTESIAN_POINT('Ctrl Pts',(-6.59446406922571,-1.53044507688767,
95.3750434155108));
#207355=CARTESIAN_POINT('Ctrl Pts',(-6.54572337338254,-1.71633170429073,
95.3841126786746));
#207356=CARTESIAN_POINT('Ctrl Pts',(-6.49676834367769,-1.90303575536812,
95.3932218233001));
#207357=CARTESIAN_POINT('Ctrl Pts',(-6.43988753964119,-2.08739105330672,
95.4023309679256));
#207358=CARTESIAN_POINT('Ctrl Pts',(-6.37534147991665,-2.26876839154069,
95.4114401125511));
#207359=CARTESIAN_POINT('Ctrl Pts',(-6.34354704243316,-2.35811219449339,
95.4159271429068));
#207360=CARTESIAN_POINT('Ctrl Pts',(-6.30989340892669,-2.44673381102486,
95.4204141732625));
#207361=CARTESIAN_POINT('Ctrl Pts',(-6.27441572084779,-2.53456038830763,
95.4249012036182));
#207362=CARTESIAN_POINT('Ctrl Pts',(-6.209349355766,-2.69563503693346,95.4331304533541));
#207363=CARTESIAN_POINT('Ctrl Pts',(-6.13798081565125,-2.85443922199044,
95.4413597030901));
#207364=CARTESIAN_POINT('Ctrl Pts',(-6.06048789807765,-3.0104443919884,
95.4495889528261));
#207365=CARTESIAN_POINT('Ctrl Pts',(-5.98308720968262,-3.1662638904549,
95.4578084084161));
#207366=CARTESIAN_POINT('Ctrl Pts',(-5.89957681572885,-3.31929068910676,
95.4660278640061));
#207367=CARTESIAN_POINT('Ctrl Pts',(-5.81018333724418,-3.46901406564027,
95.4742473195961));
#207368=CARTESIAN_POINT('Ctrl Pts',(-5.7208782991314,-3.61858931513673,
95.4824586433658));
#207369=CARTESIAN_POINT('Ctrl Pts',(-5.62570195016482,-3.76486734524126,
95.4906699671355));
#207370=CARTESIAN_POINT('Ctrl Pts',(-5.52492782207648,-3.90735992210153,
95.4988812909052));
#207371=CARTESIAN_POINT('Ctrl Pts',(-5.424233163062,-4.04974013130028,95.5070861393393));
#207372=CARTESIAN_POINT('Ctrl Pts',(-5.31794972337494,-4.18834054147748,
95.5152909877734));
#207373=CARTESIAN_POINT('Ctrl Pts',(-5.20639558216113,-4.32269985565192,
95.5234958362075));
#207374=CARTESIAN_POINT('Ctrl Pts',(-5.09490702204723,-4.45698018188821,
95.5316958611274));
#207375=CARTESIAN_POINT('Ctrl Pts',(-4.97815416155505,-4.58702410378795,
95.5398958860473));
#207376=CARTESIAN_POINT('Ctrl Pts',(-4.85649683670507,-4.71240145521088,
95.5480959109672));
#207377=CARTESIAN_POINT('Ctrl Pts',(-4.7348747222409,-4.83774251958805,
95.5562935626141));
#207378=CARTESIAN_POINT('Ctrl Pts',(-4.60835121740478,-4.95841944390518,
95.5644912142611));
#207379=CARTESIAN_POINT('Ctrl Pts',(-4.47732484351252,-5.07403697716774,
95.572688865908));
#207380=CARTESIAN_POINT('Ctrl Pts',(-4.34631601485576,-5.18963902853313,
95.5808854198391));
#207381=CARTESIAN_POINT('Ctrl Pts',(-4.21080578637142,-5.30018280022209,
95.5890819737701));
#207382=CARTESIAN_POINT('Ctrl Pts',(-4.07122776988145,-5.40531159562019,
95.5972785277012));
#207383=CARTESIAN_POINT('Ctrl Pts',(-3.93164306483399,-5.51044542877431,
95.6054754744099));
#207384=CARTESIAN_POINT('Ctrl Pts',(-3.7879904699832,-5.61016355278476,
95.6136724211186));
#207385=CARTESIAN_POINT('Ctrl Pts',(-3.64073477803065,-5.70415105655856,
95.6218693678273));
#207386=CARTESIAN_POINT('Ctrl Pts',(-3.49344525475554,-5.79816015353201,
95.6300681977471));
#207387=CARTESIAN_POINT('Ctrl Pts',(-3.34255128800087,-5.88643581505879,
95.6382670276668));
#207388=CARTESIAN_POINT('Ctrl Pts',(-3.1885446385984,-5.96870774017839,
95.6464658575866));
#207389=CARTESIAN_POINT('Ctrl Pts',(-3.03439212521109,-6.05105758732853,
95.6546724528464));
#207390=CARTESIAN_POINT('Ctrl Pts',(-2.87712135596695,-6.12739216809328,
95.6628790481062));
#207391=CARTESIAN_POINT('Ctrl Pts',(-2.71724741809939,-6.19748783531135,
95.671085643366));
#207392=CARTESIAN_POINT('Ctrl Pts',(-2.55729610032918,-6.26761742923429,
95.679296210665));
#207393=CARTESIAN_POINT('Ctrl Pts',(-2.39473943558964,-6.33150195796964,
95.6875067779639));
#207394=CARTESIAN_POINT('Ctrl Pts',(-2.23011017740507,-6.38896686457477,
95.6957173452629));
#207395=CARTESIAN_POINT('Ctrl Pts',(-2.06525387190525,-6.44651102351274,
95.7039392361096));
#207396=CARTESIAN_POINT('Ctrl Pts',(-1.89831960354303,-6.49761776133823,
95.7121611269563));
#207397=CARTESIAN_POINT('Ctrl Pts',(-1.72985408500851,-6.54216278034867,
95.720383017803));
#207398=CARTESIAN_POINT('Ctrl Pts',(-1.57667917061277,-6.58266471530269,
95.727858656958));
#207399=CARTESIAN_POINT('Ctrl Pts',(-1.42223869230681,-6.61774260765869,
95.7353342961129));
#207400=CARTESIAN_POINT('Ctrl Pts',(-1.26694830326736,-6.64734014451254,
95.7428099352679));
#207401=CARTESIAN_POINT('Ctrl Pts',(-1.08132322076399,-6.68271931546043,
95.7517458787186));
#207402=CARTESIAN_POINT('Ctrl Pts',(-0.894097159413995,-6.71034148187159,
95.7606818221693));
#207403=CARTESIAN_POINT('Ctrl Pts',(-0.705911292581039,-6.73008010702745,
95.7696177656201));
#207404=CARTESIAN_POINT('Ctrl Pts',(-0.518008319019261,-6.74978905979434,
95.7785402759777));
#207405=CARTESIAN_POINT('Ctrl Pts',(-0.329148675146541,-6.76163809135364,
95.7874627863354));
#207406=CARTESIAN_POINT('Ctrl Pts',(-0.13998152700382,-6.76555202271756,
95.796385296693));
#207407=CARTESIAN_POINT('Ctrl Pts',(0.0487221029221133,-6.76945636373504,
95.8052859441313));
#207408=CARTESIAN_POINT('Ctrl Pts',(0.237731475622388,-6.76546440491512,
95.8141865915697));
#207409=CARTESIAN_POINT('Ctrl Pts',(0.426395154337038,-6.75355285552411,
95.823087239008));
#207410=CARTESIAN_POINT('Ctrl Pts',(0.614767276621399,-6.74165971396255,
95.8319741315943));
#207411=CARTESIAN_POINT('Ctrl Pts',(0.802794514158681,-6.72187141111576,
95.8408610241805));
#207412=CARTESIAN_POINT('Ctrl Pts',(0.98982527887892,-6.69421652751779,
95.8497479167668));
#207413=CARTESIAN_POINT('Ctrl Pts',(1.17637530471704,-6.66663272729396,
95.8586119667217));
#207414=CARTESIAN_POINT('Ctrl Pts',(1.36193371398728,-6.63122273168152,
95.8674760166766));
#207415=CARTESIAN_POINT('Ctrl Pts',(1.54585465461591,-6.58806666532772,
95.8763400666316));
#207416=CARTESIAN_POINT('Ctrl Pts',(1.72169786927129,-6.54680599422853,
95.8848148114519));
#207417=CARTESIAN_POINT('Ctrl Pts',(1.89604409524305,-6.49846505228454,
95.8932895562722));
#207418=CARTESIAN_POINT('Ctrl Pts',(2.06833282201662,-6.44315825797945,
95.9017643010925));
#207419=CARTESIAN_POINT('Ctrl Pts',(2.23521730587638,-6.38958629192926,
95.9099732155216));
#207420=CARTESIAN_POINT('Ctrl Pts',(2.4000101777703,-6.32952933579917,95.9181821299508));
#207421=CARTESIAN_POINT('Ctrl Pts',(2.56218324479872,-6.26318657075396,
95.9263910443798));
#207422=CARTESIAN_POINT('Ctrl Pts',(2.72439486764991,-6.19682803305341,
95.9346019104366));
#207423=CARTESIAN_POINT('Ctrl Pts',(2.88398511517514,-6.12418084396062,
95.9428127764934));
#207424=CARTESIAN_POINT('Ctrl Pts',(3.04044665877479,-6.04549196634527,
95.9510236425502));
#207425=CARTESIAN_POINT('Ctrl Pts',(3.19697329023779,-5.96677035422664,
95.95923792432));
#207426=CARTESIAN_POINT('Ctrl Pts',(3.35036830698329,-5.88200220634624,
95.9674522060898));
#207427=CARTESIAN_POINT('Ctrl Pts',(3.50014974885115,-5.79148001253714,
95.9756664878596));
#207428=CARTESIAN_POINT('Ctrl Pts',(3.65009978155624,-5.7008559288527,95.983890015452));
#207429=CARTESIAN_POINT('Ctrl Pts',(3.79642781065042,-5.60446504751834,
95.9921135430443));
#207430=CARTESIAN_POINT('Ctrl Pts',(3.93868078967053,-5.5026432409416,96.0003370706367));
#207431=CARTESIAN_POINT('Ctrl Pts',(4.08102494731668,-5.40075617054764,
96.0085658691904));
#207432=CARTESIAN_POINT('Ctrl Pts',(4.21928856757974,-5.29343145350961,
96.0167946677441));
#207433=CARTESIAN_POINT('Ctrl Pts',(4.35305243512652,-5.18104463376249,
96.0250234662978));
#207434=CARTESIAN_POINT('Ctrl Pts',(4.48700041793267,-5.06850312255162,
96.0332635911342));
#207435=CARTESIAN_POINT('Ctrl Pts',(4.61643601421664,-4.95088583029674,
96.0415037159706));
#207436=CARTESIAN_POINT('Ctrl Pts',(4.74097682691424,-4.82860515331936,
96.049743840807));
#207437=CARTESIAN_POINT('Ctrl Pts',(4.79626780814425,-4.77431757907679,
96.0534021161771));
#207438=CARTESIAN_POINT('Ctrl Pts',(4.85059456019711,-4.71911129556049,
96.0570603915472));
#207439=CARTESIAN_POINT('Ctrl Pts',(4.90392623067133,-4.66302439669081,
96.0607186669173));
#207440=CARTESIAN_POINT('Ctrl Pts',(5.02708458277735,-4.53350342016588,
96.0691666896798));
#207441=CARTESIAN_POINT('Ctrl Pts',(5.14521543230861,-4.39898777269238,
96.0776147124423));
#207442=CARTESIAN_POINT('Ctrl Pts',(5.25790700161998,-4.25989471258571,
96.0860627352049));
#207443=CARTESIAN_POINT('Ctrl Pts',(5.3704953758957,-4.1209290241483,96.0945030218607));
#207444=CARTESIAN_POINT('Ctrl Pts',(5.47765418944091,-3.97739453621532,
96.1029433085164));
#207445=CARTESIAN_POINT('Ctrl Pts',(5.57900989112737,-3.8297438079724,96.1113835951722));
#207446=CARTESIAN_POINT('Ctrl Pts',(5.68028838151141,-3.68220555791119,
96.1198174521401));
#207447=CARTESIAN_POINT('Ctrl Pts',(5.7757723846831,-3.53055759254873,96.128251309108));
#207448=CARTESIAN_POINT('Ctrl Pts',(5.86512964378643,-3.37528417493664,
96.1366851660759));
#207449=CARTESIAN_POINT('Ctrl Pts',(5.95443256903717,-3.22010517162359,
96.145113894821));
#207450=CARTESIAN_POINT('Ctrl Pts',(6.0376160116873,-3.06130539951905,96.153542623566));
#207451=CARTESIAN_POINT('Ctrl Pts',(6.11439173269742,-2.89939696128721,
96.161971352311));
#207452=CARTESIAN_POINT('Ctrl Pts',(6.19113255998483,-2.73756210866385,
96.1703962502913));
#207453=CARTESIAN_POINT('Ctrl Pts',(6.26147133000044,-2.57262170799719,
96.1788211482716));
#207454=CARTESIAN_POINT('Ctrl Pts',(6.32516617778657,-2.40511160310386,
96.1872460462519));
#207455=CARTESIAN_POINT('Ctrl Pts',(6.38884692342967,-2.23763858522056,
96.1956690789461));
#207456=CARTESIAN_POINT('Ctrl Pts',(6.44588655879162,-2.06759730796299,
96.2040921116403));
#207457=CARTESIAN_POINT('Ctrl Pts',(6.49609151775605,-1.89554319205286,
96.2125151443344));
#207458=CARTESIAN_POINT('Ctrl Pts',(6.54629079608638,-1.72350854387056,
96.220937223972));
#207459=CARTESIAN_POINT('Ctrl Pts',(6.58965684630891,-1.5494618311258,96.2293593036096));
#207460=CARTESIAN_POINT('Ctrl Pts',(6.62604601267164,-1.37397352156373,
96.2377813832472));
#207461=CARTESIAN_POINT('Ctrl Pts',(6.66243614129735,-1.19848057144738,
96.2462036855955));
#207462=CARTESIAN_POINT('Ctrl Pts',(6.69184895089623,-1.0215462751138,96.2546259879437));
#207463=CARTESIAN_POINT('Ctrl Pts',(6.71419186056453,-0.843751538978782,
96.263048290292));
#207464=CARTESIAN_POINT('Ctrl Pts',(6.73653848014587,-0.665927281039336,
96.2714719911156));
#207465=CARTESIAN_POINT('Ctrl Pts',(6.75181281838071,-0.48724262935804,
96.2798956919392));
#207466=CARTESIAN_POINT('Ctrl Pts',(6.75997409994863,-0.308284232525387,
96.2883193927629));
#207467=CARTESIAN_POINT('Ctrl Pts',(6.76814090433038,-0.129204732909792,
96.2967487939819));
#207468=CARTESIAN_POINT('Ctrl Pts',(6.76918501836201,0.0501485485583775,
96.3051781952008));
#207469=CARTESIAN_POINT('Ctrl Pts',(6.76311778520249,0.229187310900414,
96.3136075964198));
#207470=CARTESIAN_POINT('Ctrl Pts',(6.75704838726261,0.408289954024154,
96.3220400052374));
#207471=CARTESIAN_POINT('Ctrl Pts',(6.74386260028697,0.587077521215506,
96.3304724140551));
#207472=CARTESIAN_POINT('Ctrl Pts',(6.72362376949708,0.764965624230176,
96.3389048228727));
#207473=CARTESIAN_POINT('Ctrl Pts',(6.70336621315207,0.943018314493633,
96.3473450336003));
#207474=CARTESIAN_POINT('Ctrl Pts',(6.67604261856037,1.12016954705363,96.355785244328));
#207475=CARTESIAN_POINT('Ctrl Pts',(6.64176786520474,1.29584282408544,96.3642254550556));
#207476=CARTESIAN_POINT('Ctrl Pts',(6.6222729703647,1.3957627863505,96.3690261028927));
#207477=CARTESIAN_POINT('Ctrl Pts',(6.60053021063109,1.4952048100933,96.3738267507297));
#207478=CARTESIAN_POINT('Ctrl Pts',(6.57656798188469,1.59406479782006,96.3786273985668));
#207479=CARTESIAN_POINT('Ctrl Pts',(6.53593894177013,1.76168636798307,96.3867671135996));
#207480=CARTESIAN_POINT('Ctrl Pts',(6.48884530541958,1.9279680304558,96.3949068286325));
#207481=CARTESIAN_POINT('Ctrl Pts',(6.43539258761967,2.09236976732359,96.4030465436654));
#207482=CARTESIAN_POINT('Ctrl Pts',(6.38198661924602,2.25662771941878,96.4111791397523));
#207483=CARTESIAN_POINT('Ctrl Pts',(6.32223275223909,2.41900867274407,96.4193117358393));
#207484=CARTESIAN_POINT('Ctrl Pts',(6.25628725600429,2.57898405779454,96.4274443319262));
#207485=CARTESIAN_POINT('Ctrl Pts',(6.19038684364855,2.73885007508943,96.4355713681342));
#207486=CARTESIAN_POINT('Ctrl Pts',(6.11830336860602,2.89631346119327,96.4436984043421));
#207487=CARTESIAN_POINT('Ctrl Pts',(6.04024250595037,3.05086208624881,96.4518254405501));
#207488=CARTESIAN_POINT('Ctrl Pts',(5.96221895779985,3.20533683426447,96.4599485918876));
#207489=CARTESIAN_POINT('Ctrl Pts',(5.87822387660907,3.356899269582,96.4680717432252));
#207490=CARTESIAN_POINT('Ctrl Pts',(5.78851050328361,3.50505850926563,96.4761948945628));
#207491=CARTESIAN_POINT('Ctrl Pts',(5.69882234008279,3.6531761151018,96.4843157632344));
#207492=CARTESIAN_POINT('Ctrl Pts',(5.60341927553491,3.79789211753768,96.4924366319061));
#207493=CARTESIAN_POINT('Ctrl Pts',(5.50259979239729,3.93874148995708,96.5005575005777));
#207494=CARTESIAN_POINT('Ctrl Pts',(5.40177486058888,4.0795984744157,96.5086788081322));
#207495=CARTESIAN_POINT('Ctrl Pts',(5.29553313531284,4.2165881112698,96.5168001156867));
#207496=CARTESIAN_POINT('Ctrl Pts',(5.18421570530295,4.34927540182157,96.5249214232412));
#207497=CARTESIAN_POINT('Ctrl Pts',(5.12637129907314,4.41822433044424,96.529141536958));
#207498=CARTESIAN_POINT('Ctrl Pts',(5.06715702965564,4.48601206089266,96.5333616506747));
#207499=CARTESIAN_POINT('Ctrl Pts',(5.0066249862165,4.55258116318563,96.5375817643915));
#207500=CARTESIAN_POINT('Ctrl Pts',(4.87781571041155,4.69423700974505,96.5465619633206));
#207501=CARTESIAN_POINT('Ctrl Pts',(4.74310104553792,4.83030255785421,96.5555421622498));
#207502=CARTESIAN_POINT('Ctrl Pts',(4.60297897068858,4.9603299885591,96.5645223611789));
#207503=CARTESIAN_POINT('Ctrl Pts',(4.46249551332879,5.09069276713395,96.5735257205332));
#207504=CARTESIAN_POINT('Ctrl Pts',(4.31657691694639,5.21498610547453,96.5825290798875));
#207505=CARTESIAN_POINT('Ctrl Pts',(4.16575584732585,5.33280106702571,96.5915324392419));
#207506=CARTESIAN_POINT('Ctrl Pts',(4.01474440479513,5.4507647397427,96.6005471630278));
#207507=CARTESIAN_POINT('Ctrl Pts',(3.85881831625122,5.5622335545351,96.6095618868136));
#207508=CARTESIAN_POINT('Ctrl Pts',(3.69854003538396,5.66684132534713,96.6185766105995));
#207509=CARTESIAN_POINT('Ctrl Pts',(3.53801115510602,5.77161265322739,96.6276054291489));
#207510=CARTESIAN_POINT('Ctrl Pts',(3.37311667741377,5.86950135883824,96.6366342476984));
#207511=CARTESIAN_POINT('Ctrl Pts',(3.20444633434113,5.96018562549253,96.6456630662478));
#207512=CARTESIAN_POINT('Ctrl Pts',(3.16949323645566,5.9789778802025,96.6475340838363));
#207513=CARTESIAN_POINT('Ctrl Pts',(3.13437806885556,5.99746091433267,96.6494051014248));
#207514=CARTESIAN_POINT('Ctrl Pts',(3.09910619832137,6.01563211736939,96.6512761190133));
#207515=CARTESIAN_POINT('Origin',(0.,0.,4.30282021618968));
#207516=CARTESIAN_POINT('',(3.09910619832142,6.01563211736936,99.0457552630242));
#207517=CARTESIAN_POINT('',(3.09910619832134,6.0156321173694,98.651562053011));
#207518=CARTESIAN_POINT('',(3.09910619832133,6.0156321173694,4.30282021618968));
#207519=CARTESIAN_POINT('',(-6.767,8.45744073366125E-10,97.6971797837703));
#207520=CARTESIAN_POINT('Ctrl Pts',(-6.767,4.49310309984705E-12,97.6971797838099));
#207521=CARTESIAN_POINT('Ctrl Pts',(-6.76700000000012,-0.186007249522473,
97.7059292956211));
#207522=CARTESIAN_POINT('Ctrl Pts',(-6.75932637294544,-0.372014355745619,
97.7146788074323));
#207523=CARTESIAN_POINT('Ctrl Pts',(-6.74400518264215,-0.557389537483297,
97.7234283192435));
#207524=CARTESIAN_POINT('Ctrl Pts',(-6.7286840570513,-0.742763936247776,
97.7321777940991));
#207525=CARTESIAN_POINT('Ctrl Pts',(-6.70571545645778,-0.927506130238429,
97.7409272689548));
#207526=CARTESIAN_POINT('Ctrl Pts',(-6.67517739404862,-1.11098863989795,
97.7496767438105));
#207527=CARTESIAN_POINT('Ctrl Pts',(-6.64463945808741,-1.29447038981747,
97.7584261824375));
#207528=CARTESIAN_POINT('Ctrl Pts',(-6.60653217008395,-1.47669218313505,
97.7671756210645));
#207529=CARTESIAN_POINT('Ctrl Pts',(-6.56098496092717,-1.65703510599129,
97.7759250596916));
#207530=CARTESIAN_POINT('Ctrl Pts',(-6.51543793658342,-1.83737729708539,
97.7846744628167));
#207531=CARTESIAN_POINT('Ctrl Pts',(-6.46245112167471,-2.01584035510763,
97.7934238659419));
#207532=CARTESIAN_POINT('Ctrl Pts',(-6.4022044837431,-2.19181813760625,
97.8021732690671));
#207533=CARTESIAN_POINT('Ctrl Pts',(-6.34195808526559,-2.36779522066997,
97.8109226374172));
#207534=CARTESIAN_POINT('Ctrl Pts',(-6.27445201433156,-2.54128677684038,
97.8196720057673));
#207535=CARTESIAN_POINT('Ctrl Pts',(-6.19991555071949,-2.71170355384703,
97.8284213741174));
#207536=CARTESIAN_POINT('Ctrl Pts',(-6.12537937716739,-2.88211966767378,
97.8371707084192));
#207537=CARTESIAN_POINT('Ctrl Pts',(-6.04381298052565,-3.04946076371696,
97.8459200427209));
#207538=CARTESIAN_POINT('Ctrl Pts',(-5.95549339335875,-3.21315848374467,
97.8546693770227));
#207539=CARTESIAN_POINT('Ctrl Pts',(-5.86717414255452,-3.37685558033418,
97.8634186780029));
#207540=CARTESIAN_POINT('Ctrl Pts',(-5.7721018887664,-3.53690907646688,
97.8721679789831));
#207541=CARTESIAN_POINT('Ctrl Pts',(-5.67059953347036,-3.69277536969225,
97.8809172799633));
#207542=CARTESIAN_POINT('Ctrl Pts',(-5.56909755631428,-3.8486410822486,
97.8896665483486));
#207543=CARTESIAN_POINT('Ctrl Pts',(-5.46116568196897,-4.00031938297452,
97.8984158167339));
#207544=CARTESIAN_POINT('Ctrl Pts',(-5.34717048533654,-4.14729511859788,
97.9071650851191));
#207545=CARTESIAN_POINT('Ctrl Pts',(-5.23317570391888,-4.29427031887854,
97.9159143216362));
#207546=CARTESIAN_POINT('Ctrl Pts',(-5.11311782003565,-4.43654276189488,
97.9246635581532));
#207547=CARTESIAN_POINT('Ctrl Pts',(-4.98740458984804,-4.57362924351797,
97.9334127946703));
#207548=CARTESIAN_POINT('Ctrl Pts',(-4.86169180711819,-4.71071523720187,
97.9421620000457));
#207549=CARTESIAN_POINT('Ctrl Pts',(-4.73032391204274,-4.84261509523136,
97.9509112054211));
#207550=CARTESIAN_POINT('Ctrl Pts',(-4.5937470701373,-4.96888084538208,
97.9596604107965));
#207551=CARTESIAN_POINT('Ctrl Pts',(-4.45717070301595,-5.09514615659332,
97.968409585757));
#207552=CARTESIAN_POINT('Ctrl Pts',(-4.3153856357121,-5.21577720459387,
97.9771587607174));
#207553=CARTESIAN_POINT('Ctrl Pts',(-4.16887341029699,-5.33036429232738,
97.9859079356779));
#207554=CARTESIAN_POINT('Ctrl Pts',(-4.02236168203894,-5.44495099123477,
97.9946570809499));
#207555=CARTESIAN_POINT('Ctrl Pts',(-3.8711230534835,-5.55349359438473,
98.0034062262219));
#207556=CARTESIAN_POINT('Ctrl Pts',(-3.71567117017942,-5.65562346298775,
98.0121553714939));
#207557=CARTESIAN_POINT('Ctrl Pts',(-3.56021980145993,-5.75775299351537,
98.0209044878041));
#207558=CARTESIAN_POINT('Ctrl Pts',(-3.40055544538517,-5.85346967463776,
98.0296536041143));
#207559=CARTESIAN_POINT('Ctrl Pts',(-3.23722035987013,-5.94244842986814,
98.0384027204244));
#207560=CARTESIAN_POINT('Ctrl Pts',(-3.07388580147316,-6.03142689794461,
98.0471518084993));
#207561=CARTESIAN_POINT('Ctrl Pts',(-2.90688078896689,-6.1136673465673,
98.0559008965742));
#207562=CARTESIAN_POINT('Ctrl Pts',(-2.73677250721455,-6.18889046952316,
98.064649984649));
#207563=CARTESIAN_POINT('Ctrl Pts',(-2.56666476031572,-6.2641133559629,
98.0733990452151));
#207564=CARTESIAN_POINT('Ctrl Pts',(-2.3934540257526,-6.3323188450052,98.0821481057811));
#207565=CARTESIAN_POINT('Ctrl Pts',(-2.21772856065691,-6.39327529762692,
98.0908971663471));
#207566=CARTESIAN_POINT('Ctrl Pts',(-2.042003633486,-6.45423156365084,98.0996462001308));
#207567=CARTESIAN_POINT('Ctrl Pts',(-1.86376426189351,-6.50793874375638,
98.1083952339145));
#207568=CARTESIAN_POINT('Ctrl Pts',(-1.68361577753213,-6.55421443909527,
98.1171442676982));
#207569=CARTESIAN_POINT('Ctrl Pts',(-1.50346782967874,-6.60048999661851,
98.125893275426));
#207570=CARTESIAN_POINT('Ctrl Pts',(-1.32141105795077,-6.63933404237694,
98.1346422831538));
#207571=CARTESIAN_POINT('Ctrl Pts',(-1.13806375487129,-6.67061465607543,
98.1433912908817));
#207572=CARTESIAN_POINT('Ctrl Pts',(-0.954716982604495,-6.70189517921274,
98.15214027328));
#207573=CARTESIAN_POINT('Ctrl Pts',(-0.770079968904035,-6.72561226592205,
98.1608892556784));
#207574=CARTESIAN_POINT('Ctrl Pts',(-0.584779765560561,-6.74168536983082,
98.1696382380768));
#207575=CARTESIAN_POINT('Ctrl Pts',(-0.391489830653644,-6.75845151013839,
98.1787644570867));
#207576=CARTESIAN_POINT('Ctrl Pts',(-0.197478578240707,-6.76689983031618,
98.1878906760965));
#207577=CARTESIAN_POINT('Ctrl Pts',(-0.00346287645373946,-6.76699911397118,
98.1970168951064));
#207578=CARTESIAN_POINT('Ctrl Pts',(0.184489834652353,-6.76709529501195,
98.2058579197722));
#207579=CARTESIAN_POINT('Ctrl Pts',(0.372446404247802,-6.75935639738177,
98.214698944438));
#207580=CARTESIAN_POINT('Ctrl Pts',(0.559755019486738,-6.743809258732,98.2235399691039));
#207581=CARTESIAN_POINT('Ctrl Pts',(0.745134705520139,-6.72842222659824,
98.2322899477136));
#207582=CARTESIAN_POINT('Ctrl Pts',(0.929879431226895,-6.70538706057547,
98.2410399263233));
#207583=CARTESIAN_POINT('Ctrl Pts',(1.11336163626655,-6.67478200894156,
98.2497899049331));
#207584=CARTESIAN_POINT('Ctrl Pts',(1.29684196300553,-6.64417727061045,
98.2585397939696));
#207585=CARTESIAN_POINT('Ctrl Pts',(1.4790595121735,-6.60600284890626,98.2672896830061));
#207586=CARTESIAN_POINT('Ctrl Pts',(1.65939532066929,-6.5603884160727,98.2760395720426));
#207587=CARTESIAN_POINT('Ctrl Pts',(1.83972934300659,-6.51477443503297,
98.2847893744148));
#207588=CARTESIAN_POINT('Ctrl Pts',(2.01818138406136,-6.46172066062182,
98.293539176787));
#207589=CARTESIAN_POINT('Ctrl Pts',(2.19414528354083,-6.40140730423518,
98.3022889791591));
#207590=CARTESIAN_POINT('Ctrl Pts',(2.37010749863872,-6.3410945251869,98.3110386977754));
#207591=CARTESIAN_POINT('Ctrl Pts',(2.54358134866321,-6.2735223961656,98.3197884163918));
#207592=CARTESIAN_POINT('Ctrl Pts',(2.71397759435406,-6.19892043966884,
98.3285381350081));
#207593=CARTESIAN_POINT('Ctrl Pts',(2.8843722655797,-6.12431917249587,98.3372877727768));
#207594=CARTESIAN_POINT('Ctrl Pts',(3.05168912680798,-6.04268832278878,
98.3460374105455));
#207595=CARTESIAN_POINT('Ctrl Pts',(3.21535986273693,-5.95430516123421,
98.3547870483142));
#207596=CARTESIAN_POINT('Ctrl Pts',(3.37902914072688,-5.86592278697529,
98.3635366081433));
#207597=CARTESIAN_POINT('Ctrl Pts',(3.53905210621426,-5.77078835742031,
98.3722861679723));
#207598=CARTESIAN_POINT('Ctrl Pts',(3.69488522831559,-5.66922500431719,
98.3810357278014));
#207599=CARTESIAN_POINT('Ctrl Pts',(3.8507170140682,-5.56766252217177,98.3897852125985));
#207600=CARTESIAN_POINT('Ctrl Pts',(4.00235878822301,-5.45967138329446,
98.3985346973956));
#207601=CARTESIAN_POINT('Ctrl Pts',(4.14929549611238,-5.34561838199675,
98.4072841821928));
#207602=CARTESIAN_POINT('Ctrl Pts',(4.29623099276,-5.23156632087089,98.4160335948654));
#207603=CARTESIAN_POINT('Ctrl Pts',(4.43846127435936,-5.11145267305044,
98.4247830075379));
#207604=CARTESIAN_POINT('Ctrl Pts',(4.57550326054348,-4.98568540049972,
98.4335324202105));
#207605=CARTESIAN_POINT('Ctrl Pts',(4.71254416257686,-4.85991912290452,
98.4422817636658));
#207606=CARTESIAN_POINT('Ctrl Pts',(4.84439664018666,-4.72849950385516,
98.451031107121));
#207607=CARTESIAN_POINT('Ctrl Pts',(4.9706128679465,-4.59187289861171,98.4597804505763));
#207608=CARTESIAN_POINT('Ctrl Pts',(5.09682813912586,-4.45524732884798,
98.4685297277211));
#207609=CARTESIAN_POINT('Ctrl Pts',(5.21740705147737,-4.3134150623591,98.4772790048659));
#207610=CARTESIAN_POINT('Ctrl Pts',(5.33194007545592,-4.16685781275856,
98.4860282820107));
#207611=CARTESIAN_POINT('Ctrl Pts',(5.44647226944372,-4.02030162521994,
98.4947774957519));
#207612=CARTESIAN_POINT('Ctrl Pts',(5.55495848627992,-3.86902074888107,
98.5035267094929));
#207613=CARTESIAN_POINT('Ctrl Pts',(5.6570302729166,-3.71352898080857,98.5122759232341));
#207614=CARTESIAN_POINT('Ctrl Pts',(5.75910135376881,-3.55803828789777,
98.5210250764779));
#207615=CARTESIAN_POINT('Ctrl Pts',(5.85475793592646,-3.39833700106895,
98.5297742297219));
#207616=CARTESIAN_POINT('Ctrl Pts',(5.94367514427302,-3.2349675082373,98.5385233829657));
#207617=CARTESIAN_POINT('Ctrl Pts',(6.03259176732553,-3.07159909077896,
98.5472724786187));
#207618=CARTESIAN_POINT('Ctrl Pts',(6.11476896835846,-2.90456276731599,
98.5560215742716));
#207619=CARTESIAN_POINT('Ctrl Pts',(6.18992765547817,-2.73442583003208,
98.5647706699245));
#207620=CARTESIAN_POINT('Ctrl Pts',(6.26508587282987,-2.56428995616335,
98.5735197108925));
#207621=CARTESIAN_POINT('Ctrl Pts',(6.33322554827095,-2.39105376935373,
98.5822687518606));
#207622=CARTESIAN_POINT('Ctrl Pts',(6.39411526732969,-2.21530561054258,
98.5910177928286));
#207623=CARTESIAN_POINT('Ctrl Pts',(6.45500462602788,-2.03955849185287,
98.5997667820176));
#207624=CARTESIAN_POINT('Ctrl Pts',(6.50864402040683,-1.86129970164743,
98.6085157712066));
#207625=CARTESIAN_POINT('Ctrl Pts',(6.55485128368548,-1.68113463136267,
98.6172647603957));
#207626=CARTESIAN_POINT('Ctrl Pts',(6.60199809554277,-1.49730620117087,
98.6261916458671));
#207627=CARTESIAN_POINT('Ctrl Pts',(6.64140720707828,-1.31149343245927,
98.6351185313385));
#207628=CARTESIAN_POINT('Ctrl Pts',(6.67293928722843,-1.12435326697764,
98.64404541681));
#207629=CARTESIAN_POINT('Ctrl Pts',(6.70384625876223,-0.940923067009009,
98.6527953309874));
#207630=CARTESIAN_POINT('Ctrl Pts',(6.72718554579768,-0.756217899524115,
98.6615452451649));
#207631=CARTESIAN_POINT('Ctrl Pts',(6.74287786815307,-0.570865181256975,
98.6702951593424));
#207632=CARTESIAN_POINT('Ctrl Pts',(6.75856988190831,-0.385516108076499,
98.6790449014469));
#207633=CARTESIAN_POINT('Ctrl Pts',(6.76661520773395,-0.199519795228973,
98.6877946435513));
#207634=CARTESIAN_POINT('Ctrl Pts',(6.76698651789578,-0.0135080204583415,
98.6965443856558));
#207635=CARTESIAN_POINT('Ctrl Pts',(6.7673578212491,0.172500343510199,98.7052939673208));
#207636=CARTESIAN_POINT('Ctrl Pts',(6.76005538995198,0.358523882208095,
98.7140435489857));
#207637=CARTESIAN_POINT('Ctrl Pts',(6.74510402742384,0.543930748561488,
98.7227931306507));
#207638=CARTESIAN_POINT('Ctrl Pts',(6.73015291918062,0.729334461612352,
98.7315425635074));
#207639=CARTESIAN_POINT('Ctrl Pts',(6.70755316306634,0.914121237631807,
98.7402919963641));
#207640=CARTESIAN_POINT('Ctrl Pts',(6.67738151874621,1.09766345165836,98.7490414292208));
#207641=CARTESIAN_POINT('Ctrl Pts',(6.64721034747624,1.2812027879938,98.7577907248983));
#207642=CARTESIAN_POINT('Ctrl Pts',(6.60946757205204,1.46349731860046,98.7665400205758));
#207643=CARTESIAN_POINT('Ctrl Pts',(6.56428138111593,1.64392790277881,98.7752893162533));
#207644=CARTESIAN_POINT('Ctrl Pts',(6.51909583859929,1.82435589778774,98.7840384863789));
#207645=CARTESIAN_POINT('Ctrl Pts',(6.46646716392963,2.00291972191981,98.7927876565045));
#207646=CARTESIAN_POINT('Ctrl Pts',(6.4065740987298,2.17901292274379,98.8015368266301));
#207647=CARTESIAN_POINT('Ctrl Pts',(6.34668181342182,2.35510383058693,98.8102858828292));
#207648=CARTESIAN_POINT('Ctrl Pts',(6.27952541914164,2.52872390822297,98.8190349390284));
#207649=CARTESIAN_POINT('Ctrl Pts',(6.20533299175639,2.69928350890004,98.8277839952275));
#207650=CARTESIAN_POINT('Ctrl Pts',(6.12831602991675,2.87633637965355,98.8368661313857));
#207651=CARTESIAN_POINT('Ctrl Pts',(6.04371690605399,3.05009086601207,98.8459482675438));
#207652=CARTESIAN_POINT('Ctrl Pts',(5.95184520316762,3.21991112882492,98.855030403702));
#207653=CARTESIAN_POINT('Ctrl Pts',(5.86333549509411,3.38351691182781,98.8637801840456));
#207654=CARTESIAN_POINT('Ctrl Pts',(5.76807618099509,3.54347103711775,98.8725299643892));
#207655=CARTESIAN_POINT('Ctrl Pts',(5.66639083309161,3.69923018027473,98.8812797447328));
#207656=CARTESIAN_POINT('Ctrl Pts',(5.56470914082355,3.85498372381826,98.8900292105177));
#207657=CARTESIAN_POINT('Ctrl Pts',(5.45660203372232,4.00654234701773,98.8987786763026));
#207658=CARTESIAN_POINT('Ctrl Pts',(5.34243669839392,4.15339127986444,98.9075281420875));
#207659=CARTESIAN_POINT('Ctrl Pts',(5.22827486050767,4.30023571401066,98.9162773398335));
#207660=CARTESIAN_POINT('Ctrl Pts',(5.10805534167286,4.44237052028269,98.9250265375795));
#207661=CARTESIAN_POINT('Ctrl Pts',(4.98218644340125,4.57931296628531,98.9337757353255));
#207662=CARTESIAN_POINT('Ctrl Pts',(4.85632073219772,4.71625194483169,98.9425247115372));
#207663=CARTESIAN_POINT('Ctrl Pts',(4.72480612170516,4.84799861524316,98.9512736877488));
#207664=CARTESIAN_POINT('Ctrl Pts',(4.5880892523552,4.97410554898292,98.9600226639604));
#207665=CARTESIAN_POINT('Ctrl Pts',(4.45136349474265,5.10022068121017,98.9687722089621));
#207666=CARTESIAN_POINT('Ctrl Pts',(4.30943501210306,5.22069514871648,98.9775217539638));
#207667=CARTESIAN_POINT('Ctrl Pts',(4.16278587432015,5.33511975166074,98.9862712989655));
#207668=CARTESIAN_POINT('Ctrl Pts',(4.01614535740691,5.44953762807663,98.9950203296193));
#207669=CARTESIAN_POINT('Ctrl Pts',(3.86478496658177,5.55790617532607,99.003769360273));
#207670=CARTESIAN_POINT('Ctrl Pts',(3.70921874747459,5.65985735539183,99.0125183909267));
#207671=CARTESIAN_POINT('Ctrl Pts',(3.55365041606173,5.76180991976878,99.0212675403763));
#207672=CARTESIAN_POINT('Ctrl Pts',(3.39387638174804,5.8573447855265,99.0300166898259));
#207673=CARTESIAN_POINT('Ctrl Pts',(3.23043927904829,5.94613749121074,99.0387658392756));
#207674=CARTESIAN_POINT('Ctrl Pts',(3.18691767070626,5.96978206944044,99.0410956471918));
#207675=CARTESIAN_POINT('Ctrl Pts',(3.14313645919731,5.99294880633374,99.043425455108));
#207676=CARTESIAN_POINT('Ctrl Pts',(3.09910619832142,6.01563211736936,99.0457552630242));
#207677=CARTESIAN_POINT('Ctrl Pts',(3.09910619832136,6.01563211736939,97.0457552630242));
#207678=CARTESIAN_POINT('Ctrl Pts',(2.93375330764826,6.10081787314653,97.0545047109265));
#207679=CARTESIAN_POINT('Ctrl Pts',(2.76488627843067,6.17918207037041,97.0632541588288));
#207680=CARTESIAN_POINT('Ctrl Pts',(2.59307866646696,6.25045854554,97.0720036067311));
#207681=CARTESIAN_POINT('Ctrl Pts',(2.42127244185374,6.32173444515038,97.0807529839814));
#207682=CARTESIAN_POINT('Ctrl Pts',(2.24652594672466,6.38592262741837,97.0895023612317));
#207683=CARTESIAN_POINT('Ctrl Pts',(2.06943269687126,6.4428050811056,97.098251738482));
#207684=CARTESIAN_POINT('Ctrl Pts',(1.89234081822068,6.49968709436169,97.1070010479874));
#207685=CARTESIAN_POINT('Ctrl Pts',(1.71290249405564,6.54926340459551,97.1157503574927));
#207686=CARTESIAN_POINT('Ctrl Pts',(1.53172716625019,6.59136563150393,97.1244996669981));
#207687=CARTESIAN_POINT('Ctrl Pts',(1.35055318107296,6.63346754640718,97.1332489116653));
#207688=CARTESIAN_POINT('Ctrl Pts',(1.16764249714383,6.66809542395782,97.1419981563326));
#207689=CARTESIAN_POINT('Ctrl Pts',(0.983616340614008,6.69513165624673,
97.1507474009998));
#207690=CARTESIAN_POINT('Ctrl Pts',(0.79959148671359,6.72216769715964,97.1594965837355));
#207691=CARTESIAN_POINT('Ctrl Pts',(0.614451459526558,6.74161215869372,
97.1682457664712));
#207692=CARTESIAN_POINT('Ctrl Pts',(0.428825047910227,6.75339900185713,
97.1769949492069));
#207693=CARTESIAN_POINT('Ctrl Pts',(0.243199888596869,6.76518576550222,
97.1857440729174));
#207694=CARTESIAN_POINT('Ctrl Pts',(0.0570886373916178,6.76931499599835,
97.1944931966279));
#207695=CARTESIAN_POINT('Ctrl Pts',(-0.12887662681157,6.76577266947846,
97.2032423203385));
#207696=CARTESIAN_POINT('Ctrl Pts',(-0.314840698188679,6.76223036567991,
97.21199138793));
#207697=CARTESIAN_POINT('Ctrl Pts',(-0.500658497951871,6.75101660879219,
97.2207404555216));
#207698=CARTESIAN_POINT('Ctrl Pts',(-0.685698951926932,6.73216948296211,
97.2294895231131));
#207699=CARTESIAN_POINT('Ctrl Pts',(-0.870738280460631,6.71332247176283,
97.2382385374917));
#207700=CARTESIAN_POINT('Ctrl Pts',(-1.05499998761335,6.68684221356173,
97.2469875518702));
#207701=CARTESIAN_POINT('Ctrl Pts',(-1.2378582916151,6.65281863948505,97.2557365662487));
#207702=CARTESIAN_POINT('Ctrl Pts',(-1.43007412915765,6.61705395369163,
97.2649332999471));
#207703=CARTESIAN_POINT('Ctrl Pts',(-1.62073882532453,6.57295372728561,
97.2741300336454));
#207704=CARTESIAN_POINT('Ctrl Pts',(-1.80913696086522,6.52068343479665,
97.2833267673438));
#207705=CARTESIAN_POINT('Ctrl Pts',(-1.98838356181161,6.4709521981672,97.2920767650575));
#207706=CARTESIAN_POINT('Ctrl Pts',(-2.16557827567628,6.41382586852547,
97.3008267627712));
#207707=CARTESIAN_POINT('Ctrl Pts',(-2.34011918616847,6.34949849945066,
97.3095767604848));
#207708=CARTESIAN_POINT('Ctrl Pts',(-2.51465655686291,6.28517243497474,
97.3183265807431));
#207709=CARTESIAN_POINT('Ctrl Pts',(-2.68653996290572,6.21364572244431,
97.3270764010015));
#207710=CARTESIAN_POINT('Ctrl Pts',(-2.85518555375289,6.13516132254408,
97.3358262212598));
#207711=CARTESIAN_POINT('Ctrl Pts',(-3.02382794854042,6.05667841002826,
97.3445758756973));
#207712=CARTESIAN_POINT('Ctrl Pts',(-3.18923239104692,5.97123819494532,
97.3533255301348));
#207713=CARTESIAN_POINT('Ctrl Pts',(-3.35083705963173,5.87913088813292,
97.3620751845723));
#207714=CARTESIAN_POINT('Ctrl Pts',(-3.51243888037944,5.78702520445808,
97.3708246848212));
#207715=CARTESIAN_POINT('Ctrl Pts',(-3.67024081219308,5.68825280608611,
97.3795741850702));
#207716=CARTESIAN_POINT('Ctrl Pts',(-3.82370687540098,5.58314917685451,
97.3883236853191));
#207717=CARTESIAN_POINT('Ctrl Pts',(-3.97717043813603,5.4780472601108,97.3970730430096));
#207718=CARTESIAN_POINT('Ctrl Pts',(-4.12629803718343,5.36661448087402,
97.4058224007));
#207719=CARTESIAN_POINT('Ctrl Pts',(-4.27058317202889,5.24922931207846,
97.4145717583905));
#207720=CARTESIAN_POINT('Ctrl Pts',(-4.41486614770903,5.13184589990173,
97.4233209851506));
#207721=CARTESIAN_POINT('Ctrl Pts',(-4.55430658190572,5.00851045726527,
97.4320702119107));
#207722=CARTESIAN_POINT('Ctrl Pts',(-4.68843088998099,4.87964187106718,
97.4408194386707));
#207723=CARTESIAN_POINT('Ctrl Pts',(-4.82255336914208,4.75077504211645,
97.4495685461267));
#207724=CARTESIAN_POINT('Ctrl Pts',(-4.95135966061626,4.61637541911857,
97.4583176535826));
#207725=CARTESIAN_POINT('Ctrl Pts',(-5.07441230865859,4.47689945405682,
97.4670667610386));
#207726=CARTESIAN_POINT('Ctrl Pts',(-5.1974634422312,4.33742520559466,97.4758157608149));
#207727=CARTESIAN_POINT('Ctrl Pts',(-5.31476088451563,4.19287495495397,
97.4845647605912));
#207728=CARTESIAN_POINT('Ctrl Pts',(-5.42590627625749,4.04373961590873,
97.4933137603676));
#207729=CARTESIAN_POINT('Ctrl Pts',(-5.5370638066968,3.89458798910982,97.5020637156623));
#207730=CARTESIAN_POINT('Ctrl Pts',(-5.64206777068997,3.74085050159608,
97.510813670957));
#207731=CARTESIAN_POINT('Ctrl Pts',(-5.74056148161265,3.58304938227556,
97.5195636262517));
#207732=CARTESIAN_POINT('Ctrl Pts',(-5.83905138949253,3.42525435597766,
97.5283132436928));
#207733=CARTESIAN_POINT('Ctrl Pts',(-5.93103139555138,3.26339625501752,
97.5370628611339));
#207734=CARTESIAN_POINT('Ctrl Pts',(-6.01618907818452,3.09802485069653,
97.545812478575));
#207735=CARTESIAN_POINT('Ctrl Pts',(-6.10134392542713,2.93265895254363,
97.5545618046908));
#207736=CARTESIAN_POINT('Ctrl Pts',(-6.17967677259689,2.76378023990826,
97.5633111308067));
#207737=CARTESIAN_POINT('Ctrl Pts',(-6.25092157007211,2.59196229231971,
97.5720604569226));
#207738=CARTESIAN_POINT('Ctrl Pts',(-6.32216437405876,2.42014915233994,
97.5808095382251));
#207739=CARTESIAN_POINT('Ctrl Pts',(-6.38631941547183,2.24539720667797,
97.5895586195275));
#207740=CARTESIAN_POINT('Ctrl Pts',(-6.44316881035938,2.06829994952669,
97.59830770083));
#207741=CARTESIAN_POINT('Ctrl Pts',(-6.50002334523104,1.89118668029491,
97.6070575731723));
#207742=CARTESIAN_POINT('Ctrl Pts',(-6.54957082409764,1.71172794812797,
97.6158074455146));
#207743=CARTESIAN_POINT('Ctrl Pts',(-6.59164294294889,1.53053334255483,
97.624557317857));
#207744=CARTESIAN_POINT('Ctrl Pts',(-6.63371214081082,1.34935131698771,
97.6333065827119));
#207745=CARTESIAN_POINT('Ctrl Pts',(-6.66830695238781,1.16643393834958,
97.6420558475668));
#207746=CARTESIAN_POINT('Ctrl Pts',(-6.69530988153224,0.982402458393107,
97.6508051124217));
#207747=CARTESIAN_POINT('Ctrl Pts',(-6.7223141968986,0.798361530999497,
97.6595548264287));
#207748=CARTESIAN_POINT('Ctrl Pts',(-6.74172580828798,0.613206671415178,
97.6683045404357));
#207749=CARTESIAN_POINT('Ctrl Pts',(-6.75347878027844,0.427566795166304,
97.6770542544428));
#207750=CARTESIAN_POINT('Ctrl Pts',(-6.76248992366325,0.285234494521487,
97.6837627642186));
#207751=CARTESIAN_POINT('Ctrl Pts',(-6.76699999998218,0.142617266672671,
97.6904712739945));
#207752=CARTESIAN_POINT('Ctrl Pts',(-6.767,8.45744902084614E-10,97.6971797837703));
#207753=CARTESIAN_POINT('',(-6.76699990772313,-0.00111753082879368,97.302820216166));
#207754=CARTESIAN_POINT('Ctrl Pts',(3.09910619832137,6.01563211736939,96.6512761190133));
#207755=CARTESIAN_POINT('Ctrl Pts',(2.92861376027321,6.10346564196215,96.6603199929407));
#207756=CARTESIAN_POINT('Ctrl Pts',(2.75445852336425,6.18400957271852,96.6693638668681));
#207757=CARTESIAN_POINT('Ctrl Pts',(2.57725861818762,6.25699824316562,96.6784077407955));
#207758=CARTESIAN_POINT('Ctrl Pts',(2.45885991308518,6.30576668951141,96.6844505372691));
#207759=CARTESIAN_POINT('Ctrl Pts',(2.33910235745289,6.3511631275774,96.6904933337427));
#207760=CARTESIAN_POINT('Ctrl Pts',(2.21817473501266,6.39312050918419,96.6965361302162));
#207761=CARTESIAN_POINT('Ctrl Pts',(2.04500430488565,6.45320419952089,96.7051895184445));
#207762=CARTESIAN_POINT('Ctrl Pts',(1.86928063661445,6.50628616672954,96.7138429066727));
#207763=CARTESIAN_POINT('Ctrl Pts',(1.69158385446612,6.55216247229184,96.722496294901));
#207764=CARTESIAN_POINT('Ctrl Pts',(1.51405118790107,6.59799640783171,96.7311416911114));
#207765=CARTESIAN_POINT('Ctrl Pts',(1.33454933544504,6.63663787941284,96.7397870873218));
#207766=CARTESIAN_POINT('Ctrl Pts',(1.15367393555411,6.66793262191687,96.7484324835322));
#207767=CARTESIAN_POINT('Ctrl Pts',(0.967021984688984,6.70022681307675,
96.7573539845746));
#207768=CARTESIAN_POINT('Ctrl Pts',(0.778907605749406,6.72469713327135,
96.766275485617));
#207769=CARTESIAN_POINT('Ctrl Pts',(0.589999590374173,6.74123056150421,
96.7751969866594));
#207770=CARTESIAN_POINT('Ctrl Pts',(0.407286603180601,6.75722179435357,
96.7838259170014));
#207771=CARTESIAN_POINT('Ctrl Pts',(0.223831539131578,6.76578839481647,
96.7924548473433));
#207772=CARTESIAN_POINT('Ctrl Pts',(0.0402478550319398,6.76688030854435,
96.8010837776853));
#207773=CARTESIAN_POINT('Ctrl Pts',(-0.152672653839921,6.76802775556864,
96.8101515640779));
#207774=CARTESIAN_POINT('Ctrl Pts',(-0.345734871493498,6.76092033890367,
96.8192193504706));
#207775=CARTESIAN_POINT('Ctrl Pts',(-0.538222660122076,6.74556190158619,
96.8282871368632));
#207776=CARTESIAN_POINT('Ctrl Pts',(-0.730710448750655,6.73020346426871,
96.8373549232558));
#207777=CARTESIAN_POINT('Ctrl Pts',(-0.922623416278408,6.7065940022652,
96.8464227096485));
#207778=CARTESIAN_POINT('Ctrl Pts',(-1.11324685210927,6.67480115406211,
96.8554904960411));
#207779=CARTESIAN_POINT('Ctrl Pts',(-1.29035667972246,6.64526215304662,
96.8639154521743));
#207780=CARTESIAN_POINT('Ctrl Pts',(-1.46627565472855,6.60867210523293,
96.8723404083075));
#207781=CARTESIAN_POINT('Ctrl Pts',(-1.64042712639814,6.56515710725777,
96.8807653644406));
#207782=CARTESIAN_POINT('Ctrl Pts',(-1.81461902029628,6.5216320090338,96.889192276087));
#207783=CARTESIAN_POINT('Ctrl Pts',(-1.98704227115564,6.47117883622198,
96.8976191877334));
#207784=CARTESIAN_POINT('Ctrl Pts',(-2.15713379708643,6.41397402407178,
96.9060460993798));
#207785=CARTESIAN_POINT('Ctrl Pts',(-2.32728787229691,6.35674817548384,
96.9144761099298));
#207786=CARTESIAN_POINT('Ctrl Pts',(-2.49510819871737,6.29276584266367,
96.9229061204799));
#207787=CARTESIAN_POINT('Ctrl Pts',(-2.66004976575128,6.22225234490908,
96.9313361310299));
#207788=CARTESIAN_POINT('Ctrl Pts',(-2.8251432735071,6.15167389159511,96.9397739071294));
#207789=CARTESIAN_POINT('Ctrl Pts',(-2.98735241858218,6.07455238360894,
96.9482116832288));
#207790=CARTESIAN_POINT('Ctrl Pts',(-3.14615395981322,5.99116051038124,
96.9566494593283));
#207791=CARTESIAN_POINT('Ctrl Pts',(-3.30503886014756,5.90772486256723,
96.9650916646382));
#207792=CARTESIAN_POINT('Ctrl Pts',(-3.46051229959971,5.81801244594944,
96.9735338699481));
#207793=CARTESIAN_POINT('Ctrl Pts',(-3.61207782597344,5.72234067310843,
96.9819760752581));
#207794=CARTESIAN_POINT('Ctrl Pts',(-3.76380324563791,5.62656797181121,
96.9904271866301));
#207795=CARTESIAN_POINT('Ctrl Pts',(-3.91161224098012,5.5248235392749,96.9988782980021));
#207796=CARTESIAN_POINT('Ctrl Pts',(-4.0550385142914,5.41746727240815,97.0073294093741));
#207797=CARTESIAN_POINT('Ctrl Pts',(-4.0952913200611,5.38733756981895,97.0097012268713));
#207798=CARTESIAN_POINT('Ctrl Pts',(-4.13519912412756,5.35676608945096,
97.0120730443685));
#207799=CARTESIAN_POINT('Ctrl Pts',(-4.17475210936568,5.32576133762552,
97.0144448618657));
#207800=CARTESIAN_POINT('Ctrl Pts',(-4.31130984734547,5.21871660382311,
97.0226336251251));
#207801=CARTESIAN_POINT('Ctrl Pts',(-4.44390991622575,5.10628919919418,
97.0308223883844));
#207802=CARTESIAN_POINT('Ctrl Pts',(-4.57210181061662,4.98880487024259,
97.0390111516438));
#207803=CARTESIAN_POINT('Ctrl Pts',(-4.70017891787413,4.87142574052688,
97.047192582422));
#207804=CARTESIAN_POINT('Ctrl Pts',(-4.82385544599577,4.74899894623214,
97.0553740132001));
#207805=CARTESIAN_POINT('Ctrl Pts',(-4.9427126636262,4.6218914445094,97.0635554439783));
#207806=CARTESIAN_POINT('Ctrl Pts',(-5.06148777639424,4.49487174682705,
97.0717312231413));
#207807=CARTESIAN_POINT('Ctrl Pts',(-5.17544996309289,4.36317804441761,
97.0799070023043));
#207808=CARTESIAN_POINT('Ctrl Pts',(-5.28421614999827,4.22721523938603,
97.0880827814673));
#207809=CARTESIAN_POINT('Ctrl Pts',(-5.39292945624847,4.09131853763907,
97.0962545856766));
#207810=CARTESIAN_POINT('Ctrl Pts',(-5.49645156964861,3.95115714951615,
97.104426389886));
#207811=CARTESIAN_POINT('Ctrl Pts',(-5.59443861436529,3.8071702864593,97.1125981940953));
#207812=CARTESIAN_POINT('Ctrl Pts',(-5.69241281932611,3.66320229075552,
97.1207689275103));
#207813=CARTESIAN_POINT('Ctrl Pts',(-5.78485319070877,3.51541011286518,
97.1289396609253));
#207814=CARTESIAN_POINT('Ctrl Pts',(-5.87145807933155,3.36426351861033,
97.1371103943403));
#207815=CARTESIAN_POINT('Ctrl Pts',(-5.95806023035527,3.21312170213164,
97.1452808694767));
#207816=CARTESIAN_POINT('Ctrl Pts',(-6.03882708539064,3.05862599373177,
97.1534513446129));
#207817=CARTESIAN_POINT('Ctrl Pts',(-6.11350210031256,2.90127231908244,
97.1616218197493));
#207818=CARTESIAN_POINT('Ctrl Pts',(-6.1881885961294,2.74389445212452,97.1697935510537));
#207819=CARTESIAN_POINT('Ctrl Pts',(-6.25678123120196,2.58365807037784,
97.1779652823581));
#207820=CARTESIAN_POINT('Ctrl Pts',(-6.31907090956425,2.4210807173448,97.1861370136625));
#207821=CARTESIAN_POINT('Ctrl Pts',(-6.38138171056235,2.25844823379402,
97.194311516028));
#207822=CARTESIAN_POINT('Ctrl Pts',(-6.4373851687022,2.0934735353858,97.2024860183935));
#207823=CARTESIAN_POINT('Ctrl Pts',(-6.48692151016709,1.92669102892277,
97.210660520759));
#207824=CARTESIAN_POINT('Ctrl Pts',(-6.53651203079824,1.75972610815784,
97.2188439637872));
#207825=CARTESIAN_POINT('Ctrl Pts',(-6.57962120273745,1.59094977665672,
97.2270274068155));
#207826=CARTESIAN_POINT('Ctrl Pts',(-6.61613978835074,1.42090932187888,
97.2352108498437));
#207827=CARTESIAN_POINT('Ctrl Pts',(-6.65267973177354,1.25076941933814,
97.2433990789395));
#207828=CARTESIAN_POINT('Ctrl Pts',(-6.68262134463256,1.07936427551682,
97.2515873080353));
#207829=CARTESIAN_POINT('Ctrl Pts',(-6.70590711640198,0.907247896767613,
97.259775537131));
#207830=CARTESIAN_POINT('Ctrl Pts',(-6.72922704277555,0.734879064853413,
97.2679757763816));
#207831=CARTESIAN_POINT('Ctrl Pts',(-6.74587158896306,0.561797273121107,
97.2761760156322));
#207832=CARTESIAN_POINT('Ctrl Pts',(-6.75583530513779,0.388559300305317,
97.2843762548827));
#207833=CARTESIAN_POINT('Ctrl Pts',(-6.76330542845771,0.258677136067334,
97.2905242419772));
#207834=CARTESIAN_POINT('Ctrl Pts',(-6.76702134752883,0.128707221600665,
97.2966722290716));
#207835=CARTESIAN_POINT('Ctrl Pts',(-6.76699990772313,-0.00111753082898668,
97.302820216166));
#207836=CARTESIAN_POINT('Ctrl Pts',(-6.76699990772305,-0.00111753133218596,
97.3028202161898));
#207837=CARTESIAN_POINT('Ctrl Pts',(-6.76696557723693,-0.208999305795223,
97.3126646752983));
#207838=CARTESIAN_POINT('Ctrl Pts',(-6.75735392725586,-0.416689416762483,
97.3225091344068));
#207839=CARTESIAN_POINT('Ctrl Pts',(-6.73820661880235,-0.623586852273372,
97.3323535935154));
#207840=CARTESIAN_POINT('Ctrl Pts',(-6.72251090318371,-0.79318788616753,
97.3404234395182));
#207841=CARTESIAN_POINT('Ctrl Pts',(-6.70037864351555,-0.962509125773961,
97.3484932855209));
#207842=CARTESIAN_POINT('Ctrl Pts',(-6.67181409574403,-1.13101090703462,
97.3565631315237));
#207843=CARTESIAN_POINT('Ctrl Pts',(-6.64328548580689,-1.29930069162182,
97.3646228246337));
#207844=CARTESIAN_POINT('Ctrl Pts',(-6.60834075144577,-1.46677270607685,
97.3726825177438));
#207845=CARTESIAN_POINT('Ctrl Pts',(-6.56703608254974,-1.6328888787942,
97.3807422108538));
#207846=CARTESIAN_POINT('Ctrl Pts',(-6.52577431511291,-1.79883251348143,
97.3887935326924));
#207847=CARTESIAN_POINT('Ctrl Pts',(-6.47816584801549,-1.9634227498881,
97.396844854531));
#207848=CARTESIAN_POINT('Ctrl Pts',(-6.42431843337466,-2.12612832787736,
97.4048961763696));
#207849=CARTESIAN_POINT('Ctrl Pts',(-6.37051514802313,-2.28870056461767,
97.4129408999507));
#207850=CARTESIAN_POINT('Ctrl Pts',(-6.31048320821169,-2.44939086464614,
97.4209856235317));
#207851=CARTESIAN_POINT('Ctrl Pts',(-6.24438102245941,-2.60767993556509,
97.4290303471128));
#207852=CARTESIAN_POINT('Ctrl Pts',(-6.17831853928764,-2.76587393421814,
97.4370702388372));
#207853=CARTESIAN_POINT('Ctrl Pts',(-6.10619321152113,-2.92166923139394,
97.4451101305615));
#207854=CARTESIAN_POINT('Ctrl Pts',(-6.02821267335559,-3.07456354053628,
97.4531500222859));
#207855=CARTESIAN_POINT('Ctrl Pts',(-5.9485530005616,-3.23075008303602,
97.4613630349059));
#207856=CARTESIAN_POINT('Ctrl Pts',(-5.8627832246035,-3.38390890941726,
97.4695760475258));
#207857=CARTESIAN_POINT('Ctrl Pts',(-5.7711759399275,-3.53352759581725,
97.4777890601458));
#207858=CARTESIAN_POINT('Ctrl Pts',(-5.68153092062217,-3.6799413889801,
97.4858261466883));
#207859=CARTESIAN_POINT('Ctrl Pts',(-5.58629615700854,-3.82296484362236,
97.4938632332309));
#207860=CARTESIAN_POINT('Ctrl Pts',(-5.48577255860638,-3.96214442382421,
97.5019003197735));
#207861=CARTESIAN_POINT('Ctrl Pts',(-5.38523933962797,-4.10133732415967,
97.5099381755026));
#207862=CARTESIAN_POINT('Ctrl Pts',(-5.27941649666478,-4.23668531458168,
97.5179760312318));
#207863=CARTESIAN_POINT('Ctrl Pts',(-5.16864690252021,-4.3677658129836,
97.5260138869609));
#207864=CARTESIAN_POINT('Ctrl Pts',(-5.05784476005486,-4.49888482782266,
97.5340541045179));
#207865=CARTESIAN_POINT('Ctrl Pts',(-4.94209321420227,-4.62573356948039,
97.5420943220748));
#207866=CARTESIAN_POINT('Ctrl Pts',(-4.82177374861879,-4.74792448519674,
97.5501345396318));
#207867=CARTESIAN_POINT('Ctrl Pts',(-4.69690853653508,-4.8747318519984,
97.5584785217595));
#207868=CARTESIAN_POINT('Ctrl Pts',(-4.56712381728006,-4.99652224993349,
97.5668225038873));
#207869=CARTESIAN_POINT('Ctrl Pts',(-4.43288489319439,-5.11290724771034,
97.575166486015));
#207870=CARTESIAN_POINT('Ctrl Pts',(-4.30330777794423,-5.22525046241532,
97.58322070085));
#207871=CARTESIAN_POINT('Ctrl Pts',(-4.16958096857007,-5.33255723884154,
97.5912749156851));
#207872=CARTESIAN_POINT('Ctrl Pts',(-4.03215331479852,-5.43452193352454,
97.5993291305202));
#207873=CARTESIAN_POINT('Ctrl Pts',(-3.89462281915308,-5.5365629319207,
97.6073893726032));
#207874=CARTESIAN_POINT('Ctrl Pts',(-3.75338627090088,-5.63325367911062,
97.6154496146862));
#207875=CARTESIAN_POINT('Ctrl Pts',(-3.60891848628086,-5.72433370440441,
97.6235098567692));
#207876=CARTESIAN_POINT('Ctrl Pts',(-3.46424872578826,-5.81554106582114,
97.6315813676236));
#207877=CARTESIAN_POINT('Ctrl Pts',(-3.31633903606825,-5.90112186952757,
97.6396528784779));
#207878=CARTESIAN_POINT('Ctrl Pts',(-3.16568612874992,-5.98086284195185,
97.6477243893322));
#207879=CARTESIAN_POINT('Ctrl Pts',(-3.14989613112094,-5.98922052842418,
97.6485703679431));
#207880=CARTESIAN_POINT('Ctrl Pts',(-3.13407601377241,-5.9975141077073,
97.6494163465539));
#207881=CARTESIAN_POINT('Ctrl Pts',(-3.11822635877598,-6.00574336576536,
97.6502623251648));
#207882=CARTESIAN_POINT('Ctrl Pts',(-2.96404897471086,-6.08579340347751,
97.6584915749007));
#207883=CARTESIAN_POINT('Ctrl Pts',(-2.80656053152289,-6.16002027173922,
97.6667208246367));
#207884=CARTESIAN_POINT('Ctrl Pts',(-2.64623981894299,-6.22813807013305,
97.6749500743726));
#207885=CARTESIAN_POINT('Ctrl Pts',(-2.48610991409193,-6.29617479726543,
97.6831695299627));
#207886=CARTESIAN_POINT('Ctrl Pts',(-2.32315477876337,-6.35811679331115,
97.6913889855527));
#207887=CARTESIAN_POINT('Ctrl Pts',(-2.15787869783316,-6.41372345252256,
97.6996084411428));
#207888=CARTESIAN_POINT('Ctrl Pts',(-1.99276613082334,-6.46927509794857,
97.7078197649124));
#207889=CARTESIAN_POINT('Ctrl Pts',(-1.82533752860868,-6.51850377510092,
97.7160310886821));
#207890=CARTESIAN_POINT('Ctrl Pts',(-1.65611818818594,-6.5612164685186,
97.7242424124517));
#207891=CARTESIAN_POINT('Ctrl Pts',(-1.4870322917781,-6.60389547930118,
97.7324472608858));
#207892=CARTESIAN_POINT('Ctrl Pts',(-1.31615881600288,-6.64006865346927,
97.7406521093199));
#207893=CARTESIAN_POINT('Ctrl Pts',(-1.1440393818071,-6.66959240830161,
97.748856957754));
#207894=CARTESIAN_POINT('Ctrl Pts',(-0.972021134188419,-6.69909880653672,
97.7570569826739));
#207895=CARTESIAN_POINT('Ctrl Pts',(-0.798758739862287,-6.72196351228072,
97.7652570075939));
#207896=CARTESIAN_POINT('Ctrl Pts',(-0.624805296458579,-6.73809374686323,
97.7734570325138));
#207897=CARTESIAN_POINT('Ctrl Pts',(-0.450902199122845,-6.75421931299037,
97.7816546841607));
#207898=CARTESIAN_POINT('Ctrl Pts',(-0.276308807395237,-6.76361425331227,
97.7898523358076));
#207899=CARTESIAN_POINT('Ctrl Pts',(-0.101584901233675,-6.76623747054752,
97.7980499874546));
#207900=CARTESIAN_POINT('Ctrl Pts',(0.0731156083249307,-6.7688603365179,
97.8062465413856));
#207901=CARTESIAN_POINT('Ctrl Pts',(0.247946238931239,-6.76471327913527,
97.8144430953167));
#207902=CARTESIAN_POINT('Ctrl Pts',(0.422345625779649,-6.75380730939111,
97.8226396492478));
#207903=CARTESIAN_POINT('Ctrl Pts',(0.596753369820246,-6.74290081703454,
97.8308365959565));
#207904=CARTESIAN_POINT('Ctrl Pts',(0.770729470853724,-6.72523478939104,
97.8390335426652));
#207905=CARTESIAN_POINT('Ctrl Pts',(0.943716050492217,-6.70087225785147,
97.8472304893739));
#207906=CARTESIAN_POINT('Ctrl Pts',(1.1167423730068,-6.67650412913161,97.8554293192936));
#207907=CARTESIAN_POINT('Ctrl Pts',(1.28877836616733,-6.64543648232545,
97.8636281492134));
#207908=CARTESIAN_POINT('Ctrl Pts',(1.45927467517108,-6.60778377539734,
97.8718269791331));
#207909=CARTESIAN_POINT('Ctrl Pts',(1.62993246597567,-6.57009540654226,
97.880033574393));
#207910=CARTESIAN_POINT('Ctrl Pts',(1.79904730835214,-6.52580959428659,
97.8882401696528));
#207911=CARTESIAN_POINT('Ctrl Pts',(1.96608246660753,-6.47509140742418,
97.8964467649126));
#207912=CARTESIAN_POINT('Ctrl Pts',(2.13319847083731,-6.42434867266851,
97.9046573322116));
#207913=CARTESIAN_POINT('Ctrl Pts',(2.29823244529167,-6.36716747349638,
97.9128678995105));
#207914=CARTESIAN_POINT('Ctrl Pts',(2.46066615762505,-6.30376165957429,
97.9210784668095));
#207915=CARTESIAN_POINT('Ctrl Pts',(2.62332388930164,-6.24026839995767,
97.9293003576562));
#207916=CARTESIAN_POINT('Ctrl Pts',(2.78337386297379,-6.17053351247428,
97.9375222485029));
#207917=CARTESIAN_POINT('Ctrl Pts',(2.94031992605678,-6.09481810495059,
97.9457441393496));
#207918=CARTESIAN_POINT('Ctrl Pts',(3.08302093684233,-6.02597493059229,
97.9532197785045));
#207919=CARTESIAN_POINT('Ctrl Pts',(3.22315604607831,-5.95218827169844,
97.9606954176594));
#207920=CARTESIAN_POINT('Ctrl Pts',(3.36037287420268,-5.87368565266501,
97.9681710568143));
#207921=CARTESIAN_POINT('Ctrl Pts',(3.52439387510971,-5.77984819611038,
97.9771070002651));
#207922=CARTESIAN_POINT('Ctrl Pts',(3.68458662949134,-5.67907685311374,
97.9860429437158));
#207923=CARTESIAN_POINT('Ctrl Pts',(3.8403817698925,-5.571692459341,97.9949788871666));
#207924=CARTESIAN_POINT('Ctrl Pts',(3.99594270887565,-5.46446949279397,
98.0039013975242));
#207925=CARTESIAN_POINT('Ctrl Pts',(4.14711901254683,-5.35065345771596,
98.0128239078818));
#207926=CARTESIAN_POINT('Ctrl Pts',(4.29336864012611,-5.23060940235281,
98.0217464182394));
#207927=CARTESIAN_POINT('Ctrl Pts',(4.4392599107323,-5.11085949217849,98.0306470656777));
#207928=CARTESIAN_POINT('Ctrl Pts',(4.58024839936626,-4.98491218265454,
98.039547713116));
#207929=CARTESIAN_POINT('Ctrl Pts',(4.71582408372049,-4.85317341658032,
98.0484483605543));
#207930=CARTESIAN_POINT('Ctrl Pts',(4.85119025258741,-4.72163823650974,
98.0573352531406));
#207931=CARTESIAN_POINT('Ctrl Pts',(4.98116011854419,-4.58432963179605,
98.0662221457268));
#207932=CARTESIAN_POINT('Ctrl Pts',(5.10525727675793,-4.44169304861448,
98.075109038313));
#207933=CARTESIAN_POINT('Ctrl Pts',(5.22903545895087,-4.29942309469646,
98.0839730882679));
#207934=CARTESIAN_POINT('Ctrl Pts',(5.34697088555874,-4.15185268373672,
98.0928371382229));
#207935=CARTESIAN_POINT('Ctrl Pts',(5.4586250288735,-3.99946268818148,98.1017011881778));
#207936=CARTESIAN_POINT('Ctrl Pts',(5.56537537183755,-3.85376559350265,
98.1101759329982));
#207937=CARTESIAN_POINT('Ctrl Pts',(5.66638412626853,-3.7036633459917,98.1186506778186));
#207938=CARTESIAN_POINT('Ctrl Pts',(5.76129989740328,-3.54960737155266,
98.1271254226391));
#207939=CARTESIAN_POINT('Ctrl Pts',(5.85323841115532,-3.40038372668082,
98.1353343370682));
#207940=CARTESIAN_POINT('Ctrl Pts',(5.93937073690846,-3.24759383477967,
98.1435432514973));
#207941=CARTESIAN_POINT('Ctrl Pts',(6.01942515262468,-3.09173249682915,
98.1517521659264));
#207942=CARTESIAN_POINT('Ctrl Pts',(6.09949860087152,-2.93583410363737,
98.1599630319832));
#207943=CARTESIAN_POINT('Ctrl Pts',(6.17349109755966,-2.77686312634199,
98.16817389804));
#207944=CARTESIAN_POINT('Ctrl Pts',(6.24117784354158,-2.61533709591818,
98.1763847640968));
#207945=CARTESIAN_POINT('Ctrl Pts',(6.30889274714978,-2.45374387080901,
98.1845990458666));
#207946=CARTESIAN_POINT('Ctrl Pts',(6.37029653660469,-2.2895938031936,98.1928133276365));
#207947=CARTESIAN_POINT('Ctrl Pts',(6.42521329102133,-2.1234225120976,98.2010276094063));
#207948=CARTESIAN_POINT('Ctrl Pts',(6.48019185858039,-1.95706418209532,
98.2092511369987));
#207949=CARTESIAN_POINT('Ctrl Pts',(6.52866869548075,-1.78868042282136,
98.2174746645911));
#207950=CARTESIAN_POINT('Ctrl Pts',(6.57051805780283,-1.61882100680926,
98.2256981921835));
#207951=CARTESIAN_POINT('Ctrl Pts',(6.61239424393825,-1.44885271751887,
98.2339269907372));
#207952=CARTESIAN_POINT('Ctrl Pts',(6.64763441596179,-1.27740723390562,
98.2421557892909));
#207953=CARTESIAN_POINT('Ctrl Pts',(6.67616432920691,-1.10504246498732,
98.2503845878446));
#207954=CARTESIAN_POINT('Ctrl Pts',(6.70473351159456,-0.932440449757783,
98.2586247126811));
#207955=CARTESIAN_POINT('Ctrl Pts',(6.72657394253494,-0.758916974114773,
98.2668648375175));
#207956=CARTESIAN_POINT('Ctrl Pts',(6.74166331253418,-0.585033999380091,
98.2751049623539));
#207957=CARTESIAN_POINT('Ctrl Pts',(6.74836237009857,-0.507837134482928,
98.2787632377239));
#207958=CARTESIAN_POINT('Ctrl Pts',(6.75373148684604,-0.430569403098271,
98.2824215130939));
#207959=CARTESIAN_POINT('Ctrl Pts',(6.7577719980426,-0.353279807619042,
98.2860797884639));
#207960=CARTESIAN_POINT('Ctrl Pts',(6.76710271459848,-0.174795632460588,
98.2945278112264));
#207961=CARTESIAN_POINT('Ctrl Pts',(6.76936610890676,0.00421340103325585,
98.3029758339889));
#207962=CARTESIAN_POINT('Ctrl Pts',(6.76452071377118,0.18316253154156,98.3114238567515));
#207963=CARTESIAN_POINT('Ctrl Pts',(6.75967975570863,0.361947792986718,
98.3198641434073));
#207964=CARTESIAN_POINT('Ctrl Pts',(6.74774299300604,0.540672928999616,
98.3283044300631));
#207965=CARTESIAN_POINT('Ctrl Pts',(6.72872095447458,0.718751220391842,
98.3367447167189));
#207966=CARTESIAN_POINT('Ctrl Pts',(6.70971340665599,0.896693854326269,
98.3451785736868));
#207967=CARTESIAN_POINT('Ctrl Pts',(6.6836313781627,1.07399029549173,98.3536124306547));
#207968=CARTESIAN_POINT('Ctrl Pts',(6.65053738512199,1.25005659435674,98.3620462876226));
#207969=CARTESIAN_POINT('Ctrl Pts',(6.61746351494715,1.42601583577142,98.3704750163676));
#207970=CARTESIAN_POINT('Ctrl Pts',(6.57738624223562,1.6007460992165,98.3789037451127));
#207971=CARTESIAN_POINT('Ctrl Pts',(6.53041962645837,1.77367091151864,98.3873324738577));
#207972=CARTESIAN_POINT('Ctrl Pts',(6.48347435649263,1.94651713139105,98.395757371838));
#207973=CARTESIAN_POINT('Ctrl Pts',(6.42964607422645,2.11755921500679,98.4041822698183));
#207974=CARTESIAN_POINT('Ctrl Pts',(6.36909950718439,2.28623281132599,98.4126071677985));
#207975=CARTESIAN_POINT('Ctrl Pts',(6.30856634525084,2.45486906303636,98.4210302004927));
#207976=CARTESIAN_POINT('Ctrl Pts',(6.24131797429288,2.62113755848007,98.4294532331868));
#207977=CARTESIAN_POINT('Ctrl Pts',(6.16756854401525,2.78449048388994,98.437876265881));
#207978=CARTESIAN_POINT('Ctrl Pts',(6.0938274584019,2.94782492610181,98.4462983455186));
#207979=CARTESIAN_POINT('Ctrl Pts',(6.01358691708799,3.10824415206556,98.4547204251562));
#207980=CARTESIAN_POINT('Ctrl Pts',(5.92710877035332,3.26522137448609,98.4631425047938));
#207981=CARTESIAN_POINT('Ctrl Pts',(5.84062833681939,3.4222027479599,98.471564807142));
#207982=CARTESIAN_POINT('Ctrl Pts',(5.74791013024976,3.57574164452383,98.4799871094903));
#207983=CARTESIAN_POINT('Ctrl Pts',(5.64926158926187,3.72533656145193,98.4884094118385));
#207984=CARTESIAN_POINT('Ctrl Pts',(5.5505966682449,3.87495631776503,98.4968331126622));
#207985=CARTESIAN_POINT('Ctrl Pts',(5.4459996336756,4.02063051079294,98.5052568134858));
#207986=CARTESIAN_POINT('Ctrl Pts',(5.33582101344589,4.1618869653643,98.5136805143095));
#207987=CARTESIAN_POINT('Ctrl Pts',(5.22556783433685,4.30323900946955,98.5221099155284));
#207988=CARTESIAN_POINT('Ctrl Pts',(5.10972572729284,4.44016707811551,98.5305393167474));
#207989=CARTESIAN_POINT('Ctrl Pts',(4.98868588754732,4.57223163404768,98.5389687179664));
#207990=CARTESIAN_POINT('Ctrl Pts',(4.86760286095511,4.70434331042994,98.547401126784));
#207991=CARTESIAN_POINT('Ctrl Pts',(4.7413186336268,4.83158777234661,98.5558335356016));
#207992=CARTESIAN_POINT('Ctrl Pts',(4.6102613606425,4.95356227240223,98.5642659444193));
#207993=CARTESIAN_POINT('Ctrl Pts',(4.47908282965597,5.07564962681431,98.5727061551469));
#207994=CARTESIAN_POINT('Ctrl Pts',(4.34312267796113,5.19245705453213,98.5811463658745));
#207995=CARTESIAN_POINT('Ctrl Pts',(4.20284307838113,5.3036213155262,98.5895865766021));
#207996=CARTESIAN_POINT('Ctrl Pts',(4.12305443588864,5.36684965025879,98.5943872244392));
#207997=CARTESIAN_POINT('Ctrl Pts',(4.04186896918814,5.42825310035317,98.5991878722763));
#207998=CARTESIAN_POINT('Ctrl Pts',(3.95937594541419,5.48777105233769,98.6039885201133));
#207999=CARTESIAN_POINT('Ctrl Pts',(3.81951609252751,5.5886786397657,98.612127607148));
#208000=CARTESIAN_POINT('Ctrl Pts',(3.67561726787852,5.68436515395346,98.6202666941827));
#208001=CARTESIAN_POINT('Ctrl Pts',(3.52811070582312,5.77448905509884,98.6284057812174));
#208002=CARTESIAN_POINT('Ctrl Pts',(3.38822187768102,5.85995865552304,98.636124538482));
#208003=CARTESIAN_POINT('Ctrl Pts',(3.24508879753987,5.94042546090201,98.6438432957465));
#208004=CARTESIAN_POINT('Ctrl Pts',(3.09910619832135,6.0156321173694,98.651562053011));
#208005=CARTESIAN_POINT('Origin',(0.,0.,4.30282021618968));
#208006=CARTESIAN_POINT('',(3.09910619832146,6.01563211736934,101.0456200824));
#208007=CARTESIAN_POINT('',(3.09910619832147,6.01563211736933,100.651473518761));
#208008=CARTESIAN_POINT('',(3.09910619832133,6.0156321173694,4.30282021618968));
#208009=CARTESIAN_POINT('',(-6.767,4.25434840622355E-12,99.6971797838099));
#208010=CARTESIAN_POINT('Ctrl Pts',(-6.76699999999964,2.20710901944525E-6,
99.6972269161604));
#208011=CARTESIAN_POINT('Ctrl Pts',(-6.76700005739661,-0.175976986951552,
99.7054676366832));
#208012=CARTESIAN_POINT('Ctrl Pts',(-6.76013113518234,-0.351928063196356,
99.7137083572059));
#208013=CARTESIAN_POINT('Ctrl Pts',(-6.74642581124832,-0.52728338995501,
99.7219490777287));
#208014=CARTESIAN_POINT('Ctrl Pts',(-6.73271589701395,-0.70269744816884,
99.7301925583017));
#208015=CARTESIAN_POINT('Ctrl Pts',(-6.71216504593372,-0.877515008085112,
99.7384360388747));
#208016=CARTESIAN_POINT('Ctrl Pts',(-6.6848576569018,-1.05117415634203,
99.7466795194477));
#208017=CARTESIAN_POINT('Ctrl Pts',(-6.65753639969662,-1.22492149813339,
99.7549271865072));
#208018=CARTESIAN_POINT('Ctrl Pts',(-6.62345182177918,-1.3975089083452,
99.7631748535667));
#208019=CARTESIAN_POINT('Ctrl Pts',(-6.58273933361654,-1.56838511394929,
99.7714225206262));
#208020=CARTESIAN_POINT('Ctrl Pts',(-6.54197807578351,-1.73946601291898,
99.7796800676028));
#208021=CARTESIAN_POINT('Ctrl Pts',(-6.49457313230035,-1.90883127057889,
99.7879376145793));
#208022=CARTESIAN_POINT('Ctrl Pts',(-6.4407099366649,-2.07594424581827,
99.7961951615558));
#208023=CARTESIAN_POINT('Ctrl Pts',(-6.38680837714483,-2.24317624672676,
99.8044585899431));
#208024=CARTESIAN_POINT('Ctrl Pts',(-6.32643951565873,-2.40815243731166,
99.8127220183304));
#208025=CARTESIAN_POINT('Ctrl Pts',(-6.25983675034266,-2.57035656263085,
99.8209854467177));
#208026=CARTESIAN_POINT('Ctrl Pts',(-6.19314394731612,-2.73277996545306,
99.8292600461153));
#208027=CARTESIAN_POINT('Ctrl Pts',(-6.12020055689815,-2.89242350031711,
99.8375346455128));
#208028=CARTESIAN_POINT('Ctrl Pts',(-6.04128608876983,-3.04879507242388,
99.8458092449103));
#208029=CARTESIAN_POINT('Ctrl Pts',(-6.02493670803759,-3.08119189937728,
99.8475235639593));
#208030=CARTESIAN_POINT('Ctrl Pts',(-6.00833117996067,-3.11344838274264,
99.8492378830084));
#208031=CARTESIAN_POINT('Ctrl Pts',(-5.99147222024645,-3.14556030525805,
99.8509522020574));
#208032=CARTESIAN_POINT('Ctrl Pts',(-5.90839265842365,-3.30380520868575,
99.85940022482));
#208033=CARTESIAN_POINT('Ctrl Pts',(-5.81896785728657,-3.45889409277439,
99.8678482475825));
#208034=CARTESIAN_POINT('Ctrl Pts',(-5.72346063661553,-3.6103029431216,
99.8762962703451));
#208035=CARTESIAN_POINT('Ctrl Pts',(-5.62804087475901,-3.76157314386239,
99.8847365570008));
#208036=CARTESIAN_POINT('Ctrl Pts',(-5.52654997281395,-3.90916974737669,
99.8931768436566));
#208037=CARTESIAN_POINT('Ctrl Pts',(-5.41929646235672,-4.0525935958455,
99.9016171303124));
#208038=CARTESIAN_POINT('Ctrl Pts',(-5.31212465606703,-4.19590818610826,
99.9100509872803));
#208039=CARTESIAN_POINT('Ctrl Pts',(-5.19919919151935,-4.33505609201034,
99.9184848442482));
#208040=CARTESIAN_POINT('Ctrl Pts',(-5.08087189155359,-4.46956707317618,
99.9269187012161));
#208041=CARTESIAN_POINT('Ctrl Pts',(-4.9626165407296,-4.60399626468184,
99.9353474299611));
#208042=CARTESIAN_POINT('Ctrl Pts',(-4.83896612283186,-4.73379390296965,
99.9437761587062));
#208043=CARTESIAN_POINT('Ctrl Pts',(-4.71031296775279,-4.85852248588189,
99.9522048874512));
#208044=CARTESIAN_POINT('Ctrl Pts',(-4.58171828412037,-4.98319438102243,
99.9606297854315));
#208045=CARTESIAN_POINT('Ctrl Pts',(-4.44812563610895,-5.10280158288232,
99.9690546834118));
#208046=CARTESIAN_POINT('Ctrl Pts',(-4.30996473665161,-5.21694287574817,
99.9774795813921));
#208047=CARTESIAN_POINT('Ctrl Pts',(-4.17183442624283,-5.33105889754556,
99.9859026140863));
#208048=CARTESIAN_POINT('Ctrl Pts',(-4.02913813615296,-5.43971120892498,
99.9943256467804));
#208049=CARTESIAN_POINT('Ctrl Pts',(-3.88233963739472,-5.54253804135919,
100.002748679475));
#208050=CARTESIAN_POINT('Ctrl Pts',(-3.7355577487197,-5.64535323905425,
100.011170759112));
#208051=CARTESIAN_POINT('Ctrl Pts',(-3.58467484977971,-5.74234408056313,
100.01959283875));
#208052=CARTESIAN_POINT('Ctrl Pts',(-3.43018499781208,-5.83319122614585,
100.028014918387));
#208053=CARTESIAN_POINT('Ctrl Pts',(-3.27569106056693,-5.92404077405985,
100.036437220736));
#208054=CARTESIAN_POINT('Ctrl Pts',(-3.11759026777796,-6.00874613343463,
100.044859523084));
#208055=CARTESIAN_POINT('Ctrl Pts',(-2.95640297310033,-6.08703297679942,
100.053281825432));
#208056=CARTESIAN_POINT('Ctrl Pts',(-2.79518891418851,-6.1653328192496,
100.061705526256));
#208057=CARTESIAN_POINT('Ctrl Pts',(-2.63088763181189,-6.23721187575772,
100.070129227079));
#208058=CARTESIAN_POINT('Ctrl Pts',(-2.46404156339597,-6.30244303217864,
100.078552927903));
#208059=CARTESIAN_POINT('Ctrl Pts',(-2.29708258872094,-6.3677183311192,
100.086982329122));
#208060=CARTESIAN_POINT('Ctrl Pts',(-2.1275756977702,-6.42633661894526,
100.095411730341));
#208061=CARTESIAN_POINT('Ctrl Pts',(-1.95608163936907,-6.47811960526534,
100.10384113156));
#208062=CARTESIAN_POINT('Ctrl Pts',(-1.78452639212626,-6.52992106768298,
100.112273540378));
#208063=CARTESIAN_POINT('Ctrl Pts',(-1.61098288467417,-6.57488227520103,
100.120705949195));
#208064=CARTESIAN_POINT('Ctrl Pts',(-1.43602486982045,-6.61287543911551,
100.129138358013));
#208065=CARTESIAN_POINT('Ctrl Pts',(-1.26090497872051,-6.65090375541076,
100.13757856874));
#208066=CARTESIAN_POINT('Ctrl Pts',(-1.08436829267871,-6.68195108219252,
100.146018779468));
#208067=CARTESIAN_POINT('Ctrl Pts',(-0.906997651418675,-6.70594096755415,
100.154458990196));
#208068=CARTESIAN_POINT('Ctrl Pts',(-0.806112257341587,-6.71958600498187,
100.159259638033));
#208069=CARTESIAN_POINT('Ctrl Pts',(-0.704957176500564,-6.73094880866589,
100.16406028587));
#208070=CARTESIAN_POINT('Ctrl Pts',(-0.603640110343725,-6.74002282022726,
100.168860933707));
#208071=CARTESIAN_POINT('Ctrl Pts',(-0.431852452833622,-6.75540821628614,
100.17700064874));
#208072=CARTESIAN_POINT('Ctrl Pts',(-0.25925645436591,-6.76424128893959,
100.185140363773));
#208073=CARTESIAN_POINT('Ctrl Pts',(-0.086397400190767,-6.76644843985678,
100.193280078806));
#208074=CARTESIAN_POINT('Ctrl Pts',(0.0863104724931837,-6.76865366041303,
100.201412674893));
#208075=CARTESIAN_POINT('Ctrl Pts',(0.259280579266327,-6.76424448948375,
100.20954527098));
#208076=CARTESIAN_POINT('Ctrl Pts',(0.431962167790192,-6.75319907048489,
100.217677867067));
#208077=CARTESIAN_POINT('Ctrl Pts',(0.604525701916003,-6.74216120272703,
100.225804903275));
#208078=CARTESIAN_POINT('Ctrl Pts',(0.776800746537316,-6.7244961429065,
100.233931939483));
#208079=CARTESIAN_POINT('Ctrl Pts',(0.948236242228564,-6.70023410254629,
100.242058975691));
#208080=CARTESIAN_POINT('Ctrl Pts',(1.11958978865013,-6.67598365988048,
100.250182127028));
#208081=CARTESIAN_POINT('Ctrl Pts',(1.29010422347559,-6.645142567487,100.258305278366));
#208082=CARTESIAN_POINT('Ctrl Pts',(1.45923332371553,-6.60779290739034,
100.266428429704));
#208083=CARTESIAN_POINT('Ctrl Pts',(1.6283148974206,-6.57045374282592,100.274549298375));
#208084=CARTESIAN_POINT('Ctrl Pts',(1.79601155481641,-6.52660973315067,
100.282670167047));
#208085=CARTESIAN_POINT('Ctrl Pts',(1.96178702105474,-6.47639411123359,
100.290791035719));
#208086=CARTESIAN_POINT('Ctrl Pts',(2.12757144643456,-6.42617577547188,
100.298912343273));
#208087=CARTESIAN_POINT('Ctrl Pts',(2.29143412157694,-6.36958524189536,
100.307033650828));
#208088=CARTESIAN_POINT('Ctrl Pts',(2.45285351711438,-6.30680573853196,
100.315154958382));
#208089=CARTESIAN_POINT('Ctrl Pts',(2.53673264626406,-6.27418332625592,
100.319375072099));
#208090=CARTESIAN_POINT('Ctrl Pts',(2.61995231673305,-6.23989057850436,
100.323595185816));
#208091=CARTESIAN_POINT('Ctrl Pts',(2.70244140676876,-6.20395836889495,
100.327815299532));
#208092=CARTESIAN_POINT('Ctrl Pts',(2.8780570911426,-6.12746025770365,100.336799738058));
#208093=CARTESIAN_POINT('Ctrl Pts',(3.05027322548326,-6.04356666527602,
100.345784176584));
#208094=CARTESIAN_POINT('Ctrl Pts',(3.21850490740853,-5.95260574546872,
100.354768615109));
#208095=CARTESIAN_POINT('Ctrl Pts',(3.38702694717759,-5.86148783254192,
100.36376856024));
#208096=CARTESIAN_POINT('Ctrl Pts',(3.55155057917703,-5.76327832582239,
100.372768505371));
#208097=CARTESIAN_POINT('Ctrl Pts',(3.71151804072702,-5.65834983306598,
100.381768450501));
#208098=CARTESIAN_POINT('Ctrl Pts',(3.8718624697043,-5.55317407362434,100.390789604233));
#208099=CARTESIAN_POINT('Ctrl Pts',(4.02762904515278,-5.44124777955361,
100.399810757965));
#208100=CARTESIAN_POINT('Ctrl Pts',(4.1782891585767,-5.32298682201266,100.408831911698));
#208101=CARTESIAN_POINT('Ctrl Pts',(4.32910256985377,-5.20460553301509,
100.417862244525));
#208102=CARTESIAN_POINT('Ctrl Pts',(4.47479895494853,-5.07987685601615,
100.426892577352));
#208103=CARTESIAN_POINT('Ctrl Pts',(4.61488385498987,-4.94925610621979,
100.435922910179));
#208104=CARTESIAN_POINT('Ctrl Pts',(4.75516735126224,-4.81845017737417,
100.444966045172));
#208105=CARTESIAN_POINT('Ctrl Pts',(4.88982328077036,-4.68173563655124,
100.454009180164));
#208106=CARTESIAN_POINT('Ctrl Pts',(5.0183933863659,-4.53960535946452,100.463052315157));
#208107=CARTESIAN_POINT('Ctrl Pts',(5.13079327947637,-4.41535075238996,
100.470958098557));
#208108=CARTESIAN_POINT('Ctrl Pts',(5.23854242541837,-4.28695762868836,
100.478863881957));
#208109=CARTESIAN_POINT('Ctrl Pts',(5.34135995672388,-4.15477590402981,
100.486769665357));
#208110=CARTESIAN_POINT('Ctrl Pts',(5.45390035532087,-4.01009450785711,
100.495423053585));
#208111=CARTESIAN_POINT('Ctrl Pts',(5.56063072693521,-3.86074548506657,
100.504076441813));
#208112=CARTESIAN_POINT('Ctrl Pts',(5.66117154296611,-3.70721266737029,
100.512729830042));
#208113=CARTESIAN_POINT('Ctrl Pts',(5.76161950242172,-3.55382164812173,
100.521375226252));
#208114=CARTESIAN_POINT('Ctrl Pts',(5.8558891419884,-3.39625479431927,100.530020622462));
#208115=CARTESIAN_POINT('Ctrl Pts',(5.9436429873451,-3.23502659015091,100.538666018673));
#208116=CARTESIAN_POINT('Ctrl Pts',(6.03419939491393,-3.06864930025651,
100.547587519715));
#208117=CARTESIAN_POINT('Ctrl Pts',(6.11781672766863,-2.89837317803971,
100.556509020757));
#208118=CARTESIAN_POINT('Ctrl Pts',(6.19417306280503,-2.72479523414524,
100.5654305218));
#208119=CARTESIAN_POINT('Ctrl Pts',(6.26802537688636,-2.55690958579417,
100.574059452142));
#208120=CARTESIAN_POINT('Ctrl Pts',(6.33508522134007,-2.38593553972064,
100.582688382484));
#208121=CARTESIAN_POINT('Ctrl Pts',(6.39510808107167,-2.21243793843169,
100.591317312826));
#208122=CARTESIAN_POINT('Ctrl Pts',(6.45818362452259,-2.03011647728058,
100.600385099218));
#208123=CARTESIAN_POINT('Ctrl Pts',(6.51348758383214,-1.84500838091116,
100.609452885611));
#208124=CARTESIAN_POINT('Ctrl Pts',(6.56079348986117,-1.65779304600884,
100.618520672003));
#208125=CARTESIAN_POINT('Ctrl Pts',(6.60809939589018,-1.47057771110666,
100.627588458396));
#208126=CARTESIAN_POINT('Ctrl Pts',(6.6474071188378,-1.28125550766004,100.636656244789));
#208127=CARTESIAN_POINT('Ctrl Pts',(6.67855106060494,-1.09052497949047,
100.645724031181));
#208128=CARTESIAN_POINT('Ctrl Pts',(6.70748715722669,-0.913315651490259,
100.654148987314));
#208129=CARTESIAN_POINT('Ctrl Pts',(6.7293634728444,-0.734968394205431,
100.662573943447));
#208130=CARTESIAN_POINT('Ctrl Pts',(6.74411412874157,-0.556069796435935,
100.670998899581));
#208131=CARTESIAN_POINT('Ctrl Pts',(6.75886820840767,-0.377129674583572,
100.679425811227));
#208132=CARTESIAN_POINT('Ctrl Pts',(6.76649330340398,-0.197638287575471,
100.687852722873));
#208133=CARTESIAN_POINT('Ctrl Pts',(6.76697556414859,-0.0181855496434833,
100.69627963452));
#208134=CARTESIAN_POINT('Ctrl Pts',(6.76745800223927,0.161333180051648,
100.70470964507));
#208135=CARTESIAN_POINT('Ctrl Pts',(6.76079236779913,0.340812900886664,
100.71313965562));
#208136=CARTESIAN_POINT('Ctrl Pts',(6.7470169096723,0.519665104270093,100.72156966617));
#208137=CARTESIAN_POINT('Ctrl Pts',(6.73322876188165,0.698682062561421,
100.73000744227));
#208138=CARTESIAN_POINT('Ctrl Pts',(6.71231773072315,0.87707001763686,100.738445218369));
#208139=CARTESIAN_POINT('Ctrl Pts',(6.68437391811377,1.05424585502643,100.746882994469));
#208140=CARTESIAN_POINT('Ctrl Pts',(6.65641543706287,1.23151469666869,100.755325199778));
#208141=CARTESIAN_POINT('Ctrl Pts',(6.62141687123447,1.40756982570475,100.763767405088));
#208142=CARTESIAN_POINT('Ctrl Pts',(6.57951928187132,1.58183912566465,100.772209610398));
#208143=CARTESIAN_POINT('Ctrl Pts',(6.53757749285652,1.75629227014807,100.78066072177));
#208144=CARTESIAN_POINT('Ctrl Pts',(6.48872222670304,1.92895550197544,100.789111833142));
#208145=CARTESIAN_POINT('Ctrl Pts',(6.4331444652841,2.09927160910269,100.797562944514));
#208146=CARTESIAN_POINT('Ctrl Pts',(6.41754648045252,2.14707108838575,100.799934762011));
#208147=CARTESIAN_POINT('Ctrl Pts',(6.40141928934946,2.19468581241639,100.802306579509));
#208148=CARTESIAN_POINT('Ctrl Pts',(6.38476779279114,2.2421037514212,100.804678397006));
#208149=CARTESIAN_POINT('Ctrl Pts',(6.32637599193586,2.40838423207581,100.812995649121));
#208150=CARTESIAN_POINT('Ctrl Pts',(6.26142774917761,2.57254343537232,100.821312901235));
#208151=CARTESIAN_POINT('Ctrl Pts',(6.19009908614766,2.73403772901435,100.82963015335));
#208152=CARTESIAN_POINT('Ctrl Pts',(6.11883292640286,2.89539050978544,100.837940117293));
#208153=CARTESIAN_POINT('Ctrl Pts',(6.04119762702078,3.054082717188,100.846250081235));
#208154=CARTESIAN_POINT('Ctrl Pts',(5.95741817684249,3.20958839514145,100.854560045178));
#208155=CARTESIAN_POINT('Ctrl Pts',(5.87370418750134,3.36497256917197,100.862863516153));
#208156=CARTESIAN_POINT('Ctrl Pts',(5.78385578310677,3.51717487231519,100.871166987129));
#208157=CARTESIAN_POINT('Ctrl Pts',(5.68814498861566,3.66569169304875,100.879470458105));
#208158=CARTESIAN_POINT('Ctrl Pts',(5.59247644153815,3.81414295741967,100.88777026387));
#208159=CARTESIAN_POINT('Ctrl Pts',(5.49095084781472,3.95891168854038,100.896070069636));
#208160=CARTESIAN_POINT('Ctrl Pts',(5.3838851113239,4.09952071687226,100.904369875401));
#208161=CARTESIAN_POINT('Ctrl Pts',(5.27684883973796,4.24009104905559,100.912667397028));
#208162=CARTESIAN_POINT('Ctrl Pts',(5.16427567419766,4.376503683142,100.920964918655));
#208163=CARTESIAN_POINT('Ctrl Pts',(5.04652471368958,4.5083120249291,100.929262440282));
#208164=CARTESIAN_POINT('Ctrl Pts',(4.92878659129806,4.64010599595567,100.937559057249));
#208165=CARTESIAN_POINT('Ctrl Pts',(4.80587203134584,4.76729641639244,100.945855674216));
#208166=CARTESIAN_POINT('Ctrl Pts',(4.6781792560858,4.88947112149448,100.954152291183));
#208167=CARTESIAN_POINT('Ctrl Pts',(4.55044301688451,5.01168741230249,100.962451732145));
#208168=CARTESIAN_POINT('Ctrl Pts',(4.41792556204721,5.12888433361145,100.970751173106));
#208169=CARTESIAN_POINT('Ctrl Pts',(4.28106118001807,5.24068737599776,100.979050614068));
#208170=CARTESIAN_POINT('Ctrl Pts',(4.14417377997452,5.35250922155261,100.987351450839));
#208171=CARTESIAN_POINT('Ctrl Pts',(4.00293826883781,5.4589351645489,100.99565228761));
#208172=CARTESIAN_POINT('Ctrl Pts',(3.85782082818095,5.5596319534348,101.003953124382));
#208173=CARTESIAN_POINT('Ctrl Pts',(3.71259759803485,5.66040214949917,101.012260012399));
#208174=CARTESIAN_POINT('Ctrl Pts',(3.56348707363411,5.75543465319206,101.020566900416));
#208175=CARTESIAN_POINT('Ctrl Pts',(3.41098385638364,5.84443993308941,101.028873788433));
#208176=CARTESIAN_POINT('Ctrl Pts',(3.30850409493752,5.90425008015238,101.034455886422));
#208177=CARTESIAN_POINT('Ctrl Pts',(3.20449288244415,5.96133948118201,101.040037984411));
#208178=CARTESIAN_POINT('Ctrl Pts',(3.09910619832146,6.01563211736934,101.0456200824));
#208179=CARTESIAN_POINT('Ctrl Pts',(3.09910619832142,6.01563211736936,99.0457552630242));
#208180=CARTESIAN_POINT('Ctrl Pts',(2.93375330764834,6.10081787314649,99.0545047109265));
#208181=CARTESIAN_POINT('Ctrl Pts',(2.76488627843078,6.17918207037036,99.0632541588288));
#208182=CARTESIAN_POINT('Ctrl Pts',(2.59307866646709,6.25045854553994,99.0720036067311));
#208183=CARTESIAN_POINT('Ctrl Pts',(2.42127244185378,6.32173444515037,99.0807529839814));
#208184=CARTESIAN_POINT('Ctrl Pts',(2.24652594672461,6.3859226274184,99.0895023612317));
#208185=CARTESIAN_POINT('Ctrl Pts',(2.06943269687111,6.44280508110565,99.098251738482));
#208186=CARTESIAN_POINT('Ctrl Pts',(1.89234081822067,6.49968709436169,99.1070010479874));
#208187=CARTESIAN_POINT('Ctrl Pts',(1.71290249405579,6.54926340459547,99.1157503574927));
#208188=CARTESIAN_POINT('Ctrl Pts',(1.53172716625049,6.59136563150386,99.1244996669981));
#208189=CARTESIAN_POINT('Ctrl Pts',(1.35055318107329,6.63346754640711,99.1332489116653));
#208190=CARTESIAN_POINT('Ctrl Pts',(1.16764249714419,6.66809542395776,99.1419981563325));
#208191=CARTESIAN_POINT('Ctrl Pts',(0.983616340614392,6.69513165624668,
99.1507474009998));
#208192=CARTESIAN_POINT('Ctrl Pts',(0.799591486713875,6.7221676971596,99.1594965837355));
#208193=CARTESIAN_POINT('Ctrl Pts',(0.614451459526745,6.74161215869371,
99.1682457664712));
#208194=CARTESIAN_POINT('Ctrl Pts',(0.428825047910313,6.75339900185712,
99.1769949492069));
#208195=CARTESIAN_POINT('Ctrl Pts',(0.243199888597109,6.7651857655022,99.1857440729174));
#208196=CARTESIAN_POINT('Ctrl Pts',(0.0570886373920129,6.76931499599834,
99.1944931966279));
#208197=CARTESIAN_POINT('Ctrl Pts',(-0.12887662681102,6.76577266947847,
99.2032423203385));
#208198=CARTESIAN_POINT('Ctrl Pts',(-0.314840698187974,6.76223036567994,
99.21199138793));
#208199=CARTESIAN_POINT('Ctrl Pts',(-0.500658497951012,6.75101660879225,
99.2207404555215));
#208200=CARTESIAN_POINT('Ctrl Pts',(-0.685698951925922,6.73216948296221,
99.2294895231131));
#208201=CARTESIAN_POINT('Ctrl Pts',(-0.870738280459596,6.71332247176297,
99.2382385374916));
#208202=CARTESIAN_POINT('Ctrl Pts',(-1.05499998761229,6.6868422135619,99.2469875518701));
#208203=CARTESIAN_POINT('Ctrl Pts',(-1.23785829161402,6.65281863948525,
99.2557365662487));
#208204=CARTESIAN_POINT('Ctrl Pts',(-1.43007412917382,6.61705395368866,
99.2649332999479));
#208205=CARTESIAN_POINT('Ctrl Pts',(-1.62073882535767,6.57295372727796,
99.274130033647));
#208206=CARTESIAN_POINT('Ctrl Pts',(-1.80913696091486,6.52068343478287,
99.2833267673462));
#208207=CARTESIAN_POINT('Ctrl Pts',(-1.98838356186085,6.47095219815207,
99.2920767650599));
#208208=CARTESIAN_POINT('Ctrl Pts',(-2.16557827572506,6.413825868509,99.3008267627736));
#208209=CARTESIAN_POINT('Ctrl Pts',(-2.34011918621674,6.34949849943288,
99.3095767604873));
#208210=CARTESIAN_POINT('Ctrl Pts',(-2.51465655691078,6.28517243495559,
99.3183265807456));
#208211=CARTESIAN_POINT('Ctrl Pts',(-2.68653996295314,6.21364572242381,
99.3270764010039));
#208212=CARTESIAN_POINT('Ctrl Pts',(-2.8551855537998,6.13516132252225,99.3358262212622));
#208213=CARTESIAN_POINT('Ctrl Pts',(-3.02382794858682,6.0566784100051,99.3445758756997));
#208214=CARTESIAN_POINT('Ctrl Pts',(-3.18923239109276,5.97123819492084,
99.3533255301372));
#208215=CARTESIAN_POINT('Ctrl Pts',(-3.35083705967695,5.87913088810715,
99.3620751845747));
#208216=CARTESIAN_POINT('Ctrl Pts',(-3.51243888042392,5.78702520443108,
99.3708246848236));
#208217=CARTESIAN_POINT('Ctrl Pts',(-3.67024081223679,5.68825280605791,
99.3795741850726));
#208218=CARTESIAN_POINT('Ctrl Pts',(-3.82370687544386,5.58314917682515,
99.3883236853216));
#208219=CARTESIAN_POINT('Ctrl Pts',(-3.97717043817807,5.47804726008027,
99.397073043012));
#208220=CARTESIAN_POINT('Ctrl Pts',(-4.1262980372246,5.36661448084237,99.4058224007025));
#208221=CARTESIAN_POINT('Ctrl Pts',(-4.27058317206914,5.24922931204571,
99.414571758393));
#208222=CARTESIAN_POINT('Ctrl Pts',(-4.41486614774825,5.13184589986798,
99.423320985153));
#208223=CARTESIAN_POINT('Ctrl Pts',(-4.55430658194389,5.00851045723056,
99.4320702119131));
#208224=CARTESIAN_POINT('Ctrl Pts',(-4.68843089001807,4.87964187103156,
99.4408194386731));
#208225=CARTESIAN_POINT('Ctrl Pts',(-4.82255336917816,4.75077504207982,
99.4495685461291));
#208226=CARTESIAN_POINT('Ctrl Pts',(-4.9513596606513,4.61637541908099,99.458317653585));
#208227=CARTESIAN_POINT('Ctrl Pts',(-5.07441230869255,4.47689945401832,
99.4670667610409));
#208228=CARTESIAN_POINT('Ctrl Pts',(-5.197463442264,4.33742520555534,99.4758157608173));
#208229=CARTESIAN_POINT('Ctrl Pts',(-5.31476088454725,4.19287495491389,
99.4845647605936));
#208230=CARTESIAN_POINT('Ctrl Pts',(-5.42590627628788,4.04373961586794,
99.49331376037));
#208231=CARTESIAN_POINT('Ctrl Pts',(-5.53706380672606,3.89458798906821,
99.5020637156647));
#208232=CARTESIAN_POINT('Ctrl Pts',(-5.64206777071807,3.74085050155371,
99.5108136709594));
#208233=CARTESIAN_POINT('Ctrl Pts',(-5.74056148163954,3.58304938223247,
99.5195636262541));
#208234=CARTESIAN_POINT('Ctrl Pts',(-5.83905138951829,3.42525435593374,
99.5283132436952));
#208235=CARTESIAN_POINT('Ctrl Pts',(-5.93103139557598,3.26339625497282,
99.5370628611363));
#208236=CARTESIAN_POINT('Ctrl Pts',(-6.01618907820792,3.0980248506511,99.5458124785774));
#208237=CARTESIAN_POINT('Ctrl Pts',(-6.10134392544938,2.93265895249735,
99.5545618046933));
#208238=CARTESIAN_POINT('Ctrl Pts',(-6.17967677261795,2.76378023986118,
99.5633111308091));
#208239=CARTESIAN_POINT('Ctrl Pts',(-6.25092157009195,2.59196229227187,
99.572060456925));
#208240=CARTESIAN_POINT('Ctrl Pts',(-6.32216437407727,2.42014915229159,
99.5808095382275));
#208241=CARTESIAN_POINT('Ctrl Pts',(-6.38631941548899,2.24539720662914,
99.5895586195299));
#208242=CARTESIAN_POINT('Ctrl Pts',(-6.44316881037518,2.06829994947745,
99.5983077008324));
#208243=CARTESIAN_POINT('Ctrl Pts',(-6.50002334524556,1.89118668024503,
99.6070575731747));
#208244=CARTESIAN_POINT('Ctrl Pts',(-6.54957082411084,1.71172794807748,
99.6158074455171));
#208245=CARTESIAN_POINT('Ctrl Pts',(-6.59164294296075,1.53053334250379,
99.6245573178594));
#208246=CARTESIAN_POINT('Ctrl Pts',(-6.63371214082135,1.349351316936,99.6333065827144));
#208247=CARTESIAN_POINT('Ctrl Pts',(-6.66830695239698,1.16643393829725,
99.6420558475693));
#208248=CARTESIAN_POINT('Ctrl Pts',(-6.69530988154,0.982402458340209,99.6508051124242));
#208249=CARTESIAN_POINT('Ctrl Pts',(-6.7223141969049,0.798361530946412,
99.6595548264312));
#208250=CARTESIAN_POINT('Ctrl Pts',(-6.74172580829282,0.613206671361964,
99.6683045404382));
#208251=CARTESIAN_POINT('Ctrl Pts',(-6.75347878028182,0.427566795113024,
99.6770542544453));
#208252=CARTESIAN_POINT('Ctrl Pts',(-6.7624899236821,0.285234494205959,
99.6837627642335));
#208253=CARTESIAN_POINT('Ctrl Pts',(-6.76699999999991,0.142617266093883,
99.6904712740217));
#208254=CARTESIAN_POINT('Ctrl Pts',(-6.767,4.25434840218059E-12,99.6971797838099));
#208255=CARTESIAN_POINT('',(-6.76699937651497,0.00290486591272912,99.3028202161581));
#208256=CARTESIAN_POINT('Ctrl Pts',(3.09910619832135,6.0156321173694,98.651562053011));
#208257=CARTESIAN_POINT('Ctrl Pts',(2.94539729005725,6.0948191788526,98.6596893350202));
#208258=CARTESIAN_POINT('Ctrl Pts',(2.78852930422189,6.16817400846309,98.6678166170294));
#208259=CARTESIAN_POINT('Ctrl Pts',(2.62899026849084,6.23543897157052,98.6759438990386));
#208260=CARTESIAN_POINT('Ctrl Pts',(2.4695293027883,6.30267101873633,98.6840672039827));
#208261=CARTESIAN_POINT('Ctrl Pts',(2.3074002266862,6.36381899169876,98.6921905089268));
#208262=CARTESIAN_POINT('Ctrl Pts',(2.14311362026115,6.41867221554826,98.7003138138708));
#208263=CARTESIAN_POINT('Ctrl Pts',(1.97887461140244,6.47350954717125,98.7084347653087));
#208264=CARTESIAN_POINT('Ctrl Pts',(1.81247966450007,6.52205564690004,98.7165557167466));
#208265=CARTESIAN_POINT('Ctrl Pts',(1.64445716343334,6.56414881287991,98.7246766681845));
#208266=CARTESIAN_POINT('Ctrl Pts',(1.47642585951481,6.60624418415908,98.7327980450864));
#208267=CARTESIAN_POINT('Ctrl Pts',(1.30676718520606,6.64188585278288,98.7409194219883));
#208268=CARTESIAN_POINT('Ctrl Pts',(1.13602263220171,6.67096256766035,98.7490407988902));
#208269=CARTESIAN_POINT('Ctrl Pts',(1.03859639247689,6.68755363861527,98.7536748279062));
#208270=CARTESIAN_POINT('Ctrl Pts',(0.940816821740404,6.70200822244948,
98.7583088569221));
#208271=CARTESIAN_POINT('Ctrl Pts',(0.842785732967011,6.71431315983305,
98.7629428859381));
#208272=CARTESIAN_POINT('Ctrl Pts',(0.652723416207684,6.73816992747649,
98.7719273244639));
#208273=CARTESIAN_POINT('Ctrl Pts',(0.461809585811702,6.75393194326004,
98.7809117629898));
#208274=CARTESIAN_POINT('Ctrl Pts',(0.270714710250231,6.76158284321461,
98.7898962015156));
#208275=CARTESIAN_POINT('Ctrl Pts',(0.0792900163384037,6.76924694816587,
98.7988961466462));
#208276=CARTESIAN_POINT('Ctrl Pts',(-0.112316108485565,6.7687719468986,
98.8078960917767));
#208277=CARTESIAN_POINT('Ctrl Pts',(-0.303433843249637,6.76019355512627,
98.8168960369072));
#208278=CARTESIAN_POINT('Ctrl Pts',(-0.495001951861071,6.75159494815355,
98.8259171906394));
#208279=CARTESIAN_POINT('Ctrl Pts',(-0.686079127952757,6.73485475374515,
98.8349383443717));
#208280=CARTESIAN_POINT('Ctrl Pts',(-0.87599853800856,6.71006077181175,
98.8439594981039));
#208281=CARTESIAN_POINT('Ctrl Pts',(-1.06611119256134,6.68524156180626,
98.8529898309312));
#208282=CARTESIAN_POINT('Ctrl Pts',(-1.25506349169075,6.65235222995014,
98.8620201637584));
#208283=CARTESIAN_POINT('Ctrl Pts',(-1.44219783452507,6.61153192581653,
98.8710504965857));
#208284=CARTESIAN_POINT('Ctrl Pts',(-1.62959747486912,6.57065375135901,
98.8800936315784));
#208285=CARTESIAN_POINT('Ctrl Pts',(-1.81517377197393,6.52182217369165,
98.889136766571));
#208286=CARTESIAN_POINT('Ctrl Pts',(-1.99828108366242,6.46522711980615,
98.8981799015637));
#208287=CARTESIAN_POINT('Ctrl Pts',(-2.15835905952878,6.41575000397448,
98.9060856849634));
#208288=CARTESIAN_POINT('Ctrl Pts',(-2.31655017419342,6.36034022230886,
98.9139914683632));
#208289=CARTESIAN_POINT('Ctrl Pts',(-2.47243429729272,6.29915531206928,
98.9218972517629));
#208290=CARTESIAN_POINT('Ctrl Pts',(-2.64305949249448,6.23218449396756,
98.9305506399911));
#208291=CARTESIAN_POINT('Ctrl Pts',(-2.81107101001989,6.15823428901692,
98.9392040282194));
#208292=CARTESIAN_POINT('Ctrl Pts',(-2.9758955243122,6.0775270323034,98.9478574164476));
#208293=CARTESIAN_POINT('Ctrl Pts',(-3.14056781147405,5.99689431446628,
98.956502812658));
#208294=CARTESIAN_POINT('Ctrl Pts',(-3.30205869402704,5.90951712514607,
98.9651482088684));
#208295=CARTESIAN_POINT('Ctrl Pts',(-3.45981536389501,5.81566562379201,
98.9737936050788));
#208296=CARTESIAN_POINT('Ctrl Pts',(-3.62261025037805,5.71881682163369,
98.9827151061212));
#208297=CARTESIAN_POINT('Ctrl Pts',(-3.78142815372573,5.6150734376972,98.9916366071637));
#208298=CARTESIAN_POINT('Ctrl Pts',(-3.93568751515778,5.50478453556823,
99.0005581082061));
#208299=CARTESIAN_POINT('Ctrl Pts',(-4.08488811246321,5.39811243527532,
99.009187038548));
#208300=CARTESIAN_POINT('Ctrl Pts',(-4.22982412733714,5.28531749407164,
99.0178159688899));
#208301=CARTESIAN_POINT('Ctrl Pts',(-4.36999698499979,5.16676062452024,
99.0264448992319));
#208302=CARTESIAN_POINT('Ctrl Pts',(-4.51729884988509,5.04217410847792,
99.0355126856245));
#208303=CARTESIAN_POINT('Ctrl Pts',(-4.65934014354247,4.91122447635432,
99.0445804720172));
#208304=CARTESIAN_POINT('Ctrl Pts',(-4.79557933767625,4.774380359382,99.0536482584098));
#208305=CARTESIAN_POINT('Ctrl Pts',(-4.93181853181004,4.63753624240968,
99.0627160448025));
#208306=CARTESIAN_POINT('Ctrl Pts',(-5.06225532594945,4.49479789249544,
99.0717838311951));
#208307=CARTESIAN_POINT('Ctrl Pts',(-5.1863907628446,4.34668147614708,99.0808516175878));
#208308=CARTESIAN_POINT('Ctrl Pts',(-5.30172603488717,4.20906527564233,
99.089276573721));
#208309=CARTESIAN_POINT('Ctrl Pts',(-5.41157128508455,4.06686703945213,
99.0977015298542));
#208310=CARTESIAN_POINT('Ctrl Pts',(-5.51557045188123,3.92055756115564,
99.1061264859874));
#208311=CARTESIAN_POINT('Ctrl Pts',(-5.61959375788314,3.77421412302436,
99.1145533976339));
#208312=CARTESIAN_POINT('Ctrl Pts',(-5.71776808284151,3.62375781041807,
99.1229803092803));
#208313=CARTESIAN_POINT('Ctrl Pts',(-5.80978040874206,3.46968883362715,
99.1314072209268));
#208314=CARTESIAN_POINT('Ctrl Pts',(-5.90182657115849,3.31556319967287,
99.1398372314768));
#208315=CARTESIAN_POINT('Ctrl Pts',(-5.98770604636861,3.15782253715786,
99.1482672420269));
#208316=CARTESIAN_POINT('Ctrl Pts',(-6.06715133435416,2.99699244010466,
99.156697252577));
#208317=CARTESIAN_POINT('Ctrl Pts',(-6.14666980567764,2.83601418972937,
99.1651350286765));
#208318=CARTESIAN_POINT('Ctrl Pts',(-6.21974210111039,2.67194111643444,
99.173572804776));
#208319=CARTESIAN_POINT('Ctrl Pts',(-6.28614806347648,2.50532064296189,
99.1820105808754));
#208320=CARTESIAN_POINT('Ctrl Pts',(-6.35258888407773,2.3386127060231,99.1904527861854));
#208321=CARTESIAN_POINT('Ctrl Pts',(-6.41235627723871,2.16935501259267,
99.1988949914954));
#208322=CARTESIAN_POINT('Ctrl Pts',(-6.46527952044811,1.99811153904739,
99.2073371968053));
#208323=CARTESIAN_POINT('Ctrl Pts',(-6.51825859476721,1.82668741305946,
99.2157883081774));
#208324=CARTESIAN_POINT('Ctrl Pts',(-6.56437900580895,1.65327364099432,
99.2242394195495));
#208325=CARTESIAN_POINT('Ctrl Pts',(-6.60352056647827,1.47844686346807,
99.2326905309215));
#208326=CARTESIAN_POINT('Ctrl Pts',(-6.61450570610864,1.42938145755646,
99.2350623484185));
#208327=CARTESIAN_POINT('Ctrl Pts',(-6.6249414661072,1.38020480506695,99.2374341659155));
#208328=CARTESIAN_POINT('Ctrl Pts',(-6.63482592045994,1.3309297521631,99.2398059834124));
#208329=CARTESIAN_POINT('Ctrl Pts',(-6.68056170661874,1.10293200922748,
99.2507804827604));
#208330=CARTESIAN_POINT('Ctrl Pts',(-6.71454523216173,0.872555263279585,
99.2617549821083));
#208331=CARTESIAN_POINT('Ctrl Pts',(-6.73658836297482,0.640832449109899,
99.2727294814563));
#208332=CARTESIAN_POINT('Ctrl Pts',(-6.75673488569275,0.42904724584105,
99.2827597263568));
#208333=CARTESIAN_POINT('Ctrl Pts',(-6.76690784226229,0.216137507080814,
99.2927899712574));
#208334=CARTESIAN_POINT('Ctrl Pts',(-6.76699937651497,0.00290486591292295,
99.302820216158));
#208335=CARTESIAN_POINT('Ctrl Pts',(-6.76699937651526,0.0029048652382334,
99.3028202161898));
#208336=CARTESIAN_POINT('Ctrl Pts',(-6.76707461989407,-0.172377585301011,
99.311065323018));
#208337=CARTESIAN_POINT('Ctrl Pts',(-6.7603351851076,-0.3477811383096,99.3193104298461));
#208338=CARTESIAN_POINT('Ctrl Pts',(-6.74677933403267,-0.522740488071986,
99.3275555366743));
#208339=CARTESIAN_POINT('Ctrl Pts',(-6.73323011857456,-0.697614194874938,
99.3357966075058));
#208340=CARTESIAN_POINT('Ctrl Pts',(-6.71287116233085,-0.872043779040175,
99.3440376783373));
#208341=CARTESIAN_POINT('Ctrl Pts',(-6.68575278601598,-1.04546577384418,
99.3522787491688));
#208342=CARTESIAN_POINT('Ctrl Pts',(-6.65758548255101,-1.22559565693259,
99.360838581081));
#208343=CARTESIAN_POINT('Ctrl Pts',(-6.62212542119759,-1.4046380490682,
99.3693984129932));
#208344=CARTESIAN_POINT('Ctrl Pts',(-6.57948809993647,-1.58196881852786,
99.3779582449054));
#208345=CARTESIAN_POINT('Ctrl Pts',(-6.53844634137191,-1.75266356226325,
99.3861977530242));
#208346=CARTESIAN_POINT('Ctrl Pts',(-6.49075486168368,-1.92177210105994,
99.394437261143));
#208347=CARTESIAN_POINT('Ctrl Pts',(-6.43656847215185,-2.08874969857588,
99.4026767692618));
#208348=CARTESIAN_POINT('Ctrl Pts',(-6.38237508461469,-2.25574886073428,
99.4109173414876));
#208349=CARTESIAN_POINT('Ctrl Pts',(-6.3216852249945,-2.42061619582955,
99.4191579137135));
#208350=CARTESIAN_POINT('Ctrl Pts',(-6.25470312132414,-2.58282362233624,
99.4273984859394));
#208351=CARTESIAN_POINT('Ctrl Pts',(-6.18770057383033,-2.74508055669367,
99.4356415732969));
#208352=CARTESIAN_POINT('Ctrl Pts',(-6.11440209114554,-2.90467563728018,
99.4438846606543));
#208353=CARTESIAN_POINT('Ctrl Pts',(-6.03505947804925,-3.06110210486484,
99.4521277480118));
#208354=CARTESIAN_POINT('Ctrl Pts',(-5.95567867843879,-3.21760385836821,
99.4603748026544));
#208355=CARTESIAN_POINT('Ctrl Pts',(-5.8702481127369,-3.3709336445959,99.468621857297));
#208356=CARTESIAN_POINT('Ctrl Pts',(-5.77906487104334,-3.5206104891443,
99.4768689119396));
#208357=CARTESIAN_POINT('Ctrl Pts',(-5.68777422208742,-3.67046364218768,
99.485125681016));
#208358=CARTESIAN_POINT('Ctrl Pts',(-5.59071754823313,-3.81665495715636,
99.4933824500924));
#208359=CARTESIAN_POINT('Ctrl Pts',(-5.48823504557674,-3.95873276245105,
99.5016392191688));
#208360=CARTESIAN_POINT('Ctrl Pts',(-5.38568136729878,-4.1009092428936,
99.509901722694));
#208361=CARTESIAN_POINT('Ctrl Pts',(-5.27769456590132,-4.23896624024573,
99.5181642262193));
#208362=CARTESIAN_POINT('Ctrl Pts',(-5.164654200136,-4.37248624846524,99.5264267297445));
#208363=CARTESIAN_POINT('Ctrl Pts',(-5.05146025447411,-4.50618766081338,
99.5347004589451));
#208364=CARTESIAN_POINT('Ctrl Pts',(-4.93319927158584,-4.63533951395193,
99.5429741881455));
#208365=CARTESIAN_POINT('Ctrl Pts',(-4.8102872529871,-4.75956148649745,
99.551247917346));
#208366=CARTESIAN_POINT('Ctrl Pts',(-4.77826432266308,-4.79192570617986,
99.5534035165847));
#208367=CARTESIAN_POINT('Ctrl Pts',(-4.74592585773266,-4.82395550698373,
99.5555591158233));
#208368=CARTESIAN_POINT('Ctrl Pts',(-4.7132795673047,-4.85564462460218,
99.5577147150619));
#208369=CARTESIAN_POINT('Ctrl Pts',(-4.59106272309898,-4.97427813242865,
99.5657845610646));
#208370=CARTESIAN_POINT('Ctrl Pts',(-4.464138191083,-5.08851333835254,99.5738544070674));
#208371=CARTESIAN_POINT('Ctrl Pts',(-4.33286015346576,-5.19794304417706,
99.5819242530702));
#208372=CARTESIAN_POINT('Ctrl Pts',(-4.20174728031799,-5.30723507351254,
99.5899839461802));
#208373=CARTESIAN_POINT('Ctrl Pts',(-4.06629208274724,-5.41173339663901,
99.5980436392903));
#208374=CARTESIAN_POINT('Ctrl Pts',(-3.92688715996402,-5.51106579827439,
99.6061033324003));
#208375=CARTESIAN_POINT('Ctrl Pts',(-3.78762703133491,-5.61029502743362,
99.6141546542389));
#208376=CARTESIAN_POINT('Ctrl Pts',(-3.64442564260747,-5.70436879809481,
99.6222059760775));
#208377=CARTESIAN_POINT('Ctrl Pts',(-3.49771033363369,-5.79295360088376,
99.6302572979162));
#208378=CARTESIAN_POINT('Ctrl Pts',(-3.35111526148789,-5.88146580623371,
99.6383020214972));
#208379=CARTESIAN_POINT('Ctrl Pts',(-3.20101231847573,-5.96449780500423,
99.6463467450782));
#208380=CARTESIAN_POINT('Ctrl Pts',(-3.04785954378699,-6.04175812171809,
99.6543914686593));
#208381=CARTESIAN_POINT('Ctrl Pts',(-2.89479875637982,-6.11897203400657,
99.6624313603837));
#208382=CARTESIAN_POINT('Ctrl Pts',(-2.73869211612158,-6.19042099757312,
99.6704712521081));
#208383=CARTESIAN_POINT('Ctrl Pts',(-2.5800239983328,-6.25585846771063,
99.6785111438325));
#208384=CARTESIAN_POINT('Ctrl Pts',(-2.41793932126784,-6.32270498585807,
99.6867241564524));
#208385=CARTESIAN_POINT('Ctrl Pts',(-2.2531819452021,-6.38327797982675,
99.6949371690724));
#208386=CARTESIAN_POINT('Ctrl Pts',(-2.08629218611878,-6.43736544823577,
99.7031501816923));
#208387=CARTESIAN_POINT('Ctrl Pts',(-1.92297727368812,-6.49029434102904,
99.7111872682349));
#208388=CARTESIAN_POINT('Ctrl Pts',(-1.75762077966772,-6.5370126314901,
99.7192243547775));
#208389=CARTESIAN_POINT('Ctrl Pts',(-1.59074623467904,-6.57737146714814,
99.7272614413201));
#208390=CARTESIAN_POINT('Ctrl Pts',(-1.42385571901983,-6.61773416533457,
99.7352992970492));
#208391=CARTESIAN_POINT('Ctrl Pts',(-1.25544722624345,-6.65173610887908,
99.7433371527784));
#208392=CARTESIAN_POINT('Ctrl Pts',(-1.08605603557982,-6.67927924910919,
99.7513750085075));
#208393=CARTESIAN_POINT('Ctrl Pts',(-0.916615071340223,-6.70683048256173,
99.7594152260645));
#208394=CARTESIAN_POINT('Ctrl Pts',(-0.746191203033471,-6.72791907518196,
99.7674554436214));
#208395=CARTESIAN_POINT('Ctrl Pts',(-0.575326261399993,-6.74249869803054,
99.7754956611784));
#208396=CARTESIAN_POINT('Ctrl Pts',(-0.398005932795349,-6.75762914837177,
99.7838396433062));
#208397=CARTESIAN_POINT('Ctrl Pts',(-0.220210995243738,-6.76574915837271,
99.7921836254339));
#208398=CARTESIAN_POINT('Ctrl Pts',(-0.0425475252329801,-6.76686623985553,
99.8005276075617));
#208399=CARTESIAN_POINT('Ctrl Pts',(0.128946101418613,-6.76794452766981,
99.8085818223968));
#208400=CARTESIAN_POINT('Ctrl Pts',(0.300316872996476,-6.76249820220135,
99.8166360372318));
#208401=CARTESIAN_POINT('Ctrl Pts',(0.471025049325828,-6.75058696728719,
99.8246902520669));
#208402=CARTESIAN_POINT('Ctrl Pts',(0.641860972496963,-6.73866681878332,
99.8327504941499));
#208403=CARTESIAN_POINT('Ctrl Pts',(0.812032944247111,-6.72027216779632,
99.8408107362329));
#208404=CARTESIAN_POINT('Ctrl Pts',(0.98101087477628,-6.69551392079583,
99.8488709783159));
#208405=CARTESIAN_POINT('Ctrl Pts',(1.15022504804352,-6.67072106006771,
99.8569424891702));
#208406=CARTESIAN_POINT('Ctrl Pts',(1.31824148558976,-6.63954692029786,
99.8650140000246));
#208407=CARTESIAN_POINT('Ctrl Pts',(1.48454415714527,-6.60215250092618,
99.8730855108789));
#208408=CARTESIAN_POINT('Ctrl Pts',(1.50197441346389,-6.59823317534688,
99.8739314894898));
#208409=CARTESIAN_POINT('Ctrl Pts',(1.51938586122411,-6.59424556237967,
99.8747774681007));
#208410=CARTESIAN_POINT('Ctrl Pts',(1.53677791905461,-6.59018987795543,
99.8756234467116));
#208411=CARTESIAN_POINT('Ctrl Pts',(1.70595901354953,-6.55073824224293,
99.8838526964476));
#208412=CARTESIAN_POINT('Ctrl Pts',(1.87386854883584,-6.50470971120342,
99.8920819461835));
#208413=CARTESIAN_POINT('Ctrl Pts',(2.0399568793622,-6.45219845714179,99.9003111959195));
#208414=CARTESIAN_POINT('Ctrl Pts',(2.20584753775609,-6.39974970001499,
99.9085306515096));
#208415=CARTESIAN_POINT('Ctrl Pts',(2.36992096880443,-6.34083369006769,
99.9167501070996));
#208416=CARTESIAN_POINT('Ctrl Pts',(2.53163761468347,-6.27559558830234,
99.9249695626897));
#208417=CARTESIAN_POINT('Ctrl Pts',(2.69319426812721,-6.21042202907508,
99.9331808864594));
#208418=CARTESIAN_POINT('Ctrl Pts',(2.85239844952946,-6.13893896731954,
99.941392210229));
#208419=CARTESIAN_POINT('Ctrl Pts',(3.00872558727029,-6.06134138128723,
99.9496035339987));
#208420=CARTESIAN_POINT('Ctrl Pts',(3.16492944760644,-5.98380498763109,
99.9578083824328));
#208421=CARTESIAN_POINT('Ctrl Pts',(3.31826046338572,-5.90016383237433,
99.9660132308668));
#208422=CARTESIAN_POINT('Ctrl Pts',(3.46821380881486,-5.8106610619056,99.9742180793009));
#208423=CARTESIAN_POINT('Ctrl Pts',(3.61807899879668,-5.7212109088476,99.9824181042208));
#208424=CARTESIAN_POINT('Ctrl Pts',(3.76457016697336,-5.62590618859519,
99.9906181291407));
#208425=CARTESIAN_POINT('Ctrl Pts',(3.90720680747295,-5.52503610518855,
99.9988181540606));
#208426=CARTESIAN_POINT('Ctrl Pts',(4.04980216569743,-5.4241952158692,100.007015805707));
#208427=CARTESIAN_POINT('Ctrl Pts',(4.18854492360851,-5.31779237537217,
100.015213457354));
#208428=CARTESIAN_POINT('Ctrl Pts',(4.32298310791889,-5.20616039405702,
100.023411109001));
#208429=CARTESIAN_POINT('Ctrl Pts',(4.45740329013162,-5.09454336094902,
100.031607662932));
#208430=CARTESIAN_POINT('Ctrl Pts',(4.58751977028578,-4.97769881004729,
100.039804216864));
#208431=CARTESIAN_POINT('Ctrl Pts',(4.71291325768196,-4.85600016737702,
100.048000770795));
#208432=CARTESIAN_POINT('Ctrl Pts',(4.83831275391542,-4.73429569292587,
100.056197717503));
#208433=CARTESIAN_POINT('Ctrl Pts',(4.95898854899892,-4.60773691312512,
100.064394664212));
#208434=CARTESIAN_POINT('Ctrl Pts',(5.07455783015735,-4.47673450501464,
100.072591610921));
#208435=CARTESIAN_POINT('Ctrl Pts',(5.19015366282928,-4.34570199970038,
100.08079044084));
#208436=CARTESIAN_POINT('Ctrl Pts',(5.30064040763602,-4.21022410171465,
100.08898927076));
#208437=CARTESIAN_POINT('Ctrl Pts',(5.40567517013402,-4.07074501227926,
100.09718810068));
#208438=CARTESIAN_POINT('Ctrl Pts',(5.51080941398005,-3.93113381831479,
100.10539469594));
#208439=CARTESIAN_POINT('Ctrl Pts',(5.61048114277883,-3.78751414850098,
100.1136012912));
#208440=CARTESIAN_POINT('Ctrl Pts',(5.70438996117341,-3.64036044518452,
100.121807886459));
#208441=CARTESIAN_POINT('Ctrl Pts',(5.79834423197477,-3.49313551863154,
100.130018453758));
#208442=CARTESIAN_POINT('Ctrl Pts',(5.88652985018573,-3.34237345774138,
100.138229021057));
#208443=CARTESIAN_POINT('Ctrl Pts',(5.96869219956712,-3.18857372924426,
100.146439588356));
#208444=CARTESIAN_POINT('Ctrl Pts',(6.05096786259049,-3.0345618889039,100.154661479203));
#208445=CARTESIAN_POINT('Ctrl Pts',(6.12720349859119,-2.87750433127488,
100.16288337005));
#208446=CARTESIAN_POINT('Ctrl Pts',(6.1971919971014,-2.71792206493535,100.171105260896));
#208447=CARTESIAN_POINT('Ctrl Pts',(6.26082805960978,-2.57282412324239,
100.178580900051));
#208448=CARTESIAN_POINT('Ctrl Pts',(6.31930008812324,-2.42563940340715,
100.186056539206));
#208449=CARTESIAN_POINT('Ctrl Pts',(6.37248835238525,-2.27676990464875,
100.193532178361));
#208450=CARTESIAN_POINT('Ctrl Pts',(6.43606650427784,-2.09881998025171,
100.202468121812));
#208451=CARTESIAN_POINT('Ctrl Pts',(6.49222727935702,-1.91809214767458,
100.211404065263));
#208452=CARTESIAN_POINT('Ctrl Pts',(6.54074678974077,-1.73520040124931,
100.220340008713));
#208453=CARTESIAN_POINT('Ctrl Pts',(6.58919336243151,-1.55258358962758,
100.229262519071));
#208454=CARTESIAN_POINT('Ctrl Pts',(6.63002152457474,-1.36780960388155,
100.238185029429));
#208455=CARTESIAN_POINT('Ctrl Pts',(6.66305689940416,-1.18150825443693,
100.247107539786));
#208456=CARTESIAN_POINT('Ctrl Pts',(6.69601132731341,-0.995663401113205,
100.256008187225));
#208457=CARTESIAN_POINT('Ctrl Pts',(6.7212110326332,-0.808298907264183,
100.264908834663));
#208458=CARTESIAN_POINT('Ctrl Pts',(6.7385325561776,-0.620054827684308,
100.273809482101));
#208459=CARTESIAN_POINT('Ctrl Pts',(6.75582731144526,-0.432101656095412,
100.282696374687));
#208460=CARTESIAN_POINT('Ctrl Pts',(6.76526814684622,-0.243271866040026,
100.291583267274));
#208461=CARTESIAN_POINT('Ctrl Pts',(6.76678283078964,-0.05421365999973,
100.30047015986));
#208462=CARTESIAN_POINT('Ctrl Pts',(6.76829362142991,0.134358595876913,
100.309334209815));
#208463=CARTESIAN_POINT('Ctrl Pts',(6.76191891179613,0.323157838770076,
100.31819825977));
#208464=CARTESIAN_POINT('Ctrl Pts',(6.74763828243208,0.511533585854418,
100.327062309725));
#208465=CARTESIAN_POINT('Ctrl Pts',(6.73398485196275,0.691635953849492,
100.335537054545));
#208466=CARTESIAN_POINT('Ctrl Pts',(6.71310500021671,0.871350964271029,
100.344011799366));
#208467=CARTESIAN_POINT('Ctrl Pts',(6.68502535051704,1.05010716736179,100.352486544186));
#208468=CARTESIAN_POINT('Ctrl Pts',(6.65782648536332,1.22325625986319,100.360695458615));
#208469=CARTESIAN_POINT('Ctrl Pts',(6.62389767383333,1.39533869462894,100.368904373044));
#208470=CARTESIAN_POINT('Ctrl Pts',(6.58335427138304,1.56580188320958,100.377113287473));
#208471=CARTESIAN_POINT('Ctrl Pts',(6.54280122994474,1.73630559854754,100.38532415353));
#208472=CARTESIAN_POINT('Ctrl Pts',(6.49563054694887,1.90518895431156,100.393535019587));
#208473=CARTESIAN_POINT('Ctrl Pts',(6.44200800525192,2.07191260922613,100.401745885644));
#208474=CARTESIAN_POINT('Ctrl Pts',(6.3883631566255,2.23870562103226,100.409960167414));
#208475=CARTESIAN_POINT('Ctrl Pts',(6.32826121120446,2.40333680341831,100.418174449183));
#208476=CARTESIAN_POINT('Ctrl Pts',(6.2619168459761,2.56528486022132,100.426388730953));
#208477=CARTESIAN_POINT('Ctrl Pts',(6.19549780492688,2.72741520234786,100.434612258545));
#208478=CARTESIAN_POINT('Ctrl Pts',(6.12282244519839,2.88685605718566,100.442835786138));
#208479=CARTESIAN_POINT('Ctrl Pts',(6.04415276581908,3.04310800719291,100.45105931373));
#208480=CARTESIAN_POINT('Ctrl Pts',(5.96543266223536,3.19946010862227,100.459288112284));
#208481=CARTESIAN_POINT('Ctrl Pts',(5.88071075187738,3.3526189199293,100.467516910838));
#208482=CARTESIAN_POINT('Ctrl Pts',(5.79029344738274,3.50211233303509,100.475745709391));
#208483=CARTESIAN_POINT('Ctrl Pts',(5.69975169070402,3.65181151186097,100.483985834228));
#208484=CARTESIAN_POINT('Ctrl Pts',(5.60349907709188,3.79783491887417,100.492225959064));
#208485=CARTESIAN_POINT('Ctrl Pts',(5.50188410796304,3.93974114156549,100.500466083901));
#208486=CARTESIAN_POINT('Ctrl Pts',(5.45677125516429,4.00274164818753,100.504124359271));
#208487=CARTESIAN_POINT('Ctrl Pts',(5.41060200277377,4.06493111563783,100.507782634641));
#208488=CARTESIAN_POINT('Ctrl Pts',(5.36340923191248,4.12627318667051,100.511440910011));
#208489=CARTESIAN_POINT('Ctrl Pts',(5.25442051244402,4.26793881997365,100.5198894656));
#208490=CARTESIAN_POINT('Ctrl Pts',(5.13972092806317,4.4054066894299,100.52833802119));
#208491=CARTESIAN_POINT('Ctrl Pts',(5.01965932110736,4.53820551540144,100.536786576779));
#208492=CARTESIAN_POINT('Ctrl Pts',(4.89970465433643,4.67088605600797,100.545227607148));
#208493=CARTESIAN_POINT('Ctrl Pts',(4.77439770683847,4.79890559577125,100.553668637516));
#208494=CARTESIAN_POINT('Ctrl Pts',(4.6441281338455,4.92182515703521,100.562109667885));
#208495=CARTESIAN_POINT('Ctrl Pts',(4.51397820040631,5.04463182899492,100.570542946013));
#208496=CARTESIAN_POINT('Ctrl Pts',(4.37887497366288,5.16234763637225,100.578976224141));
#208497=CARTESIAN_POINT('Ctrl Pts',(4.23924560992898,5.27456971313281,100.587409502268));
#208498=CARTESIAN_POINT('Ctrl Pts',(4.09969275739106,5.38673029677273,100.595838159304));
#208499=CARTESIAN_POINT('Ctrl Pts',(3.95561897013448,5.49340294114936,100.604266816339));
#208500=CARTESIAN_POINT('Ctrl Pts',(3.80748577284527,5.5942239041337,100.612695473375));
#208501=CARTESIAN_POINT('Ctrl Pts',(3.65942011893495,5.69499889640635,100.621120287247));
#208502=CARTESIAN_POINT('Ctrl Pts',(3.50729902106169,5.78992734033334,100.62954510112));
#208503=CARTESIAN_POINT('Ctrl Pts',(3.35161460815422,5.87868765273401,100.637969914993));
#208504=CARTESIAN_POINT('Ctrl Pts',(3.2684356934009,5.92611042499985,100.642471116249));
#208505=CARTESIAN_POINT('Ctrl Pts',(3.18424012333501,5.97177320619438,100.646972317505));
#208506=CARTESIAN_POINT('Ctrl Pts',(3.09910619832147,6.01563211736933,100.651473518761));
#208507=CARTESIAN_POINT('Origin',(0.,0.,4.30282021618968));
#208508=CARTESIAN_POINT('',(3.09910619832139,6.01563211736937,103.045799558392));
#208509=CARTESIAN_POINT('',(3.09910619832148,6.01563211736933,102.651395695404));
#208510=CARTESIAN_POINT('',(3.09910619832133,6.0156321173694,4.30282021618968));
#208511=CARTESIAN_POINT('',(-6.76699760869595,-0.00568892813878999,101.69717978384));
#208512=CARTESIAN_POINT('Ctrl Pts',(-6.76699760869595,-0.00568892813878413,
101.69717978384));
#208513=CARTESIAN_POINT('Ctrl Pts',(-6.76680510301031,-0.234675036349317,
101.707957090383));
#208514=CARTESIAN_POINT('Ctrl Pts',(-6.75498606488932,-0.463202034117518,
101.718734396925));
#208515=CARTESIAN_POINT('Ctrl Pts',(-6.73170191760452,-0.690274070583281,
101.729511703468));
#208516=CARTESIAN_POINT('Ctrl Pts',(-6.71089442214133,-0.893193263233427,
101.739142666297));
#208517=CARTESIAN_POINT('Ctrl Pts',(-6.68093182727304,-1.09495111148143,
101.748773629126));
#208518=CARTESIAN_POINT('Ctrl Pts',(-6.64196113402566,-1.29485184252585,
101.758404591954));
#208519=CARTESIAN_POINT('Ctrl Pts',(-6.6058027646821,-1.48032671769085,
101.767340535405));
#208520=CARTESIAN_POINT('Ctrl Pts',(-6.56184811814019,-1.6644043403748,
101.776276478856));
#208521=CARTESIAN_POINT('Ctrl Pts',(-6.51021806817828,-1.84644244555986,
101.785212422307));
#208522=CARTESIAN_POINT('Ctrl Pts',(-6.45866563187552,-2.02820689919009,
101.794134932664));
#208523=CARTESIAN_POINT('Ctrl Pts',(-6.39946088504986,-2.20793770507951,
101.803057443022));
#208524=CARTESIAN_POINT('Ctrl Pts',(-6.33277535008608,-2.38500426945995,
101.811979953379));
#208525=CARTESIAN_POINT('Ctrl Pts',(-6.26625321537738,-2.56163696580885,
101.820880600818));
#208526=CARTESIAN_POINT('Ctrl Pts',(-6.19228696729786,-2.73561820861534,
101.829781248256));
#208527=CARTESIAN_POINT('Ctrl Pts',(-6.11109714232497,-2.90633458450117,
101.838681895694));
#208528=CARTESIAN_POINT('Ctrl Pts',(-6.03003278620595,-3.07678713929827,
101.847568788281));
#208529=CARTESIAN_POINT('Ctrl Pts',(-5.94176723108616,-3.2439846595089,
101.856455680867));
#208530=CARTESIAN_POINT('Ctrl Pts',(-5.84656922391986,-3.40733287336491,
101.865342573453));
#208531=CARTESIAN_POINT('Ctrl Pts',(-5.7516159111686,-3.57026122133477,
101.874206623408));
#208532=CARTESIAN_POINT('Ctrl Pts',(-5.64976583255248,-3.72935978363406,
101.883070673363));
#208533=CARTESIAN_POINT('Ctrl Pts',(-5.5413334533065,-3.88405877392017,
101.891934723318));
#208534=CARTESIAN_POINT('Ctrl Pts',(-5.43766337596293,-4.03196345331075,
101.900409468139));
#208535=CARTESIAN_POINT('Ctrl Pts',(-5.32797686686972,-4.17584647143222,
101.908884212959));
#208536=CARTESIAN_POINT('Ctrl Pts',(-5.21258850367004,-4.31523001604862,
101.91735895778));
#208537=CARTESIAN_POINT('Ctrl Pts',(-5.10081956906823,-4.45024146651733,
101.925567872209));
#208538=CARTESIAN_POINT('Ctrl Pts',(-4.98380786530573,-4.58090052586389,
101.933776786638));
#208539=CARTESIAN_POINT('Ctrl Pts',(-4.86193464529849,-4.70679089240708,
101.941985701067));
#208540=CARTESIAN_POINT('Ctrl Pts',(-4.74003245055219,-4.83271118874552,
101.950196567124));
#208541=CARTESIAN_POINT('Ctrl Pts',(-4.61326668455911,-4.95386027772515,
101.958407433181));
#208542=CARTESIAN_POINT('Ctrl Pts',(-4.48205520208169,-5.06985898871877,
101.966618299238));
#208543=CARTESIAN_POINT('Ctrl Pts',(-4.35078913574405,-5.18590595507318,
101.974832581007));
#208544=CARTESIAN_POINT('Ctrl Pts',(-4.21507393505767,-5.29679803937224,
101.983046862777));
#208545=CARTESIAN_POINT('Ctrl Pts',(-4.075360289141,-5.4021965452668,101.991261144547));
#208546=CARTESIAN_POINT('Ctrl Pts',(-3.93548938448625,-5.50771368550037,
101.999484672139));
#208547=CARTESIAN_POINT('Ctrl Pts',(-3.79161132986243,-5.6077246823996,
102.007708199732));
#208548=CARTESIAN_POINT('Ctrl Pts',(-3.64420634014303,-5.70193380796913,
102.015931727324));
#208549=CARTESIAN_POINT('Ctrl Pts',(-3.49670686955903,-5.79620331792358,
102.024160525878));
#208550=CARTESIAN_POINT('Ctrl Pts',(-3.34567626392025,-5.88466336391086,
102.032389324431));
#208551=CARTESIAN_POINT('Ctrl Pts',(-3.19161899078301,-5.96706437183924,
102.040618122985));
#208552=CARTESIAN_POINT('Ctrl Pts',(-3.03734967013756,-6.04957879816098,
102.048858247822));
#208553=CARTESIAN_POINT('Ctrl Pts',(-2.8800456801906,-6.12601737330258,
102.057098372658));
#208554=CARTESIAN_POINT('Ctrl Pts',(-2.72023201364944,-6.19617840220218,
102.065338497494));
#208555=CARTESIAN_POINT('Ctrl Pts',(-2.64928134097196,-6.22732700359471,
102.068996772864));
#208556=CARTESIAN_POINT('Ctrl Pts',(-2.57783622507843,-6.25723896011439,
102.072655048234));
#208557=CARTESIAN_POINT('Ctrl Pts',(-2.50594349886725,-6.28589979084021,
102.076313323604));
#208558=CARTESIAN_POINT('Ctrl Pts',(-2.33992226588979,-6.35208599222701,
102.084761346367));
#208559=CARTESIAN_POINT('Ctrl Pts',(-2.17113314524973,-6.4117482900346,
102.093209369129));
#208560=CARTESIAN_POINT('Ctrl Pts',(-2.00011656487015,-6.4646595213462,
102.101657391892));
#208561=CARTESIAN_POINT('Ctrl Pts',(-1.82925658948067,-6.51752230026307,
102.110097678548));
#208562=CARTESIAN_POINT('Ctrl Pts',(-1.65617353726104,-6.56364623744236,
102.118537965203));
#208563=CARTESIAN_POINT('Ctrl Pts',(-1.48142639746172,-6.60285277958729,
102.126978251859));
#208564=CARTESIAN_POINT('Ctrl Pts',(-1.30681237749751,-6.64202945475739,
102.135412108827));
#208565=CARTESIAN_POINT('Ctrl Pts',(-1.13053712135248,-6.67429916704483,
102.143845965795));
#208566=CARTESIAN_POINT('Ctrl Pts',(-0.953173699982523,-6.69953348358389,
102.152279822763));
#208567=CARTESIAN_POINT('Ctrl Pts',(-0.775918124780594,-6.72475245634845,
102.160708551508));
#208568=CARTESIAN_POINT('Ctrl Pts',(-0.59757603289914,-6.74294451546294,
102.169137280253));
#208569=CARTESIAN_POINT('Ctrl Pts',(-0.41872997723262,-6.75403244041415,
102.177566008998));
#208570=CARTESIAN_POINT('Ctrl Pts',(-0.239965205135707,-6.76511532602516,
102.185990906978));
#208571=CARTESIAN_POINT('Ctrl Pts',(-0.0606972582868748,-6.76910049502238,
102.194415804958));
#208572=CARTESIAN_POINT('Ctrl Pts',(0.118486509143059,-6.76596260314459,
102.202840702939));
#208573=CARTESIAN_POINT('Ctrl Pts',(0.297630604995052,-6.76282540600117,
102.211263735633));
#208574=CARTESIAN_POINT('Ctrl Pts',(0.476690225396251,-6.75256829552415,
102.219686768327));
#208575=CARTESIAN_POINT('Ctrl Pts',(0.655077796231265,-6.73521804256438,
102.228109801021));
#208576=CARTESIAN_POINT('Ctrl Pts',(0.833445182715354,-6.71786975276603,
102.236531880659));
#208577=CARTESIAN_POINT('Ctrl Pts',(1.01114033938551,-6.69342995274387,
102.244953960296));
#208578=CARTESIAN_POINT('Ctrl Pts',(1.18758027650778,-6.66197734061365,
102.253376039934));
#208579=CARTESIAN_POINT('Ctrl Pts',(1.36402487934886,-6.63052389676105,
102.261798342282));
#208580=CARTESIAN_POINT('Ctrl Pts',(1.53921386823527,-6.59205732997234,
102.270220644631));
#208581=CARTESIAN_POINT('Ctrl Pts',(1.71257354881077,-6.5467076336059,102.278642946979));
#208582=CARTESIAN_POINT('Ctrl Pts',(1.88596201477482,-6.50135040718041,
102.287066647803));
#208583=CARTESIAN_POINT('Ctrl Pts',(2.05752024442653,-6.4491078575326,102.295490348626));
#208584=CARTESIAN_POINT('Ctrl Pts',(2.22668847037332,-6.39016020580913,
102.30391404945));
#208585=CARTESIAN_POINT('Ctrl Pts',(2.39597117400493,-6.33117266367091,
102.312343450669));
#208586=CARTESIAN_POINT('Ctrl Pts',(2.5628603268792,-6.26547106246991,102.320772851888));
#208587=CARTESIAN_POINT('Ctrl Pts',(2.72681400159689,-6.19328462132132,
102.329202253107));
#208588=CARTESIAN_POINT('Ctrl Pts',(2.8908261747581,-6.12107242415075,102.337634661924));
#208589=CARTESIAN_POINT('Ctrl Pts',(3.05190047865451,-6.04237091346222,
102.346067070742));
#208590=CARTESIAN_POINT('Ctrl Pts',(3.20951794893678,-5.95745612954495,
102.35449947956));
#208591=CARTESIAN_POINT('Ctrl Pts',(3.36728125148852,-5.87246277999895,
102.362939690287));
#208592=CARTESIAN_POINT('Ctrl Pts',(3.52158103934015,-5.78124483501094,
102.371379901015));
#208593=CARTESIAN_POINT('Ctrl Pts',(3.67192482994536,-5.68412324314232,
102.379820111743));
#208594=CARTESIAN_POINT('Ctrl Pts',(3.75743781255772,-5.62888213898156,
102.38462075958));
#208595=CARTESIAN_POINT('Ctrl Pts',(3.84167150762846,-5.57173191324348,
102.389421407417));
#208596=CARTESIAN_POINT('Ctrl Pts',(3.92453983275924,-5.51273762309491,
102.394222055254));
#208597=CARTESIAN_POINT('Ctrl Pts',(4.06504681737886,-5.41271014208249,
102.402361770287));
#208598=CARTESIAN_POINT('Ctrl Pts',(4.20190682985241,-5.30717939374251,
102.41050148532));
#208599=CARTESIAN_POINT('Ctrl Pts',(4.33465777230064,-5.19644407234733,
102.418641200352));
#208600=CARTESIAN_POINT('Ctrl Pts',(4.46729261157105,-5.08580559939988,
102.426773796439));
#208601=CARTESIAN_POINT('Ctrl Pts',(4.59582525489943,-4.96997184687442,
102.434906392526));
#208602=CARTESIAN_POINT('Ctrl Pts',(4.71982309942207,-4.84928437093164,
102.443038988613));
#208603=CARTESIAN_POINT('Ctrl Pts',(4.84373617236596,-4.72867940342205,
102.451166024821));
#208604=CARTESIAN_POINT('Ctrl Pts',(4.96312035755527,-4.60322757336693,
102.459293061029));
#208605=CARTESIAN_POINT('Ctrl Pts',(5.07757667926858,-4.47331019113899,
102.467420097237));
#208606=CARTESIAN_POINT('Ctrl Pts',(5.19197828878869,-4.34345491177097,
102.475543248574));
#208607=CARTESIAN_POINT('Ctrl Pts',(5.30145648405404,-4.20913860514696,
102.483666399912));
#208608=CARTESIAN_POINT('Ctrl Pts',(5.40564969535407,-4.07077884085079,
102.49178955125));
#208609=CARTESIAN_POINT('Ctrl Pts',(5.5098136275873,-3.93245795667675,102.499910419921));
#208610=CARTESIAN_POINT('Ctrl Pts',(5.60869531444674,-3.79009617075798,
102.508031288593));
#208611=CARTESIAN_POINT('Ctrl Pts',(5.70197400743463,-3.64414344099405,
102.516152157265));
#208612=CARTESIAN_POINT('Ctrl Pts',(5.79525774156021,-3.49818282338581,
102.524273464819));
#208613=CARTESIAN_POINT('Ctrl Pts',(5.88293767629461,-3.34863118066643,
102.532394772373));
#208614=CARTESIAN_POINT('Ctrl Pts',(5.96473677718711,-3.19596686135377,
102.540516079928));
#208615=CARTESIAN_POINT('Ctrl Pts',(6.00724243349643,-3.11663717414944,
102.544736193645));
#208616=CARTESIAN_POINT('Ctrl Pts',(6.04816088332226,-3.0364674381777,102.548956307361));
#208617=CARTESIAN_POINT('Ctrl Pts',(6.08745817512855,-2.95552735836781,
102.553176421078));
#208618=CARTESIAN_POINT('Ctrl Pts',(6.17112039993154,-2.78320944938805,
102.562160859604));
#208619=CARTESIAN_POINT('Ctrl Pts',(6.24739073536623,-2.60748418737219,
102.57114529813));
#208620=CARTESIAN_POINT('Ctrl Pts',(6.3160382512479,-2.42898122857576,102.580129736656));
#208621=CARTESIAN_POINT('Ctrl Pts',(6.3848042486448,-2.25017018432628,102.589129681786));
#208622=CARTESIAN_POINT('Ctrl Pts',(6.44592104434475,-2.06857208417301,
102.598129626917));
#208623=CARTESIAN_POINT('Ctrl Pts',(6.49920723417377,-1.8848327053782,102.607129572047));
#208624=CARTESIAN_POINT('Ctrl Pts',(6.55261899427689,-1.700660340021,102.616150725779));
#208625=CARTESIAN_POINT('Ctrl Pts',(6.59816316017791,-1.51433683027483,
102.625171879511));
#208626=CARTESIAN_POINT('Ctrl Pts',(6.63570860986035,-1.32652185998771,
102.634193033244));
#208627=CARTESIAN_POINT('Ctrl Pts',(6.6732922623338,-1.13851578648779,102.643223366071));
#208628=CARTESIAN_POINT('Ctrl Pts',(6.70286089843514,-0.949015455999851,
102.652253698898));
#208629=CARTESIAN_POINT('Ctrl Pts',(6.72433498941725,-0.758688308924628,
102.661284031725));
#208630=CARTESIAN_POINT('Ctrl Pts',(6.74583952389134,-0.568091337949582,
102.670327166718));
#208631=CARTESIAN_POINT('Ctrl Pts',(6.759226540875,-0.376665444192629,102.679370301711));
#208632=CARTESIAN_POINT('Ctrl Pts',(6.76446843892268,-0.185083059243751,
102.688413436703));
#208633=CARTESIAN_POINT('Ctrl Pts',(6.76905106547896,-0.0175959168006838,
102.696319220103));
#208634=CARTESIAN_POINT('Ctrl Pts',(6.76740934505064,0.150010698279156,
102.704225003503));
#208635=CARTESIAN_POINT('Ctrl Pts',(6.75955746518642,0.317288315010941,
102.712130786903));
#208636=CARTESIAN_POINT('Ctrl Pts',(6.75096307784368,0.500384421526346,
102.720784175131));
#208637=CARTESIAN_POINT('Ctrl Pts',(6.73491958926912,0.683248057353243,
102.72943756336));
#208638=CARTESIAN_POINT('Ctrl Pts',(6.71145332422156,0.865264859332294,
102.738090951588));
#208639=CARTESIAN_POINT('Ctrl Pts',(6.68800873193436,1.04711355588331,102.746736347798));
#208640=CARTESIAN_POINT('Ctrl Pts',(6.65715507527826,1.22811667804449,102.755381744009));
#208641=CARTESIAN_POINT('Ctrl Pts',(6.6189705599523,1.40766392526224,102.764027140219));
#208642=CARTESIAN_POINT('Ctrl Pts',(6.57956655983556,1.59294530673156,102.772948641262));
#208643=CARTESIAN_POINT('Ctrl Pts',(6.53235571106689,1.77667595712159,102.781870142304));
#208644=CARTESIAN_POINT('Ctrl Pts',(6.47748170115115,1.95819299642606,102.790791643346));
#208645=CARTESIAN_POINT('Ctrl Pts',(6.42440722333664,2.13375738638614,102.799420573688));
#208646=CARTESIAN_POINT('Ctrl Pts',(6.36416430221327,2.30725072234848,102.80804950403));
#208647=CARTESIAN_POINT('Ctrl Pts',(6.29693451022695,2.47808490046504,102.816678434372));
#208648=CARTESIAN_POINT('Ctrl Pts',(6.22628549942339,2.65760748024384,102.825746220765));
#208649=CARTESIAN_POINT('Ctrl Pts',(6.14792048194812,2.83419303824045,102.834814007157));
#208650=CARTESIAN_POINT('Ctrl Pts',(6.06210923495723,3.0071781828562,102.84388179355));
#208651=CARTESIAN_POINT('Ctrl Pts',(5.97629798796633,3.18016332747195,102.852949579943));
#208652=CARTESIAN_POINT('Ctrl Pts',(5.88304065346145,3.34954769322734,102.862017366335));
#208653=CARTESIAN_POINT('Ctrl Pts',(5.78266570200121,3.51469292810893,102.871085152728));
#208654=CARTESIAN_POINT('Ctrl Pts',(5.68940649558566,3.66813074625289,102.879510108861));
#208655=CARTESIAN_POINT('Ctrl Pts',(5.59004418751204,3.81784196527256,102.887935064994));
#208656=CARTESIAN_POINT('Ctrl Pts',(5.48491019652612,3.96333813042034,102.896360021127));
#208657=CARTESIAN_POINT('Ctrl Pts',(5.37975180293139,4.10886806662512,102.904786932774));
#208658=CARTESIAN_POINT('Ctrl Pts',(5.26881924955178,4.25018072948424,102.91321384442));
#208659=CARTESIAN_POINT('Ctrl Pts',(5.15248564259967,4.38681897310617,102.921640756067));
#208660=CARTESIAN_POINT('Ctrl Pts',(5.03610925524897,4.52350746393248,102.930070766617));
#208661=CARTESIAN_POINT('Ctrl Pts',(4.91432806894055,4.65551785569813,102.938500777167));
#208662=CARTESIAN_POINT('Ctrl Pts',(4.78755385332686,4.78242795047611,102.946930787717));
#208663=CARTESIAN_POINT('Ctrl Pts',(4.66066285595716,4.90945495217916,102.955368563816));
#208664=CARTESIAN_POINT('Ctrl Pts',(4.52876987445921,5.03137203536056,102.963806339916));
#208665=CARTESIAN_POINT('Ctrl Pts',(4.39232256178812,5.14779482042623,102.972244116015));
#208666=CARTESIAN_POINT('Ctrl Pts',(4.2558036243361,5.26427871887193,102.980686321325));
#208667=CARTESIAN_POINT('Ctrl Pts',(4.11472584479548,5.37526235816219,102.989128526635));
#208668=CARTESIAN_POINT('Ctrl Pts',(3.96956843621229,5.48040285291393,102.997570731945));
#208669=CARTESIAN_POINT('Ctrl Pts',(3.82425789454982,5.58565426510264,103.006021843317));
#208670=CARTESIAN_POINT('Ctrl Pts',(3.6748593994887,5.6850500312575,103.014472954689));
#208671=CARTESIAN_POINT('Ctrl Pts',(3.52188039471258,5.77829105232154,103.022924066061));
#208672=CARTESIAN_POINT('Ctrl Pts',(3.47894660005773,5.80445928931347,103.025295883558));
#208673=CARTESIAN_POINT('Ctrl Pts',(3.43573093221849,5.83014302523311,103.027667701055));
#208674=CARTESIAN_POINT('Ctrl Pts',(3.39224493727712,5.8553363084897,103.030039518553));
#208675=CARTESIAN_POINT('Ctrl Pts',(3.2959276597028,5.91113699695742,103.035292865166));
#208676=CARTESIAN_POINT('Ctrl Pts',(3.19817427377089,5.96459467347469,103.040546211779));
#208677=CARTESIAN_POINT('Ctrl Pts',(3.09910619832139,6.01563211736937,103.045799558392));
#208678=CARTESIAN_POINT('Ctrl Pts',(3.09910619832146,6.01563211736934,101.0456200824));
#208679=CARTESIAN_POINT('Ctrl Pts',(2.94206679343137,6.09653496906972,101.053938109991));
#208680=CARTESIAN_POINT('Ctrl Pts',(2.78197250407096,6.1712253801484,101.062256137582));
#208681=CARTESIAN_POINT('Ctrl Pts',(2.61935543177763,6.23949245708472,101.070574165172));
#208682=CARTESIAN_POINT('Ctrl Pts',(2.44988024168382,6.31063859000771,101.07924299242));
#208683=CARTESIAN_POINT('Ctrl Pts',(2.27766527045293,6.37480769062343,101.087911819667));
#208684=CARTESIAN_POINT('Ctrl Pts',(2.10332965315264,6.43181882286564,101.096580646914));
#208685=CARTESIAN_POINT('Ctrl Pts',(1.92899403585247,6.48882995510782,101.105249474161));
#208686=CARTESIAN_POINT('Ctrl Pts',(1.75253819497853,6.53868306401959,101.113918301409));
#208687=CARTESIAN_POINT('Ctrl Pts',(1.57459222930509,6.58125735034059,101.122587128656));
#208688=CARTESIAN_POINT('Ctrl Pts',(1.40894161719297,6.62088992398518,101.130656974659));
#208689=CARTESIAN_POINT('Ctrl Pts',(1.24148778099825,6.65433737297032,101.138726820661));
#208690=CARTESIAN_POINT('Ctrl Pts',(1.07274313453212,6.68143032346475,101.146796666664));
#208691=CARTESIAN_POINT('Ctrl Pts',(0.904210790295027,6.70848918758131,
101.154856359774));
#208692=CARTESIAN_POINT('Ctrl Pts',(0.734391230787464,6.72920940219974,
101.162916052884));
#208693=CARTESIAN_POINT('Ctrl Pts',(0.5638120491549,6.74347128511924,101.170975745994));
#208694=CARTESIAN_POINT('Ctrl Pts',(0.393410041095697,6.75771835480811,
101.179027067833));
#208695=CARTESIAN_POINT('Ctrl Pts',(0.222250349639107,6.76552041097045,
101.187078389672));
#208696=CARTESIAN_POINT('Ctrl Pts',(0.050870685568204,6.76680878799969,
101.19512971151));
#208697=CARTESIAN_POINT('Ctrl Pts',(-0.120368528625231,6.76809610917206,
101.203174435091));
#208698=CARTESIAN_POINT('Ctrl Pts',(-0.291826985450638,6.7628803729991,
101.211219158672));
#208699=CARTESIAN_POINT('Ctrl Pts',(-0.462962030385573,6.75114472948264,
101.219263882253));
#208700=CARTESIAN_POINT('Ctrl Pts',(-0.633994287449413,6.73941613467917,
101.227303773978));
#208701=CARTESIAN_POINT('Ctrl Pts',(-0.80470314802758,6.72117545356874,
101.235343665702));
#208702=CARTESIAN_POINT('Ctrl Pts',(-0.974546244514403,6.69645791574194,
101.243383557426));
#208703=CARTESIAN_POINT('Ctrl Pts',(-1.14804652818518,6.67120814160746,
101.251596570046));
#208704=CARTESIAN_POINT('Ctrl Pts',(-1.32064294170514,6.63919941457178,
101.259809582666));
#208705=CARTESIAN_POINT('Ctrl Pts',(-1.49176264479612,6.60052522240396,
101.268022595286));
#208706=CARTESIAN_POINT('Ctrl Pts',(-1.65921689410972,6.56267944719345,
101.276059681829));
#208707=CARTESIAN_POINT('Ctrl Pts',(-1.8252566793481,6.5184509665929,101.284096768371));
#208708=CARTESIAN_POINT('Ctrl Pts',(-1.98935582725716,6.46797900371963,
101.292133854914));
#208709=CARTESIAN_POINT('Ctrl Pts',(-2.1534706802192,6.41750221044437,101.300171710643));
#208710=CARTESIAN_POINT('Ctrl Pts',(-2.31564416887222,6.36078085483351,
101.308209566372));
#208711=CARTESIAN_POINT('Ctrl Pts',(-2.47536594874771,6.29800384405888,
101.316247422102));
#208712=CARTESIAN_POINT('Ctrl Pts',(-2.63513466095759,6.23520838701058,
101.324287639659));
#208713=CARTESIAN_POINT('Ctrl Pts',(-2.79244988291351,6.16635386959734,
101.332327857215));
#208714=CARTESIAN_POINT('Ctrl Pts',(-2.9468220355432,6.09167701793497,101.340368074772));
#208715=CARTESIAN_POINT('Ctrl Pts',(-3.1070264670085,6.01417882696987,101.3487120569));
#208716=CARTESIAN_POINT('Ctrl Pts',(-3.26406070273427,5.93040995929566,
101.357056039028));
#208717=CARTESIAN_POINT('Ctrl Pts',(-3.41740739920343,5.84068623261596,
101.365400021156));
#208718=CARTESIAN_POINT('Ctrl Pts',(-3.5654287178849,5.75407840443353,101.373454235991));
#208719=CARTESIAN_POINT('Ctrl Pts',(-3.71001404861886,5.66192263440905,
101.381508450826));
#208720=CARTESIAN_POINT('Ctrl Pts',(-3.85072973210325,5.56454576136238,
101.389562665661));
#208721=CARTESIAN_POINT('Ctrl Pts',(-3.99155071800775,5.46709601782864,
101.397622907744));
#208722=CARTESIAN_POINT('Ctrl Pts',(-4.12849599391133,5.36441761424839,
101.405683149827));
#208723=CARTESIAN_POINT('Ctrl Pts',(-4.26116633430348,5.25687649383154,
101.41374339191));
#208724=CARTESIAN_POINT('Ctrl Pts',(-4.39402215693354,5.14918502355035,
101.421814902764));
#208725=CARTESIAN_POINT('Ctrl Pts',(-4.52259084117014,5.03661751620381,
101.429886413618));
#208726=CARTESIAN_POINT('Ctrl Pts',(-4.64651082041657,4.91957581461571,
101.437957924473));
#208727=CARTESIAN_POINT('Ctrl Pts',(-4.65949892806982,4.90730862227602,
101.438803903084));
#208728=CARTESIAN_POINT('Ctrl Pts',(-4.67243600608959,4.89499230859961,
101.439649881695));
#208729=CARTESIAN_POINT('Ctrl Pts',(-4.68532166475965,4.88262735601786,
101.440495860305));
#208730=CARTESIAN_POINT('Ctrl Pts',(-4.80979550241226,4.76318347350842,
101.448667906994));
#208731=CARTESIAN_POINT('Ctrl Pts',(-4.9298945580079,4.63878884005489,101.456839953683));
#208732=CARTESIAN_POINT('Ctrl Pts',(-5.04519683654342,4.50979798666551,
101.465012000372));
#208733=CARTESIAN_POINT('Ctrl Pts',(-5.16035907248924,4.38096380158648,
101.473174121545));
#208734=CARTESIAN_POINT('Ctrl Pts',(-5.27073588981002,4.24754477950296,
101.481336242717));
#208735=CARTESIAN_POINT('Ctrl Pts',(-5.37593976111861,4.10993438935757,
101.48949836389));
#208736=CARTESIAN_POINT('Ctrl Pts',(-5.4810378177215,3.97246240859534,101.497652275551));
#208737=CARTESIAN_POINT('Ctrl Pts',(-5.58097306863981,3.83080774162944,
101.505806187212));
#208738=CARTESIAN_POINT('Ctrl Pts',(-5.67539614195182,3.68539925000243,
101.513960098873));
#208739=CARTESIAN_POINT('Ctrl Pts',(-5.76973307192783,3.54012341633825,
101.52210657162));
#208740=CARTESIAN_POINT('Ctrl Pts',(-5.85856764704998,3.39110088621093,
101.530253044366));
#208741=CARTESIAN_POINT('Ctrl Pts',(-5.94159206921411,3.23879185546895,
101.538399517113));
#208742=CARTESIAN_POINT('Ctrl Pts',(-6.02457418649144,3.08656043341291,
101.546541838845));
#208743=CARTESIAN_POINT('Ctrl Pts',(-6.10175187064456,2.93104616362484,
101.554684160576));
#208744=CARTESIAN_POINT('Ctrl Pts',(-6.17286161926892,2.7727366318056,101.562826482308));
#208745=CARTESIAN_POINT('Ctrl Pts',(-6.24394856591401,2.61447786335895,
101.570966193131));
#208746=CARTESIAN_POINT('Ctrl Pts',(-6.30897130248828,2.45342594979255,
101.579105903954));
#208747=CARTESIAN_POINT('Ctrl Pts',(-6.36771313026394,2.29009137168458,
101.587245614778));
#208748=CARTESIAN_POINT('Ctrl Pts',(-6.4264472172201,2.12677831731084,101.595384252974));
#208749=CARTESIAN_POINT('Ctrl Pts',(-6.47890192160153,1.96118354067021,
101.603522891171));
#208750=CARTESIAN_POINT('Ctrl Pts',(-6.52490938756892,1.79383569036157,
101.611661529368));
#208751=CARTESIAN_POINT('Ctrl Pts',(-6.5709326468189,1.62643039346608,101.619802961368));
#208752=CARTESIAN_POINT('Ctrl Pts',(-6.61050414693564,1.45727117161119,
101.627944393368));
#208753=CARTESIAN_POINT('Ctrl Pts',(-6.6435063304656,1.2869003990455,101.636085825369));
#208754=CARTESIAN_POINT('Ctrl Pts',(-6.67651474699476,1.11649744918802,
101.644228795011));
#208755=CARTESIAN_POINT('Ctrl Pts',(-6.7029513136287,0.944882852027836,
101.652371764653));
#208756=CARTESIAN_POINT('Ctrl Pts',(-6.72274997655316,0.772607114097821,
101.660514734295));
#208757=CARTESIAN_POINT('Ctrl Pts',(-6.74256349027035,0.600202153740679,
101.668663811903));
#208758=CARTESIAN_POINT('Ctrl Pts',(-6.75572912332282,0.427135425137091,
101.67681288951));
#208759=CARTESIAN_POINT('Ctrl Pts',(-6.76223282506295,0.253961059300643,
101.684961967118));
#208760=CARTESIAN_POINT('Ctrl Pts',(-6.76548313303249,0.167414959265863,
101.689034572682));
#208761=CARTESIAN_POINT('Ctrl Pts',(-6.76707035411167,0.0808419783983983,
101.693107178246));
#208762=CARTESIAN_POINT('Ctrl Pts',(-6.76699760869648,-0.00568892750522595,
101.69717978381));
#208763=CARTESIAN_POINT('',(-6.76727197366057,0.000320845660479878,101.303291156375));
#208764=CARTESIAN_POINT('Ctrl Pts',(3.09910619832147,6.01563211736933,100.651473518761));
#208765=CARTESIAN_POINT('Ctrl Pts',(2.93980871858144,6.09769827387746,100.659895895807));
#208766=CARTESIAN_POINT('Ctrl Pts',(2.77722459638561,6.17344596557304,100.668318272853));
#208767=CARTESIAN_POINT('Ctrl Pts',(2.61188535517925,6.24262315788805,100.6767406499));
#208768=CARTESIAN_POINT('Ctrl Pts',(2.44655248697758,6.31179768376666,100.685162702305));
#208769=CARTESIAN_POINT('Ctrl Pts',(2.27846501917269,6.37440208664836,100.693584754711));
#208770=CARTESIAN_POINT('Ctrl Pts',(2.1081747221875,6.43023237066357,100.702006807116));
#208771=CARTESIAN_POINT('Ctrl Pts',(1.93786721771301,6.48606829621581,100.710429710553));
#208772=CARTESIAN_POINT('Ctrl Pts',(1.76535675730985,6.535128634809,100.71885261399));
#208773=CARTESIAN_POINT('Ctrl Pts',(1.59121089754127,6.57725907042941,100.727275517427));
#208774=CARTESIAN_POINT('Ctrl Pts',(1.41534333340634,6.61980603134109,100.735781694447));
#208775=CARTESIAN_POINT('Ctrl Pts',(1.23780819329335,6.65528523302602,100.744287871466));
#208776=CARTESIAN_POINT('Ctrl Pts',(1.05920117056735,6.68359049316075,100.752794048485));
#208777=CARTESIAN_POINT('Ctrl Pts',(0.882174701826115,6.71164527047004,
100.761224951466));
#208778=CARTESIAN_POINT('Ctrl Pts',(0.704095583496147,6.73265256018185,
100.769655854446));
#208779=CARTESIAN_POINT('Ctrl Pts',(0.525549680055566,6.74656108945836,
100.778086757427));
#208780=CARTESIAN_POINT('Ctrl Pts',(0.3446125965744,6.76065588902703,100.786630571466));
#208781=CARTESIAN_POINT('Ctrl Pts',(0.163196488995154,6.76746039834387,
100.795174385505));
#208782=CARTESIAN_POINT('Ctrl Pts',(-0.0180881004267439,6.76697582533165,
100.803718199544));
#208783=CARTESIAN_POINT('Ctrl Pts',(-0.199372689848642,6.76649125231943,
100.812262013583));
#208784=CARTESIAN_POINT('Ctrl Pts',(-0.380525408145483,6.75871763816219,
100.820805827621));
#208785=CARTESIAN_POINT('Ctrl Pts',(-0.560940188314447,6.74371078154556,
100.82934964166));
#208786=CARTESIAN_POINT('Ctrl Pts',(-0.732821843464126,6.72941370814921,
100.837489356693));
#208787=CARTESIAN_POINT('Ctrl Pts',(-0.904376410743714,6.70852274586707,
100.845629071726));
#208788=CARTESIAN_POINT('Ctrl Pts',(-1.07505406080753,6.68105888062224,
100.853768786759));
#208789=CARTESIAN_POINT('Ctrl Pts',(-1.24558243722208,6.65361903510926,
100.861901382846));
#208790=CARTESIAN_POINT('Ctrl Pts',(-1.41523506394114,6.61961778700909,
100.870033978933));
#208791=CARTESIAN_POINT('Ctrl Pts',(-1.58346559710706,6.57912803514101,
100.87816657502));
#208792=CARTESIAN_POINT('Ctrl Pts',(-1.75158111885478,6.53866596423962,
100.886293611228));
#208793=CARTESIAN_POINT('Ctrl Pts',(-1.91827612810709,6.49172430653978,
100.894420647436));
#208794=CARTESIAN_POINT('Ctrl Pts',(-2.0830129060397,6.43842731055279,100.902547683644));
#208795=CARTESIAN_POINT('Ctrl Pts',(-2.24767093681206,6.38515579149413,
100.910670834981));
#208796=CARTESIAN_POINT('Ctrl Pts',(-2.41037225260023,6.32553509622326,
100.918793986319));
#208797=CARTESIAN_POINT('Ctrl Pts',(-2.5705927930854,6.25973974635826,100.926917137656));
#208798=CARTESIAN_POINT('Ctrl Pts',(-2.73076831040713,6.19396288547591,
100.935038006328));
#208799=CARTESIAN_POINT('Ctrl Pts',(-2.88846410278187,6.1220149657471,100.943158875));
#208800=CARTESIAN_POINT('Ctrl Pts',(-3.04317468101102,6.04411919644653,
100.951279743671));
#208801=CARTESIAN_POINT('Ctrl Pts',(-3.19789362039328,5.96621921735979,
100.959401051226));
#208802=CARTESIAN_POINT('Ctrl Pts',(-3.34962669442722,5.88237090765951,
100.96752235878));
#208803=CARTESIAN_POINT('Ctrl Pts',(-3.49789151317762,5.79284420315616,
100.975643666335));
#208804=CARTESIAN_POINT('Ctrl Pts',(-3.57493506695422,5.74632301538568,
100.979863780052));
#208805=CARTESIAN_POINT('Ctrl Pts',(-3.65104253294218,5.69826929833173,
100.984083893768));
#208806=CARTESIAN_POINT('Ctrl Pts',(-3.72614913619489,5.64872566291142,
100.988304007485));
#208807=CARTESIAN_POINT('Ctrl Pts',(-3.88604782734473,5.54324941827475,
100.997288446011));
#208808=CARTESIAN_POINT('Ctrl Pts',(-4.04132928615683,5.43107009608483,
101.006272884537));
#208809=CARTESIAN_POINT('Ctrl Pts',(-4.19147353707513,5.31261127770505,
101.015257323062));
#208810=CARTESIAN_POINT('Ctrl Pts',(-4.34187692800926,5.19394800647488,
101.024257268193));
#208811=CARTESIAN_POINT('Ctrl Pts',(-4.48712520165042,5.06898372477758,
101.033257213323));
#208812=CARTESIAN_POINT('Ctrl Pts',(-4.62673274228182,4.93818115620492,
101.042257158454));
#208813=CARTESIAN_POINT('Ctrl Pts',(-4.76666927166609,4.80707034802204,
101.051278312186));
#208814=CARTESIAN_POINT('Ctrl Pts',(-4.90093829675574,4.67009388933978,
101.060299465918));
#208815=CARTESIAN_POINT('Ctrl Pts',(-5.02909034220098,4.52775212770982,
101.06932061965));
#208816=CARTESIAN_POINT('Ctrl Pts',(-5.15737278336259,4.38526553221544,
101.078350952477));
#208817=CARTESIAN_POINT('Ctrl Pts',(-5.2795256554229,4.23740290900318,101.087381285305));
#208818=CARTESIAN_POINT('Ctrl Pts',(-5.39513988999777,4.08469761027116,
101.096411618132));
#208819=CARTESIAN_POINT('Ctrl Pts',(-5.51091802911308,3.93177582356165,
101.105454753124));
#208820=CARTESIAN_POINT('Ctrl Pts',(-5.62013885138369,3.77399782444096,
101.114497888117));
#208821=CARTESIAN_POINT('Ctrl Pts',(-5.72243539414993,3.61192776225939,
101.12354102311));
#208822=CARTESIAN_POINT('Ctrl Pts',(-5.81186614027298,3.47024118915372,
101.13144680651));
#208823=CARTESIAN_POINT('Ctrl Pts',(-5.89600542329012,3.32527480091662,
101.13935258991));
#208824=CARTESIAN_POINT('Ctrl Pts',(-5.97463653142679,3.17742148877678,
101.14725837331));
#208825=CARTESIAN_POINT('Ctrl Pts',(-6.06076738254096,3.01546610093565,
101.155918201069));
#208826=CARTESIAN_POINT('Ctrl Pts',(-6.14036378958474,2.84990385863868,
101.164578028828));
#208827=CARTESIAN_POINT('Ctrl Pts',(-6.21313452694192,2.68127737284343,
101.173237856587));
#208828=CARTESIAN_POINT('Ctrl Pts',(-6.28583775382177,2.51280732430525,
101.181889650497));
#208829=CARTESIAN_POINT('Ctrl Pts',(-6.35172782142323,2.34127897961005,
101.190541444407));
#208830=CARTESIAN_POINT('Ctrl Pts',(-6.41056020199429,2.16725792110838,
101.199193238317));
#208831=CARTESIAN_POINT('Ctrl Pts',(-6.46932382959776,1.99344022789768,
101.207834921528));
#208832=CARTESIAN_POINT('Ctrl Pts',(-6.52104613445438,1.81713592098677,
101.216476604739));
#208833=CARTESIAN_POINT('Ctrl Pts',(-6.56553126704991,1.63892897386985,
101.22511828795));
#208834=CARTESIAN_POINT('Ctrl Pts',(-6.6099838820073,1.46085229205017,101.233753654284));
#208835=CARTESIAN_POINT('Ctrl Pts',(-6.64720980163098,1.28087603669714,
101.242389020617));
#208836=CARTESIAN_POINT('Ctrl Pts',(-6.67706304938711,1.099599033516,101.251024386951));
#208837=CARTESIAN_POINT('Ctrl Pts',(-6.70690686575957,0.918379300250059,
101.259657025157));
#208838=CARTESIAN_POINT('Ctrl Pts',(-6.72938259100124,0.735859934554445,
101.268289663364));
#208839=CARTESIAN_POINT('Ctrl Pts',(-6.7443951469935,0.552650975942862,
101.27692230157));
#208840=CARTESIAN_POINT('Ctrl Pts',(-6.75940770298576,0.369442017331279,
101.285554939777));
#208841=CARTESIAN_POINT('Ctrl Pts',(-6.76695703681141,0.185543765753519,
101.294187577983));
#208842=CARTESIAN_POINT('Ctrl Pts',(-6.76699981703943,0.00157359091162204,
101.30282021619));
#208843=CARTESIAN_POINT('Ctrl Pts',(-6.767,4.55020098182511E-12,101.30282021619));
#208844=CARTESIAN_POINT('Ctrl Pts',(-6.76700000000013,-0.186007249522411,
101.311569728001));
#208845=CARTESIAN_POINT('Ctrl Pts',(-6.75932637294545,-0.372014355745552,
101.320319239812));
#208846=CARTESIAN_POINT('Ctrl Pts',(-6.74400518264216,-0.557389537483226,
101.329068751624));
#208847=CARTESIAN_POINT('Ctrl Pts',(-6.7286840570513,-0.742763936247827,
101.337818226479));
#208848=CARTESIAN_POINT('Ctrl Pts',(-6.70571545645776,-0.927506130238602,
101.346567701335));
#208849=CARTESIAN_POINT('Ctrl Pts',(-6.67517739404857,-1.11098863989824,
101.355317176191));
#208850=CARTESIAN_POINT('Ctrl Pts',(-6.64463945808735,-1.29447038981776,
101.364066614818));
#208851=CARTESIAN_POINT('Ctrl Pts',(-6.60653217008389,-1.47669218313533,
101.372816053445));
#208852=CARTESIAN_POINT('Ctrl Pts',(-6.5609849609271,-1.65703510599156,
101.381565492072));
#208853=CARTESIAN_POINT('Ctrl Pts',(-6.51543793658328,-1.83737729708591,
101.390314895197));
#208854=CARTESIAN_POINT('Ctrl Pts',(-6.46245112167449,-2.01584035510838,
101.399064298322));
#208855=CARTESIAN_POINT('Ctrl Pts',(-6.40220448374277,-2.19181813760723,
101.407813701447));
#208856=CARTESIAN_POINT('Ctrl Pts',(-6.34195808526531,-2.36779522067069,
101.416563069797));
#208857=CARTESIAN_POINT('Ctrl Pts',(-6.27445201433136,-2.54128677684086,
101.425312438147));
#208858=CARTESIAN_POINT('Ctrl Pts',(-6.19991555071939,-2.71170355384726,
101.434061806498));
#208859=CARTESIAN_POINT('Ctrl Pts',(-6.12537937716729,-2.88211966767401,
101.442811140799));
#208860=CARTESIAN_POINT('Ctrl Pts',(-6.04381298052555,-3.04946076371717,
101.451560475101));
#208861=CARTESIAN_POINT('Ctrl Pts',(-5.95549339335864,-3.21315848374487,
101.460309809403));
#208862=CARTESIAN_POINT('Ctrl Pts',(-5.86717414255447,-3.37685558033427,
101.469059110383));
#208863=CARTESIAN_POINT('Ctrl Pts',(-5.77210188876641,-3.53690907646685,
101.477808411363));
#208864=CARTESIAN_POINT('Ctrl Pts',(-5.67059953347045,-3.69277536969211,
101.486557712343));
#208865=CARTESIAN_POINT('Ctrl Pts',(-5.5690975563143,-3.84864108224857,
101.495306980729));
#208866=CARTESIAN_POINT('Ctrl Pts',(-5.46116568196893,-4.00031938297459,
101.504056249114));
#208867=CARTESIAN_POINT('Ctrl Pts',(-5.34717048533642,-4.14729511859804,
101.512805517499));
#208868=CARTESIAN_POINT('Ctrl Pts',(-5.23317570391899,-4.29427031887839,
101.521554754016));
#208869=CARTESIAN_POINT('Ctrl Pts',(-5.11311782003602,-4.43654276189444,
101.530303990533));
#208870=CARTESIAN_POINT('Ctrl Pts',(-4.98740458984869,-4.57362924351726,
101.53905322705));
#208871=CARTESIAN_POINT('Ctrl Pts',(-4.86169180711877,-4.71071523720127,
101.547802432426));
#208872=CARTESIAN_POINT('Ctrl Pts',(-4.73032391204326,-4.84261509523086,
101.556551637801));
#208873=CARTESIAN_POINT('Ctrl Pts',(-4.59374707013774,-4.96888084538168,
101.565300843177));
#208874=CARTESIAN_POINT('Ctrl Pts',(-4.45717070301659,-5.09514615659275,
101.574050018137));
#208875=CARTESIAN_POINT('Ctrl Pts',(-4.31538563571296,-5.21577720459315,
101.582799193097));
#208876=CARTESIAN_POINT('Ctrl Pts',(-4.16887341029808,-5.33036429232653,
101.591548368058));
#208877=CARTESIAN_POINT('Ctrl Pts',(-4.02236168204015,-5.44495099123387,
101.60029751333));
#208878=CARTESIAN_POINT('Ctrl Pts',(-3.87112305348485,-5.55349359438379,
101.609046658602));
#208879=CARTESIAN_POINT('Ctrl Pts',(-3.7156711701809,-5.65562346298677,
101.617795803874));
#208880=CARTESIAN_POINT('Ctrl Pts',(-3.56021980146167,-5.75775299351429,
101.626544920184));
#208881=CARTESIAN_POINT('Ctrl Pts',(-3.40055544538715,-5.8534696746366,
101.635294036494));
#208882=CARTESIAN_POINT('Ctrl Pts',(-3.23722035987238,-5.94244842986691,
101.644043152804));
#208883=CARTESIAN_POINT('Ctrl Pts',(-3.07388580147568,-6.03142689794332,
101.652792240879));
#208884=CARTESIAN_POINT('Ctrl Pts',(-2.90688078896968,-6.11366734656596,
101.661541328954));
#208885=CARTESIAN_POINT('Ctrl Pts',(-2.73677250721761,-6.18889046952181,
101.670290417029));
#208886=CARTESIAN_POINT('Ctrl Pts',(-2.5666647603187,-6.26411335596168,
101.679039477595));
#208887=CARTESIAN_POINT('Ctrl Pts',(-2.39345402575551,-6.33231884500411,
101.687788538161));
#208888=CARTESIAN_POINT('Ctrl Pts',(-2.21772856065972,-6.39327529762595,
101.696537598727));
#208889=CARTESIAN_POINT('Ctrl Pts',(-2.04200363348908,-6.45423156364986,
101.705286632511));
#208890=CARTESIAN_POINT('Ctrl Pts',(-1.86376426189688,-6.50793874375541,
101.714035666294));
#208891=CARTESIAN_POINT('Ctrl Pts',(-1.68361577753577,-6.55421443909433,
101.722784700078));
#208892=CARTESIAN_POINT('Ctrl Pts',(-1.50346782968266,-6.60048999661761,
101.731533707806));
#208893=CARTESIAN_POINT('Ctrl Pts',(-1.32141105795497,-6.6393340423761,
101.740282715534));
#208894=CARTESIAN_POINT('Ctrl Pts',(-1.13806375487577,-6.67061465607466,
101.749031723262));
#208895=CARTESIAN_POINT('Ctrl Pts',(-0.954716982608748,-6.70189517921214,
101.75778070566));
#208896=CARTESIAN_POINT('Ctrl Pts',(-0.770079968908055,-6.7256122659216,
101.766529688058));
#208897=CARTESIAN_POINT('Ctrl Pts',(-0.58477976556434,-6.74168536983049,
101.775278670457));
#208898=CARTESIAN_POINT('Ctrl Pts',(-0.391489830657309,-6.75845151013819,
101.784404889467));
#208899=CARTESIAN_POINT('Ctrl Pts',(-0.197478578244254,-6.76689983031608,
101.793531108477));
#208900=CARTESIAN_POINT('Ctrl Pts',(-0.00346287645716383,-6.76699911397117,
101.802657327486));
#208901=CARTESIAN_POINT('Ctrl Pts',(0.184489834649052,-6.76709529501204,
101.811498352152));
#208902=CARTESIAN_POINT('Ctrl Pts',(0.37244640424463,-6.75935639738194,
101.820339376818));
#208903=CARTESIAN_POINT('Ctrl Pts',(0.559755019483695,-6.74380925873225,
101.829180401484));
#208904=CARTESIAN_POINT('Ctrl Pts',(0.745134705517098,-6.72842222659857,
101.837930380094));
#208905=CARTESIAN_POINT('Ctrl Pts',(0.92987943122386,-6.70538706057589,
101.846680358703));
#208906=CARTESIAN_POINT('Ctrl Pts',(1.11336163626352,-6.67478200894206,
101.855430337313));
#208907=CARTESIAN_POINT('Ctrl Pts',(1.29684196300264,-6.64417727061102,
101.86418022635));
#208908=CARTESIAN_POINT('Ctrl Pts',(1.47905951217074,-6.60600284890688,
101.872930115386));
#208909=CARTESIAN_POINT('Ctrl Pts',(1.65939532066667,-6.56038841607336,
101.881680004423));
#208910=CARTESIAN_POINT('Ctrl Pts',(1.83972934300399,-6.51477443503371,
101.890429806795));
#208911=CARTESIAN_POINT('Ctrl Pts',(2.01818138405877,-6.46172066062263,
101.899179609167));
#208912=CARTESIAN_POINT('Ctrl Pts',(2.19414528353827,-6.40140730423606,
101.907929411539));
#208913=CARTESIAN_POINT('Ctrl Pts',(2.37010749863629,-6.34109452518781,
101.916679130155));
#208914=CARTESIAN_POINT('Ctrl Pts',(2.54358134866092,-6.27352239616653,
101.925428848772));
#208915=CARTESIAN_POINT('Ctrl Pts',(2.71397759435191,-6.19892043966979,
101.934178567388));
#208916=CARTESIAN_POINT('Ctrl Pts',(2.88437226557757,-6.12431917249688,
101.942928205157));
#208917=CARTESIAN_POINT('Ctrl Pts',(3.05168912680587,-6.04268832278984,
101.951677842925));
#208918=CARTESIAN_POINT('Ctrl Pts',(3.21535986273485,-5.95430516123533,
101.960427480694));
#208919=CARTESIAN_POINT('Ctrl Pts',(3.37902914072483,-5.86592278697647,
101.969177040523));
#208920=CARTESIAN_POINT('Ctrl Pts',(3.53905210621224,-5.77078835742155,
101.977926600352));
#208921=CARTESIAN_POINT('Ctrl Pts',(3.6948852283136,-5.66922500431849,101.986676160181));
#208922=CARTESIAN_POINT('Ctrl Pts',(3.85071701406623,-5.56766252217313,
101.995425644979));
#208923=CARTESIAN_POINT('Ctrl Pts',(4.00235878822108,-5.45967138329587,
102.004175129776));
#208924=CARTESIAN_POINT('Ctrl Pts',(4.14929549611049,-5.34561838199821,
102.012924614573));
#208925=CARTESIAN_POINT('Ctrl Pts',(4.29623099275825,-5.23156632087233,
102.021674027245));
#208926=CARTESIAN_POINT('Ctrl Pts',(4.43846127435774,-5.11145267305185,
102.030423439918));
#208927=CARTESIAN_POINT('Ctrl Pts',(4.57550326054199,-4.98568540050108,
102.039172852591));
#208928=CARTESIAN_POINT('Ctrl Pts',(4.7125441625754,-4.85991912290594,102.047922196046));
#208929=CARTESIAN_POINT('Ctrl Pts',(4.84439664018524,-4.72849950385662,
102.056671539501));
#208930=CARTESIAN_POINT('Ctrl Pts',(4.97061286794511,-4.59187289861321,
102.065420882956));
#208931=CARTESIAN_POINT('Ctrl Pts',(5.09682813912451,-4.45524732884951,
102.074170160101));
#208932=CARTESIAN_POINT('Ctrl Pts',(5.21740705147607,-4.31341506236068,
102.082919437246));
#208933=CARTESIAN_POINT('Ctrl Pts',(5.33194007545466,-4.16685781276018,
102.091668714391));
#208934=CARTESIAN_POINT('Ctrl Pts',(5.44647226944258,-4.02030162522149,
102.100417928132));
#208935=CARTESIAN_POINT('Ctrl Pts',(5.55495848627889,-3.86902074888255,
102.109167141873));
#208936=CARTESIAN_POINT('Ctrl Pts',(5.65703027291568,-3.71352898080998,
102.117916355614));
#208937=CARTESIAN_POINT('Ctrl Pts',(5.75910135376778,-3.55803828789943,
102.126665508858));
#208938=CARTESIAN_POINT('Ctrl Pts',(5.85475793592535,-3.39833700107086,
102.135414662102));
#208939=CARTESIAN_POINT('Ctrl Pts',(5.94367514427184,-3.23496750823947,
102.144163815346));
#208940=CARTESIAN_POINT('Ctrl Pts',(6.03259176732435,-3.07159909078128,
102.152912910999));
#208941=CARTESIAN_POINT('Ctrl Pts',(6.11476896835729,-2.90456276731846,
102.161662006652));
#208942=CARTESIAN_POINT('Ctrl Pts',(6.18992765547701,-2.7344258300347,102.170411102305));
#208943=CARTESIAN_POINT('Ctrl Pts',(6.26508587282888,-2.56428995616577,
102.179160143273));
#208944=CARTESIAN_POINT('Ctrl Pts',(6.33322554827012,-2.39105376935595,
102.187909184241));
#208945=CARTESIAN_POINT('Ctrl Pts',(6.39411526732899,-2.21530561054458,
102.196658225209));
#208946=CARTESIAN_POINT('Ctrl Pts',(6.45500462602724,-2.03955849185489,
102.205407214398));
#208947=CARTESIAN_POINT('Ctrl Pts',(6.50864402040625,-1.86129970164947,
102.214156203587));
#208948=CARTESIAN_POINT('Ctrl Pts',(6.55485128368495,-1.68113463136473,
102.222905192776));
#208949=CARTESIAN_POINT('Ctrl Pts',(6.6019980955423,-1.49730620117296,102.231832078247));
#208950=CARTESIAN_POINT('Ctrl Pts',(6.64140720707787,-1.31149343246137,
102.240758963719));
#208951=CARTESIAN_POINT('Ctrl Pts',(6.67293928722808,-1.12435326697976,
102.24968584919));
#208952=CARTESIAN_POINT('Ctrl Pts',(6.70384625876193,-0.940923067011138,
102.258435763367));
#208953=CARTESIAN_POINT('Ctrl Pts',(6.72718554579744,-0.756217899526259,
102.267185677545));
#208954=CARTESIAN_POINT('Ctrl Pts',(6.74287786815289,-0.570865181259129,
102.275935591722));
#208955=CARTESIAN_POINT('Ctrl Pts',(6.75856988190819,-0.385516108078663,
102.284685333827));
#208956=CARTESIAN_POINT('Ctrl Pts',(6.76661520773389,-0.199519795231143,
102.293435075931));
#208957=CARTESIAN_POINT('Ctrl Pts',(6.76698651789578,-0.0135080204605165,
102.302184818036));
#208958=CARTESIAN_POINT('Ctrl Pts',(6.76735782124915,0.172500343508018,
102.310934399701));
#208959=CARTESIAN_POINT('Ctrl Pts',(6.7600553899521,0.358523882205911,102.319683981366));
#208960=CARTESIAN_POINT('Ctrl Pts',(6.74510402742402,0.543930748559304,
102.328433563031));
#208961=CARTESIAN_POINT('Ctrl Pts',(6.73015291918085,0.729334461610168,
102.337182995887));
#208962=CARTESIAN_POINT('Ctrl Pts',(6.70755316306664,0.914121237629624,
102.345932428744));
#208963=CARTESIAN_POINT('Ctrl Pts',(6.67738151874657,1.09766345165618,102.354681861601));
#208964=CARTESIAN_POINT('Ctrl Pts',(6.64721034747666,1.28120278799162,102.363431157278));
#208965=CARTESIAN_POINT('Ctrl Pts',(6.60946757205252,1.4634973185983,102.372180452956));
#208966=CARTESIAN_POINT('Ctrl Pts',(6.56428138111647,1.64392790277666,102.380929748633));
#208967=CARTESIAN_POINT('Ctrl Pts',(6.51909583859992,1.82435589778547,102.389678918759));
#208968=CARTESIAN_POINT('Ctrl Pts',(6.46646716393037,2.00291972191743,102.398428088885));
#208969=CARTESIAN_POINT('Ctrl Pts',(6.40657409873065,2.17901292274131,102.40717725901));
#208970=CARTESIAN_POINT('Ctrl Pts',(6.34668181342273,2.35510383058447,102.415926315209));
#208971=CARTESIAN_POINT('Ctrl Pts',(6.27952541914262,2.52872390822053,102.424675371408));
#208972=CARTESIAN_POINT('Ctrl Pts',(6.20533299175744,2.69928350889762,102.433424427607));
#208973=CARTESIAN_POINT('Ctrl Pts',(6.12831602991782,2.87633637965127,102.442506563766));
#208974=CARTESIAN_POINT('Ctrl Pts',(6.04371690605507,3.05009086600993,102.451588699924));
#208975=CARTESIAN_POINT('Ctrl Pts',(5.9518452031687,3.21991112882293,102.460670836082));
#208976=CARTESIAN_POINT('Ctrl Pts',(5.86333549509518,3.38351691182596,102.469420616426));
#208977=CARTESIAN_POINT('Ctrl Pts',(5.76807618099615,3.54347103711603,102.478170396769));
#208978=CARTESIAN_POINT('Ctrl Pts',(5.66639083309265,3.69923018027314,102.486920177113));
#208979=CARTESIAN_POINT('Ctrl Pts',(5.56470914082457,3.8549837238168,102.495669642898));
#208980=CARTESIAN_POINT('Ctrl Pts',(5.4566020337233,4.0065423470164,102.504419108683));
#208981=CARTESIAN_POINT('Ctrl Pts',(5.34243669839485,4.15339127986323,102.513168574468));
#208982=CARTESIAN_POINT('Ctrl Pts',(5.22827486050865,4.30023571400948,102.521917772214));
#208983=CARTESIAN_POINT('Ctrl Pts',(5.10805534167387,4.44237052028152,102.53066696996));
#208984=CARTESIAN_POINT('Ctrl Pts',(4.9821864434023,4.57931296628418,102.539416167706));
#208985=CARTESIAN_POINT('Ctrl Pts',(4.85632073219889,4.71625194483049,102.548165143917));
#208986=CARTESIAN_POINT('Ctrl Pts',(4.72480612170645,4.84799861524189,102.556914120129));
#208987=CARTESIAN_POINT('Ctrl Pts',(4.58808925235663,4.9741055489816,102.56566309634));
#208988=CARTESIAN_POINT('Ctrl Pts',(4.45136349474412,5.10022068120889,102.574412641342));
#208989=CARTESIAN_POINT('Ctrl Pts',(4.30943501210456,5.22069514871523,102.583162186344));
#208990=CARTESIAN_POINT('Ctrl Pts',(4.1627858743217,5.33511975165954,102.591911731346));
#208991=CARTESIAN_POINT('Ctrl Pts',(4.01614535740839,5.44953762807554,102.600660761999));
#208992=CARTESIAN_POINT('Ctrl Pts',(3.86478496658317,5.5579061753251,102.609409792653));
#208993=CARTESIAN_POINT('Ctrl Pts',(3.70921874747592,5.65985735539096,102.618158823307));
#208994=CARTESIAN_POINT('Ctrl Pts',(3.55365041606298,5.76180991976801,102.626907972756));
#208995=CARTESIAN_POINT('Ctrl Pts',(3.3938763817492,5.85734478552583,102.635657122206));
#208996=CARTESIAN_POINT('Ctrl Pts',(3.23043927904936,5.94613749121016,102.644406271656));
#208997=CARTESIAN_POINT('Ctrl Pts',(3.186917670707,5.96978206944005,102.646736079572));
#208998=CARTESIAN_POINT('Ctrl Pts',(3.14313645919771,5.99294880633353,102.649065887488));
#208999=CARTESIAN_POINT('Ctrl Pts',(3.09910619832148,6.01563211736933,102.651395695404));
#209000=CARTESIAN_POINT('Origin',(0.,0.,4.30282021618968));
#209001=CARTESIAN_POINT('',(3.09910619832126,6.01563211736944,105.045908754666));
#209002=CARTESIAN_POINT('',(3.09910619832133,6.0156321173694,104.651395695404));
#209003=CARTESIAN_POINT('',(3.09910619832133,6.0156321173694,4.30282021618968));
#209004=CARTESIAN_POINT('',(-6.76699971567252,0.00196165442175408,103.697179783839));
#209005=CARTESIAN_POINT('Ctrl Pts',(-6.76699971567252,0.0019616544219389,
103.697179783839));
#209006=CARTESIAN_POINT('Ctrl Pts',(-6.76704929032538,-0.169053004476753,
103.705273455863));
#209007=CARTESIAN_POINT('Ctrl Pts',(-6.76061186475369,-0.340348538486266,
103.713367127887));
#209008=CARTESIAN_POINT('Ctrl Pts',(-6.74764967260861,-0.511383315864874,
103.72146079991));
#209009=CARTESIAN_POINT('Ctrl Pts',(-6.734702167456,-0.682224299905047,
103.729545301286));
#209010=CARTESIAN_POINT('Ctrl Pts',(-6.71524463675656,-0.852804748767579,
103.737629802663));
#209011=CARTESIAN_POINT('Ctrl Pts',(-6.68929126238576,-1.02258075816513,
103.745714304039));
#209012=CARTESIAN_POINT('Ctrl Pts',(-6.6633616594919,-1.19220126460439,
103.753791400576));
#209013=CARTESIAN_POINT('Ctrl Pts',(-6.63094811150644,-1.36101843350394,
103.761868497114));
#209014=CARTESIAN_POINT('Ctrl Pts',(-6.59211675840777,-1.52849129651413,
103.769945593652));
#209015=CARTESIAN_POINT('Ctrl Pts',(-6.55331254905335,-1.69584709328275,
103.778017044169));
#209016=CARTESIAN_POINT('Ctrl Pts',(-6.50809954936712,-1.86186009455973,
103.786088494685));
#209017=CARTESIAN_POINT('Ctrl Pts',(-6.45659533533666,-2.02599745204897,
103.794159945202));
#209018=CARTESIAN_POINT('Ctrl Pts',(-6.40511251921879,-2.19006661712142,
103.802228042358));
#209019=CARTESIAN_POINT('Ctrl Pts',(-6.347343800751,-2.35226133528762,103.810296139515));
#209020=CARTESIAN_POINT('Ctrl Pts',(-6.28345717847996,-2.51206187945453,
103.818364236671));
#209021=CARTESIAN_POINT('Ctrl Pts',(-6.21958362568529,-2.67182973274875,
103.826430683312));
#209022=CARTESIAN_POINT('Ctrl Pts',(-6.1495947971142,-2.82920404177331,
103.834497129954));
#209023=CARTESIAN_POINT('Ctrl Pts',(-6.07370756813553,-2.98368318974605,
103.842563576596));
#209024=CARTESIAN_POINT('Ctrl Pts',(-5.99782097043651,-3.13816105266013,
103.850629956135));
#209025=CARTESIAN_POINT('Ctrl Pts',(-5.91603623378747,-3.28974346894448,
103.858696335675));
#209026=CARTESIAN_POINT('Ctrl Pts',(-5.82861704916746,-3.43795175855543,
103.866762715214));
#209027=CARTESIAN_POINT('Ctrl Pts',(-5.74118143383553,-3.58618790438264,
103.874830610856));
#209028=CARTESIAN_POINT('Ctrl Pts',(-5.64810945175457,-3.73104834150695,
103.882898506497));
#209029=CARTESIAN_POINT('Ctrl Pts',(-5.54970906004895,-3.87208191401094,
103.890966402138));
#209030=CARTESIAN_POINT('Ctrl Pts',(-5.45121910266651,-4.01324385762359,
103.899041641312));
#209031=CARTESIAN_POINT('Ctrl Pts',(-5.34739126114274,-4.15057167410523,
103.907116880486));
#209032=CARTESIAN_POINT('Ctrl Pts',(-5.23857531030885,-4.28364537727186,
103.915192119661));
#209033=CARTESIAN_POINT('Ctrl Pts',(-5.12970795282688,-4.41678194689304,
103.923271173726));
#209034=CARTESIAN_POINT('Ctrl Pts',(-5.01584803700327,-4.5456601212334,
103.931350227791));
#209035=CARTESIAN_POINT('Ctrl Pts',(-4.89738310684792,-4.66989589870702,
103.939429281856));
#209036=CARTESIAN_POINT('Ctrl Pts',(-4.77875699930115,-4.794300705095,103.947519327873));
#209037=CARTESIAN_POINT('Ctrl Pts',(-4.65551362731212,-4.91405023814169,
103.955609373891));
#209038=CARTESIAN_POINT('Ctrl Pts',(-4.52807532787225,-5.02879934229978,
103.963699419908));
#209039=CARTESIAN_POINT('Ctrl Pts',(-4.42271068898769,-5.12367268865706,
103.970388184439));
#209040=CARTESIAN_POINT('Ctrl Pts',(-4.31447916453073,-5.21512852071409,
103.97707694897));
#209041=CARTESIAN_POINT('Ctrl Pts',(-4.20363434417333,-5.30299418258086,
103.983765713501));
#209042=CARTESIAN_POINT('Ctrl Pts',(-4.05554974021816,-5.4203794757939,
103.992701656952));
#209043=CARTESIAN_POINT('Ctrl Pts',(-3.9024511963491,-5.53163332063073,
104.001637600403));
#209044=CARTESIAN_POINT('Ctrl Pts',(-3.74484820815153,-5.63634641393734,
104.010573543853));
#209045=CARTESIAN_POINT('Ctrl Pts',(-3.58748213904692,-5.74090209569122,
104.019496054211));
#209046=CARTESIAN_POINT('Ctrl Pts',(-3.42562535140029,-5.83893650253526,
104.028418564569));
#209047=CARTESIAN_POINT('Ctrl Pts',(-3.25981822702301,-5.93008213490914,
104.037341074926));
#209048=CARTESIAN_POINT('Ctrl Pts',(-3.09441738155513,-6.02100443219862,
104.046241722365));
#209049=CARTESIAN_POINT('Ctrl Pts',(-2.92508574388218,-6.10507151961483,
104.055142369803));
#209050=CARTESIAN_POINT('Ctrl Pts',(-2.75238975770195,-6.18196082337129,
104.064043017241));
#209051=CARTESIAN_POINT('Ctrl Pts',(-2.57996065185501,-6.25873130419812,
104.072929909828));
#209052=CARTESIAN_POINT('Ctrl Pts',(-2.40417780321668,-6.32834602325587,
104.081816802414));
#209053=CARTESIAN_POINT('Ctrl Pts',(-2.22563183148763,-6.39052829980973,
104.090703695));
#209054=CARTESIAN_POINT('Ctrl Pts',(-2.04754478955433,-6.45255074470118,
104.099567744955));
#209055=CARTESIAN_POINT('Ctrl Pts',(-1.86670903970273,-6.50717878343272,
104.10843179491));
#209056=CARTESIAN_POINT('Ctrl Pts',(-1.68373400925483,-6.55418406714968,
104.117295844865));
#209057=CARTESIAN_POINT('Ctrl Pts',(-1.50879516082221,-6.59912489969697,
104.125770589685));
#209058=CARTESIAN_POINT('Ctrl Pts',(-1.33190114540597,-6.63709805455192,
104.134245334506));
#209059=CARTESIAN_POINT('Ctrl Pts',(-1.15360166401145,-6.66794512580825,
104.142720079326));
#209060=CARTESIAN_POINT('Ctrl Pts',(-0.980894967051109,-6.69782460580401,
104.150928993755));
#209061=CARTESIAN_POINT('Ctrl Pts',(-0.807035907377264,-6.72098828375315,
104.159137908184));
#209062=CARTESIAN_POINT('Ctrl Pts',(-0.632584836163848,-6.7373678410085,
104.167346822613));
#209063=CARTESIAN_POINT('Ctrl Pts',(-0.45809229009454,-6.75375129242037,
104.17555768867));
#209064=CARTESIAN_POINT('Ctrl Pts',(-0.283007806606332,-6.76334737652044,
104.183768554727));
#209065=CARTESIAN_POINT('Ctrl Pts',(-0.107895395442345,-6.76613978451837,
104.191979420784));
#209066=CARTESIAN_POINT('Ctrl Pts',(0.067289862329342,-6.76893335415555,
104.200193702554));
#209067=CARTESIAN_POINT('Ctrl Pts',(0.242502715178607,-6.76491760341774,
104.208407984323));
#209068=CARTESIAN_POINT('Ctrl Pts',(0.41718053097064,-6.75412832307612,
104.216622266093));
#209069=CARTESIAN_POINT('Ctrl Pts',(0.592054960434044,-6.74332689854774,
104.224845793686));
#209070=CARTESIAN_POINT('Ctrl Pts',(0.766392794454234,-6.72573673845055,
104.233069321278));
#209071=CARTESIAN_POINT('Ctrl Pts',(0.939636913868471,-6.70144547617122,
104.24129284887));
#209072=CARTESIAN_POINT('Ctrl Pts',(1.11299207602382,-6.67713864413774,
104.249521647424));
#209073=CARTESIAN_POINT('Ctrl Pts',(1.28525177658029,-6.64612221075652,
104.257750445978));
#209074=CARTESIAN_POINT('Ctrl Pts',(1.45587048673085,-6.60853464285889,
104.265979244531));
#209075=CARTESIAN_POINT('Ctrl Pts',(1.62672403988286,-6.57089533868185,
104.274219369368));
#209076=CARTESIAN_POINT('Ctrl Pts',(1.79593174760206,-6.52666692393174,
104.282459494204));
#209077=CARTESIAN_POINT('Ctrl Pts',(1.96296362499377,-6.4760375853566,104.290699619041));
#209078=CARTESIAN_POINT('Ctrl Pts',(2.03711888540524,-6.45356024842471,
104.294357894411));
#209079=CARTESIAN_POINT('Ctrl Pts',(2.11084555593323,-6.42982192959471,
104.298016169781));
#209080=CARTESIAN_POINT('Ctrl Pts',(2.18409864199947,-6.40484208408108,
104.301674445151));
#209081=CARTESIAN_POINT('Ctrl Pts',(2.3532613418849,-6.34715634909395,104.310122467913));
#209082=CARTESIAN_POINT('Ctrl Pts',(2.52028415758831,-6.28271462300916,
104.318570490676));
#209083=CARTESIAN_POINT('Ctrl Pts',(2.68460881655648,-6.21169578312293,
104.327018513438));
#209084=CARTESIAN_POINT('Ctrl Pts',(2.84878299852662,-6.14074197730947,
104.335458800094));
#209085=CARTESIAN_POINT('Ctrl Pts',(3.01026364408896,-6.06322319471181,
104.34389908675));
#209086=CARTESIAN_POINT('Ctrl Pts',(3.16850999156815,-5.97936731045458,
104.352339373406));
#209087=CARTESIAN_POINT('Ctrl Pts',(3.3266357892767,-5.89557530639284,104.360773230374));
#209088=CARTESIAN_POINT('Ctrl Pts',(3.48153190691948,-5.80545597994448,
104.369207087342));
#209089=CARTESIAN_POINT('Ctrl Pts',(3.63267947922354,-5.70928443863399,
104.37764094431));
#209090=CARTESIAN_POINT('Ctrl Pts',(3.78373514595703,-5.61317137461322,
104.386069673055));
#209091=CARTESIAN_POINT('Ctrl Pts',(3.93104653099945,-5.51101361138082,
104.3944984018));
#209092=CARTESIAN_POINT('Ctrl Pts',(4.07412086986689,-5.40313132708386,
104.402927130545));
#209093=CARTESIAN_POINT('Ctrl Pts',(4.21713018301642,-5.29529807410197,
104.411352028525));
#209094=CARTESIAN_POINT('Ctrl Pts',(4.35590602398585,-5.18174568838335,
104.419776926505));
#209095=CARTESIAN_POINT('Ctrl Pts',(4.48998571657338,-5.06283687915847,
104.428201824485));
#209096=CARTESIAN_POINT('Ctrl Pts',(4.62403572369899,-4.94395439653726,
104.43662485718));
#209097=CARTESIAN_POINT('Ctrl Pts',(4.75339140443516,-4.81971807401098,
104.445047889874));
#209098=CARTESIAN_POINT('Ctrl Pts',(4.87762380648971,-4.69053035406071,
104.453470922568));
#209099=CARTESIAN_POINT('Ctrl Pts',(5.00184215178932,-4.56135725155395,
104.461893002206));
#209100=CARTESIAN_POINT('Ctrl Pts',(5.12093814295353,-4.42723410881617,
104.470315081843));
#209101=CARTESIAN_POINT('Ctrl Pts',(5.23452007913682,-4.28859983457463,
104.478737161481));
#209102=CARTESIAN_POINT('Ctrl Pts',(5.34810501884234,-4.1499618943353,104.487159463829));
#209103=CARTESIAN_POINT('Ctrl Pts',(5.45617540181385,-4.00681284295275,
104.495581766177));
#209104=CARTESIAN_POINT('Ctrl Pts',(5.55837994643813,-3.8596245116636,104.504004068525));
#209105=CARTESIAN_POINT('Ctrl Pts',(5.6606014615458,-3.71241174058912,104.512427769349));
#209106=CARTESIAN_POINT('Ctrl Pts',(5.75695500678292,-3.5611586266538,104.520851470173));
#209107=CARTESIAN_POINT('Ctrl Pts',(5.84713254406289,-3.40636610072385,
104.529275170996));
#209108=CARTESIAN_POINT('Ctrl Pts',(5.93737110530676,-3.25146882527647,
104.537704572215));
#209109=CARTESIAN_POINT('Ctrl Pts',(6.02142513918779,-3.09302764017662,
104.546133973434));
#209110=CARTESIAN_POINT('Ctrl Pts',(6.09903202398758,-2.93156909698099,
104.554563374653));
#209111=CARTESIAN_POINT('Ctrl Pts',(6.17666659881646,-2.77005294560062,
104.562995783471));
#209112=CARTESIAN_POINT('Ctrl Pts',(6.2478492989051,-2.60551759265549,104.571428192289));
#209113=CARTESIAN_POINT('Ctrl Pts',(6.31236539513704,-2.43851022517365,
104.579860601106));
#209114=CARTESIAN_POINT('Ctrl Pts',(6.37694118353806,-2.27134833761696,
104.588300811834));
#209115=CARTESIAN_POINT('Ctrl Pts',(6.43483792971866,-2.10171017917188,
104.596741022562));
#209116=CARTESIAN_POINT('Ctrl Pts',(6.48589022627108,-1.93015983088483,
104.605181233289));
#209117=CARTESIAN_POINT('Ctrl Pts',(6.51492790138721,-1.83258492013611,
104.609981881126));
#209118=CARTESIAN_POINT('Ctrl Pts',(6.54175222038416,-1.73439164339507,
104.614782528963));
#209119=CARTESIAN_POINT('Ctrl Pts',(6.56634009650628,-1.63568540282473,
104.6195831768));
#209120=CARTESIAN_POINT('Ctrl Pts',(6.6080299499784,-1.46832451790231,104.627722891833));
#209121=CARTESIAN_POINT('Ctrl Pts',(6.6433704814629,-1.29915463673605,104.635862606866));
#209122=CARTESIAN_POINT('Ctrl Pts',(6.67220489363832,-1.12870317502381,
104.644002321899));
#209123=CARTESIAN_POINT('Ctrl Pts',(6.70101408740983,-0.958400789137468,
104.652134917986));
#209124=CARTESIAN_POINT('Ctrl Pts',(6.72332842754207,-0.786819412381466,
104.660267514073));
#209125=CARTESIAN_POINT('Ctrl Pts',(6.73904139668091,-0.614499840375114,
104.66840011016));
#209126=CARTESIAN_POINT('Ctrl Pts',(6.75474362359105,-0.442298075273033,
104.676527146368));
#209127=CARTESIAN_POINT('Ctrl Pts',(6.76385343164389,-0.269359482892504,
104.684654182576));
#209128=CARTESIAN_POINT('Ctrl Pts',(6.76631570154596,-0.0962331908053344,
104.692781218783));
#209129=CARTESIAN_POINT('Ctrl Pts',(6.76877679443847,0.0768103437815226,
104.700904370121));
#209130=CARTESIAN_POINT('Ctrl Pts',(6.76459667171424,0.250041034011858,
104.709027521459));
#209131=CARTESIAN_POINT('Ctrl Pts',(6.75377220999347,0.422906532841329,
104.717150672796));
#209132=CARTESIAN_POINT('Ctrl Pts',(6.74295079002694,0.59572345518014,104.725271541468));
#209133=CARTESIAN_POINT('Ctrl Pts',(6.72548877363209,0.768175025394373,
104.733392410139));
#209134=CARTESIAN_POINT('Ctrl Pts',(6.7014351104815,0.939710838506064,104.741513278811));
#209135=CARTESIAN_POINT('Ctrl Pts',(6.6773801473788,1.11125592207034,104.749634586366));
#209136=CARTESIAN_POINT('Ctrl Pts',(6.6467328727442,1.28188478642956,104.75775589392));
#209137=CARTESIAN_POINT('Ctrl Pts',(6.60959390715445,1.4510538868377,104.765877201475));
#209138=CARTESIAN_POINT('Ctrl Pts',(6.59029520961563,1.53896003203717,104.770097315191));
#209139=CARTESIAN_POINT('Ctrl Pts',(6.56924446865013,1.62647215923695,104.774317428908));
#209140=CARTESIAN_POINT('Ctrl Pts',(6.5464612221734,1.71351523675161,104.778537542625));
#209141=CARTESIAN_POINT('Ctrl Pts',(6.49795668150834,1.89882616235804,104.787521981151));
#209142=CARTESIAN_POINT('Ctrl Pts',(6.44162091720304,2.08191852549232,104.796506419677));
#209143=CARTESIAN_POINT('Ctrl Pts',(6.37768797078266,2.26216381973856,104.805490858203));
#209144=CARTESIAN_POINT('Ctrl Pts',(6.3136446799129,2.44272020660387,104.814490803333));
#209145=CARTESIAN_POINT('Ctrl Pts',(6.24197807890539,2.62041947783379,104.823490748463));
#209146=CARTESIAN_POINT('Ctrl Pts',(6.16297031630131,2.79465308766382,104.832490693594));
#209147=CARTESIAN_POINT('Ctrl Pts',(6.08377636987625,2.9692972834686,104.841511847326));
#209148=CARTESIAN_POINT('Ctrl Pts',(5.99720674718061,3.14045925867974,104.850533001058));
#209149=CARTESIAN_POINT('Ctrl Pts',(5.90359083813182,3.30755260214044,104.859554154791));
#209150=CARTESIAN_POINT('Ctrl Pts',(5.80987967415799,3.47481596439463,104.868584487618));
#209151=CARTESIAN_POINT('Ctrl Pts',(5.70910802255661,3.6380022191138,104.877614820445));
#209152=CARTESIAN_POINT('Ctrl Pts',(5.60164951120217,3.79655261436589,104.886645153272));
#209153=CARTESIAN_POINT('Ctrl Pts',(5.49403865755124,3.95532778410088,104.895688288265));
#209154=CARTESIAN_POINT('Ctrl Pts',(5.37972212307625,4.10945375520907,104.904731423258));
#209155=CARTESIAN_POINT('Ctrl Pts',(5.25911622901807,4.25840175296774,104.91377455825));
#209156=CARTESIAN_POINT('Ctrl Pts',(5.15367889163944,4.38861661861916,104.92168034165));
#209157=CARTESIAN_POINT('Ctrl Pts',(5.04343541851787,4.51487448688405,104.92958612505));
#209158=CARTESIAN_POINT('Ctrl Pts',(4.92868823279422,4.63684389471069,104.93749190845));
#209159=CARTESIAN_POINT('Ctrl Pts',(4.79755503406507,4.77623065608998,104.946526645635));
#209160=CARTESIAN_POINT('Ctrl Pts',(4.66041770868393,4.91014402847871,104.955561382819));
#209161=CARTESIAN_POINT('Ctrl Pts',(4.51775470906506,5.03807318215213,104.964596120004));
#209162=CARTESIAN_POINT('Ctrl Pts',(4.38125891205211,5.16047206510353,104.973240293028));
#209163=CARTESIAN_POINT('Ctrl Pts',(4.23970535783228,5.27739295980276,104.981884466052));
#209164=CARTESIAN_POINT('Ctrl Pts',(4.09355174753297,5.38842491738261,104.990528639076));
#209165=CARTESIAN_POINT('Ctrl Pts',(3.94751050382896,5.49937151078282,104.999166166241));
#209166=CARTESIAN_POINT('Ctrl Pts',(3.79687649770736,5.60443801198851,105.007803693406));
#209167=CARTESIAN_POINT('Ctrl Pts',(3.64214091206989,5.70325333267134,105.016441220571));
#209168=CARTESIAN_POINT('Ctrl Pts',(3.48754311963719,5.80198065756663,105.025071055953));
#209169=CARTESIAN_POINT('Ctrl Pts',(3.32885129101073,5.89446774573588,105.033700891335));
#209170=CARTESIAN_POINT('Ctrl Pts',(3.16658630182934,5.98038629129146,105.042330726717));
#209171=CARTESIAN_POINT('Ctrl Pts',(3.14416066484509,5.99226056018066,105.0435234027));
#209172=CARTESIAN_POINT('Ctrl Pts',(3.12166682451649,6.00400943580988,105.044716078683));
#209173=CARTESIAN_POINT('Ctrl Pts',(3.09910619832126,6.01563211736944,105.045908754666));
#209174=CARTESIAN_POINT('Ctrl Pts',(3.09910619832139,6.01563211736937,103.045799558392));
#209175=CARTESIAN_POINT('Ctrl Pts',(2.94236430513783,6.09638169833182,103.054111211667));
#209176=CARTESIAN_POINT('Ctrl Pts',(2.78233017481925,6.17107055504067,103.062422864941));
#209177=CARTESIAN_POINT('Ctrl Pts',(2.61950763306529,6.2394285603982,103.070734518215));
#209178=CARTESIAN_POINT('Ctrl Pts',(2.45680390152898,6.30773668550323,103.079040106547));
#209179=CARTESIAN_POINT('Ctrl Pts',(2.29131613225174,6.36972302967539,103.087345694879));
#209180=CARTESIAN_POINT('Ctrl Pts',(2.12357116630314,6.42516416145502,103.095651283211));
#209181=CARTESIAN_POINT('Ctrl Pts',(1.9559178560199,6.48057500026106,103.103952333379));
#209182=CARTESIAN_POINT('Ctrl Pts',(1.78601013636463,6.52944764453699,103.112253383547));
#209183=CARTESIAN_POINT('Ctrl Pts',(1.61439338256553,6.57160733811209,103.120554433714));
#209184=CARTESIAN_POINT('Ctrl Pts',(1.44283895574051,6.61375172032585,103.128852469145));
#209185=CARTESIAN_POINT('Ctrl Pts',(1.26957706925807,6.64918792812348,103.137150504576));
#209186=CARTESIAN_POINT('Ctrl Pts',(1.09516698237773,6.67779142237235,103.145448540007));
#209187=CARTESIAN_POINT('Ctrl Pts',(0.917825849735268,6.70687561215953,
103.153886027932));
#209188=CARTESIAN_POINT('Ctrl Pts',(0.739297935222967,6.72889528581189,
103.162323515856));
#209189=CARTESIAN_POINT('Ctrl Pts',(0.560181124280923,6.74377387728854,
103.170761003781));
#209190=CARTESIAN_POINT('Ctrl Pts',(0.384014197523693,6.75840743245924,
103.179059534273));
#209191=CARTESIAN_POINT('Ctrl Pts',(0.207277979361667,6.76613330032755,
103.187358064766));
#209192=CARTESIAN_POINT('Ctrl Pts',(0.0305455202347726,6.76693106002962,
103.195656595258));
#209193=CARTESIAN_POINT('Ctrl Pts',(-0.14622375551021,6.7677289859197,103.203956854486));
#209194=CARTESIAN_POINT('Ctrl Pts',(-0.322988922558483,6.76159592535089,
103.212257113715));
#209195=CARTESIAN_POINT('Ctrl Pts',(-0.499177629272033,6.74856360231082,
103.220557372943));
#209196=CARTESIAN_POINT('Ctrl Pts',(-0.675432321873086,6.73552639842783,
103.22886074077));
#209197=CARTESIAN_POINT('Ctrl Pts',(-0.851109776893836,6.71558480798511,
103.237164108598));
#209198=CARTESIAN_POINT('Ctrl Pts',(-1.02564326441134,6.68882238470777,
103.245467476425));
#209199=CARTESIAN_POINT('Ctrl Pts',(-1.20515202141174,6.66129706904963,
103.254007540906));
#209200=CARTESIAN_POINT('Ctrl Pts',(-1.38345023086992,6.62655634228058,
103.262547605388));
#209201=CARTESIAN_POINT('Ctrl Pts',(-1.55993391594156,6.58474716127318,
103.271087669869));
#209202=CARTESIAN_POINT('Ctrl Pts',(-1.73182960695066,6.54402488115492,
103.279405720825));
#209203=CARTESIAN_POINT('Ctrl Pts',(-1.90200362431914,6.49659723332589,
103.287723771781));
#209204=CARTESIAN_POINT('Ctrl Pts',(-2.0699146776535,6.44265024871245,103.296041822737));
#209205=CARTESIAN_POINT('Ctrl Pts',(-2.24454819370229,6.3865434504035,103.304692893981));
#209206=CARTESIAN_POINT('Ctrl Pts',(-2.41673340417195,6.32338468216138,
103.313343965225));
#209207=CARTESIAN_POINT('Ctrl Pts',(-2.58588599787128,6.25343766307887,
103.321995036469));
#209208=CARTESIAN_POINT('Ctrl Pts',(-2.7550385915706,6.18349064399635,103.330646107713));
#209209=CARTESIAN_POINT('Ctrl Pts',(-2.92115821549834,6.1067556047809,103.339297178958));
#209210=CARTESIAN_POINT('Ctrl Pts',(-3.08369109684616,6.02354864006524,
103.347948250202));
#209211=CARTESIAN_POINT('Ctrl Pts',(-3.23530414982311,5.94593196432015,
103.356018096205));
#209212=CARTESIAN_POINT('Ctrl Pts',(-3.38426480533369,5.86244398788228,
103.364087942207));
#209213=CARTESIAN_POINT('Ctrl Pts',(-3.5300736531061,5.7732892707404,103.37215778821));
#209214=CARTESIAN_POINT('Ctrl Pts',(-3.67569905480191,5.68424672157268,
103.38021748132));
#209215=CARTESIAN_POINT('Ctrl Pts',(-3.81818022451315,5.58955180955035,
103.38827717443));
#209216=CARTESIAN_POINT('Ctrl Pts',(-3.95703853568271,5.48945671511508,
103.39633686754));
#209217=CARTESIAN_POINT('Ctrl Pts',(-4.09575262044103,5.38946558533365,
103.404388189379));
#209218=CARTESIAN_POINT('Ctrl Pts',(-4.23085103481182,5.28408565131226,
103.412439511218));
#209219=CARTESIAN_POINT('Ctrl Pts',(-4.36188064280269,5.17361442880538,
103.420490833056));
#209220=CARTESIAN_POINT('Ctrl Pts',(-4.49280286878587,5.06323374020031,
103.428535556637));
#209221=CARTESIAN_POINT('Ctrl Pts',(-4.61966264130249,4.94777030686426,
103.436580280218));
#209222=CARTESIAN_POINT('Ctrl Pts',(-4.74203676498044,4.82756422221122,
103.444625003799));
#209223=CARTESIAN_POINT('Ctrl Pts',(-4.86433738778352,4.70743033625609,
103.452664895524));
#209224=CARTESIAN_POINT('Ctrl Pts',(-4.98215745955112,4.58255973036248,
103.460704787248));
#209225=CARTESIAN_POINT('Ctrl Pts',(-5.09510787076625,4.45333187459186,
103.468744678972));
#209226=CARTESIAN_POINT('Ctrl Pts',(-5.21049041378296,4.32132138904337,
103.476957691592));
#209227=CARTESIAN_POINT('Ctrl Pts',(-5.3207908982104,4.1847641347449,103.485170704212));
#209228=CARTESIAN_POINT('Ctrl Pts',(-5.42563495129075,4.04410365536447,
103.493383716832));
#209229=CARTESIAN_POINT('Ctrl Pts',(-5.5282332020267,3.90645618077615,103.501420803375));
#209230=CARTESIAN_POINT('Ctrl Pts',(-5.62560618959596,3.76487980538032,
103.509457889917));
#209231=CARTESIAN_POINT('Ctrl Pts',(-5.71744473488568,3.61982246850975,
103.51749497646));
#209232=CARTESIAN_POINT('Ctrl Pts',(-5.80929206955164,3.47475124897689,
103.525532832189));
#209233=CARTESIAN_POINT('Ctrl Pts',(-5.89560370729836,3.32619872024178,
103.533570687918));
#209234=CARTESIAN_POINT('Ctrl Pts',(-5.97611480369843,3.17464027143493,
103.541608543648));
#209235=CARTESIAN_POINT('Ctrl Pts',(-6.05664955732139,3.0230372889903,103.549648761205));
#209236=CARTESIAN_POINT('Ctrl Pts',(-6.13138020182837,2.86842695816172,
103.557688978762));
#209237=CARTESIAN_POINT('Ctrl Pts',(-6.20008876476533,2.71130749068245,
103.565729196319));
#209238=CARTESIAN_POINT('Ctrl Pts',(-6.27139318123286,2.54825194905253,
103.574073178446));
#209239=CARTESIAN_POINT('Ctrl Pts',(-6.33621141358448,2.38249438169519,
103.582417160574));
#209240=CARTESIAN_POINT('Ctrl Pts',(-6.39435583166184,2.21461113925045,
103.590761142702));
#209241=CARTESIAN_POINT('Ctrl Pts',(-6.45048102793904,2.05255809537398,
103.598815357537));
#209242=CARTESIAN_POINT('Ctrl Pts',(-6.50038812801885,1.88852491222502,
103.606869572372));
#209243=CARTESIAN_POINT('Ctrl Pts',(-6.54396024116556,1.72304189213275,
103.614923787207));
#209244=CARTESIAN_POINT('Ctrl Pts',(-6.58756496083387,1.55743503536424,
103.62298402929));
#209245=CARTESIAN_POINT('Ctrl Pts',(-6.62482517347593,1.39037654348746,
103.631044271373));
#209246=CARTESIAN_POINT('Ctrl Pts',(-6.65567557661696,1.2224040325623,103.639104513456));
#209247=CARTESIAN_POINT('Ctrl Pts',(-6.68656911073776,1.05419668454476,
103.647176024311));
#209248=CARTESIAN_POINT('Ctrl Pts',(-6.71103490292835,0.885073134178257,
103.655247535165));
#209249=CARTESIAN_POINT('Ctrl Pts',(-6.72905960490018,0.715573779355196,
103.663319046019));
#209250=CARTESIAN_POINT('Ctrl Pts',(-6.7309487818599,0.697808477253693,
103.66416502463));
#209251=CARTESIAN_POINT('Ctrl Pts',(-6.73276724909369,0.680039044307874,
103.665011003241));
#209252=CARTESIAN_POINT('Ctrl Pts',(-6.73451502427644,0.662266100442202,
103.665856981852));
#209253=CARTESIAN_POINT('Ctrl Pts',(-6.75608578867897,0.442915243049773,
103.676297915838));
#209254=CARTESIAN_POINT('Ctrl Pts',(-6.76693576375581,0.222572616147481,
103.686738849824));
#209255=CARTESIAN_POINT('Ctrl Pts',(-6.76699971567234,0.00196165502752502,
103.69717978381));
#209256=CARTESIAN_POINT('',(-6.767,-8.20588493674615E-10,103.302820216229));
#209257=CARTESIAN_POINT('Ctrl Pts',(3.09910619832148,6.01563211736933,102.651395695404));
#209258=CARTESIAN_POINT('Ctrl Pts',(2.93375330764841,6.10081787314646,102.660145143307));
#209259=CARTESIAN_POINT('Ctrl Pts',(2.76488627843085,6.17918207037032,102.668894591209));
#209260=CARTESIAN_POINT('Ctrl Pts',(2.59307866646717,6.25045854553991,102.677644039111));
#209261=CARTESIAN_POINT('Ctrl Pts',(2.42127244185387,6.32173444515033,102.686393416361));
#209262=CARTESIAN_POINT('Ctrl Pts',(2.2465259467247,6.38592262741836,102.695142793612));
#209263=CARTESIAN_POINT('Ctrl Pts',(2.06943269687121,6.44280508110562,102.703892170862));
#209264=CARTESIAN_POINT('Ctrl Pts',(1.89234081822078,6.49968709436166,102.712641480367));
#209265=CARTESIAN_POINT('Ctrl Pts',(1.7129024940559,6.54926340459544,102.721390789873));
#209266=CARTESIAN_POINT('Ctrl Pts',(1.53172716625061,6.59136563150383,102.730140099378));
#209267=CARTESIAN_POINT('Ctrl Pts',(1.35055318107354,6.63346754640705,102.738889344045));
#209268=CARTESIAN_POINT('Ctrl Pts',(1.16764249714457,6.66809542395769,102.747638588713));
#209269=CARTESIAN_POINT('Ctrl Pts',(0.983616340614903,6.6951316562466,102.75638783338));
#209270=CARTESIAN_POINT('Ctrl Pts',(0.799591486714394,6.72216769715954,
102.765137016116));
#209271=CARTESIAN_POINT('Ctrl Pts',(0.614451459527268,6.74161215869366,
102.773886198851));
#209272=CARTESIAN_POINT('Ctrl Pts',(0.428825047910842,6.75339900185709,
102.782635381587));
#209273=CARTESIAN_POINT('Ctrl Pts',(0.243199888597644,6.76518576550218,
102.791384505298));
#209274=CARTESIAN_POINT('Ctrl Pts',(0.057088637392555,6.76931499599834,
102.800133629008));
#209275=CARTESIAN_POINT('Ctrl Pts',(-0.128876626810473,6.76577266947848,
102.808882752719));
#209276=CARTESIAN_POINT('Ctrl Pts',(-0.314840698187551,6.76223036567996,
102.81763182031));
#209277=CARTESIAN_POINT('Ctrl Pts',(-0.500658497950714,6.75101660879227,
102.826380887902));
#209278=CARTESIAN_POINT('Ctrl Pts',(-0.685698951925747,6.73216948296223,
102.835129955493));
#209279=CARTESIAN_POINT('Ctrl Pts',(-0.870738280459417,6.71332247176299,
102.843878969872));
#209280=CARTESIAN_POINT('Ctrl Pts',(-1.05499998761211,6.68684221356193,
102.85262798425));
#209281=CARTESIAN_POINT('Ctrl Pts',(-1.23785829161383,6.65281863948529,
102.861376998629));
#209282=CARTESIAN_POINT('Ctrl Pts',(-1.43007412917363,6.6170539536887,102.870573732328));
#209283=CARTESIAN_POINT('Ctrl Pts',(-1.62073882535748,6.57295372727801,
102.879770466027));
#209284=CARTESIAN_POINT('Ctrl Pts',(-1.80913696091466,6.52068343478293,
102.888967199726));
#209285=CARTESIAN_POINT('Ctrl Pts',(-1.98838356186064,6.47095219815213,
102.89771719744));
#209286=CARTESIAN_POINT('Ctrl Pts',(-2.16557827572486,6.41382586850907,
102.906467195154));
#209287=CARTESIAN_POINT('Ctrl Pts',(-2.34011918621653,6.34949849943295,
102.915217192867));
#209288=CARTESIAN_POINT('Ctrl Pts',(-2.51465655691045,6.28517243495572,
102.923967013126));
#209289=CARTESIAN_POINT('Ctrl Pts',(-2.68653996295269,6.213645722424,102.932716833384));
#209290=CARTESIAN_POINT('Ctrl Pts',(-2.85518555379923,6.13516132252251,
102.941466653642));
#209291=CARTESIAN_POINT('Ctrl Pts',(-3.02382794858626,6.05667841000538,
102.95021630808));
#209292=CARTESIAN_POINT('Ctrl Pts',(-3.1892323910922,5.97123819492113,102.958965962517));
#209293=CARTESIAN_POINT('Ctrl Pts',(-3.3508370596764,5.87913088810746,102.967715616955));
#209294=CARTESIAN_POINT('Ctrl Pts',(-3.51243888042337,5.78702520443141,
102.976465117204));
#209295=CARTESIAN_POINT('Ctrl Pts',(-3.67024081223624,5.68825280605826,
102.985214617453));
#209296=CARTESIAN_POINT('Ctrl Pts',(-3.82370687544332,5.58314917682552,
102.993964117702));
#209297=CARTESIAN_POINT('Ctrl Pts',(-3.97717043817743,5.47804726008073,
103.002713475392));
#209298=CARTESIAN_POINT('Ctrl Pts',(-4.12629803722387,5.36661448084292,
103.011462833083));
#209299=CARTESIAN_POINT('Ctrl Pts',(-4.27058317206833,5.24922931204638,
103.020212190773));
#209300=CARTESIAN_POINT('Ctrl Pts',(-4.41486614774765,5.13184589986851,
103.028961417533));
#209301=CARTESIAN_POINT('Ctrl Pts',(-4.55430658194349,5.00851045723093,
103.037710644293));
#209302=CARTESIAN_POINT('Ctrl Pts',(-4.68843089001786,4.87964187103176,
103.046459871053));
#209303=CARTESIAN_POINT('Ctrl Pts',(-4.82255336917795,4.75077504208004,
103.055208978509));
#209304=CARTESIAN_POINT('Ctrl Pts',(-4.95135966065109,4.61637541908121,
103.063958085965));
#209305=CARTESIAN_POINT('Ctrl Pts',(-5.07441230869235,4.47689945401855,
103.072707193421));
#209306=CARTESIAN_POINT('Ctrl Pts',(-5.19746344226414,4.3374252055552,103.081456193197));
#209307=CARTESIAN_POINT('Ctrl Pts',(-5.31476088454769,4.19287495491334,
103.090205192974));
#209308=CARTESIAN_POINT('Ctrl Pts',(-5.42590627628861,4.04373961586696,
103.09895419275));
#209309=CARTESIAN_POINT('Ctrl Pts',(-5.53706380672676,3.89458798906723,
103.107704148045));
#209310=CARTESIAN_POINT('Ctrl Pts',(-5.64206777071873,3.7408505015527,103.11645410334));
#209311=CARTESIAN_POINT('Ctrl Pts',(-5.74056148164017,3.58304938223145,
103.125204058634));
#209312=CARTESIAN_POINT('Ctrl Pts',(-5.83905138951896,3.42525435593261,
103.133953676075));
#209313=CARTESIAN_POINT('Ctrl Pts',(-5.93103139557668,3.26339625497156,
103.142703293516));
#209314=CARTESIAN_POINT('Ctrl Pts',(-6.01618907820863,3.09802485064971,
103.151452910958));
#209315=CARTESIAN_POINT('Ctrl Pts',(-6.10134392544994,2.93265895249617,
103.160202237073));
#209316=CARTESIAN_POINT('Ctrl Pts',(-6.17967677261837,2.76378023986023,
103.168951563189));
#209317=CARTESIAN_POINT('Ctrl Pts',(-6.25092157009224,2.59196229227116,
103.177700889305));
#209318=CARTESIAN_POINT('Ctrl Pts',(-6.32216437407745,2.4201491522911,103.186449970608));
#209319=CARTESIAN_POINT('Ctrl Pts',(-6.38631941548907,2.2453972066289,103.19519905191));
#209320=CARTESIAN_POINT('Ctrl Pts',(-6.44316881037518,2.06829994947746,
103.203948133213));
#209321=CARTESIAN_POINT('Ctrl Pts',(-6.50002334524552,1.89118668024516,
103.212698005555));
#209322=CARTESIAN_POINT('Ctrl Pts',(-6.54957082411077,1.71172794807774,
103.221447877897));
#209323=CARTESIAN_POINT('Ctrl Pts',(-6.59164294296065,1.53053334250419,
103.23019775024));
#209324=CARTESIAN_POINT('Ctrl Pts',(-6.63371214082118,1.34935131693678,
103.238947015094));
#209325=CARTESIAN_POINT('Ctrl Pts',(-6.66830695239676,1.16643393829841,
103.247696279949));
#209326=CARTESIAN_POINT('Ctrl Pts',(-6.69530988153977,0.982402458341761,
103.256445544804));
#209327=CARTESIAN_POINT('Ctrl Pts',(-6.72231419690474,0.798361530947849,
103.265195258811));
#209328=CARTESIAN_POINT('Ctrl Pts',(-6.7417258082927,0.613206671363285,
103.273944972818));
#209329=CARTESIAN_POINT('Ctrl Pts',(-6.75347878028174,0.427566795114224,
103.282694686825));
#209330=CARTESIAN_POINT('Ctrl Pts',(-6.76248992368206,0.285234494207036,
103.289403196614));
#209331=CARTESIAN_POINT('Ctrl Pts',(-6.76699999999989,0.142617266094836,
103.296111706402));
#209332=CARTESIAN_POINT('Ctrl Pts',(-6.767,5.08377026670387E-12,103.30282021619));
#209333=CARTESIAN_POINT('Ctrl Pts',(-6.767,-8.20396992685389E-10,103.302820216229));
#209334=CARTESIAN_POINT('Ctrl Pts',(-6.76699999997745,-0.18600725034739,
103.31156972804));
#209335=CARTESIAN_POINT('Ctrl Pts',(-6.75932637290009,-0.372014356569628,
103.320319239851));
#209336=CARTESIAN_POINT('Ctrl Pts',(-6.7440051825742,-0.557389538305465,
103.329068751662));
#209337=CARTESIAN_POINT('Ctrl Pts',(-6.72868405696075,-0.742763937068103,
103.337818226518));
#209338=CARTESIAN_POINT('Ctrl Pts',(-6.7057154563447,-0.927506131055983,
103.346567701374));
#209339=CARTESIAN_POINT('Ctrl Pts',(-6.67517739391316,-1.11098864071181,
103.355317176229));
#209340=CARTESIAN_POINT('Ctrl Pts',(-6.6446394579296,-1.29447039062751,
103.364066614856));
#209341=CARTESIAN_POINT('Ctrl Pts',(-6.60653216990395,-1.47669218394034,
103.372816053483));
#209342=CARTESIAN_POINT('Ctrl Pts',(-6.56098496072521,-1.65703510679093,
103.38156549211));
#209343=CARTESIAN_POINT('Ctrl Pts',(-6.51543793635944,-1.83737729787963,
103.390314895236));
#209344=CARTESIAN_POINT('Ctrl Pts',(-6.46245112142894,-2.01584035589556,
103.399064298361));
#209345=CARTESIAN_POINT('Ctrl Pts',(-6.40220448347582,-2.19181813838697,
103.407813701486));
#209346=CARTESIAN_POINT('Ctrl Pts',(-6.34195808497692,-2.36779522144313,
103.416563069836));
#209347=CARTESIAN_POINT('Ctrl Pts',(-6.27445201402183,-2.5412867776051,
103.425312438186));
#209348=CARTESIAN_POINT('Ctrl Pts',(-6.19991555038909,-2.71170355460246,
103.434061806536));
#209349=CARTESIAN_POINT('Ctrl Pts',(-6.12537937681621,-2.88211966842015,
103.442811140838));
#209350=CARTESIAN_POINT('Ctrl Pts',(-6.04381298015407,-3.04946076445341,
103.45156047514));
#209351=CARTESIAN_POINT('Ctrl Pts',(-5.9554933929672,-3.21315848447038,
103.460309809442));
#209352=CARTESIAN_POINT('Ctrl Pts',(-5.86717414214314,-3.37685558104894,
103.469059110422));
#209353=CARTESIAN_POINT('Ctrl Pts',(-5.77210188833564,-3.53690907716986,
103.477808411402));
#209354=CARTESIAN_POINT('Ctrl Pts',(-5.67059953302075,-3.69277537038267,
103.486557712382));
#209355=CARTESIAN_POINT('Ctrl Pts',(-5.56909755584588,-3.84864108292636,
103.495306980767));
#209356=CARTESIAN_POINT('Ctrl Pts',(-5.46116568148233,-4.00031938363886,
103.504056249153));
#209357=CARTESIAN_POINT('Ctrl Pts',(-5.34717048483224,-4.14729511924808,
103.512805517538));
#209358=CARTESIAN_POINT('Ctrl Pts',(-5.23317570339677,-4.2942703195148,
103.521554754055));
#209359=CARTESIAN_POINT('Ctrl Pts',(-5.11311781949632,-4.43654276251646,
103.530303990572));
#209360=CARTESIAN_POINT('Ctrl Pts',(-4.98740458929211,-4.57362924412419,
103.539053227089));
#209361=CARTESIAN_POINT('Ctrl Pts',(-4.86169180654557,-4.71071523779284,
103.547802432465));
#209362=CARTESIAN_POINT('Ctrl Pts',(-4.73032391145408,-4.84261509580638,
103.55655163784));
#209363=CARTESIAN_POINT('Ctrl Pts',(-4.59374706953327,-4.96888084594052,
103.565300843215));
#209364=CARTESIAN_POINT('Ctrl Pts',(-4.45717070239636,-5.09514615713534,
103.574050018176));
#209365=CARTESIAN_POINT('Ctrl Pts',(-4.31538563507762,-5.21577720511883,
103.582799193136));
#209366=CARTESIAN_POINT('Ctrl Pts',(-4.16887340964834,-5.33036429283469,
103.591548368097));
#209367=CARTESIAN_POINT('Ctrl Pts',(-4.02236168137632,-5.44495099172427,
103.600297513369));
#209368=CARTESIAN_POINT('Ctrl Pts',(-3.87112305280765,-5.55349359485584,
103.609046658641));
#209369=CARTESIAN_POINT('Ctrl Pts',(-3.71567116949112,-5.65562346343995,
103.617795803913));
#209370=CARTESIAN_POINT('Ctrl Pts',(-3.56021980075929,-5.75775299394859,
103.626544920223));
#209371=CARTESIAN_POINT('Ctrl Pts',(-3.40055544467297,-5.8534696750515,
103.635294036533));
#209372=CARTESIAN_POINT('Ctrl Pts',(-3.2372203591472,-5.94244843026197,
103.644043152843));
#209373=CARTESIAN_POINT('Ctrl Pts',(-3.07388580073972,-6.03142689831839,
103.652792240918));
#209374=CARTESIAN_POINT('Ctrl Pts',(-2.90688078822377,-6.11366734692062,
103.661541328993));
#209375=CARTESIAN_POINT('Ctrl Pts',(-2.73677250646261,-6.18889046985567,
103.670290417068));
#209376=CARTESIAN_POINT('Ctrl Pts',(-2.5666647595545,-6.26411335627481,
103.679039477634));
#209377=CARTESIAN_POINT('Ctrl Pts',(-2.39345402498295,-6.33231884529611,
103.6877885382));
#209378=CARTESIAN_POINT('Ctrl Pts',(-2.2177285598797,-6.39327529789653,
103.696537598766));
#209379=CARTESIAN_POINT('Ctrl Pts',(-2.04200363270099,-6.45423156389922,
103.70528663255));
#209380=CARTESIAN_POINT('Ctrl Pts',(-1.86376426110157,-6.50793874398319,
103.714035666333));
#209381=CARTESIAN_POINT('Ctrl Pts',(-1.68361577673416,-6.55421443930025,
103.722784700117));
#209382=CARTESIAN_POINT('Ctrl Pts',(-1.50346782887536,-6.6004899968015,
103.731533707845));
#209383=CARTESIAN_POINT('Ctrl Pts',(-1.32141105714289,-6.63933404253772,
103.740282715573));
#209384=CARTESIAN_POINT('Ctrl Pts',(-1.13806375405982,-6.67061465621387,
103.749031723301));
#209385=CARTESIAN_POINT('Ctrl Pts',(-0.954716981788821,-6.70189517932895,
103.757780705699));
#209386=CARTESIAN_POINT('Ctrl Pts',(-0.770079968085066,-6.72561226601584,
103.766529688097));
#209387=CARTESIAN_POINT('Ctrl Pts',(-0.584779764739224,-6.74168536990207,
103.775278670496));
#209388=CARTESIAN_POINT('Ctrl Pts',(-0.391489829838794,-6.75845151018535,
103.784404889505));
#209389=CARTESIAN_POINT('Ctrl Pts',(-0.197478577433421,-6.7668998303395,
103.793531108515));
#209390=CARTESIAN_POINT('Ctrl Pts',(-0.0034628756550048,-6.76699911397159,
103.802657327524));
#209391=CARTESIAN_POINT('Ctrl Pts',(0.184489835442792,-6.76709529499017,
103.81149835219));
#209392=CARTESIAN_POINT('Ctrl Pts',(0.372446405029021,-6.75935639733849,
103.820339376855));
#209393=CARTESIAN_POINT('Ctrl Pts',(0.559755020257901,-6.74380925866799,
103.82918040152));
#209394=CARTESIAN_POINT('Ctrl Pts',(0.745134706289568,-6.72842222651303,
103.83793038013));
#209395=CARTESIAN_POINT('Ctrl Pts',(0.929879431993717,-6.70538706046913,
103.84668035874));
#209396=CARTESIAN_POINT('Ctrl Pts',(1.1133616370299,-6.67478200881423,103.85543033735));
#209397=CARTESIAN_POINT('Ctrl Pts',(1.29684196376553,-6.64417727046211,
103.864180226386));
#209398=CARTESIAN_POINT('Ctrl Pts',(1.47905951292928,-6.60600284873705,
103.872930115423));
#209399=CARTESIAN_POINT('Ctrl Pts',(1.65939532142,-6.56038841588281,103.881680004459));
#209400=CARTESIAN_POINT('Ctrl Pts',(1.83972934375199,-6.51477443482247,
103.890429806831));
#209401=CARTESIAN_POINT('Ctrl Pts',(2.01818138480058,-6.46172066039093,
103.899179609204));
#209402=CARTESIAN_POINT('Ctrl Pts',(2.19414528427307,-6.4014073039842,103.907929411576));
#209403=CARTESIAN_POINT('Ctrl Pts',(2.3701074993642,-6.34109452491574,103.916679130192));
#209404=CARTESIAN_POINT('Ctrl Pts',(2.5435813493811,-6.27352239587453,103.925428848808));
#209405=CARTESIAN_POINT('Ctrl Pts',(2.71397759506356,-6.19892043935821,
103.934178567425));
#209406=CARTESIAN_POINT('Ctrl Pts',(2.8843722662808,-6.12431917216568,103.942928205193));
#209407=CARTESIAN_POINT('Ctrl Pts',(3.05168912749988,-6.04268832243936,
103.951677842962));
#209408=CARTESIAN_POINT('Ctrl Pts',(3.21535986341885,-5.95430516086597,
103.960427480731));
#209409=CARTESIAN_POINT('Ctrl Pts',(3.3790291413987,-5.8659227865883,103.96917704056));
#209410=CARTESIAN_POINT('Ctrl Pts',(3.5390521068752,-5.77078835701498,103.977926600389));
#209411=CARTESIAN_POINT('Ctrl Pts',(3.69488522896492,-5.66922500389399,
103.986676160218));
#209412=CARTESIAN_POINT('Ctrl Pts',(3.85071701470592,-5.56766252173071,
103.995425645015));
#209413=CARTESIAN_POINT('Ctrl Pts',(4.00235878884838,-5.45967138283602,
104.004175129812));
#209414=CARTESIAN_POINT('Ctrl Pts',(4.14929549672471,-5.34561838152145,
104.012924614609));
#209415=CARTESIAN_POINT('Ctrl Pts',(4.29623099335929,-5.23156632037875,
104.021674027282));
#209416=CARTESIAN_POINT('Ctrl Pts',(4.4384612749449,-5.11145267254199,104.030423439955));
#209417=CARTESIAN_POINT('Ctrl Pts',(4.57550326111464,-4.98568539997555,
104.039172852627));
#209418=CARTESIAN_POINT('Ctrl Pts',(4.71254416313363,-4.85991912236464,
104.047922196082));
#209419=CARTESIAN_POINT('Ctrl Pts',(4.84439664072839,-4.72849950330015,
104.056671539538));
#209420=CARTESIAN_POINT('Ctrl Pts',(4.9706128684726,-4.59187289804222,104.065420882993));
#209421=CARTESIAN_POINT('Ctrl Pts',(5.09682813963641,-4.45524732826391,
104.074170160138));
#209422=CARTESIAN_POINT('Ctrl Pts',(5.21740705197177,-4.31341506176109,
104.082919437283));
#209423=CARTESIAN_POINT('Ctrl Pts',(5.33194007593362,-4.16685781214731,
104.091668714427));
#209424=CARTESIAN_POINT('Ctrl Pts',(5.44647226990471,-4.02030162459543,
104.100417928168));
#209425=CARTESIAN_POINT('Ctrl Pts',(5.55495848672365,-3.86902074824399,
104.10916714191));
#209426=CARTESIAN_POINT('Ctrl Pts',(5.65703027334258,-3.71352898015965,
104.117916355651));
#209427=CARTESIAN_POINT('Ctrl Pts',(5.75910135417682,-3.55803828723734,
104.126665508895));
#209428=CARTESIAN_POINT('Ctrl Pts',(5.85475793631605,-3.39833700039775,
104.135414662138));
#209429=CARTESIAN_POINT('Ctrl Pts',(5.94367514464377,-3.23496750755612,
104.144163815382));
#209430=CARTESIAN_POINT('Ctrl Pts',(6.03259176767751,-3.07159909008767,
104.152912911035));
#209431=CARTESIAN_POINT('Ctrl Pts',(6.11476896869126,-2.90456276661537,
104.161662006688));
#209432=CARTESIAN_POINT('Ctrl Pts',(6.18992765579143,-2.73442582932294,
104.170411102341));
#209433=CARTESIAN_POINT('Ctrl Pts',(6.26508587312365,-2.56428995544558,
104.179160143309));
#209434=CARTESIAN_POINT('Ctrl Pts',(6.3332255485449,-2.39105376862813,104.187909184277));
#209435=CARTESIAN_POINT('Ctrl Pts',(6.3941152675835,-2.21530560980998,104.196658225245));
#209436=CARTESIAN_POINT('Ctrl Pts',(6.45500462626153,-2.03955849111338,
104.205407214434));
#209437=CARTESIAN_POINT('Ctrl Pts',(6.50864402062003,-1.8612997009019,104.214156203623));
#209438=CARTESIAN_POINT('Ctrl Pts',(6.55485128387801,-1.68113463061194,
104.222905192812));
#209439=CARTESIAN_POINT('Ctrl Pts',(6.60199809571025,-1.49730620043037,
104.231832078283));
#209440=CARTESIAN_POINT('Ctrl Pts',(6.64140720722179,-1.31149343173021,
104.240758963754));
#209441=CARTESIAN_POINT('Ctrl Pts',(6.67293928734917,-1.1243532662611,104.249685849224));
#209442=CARTESIAN_POINT('Ctrl Pts',(6.70384625886327,-0.940923066289126,
104.258435763402));
#209443=CARTESIAN_POINT('Ctrl Pts',(6.72718554587889,-0.756217898801698,
104.267185677579));
#209444=CARTESIAN_POINT('Ctrl Pts',(6.74287786821437,-0.570865180532846,
104.275935591757));
#209445=CARTESIAN_POINT('Ctrl Pts',(6.75856988194971,-0.385516107350657,
104.284685333861));
#209446=CARTESIAN_POINT('Ctrl Pts',(6.76661520775538,-0.199519794502239,
104.293435075966));
#209447=CARTESIAN_POINT('Ctrl Pts',(6.76698651789723,-0.013508019731541,
104.30218481807));
#209448=CARTESIAN_POINT('Ctrl Pts',(6.76735782123057,0.172500344237066,
104.310934399735));
#209449=CARTESIAN_POINT('Ctrl Pts',(6.76005538991348,0.358523882934203,
104.3196839814));
#209450=CARTESIAN_POINT('Ctrl Pts',(6.74510402736542,0.543930749286017,
104.328433563065));
#209451=CARTESIAN_POINT('Ctrl Pts',(6.73015291910227,0.729334462335302,
104.337182995922));
#209452=CARTESIAN_POINT('Ctrl Pts',(6.70755316296814,0.914121238352356,
104.345932428778));
#209453=CARTESIAN_POINT('Ctrl Pts',(6.67738151862829,1.09766345237569,104.354681861635));
#209454=CARTESIAN_POINT('Ctrl Pts',(6.64721034733862,1.28120278870779,104.363431157313));
#209455=CARTESIAN_POINT('Ctrl Pts',(6.60946757189487,1.4634973193103,104.37218045299));
#209456=CARTESIAN_POINT('Ctrl Pts',(6.5642813809394,1.6439279034837,104.380929748668));
#209457=CARTESIAN_POINT('Ctrl Pts',(6.51909583840338,1.8243558984878,104.389678918793));
#209458=CARTESIAN_POINT('Ctrl Pts',(6.46646716371454,2.00291972261425,104.398428088919));
#209459=CARTESIAN_POINT('Ctrl Pts',(6.40657409849579,2.17901292343182,104.407177259044));
#209460=CARTESIAN_POINT('Ctrl Pts',(6.34668181316888,2.35510383126856,104.415926315244));
#209461=CARTESIAN_POINT('Ctrl Pts',(6.27952541887005,2.52872390889741,104.424675371443));
#209462=CARTESIAN_POINT('Ctrl Pts',(6.20533299146647,2.69928350956653,104.433424427642));
#209463=CARTESIAN_POINT('Ctrl Pts',(6.12831602961987,2.87633638028405,104.442506563799));
#209464=CARTESIAN_POINT('Ctrl Pts',(6.04371690575289,3.05009086660679,104.451588699955));
#209465=CARTESIAN_POINT('Ctrl Pts',(5.95184520286494,3.21991112938442,104.460670836112));
#209466=CARTESIAN_POINT('Ctrl Pts',(5.86333549477603,3.38351691237901,104.469420616456));
#209467=CARTESIAN_POINT('Ctrl Pts',(5.76807618066197,3.54347103766002,104.478170396799));
#209468=CARTESIAN_POINT('Ctrl Pts',(5.66639083274382,3.69923018080746,104.486920177143));
#209469=CARTESIAN_POINT('Ctrl Pts',(5.56470914046111,3.85498372434145,104.495669642928));
#209470=CARTESIAN_POINT('Ctrl Pts',(5.45660203334561,4.00654234753078,104.504419108713));
#209471=CARTESIAN_POINT('Ctrl Pts',(5.34243669800338,4.15339128036677,104.513168574498));
#209472=CARTESIAN_POINT('Ctrl Pts',(5.22827486010339,4.30023571450219,104.521917772244));
#209473=CARTESIAN_POINT('Ctrl Pts',(5.10805534125529,4.44237052076283,104.53066696999));
#209474=CARTESIAN_POINT('Ctrl Pts',(4.98218644297088,4.57931296675355,104.539416167736));
#209475=CARTESIAN_POINT('Ctrl Pts',(4.85632073175437,4.71625194528822,104.548165143947));
#209476=CARTESIAN_POINT('Ctrl Pts',(4.72480612124931,4.84799861568743,104.556914120159));
#209477=CARTESIAN_POINT('Ctrl Pts',(4.58808925188738,4.97410554941444,104.565663096371));
#209478=CARTESIAN_POINT('Ctrl Pts',(4.45136349426295,5.10022068162884,104.574412641372));
#209479=CARTESIAN_POINT('Ctrl Pts',(4.309435011612,5.22069514912182,104.583162186374));
#209480=CARTESIAN_POINT('Ctrl Pts',(4.16278587381831,5.33511975205231,104.591911731376));
#209481=CARTESIAN_POINT('Ctrl Pts',(4.01614535689419,5.44953762845449,104.600660762029));
#209482=CARTESIAN_POINT('Ctrl Pts',(3.86478496605872,5.55790617568979,104.609409792683));
#209483=CARTESIAN_POINT('Ctrl Pts',(3.70921874694181,5.65985735574099,104.618158823337));
#209484=CARTESIAN_POINT('Ctrl Pts',(3.55365041551934,5.76180992010331,104.626907972786));
#209485=CARTESIAN_POINT('Ctrl Pts',(3.39387638119663,5.857344785846,104.635657122236));
#209486=CARTESIAN_POINT('Ctrl Pts',(3.2304392784885,5.94613749151487,104.644406271686));
#209487=CARTESIAN_POINT('Ctrl Pts',(3.18691767033081,5.96978206963911,104.646736079592));
#209488=CARTESIAN_POINT('Ctrl Pts',(3.14313645900847,5.99294880643102,104.649065887498));
#209489=CARTESIAN_POINT('Ctrl Pts',(3.09910619832133,6.0156321173694,104.651395695404));
#209490=CARTESIAN_POINT('Origin',(0.,0.,4.30282021618968));
#209491=CARTESIAN_POINT('',(3.09910619832138,6.01563211736938,107.045755263024));
#209492=CARTESIAN_POINT('',(3.09910619832136,6.01563211736939,106.651504649108));
#209493=CARTESIAN_POINT('',(3.09910619832133,6.0156321173694,4.30282021618968));
#209494=CARTESIAN_POINT('',(-6.76699890702215,0.00271959186415095,105.69717978381));
#209495=CARTESIAN_POINT('Ctrl Pts',(-6.767,5.0761025263598E-12,105.69717978381));
#209496=CARTESIAN_POINT('Ctrl Pts',(-6.76700000000014,-0.186007249521759,
105.705929295621));
#209497=CARTESIAN_POINT('Ctrl Pts',(-6.75932637294548,-0.372014355744774,
105.714678807432));
#209498=CARTESIAN_POINT('Ctrl Pts',(-6.74400518264223,-0.557389537482324,
105.723428319244));
#209499=CARTESIAN_POINT('Ctrl Pts',(-6.72868405705141,-0.742763936246801,
105.732177794099));
#209500=CARTESIAN_POINT('Ctrl Pts',(-6.70571545645792,-0.927506130237453,
105.740927268955));
#209501=CARTESIAN_POINT('Ctrl Pts',(-6.67517739404878,-1.11098863989697,
105.749676743811));
#209502=CARTESIAN_POINT('Ctrl Pts',(-6.64463945808762,-1.29447038981637,
105.758426182438));
#209503=CARTESIAN_POINT('Ctrl Pts',(-6.60653217008422,-1.47669218313383,
105.767175621065));
#209504=CARTESIAN_POINT('Ctrl Pts',(-6.56098496092751,-1.65703510598994,
105.775925059692));
#209505=CARTESIAN_POINT('Ctrl Pts',(-6.51543793658379,-1.83737729708406,
105.784674462817));
#209506=CARTESIAN_POINT('Ctrl Pts',(-6.46245112167513,-2.0158403551063,
105.793423865942));
#209507=CARTESIAN_POINT('Ctrl Pts',(-6.40220448374356,-2.19181813760493,
105.802173269067));
#209508=CARTESIAN_POINT('Ctrl Pts',(-6.34195808526612,-2.36779522066854,
105.810922637417));
#209509=CARTESIAN_POINT('Ctrl Pts',(-6.27445201433218,-2.54128677683884,
105.819672005767));
#209510=CARTESIAN_POINT('Ctrl Pts',(-6.19991555072021,-2.71170355384539,
105.828421374117));
#209511=CARTESIAN_POINT('Ctrl Pts',(-6.12537937716821,-2.88211966767204,
105.837170708419));
#209512=CARTESIAN_POINT('Ctrl Pts',(-6.04381298052658,-3.04946076371513,
105.845920042721));
#209513=CARTESIAN_POINT('Ctrl Pts',(-5.95549339335978,-3.21315848374275,
105.854669377023));
#209514=CARTESIAN_POINT('Ctrl Pts',(-5.86717414255561,-3.37685558033229,
105.863418678003));
#209515=CARTESIAN_POINT('Ctrl Pts',(-5.77210188876755,-3.53690907646502,
105.872167978983));
#209516=CARTESIAN_POINT('Ctrl Pts',(-5.67059953347156,-3.69277536969041,
105.880917279963));
#209517=CARTESIAN_POINT('Ctrl Pts',(-5.56909755631545,-3.8486410822469,
105.889666548349));
#209518=CARTESIAN_POINT('Ctrl Pts',(-5.46116568197013,-4.00031938297295,
105.898415816734));
#209519=CARTESIAN_POINT('Ctrl Pts',(-5.34717048533766,-4.14729511859644,
105.907165085119));
#209520=CARTESIAN_POINT('Ctrl Pts',(-5.23317570392011,-4.29427031887703,
105.915914321636));
#209521=CARTESIAN_POINT('Ctrl Pts',(-5.11311782003702,-4.43654276189331,
105.924663558153));
#209522=CARTESIAN_POINT('Ctrl Pts',(-4.98740458984954,-4.57362924351634,
105.93341279467));
#209523=CARTESIAN_POINT('Ctrl Pts',(-4.86169180711956,-4.71071523720047,
105.942162000046));
#209524=CARTESIAN_POINT('Ctrl Pts',(-4.73032391204397,-4.84261509523018,
105.950911205421));
#209525=CARTESIAN_POINT('Ctrl Pts',(-4.59374707013837,-4.9688808453811,
105.959660410797));
#209526=CARTESIAN_POINT('Ctrl Pts',(-4.45717070301705,-5.09514615659236,
105.968409585757));
#209527=CARTESIAN_POINT('Ctrl Pts',(-4.31538563571323,-5.21577720459293,
105.977158760717));
#209528=CARTESIAN_POINT('Ctrl Pts',(-4.16887341029814,-5.33036429232648,
105.985907935678));
#209529=CARTESIAN_POINT('Ctrl Pts',(-4.02236168204012,-5.4449509912339,
105.99465708095));
#209530=CARTESIAN_POINT('Ctrl Pts',(-3.87112305348471,-5.55349359438389,
106.003406226222));
#209531=CARTESIAN_POINT('Ctrl Pts',(-3.71567117018065,-5.65562346298694,
106.012155371494));
#209532=CARTESIAN_POINT('Ctrl Pts',(-3.56021980146119,-5.75775299351459,
106.020904487804));
#209533=CARTESIAN_POINT('Ctrl Pts',(-3.40055544538645,-5.85346967463701,
106.029653604114));
#209534=CARTESIAN_POINT('Ctrl Pts',(-3.23722035987143,-5.94244842986743,
106.038402720425));
#209535=CARTESIAN_POINT('Ctrl Pts',(-3.07388580147449,-6.03142689794393,
106.047151808499));
#209536=CARTESIAN_POINT('Ctrl Pts',(-2.90688078896824,-6.11366734656666,
106.055900896574));
#209537=CARTESIAN_POINT('Ctrl Pts',(-2.73677250721591,-6.18889046952256,
106.064649984649));
#209538=CARTESIAN_POINT('Ctrl Pts',(-2.56666476031699,-6.26411335596239,
106.073399045215));
#209539=CARTESIAN_POINT('Ctrl Pts',(-2.39345402575377,-6.33231884500476,
106.082148105781));
#209540=CARTESIAN_POINT('Ctrl Pts',(-2.21772856065797,-6.39327529762656,
106.090897166347));
#209541=CARTESIAN_POINT('Ctrl Pts',(-2.04200363348683,-6.45423156365059,
106.099646200131));
#209542=CARTESIAN_POINT('Ctrl Pts',(-1.8637642618941,-6.50793874375622,
106.108395233915));
#209543=CARTESIAN_POINT('Ctrl Pts',(-1.68361577753247,-6.55421443909518,
106.117144267698));
#209544=CARTESIAN_POINT('Ctrl Pts',(-1.50346782967897,-6.60048999661846,
106.125893275426));
#209545=CARTESIAN_POINT('Ctrl Pts',(-1.32141105795088,-6.63933404237692,
106.134642283154));
#209546=CARTESIAN_POINT('Ctrl Pts',(-1.13806375487127,-6.67061465607543,
106.143391290882));
#209547=CARTESIAN_POINT('Ctrl Pts',(-0.954716982603977,-6.70189517921283,
106.15214027328));
#209548=CARTESIAN_POINT('Ctrl Pts',(-0.770079968903007,-6.72561226592218,
106.160889255679));
#209549=CARTESIAN_POINT('Ctrl Pts',(-0.584779765559023,-6.74168536983096,
106.169638238077));
#209550=CARTESIAN_POINT('Ctrl Pts',(-0.391489830652104,-6.75845151013848,
106.178764457087));
#209551=CARTESIAN_POINT('Ctrl Pts',(-0.197478578239171,-6.76689983031623,
106.187890676097));
#209552=CARTESIAN_POINT('Ctrl Pts',(-0.00346287645220683,-6.76699911397118,
106.197016895107));
#209553=CARTESIAN_POINT('Ctrl Pts',(0.184489834653883,-6.76709529501191,
106.205857919772));
#209554=CARTESIAN_POINT('Ctrl Pts',(0.372446404249327,-6.75935639738168,
106.214698944438));
#209555=CARTESIAN_POINT('Ctrl Pts',(0.559755019488257,-6.74380925873187,
106.223539969104));
#209556=CARTESIAN_POINT('Ctrl Pts',(0.74513470552165,-6.72842222659807,
106.232289947714));
#209557=CARTESIAN_POINT('Ctrl Pts',(0.9298794312284,-6.70538706057526,106.241039926324));
#209558=CARTESIAN_POINT('Ctrl Pts',(1.11336163626804,-6.67478200894131,
106.249789904933));
#209559=CARTESIAN_POINT('Ctrl Pts',(1.29684196300714,-6.64417727061014,
106.25853979397));
#209560=CARTESIAN_POINT('Ctrl Pts',(1.47905951217522,-6.60600284890588,
106.267289683006));
#209561=CARTESIAN_POINT('Ctrl Pts',(1.65939532067112,-6.56038841607224,
106.276039572043));
#209562=CARTESIAN_POINT('Ctrl Pts',(1.83972934300828,-6.51477443503249,
106.284789374415));
#209563=CARTESIAN_POINT('Ctrl Pts',(2.0181813840629,-6.46172066062133,106.293539176787));
#209564=CARTESIAN_POINT('Ctrl Pts',(2.19414528354225,-6.4014073042347,106.302288979159));
#209565=CARTESIAN_POINT('Ctrl Pts',(2.37010749864023,-6.34109452518633,
106.311038697776));
#209566=CARTESIAN_POINT('Ctrl Pts',(2.54358134866482,-6.27352239616495,
106.319788416392));
#209567=CARTESIAN_POINT('Ctrl Pts',(2.71397759435577,-6.1989204396681,106.328538135008));
#209568=CARTESIAN_POINT('Ctrl Pts',(2.88437226558162,-6.12431917249498,
106.337287772777));
#209569=CARTESIAN_POINT('Ctrl Pts',(3.0516891268101,-6.04268832278772,106.346037410546));
#209570=CARTESIAN_POINT('Ctrl Pts',(3.21535986273924,-5.95430516123296,
106.354787048314));
#209571=CARTESIAN_POINT('Ctrl Pts',(3.37902914072916,-5.86592278697398,
106.363536608144));
#209572=CARTESIAN_POINT('Ctrl Pts',(3.5390521062165,-5.77078835741894,106.372286167973));
#209573=CARTESIAN_POINT('Ctrl Pts',(3.69488522831778,-5.66922500431577,
106.381035727802));
#209574=CARTESIAN_POINT('Ctrl Pts',(3.85071701407023,-5.56766252217036,
106.389785212599));
#209575=CARTESIAN_POINT('Ctrl Pts',(4.0023587882249,-5.45967138329307,106.398534697396));
#209576=CARTESIAN_POINT('Ctrl Pts',(4.14929549611414,-5.34561838199538,
106.407284182193));
#209577=CARTESIAN_POINT('Ctrl Pts',(4.29623099276182,-5.2315663208694,106.416033594866));
#209578=CARTESIAN_POINT('Ctrl Pts',(4.43846127436122,-5.11145267304882,
106.424783007538));
#209579=CARTESIAN_POINT('Ctrl Pts',(4.57550326054539,-4.98568540049796,
106.433532420211));
#209580=CARTESIAN_POINT('Ctrl Pts',(4.71254416257872,-4.85991912290272,
106.442281763666));
#209581=CARTESIAN_POINT('Ctrl Pts',(4.84439664018847,-4.72849950385331,
106.451031107121));
#209582=CARTESIAN_POINT('Ctrl Pts',(4.97061286794825,-4.59187289860981,
106.459780450577));
#209583=CARTESIAN_POINT('Ctrl Pts',(5.09682813912764,-4.45524732884594,
106.468529727721));
#209584=CARTESIAN_POINT('Ctrl Pts',(5.21740705147918,-4.31341506235692,
106.477279004866));
#209585=CARTESIAN_POINT('Ctrl Pts',(5.33194007545775,-4.16685781275623,
106.486028282011));
#209586=CARTESIAN_POINT('Ctrl Pts',(5.44647226944556,-4.02030162521746,
106.494777495752));
#209587=CARTESIAN_POINT('Ctrl Pts',(5.55495848628176,-3.86902074887843,
106.503526709493));
#209588=CARTESIAN_POINT('Ctrl Pts',(5.65703027291843,-3.71352898080578,
106.512275923234));
#209589=CARTESIAN_POINT('Ctrl Pts',(5.75910135377042,-3.55803828789515,
106.521025076478));
#209590=CARTESIAN_POINT('Ctrl Pts',(5.85475793592787,-3.39833700106652,
106.529774229722));
#209591=CARTESIAN_POINT('Ctrl Pts',(5.94367514427424,-3.23496750823506,
106.538523382966));
#209592=CARTESIAN_POINT('Ctrl Pts',(6.03259176732663,-3.0715990907768,106.547272478619));
#209593=CARTESIAN_POINT('Ctrl Pts',(6.11476896835944,-2.90456276731392,
106.556021574272));
#209594=CARTESIAN_POINT('Ctrl Pts',(6.18992765547904,-2.7344258300301,106.564770669925));
#209595=CARTESIAN_POINT('Ctrl Pts',(6.26508587283073,-2.56428995616123,
106.573519710893));
#209596=CARTESIAN_POINT('Ctrl Pts',(6.33322554827181,-2.39105376935148,
106.582268751861));
#209597=CARTESIAN_POINT('Ctrl Pts',(6.39411526733052,-2.21530561054019,
106.591017792829));
#209598=CARTESIAN_POINT('Ctrl Pts',(6.4550046260286,-2.03955849185057,106.599766782018));
#209599=CARTESIAN_POINT('Ctrl Pts',(6.50864402040746,-1.86129970164524,
106.608515771207));
#209600=CARTESIAN_POINT('Ctrl Pts',(6.55485128368601,-1.6811346313606,106.617264760396));
#209601=CARTESIAN_POINT('Ctrl Pts',(6.60199809554324,-1.49730620116879,
106.626191645867));
#209602=CARTESIAN_POINT('Ctrl Pts',(6.64140720707869,-1.31149343245718,
106.635118531339));
#209603=CARTESIAN_POINT('Ctrl Pts',(6.67293928722879,-1.12435326697554,
106.64404541681));
#209604=CARTESIAN_POINT('Ctrl Pts',(6.70384625876252,-0.940923067006904,
106.652795330988));
#209605=CARTESIAN_POINT('Ctrl Pts',(6.72718554579792,-0.756217899522007,
106.661545245165));
#209606=CARTESIAN_POINT('Ctrl Pts',(6.74287786815325,-0.570865181254865,
106.670295159343));
#209607=CARTESIAN_POINT('Ctrl Pts',(6.75856988190843,-0.385516108074387,
106.679044901447));
#209608=CARTESIAN_POINT('Ctrl Pts',(6.76661520773401,-0.199519795226859,
106.687794643552));
#209609=CARTESIAN_POINT('Ctrl Pts',(6.76698651789579,-0.0135080204562311,
106.696544385656));
#209610=CARTESIAN_POINT('Ctrl Pts',(6.76735782124904,0.172500343512306,
106.705293967321));
#209611=CARTESIAN_POINT('Ctrl Pts',(6.76005538995187,0.358523882210194,
106.714043548986));
#209612=CARTESIAN_POINT('Ctrl Pts',(6.74510402742368,0.54393074856358,106.722793130651));
#209613=CARTESIAN_POINT('Ctrl Pts',(6.73015291918039,0.729334461614436,
106.731542563508));
#209614=CARTESIAN_POINT('Ctrl Pts',(6.70755316306606,0.91412123763388,106.740291996364));
#209615=CARTESIAN_POINT('Ctrl Pts',(6.67738151874587,1.09766345166042,106.749041429221));
#209616=CARTESIAN_POINT('Ctrl Pts',(6.64721034747585,1.28120278799584,106.757790724899));
#209617=CARTESIAN_POINT('Ctrl Pts',(6.60946757205159,1.46349731860249,106.766540020576));
#209618=CARTESIAN_POINT('Ctrl Pts',(6.56428138111543,1.64392790278083,106.775289316254));
#209619=CARTESIAN_POINT('Ctrl Pts',(6.51909583859873,1.82435589778973,106.784038486379));
#209620=CARTESIAN_POINT('Ctrl Pts',(6.46646716392902,2.00291972192179,106.792787656505));
#209621=CARTESIAN_POINT('Ctrl Pts',(6.40657409872914,2.17901292274575,106.80153682663));
#209622=CARTESIAN_POINT('Ctrl Pts',(6.3466818134211,2.35510383058887,106.810285882829));
#209623=CARTESIAN_POINT('Ctrl Pts',(6.27952541914087,2.52872390822489,106.819034939029));
#209624=CARTESIAN_POINT('Ctrl Pts',(6.20533299175557,2.69928350890193,106.827783995228));
#209625=CARTESIAN_POINT('Ctrl Pts',(6.12831602991588,2.87633637965541,106.836866131386));
#209626=CARTESIAN_POINT('Ctrl Pts',(6.04371690605307,3.0500908660139,106.845948267544));
#209627=CARTESIAN_POINT('Ctrl Pts',(5.95184520316665,3.21991112882672,106.855030403702));
#209628=CARTESIAN_POINT('Ctrl Pts',(5.86333549509308,3.38351691182958,106.863780184046));
#209629=CARTESIAN_POINT('Ctrl Pts',(5.76807618099402,3.54347103711949,106.872529964389));
#209630=CARTESIAN_POINT('Ctrl Pts',(5.66639083309049,3.69923018027644,106.881279744733));
#209631=CARTESIAN_POINT('Ctrl Pts',(5.56470914082232,3.85498372382004,106.890029210518));
#209632=CARTESIAN_POINT('Ctrl Pts',(5.45660203372097,4.00654234701958,106.898778676303));
#209633=CARTESIAN_POINT('Ctrl Pts',(5.34243669839244,4.15339127986634,106.907528142088));
#209634=CARTESIAN_POINT('Ctrl Pts',(5.22827486050622,4.30023571401242,106.916277339834));
#209635=CARTESIAN_POINT('Ctrl Pts',(5.10805534167145,4.4423705202843,106.92502653758));
#209636=CARTESIAN_POINT('Ctrl Pts',(4.98218644339989,4.5793129662868,106.933775735326));
#209637=CARTESIAN_POINT('Ctrl Pts',(4.8563207321964,4.71625194483304,106.942524711537));
#209638=CARTESIAN_POINT('Ctrl Pts',(4.7248061217039,4.84799861524438,106.951273687749));
#209639=CARTESIAN_POINT('Ctrl Pts',(4.58808925235401,4.97410554898402,106.960022663961));
#209640=CARTESIAN_POINT('Ctrl Pts',(4.45136349474143,5.10022068121123,106.968772208962));
#209641=CARTESIAN_POINT('Ctrl Pts',(4.30943501210181,5.22069514871751,106.977521753964));
#209642=CARTESIAN_POINT('Ctrl Pts',(4.16278587431888,5.33511975166174,106.986271298966));
#209643=CARTESIAN_POINT('Ctrl Pts',(4.01614535740551,5.44953762807766,106.995020329619));
#209644=CARTESIAN_POINT('Ctrl Pts',(3.86478496658024,5.55790617532714,107.003769360273));
#209645=CARTESIAN_POINT('Ctrl Pts',(3.70921874747293,5.65985735539292,107.012518390927));
#209646=CARTESIAN_POINT('Ctrl Pts',(3.55365041605993,5.76180991976989,107.021267540377));
#209647=CARTESIAN_POINT('Ctrl Pts',(3.39387638174611,5.85734478552762,107.030016689826));
#209648=CARTESIAN_POINT('Ctrl Pts',(3.23043927904622,5.94613749121187,107.038765839276));
#209649=CARTESIAN_POINT('Ctrl Pts',(3.18691767070485,5.96978206944118,107.041095647192));
#209650=CARTESIAN_POINT('Ctrl Pts',(3.14313645919658,5.99294880633411,107.043425455108));
#209651=CARTESIAN_POINT('Ctrl Pts',(3.09910619832137,6.01563211736938,107.045755263024));
#209652=CARTESIAN_POINT('Ctrl Pts',(3.09910619832126,6.01563211736944,105.045908754666));
#209653=CARTESIAN_POINT('Ctrl Pts',(2.93603787272548,6.09964092122308,105.054529422988));
#209654=CARTESIAN_POINT('Ctrl Pts',(2.76947833120977,6.17705310480651,105.063150091309));
#209655=CARTESIAN_POINT('Ctrl Pts',(2.59997745762146,6.24759203372469,105.071770759631));
#209656=CARTESIAN_POINT('Ctrl Pts',(2.4382529009184,6.31489479605329,105.079995931179));
#209657=CARTESIAN_POINT('Ctrl Pts',(2.2738510884678,6.37594069435382,105.088221102727));
#209658=CARTESIAN_POINT('Ctrl Pts',(2.10726897706669,6.43052925180287,105.096446274275));
#209659=CARTESIAN_POINT('Ctrl Pts',(1.9366406840343,6.48644373324562,105.104871230408));
#209660=CARTESIAN_POINT('Ctrl Pts',(1.76379950164895,6.53555832413088,105.113296186541));
#209661=CARTESIAN_POINT('Ctrl Pts',(1.58931484550919,6.57771748571221,105.121721142675));
#209662=CARTESIAN_POINT('Ctrl Pts',(1.41478968980506,6.61988643283982,105.130148054321));
#209663=CARTESIAN_POINT('Ctrl Pts',(1.23862062209066,6.655096653863,105.138574965967));
#209664=CARTESIAN_POINT('Ctrl Pts',(1.0613883661554,6.68324350418193,105.147001877614));
#209665=CARTESIAN_POINT('Ctrl Pts',(0.884090935017014,6.71140070519395,
105.155431888164));
#209666=CARTESIAN_POINT('Ctrl Pts',(0.705729863433054,6.73248930439252,
105.163861898714));
#209667=CARTESIAN_POINT('Ctrl Pts',(0.526892519575836,6.74645634928553,
105.172291909264));
#209668=CARTESIAN_POINT('Ctrl Pts',(0.347890434496955,6.76043626032824,
105.180729685363));
#209669=CARTESIAN_POINT('Ctrl Pts',(0.168411531428975,6.76728148447363,
105.189167461463));
#209670=CARTESIAN_POINT('Ctrl Pts',(-0.0109541556863898,6.76699113391419,
105.197605237562));
#209671=CARTESIAN_POINT('Ctrl Pts',(-0.190413996565524,6.76670063094211,
105.206047442872));
#209672=CARTESIAN_POINT('Ctrl Pts',(-0.369760171767688,6.75926709135523,
105.214489648182));
#209673=CARTESIAN_POINT('Ctrl Pts',(-0.548405656251683,6.74474167305103,
105.222931853492));
#209674=CARTESIAN_POINT('Ctrl Pts',(-0.727239601892981,6.73020093122968,
105.231382964864));
#209675=CARTESIAN_POINT('Ctrl Pts',(-0.905371050717434,6.70855340028196,
105.239834076236));
#209676=CARTESIAN_POINT('Ctrl Pts',(-1.08222000645191,6.67990185988052,
105.248285187608));
#209677=CARTESIAN_POINT('Ctrl Pts',(-1.13185293981417,6.67186076068622,
105.250657005105));
#209678=CARTESIAN_POINT('Ctrl Pts',(-1.18138492736455,6.66326829616464,
105.253028822602));
#209679=CARTESIAN_POINT('Ctrl Pts',(-1.23080332752517,6.65412745361501,
105.2554006401));
#209680=CARTESIAN_POINT('Ctrl Pts',(-1.40407841213977,6.62207703795834,
105.263716912504));
#209681=CARTESIAN_POINT('Ctrl Pts',(-1.5762688014823,6.58322310852279,105.272033184908));
#209682=CARTESIAN_POINT('Ctrl Pts',(-1.74681042239048,6.53765572267522,
105.280349457312));
#209683=CARTESIAN_POINT('Ctrl Pts',(-1.91720785015746,6.492126864106,105.288658698298));
#209684=CARTESIAN_POINT('Ctrl Pts',(-2.08595895246826,6.43989594763906,
105.296967939284));
#209685=CARTESIAN_POINT('Ctrl Pts',(-2.25250951445243,6.38110412760216,
105.30527718027));
#209686=CARTESIAN_POINT('Ctrl Pts',(-2.41894979418782,6.32235123684922,
105.313580919252));
#209687=CARTESIAN_POINT('Ctrl Pts',(-2.58319211002671,6.25704621452549,
105.321884658235));
#209688=CARTESIAN_POINT('Ctrl Pts',(-2.74469687365095,6.18538018813482,
105.330188397217));
#209689=CARTESIAN_POINT('Ctrl Pts',(-2.9061242942684,6.11374848188333,105.338488159623));
#209690=CARTESIAN_POINT('Ctrl Pts',(-3.06481645794534,6.0357619831874,105.346787922028));
#209691=CARTESIAN_POINT('Ctrl Pts',(-3.22025304185457,5.95166021765578,
105.355087684434));
#209692=CARTESIAN_POINT('Ctrl Pts',(-3.37564366520775,5.86758331991146,
105.363384992708));
#209693=CARTESIAN_POINT('Ctrl Pts',(-3.52778032193459,5.77739492497551,
105.371682300983));
#209694=CARTESIAN_POINT('Ctrl Pts',(-3.6761664216275,5.68138094484945,105.379979609258));
#209695=CARTESIAN_POINT('Ctrl Pts',(-3.82456751358164,5.58535726390455,
105.388277755855));
#209696=CARTESIAN_POINT('Ctrl Pts',(-3.96921699511729,5.48350700435032,
105.396575902452));
#209697=CARTESIAN_POINT('Ctrl Pts',(-4.10964596501876,5.37616025079285,
105.404874049049));
#209698=CARTESIAN_POINT('Ctrl Pts',(-4.2500890559367,5.26880270284391,105.413173030077));
#209699=CARTESIAN_POINT('Ctrl Pts',(-4.386310512387,5.15594777022021,105.421472011105));
#209700=CARTESIAN_POINT('Ctrl Pts',(-4.51787341058359,5.03796673728021,
105.429770992133));
#209701=CARTESIAN_POINT('Ctrl Pts',(-4.64947140252216,4.91995423349254,
105.438072186873));
#209702=CARTESIAN_POINT('Ctrl Pts',(-4.77640810036555,4.79681313647768,
105.446373381613));
#209703=CARTESIAN_POINT('Ctrl Pts',(-4.89828230214976,4.66895271859187,
105.454674576352));
#209704=CARTESIAN_POINT('Ctrl Pts',(-5.02020926976148,4.54103694312705,
105.462979365121));
#209705=CARTESIAN_POINT('Ctrl Pts',(-5.13706913301943,4.40839802634082,
105.471284153889));
#209706=CARTESIAN_POINT('Ctrl Pts',(-5.24849982706175,4.27147966931049,
105.479588942658));
#209707=CARTESIAN_POINT('Ctrl Pts',(-5.36006262119077,4.13439899679795,
105.487903576679));
#209708=CARTESIAN_POINT('Ctrl Pts',(-5.46618316670318,3.99302901800606,
105.4962182107));
#209709=CARTESIAN_POINT('Ctrl Pts',(-5.56654103991165,3.84784483197794,
105.504532844721));
#209710=CARTESIAN_POINT('Ctrl Pts',(-5.66696237029346,3.70256884470132,
105.512852736158));
#209711=CARTESIAN_POINT('Ctrl Pts',(-5.76161357549936,3.55347413394155,
105.521172627596));
#209712=CARTESIAN_POINT('Ctrl Pts',(-5.85021929934244,3.40106206200376,
105.529492519034));
#209713=CARTESIAN_POINT('Ctrl Pts',(-5.93895751747274,3.24842208459938,
105.537824851407));
#209714=CARTESIAN_POINT('Ctrl Pts',(-6.0216320250837,3.09245513978424,105.54615718378));
#209715=CARTESIAN_POINT('Ctrl Pts',(-6.0980142825194,2.9336855336231,105.554489516154));
#209716=CARTESIAN_POINT('Ctrl Pts',(-6.1555213121882,2.81415033319126,105.560762801352));
#209717=CARTESIAN_POINT('Ctrl Pts',(-6.20946265235995,2.69302694323137,
105.567036086551));
#209718=CARTESIAN_POINT('Ctrl Pts',(-6.25975931743687,2.5705451343562,105.573309371749));
#209719=CARTESIAN_POINT('Ctrl Pts',(-6.33159816989002,2.39560406057879,
105.582269520679));
#209720=CARTESIAN_POINT('Ctrl Pts',(-6.3961918499594,2.21742488974813,105.591229669609));
#209721=CARTESIAN_POINT('Ctrl Pts',(-6.45325885736035,2.03659989195232,
105.600189818539));
#209722=CARTESIAN_POINT('Ctrl Pts',(-6.51007255865339,1.85657753088988,
105.609110195619));
#209723=CARTESIAN_POINT('Ctrl Pts',(-6.55942612505177,1.67393299626588,
105.618030572699));
#209724=CARTESIAN_POINT('Ctrl Pts',(-6.60108670157509,1.48927611888747,
105.626950949779));
#209725=CARTESIAN_POINT('Ctrl Pts',(-6.64263461531691,1.30511860947664,
105.635847203465));
#209726=CARTESIAN_POINT('Ctrl Pts',(-6.67653095978652,1.11895984650007,
105.644743457152));
#209727=CARTESIAN_POINT('Ctrl Pts',(-6.70259152190307,0.931426803626106,
105.653639710838));
#209728=CARTESIAN_POINT('Ctrl Pts',(-6.72854166544343,0.74468833807128,
105.662498271106));
#209729=CARTESIAN_POINT('Ctrl Pts',(-6.74672218185817,0.556587447153096,
105.671356831374));
#209730=CARTESIAN_POINT('Ctrl Pts',(-6.75699935893056,0.367761693780166,
105.680215391642));
#209731=CARTESIAN_POINT('Ctrl Pts',(-6.76355972001835,0.247226150208622,
105.685870189032));
#209732=CARTESIAN_POINT('Ctrl Pts',(-6.7669005915834,0.126395601807584,
105.691524986421));
#209733=CARTESIAN_POINT('Ctrl Pts',(-6.76699781404431,0.0054391837232258,
105.69717978381));
#209734=CARTESIAN_POINT('',(-6.76699999713954,0.000196757566297466,105.302810960999));
#209735=CARTESIAN_POINT('Ctrl Pts',(3.09910619832133,6.0156321173694,104.651395695404));
#209736=CARTESIAN_POINT('Ctrl Pts',(2.93375330812867,6.10081787289904,104.660145143281));
#209737=CARTESIAN_POINT('Ctrl Pts',(2.76488627941195,6.17918206991506,104.668894591158));
#209738=CARTESIAN_POINT('Ctrl Pts',(2.5930786679645,6.25045854491872,104.677644039035));
#209739=CARTESIAN_POINT('Ctrl Pts',(2.42127244384742,6.32173444437152,104.686393416261));
#209740=CARTESIAN_POINT('Ctrl Pts',(2.24652594922919,6.38592262652219,104.695142793487));
#209741=CARTESIAN_POINT('Ctrl Pts',(2.0694326998963,6.44280508013396,104.703892170713));
#209742=CARTESIAN_POINT('Ctrl Pts',(1.89234082174572,6.49968709332118,104.712641480195));
#209743=CARTESIAN_POINT('Ctrl Pts',(1.7129024980898,6.5492634035263,104.721390789677));
#209744=CARTESIAN_POINT('Ctrl Pts',(1.5317271707976,6.59136563044718,104.730140099159));
#209745=CARTESIAN_POINT('Ctrl Pts',(1.35055318611214,6.63346754536789,104.738889343804));
#209746=CARTESIAN_POINT('Ctrl Pts',(1.1676425026785,6.6680954229754,104.747638588448));
#209747=CARTESIAN_POINT('Ctrl Pts',(0.983616346643032,6.69513165536098,
104.756387833093));
#209748=CARTESIAN_POINT('Ctrl Pts',(0.79959149321553,6.72216769637369,104.765137015808));
#209749=CARTESIAN_POINT('Ctrl Pts',(0.614451466500017,6.74161215804563,
104.773886198522));
#209750=CARTESIAN_POINT('Ctrl Pts',(0.428825055349143,6.75339900138477,
104.782635381236));
#209751=CARTESIAN_POINT('Ctrl Pts',(0.243199896479616,6.76518576520697,
104.791384504927));
#209752=CARTESIAN_POINT('Ctrl Pts',(0.0570886457120184,6.76931499591632,
104.800133628617));
#209753=CARTESIAN_POINT('Ctrl Pts',(-0.128876618064112,6.76577266964508,
104.808882752307));
#209754=CARTESIAN_POINT('Ctrl Pts',(-0.314840689036212,6.76223036609477,
104.817631819879));
#209755=CARTESIAN_POINT('Ctrl Pts',(-0.500658488404962,6.7510166094889,
104.826380887452));
#209756=CARTESIAN_POINT('Ctrl Pts',(-0.68569894200026,6.73216948397318,
104.835129955024));
#209757=CARTESIAN_POINT('Ctrl Pts',(-0.87073827017588,6.71332247308605,
104.843878969384));
#209758=CARTESIAN_POINT('Ctrl Pts',(-1.05499997698502,6.6868422152278,104.852627983744));
#209759=CARTESIAN_POINT('Ctrl Pts',(-1.23785828066146,6.65281864152314,
104.861376998105));
#209760=CARTESIAN_POINT('Ctrl Pts',(-1.43007008855791,6.61705470583422,
104.870573538998));
#209761=CARTESIAN_POINT('Ctrl Pts',(-1.62073082018146,6.57295557924323,
104.879770079892));
#209762=CARTESIAN_POINT('Ctrl Pts',(-1.80912510111958,6.52068672522297,
104.888966620786));
#209763=CARTESIAN_POINT('Ctrl Pts',(-1.9883717912753,6.47095581494953,104.897716618439));
#209764=CARTESIAN_POINT('Ctrl Pts',(-2.16556660782784,6.41382980803431,
104.906466616092));
#209765=CARTESIAN_POINT('Ctrl Pts',(-2.34010763414595,6.34950275695758,
104.915216613745));
#209766=CARTESIAN_POINT('Ctrl Pts',(-2.51464512074081,6.28517701044495,
104.923966433947));
#209767=CARTESIAN_POINT('Ctrl Pts',(-2.68652865581904,6.21365061114273,
104.932716254148));
#209768=CARTESIAN_POINT('Ctrl Pts',(-2.85517438840589,6.13516651866851,
104.94146607435));
#209769=CARTESIAN_POINT('Ctrl Pts',(-3.02381692500434,6.05668391353847,
104.950215728734));
#209770=CARTESIAN_POINT('Ctrl Pts',(-3.18922152202248,5.97124400003274,
104.958965383119));
#209771=CARTESIAN_POINT('Ctrl Pts',(-3.35082635730161,5.87913698796114,
104.967715037504));
#209772=CARTESIAN_POINT('Ctrl Pts',(-3.51242834481176,5.7870315989814,104.976464537703));
#209773=CARTESIAN_POINT('Ctrl Pts',(-3.67023045556651,5.68825948846204,
104.985214037903));
#209774=CARTESIAN_POINT('Ctrl Pts',(-3.82369670929241,5.58315613925908,
104.993963538103));
#209775=CARTESIAN_POINT('Ctrl Pts',(-3.97716046260951,5.47805450249345,
105.002712895749));
#209776=CARTESIAN_POINT('Ctrl Pts',(-4.12628826381138,5.36662199540506,
105.011462253394));
#209777=CARTESIAN_POINT('Ctrl Pts',(-4.27057361170237,5.24923708999997,
105.020211611039));
#209778=CARTESIAN_POINT('Ctrl Pts',(-4.41485680048839,5.13185394115808,
105.028960837758));
#209779=CARTESIAN_POINT('Ctrl Pts',(-4.5542974586771,5.00851875309314,105.037710064476));
#209780=CARTESIAN_POINT('Ctrl Pts',(-4.68842200087424,4.87965041183468,
105.046459291195));
#209781=CARTESIAN_POINT('Ctrl Pts',(-4.8225447142129,4.75078382776366,105.055208398614));
#209782=CARTESIAN_POINT('Ctrl Pts',(-4.9513512499892,4.61638444000864,105.063957506032));
#209783=CARTESIAN_POINT('Ctrl Pts',(-5.07440415163224,4.47690869975003,
105.07270661345));
#209784=CARTESIAN_POINT('Ctrl Pts',(-5.1974555388563,4.3374346760272,105.081455613193));
#209785=CARTESIAN_POINT('Ctrl Pts',(-5.31475324408513,4.1928846396816,105.090204612936));
#209786=CARTESIAN_POINT('Ctrl Pts',(-5.42589890717437,4.04374950375564,
105.098953612678));
#209787=CARTESIAN_POINT('Ctrl Pts',(-5.53705670790261,3.89459808155823,
105.107703567854));
#209788=CARTESIAN_POINT('Ctrl Pts',(-5.64206095070966,3.74086078755725,
105.116453523029));
#209789=CARTESIAN_POINT('Ctrl Pts',(-5.74055494803381,3.58305984998919,
105.125203478205));
#209790=CARTESIAN_POINT('Ctrl Pts',(-5.83904514247732,3.42526500515924,
105.133953095542));
#209791=CARTESIAN_POINT('Ctrl Pts',(-5.93102544266345,3.26340707389305,
105.142702712879));
#209792=CARTESIAN_POINT('Ctrl Pts',(-6.01618342599591,3.0980358269026,105.151452330216));
#209793=CARTESIAN_POINT('Ctrl Pts',(-6.10133857407737,2.9326700857846,105.160201656243));
#209794=CARTESIAN_POINT('Ctrl Pts',(-6.17967172863313,2.76379151780895,
105.168950982271));
#209795=CARTESIAN_POINT('Ctrl Pts',(-6.25091683900291,2.59197370200198,
105.177700308298));
#209796=CARTESIAN_POINT('Ctrl Pts',(-6.32215995600044,2.42016069349849,
105.186449389527));
#209797=CARTESIAN_POINT('Ctrl Pts',(-6.38631531590723,2.24540886642485,
105.195198470756));
#209798=CARTESIAN_POINT('Ctrl Pts',(-6.44316503369334,2.0683117145613,105.203947551986));
#209799=CARTESIAN_POINT('Ctrl Pts',(-6.50001989046453,1.89119855382987,
105.212697424096));
#209800=CARTESIAN_POINT('Ctrl Pts',(-6.54956769590024,1.71173991694497,
105.221447296207));
#209801=CARTESIAN_POINT('Ctrl Pts',(-6.59164014488978,1.53054539307967,
105.230197168318));
#209802=CARTESIAN_POINT('Ctrl Pts',(-6.63370967316269,1.34936344794161,
105.238946433003));
#209803=CARTESIAN_POINT('Ctrl Pts',(-6.66830481861374,1.16644613613568,
105.247695697688));
#209804=CARTESIAN_POINT('Ctrl Pts',(-6.69530808396591,0.982414709163446,
105.256444962373));
#209805=CARTESIAN_POINT('Ctrl Pts',(-6.72231273474192,0.798373840313651,
105.265194675946));
#209806=CARTESIAN_POINT('Ctrl Pts',(-6.74172468433312,0.61321902549096,
105.273944389519));
#209807=CARTESIAN_POINT('Ctrl Pts',(-6.75347799617534,0.427579180007128,
105.282694103092));
#209808=CARTESIAN_POINT('Ctrl Pts',(-6.76248551786179,0.285308222126213,
105.289399722394));
#209809=CARTESIAN_POINT('Ctrl Pts',(-6.76699585218083,0.142752574305234,
105.296105341697));
#209810=CARTESIAN_POINT('Ctrl Pts',(-6.76699999713954,0.000196757566300471,
105.302810960999));
#209811=CARTESIAN_POINT('Ctrl Pts',(-6.76699999690187,0.00020476833760498,
105.302983892799));
#209812=CARTESIAN_POINT('Ctrl Pts',(-6.76700511243132,-0.168848651656523,
105.310950501476));
#209813=CARTESIAN_POINT('Ctrl Pts',(-6.76067096858633,-0.338125069321827,
105.318917110153));
#209814=CARTESIAN_POINT('Ctrl Pts',(-6.74797342414344,-0.507093351419459,
105.32688371883));
#209815=CARTESIAN_POINT('Ctrl Pts',(-6.73528508990087,-0.675939071888637,
105.334844548905));
#209816=CARTESIAN_POINT('Ctrl Pts',(-6.7162425649944,-0.844476722711796,
105.34280537898));
#209817=CARTESIAN_POINT('Ctrl Pts',(-6.69087376521969,-1.01217451948514,
105.350766209054));
#209818=CARTESIAN_POINT('Ctrl Pts',(-6.6655172193102,-1.17979131336441,
105.358723193817));
#209819=CARTESIAN_POINT('Ctrl Pts',(-6.63384053379525,-1.34656868357456,
105.36668017858));
#209820=CARTESIAN_POINT('Ctrl Pts',(-6.5959235073992,-1.51197952517176,
105.374637163343));
#209821=CARTESIAN_POINT('Ctrl Pts',(-6.55801769950983,-1.67734142668037,
105.382591793874));
#209822=CARTESIAN_POINT('Ctrl Pts',(-6.51387531155373,-1.84133723257834,
105.390546424405));
#209823=CARTESIAN_POINT('Ctrl Pts',(-6.46362727444644,-2.0034498888248,
105.398501054936));
#209824=CARTESIAN_POINT('Ctrl Pts',(-6.41337338753906,-2.16558141798025,
105.406456611532));
#209825=CARTESIAN_POINT('Ctrl Pts',(-6.35701253929677,-2.32582899297134,
105.414412168129));
#209826=CARTESIAN_POINT('Ctrl Pts',(-6.29472559629214,-2.48369053373898,
105.422367724726));
#209827=CARTESIAN_POINT('Ctrl Pts',(-6.25125037920287,-2.59387517957091,
105.427920566677));
#209828=CARTESIAN_POINT('Ctrl Pts',(-6.20488913351062,-2.70289770984355,
105.433473408628));
#209829=CARTESIAN_POINT('Ctrl Pts',(-6.15571725662235,-2.81059318588119,
105.439026250579));
#209830=CARTESIAN_POINT('Ctrl Pts',(-6.07615768892623,-2.98484330726363,
105.448010689104));
#209831=CARTESIAN_POINT('Ctrl Pts',(-5.98926326254738,-3.15556498263556,
105.45699512763));
#209832=CARTESIAN_POINT('Ctrl Pts',(-5.89537231653845,-3.32217914167675,
105.465979566156));
#209833=CARTESIAN_POINT('Ctrl Pts',(-5.80131932036034,-3.48908086681252,
105.474979511286));
#209834=CARTESIAN_POINT('Ctrl Pts',(-5.70024578606546,-3.65186069775247,
105.483979456417));
#209835=CARTESIAN_POINT('Ctrl Pts',(-5.59253402486987,-3.80996747763979,
105.492979401547));
#209836=CARTESIAN_POINT('Ctrl Pts',(-5.48456843814425,-3.96844684021222,
105.502000555279));
#209837=CARTESIAN_POINT('Ctrl Pts',(-5.36993346019752,-4.12223091989116,
105.511021709011));
#209838=CARTESIAN_POINT('Ctrl Pts',(-5.24905414884304,-4.2707984666235,
105.520042862744));
#209839=CARTESIAN_POINT('Ctrl Pts',(-5.12805184183638,-4.41951718200579,
105.529073195571));
#209840=CARTESIAN_POINT('Ctrl Pts',(-5.00079266370581,-4.56300857922963,
105.538103528398));
#209841=CARTESIAN_POINT('Ctrl Pts',(-4.86774051267167,-4.7007862428848,
105.547133861225));
#209842=CARTESIAN_POINT('Ctrl Pts',(-4.73449973562801,-4.8387592318368,
105.556176996218));
#209843=CARTESIAN_POINT('Ctrl Pts',(-4.5954497304539,-4.971002118546,105.56522013121));
#209844=CARTESIAN_POINT('Ctrl Pts',(-4.45109131661908,-5.09706534106815,
105.574263266203));
#209845=CARTESIAN_POINT('Ctrl Pts',(-4.32488880469304,-5.20727364082124,
105.582169049603));
#209846=CARTESIAN_POINT('Ctrl Pts',(-4.19462979517459,-5.31275948396984,
105.590074833003));
#209847=CARTESIAN_POINT('Ctrl Pts',(-4.06066906516676,-5.41324816937093,
105.597980616403));
#209848=CARTESIAN_POINT('Ctrl Pts',(-3.91404043325983,-5.52323949639361,
105.606634004631));
#209849=CARTESIAN_POINT('Ctrl Pts',(-3.76284656150001,-5.6273400054027,
105.61528739286));
#209850=CARTESIAN_POINT('Ctrl Pts',(-3.60757784903758,-5.72517869268143,
105.623940781088));
#209851=CARTESIAN_POINT('Ctrl Pts',(-3.45245253824524,-5.82292701899217,
105.632586177298));
#209852=CARTESIAN_POINT('Ctrl Pts',(-3.2932601492652,-5.91442489684805,
105.641231573509));
#209853=CARTESIAN_POINT('Ctrl Pts',(-3.13052099310498,-5.99934390677256,
105.649876969719));
#209854=CARTESIAN_POINT('Ctrl Pts',(-2.96258449650236,-6.08697494381471,
105.658798470762));
#209855=CARTESIAN_POINT('Ctrl Pts',(-2.79087119428749,-6.16759974134333,
105.667719971804));
#209856=CARTESIAN_POINT('Ctrl Pts',(-2.6159836391453,-6.2409068731815,105.676641472846));
#209857=CARTESIAN_POINT('Ctrl Pts',(-2.44683132678979,-6.31180997919437,
105.685270403188));
#209858=CARTESIAN_POINT('Ctrl Pts',(-2.27470995381919,-6.37586761055618,
105.69389933353));
#209859=CARTESIAN_POINT('Ctrl Pts',(-2.1001885551175,-6.43284517402319,
105.702528263872));
#209860=CARTESIAN_POINT('Ctrl Pts',(-1.91679122756421,-6.49272054144567,
105.711596050265));
#209861=CARTESIAN_POINT('Ctrl Pts',(-1.73074368961585,-6.54477675029657,
105.720663836658));
#209862=CARTESIAN_POINT('Ctrl Pts',(-1.54272919699996,-6.58879925515445,
105.72973162305));
#209863=CARTESIAN_POINT('Ctrl Pts',(-1.35471470438408,-6.63282176001234,
105.738799409443));
#209864=CARTESIAN_POINT('Ctrl Pts',(-1.16473362930391,-6.66881043757078,
105.747867195835));
#209865=CARTESIAN_POINT('Ctrl Pts',(-0.97348730648406,-6.69661193919092,
105.756934982228));
#209866=CARTESIAN_POINT('Ctrl Pts',(-0.795798749362242,-6.72244254673341,
105.765359938361));
#209867=CARTESIAN_POINT('Ctrl Pts',(-0.617095979185703,-6.74119454122236,
105.773784894494));
#209868=CARTESIAN_POINT('Ctrl Pts',(-0.437966647770672,-6.75281231898537,
105.782209850627));
#209869=CARTESIAN_POINT('Ctrl Pts',(-0.258795738717023,-6.7644327933462,
105.790636762274));
#209870=CARTESIAN_POINT('Ctrl Pts',(-0.0791984019269233,-6.76891572785916,
105.79906367392));
#209871=CARTESIAN_POINT('Ctrl Pts',(0.100235296339718,-6.76625759821245,
105.807490585567));
#209872=CARTESIAN_POINT('Ctrl Pts',(0.279734979366334,-6.76359849106793,
105.815920596117));
#209873=CARTESIAN_POINT('Ctrl Pts',(0.459070572473804,-6.75379308858288,
105.824350606667));
#209874=CARTESIAN_POINT('Ctrl Pts',(0.637654326518938,-6.73688993229604,
105.832780617217));
#209875=CARTESIAN_POINT('Ctrl Pts',(0.816402588182952,-6.71997120517517,
105.841218393316));
#209876=CARTESIAN_POINT('Ctrl Pts',(0.994397296711167,-6.69594169257105,
105.849656169416));
#209877=CARTESIAN_POINT('Ctrl Pts',(1.1710570036539,-6.66490168676127,105.858093945515));
#209878=CARTESIAN_POINT('Ctrl Pts',(1.34780944392092,-6.63384538723643,
105.866536150825));
#209879=CARTESIAN_POINT('Ctrl Pts',(1.52322516012246,-6.59577132020763,
105.874978356135));
#209880=CARTESIAN_POINT('Ctrl Pts',(1.69673459188276,-6.55083053701654,
105.883420561445));
#209881=CARTESIAN_POINT('Ctrl Pts',(1.87042706654646,-6.50584234377199,
105.891871672817));
#209882=CARTESIAN_POINT('Ctrl Pts',(2.04220892088487,-6.45397305443475,
105.900322784189));
#209883=CARTESIAN_POINT('Ctrl Pts',(2.21152637024734,-6.39542337251418,
105.908773895561));
#209884=CARTESIAN_POINT('Ctrl Pts',(2.25904557468133,-6.37899131359052,
105.911145713058));
#209885=CARTESIAN_POINT('Ctrl Pts',(2.30637079135772,-6.3620333625382,105.913517530556));
#209886=CARTESIAN_POINT('Ctrl Pts',(2.35349007810657,-6.34455462993692,
105.915889348053));
#209887=CARTESIAN_POINT('Ctrl Pts',(2.51870381168923,-6.2832691803769,105.924205620457));
#209888=CARTESIAN_POINT('Ctrl Pts',(2.68168238585124,-6.2154669504817,105.932521892861));
#209889=CARTESIAN_POINT('Ctrl Pts',(2.84188552188961,-6.14133337968834,
105.940838165265));
#209890=CARTESIAN_POINT('Ctrl Pts',(3.00195320598697,-6.06726248891677,
105.949147406251));
#209891=CARTESIAN_POINT('Ctrl Pts',(3.15924981314508,-5.98687106809083,
105.957456647237));
#209892=CARTESIAN_POINT('Ctrl Pts',(3.3132535380234,-5.90039320662407,105.965765888223));
#209893=CARTESIAN_POINT('Ctrl Pts',(3.46715528860129,-5.81397260688544,
105.974069627206));
#209894=CARTESIAN_POINT('Ctrl Pts',(3.61776819921841,-5.72147376684853,
105.982373366188));
#209895=CARTESIAN_POINT('Ctrl Pts',(3.76459344286126,-5.62317750119681,
105.990677105171));
#209896=CARTESIAN_POINT('Ctrl Pts',(3.91134837337348,-5.52492830863686,
105.998976867576));
#209897=CARTESIAN_POINT('Ctrl Pts',(4.05431896323696,-5.42088741655098,
106.007276629982));
#209898=CARTESIAN_POINT('Ctrl Pts',(4.19303366394567,-5.31138001775606,
106.015576392387));
#209899=CARTESIAN_POINT('Ctrl Pts',(4.33170734853682,-5.20190499886262,
106.023873700662));
#209900=CARTESIAN_POINT('Ctrl Pts',(4.46612737956734,-5.08696691049196,
106.032171008936));
#209901=CARTESIAN_POINT('Ctrl Pts',(4.59585354289005,-4.96693257577602,
106.040468317211));
#209902=CARTESIAN_POINT('Ctrl Pts',(4.72559281315962,-4.8468861133319,106.048766463808));
#209903=CARTESIAN_POINT('Ctrl Pts',(4.85063700760493,-4.72174260644738,
106.057064610405));
#209904=CARTESIAN_POINT('Ctrl Pts',(4.97058076503971,-4.59190764913857,
106.065362757002));
#209905=CARTESIAN_POINT('Ctrl Pts',(5.09053658357387,-4.46205963610801,
106.073661738031));
#209906=CARTESIAN_POINT('Ctrl Pts',(5.20539070617779,-4.32751948769192,
106.081960719059));
#209907=CARTESIAN_POINT('Ctrl Pts',(5.31477633963618,-4.1887279047037,106.090259700087));
#209908=CARTESIAN_POINT('Ctrl Pts',(5.42419115116262,-4.04989929975816,
106.098560894826));
#209909=CARTESIAN_POINT('Ctrl Pts',(5.52813435078339,-3.90681727333276,
106.106862089566));
#209910=CARTESIAN_POINT('Ctrl Pts',(5.62628085151066,-3.75995382683412,
106.115163284305));
#209911=CARTESIAN_POINT('Ctrl Pts',(5.72446984508069,-3.61302679533455,
106.123468073074));
#209912=CARTESIAN_POINT('Ctrl Pts',(5.81685694465353,-3.46231537002372,
106.131772861842));
#209913=CARTESIAN_POINT('Ctrl Pts',(5.90316152390068,-3.30831876075123,
106.140077650611));
#209914=CARTESIAN_POINT('Ctrl Pts',(5.9895684164515,-3.15413958988138,106.148392284632));
#209915=CARTESIAN_POINT('Ctrl Pts',(6.06987821134061,-2.99666775770691,
106.156706918653));
#209916=CARTESIAN_POINT('Ctrl Pts',(6.143856690237,-2.83642626730011,106.165021552674));
#209917=CARTESIAN_POINT('Ctrl Pts',(6.21788194638141,-2.6760834547784,106.173341444112));
#209918=CARTESIAN_POINT('Ctrl Pts',(6.28556776967601,-2.51296781252368,
106.181661335549));
#209919=CARTESIAN_POINT('Ctrl Pts',(6.34672884497938,-2.34762049068981,
106.189981226987));
#209920=CARTESIAN_POINT('Ctrl Pts',(6.40798137592181,-2.18202592099595,
106.19831355936));
#209921=CARTESIAN_POINT('Ctrl Pts',(6.46268955258892,-2.01419333330978,
106.206645891734));
#209922=CARTESIAN_POINT('Ctrl Pts',(6.51071811699813,-1.84467845463441,
106.214978224107));
#209923=CARTESIAN_POINT('Ctrl Pts',(6.54687808622572,-1.71705330339534,
106.221251509305));
#209924=CARTESIAN_POINT('Ctrl Pts',(6.57925285944496,-1.58847485328167,
106.227524794504));
#209925=CARTESIAN_POINT('Ctrl Pts',(6.6078040171022,-1.45918301510402,106.233798079702));
#209926=CARTESIAN_POINT('Ctrl Pts',(6.64453173443157,-1.2928642219191,106.241867925705));
#209927=CARTESIAN_POINT('Ctrl Pts',(6.67504371885449,-1.12485071678804,
106.249937771707));
#209928=CARTESIAN_POINT('Ctrl Pts',(6.69917958941325,-0.955657798999658,
106.25800761771));
#209929=CARTESIAN_POINT('Ctrl Pts',(6.72328509397694,-0.786677747422023,
106.26606731082));
#209930=CARTESIAN_POINT('Ctrl Pts',(6.74103039415247,-0.616521600289532,
106.27412700393));
#209931=CARTESIAN_POINT('Ctrl Pts',(6.7523050586329,-0.445718964326782,
106.28218669704));
#209932=CARTESIAN_POINT('Ctrl Pts',(6.76356801258344,-0.275093734031229,
106.290238018879));
#209933=CARTESIAN_POINT('Ctrl Pts',(6.76837368089856,-0.103823720276054,
106.298289340717));
#209934=CARTESIAN_POINT('Ctrl Pts',(6.76666281810618,0.0675522468859296,
106.306340662556));
#209935=CARTESIAN_POINT('Ctrl Pts',(6.76495335740821,0.23878776720118,106.314385386137));
#209936=CARTESIAN_POINT('Ctrl Pts',(6.75673799853821,0.410128696927685,
106.322430109718));
#209937=CARTESIAN_POINT('Ctrl Pts',(6.7420093902107,0.581032169772714,106.330474833299));
#209938=CARTESIAN_POINT('Ctrl Pts',(6.7272896282436,0.751832993834989,106.338514725024));
#209939=CARTESIAN_POINT('Ctrl Pts',(6.70606443638829,0.922196513281735,
106.346554616748));
#209940=CARTESIAN_POINT('Ctrl Pts',(6.6783785299524,1.09158106005499,106.354594508472));
#209941=CARTESIAN_POINT('Ctrl Pts',(6.65009647010046,1.26461292017956,106.362807521092));
#209942=CARTESIAN_POINT('Ctrl Pts',(6.61507230951299,1.4366227708902,106.371020533712));
#209943=CARTESIAN_POINT('Ctrl Pts',(6.57340954600896,1.60703949560624,106.379233546332));
#209944=CARTESIAN_POINT('Ctrl Pts',(6.53263921587813,1.77380582462841,106.387270632875));
#209945=CARTESIAN_POINT('Ctrl Pts',(6.48551191000055,1.93904621260604,106.395307719417));
#209946=CARTESIAN_POINT('Ctrl Pts',(6.43217603789486,2.10223700317809,106.40334480596));
#209947=CARTESIAN_POINT('Ctrl Pts',(6.37883506129792,2.26544341186847,106.411382661689));
#209948=CARTESIAN_POINT('Ctrl Pts',(6.31928445129713,2.42659947738446,106.419420517418));
#209949=CARTESIAN_POINT('Ctrl Pts',(6.25372201686337,2.5851982391682,106.427458373147));
#209950=CARTESIAN_POINT('Ctrl Pts',(6.18814031769203,2.74384360330209,106.435498590704));
#209951=CARTESIAN_POINT('Ctrl Pts',(6.11654342058265,2.89992982291108,106.443538808261));
#209952=CARTESIAN_POINT('Ctrl Pts',(6.03917658274562,3.05297153645706,106.451579025818));
#209953=CARTESIAN_POINT('Ctrl Pts',(5.95888677620512,3.21179526399669,106.459923007946));
#209954=CARTESIAN_POINT('Ctrl Pts',(5.87238272970772,3.36733954811179,106.468266990074));
#209955=CARTESIAN_POINT('Ctrl Pts',(5.7799892658019,3.51909265112683,106.476610972201));
#209956=CARTESIAN_POINT('Ctrl Pts',(5.69080441422155,3.66557571818717,106.484665187037));
#209957=CARTESIAN_POINT('Ctrl Pts',(5.59613259808764,3.80852623774655,106.492719401872));
#209958=CARTESIAN_POINT('Ctrl Pts',(5.49630819495313,3.94751633639318,106.500773616707));
#209959=CARTESIAN_POINT('Ctrl Pts',(5.39640908975963,4.08661044614554,106.50883385879));
#209960=CARTESIAN_POINT('Ctrl Pts',(5.29134994779295,4.22173794091867,106.516894100873));
#209961=CARTESIAN_POINT('Ctrl Pts',(5.18150364243719,4.35250606012331,106.524954342956));
#209962=CARTESIAN_POINT('Ctrl Pts',(5.07150376441194,4.48345700212827,106.53302585381));
#209963=CARTESIAN_POINT('Ctrl Pts',(4.95670361835191,4.61003613445532,106.541097364664));
#209964=CARTESIAN_POINT('Ctrl Pts',(4.83751131274927,4.73188897788429,106.549168875519));
#209965=CARTESIAN_POINT('Ctrl Pts',(4.82501871465519,4.7446604281208,106.55001485413));
#209966=CARTESIAN_POINT('Ctrl Pts',(4.8124778957345,4.75737999694354,106.55086083274));
#209967=CARTESIAN_POINT('Ctrl Pts',(4.79988934516451,4.77004730313822,106.551706811351));
#209968=CARTESIAN_POINT('Ctrl Pts',(4.67613620380326,4.89457466039519,106.560023297831));
#209969=CARTESIAN_POINT('Ctrl Pts',(4.54735003171967,5.01446784966951,106.568339784311));
#209970=CARTESIAN_POINT('Ctrl Pts',(4.41391181903876,5.12929541494248,106.57665627079));
#209971=CARTESIAN_POINT('Ctrl Pts',(4.2820334896682,5.24278065406286,106.584875538129));
#209972=CARTESIAN_POINT('Ctrl Pts',(4.14561154969721,5.35131778996561,106.593094805467));
#209973=CARTESIAN_POINT('Ctrl Pts',(4.00505336407265,5.45452441106742,106.601314072806));
#209974=CARTESIAN_POINT('Ctrl Pts',(3.86200135286363,5.55956215506716,106.609679168856));
#209975=CARTESIAN_POINT('Ctrl Pts',(3.71466517784795,5.65907816395306,106.618044264906));
#209976=CARTESIAN_POINT('Ctrl Pts',(3.56351232619173,5.75270970074795,106.626409360957));
#209977=CARTESIAN_POINT('Ctrl Pts',(3.41235947453541,5.84634123754292,106.634774457007));
#209978=CARTESIAN_POINT('Ctrl Pts',(3.25739025212274,5.93408805306152,106.643139553057));
#209979=CARTESIAN_POINT('Ctrl Pts',(3.09910619832136,6.01563211736939,106.651504649108));
#209980=CARTESIAN_POINT('Origin',(0.,0.,4.30282021618968));
#209981=CARTESIAN_POINT('',(3.09910619832136,6.01563211736939,109.045804610872));
#209982=CARTESIAN_POINT('',(3.09910619832125,6.01563211736945,108.651395695404));
#209983=CARTESIAN_POINT('',(3.09910619832133,6.0156321173694,4.30282021618968));
#209984=CARTESIAN_POINT('',(-6.76699852330449,-0.00312165100701077,107.69717978381));
#209985=CARTESIAN_POINT('Ctrl Pts',(-6.76699697141835,-0.00640225076298612,
107.69717978381));
#209986=CARTESIAN_POINT('Ctrl Pts',(-6.7667890499928,-0.226169284123469,
107.707514248948));
#209987=CARTESIAN_POINT('Ctrl Pts',(-6.75587179968307,-0.44545334613587,
107.717848714086));
#209988=CARTESIAN_POINT('Ctrl Pts',(-6.7344074901004,-0.663358694282056,
107.728183179225));
#209989=CARTESIAN_POINT('Ctrl Pts',(-6.71267045783008,-0.884032719052677,
107.738648952714));
#209990=CARTESIAN_POINT('Ctrl Pts',(-6.68011670896827,-1.10329295106132,
107.749114726204));
#209991=CARTESIAN_POINT('Ctrl Pts',(-6.6369625513362,-1.3202337263382,107.759580499694));
#209992=CARTESIAN_POINT('Ctrl Pts',(-6.59330374048131,-1.53971144978907,
107.770168662001));
#209993=CARTESIAN_POINT('Ctrl Pts',(-6.53879512245999,-1.75681535057055,
107.780756824308));
#209994=CARTESIAN_POINT('Ctrl Pts',(-6.47370892271277,-1.9706297937434,
107.791344986615));
#209995=CARTESIAN_POINT('Ctrl Pts',(-6.45869878286014,-2.01993955075795,
107.793786822175));
#209996=CARTESIAN_POINT('Ctrl Pts',(-6.44312627285897,-2.06907444182178,
107.796228657736));
#209997=CARTESIAN_POINT('Ctrl Pts',(-6.42699509465897,-2.11802338354174,
107.798670493296));
#209998=CARTESIAN_POINT('Ctrl Pts',(-6.37368432875604,-2.27979120613193,
107.806740339298));
#209999=CARTESIAN_POINT('Ctrl Pts',(-6.31416349739519,-2.43984366545063,
107.814810185301));
#210000=CARTESIAN_POINT('Ctrl Pts',(-6.24855770860955,-2.5976557820805,
107.822880031304));
#210001=CARTESIAN_POINT('Ctrl Pts',(-6.18303446025095,-2.75526935099468,
107.830939724414));
#210002=CARTESIAN_POINT('Ctrl Pts',(-6.11144162849685,-2.91064784540945,
107.838999417524));
#210003=CARTESIAN_POINT('Ctrl Pts',(-6.03395457703162,-3.0632794783237,
107.847059110634));
#210004=CARTESIAN_POINT('Ctrl Pts',(-5.95654800817668,-3.21575257904456,
107.855110432473));
#210005=CARTESIAN_POINT('Ctrl Pts',(-5.87325957007225,-3.36548416601938,
107.863161754311));
#210006=CARTESIAN_POINT('Ctrl Pts',(-5.7843133500058,-3.51198064757547,
107.87121307615));
#210007=CARTESIAN_POINT('Ctrl Pts',(-5.69544002356877,-3.65835707163808,
107.879257799731));
#210008=CARTESIAN_POINT('Ctrl Pts',(-5.60091833632212,-3.80150334983204,
107.887302523312));
#210009=CARTESIAN_POINT('Ctrl Pts',(-5.50101906065008,-3.9409489078602,
107.895347246893));
#210010=CARTESIAN_POINT('Ctrl Pts',(-5.40117978691283,-4.08031071149452,
107.903387138617));
#210011=CARTESIAN_POINT('Ctrl Pts',(-5.29596957123947,-4.21597591722323,
107.911427030342));
#210012=CARTESIAN_POINT('Ctrl Pts',(-5.18570334754686,-4.34750155735928,
107.919466922066));
#210013=CARTESIAN_POINT('Ctrl Pts',(-5.07306278996375,-4.48185930486589,
107.927679934686));
#210014=CARTESIAN_POINT('Ctrl Pts',(-4.95514622170093,-4.61189685134965,
107.935892947306));
#210015=CARTESIAN_POINT('Ctrl Pts',(-4.83233415631449,-4.73717590994005,
107.944105959926));
#210016=CARTESIAN_POINT('Ctrl Pts',(-4.71215277541851,-4.85977144004019,
107.952143046469));
#210017=CARTESIAN_POINT('Ctrl Pts',(-4.58728378140174,-4.97781000624466,
107.960180133011));
#210018=CARTESIAN_POINT('Ctrl Pts',(-4.45812208332028,-5.09091705787985,
107.968217219554));
#210019=CARTESIAN_POINT('Ctrl Pts',(-4.32894802386315,-5.20403493438633,
107.976255075283));
#210020=CARTESIAN_POINT('Ctrl Pts',(-4.19548072331569,-5.31222011030555,
107.984292931012));
#210021=CARTESIAN_POINT('Ctrl Pts',(-4.05814904835102,-5.41513760687277,
107.992330786741));
#210022=CARTESIAN_POINT('Ctrl Pts',(-3.92077702011585,-5.51808534451568,
108.000371004298));
#210023=CARTESIAN_POINT('Ctrl Pts',(-3.77953865610771,-5.61576209794088,
108.008411221855));
#210024=CARTESIAN_POINT('Ctrl Pts',(-3.63489259999168,-5.70787568071746,
108.016451439412));
#210025=CARTESIAN_POINT('Ctrl Pts',(-3.48478172319846,-5.80346937367002,
108.02479542154));
#210026=CARTESIAN_POINT('Ctrl Pts',(-3.33100101066344,-5.89307108589456,
108.033139403668));
#210027=CARTESIAN_POINT('Ctrl Pts',(-3.17409098904519,-5.97640656191177,
108.041483385795));
#210028=CARTESIAN_POINT('Ctrl Pts',(-3.02263009129439,-6.0568479886727,
108.04953760063));
#210029=CARTESIAN_POINT('Ctrl Pts',(-2.86825394831563,-6.13145100665045,
108.057591815465));
#210030=CARTESIAN_POINT('Ctrl Pts',(-2.71146849668429,-6.20001835412514,
108.0656460303));
#210031=CARTESIAN_POINT('Ctrl Pts',(-2.55456571706835,-6.26863701292117,
108.073706272383));
#210032=CARTESIAN_POINT('Ctrl Pts',(-2.39525038420781,-6.33121087223865,
108.081766514466));
#210033=CARTESIAN_POINT('Ctrl Pts',(-2.23404361549099,-6.38759251393543,
108.089826756549));
#210034=CARTESIAN_POINT('Ctrl Pts',(-2.07261146865362,-6.44405298103477,
108.097898267404));
#210035=CARTESIAN_POINT('Ctrl Pts',(-1.90928296371488,-6.49430384919237,
108.105969778258));
#210036=CARTESIAN_POINT('Ctrl Pts',(-1.74458997759913,-6.53824860417992,
108.114041289112));
#210037=CARTESIAN_POINT('Ctrl Pts',(-1.72732843312179,-6.54285447332258,
108.114887267723));
#210038=CARTESIAN_POINT('Ctrl Pts',(-1.71005190425678,-6.54739111532215,
108.115733246334));
#210039=CARTESIAN_POINT('Ctrl Pts',(-1.69276100624007,-6.55185845205413,
108.116579224945));
#210040=CARTESIAN_POINT('Ctrl Pts',(-1.52456394296557,-6.59531443208769,
108.124808474681));
#210041=CARTESIAN_POINT('Ctrl Pts',(-1.35444527003813,-6.63235326078244,
108.133037724417));
#210042=CARTESIAN_POINT('Ctrl Pts',(-1.1829356770626,-6.66280362789813,
108.141266974153));
#210043=CARTESIAN_POINT('Ctrl Pts',(-1.01163020840378,-6.6932177541233,
108.149486429743));
#210044=CARTESIAN_POINT('Ctrl Pts',(-0.838937465623442,-6.71705897043115,
108.157705885333));
#210045=CARTESIAN_POINT('Ctrl Pts',(-0.665402832443382,-6.73420582330065,
108.165925340923));
#210046=CARTESIAN_POINT('Ctrl Pts',(-0.492039883683817,-6.75133571213568,
108.174136664693));
#210047=CARTESIAN_POINT('Ctrl Pts',(-0.317837057694991,-6.76178439201576,
108.182347988462));
#210048=CARTESIAN_POINT('Ctrl Pts',(-0.14334954881376,-6.76548149852284,
108.190559312232));
#210049=CARTESIAN_POINT('Ctrl Pts',(0.0310003616484347,-6.76917568954324,
108.198764160666));
#210050=CARTESIAN_POINT('Ctrl Pts',(0.205634150909775,-6.76612890415982,
108.2069690091));
#210051=CARTESIAN_POINT('Ctrl Pts',(0.37999179587546,-6.75632261182571,
108.215173857534));
#210052=CARTESIAN_POINT('Ctrl Pts',(0.554246938450867,-6.74652208447199,
108.223373882454));
#210053=CARTESIAN_POINT('Ctrl Pts',(0.72822590300902,-6.7299699864952,108.231573907374));
#210054=CARTESIAN_POINT('Ctrl Pts',(0.901368869000644,-6.70669987117334,
108.239773932294));
#210055=CARTESIAN_POINT('Ctrl Pts',(1.07446172349546,-6.68343649075003,
108.247971583941));
#210056=CARTESIAN_POINT('Ctrl Pts',(1.2467187058382,-6.65345900965552,108.256169235588));
#210057=CARTESIAN_POINT('Ctrl Pts',(1.41758506704369,-6.61685284540126,
108.264366887235));
#210058=CARTESIAN_POINT('Ctrl Pts',(1.58842854819504,-6.580251582937,108.272563441166));
#210059=CARTESIAN_POINT('Ctrl Pts',(1.75788142822436,-6.53702347942953,
108.280759995097));
#210060=CARTESIAN_POINT('Ctrl Pts',(1.92539909317718,-6.48730509009654,
108.288956549028));
#210061=CARTESIAN_POINT('Ctrl Pts',(2.09292478555124,-6.43758431826583,
108.297153495736));
#210062=CARTESIAN_POINT('Ctrl Pts',(2.25851473413512,-6.3813727430211,108.305350442445));
#210063=CARTESIAN_POINT('Ctrl Pts',(2.42163938254588,-6.31885683497441,
108.313547389154));
#210064=CARTESIAN_POINT('Ctrl Pts',(2.58480150809921,-6.25632656418351,
108.321746219074));
#210065=CARTESIAN_POINT('Ctrl Pts',(2.74549687047634,-6.18748920418675,
108.329945048993));
#210066=CARTESIAN_POINT('Ctrl Pts',(2.90321574677204,-6.11257943324215,
108.338143878913));
#210067=CARTESIAN_POINT('Ctrl Pts',(3.06108400300623,-6.03759871316806,
108.346350474173));
#210068=CARTESIAN_POINT('Ctrl Pts',(3.21596981635108,-5.95653424559037,
108.354557069433));
#210069=CARTESIAN_POINT('Ctrl Pts',(3.36738710586005,-5.86966720345264,
108.362763664692));
#210070=CARTESIAN_POINT('Ctrl Pts',(3.51887768220526,-5.78275811716848,
108.370974231991));
#210071=CARTESIAN_POINT('Ctrl Pts',(3.66689608377019,-5.69004104721331,
108.37918479929));
#210072=CARTESIAN_POINT('Ctrl Pts',(3.8109851959247,-5.59184055892537,108.387395366589));
#210073=CARTESIAN_POINT('Ctrl Pts',(3.95527302759268,-5.49350463810569,
108.395617257436));
#210074=CARTESIAN_POINT('Ctrl Pts',(4.09562045136291,-5.38967039883068,
108.403839148283));
#210075=CARTESIAN_POINT('Ctrl Pts',(4.23160246303918,-5.28070351324525,
108.412061039129));
#210076=CARTESIAN_POINT('Ctrl Pts',(4.35524220355758,-5.18162689794298,
108.419536678284));
#210077=CARTESIAN_POINT('Ctrl Pts',(4.47527329368927,-5.07830769704904,
108.427012317439));
#210078=CARTESIAN_POINT('Ctrl Pts',(4.5914033168387,-4.97104662843979,108.434487956594));
#210079=CARTESIAN_POINT('Ctrl Pts',(4.73021837977693,-4.84283299697727,
108.443423900045));
#210080=CARTESIAN_POINT('Ctrl Pts',(4.86374843634968,-4.70871996212397,
108.452359843496));
#210081=CARTESIAN_POINT('Ctrl Pts',(4.99151051770733,-4.56914781459488,
108.461295786946));
#210082=CARTESIAN_POINT('Ctrl Pts',(5.11908053876973,-4.42978548102292,
108.470218297304));
#210083=CARTESIAN_POINT('Ctrl Pts',(5.24089971189132,-4.28498059957015,
108.479140807662));
#210084=CARTESIAN_POINT('Ctrl Pts',(5.35652160943637,-4.13521042362311,
108.488063318019));
#210085=CARTESIAN_POINT('Ctrl Pts',(5.47186019745173,-3.985807231085,108.496963965458));
#210086=CARTESIAN_POINT('Ctrl Pts',(5.58103165945079,-3.83146323026634,
108.505864612896));
#210087=CARTESIAN_POINT('Ctrl Pts',(5.68362993773233,-3.67268835199949,
108.514765260334));
#210088=CARTESIAN_POINT('Ctrl Pts',(5.78606966303756,-3.51415884071088,
108.523652152921));
#210089=CARTESIAN_POINT('Ctrl Pts',(5.8819563278233,-3.351212326475,108.532539045507));
#210090=CARTESIAN_POINT('Ctrl Pts',(5.97092549082285,-3.18438970338775,
108.541425938093));
#210091=CARTESIAN_POINT('Ctrl Pts',(6.05966596986221,-3.01799587671501,
108.550289988048));
#210092=CARTESIAN_POINT('Ctrl Pts',(6.14152430585439,-2.84774604890684,
108.559154038003));
#210093=CARTESIAN_POINT('Ctrl Pts',(6.21618091139597,-2.67420714919326,
108.568018087958));
#210094=CARTESIAN_POINT('Ctrl Pts',(6.28755863200182,-2.50829000082916,
108.576492832778));
#210095=CARTESIAN_POINT('Ctrl Pts',(6.35235347621247,-2.33936670065238,
108.584967577599));
#210096=CARTESIAN_POINT('Ctrl Pts',(6.41032417248772,-2.16795595057179,
108.593442322419));
#210097=CARTESIAN_POINT('Ctrl Pts',(6.46647648092975,-2.00192190359221,
108.601651236848));
#210098=CARTESIAN_POINT('Ctrl Pts',(6.51617098957402,-1.83371374559318,
108.609860151277));
#210099=CARTESIAN_POINT('Ctrl Pts',(6.55925379458158,-1.66387459210939,
108.618069065706));
#210100=CARTESIAN_POINT('Ctrl Pts',(6.60234684230714,-1.49399506022973,
108.626279931763));
#210101=CARTESIAN_POINT('Ctrl Pts',(6.63882496717623,-1.32248410549377,
108.63449079782));
#210102=CARTESIAN_POINT('Ctrl Pts',(6.66858508908188,-1.14989647780781,
108.642701663877));
#210103=CARTESIAN_POINT('Ctrl Pts',(6.69835759117187,-0.977237053821706,
108.650915945647));
#210104=CARTESIAN_POINT('Ctrl Pts',(6.72140646224253,-0.80350041519878,
108.659130227416));
#210105=CARTESIAN_POINT('Ctrl Pts',(6.73768031109416,-0.629247984100162,
108.667344509186));
#210106=CARTESIAN_POINT('Ctrl Pts',(6.75397247744739,-0.454799418134226,
108.675568036779));
#210107=CARTESIAN_POINT('Ctrl Pts',(6.76347435717635,-0.279834254788,108.683791564371));
#210108=CARTESIAN_POINT('Ctrl Pts',(6.76618663175958,-0.104916462950289,
108.692015091963));
#210109=CARTESIAN_POINT('Ctrl Pts',(6.76890064480531,0.0701134443878388,
108.700243890517));
#210110=CARTESIAN_POINT('Ctrl Pts',(6.76481638580924,0.24509556462914,108.708472689071));
#210111=CARTESIAN_POINT('Ctrl Pts',(6.75398654891632,0.419469542466905,
108.716701487625));
#210112=CARTESIAN_POINT('Ctrl Pts',(6.74314180561956,0.5940835321312,108.724941612461));
#210113=CARTESIAN_POINT('Ctrl Pts',(6.72553297473834,0.76808735420976,108.733181737297));
#210114=CARTESIAN_POINT('Ctrl Pts',(6.70126427248376,0.940928344951234,
108.741421862134));
#210115=CARTESIAN_POINT('Ctrl Pts',(6.69048997021494,1.01766261195728,108.745080137504));
#210116=CARTESIAN_POINT('Ctrl Pts',(6.67840368088764,1.09416784928394,108.748738412874));
#210117=CARTESIAN_POINT('Ctrl Pts',(6.66501768919725,1.17039660059648,108.752396688244));
#210118=CARTESIAN_POINT('Ctrl Pts',(6.63410429598899,1.34643804882107,108.760845050352));
#210119=CARTESIAN_POINT('Ctrl Pts',(6.59618518998594,1.52140684464478,108.76929341246));
#210120=CARTESIAN_POINT('Ctrl Pts',(6.55135103948677,1.69472374073644,108.777741774569));
#210121=CARTESIAN_POINT('Ctrl Pts',(6.50655830089898,1.86788054939779,108.786182333187));
#210122=CARTESIAN_POINT('Ctrl Pts',(6.45486333288775,2.03938817839978,108.794622891806));
#210123=CARTESIAN_POINT('Ctrl Pts',(6.39640792026916,2.20867714198294,108.803063450425));
#210124=CARTESIAN_POINT('Ctrl Pts',(6.33799750137578,2.37783580213028,108.81149751226));
#210125=CARTESIAN_POINT('Ctrl Pts',(6.27283712005258,2.54477888714468,108.819931574094));
#210126=CARTESIAN_POINT('Ctrl Pts',(6.20111860653571,2.70895127820282,108.828365635929));
#210127=CARTESIAN_POINT('Ctrl Pts',(6.12944426910723,2.87302254482733,108.836794502678));
#210128=CARTESIAN_POINT('Ctrl Pts',(6.05121998684421,3.03432621533776,108.845223369427));
#210129=CARTESIAN_POINT('Ctrl Pts',(5.96668614481783,3.19232602489767,108.853652236176));
#210130=CARTESIAN_POINT('Ctrl Pts',(5.88219147519993,3.35025261841853,108.862077197045));
#210131=CARTESIAN_POINT('Ctrl Pts',(5.79139323334351,3.50487811038034,108.870502157914));
#210132=CARTESIAN_POINT('Ctrl Pts',(5.69457846111091,3.65568942201764,108.878927118783));
#210133=CARTESIAN_POINT('Ctrl Pts',(5.59778920128535,3.80646099220353,108.887349859526));
#210134=CARTESIAN_POINT('Ctrl Pts',(5.49498675170909,3.95342010536718,108.895772600268));
#210135=CARTESIAN_POINT('Ctrl Pts',(5.38650257052733,4.09608093886126,108.904195341011));
#210136=CARTESIAN_POINT('Ctrl Pts',(5.27803183083916,4.23872409627888,108.912617038153));
#210137=CARTESIAN_POINT('Ctrl Pts',(5.16388096519308,4.37706977073814,108.921038735294));
#210138=CARTESIAN_POINT('Ctrl Pts',(5.04442318747724,4.51066333321852,108.929460432436));
#210139=CARTESIAN_POINT('Ctrl Pts',(4.92496353609314,4.64425899108374,108.93788226167));
#210140=CARTESIAN_POINT('Ctrl Pts',(4.80019702962241,4.773102140486,108.946304090904));
#210141=CARTESIAN_POINT('Ctrl Pts',(4.67053562242961,4.89677301900099,108.954725920138));
#210142=CARTESIAN_POINT('Ctrl Pts',(4.54081539464964,5.02050000051414,108.963151569914));
#210143=CARTESIAN_POINT('Ctrl Pts',(4.40619606946129,5.13904979115333,108.971577219691));
#210144=CARTESIAN_POINT('Ctrl Pts',(4.26712540358998,5.25204053583339,108.980002869468));
#210145=CARTESIAN_POINT('Ctrl Pts',(4.12802309634482,5.36505698818064,108.988430436249));
#210146=CARTESIAN_POINT('Ctrl Pts',(3.98446769129501,5.47251166655314,108.996858003031));
#210147=CARTESIAN_POINT('Ctrl Pts',(3.83693863843192,5.57406412637209,109.005285569812));
#210148=CARTESIAN_POINT('Ctrl Pts',(3.68930056888781,5.67569162844139,109.013719364149));
#210149=CARTESIAN_POINT('Ctrl Pts',(3.53768326227873,5.77140801246674,109.022153158486));
#210150=CARTESIAN_POINT('Ctrl Pts',(3.38259450415134,5.86091660241683,109.030586952823));
#210151=CARTESIAN_POINT('Ctrl Pts',(3.28931550483894,5.91475204349728,109.035659505506));
#210152=CARTESIAN_POINT('Ctrl Pts',(3.19478121801629,5.96634269262134,109.040732058189));
#210153=CARTESIAN_POINT('Ctrl Pts',(3.09910619832136,6.01563211736939,109.045804610872));
#210154=CARTESIAN_POINT('Ctrl Pts',(3.09910619832137,6.01563211736938,107.045755263024));
#210155=CARTESIAN_POINT('Ctrl Pts',(2.9337533076483,6.10081787314651,107.054504710927));
#210156=CARTESIAN_POINT('Ctrl Pts',(2.76488627843074,6.17918207037038,107.063254158829));
#210157=CARTESIAN_POINT('Ctrl Pts',(2.59307866646705,6.25045854553996,107.072003606731));
#210158=CARTESIAN_POINT('Ctrl Pts',(2.42127244185375,6.32173444515038,107.080752983982));
#210159=CARTESIAN_POINT('Ctrl Pts',(2.24652594672458,6.38592262741841,107.089502361232));
#210160=CARTESIAN_POINT('Ctrl Pts',(2.06943269687108,6.44280508110566,107.098251738482));
#210161=CARTESIAN_POINT('Ctrl Pts',(1.89234081822065,6.4996870943617,107.107001047987));
#210162=CARTESIAN_POINT('Ctrl Pts',(1.71290249405577,6.54926340459548,107.115750357493));
#210163=CARTESIAN_POINT('Ctrl Pts',(1.53172716625047,6.59136563150386,107.124499666998));
#210164=CARTESIAN_POINT('Ctrl Pts',(1.35055318107328,6.63346754640711,107.133248911665));
#210165=CARTESIAN_POINT('Ctrl Pts',(1.16764249714418,6.66809542395776,107.141998156333));
#210166=CARTESIAN_POINT('Ctrl Pts',(0.983616340614383,6.69513165624668,
107.150747401));
#210167=CARTESIAN_POINT('Ctrl Pts',(0.799591486713997,6.72216769715959,
107.159496583736));
#210168=CARTESIAN_POINT('Ctrl Pts',(0.614451459526995,6.74161215869368,
107.168245766471));
#210169=CARTESIAN_POINT('Ctrl Pts',(0.428825047910695,6.7533990018571,107.176994949207));
#210170=CARTESIAN_POINT('Ctrl Pts',(0.243199888597368,6.7651857655022,107.185744072918));
#210171=CARTESIAN_POINT('Ctrl Pts',(0.0570886373921497,6.76931499599834,
107.194493196628));
#210172=CARTESIAN_POINT('Ctrl Pts',(-0.128876626811008,6.76577266947847,
107.203242320339));
#210173=CARTESIAN_POINT('Ctrl Pts',(-0.314840698187959,6.76223036567994,
107.21199138793));
#210174=CARTESIAN_POINT('Ctrl Pts',(-0.500658497950996,6.75101660879225,
107.220740455522));
#210175=CARTESIAN_POINT('Ctrl Pts',(-0.685698951925902,6.73216948296221,
107.229489523113));
#210176=CARTESIAN_POINT('Ctrl Pts',(-0.870738280459446,6.71332247176298,
107.238238537492));
#210177=CARTESIAN_POINT('Ctrl Pts',(-1.05499998761201,6.68684221356194,
107.24698755187));
#210178=CARTESIAN_POINT('Ctrl Pts',(-1.23785829161361,6.65281863948533,
107.255736566249));
#210179=CARTESIAN_POINT('Ctrl Pts',(-1.43007412917341,6.61705395368875,
107.264933299948));
#210180=CARTESIAN_POINT('Ctrl Pts',(-1.62073882535726,6.57295372727806,
107.274130033647));
#210181=CARTESIAN_POINT('Ctrl Pts',(-1.80913696091445,6.52068343478299,
107.283326767346));
#210182=CARTESIAN_POINT('Ctrl Pts',(-1.98838356186044,6.4709521981522,107.29207676506));
#210183=CARTESIAN_POINT('Ctrl Pts',(-2.16557827572465,6.41382586850914,
107.300826762774));
#210184=CARTESIAN_POINT('Ctrl Pts',(-2.34011918621633,6.34949849943303,
107.309576760487));
#210185=CARTESIAN_POINT('Ctrl Pts',(-2.51465655691025,6.2851724349558,107.318326580746));
#210186=CARTESIAN_POINT('Ctrl Pts',(-2.68653996295249,6.21364572242408,
107.327076401004));
#210187=CARTESIAN_POINT('Ctrl Pts',(-2.85518555379904,6.1351613225226,107.335826221262));
#210188=CARTESIAN_POINT('Ctrl Pts',(-3.02382794858607,6.05667841000547,
107.3445758757));
#210189=CARTESIAN_POINT('Ctrl Pts',(-3.18923239109202,5.97123819492123,
107.353325530137));
#210190=CARTESIAN_POINT('Ctrl Pts',(-3.35083705967622,5.87913088810757,
107.362075184575));
#210191=CARTESIAN_POINT('Ctrl Pts',(-3.5124388804232,5.78702520443151,107.370824684824));
#210192=CARTESIAN_POINT('Ctrl Pts',(-3.67024081223607,5.68825280605837,
107.379574185073));
#210193=CARTESIAN_POINT('Ctrl Pts',(-3.82370687544316,5.58314917682563,
107.388323685322));
#210194=CARTESIAN_POINT('Ctrl Pts',(-3.97717043817738,5.47804726008077,
107.397073043012));
#210195=CARTESIAN_POINT('Ctrl Pts',(-4.12629803722392,5.36661448084289,
107.405822400703));
#210196=CARTESIAN_POINT('Ctrl Pts',(-4.27058317206847,5.24922931204626,
107.414571758393));
#210197=CARTESIAN_POINT('Ctrl Pts',(-4.4148661477477,5.13184589986846,107.423320985153));
#210198=CARTESIAN_POINT('Ctrl Pts',(-4.55430658194344,5.00851045723098,
107.432070211913));
#210199=CARTESIAN_POINT('Ctrl Pts',(-4.68843089001772,4.8796418710319,107.440819438673));
#210200=CARTESIAN_POINT('Ctrl Pts',(-4.82255336917744,4.75077504208053,
107.449568546129));
#210201=CARTESIAN_POINT('Ctrl Pts',(-4.95135966065026,4.61637541908209,
107.458317653585));
#210202=CARTESIAN_POINT('Ctrl Pts',(-5.0744123086912,4.47689945401985,107.467066761041));
#210203=CARTESIAN_POINT('Ctrl Pts',(-5.19746344226278,4.33742520555681,
107.475815760817));
#210204=CARTESIAN_POINT('Ctrl Pts',(-5.31476088454614,4.19287495491529,
107.484564760594));
#210205=CARTESIAN_POINT('Ctrl Pts',(-5.42590627628689,4.04373961586927,
107.49331376037));
#210206=CARTESIAN_POINT('Ctrl Pts',(-5.53706380672511,3.89458798906957,
107.502063715665));
#210207=CARTESIAN_POINT('Ctrl Pts',(-5.64206777071714,3.7408505015551,107.510813670959));
#210208=CARTESIAN_POINT('Ctrl Pts',(-5.74056148163865,3.58304938223389,
107.519563626254));
#210209=CARTESIAN_POINT('Ctrl Pts',(-5.83905138951744,3.42525435593519,
107.528313243695));
#210210=CARTESIAN_POINT('Ctrl Pts',(-5.93103139557517,3.26339625497429,
107.537062861136));
#210211=CARTESIAN_POINT('Ctrl Pts',(-6.01618907820715,3.0980248506526,107.545812478577));
#210212=CARTESIAN_POINT('Ctrl Pts',(-6.10134392544859,2.93265895249898,
107.554561804693));
#210213=CARTESIAN_POINT('Ctrl Pts',(-6.17967677261715,2.76378023986296,
107.563311130809));
#210214=CARTESIAN_POINT('Ctrl Pts',(-6.25092157009115,2.59196229227379,
107.572060456925));
#210215=CARTESIAN_POINT('Ctrl Pts',(-6.32216437407663,2.42014915229329,
107.580809538228));
#210216=CARTESIAN_POINT('Ctrl Pts',(-6.38631941548848,2.24539720663063,
107.58955861953));
#210217=CARTESIAN_POINT('Ctrl Pts',(-6.44316881037478,2.06829994947871,
107.598307700832));
#210218=CARTESIAN_POINT('Ctrl Pts',(-6.5000233452452,1.89118668024629,107.607057573175));
#210219=CARTESIAN_POINT('Ctrl Pts',(-6.54957082411051,1.71172794807877,
107.615807445517));
#210220=CARTESIAN_POINT('Ctrl Pts',(-6.59164294296045,1.53053334250509,
107.62455731786));
#210221=CARTESIAN_POINT('Ctrl Pts',(-6.633712140821,1.34935131693768,107.633306582714));
#210222=CARTESIAN_POINT('Ctrl Pts',(-6.66830695239661,1.16643393829932,
107.642055847569));
#210223=CARTESIAN_POINT('Ctrl Pts',(-6.69530988153964,0.982402458342671,
107.650805112424));
#210224=CARTESIAN_POINT('Ctrl Pts',(-6.72231419690463,0.798361530948761,
107.659554826431));
#210225=CARTESIAN_POINT('Ctrl Pts',(-6.74172580829262,0.6132066713642,107.668304540438));
#210226=CARTESIAN_POINT('Ctrl Pts',(-6.75347878028168,0.427566795115138,
107.677054254445));
#210227=CARTESIAN_POINT('Ctrl Pts',(-6.76248992368204,0.285234494207695,
107.683762764234));
#210228=CARTESIAN_POINT('Ctrl Pts',(-6.76699999999989,0.142617266095235,
107.690471274022));
#210229=CARTESIAN_POINT('Ctrl Pts',(-6.767,5.22501239580748E-12,107.69717978381));
#210230=CARTESIAN_POINT('',(-6.76742387024867,0.00103549087071322,107.30355369317));
#210231=CARTESIAN_POINT('Ctrl Pts',(3.09910619832136,6.01563211736939,106.651504649108));
#210232=CARTESIAN_POINT('Ctrl Pts',(2.9439492773614,6.0955651594966,106.659704480459));
#210233=CARTESIAN_POINT('Ctrl Pts',(2.78560761231443,6.16953806982017,106.66790431181));
#210234=CARTESIAN_POINT('Ctrl Pts',(2.62458091016097,6.23729621278472,106.676104143161));
#210235=CARTESIAN_POINT('Ctrl Pts',(2.46359874742784,6.30503561408488,106.684301706467));
#210236=CARTESIAN_POINT('Ctrl Pts',(2.29993335547208,6.36656352928214,106.692499269774));
#210237=CARTESIAN_POINT('Ctrl Pts',(2.13410633458906,6.42167261332021,106.70069683308));
#210238=CARTESIAN_POINT('Ctrl Pts',(1.96830004468343,6.4767748078588,106.708893371562));
#210239=CARTESIAN_POINT('Ctrl Pts',(1.80033300415287,6.52545965556149,106.717089910045));
#210240=CARTESIAN_POINT('Ctrl Pts',(1.6307439661636,6.56756904164859,106.725286448527));
#210241=CARTESIAN_POINT('Ctrl Pts',(1.461145293775,6.60968081998136,106.733483452657));
#210242=CARTESIAN_POINT('Ctrl Pts',(1.28992478855158,6.64521630602577,106.741680456787));
#210243=CARTESIAN_POINT('Ctrl Pts',(1.11763349252699,6.67406805302298,106.749877460917));
#210244=CARTESIAN_POINT('Ctrl Pts',(0.945301081621044,6.7029266850816,106.758076421147));
#210245=CARTESIAN_POINT('Ctrl Pts',(0.771897724715815,6.72509834213783,
106.766275381376));
#210246=CARTESIAN_POINT('Ctrl Pts',(0.5979817694663,6.74052719031575,106.774474341605));
#210247=CARTESIAN_POINT('Ctrl Pts',(0.423900403987636,6.75597071276153,
106.782681099807));
#210248=CARTESIAN_POINT('Ctrl Pts',(0.249305823948718,6.76465858239079,
106.790887858009));
#210249=CARTESIAN_POINT('Ctrl Pts',(0.0747595227450543,6.76658702846265,
106.799094616211));
#210250=CARTESIAN_POINT('Ctrl Pts',(-0.0998726519923158,6.7685164232941,
106.807305411985));
#210251=CARTESIAN_POINT('Ctrl Pts',(-0.274456142191708,6.76367977437215,
106.815516207759));
#210252=CARTESIAN_POINT('Ctrl Pts',(-0.448432463893874,6.7521253931874,
106.823727003534));
#210253=CARTESIAN_POINT('Ctrl Pts',(-0.622646552553638,6.74055522106033,
106.831949020697));
#210254=CARTESIAN_POINT('Ctrl Pts',(-0.796251457698808,6.72224900732025,
106.84017103786));
#210255=CARTESIAN_POINT('Ctrl Pts',(-0.968695606756374,6.69730675879871,
106.848393055023));
#210256=CARTESIAN_POINT('Ctrl Pts',(-1.11706527516134,6.67584663293977,
106.855467217682));
#210257=CARTESIAN_POINT('Ctrl Pts',(-1.26457568858267,6.64947488513452,
106.862541380342));
#210258=CARTESIAN_POINT('Ctrl Pts',(-1.41088394946056,6.61828493502317,
106.869615543001));
#210259=CARTESIAN_POINT('Ctrl Pts',(-1.59569767350388,6.57888640210221,
106.878551486452));
#210260=CARTESIAN_POINT('Ctrl Pts',(-1.77897792879254,6.53171723688859,
106.887487429903));
#210261=CARTESIAN_POINT('Ctrl Pts',(-1.96008466387585,6.4769095339088,106.896423373353));
#210262=CARTESIAN_POINT('Ctrl Pts',(-2.140919147501,6.42218422144336,106.905345883711));
#210263=CARTESIAN_POINT('Ctrl Pts',(-2.31958638389205,6.35984335785542,
106.914268394069));
#210264=CARTESIAN_POINT('Ctrl Pts',(-2.49545887738146,6.2900694742823,106.923190904426));
#210265=CARTESIAN_POINT('Ctrl Pts',(-2.67090042868285,6.22046655837706,
106.932091551865));
#210266=CARTESIAN_POINT('Ctrl Pts',(-2.84356066487769,6.1434670678563,106.940992199303));
#210267=CARTESIAN_POINT('Ctrl Pts',(-3.01283012577512,6.05930223979807,
106.949892846741));
#210268=CARTESIAN_POINT('Ctrl Pts',(-3.18183800161143,5.97526747809424,
106.958779739327));
#210269=CARTESIAN_POINT('Ctrl Pts',(-3.34746532457885,5.88408958125895,
106.967666631913));
#210270=CARTESIAN_POINT('Ctrl Pts',(-3.50912261682026,5.78604765449789,
106.9765535245));
#210271=CARTESIAN_POINT('Ctrl Pts',(-3.67036438947681,5.68825773208592,
106.985417574454));
#210272=CARTESIAN_POINT('Ctrl Pts',(-3.82765627358926,5.58363911886481,
106.994281624409));
#210273=CARTESIAN_POINT('Ctrl Pts',(-3.98043407301949,5.47251620283992,
107.003145674364));
#210274=CARTESIAN_POINT('Ctrl Pts',(-4.12650193940196,5.36627375589745,
107.011620419185));
#210275=CARTESIAN_POINT('Ctrl Pts',(-4.26844347634824,5.25408617516802,
107.020095164005));
#210276=CARTESIAN_POINT('Ctrl Pts',(-4.4057864497103,5.13627635155558,107.028569908826));
#210277=CARTESIAN_POINT('Ctrl Pts',(-4.53882133626306,5.02216191136675,
107.036778823255));
#210278=CARTESIAN_POINT('Ctrl Pts',(-4.66741275280672,4.90288166908814,
107.044987737684));
#210279=CARTESIAN_POINT('Ctrl Pts',(-4.79115113310689,4.77882410428848,
107.053196652113));
#210280=CARTESIAN_POINT('Ctrl Pts',(-4.91491893157851,4.65473704543287,
107.06140751817));
#210281=CARTESIAN_POINT('Ctrl Pts',(-5.0338311436749,4.5258706533721,107.069618384227));
#210282=CARTESIAN_POINT('Ctrl Pts',(-5.14751596904057,4.39264935414522,
107.077829250284));
#210283=CARTESIAN_POINT('Ctrl Pts',(-5.2612480871909,4.25937263497819,107.086043532053));
#210284=CARTESIAN_POINT('Ctrl Pts',(-5.36974825542041,4.12173767012273,
107.094257813823));
#210285=CARTESIAN_POINT('Ctrl Pts',(-5.47268571603573,3.98020100667021,
107.102472095593));
#210286=CARTESIAN_POINT('Ctrl Pts',(-5.57573904089067,3.83850503252758,
107.110695623185));
#210287=CARTESIAN_POINT('Ctrl Pts',(-5.67321694279769,3.69289887626075,
107.118919150777));
#210288=CARTESIAN_POINT('Ctrl Pts',(-5.76483214252082,3.54386785427432,
107.12714267837));
#210289=CARTESIAN_POINT('Ctrl Pts',(-5.85650606402328,3.39474130919987,
107.135371476923));
#210290=CARTESIAN_POINT('Ctrl Pts',(-5.94230961837022,3.24218583195639,
107.143600275477));
#210291=CARTESIAN_POINT('Ctrl Pts',(-6.02200209756949,3.08671018025156,
107.151829074031));
#210292=CARTESIAN_POINT('Ctrl Pts',(-6.10180426708943,2.93102052875326,
107.160069198867));
#210293=CARTESIAN_POINT('Ctrl Pts',(-6.17547841088812,2.77240299643548,
107.168309323704));
#210294=CARTESIAN_POINT('Ctrl Pts',(-6.24283205184973,2.61138602515939,
107.17654944854));
#210295=CARTESIAN_POINT('Ctrl Pts',(-6.27273428885559,2.53990113483536,
107.18020772391));
#210296=CARTESIAN_POINT('Ctrl Pts',(-6.30139141788821,2.46794351755978,
107.18386599928));
#210297=CARTESIAN_POINT('Ctrl Pts',(-6.32878977979195,2.39556025246726,
107.18752427465));
#210298=CARTESIAN_POINT('Ctrl Pts',(-6.40195836908091,2.20225740415991,
107.197293867774));
#210299=CARTESIAN_POINT('Ctrl Pts',(-6.46627366852963,2.00558245517283,
107.207063460898));
#210300=CARTESIAN_POINT('Ctrl Pts',(-6.52147440592114,1.80628363578802,
107.216833054022));
#210301=CARTESIAN_POINT('Ctrl Pts',(-6.57653288654883,1.60749842557613,
107.226577470115));
#210302=CARTESIAN_POINT('Ctrl Pts',(-6.62252368424138,1.40610290668516,
107.236321886207));
#210303=CARTESIAN_POINT('Ctrl Pts',(-6.65923584019387,1.20285785722065,
107.2460663023));
#210304=CARTESIAN_POINT('Ctrl Pts',(-6.6956926317681,1.00102655054363,107.255742937662));
#210305=CARTESIAN_POINT('Ctrl Pts',(-6.7229993837118,0.797371419371896,
107.265419573023));
#210306=CARTESIAN_POINT('Ctrl Pts',(-6.74099766105347,0.592654649582421,
107.275096208385));
#210307=CARTESIAN_POINT('Ctrl Pts',(-6.75818629335671,0.39714697874161,
107.28433754432));
#210308=CARTESIAN_POINT('Ctrl Pts',(-6.76688532234933,0.200671188027621,
107.293578880255));
#210309=CARTESIAN_POINT('Ctrl Pts',(-6.76699887320081,0.00390513750720152,
107.30282021619));
#210310=CARTESIAN_POINT('Ctrl Pts',(-6.767,4.98895312755119E-12,107.30282021619));
#210311=CARTESIAN_POINT('Ctrl Pts',(-6.76700000000014,-0.186007249522004,
107.311569728001));
#210312=CARTESIAN_POINT('Ctrl Pts',(-6.75932637294547,-0.372014355745178,
107.320319239812));
#210313=CARTESIAN_POINT('Ctrl Pts',(-6.74400518264218,-0.557389537482884,
107.329068751624));
#210314=CARTESIAN_POINT('Ctrl Pts',(-6.72868405705135,-0.74276393624739,
107.337818226479));
#210315=CARTESIAN_POINT('Ctrl Pts',(-6.70571545645783,-0.927506130238072,
107.346567701335));
#210316=CARTESIAN_POINT('Ctrl Pts',(-6.67517739404867,-1.11098863989762,
107.355317176191));
#210317=CARTESIAN_POINT('Ctrl Pts',(-6.64463945808747,-1.29447038981717,
107.364066614818));
#210318=CARTESIAN_POINT('Ctrl Pts',(-6.60653217008401,-1.47669218313478,
107.372816053445));
#210319=CARTESIAN_POINT('Ctrl Pts',(-6.56098496092723,-1.65703510599104,
107.381565492072));
#210320=CARTESIAN_POINT('Ctrl Pts',(-6.51543793658348,-1.83737729708517,
107.390314895197));
#210321=CARTESIAN_POINT('Ctrl Pts',(-6.46245112167477,-2.01584035510744,
107.399064298322));
#210322=CARTESIAN_POINT('Ctrl Pts',(-6.40220448374316,-2.19181813760608,
107.407813701447));
#210323=CARTESIAN_POINT('Ctrl Pts',(-6.34195808526573,-2.36779522066959,
107.416563069797));
#210324=CARTESIAN_POINT('Ctrl Pts',(-6.27445201433179,-2.54128677683979,
107.425312438147));
#210325=CARTESIAN_POINT('Ctrl Pts',(-6.19991555071984,-2.71170355384624,
107.434061806497));
#210326=CARTESIAN_POINT('Ctrl Pts',(-6.12537937716775,-2.88211966767303,
107.442811140799));
#210327=CARTESIAN_POINT('Ctrl Pts',(-6.04381298052602,-3.04946076371624,
107.451560475101));
#210328=CARTESIAN_POINT('Ctrl Pts',(-5.95549339335912,-3.21315848374398,
107.460309809403));
#210329=CARTESIAN_POINT('Ctrl Pts',(-5.86717414255502,-3.3768555803333,
107.469059110383));
#210330=CARTESIAN_POINT('Ctrl Pts',(-5.77210188876704,-3.53690907646582,
107.477808411363));
#210331=CARTESIAN_POINT('Ctrl Pts',(-5.67059953347117,-3.69277536969101,
107.486557712343));
#210332=CARTESIAN_POINT('Ctrl Pts',(-5.56909755631517,-3.8486410822473,
107.495306980729));
#210333=CARTESIAN_POINT('Ctrl Pts',(-5.46116568196996,-4.00031938297317,
107.504056249114));
#210334=CARTESIAN_POINT('Ctrl Pts',(-5.34717048533763,-4.14729511859648,
107.512805517499));
#210335=CARTESIAN_POINT('Ctrl Pts',(-5.23317570392007,-4.29427031887709,
107.521554754016));
#210336=CARTESIAN_POINT('Ctrl Pts',(-5.11311782003695,-4.43654276189339,
107.530303990533));
#210337=CARTESIAN_POINT('Ctrl Pts',(-4.98740458984944,-4.57362924351643,
107.53905322705));
#210338=CARTESIAN_POINT('Ctrl Pts',(-4.86169180711944,-4.71071523720059,
107.547802432426));
#210339=CARTESIAN_POINT('Ctrl Pts',(-4.73032391204383,-4.84261509523031,
107.556551637801));
#210340=CARTESIAN_POINT('Ctrl Pts',(-4.59374707013821,-4.96888084538125,
107.565300843177));
#210341=CARTESIAN_POINT('Ctrl Pts',(-4.45717070301695,-5.09514615659244,
107.574050018137));
#210342=CARTESIAN_POINT('Ctrl Pts',(-4.3153856357132,-5.21577720459295,
107.582799193097));
#210343=CARTESIAN_POINT('Ctrl Pts',(-4.16887341029819,-5.33036429232644,
107.591548368058));
#210344=CARTESIAN_POINT('Ctrl Pts',(-4.02236168204035,-5.44495099123372,
107.60029751333));
#210345=CARTESIAN_POINT('Ctrl Pts',(-3.87112305348513,-5.55349359438359,
107.609046658602));
#210346=CARTESIAN_POINT('Ctrl Pts',(-3.71567117018127,-5.65562346298653,
107.617795803874));
#210347=CARTESIAN_POINT('Ctrl Pts',(-3.56021980146169,-5.75775299351428,
107.626544920184));
#210348=CARTESIAN_POINT('Ctrl Pts',(-3.40055544538682,-5.8534696746368,
107.635294036494));
#210349=CARTESIAN_POINT('Ctrl Pts',(-3.23722035987167,-5.9424484298673,
107.644043152804));
#210350=CARTESIAN_POINT('Ctrl Pts',(-3.07388580147504,-6.03142689794364,
107.652792240879));
#210351=CARTESIAN_POINT('Ctrl Pts',(-2.90688078896912,-6.11366734656623,
107.661541328954));
#210352=CARTESIAN_POINT('Ctrl Pts',(-2.73677250721714,-6.18889046952202,
107.670290417029));
#210353=CARTESIAN_POINT('Ctrl Pts',(-2.56666476031831,-6.26411335596184,
107.679039477595));
#210354=CARTESIAN_POINT('Ctrl Pts',(-2.3934540257552,-6.33231884500422,
107.687788538161));
#210355=CARTESIAN_POINT('Ctrl Pts',(-2.21772856065951,-6.39327529762602,
107.696537598727));
#210356=CARTESIAN_POINT('Ctrl Pts',(-2.04200363348871,-6.45423156364998,
107.705286632511));
#210357=CARTESIAN_POINT('Ctrl Pts',(-1.86376426189634,-6.50793874375556,
107.714035666294));
#210358=CARTESIAN_POINT('Ctrl Pts',(-1.68361577753508,-6.55421443909451,
107.722784700078));
#210359=CARTESIAN_POINT('Ctrl Pts',(-1.50346782968131,-6.60048999661793,
107.731533707806));
#210360=CARTESIAN_POINT('Ctrl Pts',(-1.32141105795296,-6.63933404237652,
107.740282715534));
#210361=CARTESIAN_POINT('Ctrl Pts',(-1.13806375487307,-6.67061465607512,
107.749031723262));
#210362=CARTESIAN_POINT('Ctrl Pts',(-0.954716982606139,-6.70189517921251,
107.75778070566));
#210363=CARTESIAN_POINT('Ctrl Pts',(-0.770079968905529,-6.72561226592189,
107.766529688058));
#210364=CARTESIAN_POINT('Ctrl Pts',(-0.584779765561904,-6.74168536983071,
107.775278670457));
#210365=CARTESIAN_POINT('Ctrl Pts',(-0.391489830654962,-6.75845151013832,
107.784404889467));
#210366=CARTESIAN_POINT('Ctrl Pts',(-0.197478578242002,-6.76689983031615,
107.793531108477));
#210367=CARTESIAN_POINT('Ctrl Pts',(-0.00346287645500613,-6.76699911397118,
107.802657327486));
#210368=CARTESIAN_POINT('Ctrl Pts',(0.184489834651114,-6.76709529501199,
107.811498352152));
#210369=CARTESIAN_POINT('Ctrl Pts',(0.372446404246595,-6.75935639738183,
107.820339376818));
#210370=CARTESIAN_POINT('Ctrl Pts',(0.559755019485561,-6.7438092587321,
107.829180401484));
#210371=CARTESIAN_POINT('Ctrl Pts',(0.745134705518991,-6.72842222659836,
107.837930380094));
#210372=CARTESIAN_POINT('Ctrl Pts',(0.929879431225777,-6.70538706057562,
107.846680358703));
#210373=CARTESIAN_POINT('Ctrl Pts',(1.11336163626546,-6.67478200894174,
107.855430337313));
#210374=CARTESIAN_POINT('Ctrl Pts',(1.29684196300447,-6.64417727061066,
107.86418022635));
#210375=CARTESIAN_POINT('Ctrl Pts',(1.47905951217247,-6.60600284890649,
107.872930115386));
#210376=CARTESIAN_POINT('Ctrl Pts',(1.6593953206683,-6.56038841607295,107.881680004423));
#210377=CARTESIAN_POINT('Ctrl Pts',(1.83972934300564,-6.51477443503324,
107.890429806795));
#210378=CARTESIAN_POINT('Ctrl Pts',(2.01818138406043,-6.46172066062211,
107.899179609167));
#210379=CARTESIAN_POINT('Ctrl Pts',(2.19414528353995,-6.40140730423549,
107.907929411539));
#210380=CARTESIAN_POINT('Ctrl Pts',(2.37010749863798,-6.34109452518717,
107.916679130156));
#210381=CARTESIAN_POINT('Ctrl Pts',(2.54358134866262,-6.27352239616584,
107.925428848772));
#210382=CARTESIAN_POINT('Ctrl Pts',(2.71397759435362,-6.19892043966903,
107.934178567388));
#210383=CARTESIAN_POINT('Ctrl Pts',(2.88437226557929,-6.12431917249607,
107.942928205157));
#210384=CARTESIAN_POINT('Ctrl Pts',(3.0516891268076,-6.04268832278897,107.951677842926));
#210385=CARTESIAN_POINT('Ctrl Pts',(3.21535986273659,-5.9543051612344,107.960427480694));
#210386=CARTESIAN_POINT('Ctrl Pts',(3.37902914072657,-5.86592278697547,
107.969177040523));
#210387=CARTESIAN_POINT('Ctrl Pts',(3.53905210621397,-5.77078835742049,
107.977926600352));
#210388=CARTESIAN_POINT('Ctrl Pts',(3.69488522831533,-5.66922500431736,
107.986676160182));
#210389=CARTESIAN_POINT('Ctrl Pts',(3.85071701406796,-5.56766252217194,
107.995425644979));
#210390=CARTESIAN_POINT('Ctrl Pts',(4.0023587882228,-5.45967138329462,108.004175129776));
#210391=CARTESIAN_POINT('Ctrl Pts',(4.1492954961122,-5.34561838199689,108.012924614573));
#210392=CARTESIAN_POINT('Ctrl Pts',(4.29623099275994,-5.23156632087094,
108.021674027246));
#210393=CARTESIAN_POINT('Ctrl Pts',(4.43846127435942,-5.11145267305039,
108.030423439918));
#210394=CARTESIAN_POINT('Ctrl Pts',(4.57550326054365,-4.98568540049956,
108.039172852591));
#210395=CARTESIAN_POINT('Ctrl Pts',(4.71254416257714,-4.85991912290426,
108.047922196046));
#210396=CARTESIAN_POINT('Ctrl Pts',(4.84439664018704,-4.72849950385478,
108.056671539501));
#210397=CARTESIAN_POINT('Ctrl Pts',(4.97061286794697,-4.5918728986112,108.065420882956));
#210398=CARTESIAN_POINT('Ctrl Pts',(5.09682813912642,-4.45524732884734,
108.074170160101));
#210399=CARTESIAN_POINT('Ctrl Pts',(5.21740705147802,-4.31341506235832,
108.082919437246));
#210400=CARTESIAN_POINT('Ctrl Pts',(5.33194007545664,-4.16685781275765,
108.091668714391));
#210401=CARTESIAN_POINT('Ctrl Pts',(5.44647226944451,-4.02030162521888,
108.100417928132));
#210402=CARTESIAN_POINT('Ctrl Pts',(5.55495848628077,-3.86902074887986,
108.109167141873));
#210403=CARTESIAN_POINT('Ctrl Pts',(5.6570302729175,-3.71352898080721,108.117916355614));
#210404=CARTESIAN_POINT('Ctrl Pts',(5.75910135376961,-3.55803828789647,
108.126665508858));
#210405=CARTESIAN_POINT('Ctrl Pts',(5.85475793592718,-3.39833700106772,
108.135414662102));
#210406=CARTESIAN_POINT('Ctrl Pts',(5.94367514427366,-3.23496750823614,
108.144163815346));
#210407=CARTESIAN_POINT('Ctrl Pts',(6.03259176732602,-3.07159909077798,
108.152912910999));
#210408=CARTESIAN_POINT('Ctrl Pts',(6.11476896835883,-2.9045627673152,108.161662006652));
#210409=CARTESIAN_POINT('Ctrl Pts',(6.18992765547842,-2.7344258300315,108.170411102305));
#210410=CARTESIAN_POINT('Ctrl Pts',(6.26508587283007,-2.56428995616285,
108.179160143273));
#210411=CARTESIAN_POINT('Ctrl Pts',(6.3332255482711,-2.39105376935333,108.187909184241));
#210412=CARTESIAN_POINT('Ctrl Pts',(6.39411526732979,-2.21530561054227,
108.196658225209));
#210413=CARTESIAN_POINT('Ctrl Pts',(6.4550046260279,-2.03955849185277,108.205407214398));
#210414=CARTESIAN_POINT('Ctrl Pts',(6.50864402040679,-1.86129970164755,
108.214156203587));
#210415=CARTESIAN_POINT('Ctrl Pts',(6.55485128368539,-1.68113463136301,
108.222905192776));
#210416=CARTESIAN_POINT('Ctrl Pts',(6.6019980955427,-1.49730620117119,108.231832078247));
#210417=CARTESIAN_POINT('Ctrl Pts',(6.64140720707822,-1.31149343245957,
108.240758963719));
#210418=CARTESIAN_POINT('Ctrl Pts',(6.67293928722839,-1.12435326697791,
108.24968584919));
#210419=CARTESIAN_POINT('Ctrl Pts',(6.70384625876219,-0.940923067009255,
108.258435763368));
#210420=CARTESIAN_POINT('Ctrl Pts',(6.72718554579766,-0.756217899524335,
108.267185677545));
#210421=CARTESIAN_POINT('Ctrl Pts',(6.74287786815305,-0.570865181257168,
108.275935591722));
#210422=CARTESIAN_POINT('Ctrl Pts',(6.7585698819083,-0.385516108076666,
108.284685333827));
#210423=CARTESIAN_POINT('Ctrl Pts',(6.76661520773395,-0.199519795229111,
108.293435075931));
#210424=CARTESIAN_POINT('Ctrl Pts',(6.76698651789578,-0.0135080204584527,
108.302184818036));
#210425=CARTESIAN_POINT('Ctrl Pts',(6.7673578212491,0.172500343510114,108.310934399701));
#210426=CARTESIAN_POINT('Ctrl Pts',(6.76005538995199,0.358523882208035,
108.319683981366));
#210427=CARTESIAN_POINT('Ctrl Pts',(6.74510402742385,0.543930748561455,
108.328433563031));
#210428=CARTESIAN_POINT('Ctrl Pts',(6.73015291918063,0.729334461612219,
108.337182995888));
#210429=CARTESIAN_POINT('Ctrl Pts',(6.70755316306637,0.914121237631574,
108.345932428744));
#210430=CARTESIAN_POINT('Ctrl Pts',(6.67738151874627,1.09766345165802,108.354681861601));
#210431=CARTESIAN_POINT('Ctrl Pts',(6.6472103474763,1.28120278799349,108.363431157278));
#210432=CARTESIAN_POINT('Ctrl Pts',(6.6094675720521,1.46349731860019,108.372180452956));
#210433=CARTESIAN_POINT('Ctrl Pts',(6.56428138111599,1.64392790277856,108.380929748633));
#210434=CARTESIAN_POINT('Ctrl Pts',(6.51909583859935,1.82435589778752,108.389678918759));
#210435=CARTESIAN_POINT('Ctrl Pts',(6.46646716392969,2.00291972191962,108.398428088885));
#210436=CARTESIAN_POINT('Ctrl Pts',(6.40657409872986,2.17901292274362,108.40717725901));
#210437=CARTESIAN_POINT('Ctrl Pts',(6.34668181342182,2.35510383058691,108.415926315209));
#210438=CARTESIAN_POINT('Ctrl Pts',(6.27952541914159,2.5287239082231,108.424675371408));
#210439=CARTESIAN_POINT('Ctrl Pts',(6.20533299175627,2.69928350890031,108.433424427608));
#210440=CARTESIAN_POINT('Ctrl Pts',(6.12831602991661,2.87633637965384,108.442506563766));
#210441=CARTESIAN_POINT('Ctrl Pts',(6.04371690605384,3.05009086601238,108.451588699924));
#210442=CARTESIAN_POINT('Ctrl Pts',(5.95184520316745,3.21991112882525,108.460670836082));
#210443=CARTESIAN_POINT('Ctrl Pts',(5.86333549509391,3.38351691182816,108.469420616426));
#210444=CARTESIAN_POINT('Ctrl Pts',(5.76807618099487,3.54347103711811,108.478170396769));
#210445=CARTESIAN_POINT('Ctrl Pts',(5.66639083309136,3.69923018027511,108.486920177113));
#210446=CARTESIAN_POINT('Ctrl Pts',(5.56470914082328,3.85498372381866,108.495669642898));
#210447=CARTESIAN_POINT('Ctrl Pts',(5.45660203372202,4.00654234701814,108.504419108683));
#210448=CARTESIAN_POINT('Ctrl Pts',(5.34243669839359,4.15339127986486,108.513168574468));
#210449=CARTESIAN_POINT('Ctrl Pts',(5.22827486050731,4.3002357140111,108.521917772214));
#210450=CARTESIAN_POINT('Ctrl Pts',(5.10805534167248,4.44237052028313,108.53066696996));
#210451=CARTESIAN_POINT('Ctrl Pts',(4.98218644340084,4.57931296628577,108.539416167706));
#210452=CARTESIAN_POINT('Ctrl Pts',(4.85632073219736,4.71625194483206,108.548165143917));
#210453=CARTESIAN_POINT('Ctrl Pts',(4.72480612170486,4.84799861524345,108.556914120129));
#210454=CARTESIAN_POINT('Ctrl Pts',(4.58808925235497,4.97410554898313,108.565663096341));
#210455=CARTESIAN_POINT('Ctrl Pts',(4.4513634947424,5.10022068121039,108.574412641342));
#210456=CARTESIAN_POINT('Ctrl Pts',(4.30943501210277,5.22069514871671,108.583162186344));
#210457=CARTESIAN_POINT('Ctrl Pts',(4.16278587431984,5.33511975166099,108.591911731346));
#210458=CARTESIAN_POINT('Ctrl Pts',(4.01614535740647,5.44953762807696,108.600660761999));
#210459=CARTESIAN_POINT('Ctrl Pts',(3.86478496658119,5.55790617532648,108.609409792653));
#210460=CARTESIAN_POINT('Ctrl Pts',(3.70921874747387,5.65985735539231,108.618158823307));
#210461=CARTESIAN_POINT('Ctrl Pts',(3.55365041606098,5.76180991976925,108.626907972756));
#210462=CARTESIAN_POINT('Ctrl Pts',(3.39387638174725,5.85734478552696,108.635657122206));
#210463=CARTESIAN_POINT('Ctrl Pts',(3.23043927904746,5.94613749121119,108.644406271656));
#210464=CARTESIAN_POINT('Ctrl Pts',(3.18691767070565,5.96978206944076,108.646736079572));
#210465=CARTESIAN_POINT('Ctrl Pts',(3.14313645919691,5.99294880633394,108.649065887488));
#210466=CARTESIAN_POINT('Ctrl Pts',(3.09910619832125,6.01563211736945,108.651395695404));
#210467=CARTESIAN_POINT('Origin',(0.,0.,4.30282021618968));
#210468=CARTESIAN_POINT('',(3.09910619832136,6.01563211736939,111.045833125094));
#210469=CARTESIAN_POINT('',(3.10339103771845,6.02380226238954,110.651315755419));
#210470=CARTESIAN_POINT('',(3.09910619832133,6.0156321173694,4.30282021618968));
#210471=CARTESIAN_POINT('',(-6.76699997532778,-0.000577852782592789,109.697179783856));
#210472=CARTESIAN_POINT('Ctrl Pts',(-6.76699997532778,-0.000577852782404293,
109.697179783856));
#210473=CARTESIAN_POINT('Ctrl Pts',(-6.76699458046941,-0.0637548549022476,
109.700160816967));
#210474=CARTESIAN_POINT('Ctrl Pts',(-6.76610444111257,-0.126923442093359,
109.70314185008));
#210475=CARTESIAN_POINT('Ctrl Pts',(-6.76433032192147,-0.190063925913952,
109.706122883192));
#210476=CARTESIAN_POINT('Ctrl Pts',(-6.75938101142591,-0.366208719812691,
109.714439155596));
#210477=CARTESIAN_POINT('Ctrl Pts',(-6.74754229967233,-0.542330844824209,
109.722755428001));
#210478=CARTESIAN_POINT('Ctrl Pts',(-6.72881619087231,-0.717859087464032,
109.731071700405));
#210479=CARTESIAN_POINT('Ctrl Pts',(-6.71010591501938,-0.893238920767603,
109.739380941391));
#210480=CARTESIAN_POINT('Ctrl Pts',(-6.68451988100679,-1.06802552789029,
109.747690182377));
#210481=CARTESIAN_POINT('Ctrl Pts',(-6.65211209900524,-1.2416495569476,
109.755999423363));
#210482=CARTESIAN_POINT('Ctrl Pts',(-6.61972577597116,-1.41515862002568,
109.764303162345));
#210483=CARTESIAN_POINT('Ctrl Pts',(-6.58052676930825,-1.58750629807545,
109.772606901328));
#210484=CARTESIAN_POINT('Ctrl Pts',(-6.53462072003349,-1.75812998532787,
109.78091064031));
#210485=CARTESIAN_POINT('Ctrl Pts',(-6.48873665470299,-1.9286719626164,
109.789210402716));
#210486=CARTESIAN_POINT('Ctrl Pts',(-6.43615203801171,-2.0974912591431,
109.797510165121));
#210487=CARTESIAN_POINT('Ctrl Pts',(-6.37702330088023,-2.26403684157979,
109.805809927527));
#210488=CARTESIAN_POINT('Ctrl Pts',(-6.31791204734133,-2.43053317867066,
109.814107235802));
#210489=CARTESIAN_POINT('Ctrl Pts',(-6.25226064665968,-2.59475681426828,
109.822404544076));
#210490=CARTESIAN_POINT('Ctrl Pts',(-6.18027502077515,-2.75617301118467,
109.830701852351));
#210491=CARTESIAN_POINT('Ctrl Pts',(-6.10828212178721,-2.91760551686656,
109.838999998948));
#210492=CARTESIAN_POINT('Ctrl Pts',(-6.02995385363303,-3.07622969625858,
109.847298145545));
#210493=CARTESIAN_POINT('Ctrl Pts',(-5.94554405206541,-3.23153135911594,
109.855596292142));
#210494=CARTESIAN_POINT('Ctrl Pts',(-5.86112576256122,-3.38684863853249,
109.86389527317));
#210495=CARTESIAN_POINT('Ctrl Pts',(-5.77062488649076,-3.53884242934451,
109.872194254199));
#210496=CARTESIAN_POINT('Ctrl Pts',(-5.67434089733694,-3.68702378359693,
109.880493235227));
#210497=CARTESIAN_POINT('Ctrl Pts',(-5.57803122491292,-3.83524466448086,
109.888794429966));
#210498=CARTESIAN_POINT('Ctrl Pts',(-5.47593555446037,-3.97965079007181,
109.897095624706));
#210499=CARTESIAN_POINT('Ctrl Pts',(-5.368396401207,-4.11978264954691,109.905396819445));
#210500=CARTESIAN_POINT('Ctrl Pts',(-5.26081068853162,-4.25997517956092,
109.913701608214));
#210501=CARTESIAN_POINT('Ctrl Pts',(-5.1477770077279,-4.39588947936302,
109.922006396982));
#210502=CARTESIAN_POINT('Ctrl Pts',(-5.02967792567021,-4.527099398514,109.930311185751));
#210503=CARTESIAN_POINT('Ctrl Pts',(-4.9114388382113,-4.65846486584584,
109.938625819772));
#210504=CARTESIAN_POINT('Ctrl Pts',(-4.78812258470138,-4.78511455081905,
109.946940453793));
#210505=CARTESIAN_POINT('Ctrl Pts',(-4.6601491752623,-4.90665860482489,
109.955255087814));
#210506=CARTESIAN_POINT('Ctrl Pts',(-4.53209484710205,-5.02827951221346,
109.963574979252));
#210507=CARTESIAN_POINT('Ctrl Pts',(-4.39937775159597,-5.14478812126722,
109.971894870689));
#210508=CARTESIAN_POINT('Ctrl Pts',(-4.26245079713221,-5.25583506229286,
109.980214762127));
#210509=CARTESIAN_POINT('Ctrl Pts',(-4.12531909247298,-5.36704805450229,
109.9885470945));
#210510=CARTESIAN_POINT('Ctrl Pts',(-3.98396522669826,-5.47278284874803,
109.996879426874));
#210511=CARTESIAN_POINT('Ctrl Pts',(-3.83887199634723,-5.57273279420977,
110.005211759247));
#210512=CARTESIAN_POINT('Ctrl Pts',(-3.72963352942183,-5.64798357458803,
110.011485044445));
#210513=CARTESIAN_POINT('Ctrl Pts',(-3.6182760621482,-5.71995619617045,
110.017758329644));
#210514=CARTESIAN_POINT('Ctrl Pts',(-3.50501443822741,-5.78853718894656,
110.024031614842));
#210515=CARTESIAN_POINT('Ctrl Pts',(-3.35931663649457,-5.87675859653582,
110.032101460845));
#210516=CARTESIAN_POINT('Ctrl Pts',(-3.21001676095259,-5.95963842679075,
110.040171306848));
#210517=CARTESIAN_POINT('Ctrl Pts',(-3.05755125178259,-6.03685922833411,
110.04824115285));
#210518=CARTESIAN_POINT('Ctrl Pts',(-2.90527756361614,-6.11398287628695,
110.056300845961));
#210519=CARTESIAN_POINT('Ctrl Pts',(-2.74984649503231,-6.18546149549647,
110.064360539071));
#210520=CARTESIAN_POINT('Ctrl Pts',(-2.59172408469217,-6.25102033821892,
110.072420232181));
#210521=CARTESIAN_POINT('Ctrl Pts',(-2.43376590958989,-6.31651108767043,
110.080471554019));
#210522=CARTESIAN_POINT('Ctrl Pts',(-2.27312229729032,-6.37609415478897,
110.088522875858));
#210523=CARTESIAN_POINT('Ctrl Pts',(-2.11028446764011,-6.42954029971326,
110.096574197696));
#210524=CARTESIAN_POINT('Ctrl Pts',(-1.94758008762283,-6.48294264419857,
110.104618921278));
#210525=CARTESIAN_POINT('Ctrl Pts',(-1.7826854219628,-6.53021796077703,
110.112663644859));
#210526=CARTESIAN_POINT('Ctrl Pts',(-1.6161121872759,-6.57118485496629,
110.12070836844));
#210527=CARTESIAN_POINT('Ctrl Pts',(-1.44963900052513,-6.61212714344251,
110.128748260164));
#210528=CARTESIAN_POINT('Ctrl Pts',(-1.28148961312893,-6.64676846336198,
110.136788151888));
#210529=CARTESIAN_POINT('Ctrl Pts',(-1.11219133697324,-6.67497711081931,
110.144828043613));
#210530=CARTESIAN_POINT('Ctrl Pts',(-0.939247605108738,-6.70379316773908,
110.153041056233));
#210531=CARTESIAN_POINT('Ctrl Pts',(-0.76510532443646,-6.72589625912002,
110.161254068853));
#210532=CARTESIAN_POINT('Ctrl Pts',(-0.590338581657058,-6.74120088404189,
110.169467081473));
#210533=CARTESIAN_POINT('Ctrl Pts',(-0.419315413730825,-6.75617767766082,
110.177504168015));
#210534=CARTESIAN_POINT('Ctrl Pts',(-0.247694653530352,-6.76464428539989,
110.185541254558));
#210535=CARTESIAN_POINT('Ctrl Pts',(-0.0760198752609056,-6.76657298627343,
110.1935783411));
#210536=CARTESIAN_POINT('Ctrl Pts',(0.095671333083986,-6.76850187173262,
110.20161619683));
#210537=CARTESIAN_POINT('Ctrl Pts',(0.267416196179675,-6.76389160011226,
110.209654052559));
#210538=CARTESIAN_POINT('Ctrl Pts',(0.438671077303047,-6.75276659495483,
110.217691908288));
#210539=CARTESIAN_POINT('Ctrl Pts',(0.609976279625294,-6.74163832084767,
110.225732125845));
#210540=CARTESIAN_POINT('Ctrl Pts',(0.78079084076752,-6.72399152711062,
110.233772343402));
#210541=CARTESIAN_POINT('Ctrl Pts',(0.950576331654277,-6.69990250956674,
110.241812560959));
#210542=CARTESIAN_POINT('Ctrl Pts',(1.12677642717072,-6.67490339350587,
110.250156543087));
#210543=CARTESIAN_POINT('Ctrl Pts',(1.30186773512499,-6.64296582534395,
110.258500525214));
#210544=CARTESIAN_POINT('Ctrl Pts',(1.47526128317876,-6.60423297184115,
110.266844507342));
#210545=CARTESIAN_POINT('Ctrl Pts',(1.64263327243482,-6.56684522118322,
110.274898722177));
#210546=CARTESIAN_POINT('Ctrl Pts',(1.80842310476819,-6.52312640021052,
110.282952937012));
#210547=CARTESIAN_POINT('Ctrl Pts',(1.97211815467876,-6.47325567114311,
110.291007151847));
#210548=CARTESIAN_POINT('Ctrl Pts',(2.13593570326556,-6.42334762208162,
110.29906739393));
#210549=CARTESIAN_POINT('Ctrl Pts',(2.29765499757764,-6.36727861993701,
110.307127636013));
#210550=CARTESIAN_POINT('Ctrl Pts',(2.45678429351917,-6.30527556377337,
110.315187878096));
#210551=CARTESIAN_POINT('Ctrl Pts',(2.61613606313192,-6.24318582308409,
110.323259388951));
#210552=CARTESIAN_POINT('Ctrl Pts',(2.77289027039732,-6.17514562334383,
110.331330899805));
#210553=CARTESIAN_POINT('Ctrl Pts',(2.92658010087692,-6.10142753076288,
110.339402410659));
#210554=CARTESIAN_POINT('Ctrl Pts',(2.94268839976087,-6.09370110498218,
110.34024838927));
#210555=CARTESIAN_POINT('Ctrl Pts',(2.95876306269006,-6.08591234500733,
110.341094367881));
#210556=CARTESIAN_POINT('Ctrl Pts',(2.97480357148381,-6.07806159158388,
110.341940346492));
#210557=CARTESIAN_POINT('Ctrl Pts',(3.13083748424129,-6.00169345448138,
110.350169596228));
#210558=CARTESIAN_POINT('Ctrl Pts',(3.2841580440009,-5.91920076592815,110.358398845964));
#210559=CARTESIAN_POINT('Ctrl Pts',(3.43425069767606,-5.83079849982072,
110.3666280957));
#210560=CARTESIAN_POINT('Ctrl Pts',(3.58416471667626,-5.74250144679124,
110.37484755129));
#210561=CARTESIAN_POINT('Ctrl Pts',(3.73085817330173,-5.64830900130154,
110.38306700688));
#210562=CARTESIAN_POINT('Ctrl Pts',(3.8738377741439,-5.54848356757194,110.39128646247));
#210563=CARTESIAN_POINT('Ctrl Pts',(4.01667591982277,-5.44875689494495,
110.399497786239));
#210564=CARTESIAN_POINT('Ctrl Pts',(4.15580723487193,-5.3434085363126,110.407709110009));
#210565=CARTESIAN_POINT('Ctrl Pts',(4.29076419683617,-5.2327460866307,110.415920433779));
#210566=CARTESIAN_POINT('Ctrl Pts',(4.42561473361974,-5.12217090381542,
110.424125282213));
#210567=CARTESIAN_POINT('Ctrl Pts',(4.55629719779224,-5.00629020304635,
110.432330130647));
#210568=CARTESIAN_POINT('Ctrl Pts',(4.68237410674298,-4.88545409603886,
110.440534979081));
#210569=CARTESIAN_POINT('Ctrl Pts',(4.8083768968647,-4.76468902686717,110.448735004001));
#210570=CARTESIAN_POINT('Ctrl Pts',(4.92977926722306,-4.63897460236606,
110.456935028921));
#210571=CARTESIAN_POINT('Ctrl Pts',(5.04617775972311,-4.50870036898394,
110.465135053841));
#210572=CARTESIAN_POINT('Ctrl Pts',(5.1625425638624,-4.37846383991634,110.473332705488));
#210573=CARTESIAN_POINT('Ctrl Pts',(5.27390613322989,-4.24367039513359,
110.481530357135));
#210574=CARTESIAN_POINT('Ctrl Pts',(5.37990259028466,-4.10474568262742,
110.489728008782));
#210575=CARTESIAN_POINT('Ctrl Pts',(5.48588485376347,-3.96583957299265,
110.497924562713));
#210576=CARTESIAN_POINT('Ctrl Pts',(5.58650121808187,-3.8228035820166,110.506121116644));
#210577=CARTESIAN_POINT('Ctrl Pts',(5.68142676034186,-3.67609561448984,
110.514317670575));
#210578=CARTESIAN_POINT('Ctrl Pts',(5.77635685141951,-3.52938061673941,
110.522514617283));
#210579=CARTESIAN_POINT('Ctrl Pts',(5.86559538219838,-3.37899359307046,
110.530711563992));
#210580=CARTESIAN_POINT('Ctrl Pts',(5.94886132904145,-3.22542057534132,
110.538908510701));
#210581=CARTESIAN_POINT('Ctrl Pts',(6.03214640585528,-3.07181227491323,
110.547107340621));
#210582=CARTESIAN_POINT('Ctrl Pts',(6.10945599481781,-2.91501683787723,
110.55530617054));
#210583=CARTESIAN_POINT('Ctrl Pts',(6.18055548909299,-2.75554402001539,
110.56350500046));
#210584=CARTESIAN_POINT('Ctrl Pts',(6.25172232367859,-2.59592016100806,
110.57171159572));
#210585=CARTESIAN_POINT('Ctrl Pts',(6.31666716609735,-2.43361418292214,
110.57991819098));
#210586=CARTESIAN_POINT('Ctrl Pts',(6.37520360554201,-2.26915578748664,
110.58812478624));
#210587=CARTESIAN_POINT('Ctrl Pts',(6.43376837695898,-2.10461779324486,
110.596335353539));
#210588=CARTESIAN_POINT('Ctrl Pts',(6.48591845429311,-1.93792564676811,
110.604545920838));
#210589=CARTESIAN_POINT('Ctrl Pts',(6.53151765006207,-1.7696231765344,110.612756488136));
#210590=CARTESIAN_POINT('Ctrl Pts',(6.57717973364994,-1.60108859310017,
110.620978378983));
#210591=CARTESIAN_POINT('Ctrl Pts',(6.61627279960274,-1.43093959721949,
110.62920026983));
#210592=CARTESIAN_POINT('Ctrl Pts',(6.64871178590921,-1.25973036317775,
110.637422160677));
#210593=CARTESIAN_POINT('Ctrl Pts',(6.67820648009823,-1.10406076386633,
110.644897799832));
#210594=CARTESIAN_POINT('Ctrl Pts',(6.70220079846837,-0.947514947705724,
110.652373438986));
#210595=CARTESIAN_POINT('Ctrl Pts',(6.72066816122545,-0.790511522174436,
110.659849078141));
#210596=CARTESIAN_POINT('Ctrl Pts',(6.74274297059785,-0.602838775664545,
110.668785021592));
#210597=CARTESIAN_POINT('Ctrl Pts',(6.75696648332447,-0.414121331288979,
110.677720965043));
#210598=CARTESIAN_POINT('Ctrl Pts',(6.76325812868762,-0.225007743735387,
110.686656908494));
#210599=CARTESIAN_POINT('Ctrl Pts',(6.76954031603903,-0.036178444063279,
110.695579418851));
#210600=CARTESIAN_POINT('Ctrl Pts',(6.76791441933773,0.153045553073953,
110.704501929209));
#210601=CARTESIAN_POINT('Ctrl Pts',(6.75835166428807,0.342011376732841,
110.713424439567));
#210602=CARTESIAN_POINT('Ctrl Pts',(6.74881234095588,0.530514175482277,
110.722325087005));
#210603=CARTESIAN_POINT('Ctrl Pts',(6.73137498658916,0.718759805913537,
110.731225734443));
#210604=CARTESIAN_POINT('Ctrl Pts',(6.70606274514698,0.906096826035595,
110.740126381882));
#210605=CARTESIAN_POINT('Ctrl Pts',(6.68078962064989,1.09314433991435,110.749013274468));
#210606=CARTESIAN_POINT('Ctrl Pts',(6.64766591877159,1.27928578978323,110.757900167054));
#210607=CARTESIAN_POINT('Ctrl Pts',(6.60676653390246,1.46387327542604,110.76678705964));
#210608=CARTESIAN_POINT('Ctrl Pts',(6.56597227571975,1.64798630232613,110.775651109595));
#210609=CARTESIAN_POINT('Ctrl Pts',(6.51744227172776,1.83055308395059,110.78451515955));
#210610=CARTESIAN_POINT('Ctrl Pts',(6.46130242130803,2.01093511093694,110.793379209505));
#210611=CARTESIAN_POINT('Ctrl Pts',(6.4076282081688,2.1833948394643,110.801853954325));
#210612=CARTESIAN_POINT('Ctrl Pts',(6.34699825849784,2.35385733499185,110.810328699146));
#210613=CARTESIAN_POINT('Ctrl Pts',(6.27956660306105,2.52177165455564,110.818803443966));
#210614=CARTESIAN_POINT('Ctrl Pts',(6.21425010079115,2.68441894482156,110.827012358395));
#210615=CARTESIAN_POINT('Ctrl Pts',(6.14261396346791,2.84451826535749,110.835221272824));
#210616=CARTESIAN_POINT('Ctrl Pts',(6.06489446879602,3.0015569430493,110.843430187253));
#210617=CARTESIAN_POINT('Ctrl Pts',(5.98715649670913,3.1586329558889,110.85164105331));
#210618=CARTESIAN_POINT('Ctrl Pts',(5.90333244380904,3.31264655705338,110.859851919367));
#210619=CARTESIAN_POINT('Ctrl Pts',(5.81370476294961,3.46310928635772,110.868062785424));
#210620=CARTESIAN_POINT('Ctrl Pts',(5.72403979705445,3.61363460802397,110.876277067193));
#210621=CARTESIAN_POINT('Ctrl Pts',(5.62856657547765,3.76060580934986,110.884491348963));
#210622=CARTESIAN_POINT('Ctrl Pts',(5.52761115655308,3.90356297527655,110.892705630733));
#210623=CARTESIAN_POINT('Ctrl Pts',(5.42654210433466,4.04668105077916,110.900929158325));
#210624=CARTESIAN_POINT('Ctrl Pts',(5.31997873544013,4.18577577574331,110.909152685918));
#210625=CARTESIAN_POINT('Ctrl Pts',(5.20828832234937,4.32041916384039,110.91737621351));
#210626=CARTESIAN_POINT('Ctrl Pts',(5.09652632004847,4.45514885311172,110.925605012064));
#210627=CARTESIAN_POINT('Ctrl Pts',(4.97963095984321,4.58542125363471,110.933833810618));
#210628=CARTESIAN_POINT('Ctrl Pts',(4.85800667665738,4.710844948579,110.942062609171));
#210629=CARTESIAN_POINT('Ctrl Pts',(4.73621498737851,4.83644127920258,110.950302734008));
#210630=CARTESIAN_POINT('Ctrl Pts',(4.60968163088599,4.95717532873931,110.958542858844));
#210631=CARTESIAN_POINT('Ctrl Pts',(4.47884517990586,5.0726950287233,110.966782983681));
#210632=CARTESIAN_POINT('Ctrl Pts',(4.42075919508984,5.12398100819579,110.970441259051));
#210633=CARTESIAN_POINT('Ctrl Pts',(4.36182547515876,5.17423980228559,110.974099534421));
#210634=CARTESIAN_POINT('Ctrl Pts',(4.3020842137546,5.22344334876559,110.977757809791));
#210635=CARTESIAN_POINT('Ctrl Pts',(4.16411366449314,5.33707737948233,110.986206480781));
#210636=CARTESIAN_POINT('Ctrl Pts',(4.02151831318311,5.44534026955538,110.994655151772));
#210637=CARTESIAN_POINT('Ctrl Pts',(3.87474377772024,5.54785090436092,111.003103822762));
#210638=CARTESIAN_POINT('Ctrl Pts',(3.72812333430209,5.6502539178187,111.011543623869));
#210639=CARTESIAN_POINT('Ctrl Pts',(3.57733272790036,5.74691652811108,111.019983424977));
#210640=CARTESIAN_POINT('Ctrl Pts',(3.42284988151364,5.83749841016013,111.028423226084));
#210641=CARTESIAN_POINT('Ctrl Pts',(3.31662578451512,5.89978350426696,111.034226525754));
#210642=CARTESIAN_POINT('Ctrl Pts',(3.20865666708964,5.9591944014046,111.040029825424));
#210643=CARTESIAN_POINT('Ctrl Pts',(3.09910619832136,6.01563211736939,111.045833125094));
#210644=CARTESIAN_POINT('Ctrl Pts',(3.09910619832136,6.01563211736939,109.045804610872));
#210645=CARTESIAN_POINT('Ctrl Pts',(2.94506703026755,6.09498932060019,109.053971547213));
#210646=CARTESIAN_POINT('Ctrl Pts',(2.78807013938386,6.16837911515625,109.062138483553));
#210647=CARTESIAN_POINT('Ctrl Pts',(2.62860754293066,6.23560032276348,109.070305419894));
#210648=CARTESIAN_POINT('Ctrl Pts',(2.46967645305377,6.3025974746065,109.078445134926));
#210649=CARTESIAN_POINT('Ctrl Pts',(2.30797898013572,6.36360017218061,109.086584849959));
#210650=CARTESIAN_POINT('Ctrl Pts',(2.14401205532608,6.4183721695315,109.094724564992));
#210651=CARTESIAN_POINT('Ctrl Pts',(1.98018853500527,6.47309626362207,109.102857161079));
#210652=CARTESIAN_POINT('Ctrl Pts',(1.8140998585861,6.52160038912026,109.110989757166));
#210653=CARTESIAN_POINT('Ctrl Pts',(1.64626392994504,6.56369591563792,109.119122353253));
#210654=CARTESIAN_POINT('Ctrl Pts',(1.47854274294873,6.60576266339535,109.127249389461));
#210655=CARTESIAN_POINT('Ctrl Pts',(1.30907703569928,6.64142944631574,109.135376425669));
#210656=CARTESIAN_POINT('Ctrl Pts',(1.13840086960319,6.67055713266041,109.143503461877));
#210657=CARTESIAN_POINT('Ctrl Pts',(0.967806289803363,6.69967089544386,
109.151626613215));
#210658=CARTESIAN_POINT('Ctrl Pts',(0.796002763603998,6.72225172468213,
109.159749764552));
#210659=CARTESIAN_POINT('Ctrl Pts',(0.623535550787872,6.73821136629771,
109.16787291589));
#210660=CARTESIAN_POINT('Ctrl Pts',(0.451116802540562,6.75416652313537,
109.175993784561));
#210661=CARTESIAN_POINT('Ctrl Pts',(0.278035103555909,6.76350416537771,
109.184114653233));
#210662=CARTESIAN_POINT('Ctrl Pts',(0.104841824076422,6.76618778869788,
109.192235521905));
#210663=CARTESIAN_POINT('Ctrl Pts',(-0.0683608154309681,6.76887155705133,
109.200356829459));
#210664=CARTESIAN_POINT('Ctrl Pts',(-0.24167468136091,6.76490057840372,
109.208478137014));
#210665=CARTESIAN_POINT('Ctrl Pts',(-0.414547214367548,6.75429045918667,
109.216599444568));
#210666=CARTESIAN_POINT('Ctrl Pts',(-0.504377791882841,6.74877707241437,
109.220819558285));
#210667=CARTESIAN_POINT('Ctrl Pts',(-0.594089216401721,6.74147184052699,
109.225039672002));
#210668=CARTESIAN_POINT('Ctrl Pts',(-0.683604340951769,6.73238249842,109.229259785719));
#210669=CARTESIAN_POINT('Ctrl Pts',(-0.874178147161722,6.71303168446559,
109.238244224245));
#210670=CARTESIAN_POINT('Ctrl Pts',(-1.06376744316211,6.68560121564277,
109.24722866277));
#210671=CARTESIAN_POINT('Ctrl Pts',(-1.25171515143828,6.65022542322137,
109.256213101296));
#210672=CARTESIAN_POINT('Ctrl Pts',(-1.43998724624216,6.61478857429349,
109.265213046427));
#210673=CARTESIAN_POINT('Ctrl Pts',(-1.62661185548438,6.5713790370777,109.274212991557));
#210674=CARTESIAN_POINT('Ctrl Pts',(-1.81094420582182,6.52018175232872,
109.283212936688));
#210675=CARTESIAN_POINT('Ctrl Pts',(-1.99571094007356,6.46886381986429,
109.29223409042));
#210676=CARTESIAN_POINT('Ctrl Pts',(-2.17817437618374,6.40972148465066,
109.301255244152));
#210677=CARTESIAN_POINT('Ctrl Pts',(-2.3577043264137,6.34298977684894,109.310276397884));
#210678=CARTESIAN_POINT('Ctrl Pts',(-2.53741694978348,6.27619016900839,
109.319306730711));
#210679=CARTESIAN_POINT('Ctrl Pts',(-2.71418990258968,6.2017858502352,109.328337063538));
#210680=CARTESIAN_POINT('Ctrl Pts',(-2.8874135043512,6.12005982445354,109.337367396366));
#210681=CARTESIAN_POINT('Ctrl Pts',(-3.0608826825763,6.03821793692909,109.346410531358));
#210682=CARTESIAN_POINT('Ctrl Pts',(-3.23079223220093,5.94903368960606,
109.355453666351));
#210683=CARTESIAN_POINT('Ctrl Pts',(-3.39655550842975,5.85283689147028,
109.364496801343));
#210684=CARTESIAN_POINT('Ctrl Pts',(-3.54147080147756,5.76873872745437,
109.372402584743));
#210685=CARTESIAN_POINT('Ctrl Pts',(-3.68321749238951,5.67928176416991,
109.380308368143));
#210686=CARTESIAN_POINT('Ctrl Pts',(-3.8214214506314,5.58471369871852,109.388214151543));
#210687=CARTESIAN_POINT('Ctrl Pts',(-3.97269456865795,5.48120287089162,
109.396867539771));
#210688=CARTESIAN_POINT('Ctrl Pts',(-4.11985614833642,5.37147606331934,
109.405520928));
#210689=CARTESIAN_POINT('Ctrl Pts',(-4.26239728548914,5.25587845946373,
109.414174316228));
#210690=CARTESIAN_POINT('Ctrl Pts',(-4.40480677579062,5.14038761819514,
109.422819712438));
#210691=CARTESIAN_POINT('Ctrl Pts',(-4.54260409948993,5.01903698596568,
109.431465108649));
#210692=CARTESIAN_POINT('Ctrl Pts',(-4.67531106722114,4.89221375501107,
109.440110504859));
#210693=CARTESIAN_POINT('Ctrl Pts',(-4.81225624846365,4.7613402172778,109.449032005901));
#210694=CARTESIAN_POINT('Ctrl Pts',(-4.94378028079967,4.62463891862904,
109.457953506944));
#210695=CARTESIAN_POINT('Ctrl Pts',(-5.06939464124876,4.48258039205973,
109.466875007986));
#210696=CARTESIAN_POINT('Ctrl Pts',(-5.19088961850813,4.34518051681192,
109.475503938328));
#210697=CARTESIAN_POINT('Ctrl Pts',(-5.30685614307209,4.2027694485995,109.48413286867));
#210698=CARTESIAN_POINT('Ctrl Pts',(-5.41688922042392,4.0558106678758,109.492761799012));
#210699=CARTESIAN_POINT('Ctrl Pts',(-5.53251843540277,3.90137775680674,
109.501829585405));
#210700=CARTESIAN_POINT('Ctrl Pts',(-5.64159469459853,3.74192273199829,
109.510897371797));
#210701=CARTESIAN_POINT('Ctrl Pts',(-5.74369528692449,3.57802367948584,
109.51996515819));
#210702=CARTESIAN_POINT('Ctrl Pts',(-5.84579587925052,3.41412462697329,
109.529032944582));
#210703=CARTESIAN_POINT('Ctrl Pts',(-5.94092056834331,3.2457818596018,109.538100730975));
#210704=CARTESIAN_POINT('Ctrl Pts',(-6.02869878558639,3.07361024735884,
109.547168517368));
#210705=CARTESIAN_POINT('Ctrl Pts',(-6.10946478949627,2.91519266331201,
109.555511918433));
#210706=CARTESIAN_POINT('Ctrl Pts',(-6.18398210624984,2.75359092372838,
109.563855319498));
#210707=CARTESIAN_POINT('Ctrl Pts',(-6.25201121645123,2.58933287728094,
109.572198720563));
#210708=CARTESIAN_POINT('Ctrl Pts',(-6.32005143258252,2.42504801527847,
109.58054348371));
#210709=CARTESIAN_POINT('Ctrl Pts',(-6.38160120048745,2.25810629807558,
109.588888246857));
#210710=CARTESIAN_POINT('Ctrl Pts',(-6.43646945579045,2.08905479695401,
109.597233010004));
#210711=CARTESIAN_POINT('Ctrl Pts',(-6.49138068718608,1.91987088460614,
109.605584309268));
#210712=CARTESIAN_POINT('Ctrl Pts',(-6.53959984126778,1.74857421142531,
109.613935608532));
#210713=CARTESIAN_POINT('Ctrl Pts',(-6.58098568620455,1.57572726002021,
109.622286907796));
#210714=CARTESIAN_POINT('Ctrl Pts',(-6.62238729118817,1.4028144871717,109.630641387298));
#210715=CARTESIAN_POINT('Ctrl Pts',(-6.65695032667952,1.22835059338328,
109.638995866801));
#210716=CARTESIAN_POINT('Ctrl Pts',(-6.68458481328139,1.05290781839997,
109.647350346303));
#210717=CARTESIAN_POINT('Ctrl Pts',(-6.71225178347566,0.87725881517463,
109.655714646271));
#210718=CARTESIAN_POINT('Ctrl Pts',(-6.73297388082621,0.700628970344419,
109.664078946238));
#210719=CARTESIAN_POINT('Ctrl Pts',(-6.74671295041825,0.523596566698737,
109.672443246205));
#210720=CARTESIAN_POINT('Ctrl Pts',(-6.76025690161313,0.349078327393853,
109.68068875874));
#210721=CARTESIAN_POINT('Ctrl Pts',(-6.76701489743579,0.174169205078094,
109.688934271275));
#210722=CARTESIAN_POINT('Ctrl Pts',(-6.76699997532786,-0.000577851814927111,
109.69717978381));
#210723=CARTESIAN_POINT('',(-6.76441351452996,-0.00287859500701793,109.30282021619));
#210724=CARTESIAN_POINT('Ctrl Pts',(3.09910619832125,6.01563211736945,108.651395695404));
#210725=CARTESIAN_POINT('Ctrl Pts',(2.93375330764814,6.10081787314659,108.660145143307));
#210726=CARTESIAN_POINT('Ctrl Pts',(2.76488627843055,6.17918207037046,108.668894591209));
#210727=CARTESIAN_POINT('Ctrl Pts',(2.59307866646684,6.25045854554005,108.677644039111));
#210728=CARTESIAN_POINT('Ctrl Pts',(2.42127244185362,6.32173444515042,108.686393416362));
#210729=CARTESIAN_POINT('Ctrl Pts',(2.24652594672454,6.38592262741842,108.695142793612));
#210730=CARTESIAN_POINT('Ctrl Pts',(2.06943269687114,6.44280508110564,108.703892170862));
#210731=CARTESIAN_POINT('Ctrl Pts',(1.89234081822056,6.49968709436173,108.712641480367));
#210732=CARTESIAN_POINT('Ctrl Pts',(1.71290249405552,6.54926340459555,108.721390789873));
#210733=CARTESIAN_POINT('Ctrl Pts',(1.53172716625007,6.59136563150396,108.730140099378));
#210734=CARTESIAN_POINT('Ctrl Pts',(1.35055318107284,6.6334675464072,108.738889344045));
#210735=CARTESIAN_POINT('Ctrl Pts',(1.16764249714371,6.66809542395784,108.747638588713));
#210736=CARTESIAN_POINT('Ctrl Pts',(0.983616340613883,6.69513165624675,
108.75638783338));
#210737=CARTESIAN_POINT('Ctrl Pts',(0.799591486713338,6.72216769715967,
108.765137016116));
#210738=CARTESIAN_POINT('Ctrl Pts',(0.614451459526177,6.74161215869376,
108.773886198851));
#210739=CARTESIAN_POINT('Ctrl Pts',(0.428825047909717,6.75339900185716,
108.782635381587));
#210740=CARTESIAN_POINT('Ctrl Pts',(0.243199888596486,6.76518576550223,
108.791384505298));
#210741=CARTESIAN_POINT('Ctrl Pts',(0.0570886373913634,6.76931499599835,
108.800133629008));
#210742=CARTESIAN_POINT('Ctrl Pts',(-0.128876626811696,6.76577266947846,
108.808882752719));
#210743=CARTESIAN_POINT('Ctrl Pts',(-0.314840698188805,6.7622303656799,
108.81763182031));
#210744=CARTESIAN_POINT('Ctrl Pts',(-0.500658497951997,6.75101660879218,
108.826380887902));
#210745=CARTESIAN_POINT('Ctrl Pts',(-0.685698951927058,6.7321694829621,
108.835129955493));
#210746=CARTESIAN_POINT('Ctrl Pts',(-0.870738280460756,6.71332247176282,
108.843878969872));
#210747=CARTESIAN_POINT('Ctrl Pts',(-1.05499998761347,6.68684221356171,
108.85262798425));
#210748=CARTESIAN_POINT('Ctrl Pts',(-1.23785829161522,6.65281863948503,
108.861376998629));
#210749=CARTESIAN_POINT('Ctrl Pts',(-1.43007412917492,6.61705395368842,
108.870573732328));
#210750=CARTESIAN_POINT('Ctrl Pts',(-1.62073882535866,6.57295372727771,
108.879770466027));
#210751=CARTESIAN_POINT('Ctrl Pts',(-1.80913696091575,6.52068343478263,
108.888967199726));
#210752=CARTESIAN_POINT('Ctrl Pts',(-1.98838356186176,6.47095219815179,
108.89771719744));
#210753=CARTESIAN_POINT('Ctrl Pts',(-2.16557827572599,6.41382586850869,
108.906467195154));
#210754=CARTESIAN_POINT('Ctrl Pts',(-2.34011918621768,6.34949849943253,
108.915217192867));
#210755=CARTESIAN_POINT('Ctrl Pts',(-2.51465655691162,6.28517243495525,
108.923967013126));
#210756=CARTESIAN_POINT('Ctrl Pts',(-2.68653996295387,6.21364572242349,
108.932716833384));
#210757=CARTESIAN_POINT('Ctrl Pts',(-2.85518555380043,6.13516132252196,
108.941466653642));
#210758=CARTESIAN_POINT('Ctrl Pts',(-3.02382794858735,6.05667841000483,
108.95021630808));
#210759=CARTESIAN_POINT('Ctrl Pts',(-3.1892323910932,5.9712381949206,108.958965962517));
#210760=CARTESIAN_POINT('Ctrl Pts',(-3.35083705967729,5.87913088810695,
108.967715616955));
#210761=CARTESIAN_POINT('Ctrl Pts',(-3.51243888042428,5.78702520443086,
108.976465117204));
#210762=CARTESIAN_POINT('Ctrl Pts',(-3.67024081223716,5.68825280605766,
108.985214617453));
#210763=CARTESIAN_POINT('Ctrl Pts',(-3.82370687544425,5.58314917682488,
108.993964117702));
#210764=CARTESIAN_POINT('Ctrl Pts',(-3.97717043817848,5.47804726007998,
109.002713475392));
#210765=CARTESIAN_POINT('Ctrl Pts',(-4.12629803722502,5.36661448084204,
109.011462833083));
#210766=CARTESIAN_POINT('Ctrl Pts',(-4.27058317206957,5.24922931204536,
109.020212190773));
#210767=CARTESIAN_POINT('Ctrl Pts',(-4.4148661477487,5.1318458998676,109.028961417533));
#210768=CARTESIAN_POINT('Ctrl Pts',(-4.55430658194434,5.00851045723015,
109.037710644293));
#210769=CARTESIAN_POINT('Ctrl Pts',(-4.68843089001853,4.87964187103112,
109.046459871053));
#210770=CARTESIAN_POINT('Ctrl Pts',(-4.82255336917844,4.75077504207952,
109.055208978509));
#210771=CARTESIAN_POINT('Ctrl Pts',(-4.95135966065142,4.61637541908085,
109.063958085965));
#210772=CARTESIAN_POINT('Ctrl Pts',(-5.07441230869252,4.47689945401836,
109.072707193421));
#210773=CARTESIAN_POINT('Ctrl Pts',(-5.19746344226424,4.33742520555507,
109.081456193197));
#210774=CARTESIAN_POINT('Ctrl Pts',(-5.31476088454774,4.19287495491329,
109.090205192974));
#210775=CARTESIAN_POINT('Ctrl Pts',(-5.42590627628859,4.04373961586698,
109.09895419275));
#210776=CARTESIAN_POINT('Ctrl Pts',(-5.53706380672676,3.89458798906722,
109.107704148045));
#210777=CARTESIAN_POINT('Ctrl Pts',(-5.64206777071875,3.74085050155267,
109.11645410334));
#210778=CARTESIAN_POINT('Ctrl Pts',(-5.74056148164021,3.58304938223139,
109.125204058634));
#210779=CARTESIAN_POINT('Ctrl Pts',(-5.83905138951902,3.42525435593252,
109.133953676075));
#210780=CARTESIAN_POINT('Ctrl Pts',(-5.93103139557674,3.26339625497144,
109.142703293517));
#210781=CARTESIAN_POINT('Ctrl Pts',(-6.01618907820871,3.09802485064956,
109.151452910958));
#210782=CARTESIAN_POINT('Ctrl Pts',(-6.10134392545009,2.93265895249588,
109.160202237074));
#210783=CARTESIAN_POINT('Ctrl Pts',(-6.17967677261857,2.76378023985979,
109.168951563189));
#210784=CARTESIAN_POINT('Ctrl Pts',(-6.25092157009249,2.59196229227056,
109.177700889305));
#210785=CARTESIAN_POINT('Ctrl Pts',(-6.3221643740777,2.42014915229047,109.186449970608));
#210786=CARTESIAN_POINT('Ctrl Pts',(-6.38631941548931,2.24539720662823,
109.19519905191));
#210787=CARTESIAN_POINT('Ctrl Pts',(-6.44316881037541,2.06829994947675,
109.203948133213));
#210788=CARTESIAN_POINT('Ctrl Pts',(-6.50002334524578,1.89118668024429,
109.212698005555));
#210789=CARTESIAN_POINT('Ctrl Pts',(-6.54957082411104,1.71172794807672,
109.221447877897));
#210790=CARTESIAN_POINT('Ctrl Pts',(-6.59164294296093,1.530533342503,109.23019775024));
#210791=CARTESIAN_POINT('Ctrl Pts',(-6.63371214082146,1.34935131693542,
109.238947015095));
#210792=CARTESIAN_POINT('Ctrl Pts',(-6.66830695239703,1.16643393829689,
109.247696279949));
#210793=CARTESIAN_POINT('Ctrl Pts',(-6.69530988154002,0.982402458340078,
109.256445544804));
#210794=CARTESIAN_POINT('Ctrl Pts',(-6.72231419690494,0.798361530946127,
109.265195258811));
#210795=CARTESIAN_POINT('Ctrl Pts',(-6.74172580829287,0.613206671361529,
109.273944972818));
#210796=CARTESIAN_POINT('Ctrl Pts',(-6.75347878028186,0.427566795112433,
109.282694686825));
#210797=CARTESIAN_POINT('Ctrl Pts',(-6.7624899236821,0.285234494205859,
109.289403196614));
#210798=CARTESIAN_POINT('Ctrl Pts',(-6.76699999999989,0.142617266094271,
109.296111706402));
#210799=CARTESIAN_POINT('Ctrl Pts',(-6.767,5.13485784531581E-12,109.30282021619));
#210800=CARTESIAN_POINT('Ctrl Pts',(-6.76410475442949,-0.00322222550308449,
109.30282021619));
#210801=CARTESIAN_POINT('Ctrl Pts',(-6.76710928112432,-0.786032822436749,
109.339508609526));
#210802=CARTESIAN_POINT('Ctrl Pts',(-6.2656633635301,-3.8265755522471,109.482166580078));
#210803=CARTESIAN_POINT('Ctrl Pts',(-2.76332679390342,-6.93290299659207,
109.677809339238));
#210804=CARTESIAN_POINT('Ctrl Pts',(1.90804949459011,-6.7813526609264,109.889748493671));
#210805=CARTESIAN_POINT('Ctrl Pts',(4.92590585172162,-5.05725987228767,
110.048702859496));
#210806=CARTESIAN_POINT('Ctrl Pts',(6.73094077380569,-2.07889163802113,
110.207657225321));
#210807=CARTESIAN_POINT('Ctrl Pts',(6.98677885739346,2.33141846444617,110.408528190629));
#210808=CARTESIAN_POINT('Ctrl Pts',(4.880745451628,5.09104750816176,110.556414367328));
#210809=CARTESIAN_POINT('Ctrl Pts',(3.10339103771845,6.02380226238954,110.651315755419));
#210810=CARTESIAN_POINT('Origin',(0.,0.,4.30282021618968));
#210811=CARTESIAN_POINT('',(3.09910619832131,6.01563211736942,113.045755263024));
#210812=CARTESIAN_POINT('',(3.09910619832117,6.01563211736949,112.651476300929));
#210813=CARTESIAN_POINT('',(3.09910619832133,6.0156321173694,4.30282021618968));
#210814=CARTESIAN_POINT('',(-6.767,5.13019531370174E-12,111.69717978381));
#210815=CARTESIAN_POINT('Ctrl Pts',(-6.767,5.13019525665479E-12,111.69717978381));
#210816=CARTESIAN_POINT('Ctrl Pts',(-6.76700000000014,-0.186007249521703,
111.705929295621));
#210817=CARTESIAN_POINT('Ctrl Pts',(-6.75932637294549,-0.372014355744713,
111.714678807432));
#210818=CARTESIAN_POINT('Ctrl Pts',(-6.74400518264224,-0.557389537482261,
111.723428319244));
#210819=CARTESIAN_POINT('Ctrl Pts',(-6.72868405705143,-0.742763936246609,
111.732177794099));
#210820=CARTESIAN_POINT('Ctrl Pts',(-6.70571545645796,-0.927506130237137,
111.740927268955));
#210821=CARTESIAN_POINT('Ctrl Pts',(-6.67517739404886,-1.11098863989653,
111.749676743811));
#210822=CARTESIAN_POINT('Ctrl Pts',(-6.64463945808768,-1.29447038981606,
111.758426182438));
#210823=CARTESIAN_POINT('Ctrl Pts',(-6.60653217008427,-1.47669218313364,
111.767175621065));
#210824=CARTESIAN_POINT('Ctrl Pts',(-6.56098496092752,-1.65703510598988,
111.775925059692));
#210825=CARTESIAN_POINT('Ctrl Pts',(-6.51543793658381,-1.83737729708399,
111.784674462817));
#210826=CARTESIAN_POINT('Ctrl Pts',(-6.46245112167515,-2.01584035510623,
111.793423865942));
#210827=CARTESIAN_POINT('Ctrl Pts',(-6.40220448374358,-2.19181813760486,
111.802173269067));
#210828=CARTESIAN_POINT('Ctrl Pts',(-6.34195808526619,-2.36779522066834,
111.810922637417));
#210829=CARTESIAN_POINT('Ctrl Pts',(-6.2744520143323,-2.54128677683853,
111.819672005767));
#210830=CARTESIAN_POINT('Ctrl Pts',(-6.1999155507204,-2.71170355384496,
111.828421374117));
#210831=CARTESIAN_POINT('Ctrl Pts',(-6.1253793771684,-2.88211966767162,
111.837170708419));
#210832=CARTESIAN_POINT('Ctrl Pts',(-6.04381298052679,-3.04946076371471,
111.845920042721));
#210833=CARTESIAN_POINT('Ctrl Pts',(-5.95549339336001,-3.21315848374233,
111.854669377023));
#210834=CARTESIAN_POINT('Ctrl Pts',(-5.86717414255591,-3.37685558033177,
111.863418678003));
#210835=CARTESIAN_POINT('Ctrl Pts',(-5.77210188876792,-3.53690907646439,
111.872167978983));
#210836=CARTESIAN_POINT('Ctrl Pts',(-5.67059953347203,-3.69277536968969,
111.880917279963));
#210837=CARTESIAN_POINT('Ctrl Pts',(-5.56909755631601,-3.84864108224608,
111.889666548349));
#210838=CARTESIAN_POINT('Ctrl Pts',(-5.46116568197078,-4.00031938297205,
111.898415816734));
#210839=CARTESIAN_POINT('Ctrl Pts',(-5.34717048533842,-4.14729511859546,
111.907165085119));
#210840=CARTESIAN_POINT('Ctrl Pts',(-5.23317570392075,-4.29427031887627,
111.915914321636));
#210841=CARTESIAN_POINT('Ctrl Pts',(-5.1131178200375,-4.43654276189275,
111.924663558153));
#210842=CARTESIAN_POINT('Ctrl Pts',(-4.98740458984986,-4.57362924351598,
111.93341279467));
#210843=CARTESIAN_POINT('Ctrl Pts',(-4.86169180711989,-4.71071523720012,
111.942162000046));
#210844=CARTESIAN_POINT('Ctrl Pts',(-4.73032391204432,-4.84261509522984,
111.950911205421));
#210845=CARTESIAN_POINT('Ctrl Pts',(-4.59374707013873,-4.96888084538077,
111.959660410797));
#210846=CARTESIAN_POINT('Ctrl Pts',(-4.45717070301713,-5.0951461565923,
111.968409585757));
#210847=CARTESIAN_POINT('Ctrl Pts',(-4.31538563571302,-5.21577720459312,
111.977158760717));
#210848=CARTESIAN_POINT('Ctrl Pts',(-4.16887341029762,-5.33036429232688,
111.985907935678));
#210849=CARTESIAN_POINT('Ctrl Pts',(-4.02236168203969,-5.44495099123422,
111.99465708095));
#210850=CARTESIAN_POINT('Ctrl Pts',(-3.87112305348437,-5.55349359438412,
112.003406226222));
#210851=CARTESIAN_POINT('Ctrl Pts',(-3.71567117018042,-5.65562346298709,
112.012155371494));
#210852=CARTESIAN_POINT('Ctrl Pts',(-3.56021980146096,-5.75775299351473,
112.020904487804));
#210853=CARTESIAN_POINT('Ctrl Pts',(-3.40055544538622,-5.85346967463715,
112.029653604114));
#210854=CARTESIAN_POINT('Ctrl Pts',(-3.2372203598712,-5.94244842986756,
112.038402720425));
#210855=CARTESIAN_POINT('Ctrl Pts',(-3.0738858014747,-6.0314268979438,112.047151808499));
#210856=CARTESIAN_POINT('Ctrl Pts',(-2.90688078896892,-6.11366734656631,
112.055900896574));
#210857=CARTESIAN_POINT('Ctrl Pts',(-2.73677250721709,-6.18889046952204,
112.064649984649));
#210858=CARTESIAN_POINT('Ctrl Pts',(-2.56666476031853,-6.26411335596174,
112.073399045215));
#210859=CARTESIAN_POINT('Ctrl Pts',(-2.39345402575568,-6.33231884500403,
112.082148105781));
#210860=CARTESIAN_POINT('Ctrl Pts',(-2.21772856066027,-6.39327529762576,
112.090897166347));
#210861=CARTESIAN_POINT('Ctrl Pts',(-2.04200363348964,-6.45423156364968,
112.099646200131));
#210862=CARTESIAN_POINT('Ctrl Pts',(-1.86376426189743,-6.50793874375525,
112.108395233914));
#210863=CARTESIAN_POINT('Ctrl Pts',(-1.68361577753633,-6.55421443909419,
112.117144267698));
#210864=CARTESIAN_POINT('Ctrl Pts',(-1.5034678296826,-6.60048999661764,
112.125893275426));
#210865=CARTESIAN_POINT('Ctrl Pts',(-1.32141105795429,-6.63933404237625,
112.134642283154));
#210866=CARTESIAN_POINT('Ctrl Pts',(-1.13806375487444,-6.67061465607489,
112.143391290882));
#210867=CARTESIAN_POINT('Ctrl Pts',(-0.954716982607419,-6.70189517921233,
112.15214027328));
#210868=CARTESIAN_POINT('Ctrl Pts',(-0.770079968906719,-6.72561226592175,
112.160889255678));
#210869=CARTESIAN_POINT('Ctrl Pts',(-0.584779765563001,-6.74168536983061,
112.169638238077));
#210870=CARTESIAN_POINT('Ctrl Pts',(-0.391489830656095,-6.75845151013825,
112.178764457087));
#210871=CARTESIAN_POINT('Ctrl Pts',(-0.197478578243166,-6.76689983031611,
112.187890676097));
#210872=CARTESIAN_POINT('Ctrl Pts',(-0.00346287645620368,-6.76699911397117,
112.197016895106));
#210873=CARTESIAN_POINT('Ctrl Pts',(0.184489834650012,-6.76709529501202,
112.205857919772));
#210874=CARTESIAN_POINT('Ctrl Pts',(0.37244640424559,-6.75935639738189,
112.214698944438));
#210875=CARTESIAN_POINT('Ctrl Pts',(0.559755019484654,-6.74380925873217,
112.223539969104));
#210876=CARTESIAN_POINT('Ctrl Pts',(0.745134705518054,-6.72842222659847,
112.232289947714));
#210877=CARTESIAN_POINT('Ctrl Pts',(0.929879431224811,-6.70538706057576,
112.241039926323));
#210878=CARTESIAN_POINT('Ctrl Pts',(1.11336163626447,-6.6747820089419,112.249789904933));
#210879=CARTESIAN_POINT('Ctrl Pts',(1.29684196300358,-6.64417727061084,
112.25853979397));
#210880=CARTESIAN_POINT('Ctrl Pts',(1.47905951217168,-6.60600284890667,
112.267289683006));
#210881=CARTESIAN_POINT('Ctrl Pts',(1.6593953206676,-6.56038841607313,112.276039572043));
#210882=CARTESIAN_POINT('Ctrl Pts',(1.83972934300479,-6.51477443503348,
112.284789374415));
#210883=CARTESIAN_POINT('Ctrl Pts',(2.01818138405944,-6.46172066062241,
112.293539176787));
#210884=CARTESIAN_POINT('Ctrl Pts',(2.19414528353881,-6.40140730423588,
112.302288979159));
#210885=CARTESIAN_POINT('Ctrl Pts',(2.37010749863671,-6.34109452518765,
112.311038697776));
#210886=CARTESIAN_POINT('Ctrl Pts',(2.54358134866121,-6.27352239616641,
112.319788416392));
#210887=CARTESIAN_POINT('Ctrl Pts',(2.71397759435208,-6.19892043966971,
112.328538135008));
#210888=CARTESIAN_POINT('Ctrl Pts',(2.88437226557786,-6.12431917249674,
112.337287772777));
#210889=CARTESIAN_POINT('Ctrl Pts',(3.05168912680628,-6.04268832278964,
112.346037410546));
#210890=CARTESIAN_POINT('Ctrl Pts',(3.21535986273536,-5.95430516123506,
112.354787048314));
#210891=CARTESIAN_POINT('Ctrl Pts',(3.37902914072545,-5.86592278697612,
112.363536608143));
#210892=CARTESIAN_POINT('Ctrl Pts',(3.53905210621295,-5.77078835742112,
112.372286167972));
#210893=CARTESIAN_POINT('Ctrl Pts',(3.6948852283144,-5.66922500431797,112.381035727801));
#210894=CARTESIAN_POINT('Ctrl Pts',(3.85071701406703,-5.56766252217258,
112.389785212599));
#210895=CARTESIAN_POINT('Ctrl Pts',(4.00235878822186,-5.45967138329531,
112.398534697396));
#210896=CARTESIAN_POINT('Ctrl Pts',(4.14929549611125,-5.34561838199762,
112.407284182193));
#210897=CARTESIAN_POINT('Ctrl Pts',(4.29623099275899,-5.23156632087172,
112.416033594865));
#210898=CARTESIAN_POINT('Ctrl Pts',(4.43846127435846,-5.11145267305122,
112.424783007538));
#210899=CARTESIAN_POINT('Ctrl Pts',(4.5755032605427,-4.98568540050043,112.433532420211));
#210900=CARTESIAN_POINT('Ctrl Pts',(4.71254416257609,-4.85991912290527,
112.442281763666));
#210901=CARTESIAN_POINT('Ctrl Pts',(4.84439664018591,-4.72849950385593,
112.451031107121));
#210902=CARTESIAN_POINT('Ctrl Pts',(4.97061286794577,-4.5918728986125,112.459780450576));
#210903=CARTESIAN_POINT('Ctrl Pts',(5.09682813912523,-4.45524732884869,
112.468529727721));
#210904=CARTESIAN_POINT('Ctrl Pts',(5.21740705147685,-4.31341506235974,
112.477279004866));
#210905=CARTESIAN_POINT('Ctrl Pts',(5.33194007545549,-4.16685781275912,
112.486028282011));
#210906=CARTESIAN_POINT('Ctrl Pts',(5.44647226944338,-4.02030162522041,
112.494777495752));
#210907=CARTESIAN_POINT('Ctrl Pts',(5.55495848627966,-3.86902074888145,
112.503526709493));
#210908=CARTESIAN_POINT('Ctrl Pts',(5.65703027291642,-3.71352898080885,
112.512275923234));
#210909=CARTESIAN_POINT('Ctrl Pts',(5.75910135376856,-3.55803828789817,
112.521025076478));
#210910=CARTESIAN_POINT('Ctrl Pts',(5.85475793592616,-3.39833700106948,
112.529774229722));
#210911=CARTESIAN_POINT('Ctrl Pts',(5.94367514427267,-3.23496750823795,
112.538523382966));
#210912=CARTESIAN_POINT('Ctrl Pts',(6.03259176732513,-3.07159909077973,
112.547272478619));
#210913=CARTESIAN_POINT('Ctrl Pts',(6.11476896835803,-2.90456276731689,
112.556021574272));
#210914=CARTESIAN_POINT('Ctrl Pts',(6.1899276554777,-2.73442583003312,112.564770669925));
#210915=CARTESIAN_POINT('Ctrl Pts',(6.26508587282948,-2.56428995616429,
112.573519710893));
#210916=CARTESIAN_POINT('Ctrl Pts',(6.33322554827064,-2.39105376935457,
112.582268751861));
#210917=CARTESIAN_POINT('Ctrl Pts',(6.39411526732943,-2.21530561054331,
112.591017792829));
#210918=CARTESIAN_POINT('Ctrl Pts',(6.45500462602756,-2.03955849185385,
112.599766782018));
#210919=CARTESIAN_POINT('Ctrl Pts',(6.50864402040647,-1.86129970164867,
112.608515771207));
#210920=CARTESIAN_POINT('Ctrl Pts',(6.55485128368509,-1.68113463136417,
112.617264760396));
#210921=CARTESIAN_POINT('Ctrl Pts',(6.60199809554242,-1.49730620117239,
112.626191645867));
#210922=CARTESIAN_POINT('Ctrl Pts',(6.64140720707798,-1.3114934324608,112.635118531339));
#210923=CARTESIAN_POINT('Ctrl Pts',(6.67293928722817,-1.12435326697919,
112.64404541681));
#210924=CARTESIAN_POINT('Ctrl Pts',(6.70384625876201,-0.940923067010568,
112.652795330988));
#210925=CARTESIAN_POINT('Ctrl Pts',(6.72718554579751,-0.756217899525683,
112.661545245165));
#210926=CARTESIAN_POINT('Ctrl Pts',(6.74287786815293,-0.570865181258552,
112.670295159342));
#210927=CARTESIAN_POINT('Ctrl Pts',(6.75856988190823,-0.385516108077956,
112.679044901447));
#210928=CARTESIAN_POINT('Ctrl Pts',(6.76661520773391,-0.199519795230309,
112.687794643551));
#210929=CARTESIAN_POINT('Ctrl Pts',(6.76698651789578,-0.0135080204595548,
112.696544385656));
#210930=CARTESIAN_POINT('Ctrl Pts',(6.76735782124913,0.17250034350898,112.705293967321));
#210931=CARTESIAN_POINT('Ctrl Pts',(6.76005538995205,0.358523882206871,
112.714043548986));
#210932=CARTESIAN_POINT('Ctrl Pts',(6.74510402742394,0.543930748560262,
112.722793130651));
#210933=CARTESIAN_POINT('Ctrl Pts',(6.73015291918076,0.729334461610996,
112.731542563507));
#210934=CARTESIAN_POINT('Ctrl Pts',(6.70755316306654,0.914121237630324,
112.740291996364));
#210935=CARTESIAN_POINT('Ctrl Pts',(6.67738151874648,1.09766345165675,112.749041429221));
#210936=CARTESIAN_POINT('Ctrl Pts',(6.64721034747655,1.28120278799219,112.757790724898));
#210937=CARTESIAN_POINT('Ctrl Pts',(6.6094675720524,1.46349731859886,112.766540020576));
#210938=CARTESIAN_POINT('Ctrl Pts',(6.56428138111633,1.64392790277722,112.775289316253));
#210939=CARTESIAN_POINT('Ctrl Pts',(6.51909583859973,1.82435589778615,112.784038486379));
#210940=CARTESIAN_POINT('Ctrl Pts',(6.46646716393012,2.00291972191823,112.792787656505));
#210941=CARTESIAN_POINT('Ctrl Pts',(6.40657409873034,2.17901292274222,112.80153682663));
#210942=CARTESIAN_POINT('Ctrl Pts',(6.34668181342244,2.35510383058525,112.810285882829));
#210943=CARTESIAN_POINT('Ctrl Pts',(6.27952541914236,2.52872390822118,112.819034939028));
#210944=CARTESIAN_POINT('Ctrl Pts',(6.20533299175721,2.69928350889815,112.827783995228));
#210945=CARTESIAN_POINT('Ctrl Pts',(6.12831602991758,2.8763363796518,112.836866131386));
#210946=CARTESIAN_POINT('Ctrl Pts',(6.04371690605481,3.05009086601045,112.845948267544));
#210947=CARTESIAN_POINT('Ctrl Pts',(5.95184520316843,3.21991112882343,112.855030403702));
#210948=CARTESIAN_POINT('Ctrl Pts',(5.86333549509495,3.38351691182634,112.863780184046));
#210949=CARTESIAN_POINT('Ctrl Pts',(5.76807618099598,3.5434710371163,112.872529964389));
#210950=CARTESIAN_POINT('Ctrl Pts',(5.66639083309254,3.6992301802733,112.881279744733));
#210951=CARTESIAN_POINT('Ctrl Pts',(5.56470914082445,3.85498372381696,112.890029210518));
#210952=CARTESIAN_POINT('Ctrl Pts',(5.45660203372318,4.00654234701656,112.898778676303));
#210953=CARTESIAN_POINT('Ctrl Pts',(5.34243669839474,4.15339127986338,112.907528142088));
#210954=CARTESIAN_POINT('Ctrl Pts',(5.22827486050852,4.30023571400963,112.916277339834));
#210955=CARTESIAN_POINT('Ctrl Pts',(5.10805534167375,4.44237052028167,112.92502653758));
#210956=CARTESIAN_POINT('Ctrl Pts',(4.98218644340217,4.57931296628432,112.933775735326));
#210957=CARTESIAN_POINT('Ctrl Pts',(4.85632073219849,4.71625194483091,112.942524711537));
#210958=CARTESIAN_POINT('Ctrl Pts',(4.72480612170577,4.84799861524257,112.951273687749));
#210959=CARTESIAN_POINT('Ctrl Pts',(4.58808925235564,4.97410554898252,112.960022663961));
#210960=CARTESIAN_POINT('Ctrl Pts',(4.45136349474301,5.10022068120986,112.968772208962));
#210961=CARTESIAN_POINT('Ctrl Pts',(4.30943501210333,5.22069514871626,112.977521753964));
#210962=CARTESIAN_POINT('Ctrl Pts',(4.16278587432033,5.33511975166061,112.986271298966));
#210963=CARTESIAN_POINT('Ctrl Pts',(4.016145357407,5.44953762807657,112.995020329619));
#210964=CARTESIAN_POINT('Ctrl Pts',(3.86478496658175,5.55790617532609,113.003769360273));
#210965=CARTESIAN_POINT('Ctrl Pts',(3.70921874747447,5.65985735539191,113.012518390927));
#210966=CARTESIAN_POINT('Ctrl Pts',(3.55365041606161,5.76180991976885,113.021267540376));
#210967=CARTESIAN_POINT('Ctrl Pts',(3.39387638174793,5.85734478552657,113.030016689826));
#210968=CARTESIAN_POINT('Ctrl Pts',(3.23043927904818,5.9461374912108,113.038765839276));
#210969=CARTESIAN_POINT('Ctrl Pts',(3.18691767070615,5.9697820694405,113.041095647192));
#210970=CARTESIAN_POINT('Ctrl Pts',(3.1431364591972,5.9929488063338,113.043425455108));
#210971=CARTESIAN_POINT('Ctrl Pts',(3.09910619832131,6.01563211736942,113.045755263024));
#210972=CARTESIAN_POINT('Ctrl Pts',(3.09910619832136,6.01563211736939,111.045833125094));
#210973=CARTESIAN_POINT('Ctrl Pts',(2.93996722179409,6.09761661690788,111.054263314215));
#210974=CARTESIAN_POINT('Ctrl Pts',(2.77749027747824,6.17332502379726,111.062693503336));
#210975=CARTESIAN_POINT('Ctrl Pts',(2.61219945089555,6.24249173237266,111.071123692456));
#210976=CARTESIAN_POINT('Ctrl Pts',(2.44699166283165,6.31162369309696,111.079549646433));
#210977=CARTESIAN_POINT('Ctrl Pts',(2.27897311824067,6.37422037982185,111.08797560041));
#210978=CARTESIAN_POINT('Ctrl Pts',(2.10868962993586,6.43006353348091,111.096401554387));
#210979=CARTESIAN_POINT('Ctrl Pts',(1.93845430658069,6.48589089181705,111.10482512507));
#210980=CARTESIAN_POINT('Ctrl Pts',(1.76595563272836,6.53496841996684,111.113248695752));
#210981=CARTESIAN_POINT('Ctrl Pts',(1.59175688308495,6.57712695826618,111.121672266435));
#210982=CARTESIAN_POINT('Ctrl Pts',(1.41758542984143,6.61927889045427,111.13009451717));
#210983=CARTESIAN_POINT('Ctrl Pts',(1.24171475585187,6.65451391558974,111.138516767906));
#210984=CARTESIAN_POINT('Ctrl Pts',(1.06472103315279,6.68271338017441,111.146939018641));
#210985=CARTESIAN_POINT('Ctrl Pts',(0.887730337138724,6.71091236253352,
111.155361125352));
#210986=CARTESIAN_POINT('Ctrl Pts',(0.709616960052614,6.73207597198672,
111.163783232063));
#210987=CARTESIAN_POINT('Ctrl Pts',(0.530965317924063,6.74613703026864,
111.172205338773));
#210988=CARTESIAN_POINT('Ctrl Pts',(0.352291791994926,6.76019981094948,
111.180628477143));
#210989=CARTESIAN_POINT('Ctrl Pts',(0.173080202039716,6.76715828029015,
111.189051615514));
#210990=CARTESIAN_POINT('Ctrl Pts',(-0.0060815151668908,6.7669972672651,
111.197474753884));
#210991=CARTESIAN_POINT('Ctrl Pts',(-0.185361193648259,6.76683614822799,
111.205903438105));
#210992=CARTESIAN_POINT('Ctrl Pts',(-0.364590599861592,6.75954617843287,
111.214332122326));
#210993=CARTESIAN_POINT('Ctrl Pts',(-0.543182331353419,6.74516433861366,
111.222760806547));
#210994=CARTESIAN_POINT('Ctrl Pts',(-0.721830655650253,6.73077794142413,
111.231192161681));
#210995=CARTESIAN_POINT('Ctrl Pts',(-0.899840570268462,6.70929522590876,
111.239623516814));
#210996=CARTESIAN_POINT('Ctrl Pts',(-1.07663080166935,6.68080497521794,
111.248054871948));
#210997=CARTESIAN_POINT('Ctrl Pts',(-1.25359503468112,6.65228668367059,
111.256494525444));
#210998=CARTESIAN_POINT('Ctrl Pts',(-1.42933685649182,6.61674713144458,
111.264934178939));
#210999=CARTESIAN_POINT('Ctrl Pts',(-1.60328490953062,6.57432631521066,
111.273373832435));
#211000=CARTESIAN_POINT('Ctrl Pts',(-1.75644180277676,6.53697585161046,
111.280804735437));
#211001=CARTESIAN_POINT('Ctrl Pts',(-1.90820813575328,6.4942915777034,111.288235638438));
#211002=CARTESIAN_POINT('Ctrl Pts',(-2.05820434700911,6.44640084589477,
111.29566654144));
#211003=CARTESIAN_POINT('Ctrl Pts',(-2.22250825668757,6.39394195771593,
111.303806256473));
#211004=CARTESIAN_POINT('Ctrl Pts',(-2.38501544551448,6.33513026296877,
111.311945971506));
#211005=CARTESIAN_POINT('Ctrl Pts',(-2.54519477728016,6.27010945245024,
111.320085686539));
#211006=CARTESIAN_POINT('Ctrl Pts',(-2.70523401716352,6.20514550874239,
111.328218282626));
#211007=CARTESIAN_POINT('Ctrl Pts',(-2.86294911549623,6.13398339534557,
111.336350878713));
#211008=CARTESIAN_POINT('Ctrl Pts',(-3.01782396863838,6.05681661389147,
111.3444834748));
#211009=CARTESIAN_POINT('Ctrl Pts',(-3.1725929410222,5.97970258778901,111.352610511008));
#211010=CARTESIAN_POINT('Ctrl Pts',(-3.3245252076969,5.8965922293451,111.360737547216));
#211011=CARTESIAN_POINT('Ctrl Pts',(-3.47312458013503,5.80772715017345,
111.368864583424));
#211012=CARTESIAN_POINT('Ctrl Pts',(-3.62165291938359,5.71890455011804,
111.376987734761));
#211013=CARTESIAN_POINT('Ctrl Pts',(-3.7668512233192,5.62433289475613,111.385110886099));
#211014=CARTESIAN_POINT('Ctrl Pts',(-3.90824788262623,5.52429972828662,
111.393234037436));
#211015=CARTESIAN_POINT('Ctrl Pts',(-4.04960480842116,5.42429467188032,
111.401354906108));
#211016=CARTESIAN_POINT('Ctrl Pts',(-4.18716191917053,5.31883137320026,
111.40947577478));
#211017=CARTESIAN_POINT('Ctrl Pts',(-4.32047661703014,5.20824066280504,
111.417596643451));
#211018=CARTESIAN_POINT('Ctrl Pts',(-4.45379851972622,5.09764397566459,
111.425717951006));
#211019=CARTESIAN_POINT('Ctrl Pts',(-4.58287726707774,4.98191955396713,
111.43383925856));
#211020=CARTESIAN_POINT('Ctrl Pts',(-4.70730324607933,4.86143858846855,
111.441960566115));
#211021=CARTESIAN_POINT('Ctrl Pts',(-4.77195931004163,4.79883249065824,
111.446180679832));
#211022=CARTESIAN_POINT('Ctrl Pts',(-4.83535960185525,4.73494267065707,
111.450400793548));
#211023=CARTESIAN_POINT('Ctrl Pts',(-4.89745054546376,4.66982517389428,
111.454620907265));
#211024=CARTESIAN_POINT('Ctrl Pts',(-5.02963946341902,4.53119285593014,
111.463605345791));
#211025=CARTESIAN_POINT('Ctrl Pts',(-5.15582619695452,4.38706291435779,
111.472589784317));
#211026=CARTESIAN_POINT('Ctrl Pts',(-5.27559894187177,4.23796470071679,
111.481574222843));
#211027=CARTESIAN_POINT('Ctrl Pts',(-5.3955784073981,4.08860915245797,111.490574167973));
#211028=CARTESIAN_POINT('Ctrl Pts',(-5.50912160836431,3.9342683794576,111.499574113104));
#211029=CARTESIAN_POINT('Ctrl Pts',(-5.61585899953535,3.77550217816622,
111.508574058234));
#211030=CARTESIAN_POINT('Ctrl Pts',(-5.72284792010836,3.61636184024636,
111.517595211966));
#211031=CARTESIAN_POINT('Ctrl Pts',(-5.82299880745891,3.45277540714538,
111.526616365699));
#211032=CARTESIAN_POINT('Ctrl Pts',(-5.91598577023615,3.28533124149808,
111.535637519431));
#211033=CARTESIAN_POINT('Ctrl Pts',(-6.00906734798116,3.11771670009207,
111.544667852258));
#211034=CARTESIAN_POINT('Ctrl Pts',(-6.09497032815903,2.94623679604312,
111.553698185085));
#211035=CARTESIAN_POINT('Ctrl Pts',(-6.17341559597288,2.77150300007033,
111.562728517913));
#211036=CARTESIAN_POINT('Ctrl Pts',(-6.25197207444889,2.5965214866546,111.571771652905));
#211037=CARTESIAN_POINT('Ctrl Pts',(-6.32304960230133,2.41827707563771,
111.580814787898));
#211038=CARTESIAN_POINT('Ctrl Pts',(-6.38641700203635,2.2374018137342,111.589857922891));
#211039=CARTESIAN_POINT('Ctrl Pts',(-6.44181470839864,2.07927516361074,
111.59776370629));
#211040=CARTESIAN_POINT('Ctrl Pts',(-6.49132044455546,1.91913817615428,
111.60566948969));
#211041=CARTESIAN_POINT('Ctrl Pts',(-6.53481107523639,1.75742232003802,
111.61357527309));
#211042=CARTESIAN_POINT('Ctrl Pts',(-6.58497038076436,1.57090961813762,
111.622693296875));
#211043=CARTESIAN_POINT('Ctrl Pts',(-6.62716167707037,1.38216962683381,
111.631811320661));
#211044=CARTESIAN_POINT('Ctrl Pts',(-6.66121233591839,1.19186375723432,
111.640929344446));
#211045=CARTESIAN_POINT('Ctrl Pts',(-6.69622292896478,0.99619290738016,
111.650304417674));
#211046=CARTESIAN_POINT('Ctrl Pts',(-6.7226270800968,0.798866808204857,
111.659679490901));
#211047=CARTESIAN_POINT('Ctrl Pts',(-6.74029265815554,0.600619582110436,
111.669054564128));
#211048=CARTESIAN_POINT('Ctrl Pts',(-6.75795823621427,0.402372356016142,
111.678429637355));
#211049=CARTESIAN_POINT('Ctrl Pts',(-6.76688515647705,0.203204251837742,
111.687804710583));
#211050=CARTESIAN_POINT('Ctrl Pts',(-6.76699889844774,0.00386114065237677,
111.69717978381));
#211051=CARTESIAN_POINT('',(-6.77219403443551,-0.00312713327445556,111.302818667387));
#211052=CARTESIAN_POINT('Ctrl Pts',(3.10339103771845,6.02380226238954,110.651315755419));
#211053=CARTESIAN_POINT('Ctrl Pts',(2.89610118462354,6.13258787907032,110.662383944544));
#211054=CARTESIAN_POINT('Ctrl Pts',(0.642912696893712,7.1623602499167,110.779421710886));
#211055=CARTESIAN_POINT('Ctrl Pts',(-4.56900862909321,6.49795736804409,
110.996589297456));
#211056=CARTESIAN_POINT('Ctrl Pts',(-6.75983703898571,2.11762530079817,
111.202688694898));
#211057=CARTESIAN_POINT('Ctrl Pts',(-6.77270472585136,-0.00312414668946661,
111.302818515126));
#211058=CARTESIAN_POINT('Ctrl Pts',(-6.76699926334503,-0.00315751292227859,
111.30282021619));
#211059=CARTESIAN_POINT('Ctrl Pts',(-6.7669416052657,-0.126726977238388,
111.308659406158));
#211060=CARTESIAN_POINT('Ctrl Pts',(-6.76349934956323,-0.250225686892749,
111.314498596126));
#211061=CARTESIAN_POINT('Ctrl Pts',(-6.75668362546576,-0.373517583739894,
111.320337786094));
#211062=CARTESIAN_POINT('Ctrl Pts',(-6.74625325319796,-0.562196051842372,
111.329273729545));
#211063=CARTESIAN_POINT('Ctrl Pts',(-6.72790872944149,-0.750557567481397,
111.338209672996));
#211064=CARTESIAN_POINT('Ctrl Pts',(-6.70168187751392,-0.937949365691698,
111.347145616446));
#211065=CARTESIAN_POINT('Ctrl Pts',(-6.67549445150109,-1.12505946432645,
111.356068126804));
#211066=CARTESIAN_POINT('Ctrl Pts',(-6.64144837630606,-1.311202499104,111.364990637162));
#211067=CARTESIAN_POINT('Ctrl Pts',(-6.59962724468697,-1.49573033371176,
111.373913147519));
#211068=CARTESIAN_POINT('Ctrl Pts',(-6.55790858781864,-1.67980601786048,
111.382813794957));
#211069=CARTESIAN_POINT('Ctrl Pts',(-6.50845295450852,-1.86227414942701,
111.391714442396));
#211070=CARTESIAN_POINT('Ctrl Pts',(-6.45139484191311,-2.04249690176923,
111.400615089834));
#211071=CARTESIAN_POINT('Ctrl Pts',(-6.3944249055886,-2.22244114209082,
111.40950198242));
#211072=CARTESIAN_POINT('Ctrl Pts',(-6.32987600308755,-2.40014667990826,
111.418388875006));
#211073=CARTESIAN_POINT('Ctrl Pts',(-6.25793300836317,-2.57498805100892,
111.427275767593));
#211074=CARTESIAN_POINT('Ctrl Pts',(-6.18617493399066,-2.74938001451971,
111.436139817548));
#211075=CARTESIAN_POINT('Ctrl Pts',(-6.10706078966566,-2.92092226356557,
111.445003867503));
#211076=CARTESIAN_POINT('Ctrl Pts',(-6.02082408885677,-3.08900733101137,
111.453867917457));
#211077=CARTESIAN_POINT('Ctrl Pts',(-5.93837486561982,-3.24971017699978,
111.462342662278));
#211078=CARTESIAN_POINT('Ctrl Pts',(-5.8494153568189,-3.40725273941956,
111.470817407098));
#211079=CARTESIAN_POINT('Ctrl Pts',(-5.75419177662111,-3.56111864417153,
111.479292151919));
#211080=CARTESIAN_POINT('Ctrl Pts',(-5.66195510896502,-3.71015818134007,
111.487501066348));
#211081=CARTESIAN_POINT('Ctrl Pts',(-5.56392926635857,-3.85560391963464,
111.495709980777));
#211082=CARTESIAN_POINT('Ctrl Pts',(-5.46043493019616,-3.9969912900948,
111.503918895206));
#211083=CARTESIAN_POINT('Ctrl Pts',(-5.3569159887812,-4.13841227468388,
111.512129761263));
#211084=CARTESIAN_POINT('Ctrl Pts',(-5.24792617395999,-4.27577268183795,
111.52034062732));
#211085=CARTESIAN_POINT('Ctrl Pts',(-5.13382750693869,-4.40863971412949,
111.528551493377));
#211086=CARTESIAN_POINT('Ctrl Pts',(-5.0196813749727,-4.54156201898908,
111.536765775147));
#211087=CARTESIAN_POINT('Ctrl Pts',(-4.90042238859834,-4.669986955145,111.544980056916));
#211088=CARTESIAN_POINT('Ctrl Pts',(-4.77645063442172,-4.79351732415064,
111.553194338686));
#211089=CARTESIAN_POINT('Ctrl Pts',(-4.65233934024955,-4.91718673633799,
111.561417866279));
#211090=CARTESIAN_POINT('Ctrl Pts',(-4.5235049355893,-5.03595032620794,
111.569641393871));
#211091=CARTESIAN_POINT('Ctrl Pts',(-4.39038263637481,-5.14944941777455,
111.577864921463));
#211092=CARTESIAN_POINT('Ctrl Pts',(-4.25717501094456,-5.26302125784408,
111.586093720017));
#211093=CARTESIAN_POINT('Ctrl Pts',(-4.11967429125731,-5.37132165332404,
111.594322518571));
#211094=CARTESIAN_POINT('Ctrl Pts',(-3.97834603516961,-5.47403432802995,
111.602551317124));
#211095=CARTESIAN_POINT('Ctrl Pts',(-3.83682325204705,-5.57688837851312,
111.610791441961));
#211096=CARTESIAN_POINT('Ctrl Pts',(-3.69146270466835,-5.67413914863146,
111.619031566797));
#211097=CARTESIAN_POINT('Ctrl Pts',(-3.5427568364995,-5.7655149811128,111.627271691634));
#211098=CARTESIAN_POINT('Ctrl Pts',(-3.47673756789631,-5.80608207979363,
111.630929967004));
#211099=CARTESIAN_POINT('Ctrl Pts',(-3.41005923886211,-5.84549185225258,
111.634588242374));
#211100=CARTESIAN_POINT('Ctrl Pts',(-3.34276625935395,-5.88372354341405,
111.638246517744));
#211101=CARTESIAN_POINT('Ctrl Pts',(-3.18736718051395,-5.97201164764738,
111.646694540506));
#211102=CARTESIAN_POINT('Ctrl Pts',(-3.02833327895385,-6.05421611942821,
111.655142563269));
#211103=CARTESIAN_POINT('Ctrl Pts',(-2.86616880205378,-6.13003796057852,
111.663590586031));
#211104=CARTESIAN_POINT('Ctrl Pts',(-2.70415282400838,-6.2057903694044,
111.672030872687));
#211105=CARTESIAN_POINT('Ctrl Pts',(-2.53901228559528,-6.27517165736614,
111.680471159343));
#211106=CARTESIAN_POINT('Ctrl Pts',(-2.37127647446706,-6.33792843771836,
111.688911445999));
#211107=CARTESIAN_POINT('Ctrl Pts',(-2.20366844204516,-6.40063741086619,
111.697345302967));
#211108=CARTESIAN_POINT('Ctrl Pts',(-2.03346938941416,-6.45673182006865,
111.705779159935));
#211109=CARTESIAN_POINT('Ctrl Pts',(-1.86122941383928,-6.50600599977125,
111.714213016902));
#211110=CARTESIAN_POINT('Ctrl Pts',(-1.6890941691114,-6.55525021821452,
111.722641745647));
#211111=CARTESIAN_POINT('Ctrl Pts',(-1.51492079549191,-6.59768238376883,
111.731070474393));
#211112=CARTESIAN_POINT('Ctrl Pts',(-1.33927579284736,-6.63314626332731,
111.739499203138));
#211113=CARTESIAN_POINT('Ctrl Pts',(-1.16371061892958,-6.6685940249416,
111.747924101118));
#211114=CARTESIAN_POINT('Ctrl Pts',(-0.986675476022788,-6.69707974970367,
111.756348999098));
#211115=CARTESIAN_POINT('Ctrl Pts',(-0.808748720862408,-6.71849793529055,
111.764773897078));
#211116=CARTESIAN_POINT('Ctrl Pts',(-0.630861358975024,-6.73991137885631,
111.773196929773));
#211117=CARTESIAN_POINT('Ctrl Pts',(-0.45208310891277,-6.75426036064216,
111.781619962467));
#211118=CARTESIAN_POINT('Ctrl Pts',(-0.272999678763831,-6.76149097281028,
111.790042995161));
#211119=CARTESIAN_POINT('Ctrl Pts',(-0.0939365117016369,-6.76872076684283,
111.798465074798));
#211120=CARTESIAN_POINT('Ctrl Pts',(0.0854314334736309,-6.76883378348118,
111.806887154436));
#211121=CARTESIAN_POINT('Ctrl Pts',(0.264515882139856,-6.76182818090609,
111.815309234074));
#211122=CARTESIAN_POINT('Ctrl Pts',(0.443605066455603,-6.75482239307718,
111.823731536422));
#211123=CARTESIAN_POINT('Ctrl Pts',(0.622410406113715,-6.74069762414627,
111.83215383877));
#211124=CARTESIAN_POINT('Ctrl Pts',(0.800345813124003,-6.71950411707701,
111.840576141118));
#211125=CARTESIAN_POINT('Ctrl Pts',(0.978310765296193,-6.69830709094649,
111.848999841942));
#211126=CARTESIAN_POINT('Ctrl Pts',(1.1554051658182,-6.67003902665602,111.857423542766));
#211127=CARTESIAN_POINT('Ctrl Pts',(1.33104984743644,-6.634801828513,111.865847243589));
#211128=CARTESIAN_POINT('Ctrl Pts',(1.50681338941625,-6.5995407850359,111.874276644808));
#211129=CARTESIAN_POINT('Ctrl Pts',(1.68112492485148,-6.55730124950671,
111.882706046027));
#211130=CARTESIAN_POINT('Ctrl Pts',(1.85341625176118,-6.50823610494484,
111.891135447246));
#211131=CARTESIAN_POINT('Ctrl Pts',(2.02576905197698,-6.45915345400754,
111.899567856064));
#211132=CARTESIAN_POINT('Ctrl Pts',(2.1960998874038,-6.40324043528048,111.908000264882));
#211133=CARTESIAN_POINT('Ctrl Pts',(2.36385689412829,-6.34069945542936,
111.916432673699));
#211134=CARTESIAN_POINT('Ctrl Pts',(2.53176911451663,-6.27810061084393,
111.924872884427));
#211135=CARTESIAN_POINT('Ctrl Pts',(2.69710243777705,-6.20886167498664,
111.933313095154));
#211136=CARTESIAN_POINT('Ctrl Pts',(2.8593250855342,-6.13323316491676,111.941753305882));
#211137=CARTESIAN_POINT('Ctrl Pts',(2.95159455939098,-6.09021695892334,
111.946553953719));
#211138=CARTESIAN_POINT('Ctrl Pts',(3.04285810585875,-6.04513449256421,
111.951354601556));
#211139=CARTESIAN_POINT('Ctrl Pts',(3.13302154779196,-5.99803842777547,
111.956155249393));
#211140=CARTESIAN_POINT('Ctrl Pts',(3.28589773213795,-5.91818492475652,
111.964294964426));
#211141=CARTESIAN_POINT('Ctrl Pts',(3.43591455379587,-5.83238075773,111.972434679459));
#211142=CARTESIAN_POINT('Ctrl Pts',(3.58257337921973,-5.74085855796031,
111.980574394492));
#211143=CARTESIAN_POINT('Ctrl Pts',(3.72910393771476,-5.64941640295745,
111.988706990579));
#211144=CARTESIAN_POINT('Ctrl Pts',(3.872282037274,-5.55226636213545,111.996839586666));
#211145=CARTESIAN_POINT('Ctrl Pts',(4.01163239484831,-5.44968756247582,
112.004972182753));
#211146=CARTESIAN_POINT('Ctrl Pts',(4.15088748504222,-5.34717889118685,
112.013099218961));
#211147=CARTESIAN_POINT('Ctrl Pts',(4.2863197495549,-5.23924906645606,112.021226255169));
#211148=CARTESIAN_POINT('Ctrl Pts',(4.41748177444461,-5.12622119815851,
112.029353291377));
#211149=CARTESIAN_POINT('Ctrl Pts',(4.54858110151278,-5.01324735922749,
112.037476442714));
#211150=CARTESIAN_POINT('Ctrl Pts',(4.67541397693466,-4.89518056806295,
112.045599594052));
#211151=CARTESIAN_POINT('Ctrl Pts',(4.79756507756997,-4.77238497257724,
112.053722745389));
#211152=CARTESIAN_POINT('Ctrl Pts',(4.91968185283819,-4.64962388356646,
112.061843614061));
#211153=CARTESIAN_POINT('Ctrl Pts',(5.03711921628153,-4.52213689696127,
112.069964482733));
#211154=CARTESIAN_POINT('Ctrl Pts',(5.14949784846359,-4.39032583172011,
112.078085351404));
#211155=CARTESIAN_POINT('Ctrl Pts',(5.26188255401701,-4.25850764290454,
112.086206658959));
#211156=CARTESIAN_POINT('Ctrl Pts',(5.36920774149492,-4.12236518469301,
112.094327966513));
#211157=CARTESIAN_POINT('Ctrl Pts',(5.47113350797286,-3.98233438298902,
112.102449274068));
#211158=CARTESIAN_POINT('Ctrl Pts',(5.52409767935999,-3.90956951069805,
112.106669387785));
#211159=CARTESIAN_POINT('Ctrl Pts',(5.57560456872712,-3.83575524073842,
112.110889501501));
#211160=CARTESIAN_POINT('Ctrl Pts',(5.62561100293929,-3.76095597469692,
112.115109615218));
#211161=CARTESIAN_POINT('Ctrl Pts',(5.73207252607099,-3.60171159110169,
112.124094053744));
#211162=CARTESIAN_POINT('Ctrl Pts',(5.83167813022279,-3.43808012896981,
112.13307849227));
#211163=CARTESIAN_POINT('Ctrl Pts',(5.9241128718985,-3.2706537085125,112.142062930796));
#211164=CARTESIAN_POINT('Ctrl Pts',(6.01670715042143,-3.10293832004621,
112.151062875926));
#211165=CARTESIAN_POINT('Ctrl Pts',(6.10210571370995,-2.93141509105327,
112.160062821056));
#211166=CARTESIAN_POINT('Ctrl Pts',(6.18004047149519,-2.75669889010054,
112.169062766187));
#211167=CARTESIAN_POINT('Ctrl Pts',(6.25815888453759,-2.58157096593562,
112.178083919919));
#211168=CARTESIAN_POINT('Ctrl Pts',(6.32877820230573,-2.40323523398682,
112.187105073651));
#211169=CARTESIAN_POINT('Ctrl Pts',(6.39167823989611,-2.22232722109923,
112.196126227384));
#211170=CARTESIAN_POINT('Ctrl Pts',(6.45464227877061,-2.04123513288232,
112.205156560211));
#211171=CARTESIAN_POINT('Ctrl Pts',(6.50987127351077,-1.85756576244736,
112.214186893038));
#211172=CARTESIAN_POINT('Ctrl Pts',(6.55719508516186,-1.67196938223437,
112.223217225865));
#211173=CARTESIAN_POINT('Ctrl Pts',(6.60458598706047,-1.48610988485787,
112.232260360858));
#211174=CARTESIAN_POINT('Ctrl Pts',(6.64404923801519,-1.29831814689144,
112.241303495851));
#211175=CARTESIAN_POINT('Ctrl Pts',(6.67546545442912,-1.10925649275693,
112.250346630843));
#211176=CARTESIAN_POINT('Ctrl Pts',(6.70293046544743,-0.943973049788264,
112.258252414243));
#211177=CARTESIAN_POINT('Ctrl Pts',(6.7242460679943,-0.777719274635746,
112.266158197643));
#211178=CARTESIAN_POINT('Ctrl Pts',(6.73936492970172,-0.610941359138955,
112.274063981043));
#211179=CARTESIAN_POINT('Ctrl Pts',(6.75591349589758,-0.428392207753313,
112.282717369271));
#211180=CARTESIAN_POINT('Ctrl Pts',(6.76505125333847,-0.245053711462206,
112.2913707575));
#211181=CARTESIAN_POINT('Ctrl Pts',(6.76672018542856,-0.0615380541914957,
112.300024145728));
#211182=CARTESIAN_POINT('Ctrl Pts',(6.76838757614148,0.121808113351996,
112.308669541938));
#211183=CARTESIAN_POINT('Ctrl Pts',(6.76259989693947,0.305330812575991,
112.317314938149));
#211184=CARTESIAN_POINT('Ctrl Pts',(6.74935107993639,0.488414782496964,
112.325960334359));
#211185=CARTESIAN_POINT('Ctrl Pts',(6.73567914034827,0.677345837679467,
112.334881835401));
#211186=CARTESIAN_POINT('Ctrl Pts',(6.71406156928113,0.865809353393924,
112.343803336444));
#211187=CARTESIAN_POINT('Ctrl Pts',(6.68454996728575,1.05312902099413,112.352724837486));
#211188=CARTESIAN_POINT('Ctrl Pts',(6.65600616544271,1.23430574851037,112.361353767828));
#211189=CARTESIAN_POINT('Ctrl Pts',(6.62007790720542,1.41441212660026,112.36998269817));
#211190=CARTESIAN_POINT('Ctrl Pts',(6.57686455678845,1.59284073330005,112.378611628512));
#211191=CARTESIAN_POINT('Ctrl Pts',(6.53145343219199,1.78034398431475,112.387679414905));
#211192=CARTESIAN_POINT('Ctrl Pts',(6.47799690861243,1.96599401890645,112.396747201297));
#211193=CARTESIAN_POINT('Ctrl Pts',(6.41667141943653,2.1490967625927,112.40581498769));
#211194=CARTESIAN_POINT('Ctrl Pts',(6.35534593026067,2.33219950627884,112.414882774083));
#211195=CARTESIAN_POINT('Ctrl Pts',(6.28615156612699,2.51275457758295,112.423950560475));
#211196=CARTESIAN_POINT('Ctrl Pts',(6.2093263287872,2.69008467201873,112.433018346868));
#211197=CARTESIAN_POINT('Ctrl Pts',(6.13794735860817,2.85484354502542,112.441443303001));
#211198=CARTESIAN_POINT('Ctrl Pts',(6.06001263660661,3.01674628271946,112.449868259134));
#211199=CARTESIAN_POINT('Ctrl Pts',(5.9757836028002,3.17526366346234,112.458293215267));
#211200=CARTESIAN_POINT('Ctrl Pts',(5.89153501862637,3.33381783761118,112.466720126914));
#211201=CARTESIAN_POINT('Ctrl Pts',(5.80098936528815,3.48898479525786,112.47514703856));
#211202=CARTESIAN_POINT('Ctrl Pts',(5.70445366342969,3.64026062278289,112.483573950207));
#211203=CARTESIAN_POINT('Ctrl Pts',(5.60788246163335,3.79159208032226,112.492003960757));
#211204=CARTESIAN_POINT('Ctrl Pts',(5.50531699749254,3.93902927521756,112.500433971307));
#211205=CARTESIAN_POINT('Ctrl Pts',(5.39710737483285,4.08209762065104,112.508863981857));
#211206=CARTESIAN_POINT('Ctrl Pts',(5.2887980717319,4.22529775765215,112.517301757956));
#211207=CARTESIAN_POINT('Ctrl Pts',(5.17483442258572,4.36412073994748,112.525739534055));
#211208=CARTESIAN_POINT('Ctrl Pts',(5.05560725332516,4.49812453141596,112.534177310155));
#211209=CARTESIAN_POINT('Ctrl Pts',(4.9363174985895,4.63219866499695,112.542619515465));
#211210=CARTESIAN_POINT('Ctrl Pts',(4.81175893933917,4.76144832026906,112.551061720775));
#211211=CARTESIAN_POINT('Ctrl Pts',(4.68235934424135,4.8854682448457,112.559503926085));
#211212=CARTESIAN_POINT('Ctrl Pts',(4.55282323969055,5.00961900361892,112.567955037457));
#211213=CARTESIAN_POINT('Ctrl Pts',(4.41843614209166,5.12852878730048,112.576406148829));
#211214=CARTESIAN_POINT('Ctrl Pts',(4.27965977847555,5.24183185351253,112.584857260201));
#211215=CARTESIAN_POINT('Ctrl Pts',(4.24071197706516,5.2736305345489,112.587229077698));
#211216=CARTESIAN_POINT('Ctrl Pts',(4.20141863738297,5.30498785735915,112.589600895195));
#211217=CARTESIAN_POINT('Ctrl Pts',(4.16179038218708,5.33589634595118,112.591972712692));
#211218=CARTESIAN_POINT('Ctrl Pts',(4.02282528575888,5.44428368413728,112.600290006642));
#211219=CARTESIAN_POINT('Ctrl Pts',(3.87948861439683,5.54734401221526,112.608607300593));
#211220=CARTESIAN_POINT('Ctrl Pts',(3.73222217648751,5.64471492861552,112.616924594543));
#211221=CARTESIAN_POINT('Ctrl Pts',(3.58509593048532,5.74199315169974,112.625233970754));
#211222=CARTESIAN_POINT('Ctrl Pts',(3.43404766322085,5.8335925672391,112.633543346964));
#211223=CARTESIAN_POINT('Ctrl Pts',(3.2795507336467,5.9191921733829,112.641852723175));
#211224=CARTESIAN_POINT('Ctrl Pts',(3.21990673724492,5.95223815439306,112.645060582426));
#211225=CARTESIAN_POINT('Ctrl Pts',(3.15974908850186,5.98439038696173,112.648268441677));
#211226=CARTESIAN_POINT('Ctrl Pts',(3.09910619832117,6.01563211736949,112.651476300929));
#211227=CARTESIAN_POINT('Origin',(0.,0.,4.30282021618968));
#211228=CARTESIAN_POINT('',(3.09910619832124,6.01563211736945,115.045544419485));
#211229=CARTESIAN_POINT('',(3.09910619832145,6.01563211736935,114.651477942722));
#211230=CARTESIAN_POINT('',(3.09910619832133,6.0156321173694,4.30282021618968));
#211231=CARTESIAN_POINT('',(-6.76699958356027,-0.0015344574147271,113.69717978381));
#211232=CARTESIAN_POINT('Ctrl Pts',(-6.76699900317075,-0.00367302138866391,
113.69717978381));
#211233=CARTESIAN_POINT('Ctrl Pts',(-6.76689437423714,-0.196436366462953,
113.706228878238));
#211234=CARTESIAN_POINT('Ctrl Pts',(-6.75854901500553,-0.389028701790154,
113.715277972666));
#211235=CARTESIAN_POINT('Ctrl Pts',(-6.74203162654055,-0.58077409267894,
113.724327067093));
#211236=CARTESIAN_POINT('Ctrl Pts',(-6.72548378829893,-0.772872965859097,
113.733392843511));
#211237=CARTESIAN_POINT('Ctrl Pts',(-6.70073382333768,-0.964121546945956,
113.742458619928));
#211238=CARTESIAN_POINT('Ctrl Pts',(-6.66790201356897,-1.15385082980553,
113.751524396346));
#211239=CARTESIAN_POINT('Ctrl Pts',(-6.63499621702891,-1.34400766926847,
113.76061060257));
#211240=CARTESIAN_POINT('Ctrl Pts',(-6.59397217635658,-1.53263813607671,
113.769696808794));
#211241=CARTESIAN_POINT('Ctrl Pts',(-6.54500142042759,-1.71908272244265,
113.778783015018));
#211242=CARTESIAN_POINT('Ctrl Pts',(-6.49598097478889,-1.90571649064166,
113.787878440846));
#211243=CARTESIAN_POINT('Ctrl Pts',(-6.43899776506071,-2.09015972871107,
113.796973866673));
#211244=CARTESIAN_POINT('Ctrl Pts',(-6.37427315611694,-2.27176819486651,
113.806069292501));
#211245=CARTESIAN_POINT('Ctrl Pts',(-6.30947624815692,-2.45357952224675,
113.815174878148));
#211246=CARTESIAN_POINT('Ctrl Pts',(-6.23692073063983,-2.63254953413714,
113.824280463795));
#211247=CARTESIAN_POINT('Ctrl Pts',(-6.15687675812367,-2.80805227609397,
113.833386049442));
#211248=CARTESIAN_POINT('Ctrl Pts',(-6.14061305305923,-2.84371173605658,
113.835236164507));
#211249=CARTESIAN_POINT('Ctrl Pts',(-6.12404035022347,-2.879228126544,113.837086279572));
#211250=CARTESIAN_POINT('Ctrl Pts',(-6.1071611522584,-2.91459631172927,
113.838936394636));
#211251=CARTESIAN_POINT('Ctrl Pts',(-6.02821349340788,-3.08002096187836,
113.847589782865));
#211252=CARTESIAN_POINT('Ctrl Pts',(-5.9424902228326,-3.2423417052089,113.856243171093));
#211253=CARTESIAN_POINT('Ctrl Pts',(-5.85025392639332,-3.40100249878172,
113.864896559321));
#211254=CARTESIAN_POINT('Ctrl Pts',(-5.75810281671668,-3.55951675785693,
113.873541955532));
#211255=CARTESIAN_POINT('Ctrl Pts',(-5.6594508309726,-3.71437754718037,
113.882187351742));
#211256=CARTESIAN_POINT('Ctrl Pts',(-5.55460679741111,-3.86505269383929,
113.890832747952));
#211257=CARTESIAN_POINT('Ctrl Pts',(-5.44641439859597,-4.02053989711718,
113.899754248995));
#211258=CARTESIAN_POINT('Ctrl Pts',(-5.33162803129022,-4.17156938435437,
113.908675750037));
#211259=CARTESIAN_POINT('Ctrl Pts',(-5.21063727443873,-4.31758592204368,
113.91759725108));
#211260=CARTESIAN_POINT('Ctrl Pts',(-5.09361427484186,-4.45881400983989,
113.926226181421));
#211261=CARTESIAN_POINT('Ctrl Pts',(-4.97078756366853,-4.59535245201296,
113.934855111763));
#211262=CARTESIAN_POINT('Ctrl Pts',(-4.84255263117004,-4.72672963203398,
113.943484042105));
#211263=CARTESIAN_POINT('Ctrl Pts',(-4.70779583862508,-4.86478848267864,
113.952551828498));
#211264=CARTESIAN_POINT('Ctrl Pts',(-4.56706657312259,-4.99714712081148,
113.961619614891));
#211265=CARTESIAN_POINT('Ctrl Pts',(-4.42087082812759,-5.12329875383141,
113.970687401283));
#211266=CARTESIAN_POINT('Ctrl Pts',(-4.27467508313269,-5.24945038685125,
113.979755187676));
#211267=CARTESIAN_POINT('Ctrl Pts',(-4.12301313130337,-5.36939473298295,
113.988822974069));
#211268=CARTESIAN_POINT('Ctrl Pts',(-3.96643535015231,-5.48267084668249,
113.997890760461));
#211269=CARTESIAN_POINT('Ctrl Pts',(-3.82095762488303,-5.58791663077274,
114.006315716594));
#211270=CARTESIAN_POINT('Ctrl Pts',(-3.67130032260777,-5.68736012850898,
114.014740672728));
#211271=CARTESIAN_POINT('Ctrl Pts',(-3.51795839032686,-5.78067969739968,
114.023165628861));
#211272=CARTESIAN_POINT('Ctrl Pts',(-3.36458086591139,-5.87402092665819,
114.031592540507));
#211273=CARTESIAN_POINT('Ctrl Pts',(-3.20751728954559,-5.9612352205724,
114.040019452154));
#211274=CARTESIAN_POINT('Ctrl Pts',(-3.04728888604715,-6.04204596514902,
114.0484463638));
#211275=CARTESIAN_POINT('Ctrl Pts',(-2.88700156032323,-6.12288642698431,
114.05687637435));
#211276=CARTESIAN_POINT('Ctrl Pts',(-2.72354738283741,-6.19731849490898,
114.0653063849));
#211277=CARTESIAN_POINT('Ctrl Pts',(-2.55746965732247,-6.26511276449793,
114.07373639545));
#211278=CARTESIAN_POINT('Ctrl Pts',(-2.39123894448031,-6.33296948475011,
114.08217417155));
#211279=CARTESIAN_POINT('Ctrl Pts',(-2.2223801623688,-6.39417606482082,
114.090611947649));
#211280=CARTESIAN_POINT('Ctrl Pts',(-2.05145501773262,-6.4485518769891,
114.099049723749));
#211281=CARTESIAN_POINT('Ctrl Pts',(-1.88044014999527,-6.50295623245045,
114.107491929058));
#211282=CARTESIAN_POINT('Ctrl Pts',(-1.70735707444414,-6.55052257589034,
114.115934134368));
#211283=CARTESIAN_POINT('Ctrl Pts',(-1.53278049021885,-6.59112076727505,
114.124376339678));
#211284=CARTESIAN_POINT('Ctrl Pts',(-1.35801973730266,-6.6317617875179,
114.13282745105));
#211285=CARTESIAN_POINT('Ctrl Pts',(-1.18176265275826,-6.66541990398635,
114.141278562422));
#211286=CARTESIAN_POINT('Ctrl Pts',(-1.00459297023075,-6.69201628540778,
114.149729673794));
#211287=CARTESIAN_POINT('Ctrl Pts',(-0.954870024398131,-6.69948060105082,
114.152101491292));
#211288=CARTESIAN_POINT('Ctrl Pts',(-0.905075224424326,-6.70638901133912,
114.154473308789));
#211289=CARTESIAN_POINT('Ctrl Pts',(-0.855221520991905,-6.71274050966014,
114.156845126286));
#211290=CARTESIAN_POINT('Ctrl Pts',(-0.680420138253832,-6.7350106844422,
114.16516139869));
#211291=CARTESIAN_POINT('Ctrl Pts',(-0.504578855812174,-6.75047035467769,
114.173477671094));
#211292=CARTESIAN_POINT('Ctrl Pts',(-0.32826236490003,-6.75903342348521,
114.181793943498));
#211293=CARTESIAN_POINT('Ctrl Pts',(-0.152094949788854,-6.76758925220797,
114.190103184484));
#211294=CARTESIAN_POINT('Ctrl Pts',(0.0245465275011359,-6.76926008037718,
114.19841242547));
#211295=CARTESIAN_POINT('Ctrl Pts',(0.201091196118341,-6.7640114821638,
114.206721666456));
#211296=CARTESIAN_POINT('Ctrl Pts',(0.377518964841279,-6.75876635933476,
114.215025405439));
#211297=CARTESIAN_POINT('Ctrl Pts',(0.553849705999729,-6.74661095003823,
114.223329144421));
#211298=CARTESIAN_POINT('Ctrl Pts',(0.72951125306365,-6.72756288202894,
114.231632883403));
#211299=CARTESIAN_POINT('Ctrl Pts',(0.905088677582643,-6.70852393594748,
114.239932645809));
#211300=CARTESIAN_POINT('Ctrl Pts',(1.07999720147008,-6.68259894677218,
114.248232408214));
#211301=CARTESIAN_POINT('Ctrl Pts',(1.25366826079113,-6.64985750914145,
114.25653217062));
#211302=CARTESIAN_POINT('Ctrl Pts',(1.42728796785662,-6.61712575272462,
114.264829478895));
#211303=CARTESIAN_POINT('Ctrl Pts',(1.5996705981879,-6.57758162976744,114.273126787169));
#211304=CARTESIAN_POINT('Ctrl Pts',(1.77025605793167,-6.53134614680284,
114.281424095444));
#211305=CARTESIAN_POINT('Ctrl Pts',(1.94085875286182,-6.48510599241331,
114.289722242041));
#211306=CARTESIAN_POINT('Ctrl Pts',(2.10966357660211,-6.43217321087091,
114.298020388638));
#211307=CARTESIAN_POINT('Ctrl Pts',(2.27612334854146,-6.37271931770296,
114.306318535235));
#211308=CARTESIAN_POINT('Ctrl Pts',(2.44259985905783,-6.31325944607211,
114.314617516263));
#211309=CARTESIAN_POINT('Ctrl Pts',(2.60673051971744,-6.24727727237146,
114.322916497291));
#211310=CARTESIAN_POINT('Ctrl Pts',(2.76798605330123,-6.17499329624979,
114.33121547832));
#211311=CARTESIAN_POINT('Ctrl Pts',(2.92928460098828,-6.10269003874073,
114.339516673059));
#211312=CARTESIAN_POINT('Ctrl Pts',(3.0877061754348,-6.0240817708348,114.347817867799));
#211313=CARTESIAN_POINT('Ctrl Pts',(3.24274394777183,-5.93943605817835,
114.356119062538));
#211314=CARTESIAN_POINT('Ctrl Pts',(3.39784884421087,-5.85475369788845,
114.364423851307));
#211315=CARTESIAN_POINT('Ctrl Pts',(3.5495667134581,-5.76402884992579,114.372728640075));
#211316=CARTESIAN_POINT('Ctrl Pts',(3.69741751237913,-5.66757379653341,
114.381033428844));
#211317=CARTESIAN_POINT('Ctrl Pts',(3.84544358709434,-5.57100439654156,
114.389348062865));
#211318=CARTESIAN_POINT('Ctrl Pts',(3.98959314018117,-5.46869140895762,
114.397662696886));
#211319=CARTESIAN_POINT('Ctrl Pts',(4.12941622270605,-5.36098970896719,
114.405977330907));
#211320=CARTESIAN_POINT('Ctrl Pts',(4.26932771660553,-5.25321990823708,
114.414297222344));
#211321=CARTESIAN_POINT('Ctrl Pts',(4.40490701755354,-5.14005482273073,
114.422617113782));
#211322=CARTESIAN_POINT('Ctrl Pts',(4.53573909875177,-5.02188807402699,
114.43093700522));
#211323=CARTESIAN_POINT('Ctrl Pts',(4.66676681633366,-4.90354462771839,
114.439269337593));
#211324=CARTESIAN_POINT('Ctrl Pts',(4.79303287882259,-4.78018481437875,
114.447601669967));
#211325=CARTESIAN_POINT('Ctrl Pts',(4.91415985886355,-4.6522383732494,114.45593400234));
#211326=CARTESIAN_POINT('Ctrl Pts',(5.00535450365117,-4.55590946084123,
114.462207287538));
#211327=CARTESIAN_POINT('Ctrl Pts',(5.09363692900752,-4.45698142058885,
114.468480572737));
#211328=CARTESIAN_POINT('Ctrl Pts',(5.17886189454271,-4.35564903054108,
114.474753857935));
#211329=CARTESIAN_POINT('Ctrl Pts',(5.28849382194581,-4.2252967897448,114.482823703938));
#211330=CARTESIAN_POINT('Ctrl Pts',(5.393403467879,-4.09056191938812,114.490893549941));
#211331=CARTESIAN_POINT('Ctrl Pts',(5.49320988142311,-3.95182669137141,
114.498963395943));
#211332=CARTESIAN_POINT('Ctrl Pts',(5.59289072580415,-3.81326600991792,
114.507023089053));
#211333=CARTESIAN_POINT('Ctrl Pts',(5.68748089774783,-3.67071528400997,
114.515082782164));
#211334=CARTESIAN_POINT('Ctrl Pts',(5.77663707538635,-3.52459261465377,
114.523142475274));
#211335=CARTESIAN_POINT('Ctrl Pts',(5.86570065017356,-3.3786217168986,114.531193797112));
#211336=CARTESIAN_POINT('Ctrl Pts',(5.94934126973096,-3.22908657447404,
114.539245118951));
#211337=CARTESIAN_POINT('Ctrl Pts',(6.0272566930702,-3.07643718542091,114.547296440789));
#211338=CARTESIAN_POINT('Ctrl Pts',(6.10510826279098,-2.9239128963214,114.55534116437));
#211339=CARTESIAN_POINT('Ctrl Pts',(6.17724380601086,-2.76827977091082,
114.563385887951));
#211340=CARTESIAN_POINT('Ctrl Pts',(6.24340519446697,-2.6100154362959,114.571430611533));
#211341=CARTESIAN_POINT('Ctrl Pts',(6.309526844784,-2.45184615908966,114.579470503257));
#211342=CARTESIAN_POINT('Ctrl Pts',(6.36968133983959,-2.29104916206528,
114.587510394981));
#211343=CARTESIAN_POINT('Ctrl Pts',(6.42365724300405,-2.12812514303122,
114.595550286706));
#211344=CARTESIAN_POINT('Ctrl Pts',(6.47879539524045,-1.96169292350735,
114.603763299326));
#211345=CARTESIAN_POINT('Ctrl Pts',(6.52748567183706,-1.79304139659062,
114.611976311946));
#211346=CARTESIAN_POINT('Ctrl Pts',(6.56955507424686,-1.62272459968948,
114.620189324566));
#211347=CARTESIAN_POINT('Ctrl Pts',(6.61072333291237,-1.45605605798767,
114.628226411108));
#211348=CARTESIAN_POINT('Ctrl Pts',(6.64555140720951,-1.28779324564021,
114.636263497651));
#211349=CARTESIAN_POINT('Ctrl Pts',(6.67392809233436,-1.11846896172861,
114.644300584193));
#211350=CARTESIAN_POINT('Ctrl Pts',(6.70230749324007,-0.949128472694808,
114.652338439923));
#211351=CARTESIAN_POINT('Ctrl Pts',(6.72423421368997,-0.778726678295768,
114.660376295652));
#211352=CARTESIAN_POINT('Ctrl Pts',(6.73964856015882,-0.607804479704708,
114.668414151381));
#211353=CARTESIAN_POINT('Ctrl Pts',(6.75506743594906,-0.436832057669557,
114.676454368938));
#211354=CARTESIAN_POINT('Ctrl Pts',(6.76397009529906,-0.265339298977427,
114.684494586495));
#211355=CARTESIAN_POINT('Ctrl Pts',(6.76634889959327,-0.0938699577763024,
114.692534804052));
#211356=CARTESIAN_POINT('Ctrl Pts',(6.76881757663786,0.0840776049989044,
114.70087878618));
#211357=CARTESIAN_POINT('Ctrl Pts',(6.76425981300117,0.261999501268101,
114.709222768307));
#211358=CARTESIAN_POINT('Ctrl Pts',(6.75272624786064,0.439291727049298,
114.717566750435));
#211359=CARTESIAN_POINT('Ctrl Pts',(6.74159321688892,0.610427001929132,
114.72562096527));
#211360=CARTESIAN_POINT('Ctrl Pts',(6.72396087294501,0.780975248063278,
114.733675180105));
#211361=CARTESIAN_POINT('Ctrl Pts',(6.6999271923359,0.950402345008659,114.74172939494));
#211362=CARTESIAN_POINT('Ctrl Pts',(6.67587552649109,1.11995623011949,114.749789637023));
#211363=CARTESIAN_POINT('Ctrl Pts',(6.6454130518287,1.28838693038434,114.757849879106));
#211364=CARTESIAN_POINT('Ctrl Pts',(6.60868813036923,1.45517359635093,114.765910121189));
#211365=CARTESIAN_POINT('Ctrl Pts',(6.57191186495037,1.62219344151743,114.773981632044));
#211366=CARTESIAN_POINT('Ctrl Pts',(6.52885577758208,1.78756430840956,114.782053142898));
#211367=CARTESIAN_POINT('Ctrl Pts',(6.47971719526489,1.95078293753779,114.790124653752));
#211368=CARTESIAN_POINT('Ctrl Pts',(6.47456695879007,1.96788995400967,114.790970632363));
#211369=CARTESIAN_POINT('Ctrl Pts',(6.46934994716255,1.98497334828446,114.791816610974));
#211370=CARTESIAN_POINT('Ctrl Pts',(6.46406641715298,2.00203255583794,114.792662589585));
#211371=CARTESIAN_POINT('Ctrl Pts',(6.41266291324009,2.16800171672818,114.800893121967));
#211372=CARTESIAN_POINT('Ctrl Pts',(6.35478770461155,2.33223379567073,114.809123654349));
#211373=CARTESIAN_POINT('Ctrl Pts',(6.29057391996948,2.49418699327053,114.81735418673));
#211374=CARTESIAN_POINT('Ctrl Pts',(6.22643842146596,2.65594274587407,114.825574684871));
#211375=CARTESIAN_POINT('Ctrl Pts',(6.15597986670637,2.81542481943731,114.833795183012));
#211376=CARTESIAN_POINT('Ctrl Pts',(6.07938154006315,2.97210516138635,114.842015681153));
#211377=CARTESIAN_POINT('Ctrl Pts',(6.00036179113173,3.13373847409526,114.85049604525));
#211378=CARTESIAN_POINT('Ctrl Pts',(5.914807788731,3.2923896370957,114.858976409347));
#211379=CARTESIAN_POINT('Ctrl Pts',(5.82297578598399,3.44749793268163,114.867456773444));
#211380=CARTESIAN_POINT('Ctrl Pts',(5.7341351925341,3.59755360626655,114.875660891361));
#211381=CARTESIAN_POINT('Ctrl Pts',(5.63941936316632,3.74429324906899,114.883865009278));
#211382=CARTESIAN_POINT('Ctrl Pts',(5.53910821141044,3.88723156273014,114.892069127194));
#211383=CARTESIAN_POINT('Ctrl Pts',(5.43885052391342,4.03009369252869,114.900268872446));
#211384=CARTESIAN_POINT('Ctrl Pts',(5.33300365820056,4.16915823509333,114.908468617697));
#211385=CARTESIAN_POINT('Ctrl Pts',(5.22189168595363,4.30396749757341,114.916668362949));
#211386=CARTESIAN_POINT('Ctrl Pts',(5.1108187307566,4.4387294216829,114.924865228854));
#211387=CARTESIAN_POINT('Ctrl Pts',(4.99448457957083,4.56923876574986,114.933062094759));
#211388=CARTESIAN_POINT('Ctrl Pts',(4.87325458860311,4.69506961765838,114.941258960664));
#211389=CARTESIAN_POINT('Ctrl Pts',(4.75204512506641,4.82087916308891,114.949454438623));
#211390=CARTESIAN_POINT('Ctrl Pts',(4.62594172279734,4.94201153723402,114.957649916583));
#211391=CARTESIAN_POINT('Ctrl Pts',(4.49534774608675,5.05807647646344,114.965845394543));
#211392=CARTESIAN_POINT('Ctrl Pts',(4.36472312348555,5.17416865212076,114.974042795698));
#211393=CARTESIAN_POINT('Ctrl Pts',(4.22960608763914,5.28519077688526,114.982240196853));
#211394=CARTESIAN_POINT('Ctrl Pts',(4.0904346602753,5.39079152722664,114.990437598008));
#211395=CARTESIAN_POINT('Ctrl Pts',(3.95124280374421,5.49640777884892,114.998636202471));
#211396=CARTESIAN_POINT('Ctrl Pts',(3.80799565962158,5.59660085905567,115.006834806933));
#211397=CARTESIAN_POINT('Ctrl Pts',(3.66116159176703,5.69106183404906,115.015033411396));
#211398=CARTESIAN_POINT('Ctrl Pts',(3.51424171971715,5.78557800841184,115.023236806809));
#211399=CARTESIAN_POINT('Ctrl Pts',(3.36373104430196,5.87435520186402,115.031440202222));
#211400=CARTESIAN_POINT('Ctrl Pts',(3.21012436996803,5.95712938665406,115.039643597635));
#211401=CARTESIAN_POINT('Ctrl Pts',(3.17329386362767,5.97697627905601,115.041610538251));
#211402=CARTESIAN_POINT('Ctrl Pts',(3.13628547049504,5.99647826776648,115.043577478868));
#211403=CARTESIAN_POINT('Ctrl Pts',(3.09910619832125,6.01563211736945,115.045544419485));
#211404=CARTESIAN_POINT('Ctrl Pts',(3.09910619832131,6.01563211736942,113.045755263024));
#211405=CARTESIAN_POINT('Ctrl Pts',(2.93375330764823,6.10081787314654,113.054504710927));
#211406=CARTESIAN_POINT('Ctrl Pts',(2.76488627843068,6.1791820703704,113.063254158829));
#211407=CARTESIAN_POINT('Ctrl Pts',(2.59307866646699,6.25045854553998,113.072003606731));
#211408=CARTESIAN_POINT('Ctrl Pts',(2.4212724418538,6.32173444515035,113.080752983982));
#211409=CARTESIAN_POINT('Ctrl Pts',(2.24652594672476,6.38592262741834,113.089502361232));
#211410=CARTESIAN_POINT('Ctrl Pts',(2.06943269687139,6.44280508110556,113.098251738482));
#211411=CARTESIAN_POINT('Ctrl Pts',(1.89234081822096,6.49968709436161,113.107001047987));
#211412=CARTESIAN_POINT('Ctrl Pts',(1.71290249405608,6.5492634045954,113.115750357493));
#211413=CARTESIAN_POINT('Ctrl Pts',(1.53172716625079,6.59136563150379,113.124499666998));
#211414=CARTESIAN_POINT('Ctrl Pts',(1.35055318107347,6.63346754640707,113.133248911665));
#211415=CARTESIAN_POINT('Ctrl Pts',(1.16764249714425,6.66809542395775,113.141998156333));
#211416=CARTESIAN_POINT('Ctrl Pts',(0.983616340614331,6.69513165624669,
113.150747401));
#211417=CARTESIAN_POINT('Ctrl Pts',(0.799591486713946,6.72216769715959,
113.159496583736));
#211418=CARTESIAN_POINT('Ctrl Pts',(0.614451459526949,6.74161215869368,
113.168245766471));
#211419=CARTESIAN_POINT('Ctrl Pts',(0.42882504791065,6.7533990018571,113.176994949207));
#211420=CARTESIAN_POINT('Ctrl Pts',(0.24319988859758,6.76518576550218,113.185744072918));
#211421=CARTESIAN_POINT('Ctrl Pts',(0.0570886373926176,6.76931499599833,
113.194493196628));
#211422=CARTESIAN_POINT('Ctrl Pts',(-0.128876626810283,6.76577266947849,
113.203242320339));
#211423=CARTESIAN_POINT('Ctrl Pts',(-0.314840698187232,6.76223036567997,
113.21199138793));
#211424=CARTESIAN_POINT('Ctrl Pts',(-0.500658497950266,6.7510166087923,
113.220740455522));
#211425=CARTESIAN_POINT('Ctrl Pts',(-0.685698951925173,6.73216948296229,
113.229489523113));
#211426=CARTESIAN_POINT('Ctrl Pts',(-0.870738280458717,6.71332247176308,
113.238238537492));
#211427=CARTESIAN_POINT('Ctrl Pts',(-1.05499998761128,6.68684221356206,
113.24698755187));
#211428=CARTESIAN_POINT('Ctrl Pts',(-1.23785829161289,6.65281863948547,
113.255736566249));
#211429=CARTESIAN_POINT('Ctrl Pts',(-1.43007412917269,6.6170539536889,113.264933299948));
#211430=CARTESIAN_POINT('Ctrl Pts',(-1.62073882535654,6.57295372727824,
113.274130033647));
#211431=CARTESIAN_POINT('Ctrl Pts',(-1.80913696091373,6.52068343478318,
113.283326767346));
#211432=CARTESIAN_POINT('Ctrl Pts',(-1.98838356185972,6.47095219815241,
113.29207676506));
#211433=CARTESIAN_POINT('Ctrl Pts',(-2.16557827572394,6.41382586850938,
113.300826762774));
#211434=CARTESIAN_POINT('Ctrl Pts',(-2.34011918621563,6.34949849943328,
113.309576760487));
#211435=CARTESIAN_POINT('Ctrl Pts',(-2.51465655690956,6.28517243495607,
113.318326580746));
#211436=CARTESIAN_POINT('Ctrl Pts',(-2.68653996295181,6.21364572242438,
113.327076401004));
#211437=CARTESIAN_POINT('Ctrl Pts',(-2.85518555379836,6.13516132252292,
113.335826221262));
#211438=CARTESIAN_POINT('Ctrl Pts',(-3.02382794858528,6.05667841000586,
113.3445758757));
#211439=CARTESIAN_POINT('Ctrl Pts',(-3.18923239109113,5.97123819492171,
113.353325530137));
#211440=CARTESIAN_POINT('Ctrl Pts',(-3.35083705967523,5.87913088810813,
113.362075184575));
#211441=CARTESIAN_POINT('Ctrl Pts',(-3.51243888042233,5.78702520443204,
113.370824684824));
#211442=CARTESIAN_POINT('Ctrl Pts',(-3.67024081223533,5.68825280605885,
113.379574185073));
#211443=CARTESIAN_POINT('Ctrl Pts',(-3.82370687544253,5.58314917682606,
113.388323685322));
#211444=CARTESIAN_POINT('Ctrl Pts',(-3.97717043817676,5.47804726008122,
113.397073043012));
#211445=CARTESIAN_POINT('Ctrl Pts',(-4.12629803722331,5.36661448084336,
113.405822400703));
#211446=CARTESIAN_POINT('Ctrl Pts',(-4.27058317206788,5.24922931204674,
113.414571758393));
#211447=CARTESIAN_POINT('Ctrl Pts',(-4.41486614774711,5.13184589986897,
113.423320985153));
#211448=CARTESIAN_POINT('Ctrl Pts',(-4.55430658194287,5.00851045723149,
113.432070211913));
#211449=CARTESIAN_POINT('Ctrl Pts',(-4.68843089001716,4.87964187103243,
113.440819438673));
#211450=CARTESIAN_POINT('Ctrl Pts',(-4.82255336917709,4.7507750420809,113.449568546129));
#211451=CARTESIAN_POINT('Ctrl Pts',(-4.95135966065008,4.61637541908229,
113.458317653585));
#211452=CARTESIAN_POINT('Ctrl Pts',(-5.0744123086912,4.47689945401986,113.467066761041));
#211453=CARTESIAN_POINT('Ctrl Pts',(-5.19746344226277,4.33742520555682,
113.475815760817));
#211454=CARTESIAN_POINT('Ctrl Pts',(-5.31476088454614,4.1928749549153,113.484564760594));
#211455=CARTESIAN_POINT('Ctrl Pts',(-5.42590627628689,4.04373961586928,
113.49331376037));
#211456=CARTESIAN_POINT('Ctrl Pts',(-5.5370638067251,3.89458798906959,113.502063715665));
#211457=CARTESIAN_POINT('Ctrl Pts',(-5.64206777071714,3.74085050155511,
113.510813670959));
#211458=CARTESIAN_POINT('Ctrl Pts',(-5.74056148163865,3.5830493822339,113.519563626254));
#211459=CARTESIAN_POINT('Ctrl Pts',(-5.83905138951744,3.42525435593521,
113.528313243695));
#211460=CARTESIAN_POINT('Ctrl Pts',(-5.93103139557516,3.26339625497431,
113.537062861136));
#211461=CARTESIAN_POINT('Ctrl Pts',(-6.01618907820714,3.09802485065262,
113.545812478577));
#211462=CARTESIAN_POINT('Ctrl Pts',(-6.10134392544864,2.93265895249889,
113.554561804693));
#211463=CARTESIAN_POINT('Ctrl Pts',(-6.17967677261725,2.76378023986275,
113.563311130809));
#211464=CARTESIAN_POINT('Ctrl Pts',(-6.25092157009129,2.59196229227346,
113.572060456925));
#211465=CARTESIAN_POINT('Ctrl Pts',(-6.32216437407666,2.4201491522932,113.580809538228));
#211466=CARTESIAN_POINT('Ctrl Pts',(-6.38631941548842,2.24539720663077,
113.58955861953));
#211467=CARTESIAN_POINT('Ctrl Pts',(-6.44316881037466,2.06829994947911,
113.598307700832));
#211468=CARTESIAN_POINT('Ctrl Pts',(-6.50002334524508,1.8911866802467,113.607057573175));
#211469=CARTESIAN_POINT('Ctrl Pts',(-6.5495708241104,1.71172794807917,113.615807445517));
#211470=CARTESIAN_POINT('Ctrl Pts',(-6.59164294296035,1.5305333425055,113.62455731786));
#211471=CARTESIAN_POINT('Ctrl Pts',(-6.63371214082094,1.34935131693797,
113.633306582714));
#211472=CARTESIAN_POINT('Ctrl Pts',(-6.66830695239658,1.16643393829949,
113.642055847569));
#211473=CARTESIAN_POINT('Ctrl Pts',(-6.69530988153963,0.982402458342716,
113.650805112424));
#211474=CARTESIAN_POINT('Ctrl Pts',(-6.7223141969046,0.798361530948934,
113.659554826431));
#211475=CARTESIAN_POINT('Ctrl Pts',(-6.74172580829259,0.613206671364498,
113.668304540438));
#211476=CARTESIAN_POINT('Ctrl Pts',(-6.75347878028166,0.427566795115567,
113.677054254445));
#211477=CARTESIAN_POINT('Ctrl Pts',(-6.76248992368202,0.285234494208126,
113.683762764234));
#211478=CARTESIAN_POINT('Ctrl Pts',(-6.76699999999988,0.14261726609567,
113.690471274022));
#211479=CARTESIAN_POINT('Ctrl Pts',(-6.767,5.6607593898505E-12,113.69717978381));
#211480=CARTESIAN_POINT('',(-6.76699758240985,0.00572011007101653,113.302820216219));
#211481=CARTESIAN_POINT('Ctrl Pts',(3.09910619832117,6.01563211736949,112.651476300929));
#211482=CARTESIAN_POINT('Ctrl Pts',(2.94216084648394,6.09648651524266,112.65977832277));
#211483=CARTESIAN_POINT('Ctrl Pts',(2.78196365508099,6.17123922757144,112.668080344612));
#211484=CARTESIAN_POINT('Ctrl Pts',(2.61902520880535,6.23963107528339,112.676382366453));
#211485=CARTESIAN_POINT('Ctrl Pts',(2.45615325715405,6.30799501251548,112.684681000268));
#211486=CARTESIAN_POINT('Ctrl Pts',(2.29054260050473,6.37000312427212,112.692979634083));
#211487=CARTESIAN_POINT('Ctrl Pts',(2.12272554717872,6.42544358401463,112.701278267898));
#211488=CARTESIAN_POINT('Ctrl Pts',(1.94695780854505,6.48351065195929,112.709970066916));
#211489=CARTESIAN_POINT('Ctrl Pts',(1.76876988491877,6.53437243729533,112.718661865935));
#211490=CARTESIAN_POINT('Ctrl Pts',(1.58879394997375,6.57784332319696,112.727353664953));
#211491=CARTESIAN_POINT('Ctrl Pts',(1.4169651523386,6.61934637225124,112.735652004257));
#211492=CARTESIAN_POINT('Ctrl Pts',(1.24350702150804,6.65411283860715,112.74395034356));
#211493=CARTESIAN_POINT('Ctrl Pts',(1.06898240011114,6.68203304603117,112.752248682864));
#211494=CARTESIAN_POINT('Ctrl Pts',(0.894427644215701,6.70995807433057,
112.76054845501));
#211495=CARTESIAN_POINT('Ctrl Pts',(0.718806374435361,6.73103443232346,
112.768848227156));
#211496=CARTESIAN_POINT('Ctrl Pts',(0.542688928166128,6.74520405378858,
112.777147999302));
#211497=CARTESIAN_POINT('Ctrl Pts',(0.366511802430087,6.75937847679649,
112.785450583923));
#211498=CARTESIAN_POINT('Ctrl Pts',(0.189838511953434,6.7666414708263,112.793753168544));
#211499=CARTESIAN_POINT('Ctrl Pts',(0.0132419777114451,6.76698704373123,
112.802055753166));
#211500=CARTESIAN_POINT('Ctrl Pts',(-0.163443752358986,6.76733279117901,
112.810362531278));
#211501=CARTESIAN_POINT('Ctrl Pts',(-0.340052301292425,6.76075415346924,
112.81866930939));
#211502=CARTESIAN_POINT('Ctrl Pts',(-0.516013097001385,6.74729719841383,
112.826976087502));
#211503=CARTESIAN_POINT('Ctrl Pts',(-0.692185344402196,6.73382407216583,
112.83529284785));
#211504=CARTESIAN_POINT('Ctrl Pts',(-0.867707936634538,6.71345614436573,
112.843609608199));
#211505=CARTESIAN_POINT('Ctrl Pts',(-1.04201666411697,6.68629121948054,
112.851926368547));
#211506=CARTESIAN_POINT('Ctrl Pts',(-1.21644694796818,6.6591073507956,112.860248928692));
#211507=CARTESIAN_POINT('Ctrl Pts',(-1.38966133851836,6.62511709999945,
112.868571488838));
#211508=CARTESIAN_POINT('Ctrl Pts',(-1.56110797599251,6.58446891459688,
112.876894048983));
#211509=CARTESIAN_POINT('Ctrl Pts',(-1.73279006376821,6.54376490641673,
112.885228038628));
#211510=CARTESIAN_POINT('Ctrl Pts',(-1.9026992149796,6.49638479275102,112.893562028273));
#211511=CARTESIAN_POINT('Ctrl Pts',(-2.0702998180236,6.44252649691807,112.901896017918));
#211512=CARTESIAN_POINT('Ctrl Pts',(-2.12383009348857,6.42532459334703,
112.904557826726));
#211513=CARTESIAN_POINT('Ctrl Pts',(-2.17712503241312,6.40746220700864,
112.907219635534));
#211514=CARTESIAN_POINT('Ctrl Pts',(-2.23016766295307,6.38894679858257,
112.909881444342));
#211515=CARTESIAN_POINT('Ctrl Pts',(-2.39097780782322,6.33281335495399,
112.917951290345));
#211516=CARTESIAN_POINT('Ctrl Pts',(-2.54996417962467,6.27050081463263,
112.926021136347));
#211517=CARTESIAN_POINT('Ctrl Pts',(-2.70660406864465,6.20214345332291,
112.93409098235));
#211518=CARTESIAN_POINT('Ctrl Pts',(-2.86304688476049,6.13387209426841,
112.94215067546));
#211519=CARTESIAN_POINT('Ctrl Pts',(-3.01714875451401,6.05957119371045,
112.95021036857));
#211520=CARTESIAN_POINT('Ctrl Pts',(-3.16840103803268,5.9794250444498,112.95827006168));
#211521=CARTESIAN_POINT('Ctrl Pts',(-3.31949622203139,5.89936213969483,
112.966321383519));
#211522=CARTESIAN_POINT('Ctrl Pts',(-3.46774738285662,5.81346624122508,
112.974372705358));
#211523=CARTESIAN_POINT('Ctrl Pts',(-3.61266492581227,5.72197003957604,
112.982424027196));
#211524=CARTESIAN_POINT('Ctrl Pts',(-3.75746370525339,5.63054882132965,
112.990468750777));
#211525=CARTESIAN_POINT('Ctrl Pts',(-3.89893399048018,5.5335366328246,112.998513474358));
#211526=CARTESIAN_POINT('Ctrl Pts',(-4.03661001760902,5.43121243975399,
113.006558197939));
#211527=CARTESIAN_POINT('Ctrl Pts',(-4.17420335316732,5.32894970508254,
113.014598089664));
#211528=CARTESIAN_POINT('Ctrl Pts',(-4.30800666856627,5.22138153917995,
113.022637981388));
#211529=CARTESIAN_POINT('Ctrl Pts',(-4.43758257510572,5.10883057941034,
113.030677873112));
#211530=CARTESIAN_POINT('Ctrl Pts',(-4.56994860590984,4.99385608912296,
113.038890885732));
#211531=CARTESIAN_POINT('Ctrl Pts',(-4.69790277016815,4.87368199700927,
113.047103898352));
#211532=CARTESIAN_POINT('Ctrl Pts',(-4.8210135068851,4.74869642811914,113.055316910972));
#211533=CARTESIAN_POINT('Ctrl Pts',(-4.94148716144998,4.62638810105029,
113.063353997515));
#211534=CARTESIAN_POINT('Ctrl Pts',(-5.05732251945938,4.49947262282481,
113.071391084057));
#211535=CARTESIAN_POINT('Ctrl Pts',(-5.16815199826767,4.36835139644259,
113.0794281706));
#211536=CARTESIAN_POINT('Ctrl Pts',(-5.27899208397301,4.23721762114862,
113.087466026329));
#211537=CARTESIAN_POINT('Ctrl Pts',(-5.38482509524323,4.10187758150911,
113.095503882058));
#211538=CARTESIAN_POINT('Ctrl Pts',(-5.48532360952023,3.96276594045623,
113.103541737787));
#211539=CARTESIAN_POINT('Ctrl Pts',(-5.58585165408385,3.82361342311118,
113.111581955344));
#211540=CARTESIAN_POINT('Ctrl Pts',(-5.68104186297204,3.68068740113054,
113.119622172901));
#211541=CARTESIAN_POINT('Ctrl Pts',(-5.77061012048762,3.53445156103828,
113.127662390458));
#211542=CARTESIAN_POINT('Ctrl Pts',(-5.86356232415993,3.38269083721172,
113.136006372586));
#211543=CARTESIAN_POINT('Ctrl Pts',(-5.95045924468415,3.22736569570295,
113.144350354714));
#211544=CARTESIAN_POINT('Ctrl Pts',(-6.03103612747287,3.06902137971,113.152694336841));
#211545=CARTESIAN_POINT('Ctrl Pts',(-6.10881476059825,2.9161759973266,113.160748551677));
#211546=CARTESIAN_POINT('Ctrl Pts',(-6.18070486389119,2.76051798480914,
113.168802766512));
#211547=CARTESIAN_POINT('Ctrl Pts',(-6.24651805942797,2.60255665322394,
113.176856981347));
#211548=CARTESIAN_POINT('Ctrl Pts',(-6.31238050525878,2.44447711370245,
113.18491722343));
#211549=CARTESIAN_POINT('Ctrl Pts',(-6.37215685897739,2.28409117076968,
113.192977465513));
#211550=CARTESIAN_POINT('Ctrl Pts',(-6.42570884426063,2.12192244174727,
113.201037707596));
#211551=CARTESIAN_POINT('Ctrl Pts',(-6.47933569889267,1.95952698971783,
113.20910921845));
#211552=CARTESIAN_POINT('Ctrl Pts',(-6.52672072029348,1.79534413427019,
113.217180729304));
#211553=CARTESIAN_POINT('Ctrl Pts',(-6.56777671654455,1.62990735982612,
113.225252240159));
#211554=CARTESIAN_POINT('Ctrl Pts',(-6.5720798136106,1.61256785856608,113.22609821877));
#211555=CARTESIAN_POINT('Ctrl Pts',(-6.57631343191616,1.59521458664683,
113.22694419738));
#211556=CARTESIAN_POINT('Ctrl Pts',(-6.58047750411495,1.57784816057727,
113.227790175991));
#211557=CARTESIAN_POINT('Ctrl Pts',(-6.64202959311043,1.32114276452838,
113.240295182691));
#211558=CARTESIAN_POINT('Ctrl Pts',(-6.68855950918872,1.06082125580226,
113.252800189391));
#211559=CARTESIAN_POINT('Ctrl Pts',(-6.71974545345721,0.798317005168496,
113.26530519609));
#211560=CARTESIAN_POINT('Ctrl Pts',(-6.74888740619546,0.553017828087361,
113.27699059869));
#211561=CARTESIAN_POINT('Ctrl Pts',(-6.76463117401001,0.305811782513401,
113.28867600129));
#211562=CARTESIAN_POINT('Ctrl Pts',(-6.76675232742443,0.0578959350566465,
113.30036140389));
#211563=CARTESIAN_POINT('Ctrl Pts',(-6.76690110330271,0.040507330491761,
113.30118100799));
#211564=CARTESIAN_POINT('Ctrl Pts',(-6.76698287838215,0.0231152489778019,
113.30200061209));
#211565=CARTESIAN_POINT('Ctrl Pts',(-6.76699758240933,0.00572011068525729,
113.30282021619));
#211566=CARTESIAN_POINT('Ctrl Pts',(-6.76699758240985,0.00572011007081819,
113.302820216219));
#211567=CARTESIAN_POINT('Ctrl Pts',(-6.76714174656369,-0.164828789928473,
113.310855942944));
#211568=CARTESIAN_POINT('Ctrl Pts',(-6.76083424723953,-0.335598683486344,
113.318891669669));
#211569=CARTESIAN_POINT('Ctrl Pts',(-6.7480517151586,-0.506050441700267,
113.326927396394));
#211570=CARTESIAN_POINT('Ctrl Pts',(-6.73527935231447,-0.676366595772572,
113.334956730238));
#211571=CARTESIAN_POINT('Ctrl Pts',(-6.7160422371159,-0.846364745793231,
113.342986064082));
#211572=CARTESIAN_POINT('Ctrl Pts',(-6.69036905850181,-1.01550522452696,
113.351015397926));
#211573=CARTESIAN_POINT('Ctrl Pts',(-6.66443215942169,-1.18638315098963,
113.35912721083));
#211574=CARTESIAN_POINT('Ctrl Pts',(-6.63192622110713,-1.35638529931067,
113.367239023735));
#211575=CARTESIAN_POINT('Ctrl Pts',(-6.59293474517086,-1.52495916204957,
113.37535083664));
#211576=CARTESIAN_POINT('Ctrl Pts',(-6.55437159343104,-1.69168122865691,
113.383373540691));
#211577=CARTESIAN_POINT('Ctrl Pts',(-6.50946476917128,-1.85700585832273,
113.391396244741));
#211578=CARTESIAN_POINT('Ctrl Pts',(-6.45834656910374,-2.02040802645059,
113.399418948792));
#211579=CARTESIAN_POINT('Ctrl Pts',(-6.40723257841055,-2.18379673907934,
113.407440992206));
#211580=CARTESIAN_POINT('Ctrl Pts',(-6.34990834169189,-2.34526294668844,
113.415463035619));
#211581=CARTESIAN_POINT('Ctrl Pts',(-6.28655606611847,-2.50429667322965,
113.423485079033));
#211582=CARTESIAN_POINT('Ctrl Pts',(-6.22319633607003,-2.66334911279943,
113.431508066377));
#211583=CARTESIAN_POINT('Ctrl Pts',(-6.15380729516008,-2.81996815297206,
113.439531053721));
#211584=CARTESIAN_POINT('Ctrl Pts',(-6.07861927087379,-2.97366386125968,
113.447554041065));
#211585=CARTESIAN_POINT('Ctrl Pts',(-6.0019716094381,-3.13034328893145,
113.455732779946));
#211586=CARTESIAN_POINT('Ctrl Pts',(-5.91929767150677,-3.28398434690864,
113.463911518828));
#211587=CARTESIAN_POINT('Ctrl Pts',(-5.83089016333719,-3.43409506320043,
113.472090257709));
#211588=CARTESIAN_POINT('Ctrl Pts',(-5.74405442827701,-3.5815370017811,
113.48012358901));
#211589=CARTESIAN_POINT('Ctrl Pts',(-5.65168754281564,-3.72557279410439,
113.488156920311));
#211590=CARTESIAN_POINT('Ctrl Pts',(-5.55410990549534,-3.8657666972644,
113.496190251612));
#211591=CARTESIAN_POINT('Ctrl Pts',(-5.45388295727248,-4.00976697703195,
113.504441694283));
#211592=CARTESIAN_POINT('Ctrl Pts',(-5.348158559119,-4.14971344832943,113.512693136955));
#211593=CARTESIAN_POINT('Ctrl Pts',(-5.23732671965755,-4.28517185554572,
113.520944579626));
#211594=CARTESIAN_POINT('Ctrl Pts',(-5.12649488019601,-4.42063026276211,
113.529196022298));
#211595=CARTESIAN_POINT('Ctrl Pts',(-5.01055592820781,-4.55160033312452,
113.537447464969));
#211596=CARTESIAN_POINT('Ctrl Pts',(-4.88993859368385,-4.67769062144999,
113.545698907641));
#211597=CARTESIAN_POINT('Ctrl Pts',(-4.75931541378705,-4.81424076559122,
113.554634851091));
#211598=CARTESIAN_POINT('Ctrl Pts',(-4.62288621833232,-4.94540347657821,
113.563570794542));
#211599=CARTESIAN_POINT('Ctrl Pts',(-4.48109968228315,-5.07070356434311,
113.572506737993));
#211600=CARTESIAN_POINT('Ctrl Pts',(-4.33952628900438,-5.19581529284215,
113.581429248351));
#211601=CARTESIAN_POINT('Ctrl Pts',(-4.19261181767249,-5.31508181264485,
113.590351758708));
#211602=CARTESIAN_POINT('Ctrl Pts',(-4.04084126081295,-5.4280651161267,
113.599274269066));
#211603=CARTESIAN_POINT('Ctrl Pts',(-3.88944258891635,-5.54077157545316,
113.608174916504));
#211604=CARTESIAN_POINT('Ctrl Pts',(-3.73321178635691,-5.64722539189653,
113.617075563942));
#211605=CARTESIAN_POINT('Ctrl Pts',(-3.57266581165222,-5.74702949342105,
113.625976211381));
#211606=CARTESIAN_POINT('Ctrl Pts',(-3.41236794093672,-5.84667936002457,
113.634863103967));
#211607=CARTESIAN_POINT('Ctrl Pts',(-3.2477684183083,-5.93969987462143,
113.643749996553));
#211608=CARTESIAN_POINT('Ctrl Pts',(-3.07941443254387,-6.02573611707653,
113.652636889139));
#211609=CARTESIAN_POINT('Ctrl Pts',(-2.91149317936791,-6.11155121427196,
113.661500939094));
#211610=CARTESIAN_POINT('Ctrl Pts',(-2.73983694893589,-6.19041774452342,
113.670364989049));
#211611=CARTESIAN_POINT('Ctrl Pts',(-2.56501817625615,-6.26202609029023,
113.679229039004));
#211612=CARTESIAN_POINT('Ctrl Pts',(-2.39787736637741,-6.33048942933603,
113.687703783824));
#211613=CARTESIAN_POINT('Ctrl Pts',(-2.227846061442,-6.3923182941236,113.696178528645));
#211614=CARTESIAN_POINT('Ctrl Pts',(-2.05544710604081,-6.44728052703374,
113.704653273465));
#211615=CARTESIAN_POINT('Ctrl Pts',(-1.88845585113592,-6.50051873967071,
113.712862187894));
#211616=CARTESIAN_POINT('Ctrl Pts',(-1.71940382579393,-6.54726209571515,
113.721071102323));
#211617=CARTESIAN_POINT('Ctrl Pts',(-1.54883675561019,-6.58736621909477,
113.729280016752));
#211618=CARTESIAN_POINT('Ctrl Pts',(-1.37822913397182,-6.62747987702604,
113.737490882809));
#211619=CARTESIAN_POINT('Ctrl Pts',(-1.20610609652001,-6.6609510760869,
113.745701748866));
#211620=CARTESIAN_POINT('Ctrl Pts',(-1.03302411205503,-6.68768645974921,
113.753912614923));
#211621=CARTESIAN_POINT('Ctrl Pts',(-0.859870125636911,-6.71443296530759,
113.762126896693));
#211622=CARTESIAN_POINT('Ctrl Pts',(-0.685756749089357,-6.73443801879406,
113.770341178463));
#211623=CARTESIAN_POINT('Ctrl Pts',(-0.511246217920508,-6.7476600614333,
113.778555460233));
#211624=CARTESIAN_POINT('Ctrl Pts',(-0.336539261373363,-6.76089698652525,
113.786778987825));
#211625=CARTESIAN_POINT('Ctrl Pts',(-0.161434612541626,-6.76733562461684,
113.795002515417));
#211626=CARTESIAN_POINT('Ctrl Pts',(0.0135038579698645,-6.76698652620352,
113.80322604301));
#211627=CARTESIAN_POINT('Ctrl Pts',(0.188554457236126,-6.76663720403169,
113.811454841563));
#211628=CARTESIAN_POINT('Ctrl Pts',(0.363438310991927,-6.75949148705857,
113.819683640117));
#211629=CARTESIAN_POINT('Ctrl Pts',(0.537596071852023,-6.74561186724594,
113.827912438671));
#211630=CARTESIAN_POINT('Ctrl Pts',(0.711993546933154,-6.73171314324734,
113.836152563507));
#211631=CARTESIAN_POINT('Ctrl Pts',(0.885662580337927,-6.71106204499546,
113.844392688344));
#211632=CARTESIAN_POINT('Ctrl Pts',(1.05805241666431,-6.6837724440312,113.85263281318));
#211633=CARTESIAN_POINT('Ctrl Pts',(1.13458638972954,-6.67165698740298,
113.85629108855));
#211634=CARTESIAN_POINT('Ctrl Pts',(1.21086840919001,-6.65823375249968,
113.85994936392));
#211635=CARTESIAN_POINT('Ctrl Pts',(1.28685124095268,-6.64351585259331,
113.86360763929));
#211636=CARTESIAN_POINT('Ctrl Pts',(1.46231771828376,-6.60952793729226,
113.872055662053));
#211637=CARTESIAN_POINT('Ctrl Pts',(1.63658920769549,-6.56855471427455,
113.880503684816));
#211638=CARTESIAN_POINT('Ctrl Pts',(1.80908820664905,-6.52069696125831,
113.888951707578));
#211639=CARTESIAN_POINT('Ctrl Pts',(1.98142924311719,-6.47288303301589,
113.897391994234));
#211640=CARTESIAN_POINT('Ctrl Pts',(2.15200070466085,-6.41819722998244,
113.90583228089));
#211641=CARTESIAN_POINT('Ctrl Pts',(2.32023572801532,-6.35679126340021,
113.914272567546));
#211642=CARTESIAN_POINT('Ctrl Pts',(2.48834259237072,-6.2954320749921,113.922706424513));
#211643=CARTESIAN_POINT('Ctrl Pts',(2.65411625450859,-6.22736304237392,
113.931140281481));
#211644=CARTESIAN_POINT('Ctrl Pts',(2.81700507633562,-6.15278566178762,
113.939574138449));
#211645=CARTESIAN_POINT('Ctrl Pts',(2.97979485330259,-6.07825362812041,
113.948002867194));
#211646=CARTESIAN_POINT('Ctrl Pts',(3.13970298473907,-5.99722127500127,
113.956431595939));
#211647=CARTESIAN_POINT('Ctrl Pts',(3.29619751843952,-5.90993831773507,
113.964860324684));
#211648=CARTESIAN_POINT('Ctrl Pts',(3.45262092709158,-5.8226950296152,113.973285222665));
#211649=CARTESIAN_POINT('Ctrl Pts',(3.6056335408127,-5.72920696416549,113.981710120645));
#211650=CARTESIAN_POINT('Ctrl Pts',(3.75472739085711,-5.62977008592246,
113.990135018625));
#211651=CARTESIAN_POINT('Ctrl Pts',(3.90378823128062,-5.53035522316601,
113.998558051319));
#211652=CARTESIAN_POINT('Ctrl Pts',(4.04893175922937,-5.42499435629292,
114.006981084014));
#211653=CARTESIAN_POINT('Ctrl Pts',(4.1896779737907,-5.31402742521461,114.015404116708));
#211654=CARTESIAN_POINT('Ctrl Pts',(4.3304082630777,-5.20307304991853,114.023826196345));
#211655=CARTESIAN_POINT('Ctrl Pts',(4.46674196904989,-5.08651408138716,
114.032248275983));
#211656=CARTESIAN_POINT('Ctrl Pts',(4.59823100014777,-4.96473168149902,
114.040670355621));
#211657=CARTESIAN_POINT('Ctrl Pts',(4.7297235082977,-4.84294606123773,114.049092657969));
#211658=CARTESIAN_POINT('Ctrl Pts',(4.85637084175589,-4.7159369611089,114.057514960317));
#211659=CARTESIAN_POINT('Ctrl Pts',(4.97776044134983,-4.58412368817997,
114.065937262665));
#211660=CARTESIAN_POINT('Ctrl Pts',(5.09917019699575,-4.45228852840745,
114.074360963489));
#211661=CARTESIAN_POINT('Ctrl Pts',(5.21532025281299,-4.31564785112412,
114.082784664313));
#211662=CARTESIAN_POINT('Ctrl Pts',(5.32583690300029,-4.17465570827587,
114.091208365136));
#211663=CARTESIAN_POINT('Ctrl Pts',(5.43642834081537,-4.03356815475528,
114.099637766355));
#211664=CARTESIAN_POINT('Ctrl Pts',(5.54137854941775,-3.88812351421506,
114.108067167574));
#211665=CARTESIAN_POINT('Ctrl Pts',(5.64035530496227,-3.73880743470214,
114.116496568793));
#211666=CARTESIAN_POINT('Ctrl Pts',(5.73936737527575,-3.58943807941935,
114.124928977611));
#211667=CARTESIAN_POINT('Ctrl Pts',(5.83240156368424,-3.43619481220138,
114.133361386429));
#211668=CARTESIAN_POINT('Ctrl Pts',(5.9191702635985,-3.27959027784436,114.141793795246));
#211669=CARTESIAN_POINT('Ctrl Pts',(6.00601924443839,-3.12284084841588,
114.150234005974));
#211670=CARTESIAN_POINT('Ctrl Pts',(6.08659099809977,-2.9627242330044,114.158674216701));
#211671=CARTESIAN_POINT('Ctrl Pts',(6.1606444630324,-2.79977656253284,114.167114427429));
#211672=CARTESIAN_POINT('Ctrl Pts',(6.2027648102288,-2.70709470812738,114.171915075266));
#211673=CARTESIAN_POINT('Ctrl Pts',(6.2427772754782,-2.61349734538853,114.176715723103));
#211674=CARTESIAN_POINT('Ctrl Pts',(6.2806445619527,-2.51908572430833,114.18151637094));
#211675=CARTESIAN_POINT('Ctrl Pts',(6.34485025489866,-2.35900656052433,
114.189656085973));
#211676=CARTESIAN_POINT('Ctrl Pts',(6.40301400142117,-2.19626633670184,
114.197795801006));
#211677=CARTESIAN_POINT('Ctrl Pts',(6.45490828774196,-2.03136604206138,
114.205935516039));
#211678=CARTESIAN_POINT('Ctrl Pts',(6.50675718763125,-1.86660996822941,
114.214068112126));
#211679=CARTESIAN_POINT('Ctrl Pts',(6.55234743248018,-1.69969793091769,
114.222200708213));
#211680=CARTESIAN_POINT('Ctrl Pts',(6.59149948379578,-1.53115105561796,
114.2303333043));
#211681=CARTESIAN_POINT('Ctrl Pts',(6.63062476866846,-1.36271940800526,
114.238460340507));
#211682=CARTESIAN_POINT('Ctrl Pts',(6.66332054063709,-1.19265550286258,
114.246587376715));
#211683=CARTESIAN_POINT('Ctrl Pts',(6.68945703502577,-1.0214957545405,114.254714412923));
#211684=CARTESIAN_POINT('Ctrl Pts',(6.71558103569723,-0.850417823674971,
114.262837564261));
#211685=CARTESIAN_POINT('Ctrl Pts',(6.73515194734242,-0.678245453996151,
114.270960715598));
#211686=CARTESIAN_POINT('Ctrl Pts',(6.74809107112088,-0.505525366187226,
114.279083866936));
#211687=CARTESIAN_POINT('Ctrl Pts',(6.76102655890939,-0.332853814006485,
114.287204735608));
#211688=CARTESIAN_POINT('Ctrl Pts',(6.76733394417353,-0.159635215186562,
114.295325604279));
#211689=CARTESIAN_POINT('Ctrl Pts',(6.76698637682862,0.0135785056552626,
114.303446472951));
#211690=CARTESIAN_POINT('Ctrl Pts',(6.76663879069985,0.18680158762972,114.311567780505));
#211691=CARTESIAN_POINT('Ctrl Pts',(6.75963553019068,0.360019424867068,
114.31968908806));
#211692=CARTESIAN_POINT('Ctrl Pts',(6.74600186880402,0.532679815736148,
114.327810395614));
#211693=CARTESIAN_POINT('Ctrl Pts',(6.73891734441633,0.622400156824949,
114.332030509331));
#211694=CARTESIAN_POINT('Ctrl Pts',(6.73004333439897,0.711970006935379,
114.336250623048));
#211695=CARTESIAN_POINT('Ctrl Pts',(6.7193889224893,0.801312366264337,114.340470736765));
#211696=CARTESIAN_POINT('Ctrl Pts',(6.69670614300686,0.99151836282981,114.349455175291));
#211697=CARTESIAN_POINT('Ctrl Pts',(6.66596217420908,1.1805986107691,114.358439613817));
#211698=CARTESIAN_POINT('Ctrl Pts',(6.62730282526317,1.36789848390105,114.367424052342));
#211699=CARTESIAN_POINT('Ctrl Pts',(6.58857675258871,1.55552162543339,114.376423997473));
#211700=CARTESIAN_POINT('Ctrl Pts',(6.5419080424759,1.74135801635826,114.385423942603));
#211701=CARTESIAN_POINT('Ctrl Pts',(6.4874928905115,1.92476621841792,114.394423887734));
#211702=CARTESIAN_POINT('Ctrl Pts',(6.43294950784435,2.10860662661483,114.403445041466));
#211703=CARTESIAN_POINT('Ctrl Pts',(6.37062322690239,2.29000716695555,114.412466195198));
#211704=CARTESIAN_POINT('Ctrl Pts',(6.30076006976931,2.46834186108826,114.42148734893));
#211705=CARTESIAN_POINT('Ctrl Pts',(6.23082582632298,2.64685801217841,114.430517681757));
#211706=CARTESIAN_POINT('Ctrl Pts',(6.15333947891796,2.82230186491228,114.439548014585));
#211707=CARTESIAN_POINT('Ctrl Pts',(6.06859465719012,2.99406878456785,114.448578347412));
#211708=CARTESIAN_POINT('Ctrl Pts',(5.98372969401841,3.16607921557095,114.457621482404));
#211709=CARTESIAN_POINT('Ctrl Pts',(5.8915857867474,3.33440207610212,114.466664617397));
#211710=CARTESIAN_POINT('Ctrl Pts',(5.79250295979664,3.49845658265858,114.47570775239));
#211711=CARTESIAN_POINT('Ctrl Pts',(5.70588174169629,3.64187801733197,114.48361353579));
#211712=CARTESIAN_POINT('Ctrl Pts',(5.61395799356018,3.7820375592553,114.491519319189));
#211713=CARTESIAN_POINT('Ctrl Pts',(5.51698592162353,3.91856546973607,114.499425102589));
#211714=CARTESIAN_POINT('Ctrl Pts',(5.41084110074195,4.06800778146459,114.508078707139));
#211715=CARTESIAN_POINT('Ctrl Pts',(5.29855289410897,4.21323019737577,114.516732311688));
#211716=CARTESIAN_POINT('Ctrl Pts',(5.18047536494763,4.35372989437457,114.525385916238));
#211717=CARTESIAN_POINT('Ctrl Pts',(5.0625069617822,4.49409974304853,114.534031523218));
#211718=CARTESIAN_POINT('Ctrl Pts',(4.93876010259894,4.62975534632004,114.542677130199));
#211719=CARTESIAN_POINT('Ctrl Pts',(4.8096303188304,4.76022533040059,114.551322737179));
#211720=CARTESIAN_POINT('Ctrl Pts',(4.68064926194655,4.89054504400355,114.559958386471));
#211721=CARTESIAN_POINT('Ctrl Pts',(4.54629786719942,5.01569084297337,114.568594035762));
#211722=CARTESIAN_POINT('Ctrl Pts',(4.40700993565848,5.13522661885603,114.577229685054));
#211723=CARTESIAN_POINT('Ctrl Pts',(4.26782239730844,5.25467623811453,114.585859110114));
#211724=CARTESIAN_POINT('Ctrl Pts',(4.12370564771509,5.3685237005485,114.594488535174));
#211725=CARTESIAN_POINT('Ctrl Pts',(3.97512911074323,5.47637083778315,114.603117960233));
#211726=CARTESIAN_POINT('Ctrl Pts',(3.82668177955634,5.58412418851351,114.611739880934));
#211727=CARTESIAN_POINT('Ctrl Pts',(3.67378264598822,5.6858874490197,114.620361801635));
#211728=CARTESIAN_POINT('Ctrl Pts',(3.51693309246344,5.78130354013138,114.628983722336));
#211729=CARTESIAN_POINT('Ctrl Pts',(3.38052851214159,5.8642823664752,114.636481795798));
#211730=CARTESIAN_POINT('Ctrl Pts',(3.24113685638985,5.94246140410373,114.64397986926));
#211731=CARTESIAN_POINT('Ctrl Pts',(3.09910619832145,6.01563211736934,114.651477942722));
#211732=CARTESIAN_POINT('Origin',(0.,0.,4.30282021618968));
#211733=CARTESIAN_POINT('',(3.09910619832145,6.01563211736934,117.045755263024));
#211734=CARTESIAN_POINT('',(3.09910619832134,6.0156321173694,116.651219418659));
#211735=CARTESIAN_POINT('',(3.09910619832133,6.0156321173694,4.30282021618968));
#211736=CARTESIAN_POINT('',(-6.76699999999965,-2.16894222160891E-6,115.697132037191));
#211737=CARTESIAN_POINT('Ctrl Pts',(-6.767,5.80635438534225E-12,115.69717978381));
#211738=CARTESIAN_POINT('Ctrl Pts',(-6.76700000000016,-0.18600724952103,
115.705929295621));
#211739=CARTESIAN_POINT('Ctrl Pts',(-6.75932637294552,-0.372014355744046,
115.714678807432));
#211740=CARTESIAN_POINT('Ctrl Pts',(-6.74400518264229,-0.557389537481599,
115.723428319244));
#211741=CARTESIAN_POINT('Ctrl Pts',(-6.72868405705149,-0.74276393624608,
115.732177794099));
#211742=CARTESIAN_POINT('Ctrl Pts',(-6.70571545645802,-0.927506130236736,
115.740927268955));
#211743=CARTESIAN_POINT('Ctrl Pts',(-6.6751773940489,-1.11098863989626,
115.749676743811));
#211744=CARTESIAN_POINT('Ctrl Pts',(-6.64463945808771,-1.29447038981592,
115.758426182438));
#211745=CARTESIAN_POINT('Ctrl Pts',(-6.60653217008427,-1.47669218313363,
115.767175621065));
#211746=CARTESIAN_POINT('Ctrl Pts',(-6.56098496092749,-1.65703510599,115.775925059692));
#211747=CARTESIAN_POINT('Ctrl Pts',(-6.51543793658372,-1.83737729708436,
115.784674462817));
#211748=CARTESIAN_POINT('Ctrl Pts',(-6.46245112167496,-2.01584035510685,
115.793423865942));
#211749=CARTESIAN_POINT('Ctrl Pts',(-6.40220448374329,-2.19181813760571,
115.802173269067));
#211750=CARTESIAN_POINT('Ctrl Pts',(-6.34195808526583,-2.36779522066931,
115.810922637417));
#211751=CARTESIAN_POINT('Ctrl Pts',(-6.27445201433187,-2.54128677683961,
115.819672005767));
#211752=CARTESIAN_POINT('Ctrl Pts',(-6.19991555071988,-2.71170355384615,
115.828421374117));
#211753=CARTESIAN_POINT('Ctrl Pts',(-6.1253793771679,-2.88211966767268,
115.837170708419));
#211754=CARTESIAN_POINT('Ctrl Pts',(-6.04381298052631,-3.04946076371564,
115.845920042721));
#211755=CARTESIAN_POINT('Ctrl Pts',(-5.95549339335957,-3.21315848374314,
115.854669377023));
#211756=CARTESIAN_POINT('Ctrl Pts',(-5.86717414255538,-3.37685558033268,
115.863418678003));
#211757=CARTESIAN_POINT('Ctrl Pts',(-5.77210188876731,-3.53690907646541,
115.872167978983));
#211758=CARTESIAN_POINT('Ctrl Pts',(-5.67059953347131,-3.69277536969079,
115.880917279963));
#211759=CARTESIAN_POINT('Ctrl Pts',(-5.56909755631526,-3.84864108224717,
115.889666548349));
#211760=CARTESIAN_POINT('Ctrl Pts',(-5.46116568197,-4.00031938297312,115.898415816734));
#211761=CARTESIAN_POINT('Ctrl Pts',(-5.34717048533761,-4.14729511859651,
115.907165085119));
#211762=CARTESIAN_POINT('Ctrl Pts',(-5.23317570391998,-4.29427031887719,
115.915914321636));
#211763=CARTESIAN_POINT('Ctrl Pts',(-5.1131178200368,-4.43654276189357,
115.924663558153));
#211764=CARTESIAN_POINT('Ctrl Pts',(-4.98740458984922,-4.57362924351668,
115.93341279467));
#211765=CARTESIAN_POINT('Ctrl Pts',(-4.86169180711923,-4.71071523720081,
115.942162000046));
#211766=CARTESIAN_POINT('Ctrl Pts',(-4.73032391204363,-4.84261509523051,
115.950911205421));
#211767=CARTESIAN_POINT('Ctrl Pts',(-4.59374707013802,-4.96888084538142,
115.959660410797));
#211768=CARTESIAN_POINT('Ctrl Pts',(-4.4571707030164,-5.09514615659294,
115.968409585757));
#211769=CARTESIAN_POINT('Ctrl Pts',(-4.31538563571227,-5.21577720459374,
115.977158760718));
#211770=CARTESIAN_POINT('Ctrl Pts',(-4.16887341029686,-5.33036429232748,
115.985907935678));
#211771=CARTESIAN_POINT('Ctrl Pts',(-4.022361682039,-5.44495099123472,115.99465708095));
#211772=CARTESIAN_POINT('Ctrl Pts',(-3.87112305348378,-5.55349359438453,
116.003406226222));
#211773=CARTESIAN_POINT('Ctrl Pts',(-3.71567117017992,-5.65562346298742,
116.012155371494));
#211774=CARTESIAN_POINT('Ctrl Pts',(-3.56021980146045,-5.75775299351505,
116.020904487804));
#211775=CARTESIAN_POINT('Ctrl Pts',(-3.40055544538569,-5.85346967463745,
116.029653604114));
#211776=CARTESIAN_POINT('Ctrl Pts',(-3.23722035987067,-5.94244842986785,
116.038402720425));
#211777=CARTESIAN_POINT('Ctrl Pts',(-3.07388580147382,-6.03142689794427,
116.047151808499));
#211778=CARTESIAN_POINT('Ctrl Pts',(-2.90688078896767,-6.11366734656692,
116.055900896574));
#211779=CARTESIAN_POINT('Ctrl Pts',(-2.73677250721546,-6.18889046952276,
116.064649984649));
#211780=CARTESIAN_POINT('Ctrl Pts',(-2.56666476031641,-6.26411335596263,
116.073399045215));
#211781=CARTESIAN_POINT('Ctrl Pts',(-2.39345402575306,-6.33231884500503,
116.082148105781));
#211782=CARTESIAN_POINT('Ctrl Pts',(-2.21772856065713,-6.39327529762685,
116.090897166347));
#211783=CARTESIAN_POINT('Ctrl Pts',(-2.04200363348598,-6.45423156365086,
116.099646200131));
#211784=CARTESIAN_POINT('Ctrl Pts',(-1.86376426189325,-6.50793874375646,
116.108395233915));
#211785=CARTESIAN_POINT('Ctrl Pts',(-1.68361577753161,-6.5542144390954,
116.117144267698));
#211786=CARTESIAN_POINT('Ctrl Pts',(-1.5034678296781,-6.60048999661866,
116.125893275426));
#211787=CARTESIAN_POINT('Ctrl Pts',(-1.32141105795,-6.6393340423771,116.134642283154));
#211788=CARTESIAN_POINT('Ctrl Pts',(-1.13806375487039,-6.67061465607558,
116.143391290882));
#211789=CARTESIAN_POINT('Ctrl Pts',(-0.95471698260385,-6.70189517921283,
116.15214027328));
#211790=CARTESIAN_POINT('Ctrl Pts',(-0.770079968903642,-6.72561226592209,
116.160889255679));
#211791=CARTESIAN_POINT('Ctrl Pts',(-0.584779765560425,-6.74168536983083,
116.169638238077));
#211792=CARTESIAN_POINT('Ctrl Pts',(-0.391489830653509,-6.7584515101384,
116.178764457087));
#211793=CARTESIAN_POINT('Ctrl Pts',(-0.197478578240578,-6.76689983031619,
116.187890676097));
#211794=CARTESIAN_POINT('Ctrl Pts',(-0.00346287645361174,-6.76699911397118,
116.197016895107));
#211795=CARTESIAN_POINT('Ctrl Pts',(0.184489834652479,-6.76709529501195,
116.205857919772));
#211796=CARTESIAN_POINT('Ctrl Pts',(0.372446404247931,-6.75935639738176,
116.214698944438));
#211797=CARTESIAN_POINT('Ctrl Pts',(0.559755019486866,-6.74380925873199,
116.223539969104));
#211798=CARTESIAN_POINT('Ctrl Pts',(0.745134705520392,-6.72842222659821,
116.232289947714));
#211799=CARTESIAN_POINT('Ctrl Pts',(0.929879431227269,-6.70538706057542,
116.241039926323));
#211800=CARTESIAN_POINT('Ctrl Pts',(1.11336163626704,-6.67478200894147,
116.249789904933));
#211801=CARTESIAN_POINT('Ctrl Pts',(1.29684196300602,-6.64417727061036,
116.25853979397));
#211802=CARTESIAN_POINT('Ctrl Pts',(1.47905951217398,-6.60600284890615,
116.267289683006));
#211803=CARTESIAN_POINT('Ctrl Pts',(1.65939532066977,-6.56038841607258,
116.276039572043));
#211804=CARTESIAN_POINT('Ctrl Pts',(1.83972934300695,-6.51477443503287,
116.284789374415));
#211805=CARTESIAN_POINT('Ctrl Pts',(2.01818138406158,-6.46172066062174,
116.293539176787));
#211806=CARTESIAN_POINT('Ctrl Pts',(2.19414528354094,-6.40140730423515,
116.302288979159));
#211807=CARTESIAN_POINT('Ctrl Pts',(2.37010749863894,-6.34109452518682,
116.311038697776));
#211808=CARTESIAN_POINT('Ctrl Pts',(2.54358134866354,-6.27352239616547,
116.319788416392));
#211809=CARTESIAN_POINT('Ctrl Pts',(2.71397759435451,-6.19892043966865,
116.328538135008));
#211810=CARTESIAN_POINT('Ctrl Pts',(2.88437226558026,-6.12431917249561,
116.337287772777));
#211811=CARTESIAN_POINT('Ctrl Pts',(3.05168912680864,-6.04268832278845,
116.346037410546));
#211812=CARTESIAN_POINT('Ctrl Pts',(3.2153598627377,-5.9543051612338,116.354787048314));
#211813=CARTESIAN_POINT('Ctrl Pts',(3.37902914072775,-5.8659227869748,116.363536608143));
#211814=CARTESIAN_POINT('Ctrl Pts',(3.53905210621522,-5.77078835741973,
116.372286167973));
#211815=CARTESIAN_POINT('Ctrl Pts',(3.69488522831663,-5.66922500431651,
116.381035727802));
#211816=CARTESIAN_POINT('Ctrl Pts',(3.85071701406922,-5.56766252217106,
116.389785212599));
#211817=CARTESIAN_POINT('Ctrl Pts',(4.00235878822401,-5.45967138329373,
116.398534697396));
#211818=CARTESIAN_POINT('Ctrl Pts',(4.14929549611337,-5.34561838199598,
116.407284182193));
#211819=CARTESIAN_POINT('Ctrl Pts',(4.29623099276106,-5.23156632087002,
116.416033594866));
#211820=CARTESIAN_POINT('Ctrl Pts',(4.43846127436049,-5.11145267304946,
116.424783007538));
#211821=CARTESIAN_POINT('Ctrl Pts',(4.57550326054468,-4.98568540049862,
116.433532420211));
#211822=CARTESIAN_POINT('Ctrl Pts',(4.71254416257812,-4.85991912290331,
116.442281763666));
#211823=CARTESIAN_POINT('Ctrl Pts',(4.84439664018797,-4.72849950385382,
116.451031107121));
#211824=CARTESIAN_POINT('Ctrl Pts',(4.97061286794785,-4.59187289861024,
116.459780450576));
#211825=CARTESIAN_POINT('Ctrl Pts',(5.09682813912717,-4.45524732884647,
116.468529727721));
#211826=CARTESIAN_POINT('Ctrl Pts',(5.21740705147865,-4.31341506235756,
116.477279004866));
#211827=CARTESIAN_POINT('Ctrl Pts',(5.33194007545716,-4.16685781275699,
116.486028282011));
#211828=CARTESIAN_POINT('Ctrl Pts',(5.44647226944499,-4.02030162521823,
116.494777495752));
#211829=CARTESIAN_POINT('Ctrl Pts',(5.55495848628121,-3.86902074887922,
116.503526709493));
#211830=CARTESIAN_POINT('Ctrl Pts',(5.65703027291791,-3.71352898080658,
116.512275923234));
#211831=CARTESIAN_POINT('Ctrl Pts',(5.75910135376999,-3.55803828789586,
116.521025076478));
#211832=CARTESIAN_POINT('Ctrl Pts',(5.85475793592752,-3.39833700106712,
116.529774229722));
#211833=CARTESIAN_POINT('Ctrl Pts',(5.94367514427397,-3.23496750823556,
116.538523382966));
#211834=CARTESIAN_POINT('Ctrl Pts',(6.03259176732643,-3.07159909077719,
116.547272478619));
#211835=CARTESIAN_POINT('Ctrl Pts',(6.11476896835931,-2.9045627673142,116.556021574272));
#211836=CARTESIAN_POINT('Ctrl Pts',(6.18992765547897,-2.73442583003026,
116.564770669925));
#211837=CARTESIAN_POINT('Ctrl Pts',(6.26508587283062,-2.56428995616152,
116.573519710893));
#211838=CARTESIAN_POINT('Ctrl Pts',(6.33322554827165,-2.39105376935188,
116.582268751861));
#211839=CARTESIAN_POINT('Ctrl Pts',(6.39411526733033,-2.21530561054071,
116.591017792829));
#211840=CARTESIAN_POINT('Ctrl Pts',(6.45500462602851,-2.03955849185086,
116.599766782018));
#211841=CARTESIAN_POINT('Ctrl Pts',(6.50864402040745,-1.86129970164529,
116.608515771207));
#211842=CARTESIAN_POINT('Ctrl Pts',(6.55485128368606,-1.68113463136039,
116.617264760396));
#211843=CARTESIAN_POINT('Ctrl Pts',(6.60199809554329,-1.49730620116858,
116.626191645867));
#211844=CARTESIAN_POINT('Ctrl Pts',(6.64140720707874,-1.31149343245696,
116.635118531339));
#211845=CARTESIAN_POINT('Ctrl Pts',(6.67293928722883,-1.12435326697532,
116.64404541681));
#211846=CARTESIAN_POINT('Ctrl Pts',(6.70384625876255,-0.940923067006682,
116.652795330988));
#211847=CARTESIAN_POINT('Ctrl Pts',(6.72718554579795,-0.756217899521783,
116.661545245165));
#211848=CARTESIAN_POINT('Ctrl Pts',(6.74287786815327,-0.570865181254639,
116.670295159343));
#211849=CARTESIAN_POINT('Ctrl Pts',(6.75856988190844,-0.385516108074159,
116.679044901447));
#211850=CARTESIAN_POINT('Ctrl Pts',(6.76661520773402,-0.199519795226629,
116.687794643552));
#211851=CARTESIAN_POINT('Ctrl Pts',(6.76698651789579,-0.0135080204559997,
116.696544385656));
#211852=CARTESIAN_POINT('Ctrl Pts',(6.76735782124904,0.172500343512539,
116.705293967321));
#211853=CARTESIAN_POINT('Ctrl Pts',(6.76005538995186,0.35852388221043,116.714043548986));
#211854=CARTESIAN_POINT('Ctrl Pts',(6.74510402742366,0.543930748563817,
116.722793130651));
#211855=CARTESIAN_POINT('Ctrl Pts',(6.73015291918037,0.729334461614674,
116.731542563508));
#211856=CARTESIAN_POINT('Ctrl Pts',(6.70755316306602,0.914121237634118,
116.740291996364));
#211857=CARTESIAN_POINT('Ctrl Pts',(6.67738151874583,1.09766345166066,116.749041429221));
#211858=CARTESIAN_POINT('Ctrl Pts',(6.6472103474758,1.28120278799608,116.757790724899));
#211859=CARTESIAN_POINT('Ctrl Pts',(6.60946757205154,1.46349731860273,116.766540020576));
#211860=CARTESIAN_POINT('Ctrl Pts',(6.56428138111537,1.64392790278107,116.775289316254));
#211861=CARTESIAN_POINT('Ctrl Pts',(6.51909583859866,1.82435589778997,116.784038486379));
#211862=CARTESIAN_POINT('Ctrl Pts',(6.46646716392894,2.00291972192203,116.792787656505));
#211863=CARTESIAN_POINT('Ctrl Pts',(6.40657409872906,2.17901292274598,116.80153682663));
#211864=CARTESIAN_POINT('Ctrl Pts',(6.34668181342101,2.35510383058911,116.810285882829));
#211865=CARTESIAN_POINT('Ctrl Pts',(6.27952541914077,2.52872390822512,116.819034939029));
#211866=CARTESIAN_POINT('Ctrl Pts',(6.20533299175547,2.69928350890216,116.827783995228));
#211867=CARTESIAN_POINT('Ctrl Pts',(6.12831602991577,2.87633637965564,116.836866131386));
#211868=CARTESIAN_POINT('Ctrl Pts',(6.04371690605295,3.05009086601413,116.845948267544));
#211869=CARTESIAN_POINT('Ctrl Pts',(5.95184520316652,3.21991112882695,116.855030403702));
#211870=CARTESIAN_POINT('Ctrl Pts',(5.86333549509295,3.38351691182981,116.863780184046));
#211871=CARTESIAN_POINT('Ctrl Pts',(5.76807618099388,3.54347103711972,116.872529964389));
#211872=CARTESIAN_POINT('Ctrl Pts',(5.66639083309035,3.69923018027666,116.881279744733));
#211873=CARTESIAN_POINT('Ctrl Pts',(5.56470914082217,3.85498372382026,116.890029210518));
#211874=CARTESIAN_POINT('Ctrl Pts',(5.45660203372081,4.0065423470198,116.898778676303));
#211875=CARTESIAN_POINT('Ctrl Pts',(5.34243669839227,4.15339127986656,116.907528142088));
#211876=CARTESIAN_POINT('Ctrl Pts',(5.22827486050597,4.30023571401274,116.916277339834));
#211877=CARTESIAN_POINT('Ctrl Pts',(5.1080553416711,4.44237052028471,116.92502653758));
#211878=CARTESIAN_POINT('Ctrl Pts',(4.98218644339944,4.57931296628729,116.933775735326));
#211879=CARTESIAN_POINT('Ctrl Pts',(4.85632073219594,4.71625194483352,116.942524711537));
#211880=CARTESIAN_POINT('Ctrl Pts',(4.72480612170342,4.84799861524485,116.951273687749));
#211881=CARTESIAN_POINT('Ctrl Pts',(4.58808925235352,4.97410554898447,116.960022663961));
#211882=CARTESIAN_POINT('Ctrl Pts',(4.45136349474093,5.10022068121167,116.968772208962));
#211883=CARTESIAN_POINT('Ctrl Pts',(4.30943501210129,5.22069514871793,116.977521753964));
#211884=CARTESIAN_POINT('Ctrl Pts',(4.16278587431835,5.33511975166215,116.986271298966));
#211885=CARTESIAN_POINT('Ctrl Pts',(4.01614535740487,5.44953762807814,116.99502032962));
#211886=CARTESIAN_POINT('Ctrl Pts',(3.86478496657947,5.55790617532767,117.003769360273));
#211887=CARTESIAN_POINT('Ctrl Pts',(3.70921874747204,5.65985735539351,117.012518390927));
#211888=CARTESIAN_POINT('Ctrl Pts',(3.55365041605914,5.76180991977038,117.021267540377));
#211889=CARTESIAN_POINT('Ctrl Pts',(3.3938763817454,5.85734478552803,117.030016689826));
#211890=CARTESIAN_POINT('Ctrl Pts',(3.23043927904562,5.9461374912122,117.038765839276));
#211891=CARTESIAN_POINT('Ctrl Pts',(3.18691767070448,5.96978206944138,117.041095647192));
#211892=CARTESIAN_POINT('Ctrl Pts',(3.14313645919642,5.99294880633419,117.043425455108));
#211893=CARTESIAN_POINT('Ctrl Pts',(3.09910619832145,6.01563211736934,117.045755263024));
#211894=CARTESIAN_POINT('Ctrl Pts',(3.09910619832125,6.01563211736945,115.045544419485));
#211895=CARTESIAN_POINT('Ctrl Pts',(2.9438845807917,6.09559848958332,115.053756299016));
#211896=CARTESIAN_POINT('Ctrl Pts',(2.78568313497432,6.1694928599194,115.061968178546));
#211897=CARTESIAN_POINT('Ctrl Pts',(2.62502327036983,6.23711005434543,115.070180058077));
#211898=CARTESIAN_POINT('Ctrl Pts',(2.4641528064675,6.30481588406133,115.078402702064));
#211899=CARTESIAN_POINT('Ctrl Pts',(2.30081782092016,6.36622797282393,115.08662534605));
#211900=CARTESIAN_POINT('Ctrl Pts',(2.13555632712065,6.42119055734176,115.094847990037));
#211901=CARTESIAN_POINT('Ctrl Pts',(2.03021870881675,6.45622368947572,115.100089100436));
#211902=CARTESIAN_POINT('Ctrl Pts',(1.92409866911816,6.48863754529247,115.105330210835));
#211903=CARTESIAN_POINT('Ctrl Pts',(1.81733761904495,6.5184026400955,115.110571321234));
#211904=CARTESIAN_POINT('Ctrl Pts',(1.63531307967276,6.56915127611188,115.119507264685));
#211905=CARTESIAN_POINT('Ctrl Pts',(1.4510457212125,6.61230359623252,115.128443208136));
#211906=CARTESIAN_POINT('Ctrl Pts',(1.26516391868083,6.64767999070865,115.137379151587));
#211907=CARTESIAN_POINT('Ctrl Pts',(1.0795615458007,6.68300320508084,115.146301661944));
#211908=CARTESIAN_POINT('Ctrl Pts',(0.8923498244926,6.71057376976984,115.155224172302));
#211909=CARTESIAN_POINT('Ctrl Pts',(0.704169381055813,6.73026258646596,
115.164146682659));
#211910=CARTESIAN_POINT('Ctrl Pts',(0.516450038102957,6.7499031594512,115.173047330098));
#211911=CARTESIAN_POINT('Ctrl Pts',(0.327766966782434,6.76170050240035,
115.181947977536));
#211912=CARTESIAN_POINT('Ctrl Pts',(0.138767386962045,6.76557703468934,
115.190848624974));
#211913=CARTESIAN_POINT('Ctrl Pts',(-0.0499401173342233,6.76944757627611,
115.19973551756));
#211914=CARTESIAN_POINT('Ctrl Pts',(-0.238962897593013,6.76542171879273,
115.208622410147));
#211915=CARTESIAN_POINT('Ctrl Pts',(-0.427649253809822,6.75347355926681,
115.217509302733));
#211916=CARTESIAN_POINT('Ctrl Pts',(-0.615850615656471,6.741556110971,115.226373352688));
#211917=CARTESIAN_POINT('Ctrl Pts',(-0.803717022064636,6.72175701040347,
115.235237402643));
#211918=CARTESIAN_POINT('Ctrl Pts',(-0.990598186963022,6.69410219760541,
115.244101452598));
#211919=CARTESIAN_POINT('Ctrl Pts',(-1.16927161415724,6.66766197189443,
115.252576197418));
#211920=CARTESIAN_POINT('Ctrl Pts',(-1.34704421969019,6.63404123570768,
115.261050942239));
#211921=CARTESIAN_POINT('Ctrl Pts',(-1.52334789899765,6.59330722616651,
115.269525687059));
#211922=CARTESIAN_POINT('Ctrl Pts',(-1.69412139691798,6.55385093506134,
115.277734601488));
#211923=CARTESIAN_POINT('Ctrl Pts',(-1.86335184044806,6.50775770790848,
115.285943515917));
#211924=CARTESIAN_POINT('Ctrl Pts',(-2.03049625529198,6.45518194609922,
115.294152430346));
#211925=CARTESIAN_POINT('Ctrl Pts',(-2.19768040787136,6.40259368466969,
115.302363296403));
#211926=CARTESIAN_POINT('Ctrl Pts',(-2.36277720402664,6.34351992494846,
115.31057416246));
#211927=CARTESIAN_POINT('Ctrl Pts',(-2.52526047293741,6.27816442472001,
115.318785028517));
#211928=CARTESIAN_POINT('Ctrl Pts',(-2.68781133474426,6.2127817366613,115.326999310287));
#211929=CARTESIAN_POINT('Ctrl Pts',(-2.84774617323817,6.14111223482421,
115.335213592057));
#211930=CARTESIAN_POINT('Ctrl Pts',(-3.00456029768648,6.06340716244309,
115.343427873826));
#211931=CARTESIAN_POINT('Ctrl Pts',(-3.16155092881134,5.98561462686868,
115.351651401419));
#211932=CARTESIAN_POINT('Ctrl Pts',(-3.3154135108691,5.9017731100307,115.359874929011));
#211933=CARTESIAN_POINT('Ctrl Pts',(-3.46566854508051,5.81217949960594,
115.368098456604));
#211934=CARTESIAN_POINT('Ctrl Pts',(-3.61601988692384,5.72252846316214,
115.376327255157));
#211935=CARTESIAN_POINT('Ctrl Pts',(-3.76275877374925,5.62711817719222,
115.384556053711));
#211936=CARTESIAN_POINT('Ctrl Pts',(-3.90543610874289,5.52628788614267,
115.392784852265));
#211937=CARTESIAN_POINT('Ctrl Pts',(-4.04830982767065,5.42531881026625,
115.401024977101));
#211938=CARTESIAN_POINT('Ctrl Pts',(-4.18711054668306,5.31891504424023,
115.409265101938));
#211939=CARTESIAN_POINT('Ctrl Pts',(-4.32142278294332,5.2074556292933,115.417505226774));
#211940=CARTESIAN_POINT('Ctrl Pts',(-4.38105187298164,5.157972248817,115.421163502144));
#211941=CARTESIAN_POINT('Ctrl Pts',(-4.43979677683306,5.10749288670311,
115.424821777514));
#211942=CARTESIAN_POINT('Ctrl Pts',(-4.49762357029527,5.05605292890852,
115.428480052884));
#211943=CARTESIAN_POINT('Ctrl Pts',(-4.62926406240587,4.93895182485625,
115.436807977383));
#211944=CARTESIAN_POINT('Ctrl Pts',(-4.75646792189858,4.81658222905124,
115.445135901882));
#211945=CARTESIAN_POINT('Ctrl Pts',(-4.87879671095418,4.6893103600831,115.453463826381));
#211946=CARTESIAN_POINT('Ctrl Pts',(-5.00100731009477,4.56216145686564,
115.461783704723));
#211947=CARTESIAN_POINT('Ctrl Pts',(-5.11835198390155,4.43011996680556,
115.470103583065));
#211948=CARTESIAN_POINT('Ctrl Pts',(-5.23042689719935,4.29359097645008,
115.478423461407));
#211949=CARTESIAN_POINT('Ctrl Pts',(-5.34241403046563,4.15716891920502,
115.4867368234));
#211950=CARTESIAN_POINT('Ctrl Pts',(-5.44913940828953,4.0162666332726,115.495050185394));
#211951=CARTESIAN_POINT('Ctrl Pts',(-5.5502373195323,3.87132466952476,115.503363547387));
#211952=CARTESIAN_POINT('Ctrl Pts',(-5.65127056400372,3.72647541717632,
115.51167159178));
#211953=CARTESIAN_POINT('Ctrl Pts',(-5.74668331921865,3.57759192253999,
115.519979636173));
#211954=CARTESIAN_POINT('Ctrl Pts',(-5.83615121480684,3.4251464199226,115.528287680566));
#211955=CARTESIAN_POINT('Ctrl Pts',(-5.92558733207976,3.27275506478697,
115.536592774005));
#211956=CARTESIAN_POINT('Ctrl Pts',(-6.00908262087056,3.11680452169815,
115.544897867444));
#211957=CARTESIAN_POINT('Ctrl Pts',(-6.08635676429967,2.95779484374147,
115.553202960883));
#211958=CARTESIAN_POINT('Ctrl Pts',(-6.1636162693674,2.79881528764738,115.561506481054));
#211959=CARTESIAN_POINT('Ctrl Pts',(-6.23465682574867,2.63677806402313,
115.569810001224));
#211960=CARTESIAN_POINT('Ctrl Pts',(-6.29924461315929,2.47220676796736,
115.578113521395));
#211961=CARTESIAN_POINT('Ctrl Pts',(-6.36383087010756,2.30763937156792,
115.586416844807));
#211962=CARTESIAN_POINT('Ctrl Pts',(-6.42196453669024,2.14053834627063,
115.594720168219));
#211963=CARTESIAN_POINT('Ctrl Pts',(-6.47346030690991,1.97144633578038,
115.60302349163));
#211964=CARTESIAN_POINT('Ctrl Pts',(-6.52498103083715,1.80227238705392,
115.611330838648));
#211965=CARTESIAN_POINT('Ctrl Pts',(-6.56985732780373,1.63110585761185,
115.619638185666));
#211966=CARTESIAN_POINT('Ctrl Pts',(-6.60795384897111,1.45850434688001,
115.627945532684));
#211967=CARTESIAN_POINT('Ctrl Pts',(-6.64605950621598,1.28586144389693,
115.63625487192));
#211968=CARTESIAN_POINT('Ctrl Pts',(-6.67738207840241,1.111783214658,115.644564211156));
#211969=CARTESIAN_POINT('Ctrl Pts',(-6.70183750366304,0.936836738442482,
115.652873550392));
#211970=CARTESIAN_POINT('Ctrl Pts',(-6.72631443957702,0.761736381729536,
115.661190198407));
#211971=CARTESIAN_POINT('Ctrl Pts',(-6.7439121175271,0.58576659754841,115.669506846423));
#211972=CARTESIAN_POINT('Ctrl Pts',(-6.75459834917407,0.409499867319873,
115.677823494438));
#211973=CARTESIAN_POINT('Ctrl Pts',(-6.76286833007035,0.273088591596379,
115.684259675356));
#211974=CARTESIAN_POINT('Ctrl Pts',(-6.76700004375086,0.136499598629859,
115.690695856274));
#211975=CARTESIAN_POINT('Ctrl Pts',(-6.76699999999965,-2.1689422216089E-6,
115.697132037191));
#211976=CARTESIAN_POINT('',(-6.76699990640493,-0.00112548466659665,115.302820216217));
#211977=CARTESIAN_POINT('Ctrl Pts',(3.09910619832145,6.01563211736934,114.651477942722));
#211978=CARTESIAN_POINT('Ctrl Pts',(3.05552930528257,6.0380818644093,114.653778451286));
#211979=CARTESIAN_POINT('Ctrl Pts',(3.01170410465358,6.0600603354701,114.65607895985));
#211980=CARTESIAN_POINT('Ctrl Pts',(2.96764094135406,6.08156199040996,114.658379468414));
#211981=CARTESIAN_POINT('Ctrl Pts',(2.80627217981612,6.16030566582604,114.666804424547));
#211982=CARTESIAN_POINT('Ctrl Pts',(2.64178059318266,6.23261635171114,114.675229380681));
#211983=CARTESIAN_POINT('Ctrl Pts',(2.47470894753367,6.29826203210035,114.683654336814));
#211984=CARTESIAN_POINT('Ctrl Pts',(2.30759852295219,6.36392294948203,114.69208124846));
#211985=CARTESIAN_POINT('Ctrl Pts',(2.13790715396069,6.42291565558589,114.700508160106));
#211986=CARTESIAN_POINT('Ctrl Pts',(1.9661957747478,6.4750570017077,114.708935071753));
#211987=CARTESIAN_POINT('Ctrl Pts',(1.79442125057133,6.52721752223378,114.717365082303));
#211988=CARTESIAN_POINT('Ctrl Pts',(1.62062555217479,6.57252156280522,114.725795092853));
#211989=CARTESIAN_POINT('Ctrl Pts',(1.4453832711689,6.61083627080758,114.734225103403));
#211990=CARTESIAN_POINT('Ctrl Pts',(1.26997956063984,6.6491862735174,114.742662879503));
#211991=CARTESIAN_POINT('Ctrl Pts',(1.0931269293425,6.6805340093711,114.751100655602));
#211992=CARTESIAN_POINT('Ctrl Pts',(0.915409736141963,6.70479783550381,
114.759538431702));
#211993=CARTESIAN_POINT('Ctrl Pts',(0.737599254515185,6.72907439835665,
114.767980637011));
#211994=CARTESIAN_POINT('Ctrl Pts',(0.55892363509588,6.74625959825403,114.776422842321));
#211995=CARTESIAN_POINT('Ctrl Pts',(0.379971380147108,6.75632376002432,
114.784865047631));
#211996=CARTESIAN_POINT('Ctrl Pts',(0.200830340415839,6.76639853893151,
114.793316159003));
#211997=CARTESIAN_POINT('Ctrl Pts',(0.0214124133284428,6.76933726242584,
114.801767270375));
#211998=CARTESIAN_POINT('Ctrl Pts',(-0.15769379551268,6.76516235332581,
114.810218381747));
#211999=CARTESIAN_POINT('Ctrl Pts',(-0.207960230455875,6.76399065862004,
114.812590199244));
#212000=CARTESIAN_POINT('Ctrl Pts',(-0.25820214019769,6.76225897079329,
114.814962016742));
#212001=CARTESIAN_POINT('Ctrl Pts',(-0.308406593246736,6.75996851865761,
114.817333834239));
#212002=CARTESIAN_POINT('Ctrl Pts',(-0.484437804735678,6.75193753654718,
114.825650106643));
#212003=CARTESIAN_POINT('Ctrl Pts',(-0.660325790370236,6.73701860481971,
114.833966379047));
#212004=CARTESIAN_POINT('Ctrl Pts',(-0.83549945920629,6.71522372327728,
114.842282651451));
#212005=CARTESIAN_POINT('Ctrl Pts',(-1.01052501849841,6.69344726933295,
114.850591892437));
#212006=CARTESIAN_POINT('Ctrl Pts',(-1.18483712075597,6.66480649119529,
114.858901133423));
#212007=CARTESIAN_POINT('Ctrl Pts',(-1.35786744642325,6.62936535408511,
114.867210374409));
#212008=CARTESIAN_POINT('Ctrl Pts',(-1.53078319923608,6.59394768449271,
114.875514113392));
#212009=CARTESIAN_POINT('Ctrl Pts',(-1.70241852693393,6.55173869802239,
114.883817852374));
#212010=CARTESIAN_POINT('Ctrl Pts',(-1.87221275855266,6.50285386478219,
114.892121591356));
#212011=CARTESIAN_POINT('Ctrl Pts',(-2.04192567742581,6.45399244199575,
114.900421353762));
#212012=CARTESIAN_POINT('Ctrl Pts',(-2.20979892364782,6.39846163977165,
114.908721116168));
#212013=CARTESIAN_POINT('Ctrl Pts',(-2.37528428571661,6.3364275078334,114.917020878573));
#212014=CARTESIAN_POINT('Ctrl Pts',(-2.54072071593177,6.27441171857528,
114.925318186848));
#212015=CARTESIAN_POINT('Ctrl Pts',(-2.70377034396579,6.20589655457228,
114.933615495122));
#212016=CARTESIAN_POINT('Ctrl Pts',(-2.86390211802493,6.13109726381602,
114.941912803397));
#212017=CARTESIAN_POINT('Ctrl Pts',(-3.02405007107716,6.05629041567639,
114.950210949994));
#212018=CARTESIAN_POINT('Ctrl Pts',(-3.1812792626631,5.97519831252793,114.958509096591));
#212019=CARTESIAN_POINT('Ctrl Pts',(-3.33508002324927,5.88808374927902,
114.966807243189));
#212020=CARTESIAN_POINT('Ctrl Pts',(-3.48889624946947,5.80096042611274,
114.975106224217));
#212021=CARTESIAN_POINT('Ctrl Pts',(-3.63928305433931,5.70781360686508,
114.983405205245));
#212022=CARTESIAN_POINT('Ctrl Pts',(-3.785756805383,5.60895127546106,114.991704186273));
#212023=CARTESIAN_POINT('Ctrl Pts',(-3.93226962756321,5.5100625730273,115.000005381013));
#212024=CARTESIAN_POINT('Ctrl Pts',(-4.0748670270541,5.40545551451027,115.008306575752));
#212025=CARTESIAN_POINT('Ctrl Pts',(-4.21309555720953,5.29548060385659,
115.016607770492));
#212026=CARTESIAN_POINT('Ctrl Pts',(-4.35138393385082,5.18545807921231,
115.02491255926));
#212027=CARTESIAN_POINT('Ctrl Pts',(-4.48529939917705,5.07006328716004,
115.033217348029));
#212028=CARTESIAN_POINT('Ctrl Pts',(-4.61442256269739,4.9496861933732,115.041522136797));
#212029=CARTESIAN_POINT('Ctrl Pts',(-4.74369880056909,4.82916639362216,
115.049836770818));
#212030=CARTESIAN_POINT('Ctrl Pts',(-4.8681711307963,4.70365272866408,115.058151404839));
#212031=CARTESIAN_POINT('Ctrl Pts',(-4.98745711439453,4.57357196642574,
115.06646603886));
#212032=CARTESIAN_POINT('Ctrl Pts',(-5.10681852357731,4.44340895296866,
115.074785930298));
#212033=CARTESIAN_POINT('Ctrl Pts',(-5.22098682158818,4.3086733483489,115.083105821735));
#212034=CARTESIAN_POINT('Ctrl Pts',(-5.32962061785988,4.16982410536498,
115.091425713173));
#212035=CARTESIAN_POINT('Ctrl Pts',(-5.43841685688205,4.03076723774025,
115.099758045547));
#212036=CARTESIAN_POINT('Ctrl Pts',(-5.54166185148013,3.88758472074133,
115.10809037792));
#212037=CARTESIAN_POINT('Ctrl Pts',(-5.63905744644338,3.74076464318613,
115.116422710293));
#212038=CARTESIAN_POINT('Ctrl Pts',(-5.71238509552381,3.63022605949566,
115.122695995492));
#212039=CARTESIAN_POINT('Ctrl Pts',(-5.78239800653076,3.51762616576756,
115.12896928069));
#212040=CARTESIAN_POINT('Ctrl Pts',(-5.84898648646649,3.40318175846257,
115.135242565889));
#212041=CARTESIAN_POINT('Ctrl Pts',(-5.93760450071311,3.25087559188858,
115.143591248388));
#212042=CARTESIAN_POINT('Ctrl Pts',(-6.02041506441768,3.09485622417132,
115.151939930887));
#212043=CARTESIAN_POINT('Ctrl Pts',(-6.09709480253619,2.9355960159542,115.160288613387));
#212044=CARTESIAN_POINT('Ctrl Pts',(-6.17365467097237,2.77658477142731,
115.168624244799));
#212045=CARTESIAN_POINT('Ctrl Pts',(-6.24410265488161,2.61434308122859,
115.176959876212));
#212046=CARTESIAN_POINT('Ctrl Pts',(-6.30815875215348,2.44937178836318,
115.185295507624));
#212047=CARTESIAN_POINT('Ctrl Pts',(-6.37212489898538,2.28463215557399,
115.19361943377));
#212048=CARTESIAN_POINT('Ctrl Pts',(-6.4297169150105,2.11717087142884,115.201943359916));
#212049=CARTESIAN_POINT('Ctrl Pts',(-6.48070071169988,1.94751310274738,
115.210267286061));
#212050=CARTESIAN_POINT('Ctrl Pts',(-6.53160010017454,1.77813621760732,
115.218577431206));
#212051=CARTESIAN_POINT('Ctrl Pts',(-6.57591298334361,1.60657042382224,
115.226887576351));
#212052=CARTESIAN_POINT('Ctrl Pts',(-6.61345353604174,1.43336015244495,
115.235197721496));
#212053=CARTESIAN_POINT('Ctrl Pts',(-6.65095821626886,1.26031539489182,
115.243499925749));
#212054=CARTESIAN_POINT('Ctrl Pts',(-6.68170338189337,1.08562962205983,
115.251802130003));
#212055=CARTESIAN_POINT('Ctrl Pts',(-6.70555282026724,0.909862832852349,
115.260104334257));
#212056=CARTESIAN_POINT('Ctrl Pts',(-6.72937745224773,0.734278863049114,
115.268397903182));
#212057=CARTESIAN_POINT('Ctrl Pts',(-6.74632060922838,0.557616456564615,
115.276691472106));
#212058=CARTESIAN_POINT('Ctrl Pts',(-6.75629704702972,0.380446070156476,
115.284985041031));
#212059=CARTESIAN_POINT('Ctrl Pts',(-6.76344843212745,0.253445462690426,
115.290930099418));
#212060=CARTESIAN_POINT('Ctrl Pts',(-6.76702108047258,0.126184102351834,
115.296875157804));
#212061=CARTESIAN_POINT('Ctrl Pts',(-6.76699990640502,-0.00112548408345884,
115.30282021619));
#212062=CARTESIAN_POINT('Ctrl Pts',(-6.76699990640493,-0.00112548466660582,
115.302820216217));
#212063=CARTESIAN_POINT('Ctrl Pts',(-6.76696947764202,-0.184079052889598,
115.311363717736));
#212064=CARTESIAN_POINT('Ctrl Pts',(-6.75951525884011,-0.366837573503022,
115.319907219255));
#212065=CARTESIAN_POINT('Ctrl Pts',(-6.74471008487077,-0.548794015130008,
115.328450720773));
#212066=CARTESIAN_POINT('Ctrl Pts',(-6.72988099850545,-0.731044341482288,
115.337008021224));
#212067=CARTESIAN_POINT('Ctrl Pts',(-6.70767727598725,-0.912489697216475,
115.345565321675));
#212068=CARTESIAN_POINT('Ctrl Pts',(-6.67822298376905,-1.0925322782686,
115.354122622126));
#212069=CARTESIAN_POINT('Ctrl Pts',(-6.64868572237082,-1.27308201750368,
115.362704027458));
#212070=CARTESIAN_POINT('Ctrl Pts',(-6.61185708748473,-1.45222077415082,
115.371285432789));
#212071=CARTESIAN_POINT('Ctrl Pts',(-6.56791194030996,-1.62936237354798,
115.379866838121));
#212072=CARTESIAN_POINT('Ctrl Pts',(-6.52390165183023,-1.8067665556349,
115.388460963946));
#212073=CARTESIAN_POINT('Ctrl Pts',(-6.47275387666453,-1.98216737667207,
115.397055089771));
#212074=CARTESIAN_POINT('Ctrl Pts',(-6.41469224619908,-2.15499707344428,
115.405649215595));
#212075=CARTESIAN_POINT('Ctrl Pts',(-6.35647289287564,-2.32829625744071,
115.414266687132));
#212076=CARTESIAN_POINT('Ctrl Pts',(-6.29130222624172,-2.49901005935072,
115.422884158668));
#212077=CARTESIAN_POINT('Ctrl Pts',(-6.21945171751244,-2.6665913323064,
115.431501630205));
#212078=CARTESIAN_POINT('Ctrl Pts',(-6.15928172429549,-2.80692943478278,
115.438718185983));
#212079=CARTESIAN_POINT('Ctrl Pts',(-6.09442806186373,-2.94507108580868,
115.44593474176));
#212080=CARTESIAN_POINT('Ctrl Pts',(-6.02507358098221,-3.080710525796,115.453151297538));
#212081=CARTESIAN_POINT('Ctrl Pts',(-5.94598663686851,-3.23538414851715,
115.461380547274));
#212082=CARTESIAN_POINT('Ctrl Pts',(-5.86082356120344,-3.38723765770617,
115.46960979701));
#212083=CARTESIAN_POINT('Ctrl Pts',(-5.76980829933938,-3.53576034098388,
115.477839046746));
#212084=CARTESIAN_POINT('Ctrl Pts',(-5.6789013604433,-3.68410625810681,
115.486058502336));
#212085=CARTESIAN_POINT('Ctrl Pts',(-5.58215628975952,-3.82912894013437,
115.494277957926));
#212086=CARTESIAN_POINT('Ctrl Pts',(-5.47984408366963,-3.97033976111252,
115.502497413516));
#212087=CARTESIAN_POINT('Ctrl Pts',(-5.37763309894116,-4.11141087684832,
115.510708737286));
#212088=CARTESIAN_POINT('Ctrl Pts',(-5.26986615637442,-4.24867735339501,
115.518920061055));
#212089=CARTESIAN_POINT('Ctrl Pts',(-5.1568589851902,-4.38167712261676,
115.527131384825));
#212090=CARTESIAN_POINT('Ctrl Pts',(-5.04394092988708,-4.51457201007308,
115.535336233259));
#212091=CARTESIAN_POINT('Ctrl Pts',(-4.92579110784487,-4.64320661974069,
115.543541081693));
#212092=CARTESIAN_POINT('Ctrl Pts',(-4.80276723285398,-4.76714966274651,
115.551745930127));
#212093=CARTESIAN_POINT('Ctrl Pts',(-4.67981568185696,-4.8910198413926,
115.559945955047));
#212094=CARTESIAN_POINT('Ctrl Pts',(-4.55199603802627,-5.01020369393627,
115.568145979967));
#212095=CARTESIAN_POINT('Ctrl Pts',(-4.41970484843799,-5.12430464089458,
115.576346004887));
#212096=CARTESIAN_POINT('Ctrl Pts',(-4.28745194691695,-5.23837256445396,
115.584543656534));
#212097=CARTESIAN_POINT('Ctrl Pts',(-4.1507303461087,-5.34736027573843,
115.592741308181));
#212098=CARTESIAN_POINT('Ctrl Pts',(-4.00997203146715,-5.45090940182014,
115.600938959828));
#212099=CARTESIAN_POINT('Ctrl Pts',(-3.86923256522737,-5.55444466203868,
115.609135513759));
#212100=CARTESIAN_POINT('Ctrl Pts',(-3.72445775009467,-5.65254257428186,
115.61733206769));
#212101=CARTESIAN_POINT('Ctrl Pts',(-3.57611110670047,-5.74488627846832,
115.625528621621));
#212102=CARTESIAN_POINT('Ctrl Pts',(-3.42775735455738,-5.83723440775123,
115.63372556833));
#212103=CARTESIAN_POINT('Ctrl Pts',(-3.27583173771128,-5.9238275899862,
115.641922515038));
#212104=CARTESIAN_POINT('Ctrl Pts',(-3.12082513134332,-6.00439334983776,
115.650119461747));
#212105=CARTESIAN_POINT('Ctrl Pts',(-2.96578291291584,-6.08497761930452,
115.658318291667));
#212106=CARTESIAN_POINT('Ctrl Pts',(-2.80765861341052,-6.15953154292312,
115.666517121587));
#212107=CARTESIAN_POINT('Ctrl Pts',(-2.64696601603294,-6.22782947020603,
115.674715951506));
#212108=CARTESIAN_POINT('Ctrl Pts',(-2.48612122222321,-6.29619208435707,
115.682922546766));
#212109=CARTESIAN_POINT('Ctrl Pts',(-2.32270360121288,-6.35828672359817,
115.691129142026));
#212110=CARTESIAN_POINT('Ctrl Pts',(-2.15724603569831,-6.41393627513277,
115.699335737286));
#212111=CARTESIAN_POINT('Ctrl Pts',(-1.99170838777328,-6.4696127613694,
115.707546304585));
#212112=CARTESIAN_POINT('Ctrl Pts',(-1.82412917081494,-6.51883783939465,
115.715756871884));
#212113=CARTESIAN_POINT('Ctrl Pts',(-1.65505451322706,-6.56148485925608,
115.723967439183));
#212114=CARTESIAN_POINT('Ctrl Pts',(-1.48574667748174,-6.60419069546322,
115.732189330029));
#212115=CARTESIAN_POINT('Ctrl Pts',(-1.31493963041393,-6.64030026866411,
115.740411220876));
#212116=CARTESIAN_POINT('Ctrl Pts',(-1.14318894998513,-6.66973822759424,
115.748633111723));
#212117=CARTESIAN_POINT('Ctrl Pts',(-0.987027048126935,-6.69650427965223,
115.756108750878));
#212118=CARTESIAN_POINT('Ctrl Pts',(-0.830085316907989,-6.7177554648684,
115.763584390033));
#212119=CARTESIAN_POINT('Ctrl Pts',(-0.672782764837577,-6.73347253290139,
115.771060029188));
#212120=CARTESIAN_POINT('Ctrl Pts',(-0.484752459891771,-6.75225980021652,
115.779995972638));
#212121=CARTESIAN_POINT('Ctrl Pts',(-0.295815010088564,-6.76317869153292,
115.788931916089));
#212122=CARTESIAN_POINT('Ctrl Pts',(-0.106620280744591,-6.76615999779298,
115.79786785954));
#212123=CARTESIAN_POINT('Ctrl Pts',(0.0822900387402636,-6.769136822359,
115.806790369898));
#212124=CARTESIAN_POINT('Ctrl Pts',(0.2714566084682,-6.76419986683672,115.815712880255));
#212125=CARTESIAN_POINT('Ctrl Pts',(0.460226153934383,-6.75133178619113,
115.824635390613));
#212126=CARTESIAN_POINT('Ctrl Pts',(0.648533155433595,-6.73849523633646,
115.833536038051));
#212127=CARTESIAN_POINT('Ctrl Pts',(0.836444817132283,-6.7177663651371,
115.84243668549));
#212128=CARTESIAN_POINT('Ctrl Pts',(1.02331020179792,-6.6891797128569,115.851337332928));
#212129=CARTESIAN_POINT('Ctrl Pts',(1.20988680907452,-6.66063723771962,
115.860224225514));
#212130=CARTESIAN_POINT('Ctrl Pts',(1.39542011063273,-6.62426124291457,
115.8691111181));
#212131=CARTESIAN_POINT('Ctrl Pts',(1.5792636160744,-6.58013794923356,115.877998010687));
#212132=CARTESIAN_POINT('Ctrl Pts',(1.76263457508044,-6.53612806888802,
115.886862060642));
#212133=CARTESIAN_POINT('Ctrl Pts',(1.94432415461541,-6.48441068565554,
115.895726110596));
#212134=CARTESIAN_POINT('Ctrl Pts',(2.12369614625398,-6.42512285317456,
115.904590160551));
#212135=CARTESIAN_POINT('Ctrl Pts',(2.29519019974067,-6.368438915946,115.913064905372));
#212136=CARTESIAN_POINT('Ctrl Pts',(2.46456560479013,-6.30483525768566,
115.921539650192));
#212137=CARTESIAN_POINT('Ctrl Pts',(2.63127419824938,-6.23447552674859,
115.930014395013));
#212138=CARTESIAN_POINT('Ctrl Pts',(2.79275358285557,-6.16632279498463,
115.938223309442));
#212139=CARTESIAN_POINT('Ctrl Pts',(2.95157479802554,-6.09189598382998,
115.946432223871));
#212140=CARTESIAN_POINT('Ctrl Pts',(3.10722938386873,-6.01144030628458,
115.9546411383));
#212141=CARTESIAN_POINT('Ctrl Pts',(3.26292097579913,-5.93096550081047,
115.962852004357));
#212142=CARTESIAN_POINT('Ctrl Pts',(3.41544412218355,-5.84445913685158,
115.971062870414));
#212143=CARTESIAN_POINT('Ctrl Pts',(3.56431538039064,-5.7522121717745,115.97927373647));
#212144=CARTESIAN_POINT('Ctrl Pts',(3.71324856890886,-5.65992683204192,
115.98748801824));
#212145=CARTESIAN_POINT('Ctrl Pts',(3.85852654028454,-5.56189632102397,
115.99570230001));
#212146=CARTESIAN_POINT('Ctrl Pts',(3.99969515571156,-5.45845469536731,
116.00391658178));
#212147=CARTESIAN_POINT('Ctrl Pts',(4.14102266755972,-5.35489663799485,
116.012140109372));
#212148=CARTESIAN_POINT('Ctrl Pts',(4.27823129766527,-5.24591551152056,
116.020363636965));
#212149=CARTESIAN_POINT('Ctrl Pts',(4.4108995522863,-5.13188602169227,116.028587164557));
#212150=CARTESIAN_POINT('Ctrl Pts',(4.54365284209776,-5.01778344339674,
116.036815963111));
#212151=CARTESIAN_POINT('Ctrl Pts',(4.67185969496866,-4.89862629316028,
116.045044761664));
#212152=CARTESIAN_POINT('Ctrl Pts',(4.79513583137633,-4.77482579353958,
116.053273560218));
#212153=CARTESIAN_POINT('Ctrl Pts',(4.91858164752081,-4.65085489243805,
116.061513685054));
#212154=CARTESIAN_POINT('Ctrl Pts',(5.03708295075616,-4.52222813723402,
116.069753809891));
#212155=CARTESIAN_POINT('Ctrl Pts',(5.15029540129018,-4.38939019448594,
116.077993934727));
#212156=CARTESIAN_POINT('Ctrl Pts',(5.20055705722302,-4.33041562992402,
116.081652210097));
#212157=CARTESIAN_POINT('Ctrl Pts',(5.24977685020032,-4.27061143519299,
116.085310485467));
#212158=CARTESIAN_POINT('Ctrl Pts',(5.29792742565693,-4.21001828885246,
116.088968760837));
#212159=CARTESIAN_POINT('Ctrl Pts',(5.40912112113917,-4.07009107513575,
116.0974167836));
#212160=CARTESIAN_POINT('Ctrl Pts',(5.51486440411148,-3.92563445489108,
116.105864806362));
#212161=CARTESIAN_POINT('Ctrl Pts',(5.61478410077162,-3.77710054164861,
116.114312829125));
#212162=CARTESIAN_POINT('Ctrl Pts',(5.71461229798134,-3.6287026453466,116.12275311578));
#212163=CARTESIAN_POINT('Ctrl Pts',(5.80862735353041,-3.47623517380994,
116.131193402436));
#212164=CARTESIAN_POINT('Ctrl Pts',(5.89649729853568,-3.3201820143422,116.139633689092));
#212165=CARTESIAN_POINT('Ctrl Pts',(5.98430030549211,-3.16424773390653,
116.14806754606));
#212166=CARTESIAN_POINT('Ctrl Pts',(6.06596737094342,-3.00473350043247,
116.156501403028));
#212167=CARTESIAN_POINT('Ctrl Pts',(6.14121046779082,-2.84215112024263,
116.164935259996));
#212168=CARTESIAN_POINT('Ctrl Pts',(6.21640781292909,-2.67966759858042,
116.173363988741));
#212169=CARTESIAN_POINT('Ctrl Pts',(6.28518883746487,-2.51411995161613,
116.181792717486));
#212170=CARTESIAN_POINT('Ctrl Pts',(6.34731182640543,-2.34604381424853,
116.190221446231));
#212171=CARTESIAN_POINT('Ctrl Pts',(6.40940658112922,-2.17804406564098,
116.198646344211));
#212172=CARTESIAN_POINT('Ctrl Pts',(6.46484921870031,-2.0075184303876,116.207071242191));
#212173=CARTESIAN_POINT('Ctrl Pts',(6.51344631996132,-1.83502208078876,
116.215496140172));
#212174=CARTESIAN_POINT('Ctrl Pts',(6.56203266174497,-1.66256392216267,
116.223919172866));
#212175=CARTESIAN_POINT('Ctrl Pts',(6.60377639616261,-1.48813623912324,
116.23234220556));
#212176=CARTESIAN_POINT('Ctrl Pts',(6.6385339479833,-1.31230942291568,116.240765238254));
#212177=CARTESIAN_POINT('Ctrl Pts',(6.67328756702648,-1.13650250131269,
116.249187317892));
#212178=CARTESIAN_POINT('Ctrl Pts',(6.70105651467291,-0.959297089217605,
116.257609397529));
#212179=CARTESIAN_POINT('Ctrl Pts',(6.72174826329795,-0.781274141931635,
116.266031477167));
#212180=CARTESIAN_POINT('Ctrl Pts',(6.74244055908869,-0.60324648706626,
116.274453779515));
#212181=CARTESIAN_POINT('Ctrl Pts',(6.75605524461533,-0.424401585194312,
116.282876081863));
#212182=CARTESIAN_POINT('Ctrl Pts',(6.76255159130435,-0.245326262244779,
116.291298384212));
#212183=CARTESIAN_POINT('Ctrl Pts',(6.76904901667478,-0.0662212048566616,
116.299722085035));
#212184=CARTESIAN_POINT('Ctrl Pts',(6.76842573524668,0.113114016656728,
116.308145785859));
#212185=CARTESIAN_POINT('Ctrl Pts',(6.76069312908836,0.292091448518292,
116.316569486682));
#212186=CARTESIAN_POINT('Ctrl Pts',(6.75295529020476,0.471189996044104,
116.324998887901));
#212187=CARTESIAN_POINT('Ctrl Pts',(6.73809852757025,0.64992993660467,116.33342828912));
#212188=CARTESIAN_POINT('Ctrl Pts',(6.71618628306615,0.827726289998191,
116.341857690339));
#212189=CARTESIAN_POINT('Ctrl Pts',(6.69426622030366,1.0055860808835,116.350290099157));
#212190=CARTESIAN_POINT('Ctrl Pts',(6.66528570302216,1.18250128310897,116.358722507975));
#212191=CARTESIAN_POINT('Ctrl Pts',(6.62935962369917,1.35789542294949,116.367154916792));
#212192=CARTESIAN_POINT('Ctrl Pts',(6.59340030452226,1.53345184255162,116.37559512752));
#212193=CARTESIAN_POINT('Ctrl Pts',(6.55048265670781,1.70748406234172,116.384035338248));
#212194=CARTESIAN_POINT('Ctrl Pts',(6.500772204812,1.87942803563843,116.392475548975));
#212195=CARTESIAN_POINT('Ctrl Pts',(6.47249774803957,1.97722683357428,116.397276196812));
#212196=CARTESIAN_POINT('Ctrl Pts',(6.4420266348651,2.07435033715814,116.402076844649));
#212197=CARTESIAN_POINT('Ctrl Pts',(6.40939637597011,2.1706973754306,116.406877492486));
#212198=CARTESIAN_POINT('Ctrl Pts',(6.35407029960003,2.33405812640248,116.415017207519));
#212199=CARTESIAN_POINT('Ctrl Pts',(6.29242383099363,2.49551126129875,116.423156922552));
#212200=CARTESIAN_POINT('Ctrl Pts',(6.22460993351384,2.65452823974445,116.431296637585));
#212201=CARTESIAN_POINT('Ctrl Pts',(6.15685534566194,2.81340614289484,116.439429233672));
#212202=CARTESIAN_POINT('Ctrl Pts',(6.0829442083237,2.96985179608627,116.447561829759));
#212203=CARTESIAN_POINT('Ctrl Pts',(6.00307902500841,3.12335256087175,116.455694425846));
#212204=CARTESIAN_POINT('Ctrl Pts',(5.92326844181703,3.27674838429942,116.463821462054));
#212205=CARTESIAN_POINT('Ctrl Pts',(5.83751208514919,3.42720300413067,116.471948498261));
#212206=CARTESIAN_POINT('Ctrl Pts',(5.74606021262659,3.57422453587764,116.480075534469));
#212207=CARTESIAN_POINT('Ctrl Pts',(5.6546520557542,3.72117578867155,116.488198685807));
#212208=CARTESIAN_POINT('Ctrl Pts',(5.55755399755129,3.86469691100852,116.496321837145));
#212209=CARTESIAN_POINT('Ctrl Pts',(5.45506179106966,4.00432139764178,116.504444988482));
#212210=CARTESIAN_POINT('Ctrl Pts',(5.35259838565977,4.14390664875663,116.512565857154));
#212211=CARTESIAN_POINT('Ctrl Pts',(5.24474406828782,4.27959715067328,116.520686725825));
#212212=CARTESIAN_POINT('Ctrl Pts',(5.13183736405347,4.4109561626596,116.528807594497));
#212213=CARTESIAN_POINT('Ctrl Pts',(5.01892455790864,4.54232227378975,116.536928902052));
#212214=CARTESIAN_POINT('Ctrl Pts',(4.90095905510152,4.66935614699891,116.545050209606));
#212215=CARTESIAN_POINT('Ctrl Pts',(4.77831915753368,4.79165472762246,116.553171517161));
#212216=CARTESIAN_POINT('Ctrl Pts',(4.71459120357028,4.8552053214368,116.557391630878));
#212217=CARTESIAN_POINT('Ctrl Pts',(4.64960169925592,4.91747787101678,116.561611744594));
#212218=CARTESIAN_POINT('Ctrl Pts',(4.58340761898701,4.97841978927167,116.565831858311));
#212219=CARTESIAN_POINT('Ctrl Pts',(4.44246601318343,5.10817839887396,116.574817399035));
#212220=CARTESIAN_POINT('Ctrl Pts',(4.29613133671346,5.23183804094533,116.583802939758));
#212221=CARTESIAN_POINT('Ctrl Pts',(4.14494026557815,5.34899609223908,116.592788480482));
#212222=CARTESIAN_POINT('Ctrl Pts',(3.99352790923918,5.46632561756927,116.601787172559));
#212223=CARTESIAN_POINT('Ctrl Pts',(3.83724514719207,5.57713439577659,116.610785864636));
#212224=CARTESIAN_POINT('Ctrl Pts',(3.67665792189673,5.68106288693886,116.619784556714));
#212225=CARTESIAN_POINT('Ctrl Pts',(3.51577657434522,5.78518172750311,116.628799730274));
#212226=CARTESIAN_POINT('Ctrl Pts',(3.35057519985205,5.88239495346927,116.637814903834));
#212227=CARTESIAN_POINT('Ctrl Pts',(3.18164658582711,5.97238762999311,116.646830077394));
#212228=CARTESIAN_POINT('Ctrl Pts',(3.15423038832485,5.98699295312072,116.648293191149));
#212229=CARTESIAN_POINT('Ctrl Pts',(3.12671606358679,6.00140819161904,116.649756304904));
#212230=CARTESIAN_POINT('Ctrl Pts',(3.09910619832135,6.0156321173694,116.651219418659));
#212231=CARTESIAN_POINT('Origin',(0.,0.,4.30282021618968));
#212232=CARTESIAN_POINT('',(3.09910619832142,6.01563211736936,119.045959136766));
#212233=CARTESIAN_POINT('',(3.09910619832126,6.01563211736944,118.651553971577));
#212234=CARTESIAN_POINT('',(3.09910619832133,6.0156321173694,4.30282021618968));
#212235=CARTESIAN_POINT('',(-6.76699999999861,4.3460530827503E-6,117.697273959568));
#212236=CARTESIAN_POINT('Ctrl Pts',(-6.76699999999861,4.34605308275028E-6,
117.697273959568));
#212237=CARTESIAN_POINT('Ctrl Pts',(-6.76700011305956,-0.176036644547901,
117.705588278987));
#212238=CARTESIAN_POINT('Ctrl Pts',(-6.760126440919,-0.352257286263359,
117.713902598407));
#212239=CARTESIAN_POINT('Ctrl Pts',(-6.74636291712061,-0.528087483756204,
117.722216917826));
#212240=CARTESIAN_POINT('Ctrl Pts',(-6.73261188350642,-0.703758118074181,
117.73052369213));
#212241=CARTESIAN_POINT('Ctrl Pts',(-6.71198348273243,-0.879038668276297,
117.738830466434));
#212242=CARTESIAN_POINT('Ctrl Pts',(-6.68451369221068,-1.05335924482007,
117.747137240738));
#212243=CARTESIAN_POINT('Ctrl Pts',(-6.6570637548589,-1.22755383510886,
117.755438011508));
#212244=CARTESIAN_POINT('Ctrl Pts',(-6.62278233466031,-1.40078949100303,
117.763738782278));
#212245=CARTESIAN_POINT('Ctrl Pts',(-6.58175723051189,-1.57250143357788,
117.772039553049));
#212246=CARTESIAN_POINT('Ctrl Pts',(-6.54063083866197,-1.74463731920768,
117.780360817758));
#212247=CARTESIAN_POINT('Ctrl Pts',(-6.49272745480837,-1.91524160647387,
117.788682082468));
#212248=CARTESIAN_POINT('Ctrl Pts',(-6.43818734215969,-2.08375448343962,
117.797003347178));
#212249=CARTESIAN_POINT('Ctrl Pts',(-6.38382669575631,-2.25171286259,117.80529723046));
#212250=CARTESIAN_POINT('Ctrl Pts',(-6.32287304359227,-2.41759324207099,
117.813591113742));
#212251=CARTESIAN_POINT('Ctrl Pts',(-6.2555154742714,-2.5808555076081,117.821884997024));
#212252=CARTESIAN_POINT('Ctrl Pts',(-6.18816636687098,-2.74409726301817,
117.830177838372));
#212253=CARTESIAN_POINT('Ctrl Pts',(-6.11441507831726,-2.90472123763043,
117.83847067972));
#212254=CARTESIAN_POINT('Ctrl Pts',(-6.03449910347032,-3.06220665047544,
117.846763521067));
#212255=CARTESIAN_POINT('Ctrl Pts',(-5.95457978942486,-3.21969864367007,
117.855056708922));
#212256=CARTESIAN_POINT('Ctrl Pts',(-5.86849543416824,-3.37405150315763,
117.863349896777));
#212257=CARTESIAN_POINT('Ctrl Pts',(-5.77652989209185,-3.5247682768899,
117.871643084631));
#212258=CARTESIAN_POINT('Ctrl Pts',(-5.68402045079509,-3.67637641421203,
117.879985319752));
#212259=CARTESIAN_POINT('Ctrl Pts',(-5.5855602058369,-3.8243050052865,117.888327554873));
#212260=CARTESIAN_POINT('Ctrl Pts',(-5.48148265944007,-3.96807722382741,
117.896669789994));
#212261=CARTESIAN_POINT('Ctrl Pts',(-5.37792086648259,-4.11113698306501,
117.904970685396));
#212262=CARTESIAN_POINT('Ctrl Pts',(-5.26879756661816,-4.25008121831449,
117.913271580798));
#212263=CARTESIAN_POINT('Ctrl Pts',(-5.15448211887255,-4.38447295421276,
117.921572476201));
#212264=CARTESIAN_POINT('Ctrl Pts',(-5.0393127087195,-4.51986862695938,
117.929935381181));
#212265=CARTESIAN_POINT('Ctrl Pts',(-4.91887349889496,-4.6506432355397,
117.93829828616));
#212266=CARTESIAN_POINT('Ctrl Pts',(-4.79358027298436,-4.77638745983355,
117.94666119114));
#212267=CARTESIAN_POINT('Ctrl Pts',(-4.66828704707384,-4.90213168412732,
117.95502409612));
#212268=CARTESIAN_POINT('Ctrl Pts',(-4.5381400908651,-5.02284530400535,
117.9633870011));
#212269=CARTESIAN_POINT('Ctrl Pts',(-4.40358931946243,-5.13816018682917,
117.97174990608));
#212270=CARTESIAN_POINT('Ctrl Pts',(-4.27262945093562,-5.25039753587118,
117.979889621113));
#212271=CARTESIAN_POINT('Ctrl Pts',(-4.1372082456562,-5.35776838396358,
117.988029336146));
#212272=CARTESIAN_POINT('Ctrl Pts',(-3.99772702156077,-5.4598963049753,
117.996169051179));
#212273=CARTESIAN_POINT('Ctrl Pts',(-3.85836778690731,-5.56193490551987,
118.004301647266));
#212274=CARTESIAN_POINT('Ctrl Pts',(-3.71495589486778,-5.65873949139583,
118.012434243353));
#212275=CARTESIAN_POINT('Ctrl Pts',(-3.56792714719738,-5.74997259752531,
118.020566839439));
#212276=CARTESIAN_POINT('Ctrl Pts',(-3.42099891626635,-5.84114333180918,
118.028693875647));
#212277=CARTESIAN_POINT('Ctrl Pts',(-3.2704590625712,-5.92674997750293,
118.036820911855));
#212278=CARTESIAN_POINT('Ctrl Pts',(-3.11677385922776,-6.00649729130335,
118.044947948063));
#212279=CARTESIAN_POINT('Ctrl Pts',(-2.96316212019301,-6.08620648444446,
118.053071099401));
#212280=CARTESIAN_POINT('Ctrl Pts',(-2.80640834990148,-6.16006175482521,
118.061194250739));
#212281=CARTESIAN_POINT('Ctrl Pts',(-2.6470049896705,-6.22781290539942,
118.069317402076));
#212282=CARTESIAN_POINT('Ctrl Pts',(-2.48764642296852,-6.29554501739674,
118.077438270748));
#212283=CARTESIAN_POINT('Ctrl Pts',(-2.32564008637862,-6.35717628373792,
118.085559139419));
#212284=CARTESIAN_POINT('Ctrl Pts',(-2.16150000916222,-6.41250393453226,
118.093680008091));
#212285=CARTESIAN_POINT('Ctrl Pts',(-1.99735106118775,-6.46783457544463,
118.101801315646));
#212286=CARTESIAN_POINT('Ctrl Pts',(-1.83106848797845,-6.51686079946705,
118.1099226232));
#212287=CARTESIAN_POINT('Ctrl Pts',(-1.66318332939714,-6.559429107233,118.118043930755));
#212288=CARTESIAN_POINT('Ctrl Pts',(-1.57594436500362,-6.58154907970029,
118.122264044471));
#212289=CARTESIAN_POINT('Ctrl Pts',(-1.488272916242,-6.6019261053456,118.126484158188));
#212290=CARTESIAN_POINT('Ctrl Pts',(-1.40024481847838,-6.62054404473865,
118.130704271905));
#212291=CARTESIAN_POINT('Ctrl Pts',(-1.21283682760999,-6.66018082781594,
118.139688710431));
#212292=CARTESIAN_POINT('Ctrl Pts',(-1.02390467830441,-6.69182217318139,
118.148673148957));
#212293=CARTESIAN_POINT('Ctrl Pts',(-0.834115133867594,-6.71539581435473,
118.157657587482));
#212294=CARTESIAN_POINT('Ctrl Pts',(-0.643998024004414,-6.73901014222578,
118.166657532613));
#212295=CARTESIAN_POINT('Ctrl Pts',(-0.45302079843496,-6.75452890537391,
118.175657477743));
#212296=CARTESIAN_POINT('Ctrl Pts',(-0.261853921974926,-6.76193178932961,
118.184657422874));
#212297=CARTESIAN_POINT('Ctrl Pts',(-0.070236555863476,-6.76935211837138,
118.193678576606));
#212298=CARTESIAN_POINT('Ctrl Pts',(0.121571115597132,-6.7686182923628,
118.202699730338));
#212299=CARTESIAN_POINT('Ctrl Pts',(0.312897257496911,-6.7597621486448,
118.211720884071));
#212300=CARTESIAN_POINT('Ctrl Pts',(0.504418075254281,-6.75089699373075,
118.220751216898));
#212301=CARTESIAN_POINT('Ctrl Pts',(0.69545614641719,-6.73389302765554,
118.229781549725));
#212302=CARTESIAN_POINT('Ctrl Pts',(0.885344550686241,-6.70883402884363,
118.238811882552));
#212303=CARTESIAN_POINT('Ctrl Pts',(1.07550215685612,-6.68373950427047,
118.247855017545));
#212304=CARTESIAN_POINT('Ctrl Pts',(1.26450660014674,-6.65056714468046,
118.256898152538));
#212305=CARTESIAN_POINT('Ctrl Pts',(1.4516986391693,-6.60945232685992,118.26594128753));
#212306=CARTESIAN_POINT('Ctrl Pts',(1.61534760779666,-6.57350850378515,
118.27384707093));
#212307=CARTESIAN_POINT('Ctrl Pts',(1.77761145950585,-6.53149523096438,
118.28175285433));
#212308=CARTESIAN_POINT('Ctrl Pts',(1.93805838123315,-6.48353443045782,
118.28965863773));
#212309=CARTESIAN_POINT('Ctrl Pts',(2.11367785289102,-6.43103825069584,
118.298312025958));
#212310=CARTESIAN_POINT('Ctrl Pts',(2.28727529007613,-6.37136888974459,
118.306965414187));
#212311=CARTESIAN_POINT('Ctrl Pts',(2.45826081080456,-6.30470005520187,
118.315618802415));
#212312=CARTESIAN_POINT('Ctrl Pts',(2.62908841427546,-6.23809279405712,
118.324264198625));
#212313=CARTESIAN_POINT('Ctrl Pts',(2.79730863038597,-6.16449906298657,
118.332909594836));
#212314=CARTESIAN_POINT('Ctrl Pts',(2.96234803145788,-6.08414193954395,
118.341554991046));
#212315=CARTESIAN_POINT('Ctrl Pts',(3.13265823504674,-6.00121848027034,
118.350476492089));
#212316=CARTESIAN_POINT('Ctrl Pts',(3.29958077737196,-5.911092562811,118.359397993131));
#212317=CARTESIAN_POINT('Ctrl Pts',(3.4625069947561,-5.81406349391414,118.368319494173));
#212318=CARTESIAN_POINT('Ctrl Pts',(3.62009022811629,-5.72021638537515,
118.376948424515));
#212319=CARTESIAN_POINT('Ctrl Pts',(3.77393479224612,-5.6199118627624,118.385577354857));
#212320=CARTESIAN_POINT('Ctrl Pts',(3.92351372896765,-5.51346796658894,
118.394206285199));
#212321=CARTESIAN_POINT('Ctrl Pts',(4.08070005372313,-5.4016104738237,118.403274071592));
#212322=CARTESIAN_POINT('Ctrl Pts',(4.23317524980973,-5.28297300151781,
118.412341857984));
#212323=CARTESIAN_POINT('Ctrl Pts',(4.38036056483422,-5.15797734795775,
118.421409644377));
#212324=CARTESIAN_POINT('Ctrl Pts',(4.52754587985881,-5.0329816943976,118.43047743077));
#212325=CARTESIAN_POINT('Ctrl Pts',(4.66944099337389,-4.90162808553282,
118.439545217162));
#212326=CARTESIAN_POINT('Ctrl Pts',(4.80550560803706,-4.764389242193,118.448613003555));
#212327=CARTESIAN_POINT('Ctrl Pts',(4.93192437885736,-4.63687948569408,
118.457037959688));
#212328=CARTESIAN_POINT('Ctrl Pts',(5.05325471587774,-4.50434546483646,
118.465462915821));
#212329=CARTESIAN_POINT('Ctrl Pts',(5.16910250584504,-4.36722661240135,
118.473887871954));
#212330=CARTESIAN_POINT('Ctrl Pts',(5.28497718519686,-4.23007593336385,
118.482314783601));
#212331=CARTESIAN_POINT('Ctrl Pts',(5.39536656620621,-4.08833855422847,
118.490741695247));
#212332=CARTESIAN_POINT('Ctrl Pts',(5.49991697375534,-3.94248681441016,
118.499168606893));
#212333=CARTESIAN_POINT('Ctrl Pts',(5.60450582856158,-3.79658143922616,
118.507598617443));
#212334=CARTESIAN_POINT('Ctrl Pts',(5.70325123545573,-3.64655895594379,
118.516028627993));
#212335=CARTESIAN_POINT('Ctrl Pts',(5.79584275988278,-3.49292079823096,
118.524458638544));
#212336=CARTESIAN_POINT('Ctrl Pts',(5.88851957768537,-3.33914111226093,
118.532896414643));
#212337=CARTESIAN_POINT('Ctrl Pts',(5.975031015918,-3.18173938166461,118.541334190742));
#212338=CARTESIAN_POINT('Ctrl Pts',(6.05511199578107,-3.02124274406216,
118.549771966842));
#212339=CARTESIAN_POINT('Ctrl Pts',(6.13523501225579,-2.8606618575552,118.558214172152));
#212340=CARTESIAN_POINT('Ctrl Pts',(6.20892069740678,-2.69698312382876,
118.566656377462));
#212341=CARTESIAN_POINT('Ctrl Pts',(6.27595185299024,-2.53075430236687,
118.575098582771));
#212342=CARTESIAN_POINT('Ctrl Pts',(6.34305372275449,-2.36435011864497,
118.583549694143));
#212343=CARTESIAN_POINT('Ctrl Pts',(6.40348692293132,-2.19539078338207,
118.592000805515));
#212344=CARTESIAN_POINT('Ctrl Pts',(6.457083557366,-2.02444089397384,118.600451916887));
#212345=CARTESIAN_POINT('Ctrl Pts',(6.47212553584083,-1.97646354271147,
118.602823734385));
#212346=CARTESIAN_POINT('Ctrl Pts',(6.48662933657987,-1.92832947991222,
118.605195551882));
#212347=CARTESIAN_POINT('Ctrl Pts',(6.50059196810422,-1.88005134616555,
118.607567369379));
#212348=CARTESIAN_POINT('Ctrl Pts',(6.54954895883781,-1.71077436264357,
118.615883641783));
#212349=CARTESIAN_POINT('Ctrl Pts',(6.59193723883534,-1.53941978367531,
118.624199914187));
#212350=CARTESIAN_POINT('Ctrl Pts',(6.62758466943129,-1.36653227167141,
118.632516186591));
#212351=CARTESIAN_POINT('Ctrl Pts',(6.66320196008258,-1.19379093626301,
118.640825427577));
#212352=CARTESIAN_POINT('Ctrl Pts',(6.69208968671876,-1.01951958917555,
118.649134668563));
#212353=CARTESIAN_POINT('Ctrl Pts',(6.71412581092551,-0.844276965849392,
118.657443909549));
#212354=CARTESIAN_POINT('Ctrl Pts',(6.73614734380756,-0.669150380261748,
118.665747648532));
#212355=CARTESIAN_POINT('Ctrl Pts',(6.75132627111712,-0.493054144020304,
118.674051387514));
#212356=CARTESIAN_POINT('Ctrl Pts',(6.75959178571707,-0.316556299047095,
118.682355126497));
#212357=CARTESIAN_POINT('Ctrl Pts',(6.7678533420454,-0.140142977112431,
118.690654888902));
#212358=CARTESIAN_POINT('Ctrl Pts',(6.76920806741503,0.0366712234252294,
118.698954651308));
#212359=CARTESIAN_POINT('Ctrl Pts',(6.7636370555824,0.21331380722471,118.707254413713));
#212360=CARTESIAN_POINT('Ctrl Pts',(6.75806769102494,0.389904160127534,
118.715551721988));
#212361=CARTESIAN_POINT('Ctrl Pts',(6.74557668216467,0.566322650083412,
118.723849030263));
#212362=CARTESIAN_POINT('Ctrl Pts',(6.72619722583197,0.741997223182337,
118.732146338537));
#212363=CARTESIAN_POINT('Ctrl Pts',(6.70681581148639,0.917689545647974,
118.740444485135));
#212364=CARTESIAN_POINT('Ctrl Pts',(6.68054458964911,1.09263745441796,118.748742631732));
#212365=CARTESIAN_POINT('Ctrl Pts',(6.64746865322672,1.26627386625808,118.757040778329));
#212366=CARTESIAN_POINT('Ctrl Pts',(6.61438939081074,1.43992773833226,118.765339759357));
#212367=CARTESIAN_POINT('Ctrl Pts',(6.57450411454754,1.61226950852305,118.773638740385));
#212368=CARTESIAN_POINT('Ctrl Pts',(6.52794907622942,1.7827422298682,118.781937721413));
#212369=CARTESIAN_POINT('Ctrl Pts',(6.48138161958898,1.95326042395439,118.790238916153));
#212370=CARTESIAN_POINT('Ctrl Pts',(6.42814094661717,2.1219082397564,118.798540110892));
#212371=CARTESIAN_POINT('Ctrl Pts',(6.36841327360824,2.2881436529489,118.806841305632));
#212372=CARTESIAN_POINT('Ctrl Pts',(6.30865974131138,2.45445103829766,118.8151460944));
#212373=CARTESIAN_POINT('Ctrl Pts',(6.24241372907965,2.61834361210753,118.823450883169));
#212374=CARTESIAN_POINT('Ctrl Pts',(6.16990976519984,2.77929892046388,118.831755671937));
#212375=CARTESIAN_POINT('Ctrl Pts',(6.09731984852195,2.94044503989287,118.840070305958));
#212376=CARTESIAN_POINT('Ctrl Pts',(6.01845730074957,3.09864661903254,118.848384939979));
#212377=CARTESIAN_POINT('Ctrl Pts',(5.93360337404752,3.25340437073105,118.856699574));
#212378=CARTESIAN_POINT('Ctrl Pts',(5.84869579345521,3.40825997712822,118.865019465438));
#212379=CARTESIAN_POINT('Ctrl Pts',(5.75778945781166,3.55966711554366,118.873339356876));
#212380=CARTESIAN_POINT('Ctrl Pts',(5.66120928704602,3.70715502889533,118.881659248314));
#212381=CARTESIAN_POINT('Ctrl Pts',(5.56448469760912,3.85486348450018,118.889991580687));
#212382=CARTESIAN_POINT('Ctrl Pts',(5.46206951923441,3.99864071956232,118.89832391306));
#212383=CARTESIAN_POINT('Ctrl Pts',(5.35433015514444,4.13804755769081,118.906656245434));
#212384=CARTESIAN_POINT('Ctrl Pts',(5.27321484099762,4.24300482715794,118.912929530632));
#212385=CARTESIAN_POINT('Ctrl Pts',(5.18908243876761,4.34548547249859,118.91920281583));
#212386=CARTESIAN_POINT('Ctrl Pts',(5.10210300205094,4.44531595687672,118.925476101029));
#212387=CARTESIAN_POINT('Ctrl Pts',(4.9901919625416,4.573761641319,118.933547547502));
#212388=CARTESIAN_POINT('Ctrl Pts',(4.8732205556082,4.69821570632098,118.941618993974));
#212389=CARTESIAN_POINT('Ctrl Pts',(4.75150793565389,4.81824255693071,118.949690440447));
#212390=CARTESIAN_POINT('Ctrl Pts',(4.6299902243914,4.93807719841335,118.957748961431));
#212391=CARTESIAN_POINT('Ctrl Pts',(4.50374668384009,5.05349848643888,118.965807482416));
#212392=CARTESIAN_POINT('Ctrl Pts',(4.37313732504745,5.16410291689436,118.9738660034));
#212393=CARTESIAN_POINT('Ctrl Pts',(4.24264786178556,5.274605815752,118.9819171269));
#212394=CARTESIAN_POINT('Ctrl Pts',(4.10780083282578,5.38030041198575,118.9899682504));
#212395=CARTESIAN_POINT('Ctrl Pts',(3.96899422323161,5.48081872131839,118.9980193739));
#212396=CARTESIAN_POINT('Ctrl Pts',(3.83030672184986,5.5812507771493,119.006063588832));
#212397=CARTESIAN_POINT('Ctrl Pts',(3.68766670429912,5.67651517070081,119.014107803764));
#212398=CARTESIAN_POINT('Ctrl Pts',(3.54150620200399,5.76628327618122,119.022152018696));
#212399=CARTESIAN_POINT('Ctrl Pts',(3.39731726769152,5.85484049417939,119.030087724719));
#212400=CARTESIAN_POINT('Ctrl Pts',(3.24970253348462,5.93804857724542,119.038023430743));
#212401=CARTESIAN_POINT('Ctrl Pts',(3.09910619832142,6.01563211736936,119.045959136766));
#212402=CARTESIAN_POINT('Ctrl Pts',(3.09910619832145,6.01563211736934,117.045755263024));
#212403=CARTESIAN_POINT('Ctrl Pts',(2.93375330764837,6.10081787314648,117.054504710927));
#212404=CARTESIAN_POINT('Ctrl Pts',(2.76488627843081,6.17918207037034,117.063254158829));
#212405=CARTESIAN_POINT('Ctrl Pts',(2.59307866646713,6.25045854553993,117.072003606731));
#212406=CARTESIAN_POINT('Ctrl Pts',(2.42127244185382,6.32173444515035,117.080752983982));
#212407=CARTESIAN_POINT('Ctrl Pts',(2.24652594672465,6.38592262741838,117.089502361232));
#212408=CARTESIAN_POINT('Ctrl Pts',(2.06943269687116,6.44280508110563,117.098251738482));
#212409=CARTESIAN_POINT('Ctrl Pts',(1.89234081822072,6.49968709436168,117.107001047987));
#212410=CARTESIAN_POINT('Ctrl Pts',(1.71290249405584,6.54926340459546,117.115750357493));
#212411=CARTESIAN_POINT('Ctrl Pts',(1.53172716625054,6.59136563150385,117.124499666998));
#212412=CARTESIAN_POINT('Ctrl Pts',(1.35055318107334,6.6334675464071,117.133248911665));
#212413=CARTESIAN_POINT('Ctrl Pts',(1.16764249714424,6.66809542395775,117.141998156333));
#212414=CARTESIAN_POINT('Ctrl Pts',(0.983616340614447,6.69513165624667,
117.150747401));
#212415=CARTESIAN_POINT('Ctrl Pts',(0.799591486713932,6.7221676971596,117.159496583736));
#212416=CARTESIAN_POINT('Ctrl Pts',(0.614451459526802,6.7416121586937,117.168245766471));
#212417=CARTESIAN_POINT('Ctrl Pts',(0.428825047910371,6.75339900185712,
117.176994949207));
#212418=CARTESIAN_POINT('Ctrl Pts',(0.243199888597042,6.76518576550221,
117.185744072918));
#212419=CARTESIAN_POINT('Ctrl Pts',(0.0570886373918207,6.76931499599835,
117.194493196628));
#212420=CARTESIAN_POINT('Ctrl Pts',(-0.128876626811339,6.76577266947846,
117.203242320339));
#212421=CARTESIAN_POINT('Ctrl Pts',(-0.314840698188291,6.76223036567992,
117.21199138793));
#212422=CARTESIAN_POINT('Ctrl Pts',(-0.500658497951327,6.75101660879222,
117.220740455522));
#212423=CARTESIAN_POINT('Ctrl Pts',(-0.685698951926234,6.73216948296218,
117.229489523113));
#212424=CARTESIAN_POINT('Ctrl Pts',(-0.870738280459779,6.71332247176294,
117.238238537492));
#212425=CARTESIAN_POINT('Ctrl Pts',(-1.05499998761234,6.68684221356189,
117.24698755187));
#212426=CARTESIAN_POINT('Ctrl Pts',(-1.23785829161395,6.65281863948527,
117.255736566249));
#212427=CARTESIAN_POINT('Ctrl Pts',(-1.43007412917375,6.61705395368867,
117.264933299948));
#212428=CARTESIAN_POINT('Ctrl Pts',(-1.6207388253576,6.57295372727798,117.274130033647));
#212429=CARTESIAN_POINT('Ctrl Pts',(-1.80913696091478,6.52068343478289,
117.283326767346));
#212430=CARTESIAN_POINT('Ctrl Pts',(-1.98838356186077,6.47095219815209,
117.29207676506));
#212431=CARTESIAN_POINT('Ctrl Pts',(-2.16557827572498,6.41382586850902,
117.300826762774));
#212432=CARTESIAN_POINT('Ctrl Pts',(-2.34011918621666,6.3494984994329,117.309576760487));
#212433=CARTESIAN_POINT('Ctrl Pts',(-2.5146565569107,6.28517243495562,117.318326580746));
#212434=CARTESIAN_POINT('Ctrl Pts',(-2.68653996295305,6.21364572242384,
117.327076401004));
#212435=CARTESIAN_POINT('Ctrl Pts',(-2.85518555379971,6.13516132252229,
117.335826221262));
#212436=CARTESIAN_POINT('Ctrl Pts',(-3.02382794858662,6.0566784100052,117.3445758757));
#212437=CARTESIAN_POINT('Ctrl Pts',(-3.18923239109245,5.971238194921,117.353325530137));
#212438=CARTESIAN_POINT('Ctrl Pts',(-3.35083705967653,5.87913088810739,
117.362075184575));
#212439=CARTESIAN_POINT('Ctrl Pts',(-3.51243888042351,5.78702520443133,
117.370824684824));
#212440=CARTESIAN_POINT('Ctrl Pts',(-3.67024081223638,5.68825280605817,
117.379574185073));
#212441=CARTESIAN_POINT('Ctrl Pts',(-3.82370687544346,5.58314917682543,
117.388323685322));
#212442=CARTESIAN_POINT('Ctrl Pts',(-3.97717043817757,5.47804726008063,
117.397073043012));
#212443=CARTESIAN_POINT('Ctrl Pts',(-4.126298037224,5.36661448084282,117.405822400703));
#212444=CARTESIAN_POINT('Ctrl Pts',(-4.27058317206846,5.24922931204626,
117.414571758393));
#212445=CARTESIAN_POINT('Ctrl Pts',(-4.41486614774769,5.13184589986847,
117.423320985153));
#212446=CARTESIAN_POINT('Ctrl Pts',(-4.55430658194343,5.00851045723098,
117.432070211913));
#212447=CARTESIAN_POINT('Ctrl Pts',(-4.68843089001771,4.8796418710319,117.440819438673));
#212448=CARTESIAN_POINT('Ctrl Pts',(-4.82255336917744,4.75077504208053,
117.449568546129));
#212449=CARTESIAN_POINT('Ctrl Pts',(-4.95135966065025,4.61637541908209,
117.458317653585));
#212450=CARTESIAN_POINT('Ctrl Pts',(-5.0744123086912,4.47689945401985,117.467066761041));
#212451=CARTESIAN_POINT('Ctrl Pts',(-5.19746344226295,4.33742520555662,
117.475815760817));
#212452=CARTESIAN_POINT('Ctrl Pts',(-5.31476088454647,4.19287495491489,
117.484564760594));
#212453=CARTESIAN_POINT('Ctrl Pts',(-5.42590627628735,4.04373961586865,
117.49331376037));
#212454=CARTESIAN_POINT('Ctrl Pts',(-5.53706380672555,3.89458798906894,
117.502063715665));
#212455=CARTESIAN_POINT('Ctrl Pts',(-5.64206777071757,3.74085050155445,
117.510813670959));
#212456=CARTESIAN_POINT('Ctrl Pts',(-5.74056148163907,3.58304938223323,
117.519563626254));
#212457=CARTESIAN_POINT('Ctrl Pts',(-5.83905138951784,3.42525435593452,
117.528313243695));
#212458=CARTESIAN_POINT('Ctrl Pts',(-5.93103139557555,3.26339625497361,
117.537062861136));
#212459=CARTESIAN_POINT('Ctrl Pts',(-6.01618907820751,3.0980248506519,117.545812478578));
#212460=CARTESIAN_POINT('Ctrl Pts',(-6.10134392544887,2.93265895249839,
117.554561804693));
#212461=CARTESIAN_POINT('Ctrl Pts',(-6.17967677261736,2.76378023986248,
117.563311130809));
#212462=CARTESIAN_POINT('Ctrl Pts',(-6.2509215700913,2.59196229227342,117.572060456925));
#212463=CARTESIAN_POINT('Ctrl Pts',(-6.32216437407667,2.42014915229315,
117.580809538228));
#212464=CARTESIAN_POINT('Ctrl Pts',(-6.38631941548843,2.24539720663073,
117.58955861953));
#212465=CARTESIAN_POINT('Ctrl Pts',(-6.44316881037467,2.06829994947905,
117.598307700832));
#212466=CARTESIAN_POINT('Ctrl Pts',(-6.5000233452451,1.89118668024664,117.607057573175));
#212467=CARTESIAN_POINT('Ctrl Pts',(-6.54957082411042,1.71172794807911,
117.615807445517));
#212468=CARTESIAN_POINT('Ctrl Pts',(-6.59164294296036,1.53053334250543,
117.62455731786));
#212469=CARTESIAN_POINT('Ctrl Pts',(-6.63371214082099,1.34935131693778,
117.633306582714));
#212470=CARTESIAN_POINT('Ctrl Pts',(-6.66830695239664,1.16643393829917,
117.642055847569));
#212471=CARTESIAN_POINT('Ctrl Pts',(-6.6953098815397,0.982402458342261,
117.650805112424));
#212472=CARTESIAN_POINT('Ctrl Pts',(-6.72231419690466,0.798361530948474,
117.659554826431));
#212473=CARTESIAN_POINT('Ctrl Pts',(-6.74172580829263,0.613206671364035,
117.668304540438));
#212474=CARTESIAN_POINT('Ctrl Pts',(-6.75347878028169,0.427566795115099,
117.677054254445));
#212475=CARTESIAN_POINT('Ctrl Pts',(-6.76248992368203,0.285234494207782,
117.683762764234));
#212476=CARTESIAN_POINT('Ctrl Pts',(-6.76699999999988,0.142617266095451,
117.690471274022));
#212477=CARTESIAN_POINT('Ctrl Pts',(-6.767,5.56759968767579E-12,117.69717978381));
#212478=CARTESIAN_POINT('',(-6.7669984993276,-0.00450667260642098,117.302820216158));
#212479=CARTESIAN_POINT('Ctrl Pts',(3.09910619832135,6.0156321173694,116.651219418659));
#212480=CARTESIAN_POINT('Ctrl Pts',(2.92867251040946,6.10343537533217,116.660251113336));
#212481=CARTESIAN_POINT('Ctrl Pts',(2.75459674554507,6.1839446942324,116.669282808013));
#212482=CARTESIAN_POINT('Ctrl Pts',(2.57749842811073,6.25689946004303,116.67831450269));
#212483=CARTESIAN_POINT('Ctrl Pts',(2.40016442018673,6.32995131737167,116.687358217157));
#212484=CARTESIAN_POINT('Ctrl Pts',(2.21980003807894,6.3954284291477,116.696401931623));
#212485=CARTESIAN_POINT('Ctrl Pts',(2.0370438345111,6.45311873564096,116.70544564609));
#212486=CARTESIAN_POINT('Ctrl Pts',(1.90676511509041,6.49424357357369,116.711892505438));
#212487=CARTESIAN_POINT('Ctrl Pts',(1.77527131444625,6.53141248191877,116.718339364787));
#212488=CARTESIAN_POINT('Ctrl Pts',(1.64279789201603,6.56456427236322,116.724786224136));
#212489=CARTESIAN_POINT('Ctrl Pts',(1.46498356534959,6.60906273241299,116.733439612364));
#212490=CARTESIAN_POINT('Ctrl Pts',(1.28524663887641,6.64636072291105,116.742093000592));
#212491=CARTESIAN_POINT('Ctrl Pts',(1.10418302950636,6.67630652661711,116.750746388821));
#212492=CARTESIAN_POINT('Ctrl Pts',(0.92328664522348,6.70622467324921,116.759391785031));
#212493=CARTESIAN_POINT('Ctrl Pts',(0.741066320808893,6.72880412698695,
116.768037181241));
#212494=CARTESIAN_POINT('Ctrl Pts',(0.558129023558517,6.7439440235712,116.776682577452));
#212495=CARTESIAN_POINT('Ctrl Pts',(0.369349325277105,6.75956743745204,
116.785604078494));
#212496=CARTESIAN_POINT('Ctrl Pts',(0.179806414240386,6.7672681523581,116.794525579537));
#212497=CARTESIAN_POINT('Ctrl Pts',(-0.00982353260787742,6.76699286967314,
116.803447080579));
#212498=CARTESIAN_POINT('Ctrl Pts',(-0.193234776334296,6.76672661457755,
116.812076010921));
#212499=CARTESIAN_POINT('Ctrl Pts',(-0.376727102741681,6.75899917527757,
116.820704941263));
#212500=CARTESIAN_POINT('Ctrl Pts',(-0.559685032912536,6.74381506744763,
116.829333871605));
#212501=CARTESIAN_POINT('Ctrl Pts',(-0.7519479628348,6.72785871585952,116.838401657998));
#212502=CARTESIAN_POINT('Ctrl Pts',(-0.943620383670555,6.70366742924272,
116.84746944439));
#212503=CARTESIAN_POINT('Ctrl Pts',(-1.13398931675573,6.67130850954173,
116.856537230783));
#212504=CARTESIAN_POINT('Ctrl Pts',(-1.32435824984104,6.63894958984072,
116.865605017176));
#212505=CARTESIAN_POINT('Ctrl Pts',(-1.51342330428553,6.59842306778905,
116.874672803568));
#212506=CARTESIAN_POINT('Ctrl Pts',(-1.7004785774534,6.54985966320059,116.883740589961));
#212507=CARTESIAN_POINT('Ctrl Pts',(-1.87427319531016,6.50473899806595,
116.892165546094));
#212508=CARTESIAN_POINT('Ctrl Pts',(-2.04625668617868,6.45270058691727,
116.900590502227));
#212509=CARTESIAN_POINT('Ctrl Pts',(-2.21586584529398,6.39392114086963,
116.90901545836));
#212510=CARTESIAN_POINT('Ctrl Pts',(-2.38551437232335,6.33512805154828,
116.917442370007));
#212511=CARTESIAN_POINT('Ctrl Pts',(-2.5527871554529,6.26959091621465,116.925869281653));
#212512=CARTESIAN_POINT('Ctrl Pts',(-2.71713896705784,6.19753538381959,
116.9342961933));
#212513=CARTESIAN_POINT('Ctrl Pts',(-2.88155121722582,6.12545335379853,
116.94272620385));
#212514=CARTESIAN_POINT('Ctrl Pts',(-3.04304005055162,6.04684828027295,
116.9511562144));
#212515=CARTESIAN_POINT('Ctrl Pts',(-3.2010825723603,5.96199290212016,116.95958622495));
#212516=CARTESIAN_POINT('Ctrl Pts',(-3.35927067963495,5.87705935696759,
116.968024001049));
#212517=CARTESIAN_POINT('Ctrl Pts',(-3.51400584031833,5.78586416088612,
116.976461777149));
#212518=CARTESIAN_POINT('Ctrl Pts',(-3.66479104208636,5.68872530694211,
116.984899553248));
#212519=CARTESIAN_POINT('Ctrl Pts',(-3.81565539497006,5.59153546226045,
116.993341758558));
#212520=CARTESIAN_POINT('Ctrl Pts',(-3.96256537950829,5.48839592322071,
117.001783963868));
#212521=CARTESIAN_POINT('Ctrl Pts',(-4.10505463089388,5.3796668556126,117.010226169178));
#212522=CARTESIAN_POINT('Ctrl Pts',(-4.24769420059981,5.27082308482052,
117.01867728055));
#212523=CARTESIAN_POINT('Ctrl Pts',(-4.38590346256215,5.15637821353292,
117.027128391922));
#212524=CARTESIAN_POINT('Ctrl Pts',(-4.51924985333012,5.0367320519535,117.035579503294));
#212525=CARTESIAN_POINT('Ctrl Pts',(-4.55667372445094,5.00315317137592,
117.037951320791));
#212526=CARTESIAN_POINT('Ctrl Pts',(-4.59371479524521,4.96916483055476,
117.040323138288));
#212527=CARTESIAN_POINT('Ctrl Pts',(-4.63036404117311,4.93477637246218,
117.042694955786));
#212528=CARTESIAN_POINT('Ctrl Pts',(-4.75612322711841,4.81677491332864,
117.050833672698));
#212529=CARTESIAN_POINT('Ctrl Pts',(-4.87752809522168,4.69381341047697,
117.05897238961));
#212530=CARTESIAN_POINT('Ctrl Pts',(-4.9941613067096,4.56625030441441,117.067111106523));
#212531=CARTESIAN_POINT('Ctrl Pts',(-5.11068809710025,4.43880359234927,
117.075242397324));
#212532=CARTESIAN_POINT('Ctrl Pts',(-5.22245165363688,4.30676390536643,
117.083373688126));
#212533=CARTESIAN_POINT('Ctrl Pts',(-5.32906974451272,4.17052810302474,
117.091504978927));
#212534=CARTESIAN_POINT('Ctrl Pts',(-5.43561306016616,4.03438784790524,
117.099630566952));
#212535=CARTESIAN_POINT('Ctrl Pts',(-5.53701787134075,3.89405762520549,
117.107756154978));
#212536=CARTESIAN_POINT('Ctrl Pts',(-5.63294069499284,3.7499690834317,117.115881743003));
#212537=CARTESIAN_POINT('Ctrl Pts',(-5.72882107426334,3.6059442986327,117.12400373558));
#212538=CARTESIAN_POINT('Ctrl Pts',(-5.81922409260315,3.45816481004148,
117.132125728157));
#212539=CARTESIAN_POINT('Ctrl Pts',(-5.9038482315136,3.30709314341972,117.140247720735));
#212540=CARTESIAN_POINT('Ctrl Pts',(-5.98845380005447,3.15605462876521,
117.148367930979));
#212541=CARTESIAN_POINT('Ctrl Pts',(-6.06728283432045,3.00172569360243,
117.156488141223));
#212542=CARTESIAN_POINT('Ctrl Pts',(-6.14007862740587,2.84459548077994,
117.164608351467));
#212543=CARTESIAN_POINT('Ctrl Pts',(-6.2128723581993,2.6874697194287,117.172728331666));
#212544=CARTESIAN_POINT('Ctrl Pts',(-6.27963303420768,2.52754317104278,
117.180848311866));
#212545=CARTESIAN_POINT('Ctrl Pts',(-6.34015118731402,2.36532702221082,
117.188968292066));
#212546=CARTESIAN_POINT('Ctrl Pts',(-6.40067919224474,2.20308446601299,
117.197089594128));
#212547=CARTESIAN_POINT('Ctrl Pts',(-6.45496252354291,2.03855191085368,
117.205210896189));
#212548=CARTESIAN_POINT('Ctrl Pts',(-6.50284089981284,1.87225778986797,
117.21333219825));
#212549=CARTESIAN_POINT('Ctrl Pts',(-6.55075870739758,1.70582671361466,
117.221460188793));
#212550=CARTESIAN_POINT('Ctrl Pts',(-6.59226092228593,1.53763152631706,
117.229588179336));
#212551=CARTESIAN_POINT('Ctrl Pts',(-6.62723775543208,1.36821370150117,
117.237716169878));
#212552=CARTESIAN_POINT('Ctrl Pts',(-6.66223011155152,1.19872068782076,
117.245847767682));
#212553=CARTESIAN_POINT('Ctrl Pts',(-6.6906912538452,1.02800431633688,117.253979365486));
#212554=CARTESIAN_POINT('Ctrl Pts',(-6.71256307327743,0.856613090766393,
117.26211096329));
#212555=CARTESIAN_POINT('Ctrl Pts',(-6.73446153202622,0.685013115067537,
117.270252465172));
#212556=CARTESIAN_POINT('Ctrl Pts',(-6.74975460336435,0.512737007993231,
117.278393967054));
#212557=CARTESIAN_POINT('Ctrl Pts',(-6.75843623491466,0.340336096517249,
117.286535468936));
#212558=CARTESIAN_POINT('Ctrl Pts',(-6.7642246089892,0.225389849301825,
117.29196371801));
#212559=CARTESIAN_POINT('Ctrl Pts',(-6.76707501674682,0.110388130318301,
117.297391967084));
#212560=CARTESIAN_POINT('Ctrl Pts',(-6.7669984993276,-0.00450667260661398,
117.302820216158));
#212561=CARTESIAN_POINT('Ctrl Pts',(-6.76699849932715,-0.00450667328524485,
117.30282021619));
#212562=CARTESIAN_POINT('Ctrl Pts',(-6.76678083879045,-0.331335008064387,
117.31826134634));
#212563=CARTESIAN_POINT('Ctrl Pts',(-6.74288468106681,-0.657266287959785,
117.33370247649));
#212564=CARTESIAN_POINT('Ctrl Pts',(-6.69570264497888,-0.979721945259407,
117.34914360664));
#212565=CARTESIAN_POINT('Ctrl Pts',(-6.68403014129684,-1.05949520557632,
117.352963633572));
#212566=CARTESIAN_POINT('Ctrl Pts',(-6.67093255580375,-1.13905600377084,
117.356783660503));
#212567=CARTESIAN_POINT('Ctrl Pts',(-6.65641602025991,-1.21836561229676,
117.360603687435));
#212568=CARTESIAN_POINT('Ctrl Pts',(-6.62574969030051,-1.38590797229451,
117.368673533438));
#212569=CARTESIAN_POINT('Ctrl Pts',(-6.58869694798007,-1.5526011436797,
117.37674337944));
#212570=CARTESIAN_POINT('Ctrl Pts',(-6.54530986498409,-1.71790796358302,
117.384813225443));
#212571=CARTESIAN_POINT('Ctrl Pts',(-6.50197736845718,-1.88300680648052,
117.392872918553));
#212572=CARTESIAN_POINT('Ctrl Pts',(-6.45232648168555,-2.04672241211413,
117.400932611663));
#212573=CARTESIAN_POINT('Ctrl Pts',(-6.39646086475483,-2.20852380690358,
117.408992304773));
#212574=CARTESIAN_POINT('Ctrl Pts',(-6.34065327314052,-2.37015714524538,
117.417043626612));
#212575=CARTESIAN_POINT('Ctrl Pts',(-6.27864391757971,-2.52987987964089,
117.425094948451));
#212576=CARTESIAN_POINT('Ctrl Pts',(-6.21058721372502,-2.68717239132798,
117.433146270289));
#212577=CARTESIAN_POINT('Ctrl Pts',(-6.14258628402404,-2.84433599790761,
117.44119099387));
#212578=CARTESIAN_POINT('Ctrl Pts',(-6.06854801736682,-2.99907300508787,
117.449235717451));
#212579=CARTESIAN_POINT('Ctrl Pts',(-5.98867622569187,-3.15088020461473,
117.457280441032));
#212580=CARTESIAN_POINT('Ctrl Pts',(-5.90885240695776,-3.30259622504508,
117.465320332757));
#212581=CARTESIAN_POINT('Ctrl Pts',(-5.82320221138867,-3.45138561151586,
117.473360224481));
#212582=CARTESIAN_POINT('Ctrl Pts',(-5.73197697556836,-3.59676645774426,
117.481400116206));
#212583=CARTESIAN_POINT('Ctrl Pts',(-5.63878741049257,-3.74527775188946,
117.489613128826));
#212584=CARTESIAN_POINT('Ctrl Pts',(-5.53978014798251,-3.8902316843531,
117.497826141446));
#212585=CARTESIAN_POINT('Ctrl Pts',(-5.43527212771515,-4.03114200911886,
117.506039154066));
#212586=CARTESIAN_POINT('Ctrl Pts',(-5.33300271183239,-4.16903397730253,
117.514076240608));
#212587=CARTESIAN_POINT('Ctrl Pts',(-5.22546604999359,-4.30305350997931,
117.522113327151));
#212588=CARTESIAN_POINT('Ctrl Pts',(-5.11300206604545,-4.4327755269825,
117.530150413693));
#212589=CARTESIAN_POINT('Ctrl Pts',(-5.00052731877043,-4.56250995898668,
117.538188269423));
#212590=CARTESIAN_POINT('Ctrl Pts',(-4.88312455507379,-4.68794577397006,
117.546226125152));
#212591=CARTESIAN_POINT('Ctrl Pts',(-4.76117275337515,-4.80869244311987,
117.554263980881));
#212592=CARTESIAN_POINT('Ctrl Pts',(-4.63918511759793,-4.92947459223446,
117.562304198438));
#212593=CARTESIAN_POINT('Ctrl Pts',(-4.51264604855618,-5.04556459022498,
117.570344415995));
#212594=CARTESIAN_POINT('Ctrl Pts',(-4.3819698787759,-5.15661022198699,
117.578384633552));
#212595=CARTESIAN_POINT('Ctrl Pts',(-4.24635667957483,-5.27185122886583,
117.58672861568));
#212596=CARTESIAN_POINT('Ctrl Pts',(-4.10628800815647,-5.38165897753822,
117.595072597807));
#212597=CARTESIAN_POINT('Ctrl Pts',(-3.96226176371165,-5.48568780699637,
117.603416579935));
#212598=CARTESIAN_POINT('Ctrl Pts',(-3.82323721920956,-5.58610395466622,
117.61147079477));
#212599=CARTESIAN_POINT('Ctrl Pts',(-3.68052571141551,-5.68113568281839,
117.619525009605));
#212600=CARTESIAN_POINT('Ctrl Pts',(-3.53460141385745,-5.77051833418428,
117.62757922444));
#212601=CARTESIAN_POINT('Ctrl Pts',(-3.38856791609294,-5.85996787368426,
117.635639466523));
#212602=CARTESIAN_POINT('Ctrl Pts',(-3.23931716494388,-5.94375973746419,
117.643699708606));
#212603=CARTESIAN_POINT('Ctrl Pts',(-3.08734519441779,-6.02167656475382,
117.651759950689));
#212604=CARTESIAN_POINT('Ctrl Pts',(-2.93516075665225,-6.09970232511277,
117.659831461544));
#212605=CARTESIAN_POINT('Ctrl Pts',(-2.78024784445155,-6.17183650501122,
117.667902972398));
#212606=CARTESIAN_POINT('Ctrl Pts',(-2.62312011777808,-6.23791069571438,
117.675974483252));
#212607=CARTESIAN_POINT('Ctrl Pts',(-2.60665149147746,-6.24483596077004,
117.676820461863));
#212608=CARTESIAN_POINT('Ctrl Pts',(-2.59015854606553,-6.25169470131863,
117.677666440474));
#212609=CARTESIAN_POINT('Ctrl Pts',(-2.57364188029386,-6.25848675575794,
117.678512419085));
#212610=CARTESIAN_POINT('Ctrl Pts',(-2.41297615459709,-6.32455640749932,
117.686741668821));
#212611=CARTESIAN_POINT('Ctrl Pts',(-2.24952853096778,-6.3845323363346,
117.694970918557));
#212612=CARTESIAN_POINT('Ctrl Pts',(-2.08380125520086,-6.43817220403612,
117.703200168293));
#212613=CARTESIAN_POINT('Ctrl Pts',(-1.91827122185263,-6.49174823156894,
117.711419623883));
#212614=CARTESIAN_POINT('Ctrl Pts',(-1.750467276677,-6.53900310420169,117.719639079473));
#212615=CARTESIAN_POINT('Ctrl Pts',(-1.58091304563219,-6.57974185984146,
117.727858535063));
#212616=CARTESIAN_POINT('Ctrl Pts',(-1.41152656104436,-6.62044031107905,
117.736069858833));
#212617=CARTESIAN_POINT('Ctrl Pts',(-1.24039358538537,-6.65463540043232,
117.744281182602));
#212618=CARTESIAN_POINT('Ctrl Pts',(-1.06805445592739,-6.68218143117752,
117.752492506372));
#212619=CARTESIAN_POINT('Ctrl Pts',(-0.895851230706605,-6.70970573950653,
117.760697354806));
#212620=CARTESIAN_POINT('Ctrl Pts',(-0.722444098717129,-6.73059137639154,
117.76890220324));
#212621=CARTESIAN_POINT('Ctrl Pts',(-0.548385275521854,-6.74474333014911,
117.777107051674));
#212622=CARTESIAN_POINT('Ctrl Pts',(-0.374428779043003,-6.75888696417354,
117.785307076594));
#212623=CARTESIAN_POINT('Ctrl Pts',(-0.19982171108126,-6.76630477208352,
117.793507101514));
#212624=CARTESIAN_POINT('Ctrl Pts',(-0.0251232157561799,-6.76695336351819,
117.801707126434));
#212625=CARTESIAN_POINT('Ctrl Pts',(0.149524717866146,-6.76760176723579,
117.809904778081));
#212626=CARTESIAN_POINT('Ctrl Pts',(0.324263667964969,-6.76148485159074,
117.818102429728));
#212627=CARTESIAN_POINT('Ctrl Pts',(0.49853241511165,-6.74861129648782,
117.826300081375));
#212628=CARTESIAN_POINT('Ctrl Pts',(0.672777826603831,-6.73573946523291,
117.834496635306));
#212629=CARTESIAN_POINT('Ctrl Pts',(0.846552802823156,-6.71611282203787,
117.842693189237));
#212630=CARTESIAN_POINT('Ctrl Pts',(1.01929916428635,-6.68979209046777,
117.850889743168));
#212631=CARTESIAN_POINT('Ctrl Pts',(1.19205380372901,-6.66347009761221,
117.859086689877));
#212632=CARTESIAN_POINT('Ctrl Pts',(1.36377937552539,-6.63045343129485,
117.867283636585));
#212633=CARTESIAN_POINT('Ctrl Pts',(1.53392578365535,-6.59085432172775,
117.875480583294));
#212634=CARTESIAN_POINT('Ctrl Pts',(1.70411128214523,-6.55124611444614,
117.883679413214));
#212635=CARTESIAN_POINT('Ctrl Pts',(1.87271654503031,-6.50505253320008,
117.891878243133));
#212636=CARTESIAN_POINT('Ctrl Pts',(2.03920452446303,-6.45243627689647,
117.900077073053));
#212637=CARTESIAN_POINT('Ctrl Pts',(2.20585018929581,-6.39977018627176,
117.908283668313));
#212638=CARTESIAN_POINT('Ctrl Pts',(2.37037422167481,-6.34066937537288,
117.916490263573));
#212639=CARTESIAN_POINT('Ctrl Pts',(2.53225662902831,-6.27534583626609,
117.924696858833));
#212640=CARTESIAN_POINT('Ctrl Pts',(2.69421738839498,-6.2099906801919,117.932907426132));
#212641=CARTESIAN_POINT('Ctrl Pts',(2.85353364655053,-6.13840693797222,
117.941117993431));
#212642=CARTESIAN_POINT('Ctrl Pts',(3.00970816508193,-6.06085355053553,
117.949328560729));
#212643=CARTESIAN_POINT('Ctrl Pts',(3.16609807063245,-5.98319320587497,
117.957550451576));
#212644=CARTESIAN_POINT('Ctrl Pts',(3.31933726223946,-5.89954693422829,
117.965772342423));
#212645=CARTESIAN_POINT('Ctrl Pts',(3.46895468302242,-5.8102187916753,117.97399423327));
#212646=CARTESIAN_POINT('Ctrl Pts',(3.6049922283895,-5.72899842855505,117.981469872424));
#212647=CARTESIAN_POINT('Ctrl Pts',(3.73803581094111,-5.64308146275042,
117.988945511579));
#212648=CARTESIAN_POINT('Ctrl Pts',(3.86775460434079,-5.5527257559329,117.996421150734));
#212649=CARTESIAN_POINT('Ctrl Pts',(4.02281289143836,-5.44471980890373,
118.005357094185));
#212650=CARTESIAN_POINT('Ctrl Pts',(4.17344342205021,-5.33014657741647,
118.014293037636));
#212651=CARTESIAN_POINT('Ctrl Pts',(4.31910750648569,-5.20937609963218,
118.023228981086));
#212652=CARTESIAN_POINT('Ctrl Pts',(4.46455261916716,-5.08878717190847,
118.032151491444));
#212653=CARTESIAN_POINT('Ctrl Pts',(4.60504598436316,-4.96201975113923,
118.041074001802));
#212654=CARTESIAN_POINT('Ctrl Pts',(4.74008005023805,-4.82948549198931,
118.049996512159));
#212655=CARTESIAN_POINT('Ctrl Pts',(4.87478324074672,-4.69727598290337,
118.058897159598));
#212656=CARTESIAN_POINT('Ctrl Pts',(5.00405364606396,-4.55932801802952,
118.067797807036));
#212657=CARTESIAN_POINT('Ctrl Pts',(5.12741923145142,-4.41609114771674,
118.076698454474));
#212658=CARTESIAN_POINT('Ctrl Pts',(5.25059417055246,-4.27307563230872,
118.085585347061));
#212659=CARTESIAN_POINT('Ctrl Pts',(5.36788232438541,-4.12478770982086,
118.094472239647));
#212660=CARTESIAN_POINT('Ctrl Pts',(5.4788486447128,-3.9717132988584,118.103359132233));
#212661=CARTESIAN_POINT('Ctrl Pts',(5.58952974017444,-3.81903234627313,
118.112223182188));
#212662=CARTESIAN_POINT('Ctrl Pts',(5.69392127573436,-3.6615896635484,118.121087232143));
#212663=CARTESIAN_POINT('Ctrl Pts',(5.79162907117197,-3.49990309893799,
118.129951282098));
#212664=CARTESIAN_POINT('Ctrl Pts',(5.88504558365832,-3.34531773638677,
118.138426026918));
#212665=CARTESIAN_POINT('Ctrl Pts',(5.97235265936608,-3.18685345741418,
118.146900771739));
#212666=CARTESIAN_POINT('Ctrl Pts',(6.05324029812882,-3.02499105669906,
118.155375516559));
#212667=CARTESIAN_POINT('Ctrl Pts',(6.13159070502032,-2.86820585255108,
118.163584430988));
#212668=CARTESIAN_POINT('Ctrl Pts',(6.20384168534277,-2.70838306178184,
118.171793345417));
#212669=CARTESIAN_POINT('Ctrl Pts',(6.26976644258405,-2.54603962173548,
118.180002259846));
#212670=CARTESIAN_POINT('Ctrl Pts',(6.33570687310144,-2.38365758536103,
118.188213125903));
#212671=CARTESIAN_POINT('Ctrl Pts',(6.39531795011633,-2.218754035716,118.19642399196));
#212672=CARTESIAN_POINT('Ctrl Pts',(6.44842162997804,-2.05186439172557,
118.204634858017));
#212673=CARTESIAN_POINT('Ctrl Pts',(6.50154740092355,-1.88490532179105,
118.212849139787));
#212674=CARTESIAN_POINT('Ctrl Pts',(6.54816027377841,-1.71595885055863,
118.221063421556));
#212675=CARTESIAN_POINT('Ctrl Pts',(6.5881324939963,-1.54557408154707,118.229277703326));
#212676=CARTESIAN_POINT('Ctrl Pts',(6.62814970610357,-1.37499753102733,
118.237501230919));
#212677=CARTESIAN_POINT('Ctrl Pts',(6.66151125501597,-1.20297979601922,
118.245724758511));
#212678=CARTESIAN_POINT('Ctrl Pts',(6.68814062014948,-1.03007963046874,
118.253948286103));
#212679=CARTESIAN_POINT('Ctrl Pts',(6.71478705367018,-0.857068642637813,
118.262177084657));
#212680=CARTESIAN_POINT('Ctrl Pts',(6.73469266120561,-0.683174449622825,
118.270405883211));
#212681=CARTESIAN_POINT('Ctrl Pts',(6.74783293990576,-0.508959345255335,
118.278634681765));
#212682=CARTESIAN_POINT('Ctrl Pts',(6.76099130514803,-0.334504447737934,
118.286874806601));
#212683=CARTESIAN_POINT('Ctrl Pts',(6.76736572887999,-0.159728111396207,
118.295114931437));
#212684=CARTESIAN_POINT('Ctrl Pts',(6.7669837981931,0.0148079367960404,
118.303355056274));
#212685=CARTESIAN_POINT('Ctrl Pts',(6.76681423672981,0.0922947393577986,
118.307013331644));
#212686=CARTESIAN_POINT('Ctrl Pts',(6.76531368755961,0.169734251754895,
118.310671607014));
#212687=CARTESIAN_POINT('Ctrl Pts',(6.76248782396277,0.247077782803955,
118.314329882384));
#212688=CARTESIAN_POINT('Ctrl Pts',(6.75596208230168,0.425686510891996,
118.322777905146));
#212689=CARTESIAN_POINT('Ctrl Pts',(6.74235031320975,0.604191627816968,
118.331225927909));
#212690=CARTESIAN_POINT('Ctrl Pts',(6.72166304232655,0.782006998319967,
118.339673950672));
#212691=CARTESIAN_POINT('Ctrl Pts',(6.70099471539513,0.959659537977716,
118.348114237327));
#212692=CARTESIAN_POINT('Ctrl Pts',(6.67326384008797,1.13662326053509,118.356554523983));
#212693=CARTESIAN_POINT('Ctrl Pts',(6.63853290694353,1.31231468917632,118.364994810639));
#212694=CARTESIAN_POINT('Ctrl Pts',(6.6038284313199,1.48787227863704,118.373428667607));
#212695=CARTESIAN_POINT('Ctrl Pts',(6.56213459275031,1.66215918028363,118.381862524575));
#212696=CARTESIAN_POINT('Ctrl Pts',(6.51356541899638,1.83459928389132,118.390296381543));
#212697=CARTESIAN_POINT('Ctrl Pts',(6.46502577782156,2.00693453496379,118.398725110288));
#212698=CARTESIAN_POINT('Ctrl Pts',(6.40961922657633,2.17742490662948,118.407153839033));
#212699=CARTESIAN_POINT('Ctrl Pts',(6.34751047084745,2.34550630408062,118.415582567778));
#212700=CARTESIAN_POINT('Ctrl Pts',(6.28542994286655,2.51351131038094,118.424007465758));
#212701=CARTESIAN_POINT('Ctrl Pts',(6.21665339970778,2.67910921329788,118.432432363738));
#212702=CARTESIAN_POINT('Ctrl Pts',(6.14139494116504,2.84175248335115,118.440857261719));
#212703=CARTESIAN_POINT('Ctrl Pts',(6.06615314496755,3.00435974391965,118.449280294413));
#212704=CARTESIAN_POINT('Ctrl Pts',(5.98443243223829,3.16401337239285,118.457703327107));
#212705=CARTESIAN_POINT('Ctrl Pts',(5.89649466467768,3.32018669195388,118.466126359801));
#212706=CARTESIAN_POINT('Ctrl Pts',(5.80856684717554,3.47634234068128,118.474548439439));
#212707=CARTESIAN_POINT('Ctrl Pts',(5.71442354079235,3.62901817502473,118.482970519076));
#212708=CARTESIAN_POINT('Ctrl Pts',(5.61437225641073,3.77771268976951,118.491392598714));
#212709=CARTESIAN_POINT('Ctrl Pts',(5.5143183263064,3.92641113654229,118.499814901062));
#212710=CARTESIAN_POINT('Ctrl Pts',(5.40835629320467,4.07112777735644,118.50823720341));
#212711=CARTESIAN_POINT('Ctrl Pts',(5.29683683583468,4.21139033272206,118.516659505759));
#212712=CARTESIAN_POINT('Ctrl Pts',(5.18529886129325,4.35167617788703,118.525083206582));
#212713=CARTESIAN_POINT('Ctrl Pts',(5.06820183071655,4.48750620249545,118.533506907406));
#212714=CARTESIAN_POINT('Ctrl Pts',(4.94593674310747,4.61844115835413,118.54193060823));
#212715=CARTESIAN_POINT('Ctrl Pts',(4.82358891759602,4.74946471909428,118.550360009448));
#212716=CARTESIAN_POINT('Ctrl Pts',(4.69606627448414,4.87558634785518,118.558789410668));
#212717=CARTESIAN_POINT('Ctrl Pts',(4.56379742723748,4.9964029104087,118.567218811887));
#212718=CARTESIAN_POINT('Ctrl Pts',(4.43148138664995,5.11726258014383,118.575651220704));
#212719=CARTESIAN_POINT('Ctrl Pts',(4.29441601564268,5.23281318910369,118.584083629522));
#212720=CARTESIAN_POINT('Ctrl Pts',(4.15306348123833,5.34269152401714,118.592516038339));
#212721=CARTESIAN_POINT('Ctrl Pts',(4.01158016335622,5.45267152156317,118.600956249067));
#212722=CARTESIAN_POINT('Ctrl Pts',(3.86580202399501,5.5569685594087,118.609396459795));
#212723=CARTESIAN_POINT('Ctrl Pts',(3.71622161234702,5.65526179128119,118.617836670522));
#212724=CARTESIAN_POINT('Ctrl Pts',(3.63114282666162,5.71116930428152,118.622637318359));
#212725=CARTESIAN_POINT('Ctrl Pts',(3.54483446078583,5.76513530901095,118.627437966196));
#212726=CARTESIAN_POINT('Ctrl Pts',(3.45739080292736,5.81710734264319,118.632238614033));
#212727=CARTESIAN_POINT('Ctrl Pts',(3.34011458148202,5.8868103248204,118.638677066548));
#212728=CARTESIAN_POINT('Ctrl Pts',(3.22061103733692,5.9530358029053,118.645115519062));
#212729=CARTESIAN_POINT('Ctrl Pts',(3.09910619832126,6.01563211736944,118.651553971577));
#212730=CARTESIAN_POINT('Origin',(0.,0.,4.30282021618968));
#212731=CARTESIAN_POINT('',(3.09910619832141,6.01563211736936,121.045612484544));
#212732=CARTESIAN_POINT('',(3.09910619832143,6.01563211736935,120.651489390257));
#212733=CARTESIAN_POINT('',(3.09910619832133,6.0156321173694,4.30282021618968));
#212734=CARTESIAN_POINT('',(-6.76699914956147,0.00339261468657372,119.697179783785));
#212735=CARTESIAN_POINT('Ctrl Pts',(-6.76699914956174,0.00339261414470956,
119.69717978381));
#212736=CARTESIAN_POINT('Ctrl Pts',(-6.76708137641015,-0.160619262692798,
119.704869165924));
#212737=CARTESIAN_POINT('Ctrl Pts',(-6.76119737850267,-0.324736712568498,
119.712558548038));
#212738=CARTESIAN_POINT('Ctrl Pts',(-6.74934578577639,-0.488487936414527,
119.720247930153));
#212739=CARTESIAN_POINT('Ctrl Pts',(-6.73669344140177,-0.663302994923102,
119.728456844582));
#212740=CARTESIAN_POINT('Ctrl Pts',(-6.71724560558489,-0.837616821938097,
119.736665759011));
#212741=CARTESIAN_POINT('Ctrl Pts',(-6.69107111035296,-1.01086912911614,
119.74487467344));
#212742=CARTESIAN_POINT('Ctrl Pts',(-6.66489039226773,-1.18416262615027,
119.753085539497));
#212743=CARTESIAN_POINT('Ctrl Pts',(-6.63197988184707,-1.35639374846011,
119.761296405554));
#212744=CARTESIAN_POINT('Ctrl Pts',(-6.59245976822417,-1.52701119981019,
119.769507271611));
#212745=CARTESIAN_POINT('Ctrl Pts',(-6.55292321426923,-1.69769962786792,
119.77772155338));
#212746=CARTESIAN_POINT('Ctrl Pts',(-6.50677165963721,-1.86677270101151,
119.78593583515));
#212747=CARTESIAN_POINT('Ctrl Pts',(-6.4541755230999,-2.0336930242832,119.79415011692));
#212748=CARTESIAN_POINT('Ctrl Pts',(-6.4015201854586,-2.20080122955663,
119.802373644512));
#212749=CARTESIAN_POINT('Ctrl Pts',(-6.3424058845656,-2.36575150549719,
119.810597172105));
#212750=CARTESIAN_POINT('Ctrl Pts',(-6.27705202218472,-2.52802430976974,
119.818820699697));
#212751=CARTESIAN_POINT('Ctrl Pts',(-6.2116562705203,-2.69040112459744,
119.827049498251));
#212752=CARTESIAN_POINT('Ctrl Pts',(-6.14001313035681,-2.85009672266746,
119.835278296805));
#212753=CARTESIAN_POINT('Ctrl Pts',(-6.06238854144283,-3.00661506890768,
119.843507095358));
#212754=CARTESIAN_POINT('Ctrl Pts',(-5.98465710849403,-3.16334885012628,
119.851747220195));
#212755=CARTESIAN_POINT('Ctrl Pts',(-5.90092795213283,-3.3168963326771,
119.859987345031));
#212756=CARTESIAN_POINT('Ctrl Pts',(-5.81151151599038,-3.4667885570815,
119.868227469867));
#212757=CARTESIAN_POINT('Ctrl Pts',(-5.77181430842122,-3.53333451889667,
119.871885745237));
#212758=CARTESIAN_POINT('Ctrl Pts',(-5.73099669508534,-3.5991604421339,
119.875544020608));
#212759=CARTESIAN_POINT('Ctrl Pts',(-5.68908840787528,-3.66422735203196,
119.879202295978));
#212760=CARTESIAN_POINT('Ctrl Pts',(-5.59230997310274,-3.81448578812258,
119.88765031874));
#212761=CARTESIAN_POINT('Ctrl Pts',(-5.48949100218155,-3.9610382232606,
119.896098341503));
#212762=CARTESIAN_POINT('Ctrl Pts',(-5.38093972590706,-4.10338600014126,
119.904546364265));
#212763=CARTESIAN_POINT('Ctrl Pts',(-5.27248785327816,-4.24560342491138,
119.912986650921));
#212764=CARTESIAN_POINT('Ctrl Pts',(-5.15831433985564,-4.38362360234712,
119.921426937577));
#212765=CARTESIAN_POINT('Ctrl Pts',(-5.03877074518791,-4.51697668550973,
119.929867224233));
#212766=CARTESIAN_POINT('Ctrl Pts',(-4.91931821709575,-4.65022818222885,
119.9383010812));
#212767=CARTESIAN_POINT('Ctrl Pts',(-4.79450398471884,-4.77881942476241,
119.946734938168));
#212768=CARTESIAN_POINT('Ctrl Pts',(-4.66472016542312,-4.90231320687437,
119.955168795136));
#212769=CARTESIAN_POINT('Ctrl Pts',(-4.53501526142728,-5.02573189835563,
119.963597523881));
#212770=CARTESIAN_POINT('Ctrl Pts',(-4.40034703612036,-5.14405907969709,
119.972026252626));
#212771=CARTESIAN_POINT('Ctrl Pts',(-4.26114505278284,-5.256893744327,119.980454981371));
#212772=CARTESIAN_POINT('Ctrl Pts',(-4.12200633521901,-5.3696771268402,
119.988879879351));
#212773=CARTESIAN_POINT('Ctrl Pts',(-3.97833822701335,-5.47697276060053,
119.997304777332));
#212774=CARTESIAN_POINT('Ctrl Pts',(-3.83060431115137,-5.57841909606911,
120.005729675312));
#212775=CARTESIAN_POINT('Ctrl Pts',(-3.68290310381919,-5.67984297115365,
120.014152708006));
#212776=CARTESIAN_POINT('Ctrl Pts',(-3.53113815678626,-5.77541993922471,
120.0225757407));
#212777=CARTESIAN_POINT('Ctrl Pts',(-3.3758034807196,-5.86483076137423,
120.030998773394));
#212778=CARTESIAN_POINT('Ctrl Pts',(-3.22048638059502,-5.95423146679083,
120.039420853032));
#212779=CARTESIAN_POINT('Ctrl Pts',(-3.06160064560909,-6.03746725084514,
120.04784293267));
#212780=CARTESIAN_POINT('Ctrl Pts',(-2.89966669282957,-6.11426382081235,
120.056265012307));
#212781=CARTESIAN_POINT('Ctrl Pts',(-2.73772845792289,-6.19106242156231,
120.064687314655));
#212782=CARTESIAN_POINT('Ctrl Pts',(-2.57274214598494,-6.26142132619124,
120.073109617004));
#212783=CARTESIAN_POINT('Ctrl Pts',(-2.40525037739631,-6.32511340783981,
120.081531919352));
#212784=CARTESIAN_POINT('Ctrl Pts',(-2.23773079775204,-6.38881606519631,
120.089955620175));
#212785=CARTESIAN_POINT('Ctrl Pts',(-2.06770524391366,-6.44584957461821,
120.098379320999));
#212786=CARTESIAN_POINT('Ctrl Pts',(-1.89573414841888,-6.49603579412233,
120.106803021823));
#212787=CARTESIAN_POINT('Ctrl Pts',(-1.72364667851209,-6.54625597509986,
120.115232423042));
#212788=CARTESIAN_POINT('Ctrl Pts',(-1.54961135657742,-6.58961951354594,
120.123661824261));
#212789=CARTESIAN_POINT('Ctrl Pts',(-1.37420252704782,-6.6259985220837,
120.13209122548));
#212790=CARTESIAN_POINT('Ctrl Pts',(-1.1987311118915,-6.66239051060118,
120.140523634297));
#212791=CARTESIAN_POINT('Ctrl Pts',(-1.02188553972036,-6.6917929384565,
120.148956043115));
#212792=CARTESIAN_POINT('Ctrl Pts',(-0.844248631611878,-6.71412937379237,
120.157388451933));
#212793=CARTESIAN_POINT('Ctrl Pts',(-0.666447368667443,-6.73648647544811,
120.16582866266));
#212794=CARTESIAN_POINT('Ctrl Pts',(-0.487853638694062,-6.75176448687257,
120.174268873388));
#212795=CARTESIAN_POINT('Ctrl Pts',(-0.309054763744897,-6.75993891636652,
120.182709084115));
#212796=CARTESIAN_POINT('Ctrl Pts',(-0.207357014719193,-6.76458839237324,
120.187509731952));
#212797=CARTESIAN_POINT('Ctrl Pts',(-0.105592923447541,-6.76694071350546,
120.19231037979));
#212798=CARTESIAN_POINT('Ctrl Pts',(-0.00387034878925978,-6.76699889318746,
120.197111027627));
#212799=CARTESIAN_POINT('Ctrl Pts',(0.168604866686761,-6.76709753946359,
120.20525074266));
#212800=CARTESIAN_POINT('Ctrl Pts',(0.341304484230173,-6.76059800410953,
120.213390457692));
#212801=CARTESIAN_POINT('Ctrl Pts',(0.513678841380611,-6.74747530917438,
120.221530172725));
#212802=CARTESIAN_POINT('Ctrl Pts',(0.685902440952836,-6.73436409126946,
120.229662768812));
#212803=CARTESIAN_POINT('Ctrl Pts',(0.857800983717736,-6.71464127147748,
120.237795364899));
#212804=CARTESIAN_POINT('Ctrl Pts',(1.02882394771252,-6.68833389452211,
120.245927960986));
#212805=CARTESIAN_POINT('Ctrl Pts',(1.19972999123408,-6.66204450270096,
120.254054997194));
#212806=CARTESIAN_POINT('Ctrl Pts',(1.3697612872857,-6.62917957153362,120.262182033402));
#212807=CARTESIAN_POINT('Ctrl Pts',(1.53837162302158,-6.58981803614348,
120.27030906961));
#212808=CARTESIAN_POINT('Ctrl Pts',(1.70690135996525,-6.55047531627968,
120.278432220948));
#212809=CARTESIAN_POINT('Ctrl Pts',(1.87401113332999,-6.50464225932621,
120.286555372285));
#212810=CARTESIAN_POINT('Ctrl Pts',(2.03916414515222,-6.45244903808822,
120.294678523623));
#212811=CARTESIAN_POINT('Ctrl Pts',(2.20427074775036,-6.40027048353341,
120.302799392295));
#212812=CARTESIAN_POINT('Ctrl Pts',(2.36742133538362,-6.3417354355619,120.310920260966));
#212813=CARTESIAN_POINT('Ctrl Pts',(2.52809355277149,-6.27702413476603,
120.319041129638));
#212814=CARTESIAN_POINT('Ctrl Pts',(2.68877445350089,-6.21230933672381,
120.327162437193));
#212815=CARTESIAN_POINT('Ctrl Pts',(2.84697637520379,-6.14141775214237,
120.335283744747));
#212816=CARTESIAN_POINT('Ctrl Pts',(3.00219608130839,-6.06457811305754,
120.343405052302));
#212817=CARTESIAN_POINT('Ctrl Pts',(3.08285363631955,-6.0246495655035,120.347625166018));
#212818=CARTESIAN_POINT('Ctrl Pts',(3.16270627987442,-5.98311570679573,
120.351845279735));
#212819=CARTESIAN_POINT('Ctrl Pts',(3.24168590658268,-5.94001359283489,
120.356065393452));
#212820=CARTESIAN_POINT('Ctrl Pts',(3.40983009619075,-5.84825106717607,
120.365049831978));
#212821=CARTESIAN_POINT('Ctrl Pts',(3.57393262566276,-5.74942348196402,
120.374034270503));
#212822=CARTESIAN_POINT('Ctrl Pts',(3.73343998016136,-5.64390954166815,
120.383018709029));
#212823=CARTESIAN_POINT('Ctrl Pts',(3.89322263483352,-5.538213490609,120.39201865416));
#212824=CARTESIAN_POINT('Ctrl Pts',(4.04839406327755,-5.42580815047542,
120.40101859929));
#212825=CARTESIAN_POINT('Ctrl Pts',(4.19843172366319,-5.30711409918221,
120.410018544421));
#212826=CARTESIAN_POINT('Ctrl Pts',(4.34882295164683,-5.18814034231037,
120.419039698153));
#212827=CARTESIAN_POINT('Ctrl Pts',(4.49405601755882,-5.0628483717073,120.428060851885));
#212828=CARTESIAN_POINT('Ctrl Pts',(4.63364125361111,-4.93169927437118,
120.437082005617));
#212829=CARTESIAN_POINT('Ctrl Pts',(4.77336851874162,-4.80041673179451,
120.446112338444));
#212830=CARTESIAN_POINT('Ctrl Pts',(4.9074363036084,-4.66326532437559,120.455142671272));
#212831=CARTESIAN_POINT('Ctrl Pts',(5.03539245172121,-4.52074240110505,
120.464173004099));
#212832=CARTESIAN_POINT('Ctrl Pts',(5.16353000131758,-4.37801742525553,
120.473216139091));
#212833=CARTESIAN_POINT('Ctrl Pts',(5.28553842981156,-4.22990588485169,
120.482259274084));
#212834=CARTESIAN_POINT('Ctrl Pts',(5.40100496908738,-4.0769393328689,120.491302409077));
#212835=CARTESIAN_POINT('Ctrl Pts',(5.50194932634741,-3.94321132500592,
120.499208192477));
#212836=CARTESIAN_POINT('Ctrl Pts',(5.59789442793137,-3.80577330207824,
120.507113975876));
#212837=CARTESIAN_POINT('Ctrl Pts',(5.68859152615184,-3.66499869694295,
120.515019759276));
#212838=CARTESIAN_POINT('Ctrl Pts',(5.78786533146371,-3.51091184061282,
120.523673147504));
#212839=CARTESIAN_POINT('Ctrl Pts',(5.88093826684653,-3.35269069306102,
120.532326535733));
#212840=CARTESIAN_POINT('Ctrl Pts',(5.9674751812739,-3.19085082084388,120.540979923961));
#212841=CARTESIAN_POINT('Ctrl Pts',(6.05393217272209,-3.02916041922923,
120.549625320171));
#212842=CARTESIAN_POINT('Ctrl Pts',(6.13386504024526,-2.86385822610878,
120.558270716382));
#212843=CARTESIAN_POINT('Ctrl Pts',(6.20698323842898,-2.69548661244342,
120.566916112592));
#212844=CARTESIAN_POINT('Ctrl Pts',(6.2824365855564,-2.52173777661496,120.575837613634));
#212845=CARTESIAN_POINT('Ctrl Pts',(6.35063259972096,-2.34472048992701,
120.584759114677));
#212846=CARTESIAN_POINT('Ctrl Pts',(6.41130354045417,-2.16505794660555,
120.593680615719));
#212847=CARTESIAN_POINT('Ctrl Pts',(6.46998484518969,-1.99128723649631,
120.602309546061));
#212848=CARTESIAN_POINT('Ctrl Pts',(6.52162667706992,-1.81504232630351,
120.610938476403));
#212849=CARTESIAN_POINT('Ctrl Pts',(6.56603554749569,-1.63690750777894,
120.619567406745));
#212850=CARTESIAN_POINT('Ctrl Pts',(6.61270299467635,-1.44971298662063,
120.628635193138));
#212851=CARTESIAN_POINT('Ctrl Pts',(6.65138245437574,-1.26043162289371,
120.63770297953));
#212852=CARTESIAN_POINT('Ctrl Pts',(6.68190856630119,-1.06976021219282,
120.646770765923));
#212853=CARTESIAN_POINT('Ctrl Pts',(6.71243467822665,-0.879088801491813,
120.655838552316));
#212854=CARTESIAN_POINT('Ctrl Pts',(6.73480734588162,-0.687027723853866,
120.664906338708));
#212855=CARTESIAN_POINT('Ctrl Pts',(6.74892353752581,-0.494287451418825,
120.673974125101));
#212856=CARTESIAN_POINT('Ctrl Pts',(6.76203900917683,-0.315210853222223,
120.682399081234));
#212857=CARTESIAN_POINT('Ctrl Pts',(6.76802162613719,-0.135626539707275,
120.690824037367));
#212858=CARTESIAN_POINT('Ctrl Pts',(6.76685776057962,0.0438753698941443,
120.699248993501));
#212859=CARTESIAN_POINT('Ctrl Pts',(6.76569362487769,0.223418943612258,
120.707675905147));
#212860=CARTESIAN_POINT('Ctrl Pts',(6.75737970147142,0.402879743681405,
120.716102816793));
#212861=CARTESIAN_POINT('Ctrl Pts',(6.74195448164165,0.581668950066981,
120.72452972844));
#212862=CARTESIAN_POINT('Ctrl Pts',(6.72652358935783,0.760523904206612,
120.73295973899));
#212863=CARTESIAN_POINT('Ctrl Pts',(6.70397621487706,0.938706442005982,
120.74138974954));
#212864=CARTESIAN_POINT('Ctrl Pts',(6.67440261827401,1.11563376122145,120.74981976009));
#212865=CARTESIAN_POINT('Ctrl Pts',(6.64480177909213,1.29272406218394,120.758257536189));
#212866=CARTESIAN_POINT('Ctrl Pts',(6.60816184119489,1.46855650711627,120.766695312289));
#212867=CARTESIAN_POINT('Ctrl Pts',(6.56462423554889,1.64255826260264,120.775133088388));
#212868=CARTESIAN_POINT('Ctrl Pts',(6.52106377586943,1.81665135618357,120.783575293698));
#212869=CARTESIAN_POINT('Ctrl Pts',(6.47059851522227,1.9889115243536,120.792017499008));
#212870=CARTESIAN_POINT('Ctrl Pts',(6.41341966854322,2.15878140513183,120.800459704318));
#212871=CARTESIAN_POINT('Ctrl Pts',(6.35618050132671,2.32883048928864,120.80891081569));
#212872=CARTESIAN_POINT('Ctrl Pts',(6.29221371330304,2.49648393746741,120.817361927062));
#212873=CARTESIAN_POINT('Ctrl Pts',(6.22175892252848,2.66120365810985,120.825813038434));
#212874=CARTESIAN_POINT('Ctrl Pts',(6.20198567636399,2.70743250285698,120.828184855931));
#212875=CARTESIAN_POINT('Ctrl Pts',(6.18170168230166,2.75343041392113,120.830556673428));
#212876=CARTESIAN_POINT('Ctrl Pts',(6.1609128881143,2.79918584325284,120.832928490926));
#212877=CARTESIAN_POINT('Ctrl Pts',(6.08800916389898,2.95964446203028,120.841246160876));
#212878=CARTESIAN_POINT('Ctrl Pts',(6.00876218134742,3.11740875883951,120.849563830826));
#212879=CARTESIAN_POINT('Ctrl Pts',(5.92339548843894,3.27195276364761,120.857881500775));
#212880=CARTESIAN_POINT('Ctrl Pts',(5.83812063497889,3.42633050646668,120.866190222385));
#212881=CARTESIAN_POINT('Ctrl Pts',(5.74673936565344,3.57749456176352,120.874498943995));
#212882=CARTESIAN_POINT('Ctrl Pts',(5.64952227878135,3.72494121048282,120.882807665604));
#212883=CARTESIAN_POINT('Ctrl Pts',(5.55236581984638,3.8722959063733,120.891111205608));
#212884=CARTESIAN_POINT('Ctrl Pts',(5.44938098450012,4.01593752467037,120.899414745611));
#212885=CARTESIAN_POINT('Ctrl Pts',(5.34088336776008,4.15538853201283,120.907718285615));
#212886=CARTESIAN_POINT('Ctrl Pts',(5.23243537626774,4.2947757564724,120.916018027699));
#212887=CARTESIAN_POINT('Ctrl Pts',(5.11847984071684,4.42997591510587,120.924317769783));
#212888=CARTESIAN_POINT('Ctrl Pts',(4.99937469894725,4.56054181205766,120.932617511866));
#212889=CARTESIAN_POINT('Ctrl Pts',(4.88030423815276,4.69106969089743,120.940914837236));
#212890=CARTESIAN_POINT('Ctrl Pts',(4.75608739403087,4.81696574089087,120.949212162605));
#212891=CARTESIAN_POINT('Ctrl Pts',(4.62712140323199,4.93781697916725,120.957509487974));
#212892=CARTESIAN_POINT('Ctrl Pts',(4.49814918357328,5.05867405437335,120.965807214091));
#212893=CARTESIAN_POINT('Ctrl Pts',(4.3644276084,5.17448558849553,120.974104940208));
#212894=CARTESIAN_POINT('Ctrl Pts',(4.22639003624488,5.28487618223265,120.982402666325));
#212895=CARTESIAN_POINT('Ctrl Pts',(4.08835066300326,5.39526821632406,120.99070050071));
#212896=CARTESIAN_POINT('Ctrl Pts',(3.94599545500002,5.50023895518012,120.998998335094));
#212897=CARTESIAN_POINT('Ctrl Pts',(3.79978991268035,5.59945404655602,121.007296169478));
#212898=CARTESIAN_POINT('Ctrl Pts',(3.65351899532164,5.69871350143806,121.015597714196));
#212899=CARTESIAN_POINT('Ctrl Pts',(3.50339459407795,5.79221197473081,121.023899258913));
#212900=CARTESIAN_POINT('Ctrl Pts',(3.34991071589721,5.87965876522754,121.03220080363));
#212901=CARTESIAN_POINT('Ctrl Pts',(3.26725634776005,5.92675074192114,121.036671363935));
#212902=CARTESIAN_POINT('Ctrl Pts',(3.18362816542099,5.97208847191001,121.041141924239));
#212903=CARTESIAN_POINT('Ctrl Pts',(3.09910619832141,6.01563211736936,121.045612484544));
#212904=CARTESIAN_POINT('Ctrl Pts',(3.09910619832142,6.01563211736936,119.045959136766));
#212905=CARTESIAN_POINT('Ctrl Pts',(2.94299959721802,6.0960544114258,119.054185207429));
#212906=CARTESIAN_POINT('Ctrl Pts',(2.78368938707234,6.17043254245761,119.062411278092));
#212907=CARTESIAN_POINT('Ctrl Pts',(2.62169848255776,6.23850832062877,119.070637348755));
#212908=CARTESIAN_POINT('Ctrl Pts',(2.46342911699797,6.30502014271794,119.078674435706));
#212909=CARTESIAN_POINT('Ctrl Pts',(2.30260124994709,6.36551589321831,119.086711522657));
#212910=CARTESIAN_POINT('Ctrl Pts',(2.13972395147972,6.41980298852418,119.094748609608));
#212911=CARTESIAN_POINT('Ctrl Pts',(1.97683143186611,6.47409515704667,119.102786447638));
#212912=CARTESIAN_POINT('Ctrl Pts',(1.8118894539032,6.52217739679846,119.110824285668));
#212913=CARTESIAN_POINT('Ctrl Pts',(1.64542309271336,6.56390675177258,119.118862123698));
#212914=CARTESIAN_POINT('Ctrl Pts',(1.47890819253908,6.60564827437322,119.126902305436));
#212915=CARTESIAN_POINT('Ctrl Pts',(1.31086838661548,6.64103313425422,119.134942487173));
#212916=CARTESIAN_POINT('Ctrl Pts',(1.14183965418601,6.66996935556142,119.142982668911));
#212917=CARTESIAN_POINT('Ctrl Pts',(0.965943438688855,6.70008122912024,
119.151349515892));
#212918=CARTESIAN_POINT('Ctrl Pts',(0.788976697826705,6.7232093964497,119.159716362872));
#212919=CARTESIAN_POINT('Ctrl Pts',(0.611548981277227,6.73930981952149,
119.168083209853));
#212920=CARTESIAN_POINT('Ctrl Pts',(0.440751913338224,6.75480855391721,
119.176137379517));
#212921=CARTESIAN_POINT('Ctrl Pts',(0.269528071443023,6.76379536032711,
119.184191549181));
#212922=CARTESIAN_POINT('Ctrl Pts',(0.0984203184121964,6.76628424180685,
119.192245718845));
#212923=CARTESIAN_POINT('Ctrl Pts',(-0.0728152208507917,6.76877498202636,
119.200305903502));
#212924=CARTESIAN_POINT('Ctrl Pts',(-0.243934127675586,6.76475814353421,
119.208366088159));
#212925=CARTESIAN_POINT('Ctrl Pts',(-0.414398837444021,6.7542995642424,
119.216426272817));
#212926=CARTESIAN_POINT('Ctrl Pts',(-0.585102261964316,6.74382633900326,
119.224497744766));
#212927=CARTESIAN_POINT('Ctrl Pts',(-0.755149293307429,6.72689341119881,
119.232569216715));
#212928=CARTESIAN_POINT('Ctrl Pts',(-0.924012146161016,6.70361772133129,
119.240640688665));
#212929=CARTESIAN_POINT('Ctrl Pts',(-0.943148845126037,6.7009799601975,
119.241555403336));
#212930=CARTESIAN_POINT('Ctrl Pts',(-0.962270351802463,6.69826079176369,
119.242470118007));
#212931=CARTESIAN_POINT('Ctrl Pts',(-0.981375910956522,6.69546042639297,
119.243384832678));
#212932=CARTESIAN_POINT('Ctrl Pts',(-1.15325947486922,6.67026688056177,
119.251614082414));
#212933=CARTESIAN_POINT('Ctrl Pts',(-1.32442484658178,6.63841325853528,
119.25984333215));
#212934=CARTESIAN_POINT('Ctrl Pts',(-1.49431643839945,6.59994752872545,
119.268072581886));
#212935=CARTESIAN_POINT('Ctrl Pts',(-1.66400583158525,6.56152757939162,
119.276292037476));
#212936=CARTESIAN_POINT('Ctrl Pts',(-1.83242411721639,6.51651127046675,
119.284511493066));
#212937=CARTESIAN_POINT('Ctrl Pts',(-1.99902150443574,6.46499822310907,
119.292730948656));
#212938=CARTESIAN_POINT('Ctrl Pts',(-2.16545407051533,6.41353613957094,
119.300942272426));
#212939=CARTESIAN_POINT('Ctrl Pts',(-2.33006898551629,6.35559022295231,
119.309153596195));
#212940=CARTESIAN_POINT('Ctrl Pts',(-2.49232723457679,6.29131098864035,
119.317364919965));
#212941=CARTESIAN_POINT('Ctrl Pts',(-2.65445752904232,6.22708244403717,
119.325569768399));
#212942=CARTESIAN_POINT('Ctrl Pts',(-2.81423452719401,6.15653066082484,
119.333774616833));
#212943=CARTESIAN_POINT('Ctrl Pts',(-2.97113487082171,6.07985580251598,
119.341979465267));
#212944=CARTESIAN_POINT('Ctrl Pts',(-3.12794297496018,6.00322602027009,
119.350179490187));
#212945=CARTESIAN_POINT('Ctrl Pts',(-3.2818774721375,5.9204804908737,119.358379515107));
#212946=CARTESIAN_POINT('Ctrl Pts',(-3.43243539507857,5.8318673046128,119.366579540027));
#212947=CARTESIAN_POINT('Ctrl Pts',(-3.5829497431455,5.74327976501576,119.374777191674));
#212948=CARTESIAN_POINT('Ctrl Pts',(-3.73008915283969,5.64882812949028,
119.382974843321));
#212949=CARTESIAN_POINT('Ctrl Pts',(-3.87337545038235,5.54880632392007,
119.391172494968));
#212950=CARTESIAN_POINT('Ctrl Pts',(-4.01664256101049,5.4487979118834,119.399369048899));
#212951=CARTESIAN_POINT('Ctrl Pts',(-4.15605729252507,5.34322101990534,
119.40756560283));
#212952=CARTESIAN_POINT('Ctrl Pts',(-4.29117064977704,5.23241277562198,
119.415762156761));
#212953=CARTESIAN_POINT('Ctrl Pts',(-4.42629048164051,5.12159922142443,
119.423959103469));
#212954=CARTESIAN_POINT('Ctrl Pts',(-4.55710825114736,5.00555404296093,
119.432156050178));
#212955=CARTESIAN_POINT('Ctrl Pts',(-4.6832082046975,4.88465453348075,119.440352996887));
#212956=CARTESIAN_POINT('Ctrl Pts',(-4.80933712913686,4.76372724788965,
119.448551826807));
#212957=CARTESIAN_POINT('Ctrl Pts',(-4.93074581991987,4.6379436582462,119.456750656726));
#212958=CARTESIAN_POINT('Ctrl Pts',(-5.04705550445287,4.50771779673173,
119.464949486646));
#212959=CARTESIAN_POINT('Ctrl Pts',(-5.16347534912545,4.37736859467913,
119.473156081906));
#212960=CARTESIAN_POINT('Ctrl Pts',(-5.27478629954112,4.24256898267375,
119.481362677166));
#212961=CARTESIAN_POINT('Ctrl Pts',(-5.38064940987826,4.10376667562579,
119.489569272426));
#212962=CARTESIAN_POINT('Ctrl Pts',(-5.48656375856759,3.96489718746562,
119.497779839725));
#212963=CARTESIAN_POINT('Ctrl Pts',(-5.58702480383399,3.82202143498506,
119.505990407024));
#212964=CARTESIAN_POINT('Ctrl Pts',(-5.68173713062174,3.6756158910466,119.514200974323));
#212965=CARTESIAN_POINT('Ctrl Pts',(-5.77658007926708,3.52900843290373,
119.522422865169));
#212966=CARTESIAN_POINT('Ctrl Pts',(-5.86565828156683,3.37886176301135,
119.530644756016));
#212967=CARTESIAN_POINT('Ctrl Pts',(-5.94872186452454,3.22567778591224,
119.538866646863));
#212968=CARTESIAN_POINT('Ctrl Pts',(-6.02424626453097,3.08639739914034,
119.546342286018));
#212969=CARTESIAN_POINT('Ctrl Pts',(-6.0947988183756,2.94460650726778,119.553817925173));
#212970=CARTESIAN_POINT('Ctrl Pts',(-6.16022666132065,2.8006957137744,119.561293564328));
#212971=CARTESIAN_POINT('Ctrl Pts',(-6.24075632375582,2.62356794829797,
119.570494703637));
#212972=CARTESIAN_POINT('Ctrl Pts',(-6.3136817809473,2.44287871718486,119.579695842946));
#212973=CARTESIAN_POINT('Ctrl Pts',(-6.37871688280959,2.25926092538245,
119.588896982256));
#212974=CARTESIAN_POINT('Ctrl Pts',(-6.44355477530049,2.07619992749991,
119.598070220465));
#212975=CARTESIAN_POINT('Ctrl Pts',(-6.50055000002209,1.89022828930608,
119.607243458674));
#212976=CARTESIAN_POINT('Ctrl Pts',(-6.54946562842066,1.70199558816595,
119.616416696883));
#212977=CARTESIAN_POINT('Ctrl Pts',(-6.59827946816817,1.51415458091512,
119.625570846478));
#212978=CARTESIAN_POINT('Ctrl Pts',(-6.63904720679574,1.3240620983253,119.634724996073));
#212979=CARTESIAN_POINT('Ctrl Pts',(-6.67158131231452,1.13238323600081,
119.643879145668));
#212980=CARTESIAN_POINT('Ctrl Pts',(-6.70398688902506,0.941461617662176,
119.652997131));
#212981=CARTESIAN_POINT('Ctrl Pts',(-6.72822368441412,0.748966325945265,
119.662115116333));
#212982=CARTESIAN_POINT('Ctrl Pts',(-6.74415522421459,0.555571158087826,
119.671233101665));
#212983=CARTESIAN_POINT('Ctrl Pts',(-6.75926713705514,0.372125555399899,
119.679881995705));
#212984=CARTESIAN_POINT('Ctrl Pts',(-6.76690666210251,0.187870551008656,
119.688530889745));
#212985=CARTESIAN_POINT('Ctrl Pts',(-6.76699914956147,0.00339261468657305,
119.697179783785));
#212986=CARTESIAN_POINT('',(-6.76699963580264,0.00222014570200688,119.302820216224));
#212987=CARTESIAN_POINT('Ctrl Pts',(3.09910619832126,6.01563211736944,118.651553971577));
#212988=CARTESIAN_POINT('Ctrl Pts',(2.94560425794161,6.09471255407224,118.65968792708));
#212989=CARTESIAN_POINT('Ctrl Pts',(2.78890749860663,6.167999247523,118.667821882584));
#212990=CARTESIAN_POINT('Ctrl Pts',(2.62949778773241,6.23522496661591,118.675955838087));
#212991=CARTESIAN_POINT('Ctrl Pts',(2.47020342135523,6.30240204302128,118.684083908083));
#212992=CARTESIAN_POINT('Ctrl Pts',(2.30820034737353,6.36352673437524,118.69221197808));
#212993=CARTESIAN_POINT('Ctrl Pts',(2.14399417848796,6.41837814113579,118.700340048076));
#212994=CARTESIAN_POINT('Ctrl Pts',(1.97987418690326,6.47320076124225,118.708463852367));
#212995=CARTESIAN_POINT('Ctrl Pts',(1.81355374925965,6.52175653697069,118.716587656658));
#212996=CARTESIAN_POINT('Ctrl Pts',(1.64555753385012,6.56387304895434,118.724711460949));
#212997=CARTESIAN_POINT('Ctrl Pts',(1.47761453133848,6.60597622050859,118.73283269202));
#212998=CARTESIAN_POINT('Ctrl Pts',(1.30799716315632,6.64164410195529,118.740953923091));
#212999=CARTESIAN_POINT('Ctrl Pts',(1.13724428424649,6.67075441295426,118.749075154162));
#213000=CARTESIAN_POINT('Ctrl Pts',(0.966483224829056,6.69986611858342,
118.757196774309));
#213001=CARTESIAN_POINT('Ctrl Pts',(0.79458690590592,6.72241955796674,118.765318394456));
#213002=CARTESIAN_POINT('Ctrl Pts',(0.62210361561856,6.73834372019077,118.773440014603));
#213003=CARTESIAN_POINT('Ctrl Pts',(0.496427137110643,6.74994654054612,
118.779357669688));
#213004=CARTESIAN_POINT('Ctrl Pts',(0.37043925022077,6.75803093605965,118.785275324773));
#213005=CARTESIAN_POINT('Ctrl Pts',(0.244353506160759,6.76258681009175,
118.791192979858));
#213006=CARTESIAN_POINT('Ctrl Pts',(0.0529247053570507,6.76950373403966,
118.800177418384));
#213007=CARTESIAN_POINT('Ctrl Pts',(-0.138634788944055,6.76828229191352,
118.80916185691));
#213008=CARTESIAN_POINT('Ctrl Pts',(-0.329655696648002,6.75896561033325,
118.818146295435));
#213009=CARTESIAN_POINT('Ctrl Pts',(-0.521006295037945,6.74963284871662,
118.827146240566));
#213010=CARTESIAN_POINT('Ctrl Pts',(-0.71181621016391,6.73217693322853,
118.836146185696));
#213011=CARTESIAN_POINT('Ctrl Pts',(-0.901421422903568,6.70669280781001,
118.845146130827));
#213012=CARTESIAN_POINT('Ctrl Pts',(-1.09147344519387,6.68114862839581,
118.854167284559));
#213013=CARTESIAN_POINT('Ctrl Pts',(-1.28031484710437,6.64753841780098,
118.863188438291));
#213014=CARTESIAN_POINT('Ctrl Pts',(-1.46728920163244,6.60600873438515,
118.872209592024));
#213015=CARTESIAN_POINT('Ctrl Pts',(-1.65445380404015,6.56443679418906,
118.881239924851));
#213016=CARTESIAN_POINT('Ctrl Pts',(-1.8397473320953,6.51492934064104,118.890270257678));
#213017=CARTESIAN_POINT('Ctrl Pts',(-2.02252710641955,6.45768326134057,
118.899300590505));
#213018=CARTESIAN_POINT('Ctrl Pts',(-2.20556600484802,6.40035602514473,
118.908343725498));
#213019=CARTESIAN_POINT('Ctrl Pts',(-2.38608379566362,6.33526829801148,
118.91738686049));
#213020=CARTESIAN_POINT('Ctrl Pts',(-2.56345421171337,6.2626664851682,118.926429995483));
#213021=CARTESIAN_POINT('Ctrl Pts',(-2.71851681909309,6.19919577426443,
118.934335778883));
#213022=CARTESIAN_POINT('Ctrl Pts',(-2.87117415656889,6.12998298657736,
118.942241562283));
#213023=CARTESIAN_POINT('Ctrl Pts',(-3.02102171042347,6.05522227710511,
118.950147345683));
#213024=CARTESIAN_POINT('Ctrl Pts',(-3.18503949246517,5.97339187389812,
118.958800733911));
#213025=CARTESIAN_POINT('Ctrl Pts',(-3.34583527378926,5.88484121302058,
118.967454122139));
#213026=CARTESIAN_POINT('Ctrl Pts',(-3.5028576916983,5.78984257054629,118.976107510368));
#213027=CARTESIAN_POINT('Ctrl Pts',(-3.65973508826632,5.69493166605687,
118.984752906578));
#213028=CARTESIAN_POINT('Ctrl Pts',(-3.81284581304721,5.59358481451052,
118.993398302788));
#213029=CARTESIAN_POINT('Ctrl Pts',(-3.96166317892922,5.48612010957803,
119.002043698999));
#213030=CARTESIAN_POINT('Ctrl Pts',(-4.11523327016959,5.37522334397685,
119.010965200041));
#213031=CARTESIAN_POINT('Ctrl Pts',(-4.264230937423,5.25781162698386,119.019886701083));
#213032=CARTESIAN_POINT('Ctrl Pts',(-4.40810784960378,5.1342841941464,119.028808202126));
#213033=CARTESIAN_POINT('Ctrl Pts',(-4.54726647853002,5.01480770602967,
119.037437132468));
#213034=CARTESIAN_POINT('Ctrl Pts',(-4.68163461842893,4.88961046105629,
119.04606606281));
#213035=CARTESIAN_POINT('Ctrl Pts',(-4.81074764583352,4.7590961419273,119.054694993152));
#213036=CARTESIAN_POINT('Ctrl Pts',(-4.94642719203587,4.62194403614605,
119.063762779544));
#213037=CARTESIAN_POINT('Ctrl Pts',(-5.07630288384259,4.47892012229055,
119.072830565937));
#213038=CARTESIAN_POINT('Ctrl Pts',(-5.19987686084161,4.33053918491497,
119.081898352329));
#213039=CARTESIAN_POINT('Ctrl Pts',(-5.32345083784064,4.18215824753938,
119.090966138722));
#213040=CARTESIAN_POINT('Ctrl Pts',(-5.44072282307123,4.02842056419096,
119.100033925115));
#213041=CARTESIAN_POINT('Ctrl Pts',(-5.55124157285252,3.86988449437885,
119.109101711507));
#213042=CARTESIAN_POINT('Ctrl Pts',(-5.6539254670784,3.7225873067452,119.11752666764));
#213043=CARTESIAN_POINT('Ctrl Pts',(-5.75073482331306,3.57121271868087,
119.125951623774));
#213044=CARTESIAN_POINT('Ctrl Pts',(-5.84135670959601,3.41626122994974,
119.134376579907));
#213045=CARTESIAN_POINT('Ctrl Pts',(-5.93199963008893,3.2612737754902,119.142803491553));
#213046=CARTESIAN_POINT('Ctrl Pts',(-6.01645204970856,3.10270805124885,
119.1512304032));
#213047=CARTESIAN_POINT('Ctrl Pts',(-6.09444651794385,2.94109004281102,
119.159657314846));
#213048=CARTESIAN_POINT('Ctrl Pts',(-6.17246966778262,2.77941260113724,
119.168087325396));
#213049=CARTESIAN_POINT('Ctrl Pts',(-6.24402998697614,2.61468093572495,
119.176517335946));
#213050=CARTESIAN_POINT('Ctrl Pts',(-6.30890761372049,2.44744228155429,
119.184947346496));
#213051=CARTESIAN_POINT('Ctrl Pts',(-6.37384500437809,2.28004957063213,
119.193385122596));
#213052=CARTESIAN_POINT('Ctrl Pts',(-6.4320872835115,2.11014556637865,119.201822898695));
#213053=CARTESIAN_POINT('Ctrl Pts',(-6.48346368059371,1.93829505040443,
119.210260674795));
#213054=CARTESIAN_POINT('Ctrl Pts',(-6.5348670464971,1.76635432557756,119.218702880105));
#213055=CARTESIAN_POINT('Ctrl Pts',(-6.57939725504807,1.59246537079121,
119.227145085415));
#213056=CARTESIAN_POINT('Ctrl Pts',(-6.61693424303508,1.41720507455688,
119.235587290724));
#213057=CARTESIAN_POINT('Ctrl Pts',(-6.65451083047907,1.24175988835311,
119.244038402097));
#213058=CARTESIAN_POINT('Ctrl Pts',(-6.68507939849873,1.0649407963259,119.252489513469));
#213059=CARTESIAN_POINT('Ctrl Pts',(-6.70857134288537,0.887332822235909,
119.260940624841));
#213060=CARTESIAN_POINT('Ctrl Pts',(-6.71516439346638,0.837486869193784,
119.263312442338));
#213061=CARTESIAN_POINT('Ctrl Pts',(-6.72120036641145,0.787578801027417,
119.265684259835));
#213062=CARTESIAN_POINT('Ctrl Pts',(-6.72667848189145,0.737621584051423,
119.268056077332));
#213063=CARTESIAN_POINT('Ctrl Pts',(-6.75344304358904,0.493544397129153,
119.279644123618));
#213064=CARTESIAN_POINT('Ctrl Pts',(-6.76691898797299,0.248034488533764,
119.291232169904));
#213065=CARTESIAN_POINT('Ctrl Pts',(-6.7669996358024,0.00222014642263019,
119.30282021619));
#213066=CARTESIAN_POINT('Ctrl Pts',(-6.76699963580264,0.00222014570181755,
119.302820216224));
#213067=CARTESIAN_POINT('Ctrl Pts',(-6.76705696129302,-0.172507833740427,
119.311057147787));
#213068=CARTESIAN_POINT('Ctrl Pts',(-6.76034264214386,-0.347406008666543,
119.31929407935));
#213069=CARTESIAN_POINT('Ctrl Pts',(-6.74684347290728,-0.521912015658256,
119.327531010913));
#213070=CARTESIAN_POINT('Ctrl Pts',(-6.73335440568663,-0.696287432209061,
119.335761778422));
#213071=CARTESIAN_POINT('Ctrl Pts',(-6.71309062957964,-0.870270911770145,
119.34399254593));
#213072=CARTESIAN_POINT('Ctrl Pts',(-6.68609099639552,-1.0433006220255,
119.352223313439));
#213073=CARTESIAN_POINT('Ctrl Pts',(-6.65910624848612,-1.21623493858593,
119.360449543211));
#213074=CARTESIAN_POINT('Ctrl Pts',(-6.62539309662568,-1.38821618236226,
119.368675772982));
#213075=CARTESIAN_POINT('Ctrl Pts',(-6.58504218384844,-1.55868804991138,
119.376902002754));
#213076=CARTESIAN_POINT('Ctrl Pts',(-6.54470556828706,-1.72909951552858,
119.385125317791));
#213077=CARTESIAN_POINT('Ctrl Pts',(-6.497735960321,-1.89800232445434,119.393348632829));
#213078=CARTESIAN_POINT('Ctrl Pts',(-6.44427504019162,-2.06485064989295,
119.401571947866));
#213079=CARTESIAN_POINT('Ctrl Pts',(-6.39081239929268,-2.23170434575012,
119.409795527591));
#213080=CARTESIAN_POINT('Ctrl Pts',(-6.330858129143,-2.39650308418088,119.418019107316));
#213081=CARTESIAN_POINT('Ctrl Pts',(-6.26460382614251,-2.55871606503744,
119.426242687041));
#213082=CARTESIAN_POINT('Ctrl Pts',(-6.19834462893252,-2.72094102857702,
119.434466874242));
#213083=CARTESIAN_POINT('Ctrl Pts',(-6.12578460586727,-2.8805795238249,
119.442691061443));
#213084=CARTESIAN_POINT('Ctrl Pts',(-6.0471635143063,-3.03712074689873,
119.450915248645));
#213085=CARTESIAN_POINT('Ctrl Pts',(-5.96852257831873,-3.19370148189932,
119.459141511679));
#213086=CARTESIAN_POINT('Ctrl Pts',(-5.88381768582728,-3.34718306880869,
119.467367774714));
#213087=CARTESIAN_POINT('Ctrl Pts',(-5.79333459240561,-3.49707925281034,
119.475594037748));
#213088=CARTESIAN_POINT('Ctrl Pts',(-5.70281250573809,-3.64704003383819,
119.48382384585));
#213089=CARTESIAN_POINT('Ctrl Pts',(-5.60650744128516,-3.79341202898163,
119.492053653953));
#213090=CARTESIAN_POINT('Ctrl Pts',(-5.50474854942942,-3.93573784792061,
119.500283462055));
#213091=CARTESIAN_POINT('Ctrl Pts',(-5.40287236336662,-4.07822772126085,
119.508522756393));
#213092=CARTESIAN_POINT('Ctrl Pts',(-5.29553000096965,-4.21666181303084,
119.516762050731));
#213093=CARTESIAN_POINT('Ctrl Pts',(-5.18309160179715,-4.35061495048457,
119.525001345068));
#213094=CARTESIAN_POINT('Ctrl Pts',(-5.07057965381129,-4.48465571008855,
119.533246028938));
#213095=CARTESIAN_POINT('Ctrl Pts',(-4.95296526303893,-4.61420940946759,
119.541490712807));
#213096=CARTESIAN_POINT('Ctrl Pts',(-4.83065545569473,-4.73888772481125,
119.549735396677));
#213097=CARTESIAN_POINT('Ctrl Pts',(-4.7081736682752,-4.86374135059429,
119.557991673414));
#213098=CARTESIAN_POINT('Ctrl Pts',(-4.58098353516427,-4.98370565562182,
119.56624795015));
#213099=CARTESIAN_POINT('Ctrl Pts',(-4.44952594158702,-5.09843190551214,
119.574504226887));
#213100=CARTESIAN_POINT('Ctrl Pts',(-4.3887002776264,-5.15151594678656,
119.578324420919));
#213101=CARTESIAN_POINT('Ctrl Pts',(-4.32696140432062,-5.20347915514866,
119.58214461495));
#213102=CARTESIAN_POINT('Ctrl Pts',(-4.2643550524789,-5.25429015057198,
119.585964808981));
#213103=CARTESIAN_POINT('Ctrl Pts',(-4.13210427829957,-5.36162420348957,
119.594034654984));
#213104=CARTESIAN_POINT('Ctrl Pts',(-3.99555418278254,-5.46416000462343,
119.602104500987));
#213105=CARTESIAN_POINT('Ctrl Pts',(-3.85509364570755,-5.56152335091972,
119.610174346989));
#213106=CARTESIAN_POINT('Ctrl Pts',(-3.71480982585413,-5.6587642017422,
119.618234040099));
#213107=CARTESIAN_POINT('Ctrl Pts',(-3.57062565627738,-5.75084533623054,
119.62629373321));
#213108=CARTESIAN_POINT('Ctrl Pts',(-3.42296518189044,-5.83743080160834,
119.63435342632));
#213109=CARTESIAN_POINT('Ctrl Pts',(-3.27545807635908,-5.92392633422796,
119.642404748158));
#213110=CARTESIAN_POINT('Ctrl Pts',(-3.12448217044023,-6.00493736984605,
119.650456069997));
#213111=CARTESIAN_POINT('Ctrl Pts',(-2.97049268230625,-6.08016958845434,
119.658507391835));
#213112=CARTESIAN_POINT('Ctrl Pts',(-2.81662939237062,-6.15534015239671,
119.666552115416));
#213113=CARTESIAN_POINT('Ctrl Pts',(-2.65975776924429,-6.22474116231977,
119.674596838998));
#213114=CARTESIAN_POINT('Ctrl Pts',(-2.50035988398835,-6.28812288767815,
119.682641562579));
#213115=CARTESIAN_POINT('Ctrl Pts',(-2.34105773697832,-6.35146654443104,
119.690681454303));
#213116=CARTESIAN_POINT('Ctrl Pts',(-2.17923269420338,-6.4087979761119,
119.698721346027));
#213117=CARTESIAN_POINT('Ctrl Pts',(-2.01538907681763,-6.45991454038242,
119.706761237752));
#213118=CARTESIAN_POINT('Ctrl Pts',(-1.84801745747078,-6.51213178432462,
119.714974250372));
#213119=CARTESIAN_POINT('Ctrl Pts',(-1.67853970456727,-6.5578633034028,
119.723187262992));
#213120=CARTESIAN_POINT('Ctrl Pts',(-1.50751279804986,-6.59694582088681,
119.731400275612));
#213121=CARTESIAN_POINT('Ctrl Pts',(-1.34014935756891,-6.63519117491895,
119.739437362154));
#213122=CARTESIAN_POINT('Ctrl Pts',(-1.1713028400355,-6.6670694166407,119.747474448697));
#213123=CARTESIAN_POINT('Ctrl Pts',(-1.0015079089637,-6.69247868194462,
119.755511535239));
#213124=CARTESIAN_POINT('Ctrl Pts',(-0.831696727726329,-6.71789037903355,
119.763549390969));
#213125=CARTESIAN_POINT('Ctrl Pts',(-0.660937321720731,-6.73683181152722,
119.771587246698));
#213126=CARTESIAN_POINT('Ctrl Pts',(-0.48977155389521,-6.74925276049098,
119.779625102427));
#213127=CARTESIAN_POINT('Ctrl Pts',(-0.318555491056461,-6.761677359202,
119.787665319984));
#213128=CARTESIAN_POINT('Ctrl Pts',(-0.146933201163257,-6.76757763369418,
119.795705537541));
#213129=CARTESIAN_POINT('Ctrl Pts',(0.0245515112282709,-6.76695546189691,
119.803745755098));
#213130=CARTESIAN_POINT('Ctrl Pts',(0.202515025927437,-6.76630978405051,
119.812089737226));
#213131=CARTESIAN_POINT('Ctrl Pts',(0.380329919503763,-6.75863919060469,
119.820433719353));
#213132=CARTESIAN_POINT('Ctrl Pts',(0.557393166619768,-6.74400488269438,
119.828777701481));
#213133=CARTESIAN_POINT('Ctrl Pts',(0.728307414736377,-6.72987879061182,
119.836831916316));
#213134=CARTESIAN_POINT('Ctrl Pts',(0.898520989872278,-6.70926465342827,
119.844886131151));
#213135=CARTESIAN_POINT('Ctrl Pts',(1.0675015678996,-6.68226977923908,119.852940345986));
#213136=CARTESIAN_POINT('Ctrl Pts',(1.2366085999468,-6.65525470385046,119.861000588069));
#213137=CARTESIAN_POINT('Ctrl Pts',(1.40448043378287,-6.62184945637709,
119.869060830152));
#213138=CARTESIAN_POINT('Ctrl Pts',(1.57059889595873,-6.58221149067798,
119.877121072235));
#213139=CARTESIAN_POINT('Ctrl Pts',(1.73694960313938,-6.54251810838391,
119.88519258309));
#213140=CARTESIAN_POINT('Ctrl Pts',(1.90154169138591,-6.49657472188905,
119.893264093944));
#213141=CARTESIAN_POINT('Ctrl Pts',(2.06387543137661,-6.44458743472071,
119.901335604798));
#213142=CARTESIAN_POINT('Ctrl Pts',(2.08088970222854,-6.43913862423442,
119.902181583409));
#213143=CARTESIAN_POINT('Ctrl Pts',(2.09787918597496,-6.43362346219491,
119.90302756202));
#213144=CARTESIAN_POINT('Ctrl Pts',(2.11484332267144,-6.42804221521234,
119.903873540631));
#213145=CARTESIAN_POINT('Ctrl Pts',(2.27986181797582,-6.37375068270096,
119.912102790367));
#213146=CARTESIAN_POINT('Ctrl Pts',(2.44303082318764,-6.31302084285292,
119.920332040103));
#213147=CARTESIAN_POINT('Ctrl Pts',(2.60381120285945,-6.24599521452455,
119.928561289839));
#213148=CARTESIAN_POINT('Ctrl Pts',(2.76440022772322,-6.17904935759783,
119.936780745429));
#213149=CARTESIAN_POINT('Ctrl Pts',(2.92260595999053,-6.10582276897258,
119.945000201019));
#213150=CARTESIAN_POINT('Ctrl Pts',(3.07790383156231,-6.02650786141145,
119.953219656609));
#213151=CARTESIAN_POINT('Ctrl Pts',(3.23304806103674,-5.94727142310831,
119.961430980379));
#213152=CARTESIAN_POINT('Ctrl Pts',(3.38528984180507,-5.86195882332208,
119.969642304148));
#213153=CARTESIAN_POINT('Ctrl Pts',(3.53412394848384,-5.77081076771306,
119.977853627918));
#213154=CARTESIAN_POINT('Ctrl Pts',(3.68284068665845,-5.67973459019155,
119.986058476352));
#213155=CARTESIAN_POINT('Ctrl Pts',(3.82815479862485,-5.58283230891746,
119.994263324786));
#213156=CARTESIAN_POINT('Ctrl Pts',(3.96958499643833,-5.48039085796367,
120.00246817322));
#213157=CARTESIAN_POINT('Ctrl Pts',(4.11093204944244,-5.3780096308874,120.01066819814));
#213158=CARTESIAN_POINT('Ctrl Pts',(4.24839944717174,-5.27009593102541,
120.01886822306));
#213159=CARTESIAN_POINT('Ctrl Pts',(4.38153420815219,-5.15698041326435,
120.02706824798));
#213160=CARTESIAN_POINT('Ctrl Pts',(4.51463043691663,-5.04389763369678,
120.035265899627));
#213161=CARTESIAN_POINT('Ctrl Pts',(4.6433962511269,-4.92561626394849,120.043463551274));
#213162=CARTESIAN_POINT('Ctrl Pts',(4.76741095459218,-4.80250786465097,
120.051661202921));
#213163=CARTESIAN_POINT('Ctrl Pts',(4.89140905172758,-4.67941595032366,
120.059857756852));
#213164=CARTESIAN_POINT('Ctrl Pts',(5.01065705008485,-4.55149854583567,
120.068054310783));
#213165=CARTESIAN_POINT('Ctrl Pts',(5.12477040735327,-4.41916477084938,
120.076250864714));
#213166=CARTESIAN_POINT('Ctrl Pts',(5.23888923291697,-4.28682465444807,
120.084447811423));
#213167=CARTESIAN_POINT('Ctrl Pts',(5.34787269285735,-4.15006801759549,
120.092644758131));
#213168=CARTESIAN_POINT('Ctrl Pts',(5.45137588092092,-4.00933785118112,
120.10084170484));
#213169=CARTESIAN_POINT('Ctrl Pts',(5.55490284836831,-3.86857535265501,
120.10904053476));
#213170=CARTESIAN_POINT('Ctrl Pts',(5.65294682374694,-3.72383779528758,
120.11723936468));
#213171=CARTESIAN_POINT('Ctrl Pts',(5.74520563340386,-3.57559802409394,
120.125438194599));
#213172=CARTESIAN_POINT('Ctrl Pts',(5.83755182394802,-3.42721785088582,
120.133644789859));
#213173=CARTESIAN_POINT('Ctrl Pts',(5.92410171184173,-3.27532914167813,
120.141851385119));
#213174=CARTESIAN_POINT('Ctrl Pts',(6.00459813564056,-3.12043109673358,
120.150057980379));
#213175=CARTESIAN_POINT('Ctrl Pts',(6.0851335201702,-2.96545808024686,120.158268547678));
#213176=CARTESIAN_POINT('Ctrl Pts',(6.1596094461796,-2.80747314834473,120.166479114977));
#213177=CARTESIAN_POINT('Ctrl Pts',(6.22781656917511,-2.64699636960612,
120.174689682276));
#213178=CARTESIAN_POINT('Ctrl Pts',(6.29611775955756,-2.48629827041624,
120.182911573123));
#213179=CARTESIAN_POINT('Ctrl Pts',(6.35813274121453,-2.32310179173224,
120.191133463969));
#213180=CARTESIAN_POINT('Ctrl Pts',(6.41370139779053,-2.15794424858009,
120.199355354816));
#213181=CARTESIAN_POINT('Ctrl Pts',(6.46422642088154,-2.00777706449482,
120.206830993971));
#213182=CARTESIAN_POINT('Ctrl Pts',(6.50942277505385,-1.85598902333105,
120.214306633126));
#213183=CARTESIAN_POINT('Ctrl Pts',(6.54920683200432,-1.70299115430115,
120.221782272281));
#213184=CARTESIAN_POINT('Ctrl Pts',(6.59676237552186,-1.52010641663347,
120.230718215731));
#213185=CARTESIAN_POINT('Ctrl Pts',(6.6366835183352,-1.33511213433792,120.239654159182));
#213186=CARTESIAN_POINT('Ctrl Pts',(6.66880167438889,-1.14863972927456,
120.248590102633));
#213187=CARTESIAN_POINT('Ctrl Pts',(6.70087154833531,-0.962447641694246,
120.25751261299));
#213188=CARTESIAN_POINT('Ctrl Pts',(6.72516179708992,-0.774782118893723,
120.266435123348));
#213189=CARTESIAN_POINT('Ctrl Pts',(6.74155455269187,-0.586285948219416,
120.275357633706));
#213190=CARTESIAN_POINT('Ctrl Pts',(6.7579071409554,-0.398251651659642,
120.284258281144));
#213191=CARTESIAN_POINT('Ctrl Pts',(6.76640083551289,-0.209391026181027,
120.293158928582));
#213192=CARTESIAN_POINT('Ctrl Pts',(6.76696939358396,-0.0203525501598814,
120.302059576021));
#213193=CARTESIAN_POINT('Ctrl Pts',(6.76753707301869,0.168393790227225,
120.310946468607));
#213194=CARTESIAN_POINT('Ctrl Pts',(6.76020404538767,0.357317175996606,
120.319833361193));
#213195=CARTESIAN_POINT('Ctrl Pts',(6.74495581604873,0.545765553649547,
120.328720253779));
#213196=CARTESIAN_POINT('Ctrl Pts',(6.72974678035114,0.733729548626838,
120.337584303734));
#213197=CARTESIAN_POINT('Ctrl Pts',(6.70666316079215,0.921220715213209,
120.346448353689));
#213198=CARTESIAN_POINT('Ctrl Pts',(6.67574227306163,1.10758932084862,120.355312403644));
#213199=CARTESIAN_POINT('Ctrl Pts',(6.64617941697724,1.28577270015728,120.363787148465));
#213200=CARTESIAN_POINT('Ctrl Pts',(6.60945291378741,1.46292974106706,120.372261893285));
#213201=CARTESIAN_POINT('Ctrl Pts',(6.56563993181082,1.63849360261527,120.380736638106));
#213202=CARTESIAN_POINT('Ctrl Pts',(6.52320124751472,1.80855048890599,120.388945552535));
#213203=CARTESIAN_POINT('Ctrl Pts',(6.47415364599792,1.97694841464193,120.397154466964));
#213204=CARTESIAN_POINT('Ctrl Pts',(6.41866100673713,2.14314719060364,120.405363381393));
#213205=CARTESIAN_POINT('Ctrl Pts',(6.36315517438321,2.30938547948022,120.41357424745));
#213206=CARTESIAN_POINT('Ctrl Pts',(6.30120136433841,2.47342323918611,120.421785113507));
#213207=CARTESIAN_POINT('Ctrl Pts',(6.23301251086401,2.63473794511195,120.429995979563));
#213208=CARTESIAN_POINT('Ctrl Pts',(6.16479529088696,2.79611975781258,120.438210261333));
#213209=CARTESIAN_POINT('Ctrl Pts',(6.09033799866573,2.95477593226773,120.446424543103));
#213210=CARTESIAN_POINT('Ctrl Pts',(6.00990067075137,3.11020625163384,120.454638824873));
#213211=CARTESIAN_POINT('Ctrl Pts',(5.92937280427444,3.26581152009463,120.462862352465));
#213212=CARTESIAN_POINT('Ctrl Pts',(5.84285162179691,3.41818336488845,120.471085880058));
#213213=CARTESIAN_POINT('Ctrl Pts',(5.75064235647865,3.5668475560183,120.47930940765));
#213214=CARTESIAN_POINT('Ctrl Pts',(5.65837398860826,3.71560703511164,120.487538206204));
#213215=CARTESIAN_POINT('Ctrl Pts',(5.56041046892615,3.86065382889616,120.495767004757));
#213216=CARTESIAN_POINT('Ctrl Pts',(5.45709884885961,4.00154484590329,120.503995803311));
#213217=CARTESIAN_POINT('Ctrl Pts',(5.35364502861537,4.14262978812077,120.512235928147));
#213218=CARTESIAN_POINT('Ctrl Pts',(5.24482862550006,4.27954725025028,120.520476052984));
#213219=CARTESIAN_POINT('Ctrl Pts',(5.13103589340455,4.41188844607319,120.52871617782));
#213220=CARTESIAN_POINT('Ctrl Pts',(5.08051661640693,4.47064247549893,120.53237445319));
#213221=CARTESIAN_POINT('Ctrl Pts',(5.02901698301694,4.52849502504167,120.53603272856));
#213222=CARTESIAN_POINT('Ctrl Pts',(4.97657296742637,4.58541279492709,120.53969100393));
#213223=CARTESIAN_POINT('Ctrl Pts',(4.85544412036637,4.71687457880862,120.548140446117));
#213224=CARTESIAN_POINT('Ctrl Pts',(4.72899783207813,4.84364795984233,120.556589888304));
#213225=CARTESIAN_POINT('Ctrl Pts',(4.59762346793425,4.96529429612186,120.565039330491));
#213226=CARTESIAN_POINT('Ctrl Pts',(4.46639956677605,5.08680131092057,120.573479095537));
#213227=CARTESIAN_POINT('Ctrl Pts',(4.33025909046391,5.20319276688578,120.581918860583));
#213228=CARTESIAN_POINT('Ctrl Pts',(4.18962887805883,5.31406613283421,120.590358625629));
#213229=CARTESIAN_POINT('Ctrl Pts',(4.04909396097928,5.42486436760478,120.598792671632));
#213230=CARTESIAN_POINT('Ctrl Pts',(3.90407563137865,5.53015175787443,120.607226717635));
#213231=CARTESIAN_POINT('Ctrl Pts',(3.75503519795098,5.62956478443487,120.615660763638));
#213232=CARTESIAN_POINT('Ctrl Pts',(3.60609226047604,5.72891277919478,120.624089292445));
#213233=CARTESIAN_POINT('Ctrl Pts',(3.45313274279014,5.82239388875738,120.632517821252));
#213234=CARTESIAN_POINT('Ctrl Pts',(3.29664857169228,5.90968672560223,120.640946350059));
#213235=CARTESIAN_POINT('Ctrl Pts',(3.23140116635628,5.94608421595916,120.644460696791));
#213236=CARTESIAN_POINT('Ctrl Pts',(3.16554133918318,5.98140636140324,120.647975043524));
#213237=CARTESIAN_POINT('Ctrl Pts',(3.09910619832143,6.01563211736935,120.651489390257));
#213238=CARTESIAN_POINT('Origin',(0.,0.,4.30282021618968));
#213239=CARTESIAN_POINT('',(3.09910619832136,6.01563211736939,123.045720569644));
#213240=CARTESIAN_POINT('',(3.09910619832147,6.01563211736933,122.651395695404));
#213241=CARTESIAN_POINT('',(3.09910619832133,6.0156321173694,4.30282021618968));
#213242=CARTESIAN_POINT('',(-6.76699803762956,-0.00515351508554775,121.69717978385));
#213243=CARTESIAN_POINT('Ctrl Pts',(-6.76699803762956,-0.0051535150855464,
121.69717978385));
#213244=CARTESIAN_POINT('Ctrl Pts',(-6.76684306719459,-0.208642708749951,
121.706729803712));
#213245=CARTESIAN_POINT('Ctrl Pts',(-6.75750558641317,-0.411774755921207,
121.716279823574));
#213246=CARTESIAN_POINT('Ctrl Pts',(-6.73910552699447,-0.613796135563451,
121.725829843436));
#213247=CARTESIAN_POINT('Ctrl Pts',(-6.72060756771969,-0.816892395647138,
121.735430675392));
#213248=CARTESIAN_POINT('Ctrl Pts',(-6.69295042803033,-1.01886605019071,
121.745031507349));
#213249=CARTESIAN_POINT('Ctrl Pts',(-6.65630536300722,-1.21897002194531,
121.754632339306));
#213250=CARTESIAN_POINT('Ctrl Pts',(-6.61944545005337,-1.42024719189828,
121.764289460394));
#213251=CARTESIAN_POINT('Ctrl Pts',(-6.57349197828484,-1.61963260654731,
121.773946581483));
#213252=CARTESIAN_POINT('Ctrl Pts',(-6.51866788492275,-1.81638597387141,
121.783603702571));
#213253=CARTESIAN_POINT('Ctrl Pts',(-6.51289434254675,-1.83710613236748,
121.784620697005));
#213254=CARTESIAN_POINT('Ctrl Pts',(-6.50702246635849,-1.85779711962993,
121.78563769144));
#213255=CARTESIAN_POINT('Ctrl Pts',(-6.50105254746679,-1.87845808446065,
121.786654685875));
#213256=CARTESIAN_POINT('Ctrl Pts',(-6.44859713984116,-2.05999812743206,
121.795590629325));
#213257=CARTESIAN_POINT('Ctrl Pts',(-6.38849998283156,-2.23945540325317,
121.804526572776));
#213258=CARTESIAN_POINT('Ctrl Pts',(-6.32093840089574,-2.41620088818825,
121.813462516227));
#213259=CARTESIAN_POINT('Ctrl Pts',(-6.25347838193716,-2.59268067778064,
121.822385026584));
#213260=CARTESIAN_POINT('Ctrl Pts',(-6.17857641980313,-2.76645656995512,
121.831307536942));
#213261=CARTESIAN_POINT('Ctrl Pts',(-6.09645925375148,-2.93691565547054,
121.8402300473));
#213262=CARTESIAN_POINT('Ctrl Pts',(-6.01454330024006,-3.10695706332791,
121.849130694738));
#213263=CARTESIAN_POINT('Ctrl Pts',(-5.92544753979026,-3.27369765278781,
121.858031342176));
#213264=CARTESIAN_POINT('Ctrl Pts',(-5.82944601008305,-3.43654597168827,
121.866931989614));
#213265=CARTESIAN_POINT('Ctrl Pts',(-5.73359283889089,-3.59914262861163,
121.875818882201));
#213266=CARTESIAN_POINT('Ctrl Pts',(-5.63085531678332,-3.75785879205058,
121.884705774787));
#213267=CARTESIAN_POINT('Ctrl Pts',(-5.52155380558094,-3.91212634919614,
121.893592667373));
#213268=CARTESIAN_POINT('Ctrl Pts',(-5.412533240064,-4.0659973811326,121.902456717328));
#213269=CARTESIAN_POINT('Ctrl Pts',(-5.29698250099016,-4.21544241363451,
121.911320767283));
#213270=CARTESIAN_POINT('Ctrl Pts',(-5.1752653182894,-4.35992177513667,
121.920184817238));
#213271=CARTESIAN_POINT('Ctrl Pts',(-5.05889390015725,-4.49805566729363,
121.928659562058));
#213272=CARTESIAN_POINT('Ctrl Pts',(-4.93688618450119,-4.63165046696655,
121.937134306879));
#213273=CARTESIAN_POINT('Ctrl Pts',(-4.80959786120011,-4.76025812467552,
121.945609051699));
#213274=CARTESIAN_POINT('Ctrl Pts',(-4.6863022368542,-4.88483169938894,
121.953817966128));
#213275=CARTESIAN_POINT('Ctrl Pts',(-4.55817024650373,-5.0046053261003,
121.962026880557));
#213276=CARTESIAN_POINT('Ctrl Pts',(-4.42561854096926,-5.11919813348039,
121.970235794986));
#213277=CARTESIAN_POINT('Ctrl Pts',(-4.29303532194022,-5.23381818471826,
121.978446661043));
#213278=CARTESIAN_POINT('Ctrl Pts',(-4.15603056368776,-5.34325472982332,
121.9866575271));
#213279=CARTESIAN_POINT('Ctrl Pts',(-4.01505408375687,-5.44716712654452,
121.994868393157));
#213280=CARTESIAN_POINT('Ctrl Pts',(-3.87401895773528,-5.55112275073066,
122.003082674927));
#213281=CARTESIAN_POINT('Ctrl Pts',(-3.72900910483554,-5.64954943725195,
122.011296956696));
#213282=CARTESIAN_POINT('Ctrl Pts',(-3.58050346034168,-5.74214976907441,
122.019511238466));
#213283=CARTESIAN_POINT('Ctrl Pts',(-3.43183066102137,-5.83485432988054,
122.027734766059));
#213284=CARTESIAN_POINT('Ctrl Pts',(-3.27965451330539,-5.92171924897578,
122.035958293651));
#213285=CARTESIAN_POINT('Ctrl Pts',(-3.12447955357813,-6.00249252554905,
122.044181821243));
#213286=CARTESIAN_POINT('Ctrl Pts',(-2.96920513273786,-6.08331757465059,
122.052410619797));
#213287=CARTESIAN_POINT('Ctrl Pts',(-2.81092838942147,-6.15804304621675,
122.060639418351));
#213288=CARTESIAN_POINT('Ctrl Pts',(-2.65017392644733,-6.22646506129913,
122.068868216904));
#213289=CARTESIAN_POINT('Ctrl Pts',(-2.48919819781889,-6.29498125380996,
122.077108341741));
#213290=CARTESIAN_POINT('Ctrl Pts',(-2.32573826943377,-6.35717653365713,
122.085348466577));
#213291=CARTESIAN_POINT('Ctrl Pts',(-2.1603349447785,-6.41289653170616,
122.093588591414));
#213292=CARTESIAN_POINT('Ctrl Pts',(-2.08690269457443,-6.43763391136062,
122.097246866784));
#213293=CARTESIAN_POINT('Ctrl Pts',(-2.01308755571051,-6.46109568883975,
122.100905142154));
#213294=CARTESIAN_POINT('Ctrl Pts',(-1.93893746026329,-6.48327159119435,
122.104563417524));
#213295=CARTESIAN_POINT('Ctrl Pts',(-1.76770330459528,-6.53448220519242,
122.113011440286));
#213296=CARTESIAN_POINT('Ctrl Pts',(-1.59429039342887,-6.57894926341465,
122.121459463049));
#213297=CARTESIAN_POINT('Ctrl Pts',(-1.41925716203101,-6.61649439718826,
122.129907485811));
#213298=CARTESIAN_POINT('Ctrl Pts',(-1.24438421379054,-6.6540051497616,
122.138347772467));
#213299=CARTESIAN_POINT('Ctrl Pts',(-1.067894227451,-6.68460654300549,122.146788059123));
#213300=CARTESIAN_POINT('Ctrl Pts',(-0.890359818097933,-6.70817027171468,
122.155228345779));
#213301=CARTESIAN_POINT('Ctrl Pts',(-0.712960651881478,-6.7317160499173,
122.163662202747));
#213302=CARTESIAN_POINT('Ctrl Pts',(-0.534518978186544,-6.74823480740924,
122.172096059714));
#213303=CARTESIAN_POINT('Ctrl Pts',(-0.355616996016955,-6.75764941027158,
122.180529916682));
#213304=CARTESIAN_POINT('Ctrl Pts',(-0.176823795539978,-6.76705828856664,
122.188958645427));
#213305=CARTESIAN_POINT('Ctrl Pts',(0.00242882315528636,-6.76937160706409,
122.197387374172));
#213306=CARTESIAN_POINT('Ctrl Pts',(0.181553755591427,-6.76456408306039,
122.205816102917));
#213307=CARTESIAN_POINT('Ctrl Pts',(0.360597277710887,-6.75975874402361,
122.214241000898));
#213308=CARTESIAN_POINT('Ctrl Pts',(0.539512896455443,-6.74783902471258,
122.222665898878));
#213309=CARTESIAN_POINT('Ctrl Pts',(0.717713322958444,-6.72883174006067,
122.231090796858));
#213310=CARTESIAN_POINT('Ctrl Pts',(0.895874295597169,-6.70982866365251,
122.239513829552));
#213311=CARTESIAN_POINT('Ctrl Pts',(1.07332006010618,-6.68374118329547,
122.247936862247));
#213312=CARTESIAN_POINT('Ctrl Pts',(1.24946772770158,-6.65064804341895,
122.256359894941));
#213313=CARTESIAN_POINT('Ctrl Pts',(1.42559546438857,-6.6175586479936,122.264781974578));
#213314=CARTESIAN_POINT('Ctrl Pts',(1.60042506929696,-6.57746523485965,
122.273204054216));
#213315=CARTESIAN_POINT('Ctrl Pts',(1.77338282249357,-6.53049786500882,
122.281626133854));
#213316=CARTESIAN_POINT('Ctrl Pts',(1.94634514932715,-6.48352925316857,
122.290048436202));
#213317=CARTESIAN_POINT('Ctrl Pts',(2.11743520404457,-6.42968640996452,
122.29847073855));
#213318=CARTESIAN_POINT('Ctrl Pts',(2.28609307199985,-6.36914966586234,
122.306893040898));
#213319=CARTESIAN_POINT('Ctrl Pts',(2.45477894463458,-6.3086028699782,122.315316741722));
#213320=CARTESIAN_POINT('Ctrl Pts',(2.62103151172699,-6.2413600704372,122.323740442546));
#213321=CARTESIAN_POINT('Ctrl Pts',(2.7843091826631,-6.1676503934106,122.332164143369));
#213322=CARTESIAN_POINT('Ctrl Pts',(2.94769734509162,-6.0938908363718,122.340593544588));
#213323=CARTESIAN_POINT('Ctrl Pts',(3.1081062843796,-6.01365579450131,122.349022945807));
#213324=CARTESIAN_POINT('Ctrl Pts',(3.26501652257053,-5.92722161786966,
122.357452347026));
#213325=CARTESIAN_POINT('Ctrl Pts',(3.42198274611659,-5.8407566016438,122.365884755844));
#213326=CARTESIAN_POINT('Ctrl Pts',(3.57544749035845,-5.74808820662621,
122.374317164661));
#213327=CARTESIAN_POINT('Ctrl Pts',(3.72491829995301,-5.64953738448337,
122.382749573479));
#213328=CARTESIAN_POINT('Ctrl Pts',(3.87452740428954,-5.55089538025249,
122.391189784207));
#213329=CARTESIAN_POINT('Ctrl Pts',(4.02013491565663,-5.44636026341438,
122.399629994934));
#213330=CARTESIAN_POINT('Ctrl Pts',(4.16127873668112,-5.33629536997771,
122.408070205662));
#213331=CARTESIAN_POINT('Ctrl Pts',(4.24155893358552,-5.27369233675089,
122.412870853499));
#213332=CARTESIAN_POINT('Ctrl Pts',(4.32039566512156,-5.20930108386711,
122.417671501336));
#213333=CARTESIAN_POINT('Ctrl Pts',(4.39770895395286,-5.14319404225845,
122.422472149173));
#213334=CARTESIAN_POINT('Ctrl Pts',(4.52879712386033,-5.03110657018901,
122.430611864206));
#213335=CARTESIAN_POINT('Ctrl Pts',(4.6557648994597,-4.91386073521467,122.438751579239));
#213336=CARTESIAN_POINT('Ctrl Pts',(4.77817847597647,-4.79179501353253,
122.446891294272));
#213337=CARTESIAN_POINT('Ctrl Pts',(4.90048499031364,-4.66983604979823,
122.455023890359));
#213338=CARTESIAN_POINT('Ctrl Pts',(5.01824497631346,-4.54306584698048,
122.463156486446));
#213339=CARTESIAN_POINT('Ctrl Pts',(5.13105780714589,-4.41186296021616,
122.471289082533));
#213340=CARTESIAN_POINT('Ctrl Pts',(5.24379351307515,-4.28074977078379,
122.479416118741));
#213341=CARTESIAN_POINT('Ctrl Pts',(5.35158855972921,-4.14521020735507,
122.487543154949));
#213342=CARTESIAN_POINT('Ctrl Pts',(5.45407933864111,-4.0056594423151,122.495670191157));
#213343=CARTESIAN_POINT('Ctrl Pts',(5.55652112510568,-3.8661753850666,122.503793342494));
#213344=CARTESIAN_POINT('Ctrl Pts',(5.65366347659911,-3.72268423896338,
122.511916493832));
#213345=CARTESIAN_POINT('Ctrl Pts',(5.7451832572382,-3.57563397745768,122.520039645169));
#213346=CARTESIAN_POINT('Ctrl Pts',(5.8366773201387,-3.42862503816844,122.528160513841));
#213347=CARTESIAN_POINT('Ctrl Pts',(5.92255176653967,-3.27805928661287,
122.536281382513));
#213348=CARTESIAN_POINT('Ctrl Pts',(6.00252699181003,-3.12441333894733,
122.544402251184));
#213349=CARTESIAN_POINT('Ctrl Pts',(6.08250653924776,-2.97075908766654,
122.552523558739));
#213350=CARTESIAN_POINT('Ctrl Pts',(6.15658605600262,-2.81402463072592,
122.560644866293));
#213351=CARTESIAN_POINT('Ctrl Pts',(6.22453199581333,-2.65471098861932,
122.568766173848));
#213352=CARTESIAN_POINT('Ctrl Pts',(6.25983906806303,-2.57192608214969,
122.572986287565));
#213353=CARTESIAN_POINT('Ctrl Pts',(6.29349072389814,-2.48844511329279,
122.577206401281));
#213354=CARTESIAN_POINT('Ctrl Pts',(6.32545932362092,-2.40434052189309,
122.581426514998));
#213355=CARTESIAN_POINT('Ctrl Pts',(6.39351908178095,-2.22528550539411,
122.590410953524));
#213356=CARTESIAN_POINT('Ctrl Pts',(6.45391403626528,-2.04349171768177,
122.59939539205));
#213357=CARTESIAN_POINT('Ctrl Pts',(6.50646997460851,-1.85960680508486,
122.608379830575));
#213358=CARTESIAN_POINT('Ctrl Pts',(6.5591166213646,-1.67540451810375,122.617379775706));
#213359=CARTESIAN_POINT('Ctrl Pts',(6.60389714413356,-1.4891041223001,122.626379720836));
#213360=CARTESIAN_POINT('Ctrl Pts',(6.6406880904066,-1.30136493188191,122.635379665967));
#213361=CARTESIAN_POINT('Ctrl Pts',(6.67756573548888,-1.11318332924256,
122.644400819699));
#213362=CARTESIAN_POINT('Ctrl Pts',(6.70641608688096,-0.923556383487338,
122.653421973431));
#213363=CARTESIAN_POINT('Ctrl Pts',(6.72716700892878,-0.733152803977599,
122.662443127164));
#213364=CARTESIAN_POINT('Ctrl Pts',(6.74793904520336,-0.542555487324775,
122.671473459991));
#213365=CARTESIAN_POINT('Ctrl Pts',(6.76059516827323,-0.351180196221352,
122.680503792818));
#213366=CARTESIAN_POINT('Ctrl Pts',(6.7651153201899,-0.159698793144974,
122.689534125645));
#213367=CARTESIAN_POINT('Ctrl Pts',(6.76964188025714,0.0320540702023941,
122.698577260638));
#213368=CARTESIAN_POINT('Ctrl Pts',(6.76600940053277,0.223913107298821,
122.707620395631));
#213369=CARTESIAN_POINT('Ctrl Pts',(6.75424998838656,0.415206086636707,
122.716663530623));
#213370=CARTESIAN_POINT('Ctrl Pts',(6.74396955296085,0.582440221899917,
122.724569314023));
#213371=CARTESIAN_POINT('Ctrl Pts',(6.72747867853568,0.749241671908771,
122.732475097423));
#213372=CARTESIAN_POINT('Ctrl Pts',(6.70483124652019,0.915164988232458,
122.740380880823));
#213373=CARTESIAN_POINT('Ctrl Pts',(6.68004217607765,1.09677872587814,122.749034269051));
#213374=CARTESIAN_POINT('Ctrl Pts',(6.64785392676412,1.27750066544207,122.75768765728));
#213375=CARTESIAN_POINT('Ctrl Pts',(6.60834717308811,1.45672119499182,122.766341045508));
#213376=CARTESIAN_POINT('Ctrl Pts',(6.56887690670154,1.63577620166947,122.774986441718));
#213377=CARTESIAN_POINT('Ctrl Pts',(6.52210168245897,1.81333226819031,122.783631837929));
#213378=CARTESIAN_POINT('Ctrl Pts',(6.46815349153584,1.98878842764451,122.792277234139));
#213379=CARTESIAN_POINT('Ctrl Pts',(6.41248237712525,2.16984806578764,122.801198735182));
#213380=CARTESIAN_POINT('Ctrl Pts',(6.34917258687866,2.34867112524306,122.810120236224));
#213381=CARTESIAN_POINT('Ctrl Pts',(6.27842599637712,2.52461007048931,122.819041737266));
#213382=CARTESIAN_POINT('Ctrl Pts',(6.20999946159672,2.69477929378009,122.827670667608));
#213383=CARTESIAN_POINT('Ctrl Pts',(6.13461626194751,2.86225024761858,122.83629959795));
#213384=CARTESIAN_POINT('Ctrl Pts',(6.05250938115007,3.02645323623056,122.844928528292));
#213385=CARTESIAN_POINT('Ctrl Pts',(5.96622665236134,3.19900737292537,122.853996314685));
#213386=CARTESIAN_POINT('Ctrl Pts',(5.8725186044353,3.36795214795712,122.863064101078));
#213387=CARTESIAN_POINT('Ctrl Pts',(5.77171275169471,3.53265069203349,122.87213188747));
#213388=CARTESIAN_POINT('Ctrl Pts',(5.67090689895412,3.69734923610987,122.881199673863));
#213389=CARTESIAN_POINT('Ctrl Pts',(5.56300341523561,3.85780119777594,122.890267460255));
#213390=CARTESIAN_POINT('Ctrl Pts',(5.44838605790935,4.01339985099653,122.899335246648));
#213391=CARTESIAN_POINT('Ctrl Pts',(5.34189812586908,4.15796241286531,122.907759885321));
#213392=CARTESIAN_POINT('Ctrl Pts',(5.22966184849886,4.29827242193654,122.916184523994));
#213393=CARTESIAN_POINT('Ctrl Pts',(5.11205059082547,4.43387277183739,122.924609162667));
#213394=CARTESIAN_POINT('Ctrl Pts',(4.99441265715437,4.56950387793195,122.933035712175));
#213395=CARTESIAN_POINT('Ctrl Pts',(4.87139752987366,4.7004229447189,122.941462261682));
#213396=CARTESIAN_POINT('Ctrl Pts',(4.74341731004143,4.82620774757981,122.949888811189));
#213397=CARTESIAN_POINT('Ctrl Pts',(4.61533543104192,4.95209246571146,122.9583220542));
#213398=CARTESIAN_POINT('Ctrl Pts',(4.48228081448538,5.07283453686664,122.966755297211));
#213399=CARTESIAN_POINT('Ctrl Pts',(4.3447015490879,5.18804948408872,122.975188540221));
#213400=CARTESIAN_POINT('Ctrl Pts',(4.20706729330589,5.30331048268513,122.983625153996));
#213401=CARTESIAN_POINT('Ctrl Pts',(4.06490504063142,5.41303974396053,122.992061767771));
#213402=CARTESIAN_POINT('Ctrl Pts',(3.91869455972253,5.51689423023508,123.000498381546));
#213403=CARTESIAN_POINT('Ctrl Pts',(3.7723277024002,5.62085979193994,123.008944018528));
#213404=CARTESIAN_POINT('Ctrl Pts',(3.62190423832323,5.71893783470141,123.01738965551));
#213405=CARTESIAN_POINT('Ctrl Pts',(3.46793251418037,5.81082894921978,123.025835292491));
#213406=CARTESIAN_POINT('Ctrl Pts',(3.34709022149075,5.88294824916281,123.032463718209));
#213407=CARTESIAN_POINT('Ctrl Pts',(3.22406290923529,5.95125748312322,123.039092143926));
#213408=CARTESIAN_POINT('Ctrl Pts',(3.09910619832137,6.01563211736939,123.045720569644));
#213409=CARTESIAN_POINT('Ctrl Pts',(3.09910619832141,6.01563211736936,121.045612484544));
#213410=CARTESIAN_POINT('Ctrl Pts',(2.94204558016879,6.09654589762258,121.053919780138));
#213411=CARTESIAN_POINT('Ctrl Pts',(2.7818976882948,6.171261813576,121.062227075732));
#213412=CARTESIAN_POINT('Ctrl Pts',(2.61919150026186,6.2395612734355,121.070534371327));
#213413=CARTESIAN_POINT('Ctrl Pts',(2.4562892289586,6.3079430435108,121.078851678351));
#213414=CARTESIAN_POINT('Ctrl Pts',(2.29082282420696,6.36989277750003,121.087168985376));
#213415=CARTESIAN_POINT('Ctrl Pts',(2.12333909727934,6.42524085758386,121.095486292401));
#213416=CARTESIAN_POINT('Ctrl Pts',(1.95573595193907,6.48062840168004,121.103809529791));
#213417=CARTESIAN_POINT('Ctrl Pts',(1.78611294965967,6.52940480989312,121.11213276718));
#213418=CARTESIAN_POINT('Ctrl Pts',(1.61502892522468,6.57145117692338,121.12045600457));
#213419=CARTESIAN_POINT('Ctrl Pts',(1.44371479025191,6.61355409693783,121.128790436836));
#213420=CARTESIAN_POINT('Ctrl Pts',(1.27093604800497,6.64890882715584,121.137124869103));
#213421=CARTESIAN_POINT('Ctrl Pts',(1.09725947931928,6.67744791331569,121.14545930137));
#213422=CARTESIAN_POINT('Ctrl Pts',(1.05990364943842,6.68358634209517,121.147251941772));
#213423=CARTESIAN_POINT('Ctrl Pts',(1.02250629318168,6.68940964984961,121.149044582174));
#213424=CARTESIAN_POINT('Ctrl Pts',(0.985073060578742,6.69491748009802,
121.150837222576));
#213425=CARTESIAN_POINT('Ctrl Pts',(0.81656161670387,6.71971182360619,121.158907068579));
#213426=CARTESIAN_POINT('Ctrl Pts',(0.646802256991129,6.73818555874121,
121.166976914581));
#213427=CARTESIAN_POINT('Ctrl Pts',(0.476320390783657,6.75021539547619,
121.175046760584));
#213428=CARTESIAN_POINT('Ctrl Pts',(0.306053012448628,6.76223009714639,
121.183106453694));
#213429=CARTESIAN_POINT('Ctrl Pts',(0.135065303714053,6.76781700567055,
121.191166146804));
#213430=CARTESIAN_POINT('Ctrl Pts',(-0.0361066108435397,6.76690367248222,
121.199225839914));
#213431=CARTESIAN_POINT('Ctrl Pts',(-0.207100736180612,6.76599128793548,
121.207277161753));
#213432=CARTESIAN_POINT('Ctrl Pts',(-0.378278316683939,6.75859209926884,
121.215328483592));
#213433=CARTESIAN_POINT('Ctrl Pts',(-0.549097671755492,6.74468537048784,
121.22337980543));
#213434=CARTESIAN_POINT('Ctrl Pts',(-0.719777036137056,6.73079003861533,
121.231424529011));
#213435=CARTESIAN_POINT('Ctrl Pts',(-0.890098389427189,6.7103978113129,
121.239469252592));
#213436=CARTESIAN_POINT('Ctrl Pts',(-1.0595197193612,6.68354000244517,121.247513976173));
#213437=CARTESIAN_POINT('Ctrl Pts',(-1.22883929072215,6.65669832503094,
121.255553867898));
#213438=CARTESIAN_POINT('Ctrl Pts',(-1.39725954727955,6.6233988549412,121.263593759622));
#213439=CARTESIAN_POINT('Ctrl Pts',(-1.56424337856943,6.58372475522798,
121.271633651346));
#213440=CARTESIAN_POINT('Ctrl Pts',(-1.73482282923047,6.5431963634533,121.279846663966));
#213441=CARTESIAN_POINT('Ctrl Pts',(-1.90390289527555,6.49601573360834,
121.288059676586));
#213442=CARTESIAN_POINT('Ctrl Pts',(-2.0709212771454,6.44232675854512,121.296272689206));
#213443=CARTESIAN_POINT('Ctrl Pts',(-2.23436205721034,6.3897878232077,121.304309775749));
#213444=CARTESIAN_POINT('Ctrl Pts',(-2.39582821654682,6.33101667239781,
121.312346862291));
#213445=CARTESIAN_POINT('Ctrl Pts',(-2.55480799265003,6.26619861803722,
121.320383948834));
#213446=CARTESIAN_POINT('Ctrl Pts',(-2.71380298385776,6.20137436028714,
121.328421804563));
#213447=CARTESIAN_POINT('Ctrl Pts',(-2.87031077198364,6.13050218760935,
121.336459660292));
#213448=CARTESIAN_POINT('Ctrl Pts',(-3.02383976469844,6.0538154974717,121.344497516021));
#213449=CARTESIAN_POINT('Ctrl Pts',(-3.1774138700719,5.97710627386715,121.352537733578));
#213450=CARTESIAN_POINT('Ctrl Pts',(-3.32800710375322,5.89457929890251,
121.360577951135));
#213451=CARTESIAN_POINT('Ctrl Pts',(-3.47515279545853,5.80651376027103,
121.368618168692));
#213452=CARTESIAN_POINT('Ctrl Pts',(-3.62785774567492,5.71512104916513,
121.37696215082));
#213453=CARTESIAN_POINT('Ctrl Pts',(-3.7768491831015,5.61776332756665,121.385306132948));
#213454=CARTESIAN_POINT('Ctrl Pts',(-3.92163979247268,5.51480102434302,
121.393650115075));
#213455=CARTESIAN_POINT('Ctrl Pts',(-4.061402157267,5.41541436490633,121.40170432991));
#213456=CARTESIAN_POINT('Ctrl Pts',(-4.1972503219034,5.31080614354025,121.409758544745));
#213457=CARTESIAN_POINT('Ctrl Pts',(-4.32878130281717,5.20134034960033,
121.41781275958));
#213458=CARTESIAN_POINT('Ctrl Pts',(-4.46041071291908,5.09179263861584,
121.425873001663));
#213459=CARTESIAN_POINT('Ctrl Pts',(-4.58771623060037,4.97738036514048,
121.433933243746));
#213460=CARTESIAN_POINT('Ctrl Pts',(-4.7103326365377,4.8585034170172,121.441993485829));
#213461=CARTESIAN_POINT('Ctrl Pts',(-4.83312046862225,4.73946027076525,
121.450064996684));
#213462=CARTESIAN_POINT('Ctrl Pts',(-4.95120585348521,4.61594026364948,
121.458136507538));
#213463=CARTESIAN_POINT('Ctrl Pts',(-5.06426426442198,4.48837570398229,
121.466208018392));
#213464=CARTESIAN_POINT('Ctrl Pts',(-5.07611396631286,4.47500560624809,
121.467053997003));
#213465=CARTESIAN_POINT('Ctrl Pts',(-5.08790848559677,4.46159110345672,
121.467899975614));
#213466=CARTESIAN_POINT('Ctrl Pts',(-5.09964747685105,4.44813271068285,
121.468745954225));
#213467=CARTESIAN_POINT('Ctrl Pts',(-5.21424242035397,4.31675312906851,
121.477004318936));
#213468=CARTESIAN_POINT('Ctrl Pts',(-5.32392444122093,4.1807505237948,121.485262683647));
#213469=CARTESIAN_POINT('Ctrl Pts',(-5.42830024888106,4.04052538761951,
121.493521048358));
#213470=CARTESIAN_POINT('Ctrl Pts',(-5.53555032069353,3.89643878113611,
121.502006829002));
#213471=CARTESIAN_POINT('Ctrl Pts',(-5.63719743999163,3.74789396437864,
121.510492609646));
#213472=CARTESIAN_POINT('Ctrl Pts',(-5.73285536328357,3.59536623776644,
121.51897839029));
#213473=CARTESIAN_POINT('Ctrl Pts',(-5.82570433800763,3.44731741394123,
121.527214990097));
#213474=CARTESIAN_POINT('Ctrl Pts',(-5.91291065018202,3.29551660341996,
121.535451589903));
#213475=CARTESIAN_POINT('Ctrl Pts',(-5.99416188644328,3.14043186187996,
121.54368818971));
#213476=CARTESIAN_POINT('Ctrl Pts',(-6.07534980920209,2.98546796721707,
121.551918371301));
#213477=CARTESIAN_POINT('Ctrl Pts',(-6.15059173290633,2.82722555084991,
121.560148552892));
#213478=CARTESIAN_POINT('Ctrl Pts',(-6.21961939842397,2.66620020605135,
121.568378734483));
#213479=CARTESIAN_POINT('Ctrl Pts',(-6.28860554740525,2.50527170958934,
121.576603966049));
#213480=CARTESIAN_POINT('Ctrl Pts',(-6.35138474309997,2.34156394440105,
121.584829197616));
#213481=CARTESIAN_POINT('Ctrl Pts',(-6.40773536301101,2.17559566960826,
121.593054429182));
#213482=CARTESIAN_POINT('Ctrl Pts',(-6.46406210785872,2.00969771352849,
121.601276175819));
#213483=CARTESIAN_POINT('Ctrl Pts',(-6.51396558948852,1.84154149221128,
121.609497922457));
#213484=CARTESIAN_POINT('Ctrl Pts',(-6.55727285957674,1.67166433384763,
121.617719669094));
#213485=CARTESIAN_POINT('Ctrl Pts',(-6.60057367130336,1.5018125090623,121.625940189632));
#213486=CARTESIAN_POINT('Ctrl Pts',(-6.63728013996174,1.33024060200164,
121.63416071017));
#213487=CARTESIAN_POINT('Ctrl Pts',(-6.66726953062416,1.15749989460504,
121.642381230707));
#213488=CARTESIAN_POINT('Ctrl Pts',(-6.69725658057649,0.984772669840407,
121.650601109623));
#213489=CARTESIAN_POINT('Ctrl Pts',(-6.72052754009912,0.810877177457831,
121.658820988539));
#213490=CARTESIAN_POINT('Ctrl Pts',(-6.73701103441075,0.636373571283254,
121.667040867455));
#213491=CARTESIAN_POINT('Ctrl Pts',(-6.75349872518262,0.461825539003984,
121.675262839033));
#213492=CARTESIAN_POINT('Ctrl Pts',(-6.76319546963717,0.286669438060289,
121.683484810612));
#213493=CARTESIAN_POINT('Ctrl Pts',(-6.76608184523593,0.111469563418846,
121.691706782191));
#213494=CARTESIAN_POINT('Ctrl Pts',(-6.76672228928576,0.0725953028088449,
121.693531116064));
#213495=CARTESIAN_POINT('Ctrl Pts',(-6.76702764152326,0.0337188896224528,
121.695355449937));
#213496=CARTESIAN_POINT('Ctrl Pts',(-6.76699803763021,-0.00515351422502416,
121.69717978381));
#213497=CARTESIAN_POINT('',(-6.76699969784176,0.00142993171423264,121.30282021619));
#213498=CARTESIAN_POINT('Ctrl Pts',(3.09910619832143,6.01563211736935,120.651489390257));
#213499=CARTESIAN_POINT('Ctrl Pts',(2.93676012016632,6.0992688370469,120.660077321312));
#213500=CARTESIAN_POINT('Ctrl Pts',(2.77097677061675,6.17635490515243,120.668665252367));
#213501=CARTESIAN_POINT('Ctrl Pts',(2.6023165691788,6.24661808291315,120.677253183423));
#213502=CARTESIAN_POINT('Ctrl Pts',(2.43690585560943,6.31552753678527,120.685675655303));
#213503=CARTESIAN_POINT('Ctrl Pts',(2.2687284581089,6.37787448913762,120.694098127183));
#213504=CARTESIAN_POINT('Ctrl Pts',(2.09833435009174,6.43345023725412,120.702520599063));
#213505=CARTESIAN_POINT('Ctrl Pts',(1.92794913531729,6.48902308475027,120.710942631356));
#213506=CARTESIAN_POINT('Ctrl Pts',(1.75534775773976,6.53782532931774,120.719364663649));
#213507=CARTESIAN_POINT('Ctrl Pts',(1.58109654221623,6.5796977684535,120.727786695941));
#213508=CARTESIAN_POINT('Ctrl Pts',(1.40683009712605,6.62157386724293,120.73620946432));
#213509=CARTESIAN_POINT('Ctrl Pts',(1.23091385096143,6.65651887566472,120.744632232699));
#213510=CARTESIAN_POINT('Ctrl Pts',(1.05392590273805,6.68442437248996,120.753055001078));
#213511=CARTESIAN_POINT('Ctrl Pts',(0.87085903342554,6.71328832617544,120.761767062287));
#213512=CARTESIAN_POINT('Ctrl Pts',(0.686645910593815,6.73462053310505,
120.770479123495));
#213513=CARTESIAN_POINT('Ctrl Pts',(0.501933752710862,6.74835917152382,
120.779191184704));
#213514=CARTESIAN_POINT('Ctrl Pts',(0.323187364936479,6.76165408409719,
120.787621866739));
#213515=CARTESIAN_POINT('Ctrl Pts',(0.14397401722713,6.76783830706771,120.796052548774));
#213516=CARTESIAN_POINT('Ctrl Pts',(-0.0351181501188691,6.76690887448119,
120.804483230808));
#213517=CARTESIAN_POINT('Ctrl Pts',(-0.22317628353502,6.7659329113224,120.813335981604));
#213518=CARTESIAN_POINT('Ctrl Pts',(-0.411100371938996,6.75711274275371,
120.822188732399));
#213519=CARTESIAN_POINT('Ctrl Pts',(-0.598213628239119,6.74050661708666,
120.831041483194));
#213520=CARTESIAN_POINT('Ctrl Pts',(-0.785326884539114,6.72390049141962,
120.839894233989));
#213521=CARTESIAN_POINT('Ctrl Pts',(-0.971628892828559,6.69950849344904,
120.848746984785));
#213522=CARTESIAN_POINT('Ctrl Pts',(-1.15645336321467,6.66745113358242,
120.85759973558));
#213523=CARTESIAN_POINT('Ctrl Pts',(-1.32639133558461,6.63797580099314,
120.865739450613));
#213524=CARTESIAN_POINT('Ctrl Pts',(-1.49541906581941,6.60196152228329,
120.873879165646));
#213525=CARTESIAN_POINT('Ctrl Pts',(-1.66299074861171,6.55947793425909,
120.882018880678));
#213526=CARTESIAN_POINT('Ctrl Pts',(-1.83041587421548,6.51703150212612,
120.890151476765));
#213527=CARTESIAN_POINT('Ctrl Pts',(-1.99638713462422,6.46812711231021,
120.898284072852));
#213528=CARTESIAN_POINT('Ctrl Pts',(-2.16036679753926,6.41288580126685,
120.906416668939));
#213529=CARTESIAN_POINT('Ctrl Pts',(-2.32423435516029,6.35768225614706,
120.914543705147));
#213530=CARTESIAN_POINT('Ctrl Pts',(-2.48611268046784,6.29615053153927,
120.922670741355));
#213531=CARTESIAN_POINT('Ctrl Pts',(-2.64547718357034,6.22846204702323,
120.930797777563));
#213532=CARTESIAN_POINT('Ctrl Pts',(-2.80476550755562,6.16080591882805,
120.9389209289));
#213533=CARTESIAN_POINT('Ctrl Pts',(-2.96154206587183,6.08699903414881,
120.947044080238));
#213534=CARTESIAN_POINT('Ctrl Pts',(-3.11530032927466,6.00726167720545,
120.955167231575));
#213535=CARTESIAN_POINT('Ctrl Pts',(-3.26901538546231,5.92754672705222,
120.963288100247));
#213536=CARTESIAN_POINT('Ctrl Pts',(-3.41971351166351,5.84190479313356,
120.971408968919));
#213537=CARTESIAN_POINT('Ctrl Pts',(-3.56691099203656,5.75060300967549,
120.97952983759));
#213538=CARTESIAN_POINT('Ctrl Pts',(-3.71411642752588,5.65929629191894,
120.987651145145));
#213539=CARTESIAN_POINT('Ctrl Pts',(-3.85782052591071,5.56232930319305,
120.995772452699));
#213540=CARTESIAN_POINT('Ctrl Pts',(-3.99756672125206,5.46001367298087,
121.003893760254));
#213541=CARTESIAN_POINT('Ctrl Pts',(-4.07018370218445,5.40684691484442,
121.008113873971));
#213542=CARTESIAN_POINT('Ctrl Pts',(-4.14173244557785,5.35223662807531,
121.012333987688));
#213543=CARTESIAN_POINT('Ctrl Pts',(-4.21215220819042,5.29623099713717,
121.016554101404));
#213544=CARTESIAN_POINT('Ctrl Pts',(-4.36207281949341,5.17699744514624,
121.02553853993));
#213545=CARTESIAN_POINT('Ctrl Pts',(-4.50680025120209,5.05149644001659,
121.034522978456));
#213546=CARTESIAN_POINT('Ctrl Pts',(-4.64585411787622,4.92019598343527,
121.043507416982));
#213547=CARTESIAN_POINT('Ctrl Pts',(-4.78514798322573,4.78866891010168,
121.052507362112));
#213548=CARTESIAN_POINT('Ctrl Pts',(-4.91874853773518,4.65132254309186,
121.061507307243));
#213549=CARTESIAN_POINT('Ctrl Pts',(-5.0462130898982,4.50866082682432,121.070507252373));
#213550=CARTESIAN_POINT('Ctrl Pts',(-5.17397801554991,4.3656629245608,121.079528406106));
#213551=CARTESIAN_POINT('Ctrl Pts',(-5.29557784759204,4.21732478995254,
121.088549559838));
#213552=CARTESIAN_POINT('Ctrl Pts',(-5.41060922740221,4.0641846400416,121.09757071357));
#213553=CARTESIAN_POINT('Ctrl Pts',(-5.52575765254882,3.91088866882001,
121.106601046397));
#213554=CARTESIAN_POINT('Ctrl Pts',(-5.63432413497768,3.75278111558691,
121.115631379225));
#213555=CARTESIAN_POINT('Ctrl Pts',(-5.73594848932957,3.5904294907097,121.124661712052));
#213556=CARTESIAN_POINT('Ctrl Pts',(-5.83771691498145,3.42784770240559,
121.133704847044));
#213557=CARTESIAN_POINT('Ctrl Pts',(-5.93252340688742,3.26101001446649,
121.142747982037));
#213558=CARTESIAN_POINT('Ctrl Pts',(-6.02005244936564,3.09051088121152,
121.15179111703));
#213559=CARTESIAN_POINT('Ctrl Pts',(-6.09657299800208,2.94145535804667,
121.15969690043));
#213560=CARTESIAN_POINT('Ctrl Pts',(-6.16753220670303,2.78960193080615,
121.16760268383));
#213561=CARTESIAN_POINT('Ctrl Pts',(-6.23274904006365,2.63536115240125,
121.175508467229));
#213562=CARTESIAN_POINT('Ctrl Pts',(-6.30502491071771,2.46442542959591,
121.184269968654));
#213563=CARTESIAN_POINT('Ctrl Pts',(-6.37030605864747,2.29041717942685,
121.19303147008));
#213564=CARTESIAN_POINT('Ctrl Pts',(-6.42834697419434,2.11391678629187,
121.201792971505));
#213565=CARTESIAN_POINT('Ctrl Pts',(-6.48630562091307,1.93766656978438,
121.210542054131));
#213566=CARTESIAN_POINT('Ctrl Pts',(-6.537044430923,1.75893153360658,121.219291136757));
#213567=CARTESIAN_POINT('Ctrl Pts',(-6.58036679249632,1.57830981629455,
121.228040219383));
#213568=CARTESIAN_POINT('Ctrl Pts',(-6.62365002613026,1.39785123310881,
121.236781400003));
#213569=CARTESIAN_POINT('Ctrl Pts',(-6.65953010532025,1.2155096460269,121.245522580623));
#213570=CARTESIAN_POINT('Ctrl Pts',(-6.68786034475579,1.03189777063573,
121.254263761243));
#213571=CARTESIAN_POINT('Ctrl Pts',(-6.71615447184363,0.848519943950757,
121.262993799544));
#213572=CARTESIAN_POINT('Ctrl Pts',(-6.73691792362148,0.663875343858194,
121.271723837846));
#213573=CARTESIAN_POINT('Ctrl Pts',(-6.75005511578671,0.47858639119979,
121.280453876147));
#213574=CARTESIAN_POINT('Ctrl Pts',(-6.76127426882419,0.320349753577202,
121.287909322828));
#213575=CARTESIAN_POINT('Ctrl Pts',(-6.76693229069058,0.161643476358914,
121.295364769509));
#213576=CARTESIAN_POINT('Ctrl Pts',(-6.76699939568353,0.00285986342245457,
121.30282021619));
#213577=CARTESIAN_POINT('Ctrl Pts',(-6.767,6.39536411522111E-12,121.30282021619));
#213578=CARTESIAN_POINT('Ctrl Pts',(-6.76700000000018,-0.18600724952047,
121.311569728001));
#213579=CARTESIAN_POINT('Ctrl Pts',(-6.75932637294556,-0.372014355743516,
121.320319239812));
#213580=CARTESIAN_POINT('Ctrl Pts',(-6.74400518264233,-0.557389537481099,
121.329068751624));
#213581=CARTESIAN_POINT('Ctrl Pts',(-6.72868405705155,-0.742763936245481,
121.337818226479));
#213582=CARTESIAN_POINT('Ctrl Pts',(-6.70571545645811,-0.927506130236042,
121.346567701335));
#213583=CARTESIAN_POINT('Ctrl Pts',(-6.67517739404903,-1.11098863989547,
121.355317176191));
#213584=CARTESIAN_POINT('Ctrl Pts',(-6.64463945808788,-1.29447038981503,
121.364066614818));
#213585=CARTESIAN_POINT('Ctrl Pts',(-6.60653217008449,-1.47669218313265,
121.372816053445));
#213586=CARTESIAN_POINT('Ctrl Pts',(-6.56098496092776,-1.65703510598893,
121.381565492072));
#213587=CARTESIAN_POINT('Ctrl Pts',(-6.51543793658404,-1.8373772970832,
121.390314895197));
#213588=CARTESIAN_POINT('Ctrl Pts',(-6.46245112167535,-2.01584035510561,
121.399064298322));
#213589=CARTESIAN_POINT('Ctrl Pts',(-6.40220448374374,-2.19181813760439,
121.407813701447));
#213590=CARTESIAN_POINT('Ctrl Pts',(-6.34195808526631,-2.36779522066803,
121.416563069797));
#213591=CARTESIAN_POINT('Ctrl Pts',(-6.27445201433237,-2.54128677683837,
121.425312438147));
#213592=CARTESIAN_POINT('Ctrl Pts',(-6.1999155507204,-2.71170355384495,
121.434061806497));
#213593=CARTESIAN_POINT('Ctrl Pts',(-6.1253793771684,-2.88211966767164,
121.442811140799));
#213594=CARTESIAN_POINT('Ctrl Pts',(-6.04381298052677,-3.04946076371475,
121.451560475101));
#213595=CARTESIAN_POINT('Ctrl Pts',(-5.95549339335997,-3.2131584837424,
121.460309809403));
#213596=CARTESIAN_POINT('Ctrl Pts',(-5.86717414255579,-3.37685558033198,
121.469059110383));
#213597=CARTESIAN_POINT('Ctrl Pts',(-5.77210188876772,-3.53690907646473,
121.477808411363));
#213598=CARTESIAN_POINT('Ctrl Pts',(-5.67059953347172,-3.69277536969016,
121.486557712343));
#213599=CARTESIAN_POINT('Ctrl Pts',(-5.56909755631575,-3.84864108224646,
121.495306980729));
#213600=CARTESIAN_POINT('Ctrl Pts',(-5.46116568197057,-4.00031938297234,
121.504056249114));
#213601=CARTESIAN_POINT('Ctrl Pts',(-5.34717048533825,-4.14729511859567,
121.512805517499));
#213602=CARTESIAN_POINT('Ctrl Pts',(-5.23317570392064,-4.2942703188764,
121.521554754016));
#213603=CARTESIAN_POINT('Ctrl Pts',(-5.11311782003745,-4.43654276189281,
121.530303990533));
#213604=CARTESIAN_POINT('Ctrl Pts',(-4.98740458984987,-4.57362924351597,
121.53905322705));
#213605=CARTESIAN_POINT('Ctrl Pts',(-4.86169180711989,-4.71071523720013,
121.547802432426));
#213606=CARTESIAN_POINT('Ctrl Pts',(-4.73032391204428,-4.84261509522987,
121.556551637801));
#213607=CARTESIAN_POINT('Ctrl Pts',(-4.59374707013867,-4.96888084538082,
121.565300843177));
#213608=CARTESIAN_POINT('Ctrl Pts',(-4.45717070301724,-5.0951461565922,
121.574050018137));
#213609=CARTESIAN_POINT('Ctrl Pts',(-4.3153856357133,-5.21577720459288,
121.582799193098));
#213610=CARTESIAN_POINT('Ctrl Pts',(-4.16887341029809,-5.33036429232652,
121.591548368058));
#213611=CARTESIAN_POINT('Ctrl Pts',(-4.02236168204004,-5.44495099123396,
121.60029751333));
#213612=CARTESIAN_POINT('Ctrl Pts',(-3.8711230534846,-5.55349359438396,
121.609046658602));
#213613=CARTESIAN_POINT('Ctrl Pts',(-3.71567117018052,-5.65562346298703,
121.617795803874));
#213614=CARTESIAN_POINT('Ctrl Pts',(-3.56021980146092,-5.75775299351476,
121.626544920184));
#213615=CARTESIAN_POINT('Ctrl Pts',(-3.40055544538604,-5.85346967463726,
121.635294036494));
#213616=CARTESIAN_POINT('Ctrl Pts',(-3.23722035987088,-5.94244842986773,
121.644043152805));
#213617=CARTESIAN_POINT('Ctrl Pts',(-3.07388580147412,-6.03142689794411,
121.652792240879));
#213618=CARTESIAN_POINT('Ctrl Pts',(-2.90688078896807,-6.11366734656673,
121.661541328954));
#213619=CARTESIAN_POINT('Ctrl Pts',(-2.73677250721596,-6.18889046952254,
121.670290417029));
#213620=CARTESIAN_POINT('Ctrl Pts',(-2.56666476031712,-6.26411335596233,
121.679039477595));
#213621=CARTESIAN_POINT('Ctrl Pts',(-2.393454025754,-6.33231884500468,121.687788538161));
#213622=CARTESIAN_POINT('Ctrl Pts',(-2.21772856065829,-6.39327529762645,
121.696537598727));
#213623=CARTESIAN_POINT('Ctrl Pts',(-2.04200363348737,-6.45423156365041,
121.705286632511));
#213624=CARTESIAN_POINT('Ctrl Pts',(-1.86376426189486,-6.50793874375599,
121.714035666295));
#213625=CARTESIAN_POINT('Ctrl Pts',(-1.68361577753346,-6.55421443909493,
121.722784700078));
#213626=CARTESIAN_POINT('Ctrl Pts',(-1.50346782967993,-6.60048999661824,
121.731533707806));
#213627=CARTESIAN_POINT('Ctrl Pts',(-1.32141105795182,-6.63933404237674,
121.740282715534));
#213628=CARTESIAN_POINT('Ctrl Pts',(-1.13806375487219,-6.67061465607527,
121.749031723262));
#213629=CARTESIAN_POINT('Ctrl Pts',(-0.954716982604867,-6.7018951792127,
121.75778070566));
#213630=CARTESIAN_POINT('Ctrl Pts',(-0.770079968903871,-6.72561226592209,
121.766529688059));
#213631=CARTESIAN_POINT('Ctrl Pts',(-0.584779765559858,-6.74168536983088,
121.775278670457));
#213632=CARTESIAN_POINT('Ctrl Pts',(-0.39148983065291,-6.75845151013844,
121.784404889467));
#213633=CARTESIAN_POINT('Ctrl Pts',(-0.197478578239945,-6.76689983031621,
121.793531108477));
#213634=CARTESIAN_POINT('Ctrl Pts',(-0.0034628764529491,-6.76699911397118,
121.802657327487));
#213635=CARTESIAN_POINT('Ctrl Pts',(0.184489834653171,-6.76709529501193,
121.811498352152));
#213636=CARTESIAN_POINT('Ctrl Pts',(0.372446404248647,-6.75935639738172,
121.820339376818));
#213637=CARTESIAN_POINT('Ctrl Pts',(0.559755019487608,-6.74380925873193,
121.829180401484));
#213638=CARTESIAN_POINT('Ctrl Pts',(0.745134705521033,-6.72842222659814,
121.837930380094));
#213639=CARTESIAN_POINT('Ctrl Pts',(0.929879431227813,-6.70538706057534,
121.846680358704));
#213640=CARTESIAN_POINT('Ctrl Pts',(1.11336163626749,-6.6747820089414,121.855430337313));
#213641=CARTESIAN_POINT('Ctrl Pts',(1.29684196300662,-6.64417727061024,
121.86418022635));
#213642=CARTESIAN_POINT('Ctrl Pts',(1.47905951217473,-6.60600284890599,
121.872930115386));
#213643=CARTESIAN_POINT('Ctrl Pts',(1.65939532067066,-6.56038841607235,
121.881680004423));
#213644=CARTESIAN_POINT('Ctrl Pts',(1.83972934300786,-6.51477443503261,
121.890429806795));
#213645=CARTESIAN_POINT('Ctrl Pts',(2.01818138406251,-6.46172066062145,
121.899179609167));
#213646=CARTESIAN_POINT('Ctrl Pts',(2.19414528354189,-6.40140730423482,
121.907929411539));
#213647=CARTESIAN_POINT('Ctrl Pts',(2.37010749863978,-6.3410945251865,121.916679130156));
#213648=CARTESIAN_POINT('Ctrl Pts',(2.54358134866429,-6.27352239616516,
121.925428848772));
#213649=CARTESIAN_POINT('Ctrl Pts',(2.71397759435515,-6.19892043966837,
121.934178567388));
#213650=CARTESIAN_POINT('Ctrl Pts',(2.88437226558081,-6.12431917249535,
121.942928205157));
#213651=CARTESIAN_POINT('Ctrl Pts',(3.05168912680909,-6.04268832278822,
121.951677842926));
#213652=CARTESIAN_POINT('Ctrl Pts',(3.21535986273805,-5.9543051612336,121.960427480694));
#213653=CARTESIAN_POINT('Ctrl Pts',(3.37902914072801,-5.86592278697464,
121.969177040524));
#213654=CARTESIAN_POINT('Ctrl Pts',(3.5390521062154,-5.77078835741962,121.977926600353));
#213655=CARTESIAN_POINT('Ctrl Pts',(3.69488522831672,-5.66922500431645,
121.986676160182));
#213656=CARTESIAN_POINT('Ctrl Pts',(3.85071701406922,-5.56766252217106,
121.995425644979));
#213657=CARTESIAN_POINT('Ctrl Pts',(4.00235878822393,-5.45967138329378,
122.004175129776));
#213658=CARTESIAN_POINT('Ctrl Pts',(4.14929549611321,-5.3456183819961,122.012924614573));
#213659=CARTESIAN_POINT('Ctrl Pts',(4.29623099276083,-5.23156632087021,
122.021674027246));
#213660=CARTESIAN_POINT('Ctrl Pts',(4.43846127436019,-5.11145267304972,
122.030423439918));
#213661=CARTESIAN_POINT('Ctrl Pts',(4.57550326054431,-4.98568540049895,
122.039172852591));
#213662=CARTESIAN_POINT('Ctrl Pts',(4.7125441625776,-4.8599191229038,122.047922196046));
#213663=CARTESIAN_POINT('Ctrl Pts',(4.84439664018731,-4.7284995038545,122.056671539501));
#213664=CARTESIAN_POINT('Ctrl Pts',(4.97061286794706,-4.5918728986111,122.065420882957));
#213665=CARTESIAN_POINT('Ctrl Pts',(5.09682813912642,-4.45524732884733,
122.074170160101));
#213666=CARTESIAN_POINT('Ctrl Pts',(5.21740705147794,-4.31341506235842,
122.082919437246));
#213667=CARTESIAN_POINT('Ctrl Pts',(5.33194007545648,-4.16685781275785,
122.091668714391));
#213668=CARTESIAN_POINT('Ctrl Pts',(5.44647226944436,-4.02030162521908,
122.100417928132));
#213669=CARTESIAN_POINT('Ctrl Pts',(5.55495848628062,-3.86902074888007,
122.109167141873));
#213670=CARTESIAN_POINT('Ctrl Pts',(5.65703027291736,-3.71352898080742,
122.117916355614));
#213671=CARTESIAN_POINT('Ctrl Pts',(5.7591013537694,-3.5580382878968,122.126665508858));
#213672=CARTESIAN_POINT('Ctrl Pts',(5.85475793592692,-3.39833700106816,
122.135414662102));
#213673=CARTESIAN_POINT('Ctrl Pts',(5.94367514427335,-3.2349675082367,122.144163815346));
#213674=CARTESIAN_POINT('Ctrl Pts',(6.0325917673258,-3.07159909077844,122.152912910999));
#213675=CARTESIAN_POINT('Ctrl Pts',(6.11476896835867,-2.90456276731555,
122.161662006652));
#213676=CARTESIAN_POINT('Ctrl Pts',(6.18992765547832,-2.73442583003173,
122.170411102305));
#213677=CARTESIAN_POINT('Ctrl Pts',(6.26508587283002,-2.56428995616297,
122.179160143273));
#213678=CARTESIAN_POINT('Ctrl Pts',(6.33322554827111,-2.39105376935333,
122.187909184241));
#213679=CARTESIAN_POINT('Ctrl Pts',(6.39411526732984,-2.21530561054214,
122.196658225209));
#213680=CARTESIAN_POINT('Ctrl Pts',(6.45500462602798,-2.03955849185252,
122.205407214398));
#213681=CARTESIAN_POINT('Ctrl Pts',(6.5086440204069,-1.86129970164718,122.214156203587));
#213682=CARTESIAN_POINT('Ctrl Pts',(6.55485128368551,-1.68113463136251,
122.222905192776));
#213683=CARTESIAN_POINT('Ctrl Pts',(6.60199809554281,-1.49730620117069,
122.231832078247));
#213684=CARTESIAN_POINT('Ctrl Pts',(6.64140720707832,-1.31149343245906,
122.240758963719));
#213685=CARTESIAN_POINT('Ctrl Pts',(6.67293928722847,-1.1243532669774,122.24968584919));
#213686=CARTESIAN_POINT('Ctrl Pts',(6.70384625876226,-0.940923067008742,
122.258435763368));
#213687=CARTESIAN_POINT('Ctrl Pts',(6.72718554579772,-0.756217899523822,
122.267185677545));
#213688=CARTESIAN_POINT('Ctrl Pts',(6.7428778681531,-0.570865181256655,
122.275935591723));
#213689=CARTESIAN_POINT('Ctrl Pts',(6.75856988190833,-0.385516108076151,
122.284685333827));
#213690=CARTESIAN_POINT('Ctrl Pts',(6.76661520773396,-0.199519795228596,
122.293435075932));
#213691=CARTESIAN_POINT('Ctrl Pts',(6.76698651789579,-0.0135080204579373,
122.302184818036));
#213692=CARTESIAN_POINT('Ctrl Pts',(6.76735782124909,0.17250034351063,122.310934399701));
#213693=CARTESIAN_POINT('Ctrl Pts',(6.76005538995196,0.358523882208551,
122.319683981366));
#213694=CARTESIAN_POINT('Ctrl Pts',(6.7451040274238,0.54393074856197,122.328433563031));
#213695=CARTESIAN_POINT('Ctrl Pts',(6.73015291918057,0.729334461612732,
122.337182995888));
#213696=CARTESIAN_POINT('Ctrl Pts',(6.7075531630663,0.914121237632085,122.345932428744));
#213697=CARTESIAN_POINT('Ctrl Pts',(6.67738151874618,1.09766345165853,122.354681861601));
#213698=CARTESIAN_POINT('Ctrl Pts',(6.64721034747622,1.28120278799387,122.363431157279));
#213699=CARTESIAN_POINT('Ctrl Pts',(6.60946757205205,1.46349731860044,122.372180452956));
#213700=CARTESIAN_POINT('Ctrl Pts',(6.56428138111596,1.64392790277869,122.380929748634));
#213701=CARTESIAN_POINT('Ctrl Pts',(6.51909583859932,1.82435589778764,122.389678918759));
#213702=CARTESIAN_POINT('Ctrl Pts',(6.46646716392965,2.00291972191975,122.398428088885));
#213703=CARTESIAN_POINT('Ctrl Pts',(6.40657409872982,2.17901292274375,122.40717725901));
#213704=CARTESIAN_POINT('Ctrl Pts',(6.34668181342186,2.35510383058679,122.415926315209));
#213705=CARTESIAN_POINT('Ctrl Pts',(6.27952541914173,2.52872390822274,122.424675371409));
#213706=CARTESIAN_POINT('Ctrl Pts',(6.20533299175653,2.69928350889972,122.433424427608));
#213707=CARTESIAN_POINT('Ctrl Pts',(6.12831602991689,2.87633637965326,122.442506563766));
#213708=CARTESIAN_POINT('Ctrl Pts',(6.04371690605412,3.05009086601181,122.451588699924));
#213709=CARTESIAN_POINT('Ctrl Pts',(5.95184520316775,3.21991112882469,122.460670836082));
#213710=CARTESIAN_POINT('Ctrl Pts',(5.86333549509423,3.38351691182761,122.469420616426));
#213711=CARTESIAN_POINT('Ctrl Pts',(5.7680761809952,3.54347103711757,122.478170396769));
#213712=CARTESIAN_POINT('Ctrl Pts',(5.66639083309171,3.69923018027458,122.486920177113));
#213713=CARTESIAN_POINT('Ctrl Pts',(5.56470914082364,3.85498372381813,122.495669642898));
#213714=CARTESIAN_POINT('Ctrl Pts',(5.4566020337224,4.00654234701763,122.504419108683));
#213715=CARTESIAN_POINT('Ctrl Pts',(5.34243669839398,4.15339127986435,122.513168574468));
#213716=CARTESIAN_POINT('Ctrl Pts',(5.2282748605078,4.30023571401051,122.521917772214));
#213717=CARTESIAN_POINT('Ctrl Pts',(5.10805534167306,4.44237052028245,122.53066696996));
#213718=CARTESIAN_POINT('Ctrl Pts',(4.98218644340153,4.57931296628501,122.539416167706));
#213719=CARTESIAN_POINT('Ctrl Pts',(4.85632073219798,4.71625194483142,122.548165143917));
#213720=CARTESIAN_POINT('Ctrl Pts',(4.72480612170541,4.84799861524291,122.556914120129));
#213721=CARTESIAN_POINT('Ctrl Pts',(4.58808925235544,4.9741055489827,122.565663096341));
#213722=CARTESIAN_POINT('Ctrl Pts',(4.45136349474297,5.10022068120989,122.574412641342));
#213723=CARTESIAN_POINT('Ctrl Pts',(4.30943501210346,5.22069514871614,122.583162186344));
#213724=CARTESIAN_POINT('Ctrl Pts',(4.16278587432065,5.33511975166036,122.591911731346));
#213725=CARTESIAN_POINT('Ctrl Pts',(4.0161453574073,5.44953762807635,122.600660761999));
#213726=CARTESIAN_POINT('Ctrl Pts',(3.86478496658203,5.5579061753259,122.609409792653));
#213727=CARTESIAN_POINT('Ctrl Pts',(3.70921874747473,5.65985735539175,122.618158823307));
#213728=CARTESIAN_POINT('Ctrl Pts',(3.55365041606185,5.76180991976871,122.626907972757));
#213729=CARTESIAN_POINT('Ctrl Pts',(3.39387638174814,5.85734478552645,122.635657122206));
#213730=CARTESIAN_POINT('Ctrl Pts',(3.23043927904836,5.9461374912107,122.644406271656));
#213731=CARTESIAN_POINT('Ctrl Pts',(3.18691767070633,5.9697820694404,122.646736079572));
#213732=CARTESIAN_POINT('Ctrl Pts',(3.14313645919737,5.9929488063337,122.649065887488));
#213733=CARTESIAN_POINT('Ctrl Pts',(3.09910619832147,6.01563211736933,122.651395695404));
#213734=CARTESIAN_POINT('Origin',(0.,0.,4.30282021618968));
#213735=CARTESIAN_POINT('',(3.09910619832122,6.01563211736946,125.045920265688));
#213736=CARTESIAN_POINT('',(3.09910619832142,6.01563211736936,124.651395695404));
#213737=CARTESIAN_POINT('',(3.09910619832133,6.0156321173694,4.30282021618968));
#213738=CARTESIAN_POINT('',(-6.7669996714996,-0.00210853606402713,123.69717978384));
#213739=CARTESIAN_POINT('Ctrl Pts',(-6.7669996714996,-0.00210853606383412,
123.69717978384));
#213740=CARTESIAN_POINT('Ctrl Pts',(-6.76694565606682,-0.175462182760706,
123.705392103411));
#213741=CARTESIAN_POINT('Ctrl Pts',(-6.76022593160184,-0.349074621583547,
123.713604422982));
#213742=CARTESIAN_POINT('Ctrl Pts',(-6.74680638395335,-0.522391249396756,
123.721816742553));
#213743=CARTESIAN_POINT('Ctrl Pts',(-6.73340288079994,-0.695500658766133,
123.730019243423));
#213744=CARTESIAN_POINT('Ctrl Pts',(-6.7133155311019,-0.868314605660701,
123.738221744294));
#213745=CARTESIAN_POINT('Ctrl Pts',(-6.68656216370095,-1.04027661271554,
123.746424245164));
#213746=CARTESIAN_POINT('Ctrl Pts',(-6.65983534449266,-1.2120679765603,
123.75461860644));
#213747=CARTESIAN_POINT('Ctrl Pts',(-6.6264557350455,-1.38300873047955,
123.762812967715));
#213748=CARTESIAN_POINT('Ctrl Pts',(-6.58649308931571,-1.5525455820672,
123.771007328991));
#213749=CARTESIAN_POINT('Ctrl Pts',(-6.54656197943612,-1.72194864649799,
123.779195223824));
#213750=CARTESIAN_POINT('Ctrl Pts',(-6.50005826186666,-1.88994966590426,
123.787383118657));
#213751=CARTESIAN_POINT('Ctrl Pts',(-6.44710309644667,-2.05600356609314,
123.79557101349));
#213752=CARTESIAN_POINT('Ctrl Pts',(-6.39417896219739,-2.22196016044074,
123.803754110303));
#213753=CARTESIAN_POINT('Ctrl Pts',(-6.3348110199199,-2.38597156598849,
123.811937207115));
#213754=CARTESIAN_POINT('Ctrl Pts',(-6.269170819976,-2.54750588418583,123.820120303928));
#213755=CARTESIAN_POINT('Ctrl Pts',(-6.2035492622953,-2.70899432553823,
123.828301076686));
#213756=CARTESIAN_POINT('Ctrl Pts',(-6.13165912670626,-2.86800674577733,
123.836481849443));
#213757=CARTESIAN_POINT('Ctrl Pts',(-6.05372092055435,-3.02402910304161,
123.844662622201));
#213758=CARTESIAN_POINT('Ctrl Pts',(-5.97579265206773,-3.1800315663663,
123.852842351853));
#213759=CARTESIAN_POINT('Ctrl Pts',(-5.89181800912137,-3.33304440324049,
123.861022081505));
#213760=CARTESIAN_POINT('Ctrl Pts',(-5.80206447742371,-3.48257617286656,
123.869201811157));
#213761=CARTESIAN_POINT('Ctrl Pts',(-5.71230587318667,-3.63211639347809,
123.877382003097));
#213762=CARTESIAN_POINT('Ctrl Pts',(-5.61676791513734,-3.7781748458478,
123.885562195037));
#213763=CARTESIAN_POINT('Ctrl Pts',(-5.51576264018297,-3.92028717024172,
123.893742386977));
#213764=CARTESIAN_POINT('Ctrl Pts',(-5.41473306938529,-4.06243367838265,
123.901924546583));
#213765=CARTESIAN_POINT('Ctrl Pts',(-5.30823377140609,-4.20063187445824,
123.91010670619));
#213766=CARTESIAN_POINT('Ctrl Pts',(-5.19661846995674,-4.33444869362927,
123.918288865796));
#213767=CARTESIAN_POINT('Ctrl Pts',(-5.08489707745208,-4.46839270653969,
123.926478802597));
#213768=CARTESIAN_POINT('Ctrl Pts',(-4.96805019817738,-4.59794674588749,
123.934668739398));
#213769=CARTESIAN_POINT('Ctrl Pts',(-4.84647059857533,-4.72271232843426,
123.942858676199));
#213770=CARTESIAN_POINT('Ctrl Pts',(-4.72483049168749,-4.84754000385503,
123.951052688938));
#213771=CARTESIAN_POINT('Ctrl Pts',(-4.59845323018682,-4.96757422375864,
123.959246701677));
#213772=CARTESIAN_POINT('Ctrl Pts',(-4.46776627529135,-5.08245546063803,
123.967440714415));
#213773=CARTESIAN_POINT('Ctrl Pts',(-4.33690206909243,-5.19749251145458,
123.97564584073));
#213774=CARTESIAN_POINT('Ctrl Pts',(-4.20171676916172,-5.30736238659324,
123.983850967045));
#213775=CARTESIAN_POINT('Ctrl Pts',(-4.06266945072584,-5.41174703160994,
123.99205609336));
#213776=CARTESIAN_POINT('Ctrl Pts',(-3.94992104562226,-5.49638873757973,
123.99870933138));
#213777=CARTESIAN_POINT('Ctrl Pts',(-3.83463399959578,-5.57742468112581,
124.005362569401));
#213778=CARTESIAN_POINT('Ctrl Pts',(-3.71706534913166,-5.65470725946841,
124.012015807422));
#213779=CARTESIAN_POINT('Ctrl Pts',(-3.55915925756001,-5.75850525191355,
124.020951750872));
#213780=CARTESIAN_POINT('Ctrl Pts',(-3.39680241327116,-5.85575152298949,
124.029887694323));
#213781=CARTESIAN_POINT('Ctrl Pts',(-3.23053858472132,-5.94608353898823,
124.038823637774));
#213782=CARTESIAN_POINT('Ctrl Pts',(-3.06452469480442,-6.03627976200791,
124.047746148131));
#213783=CARTESIAN_POINT('Ctrl Pts',(-2.89461576610477,-6.11958234648515,
124.056668658489));
#213784=CARTESIAN_POINT('Ctrl Pts',(-2.72138262653257,-6.19567313534266,
124.065591168846));
#213785=CARTESIAN_POINT('Ctrl Pts',(-2.54857396191163,-6.27157747815426,
124.074491816285));
#213786=CARTESIAN_POINT('Ctrl Pts',(-2.3724575790633,-6.34030519014817,
124.083392463723));
#213787=CARTESIAN_POINT('Ctrl Pts',(-2.19362628326869,-6.40158517317022,
124.092293111161));
#213788=CARTESIAN_POINT('Ctrl Pts',(-2.01507134917033,-6.4627704555417,
124.101180003748));
#213789=CARTESIAN_POINT('Ctrl Pts',(-1.83381011421601,-6.51653088418503,
124.110066896334));
#213790=CARTESIAN_POINT('Ctrl Pts',(-1.65045539686298,-6.56264321618705,
124.11895378892));
#213791=CARTESIAN_POINT('Ctrl Pts',(-1.46757196957798,-6.60863702228256,
124.127817838875));
#213792=CARTESIAN_POINT('Ctrl Pts',(-1.28260604702592,-6.64702189605218,
124.13668188883));
#213793=CARTESIAN_POINT('Ctrl Pts',(-1.09618489742445,-6.67762440323343,
124.145545938785));
#213794=CARTESIAN_POINT('Ctrl Pts',(-0.917951281858252,-6.70688286190061,
124.154020683605));
#213795=CARTESIAN_POINT('Ctrl Pts',(-0.738387766226628,-6.72902777179274,
124.162495428426));
#213796=CARTESIAN_POINT('Ctrl Pts',(-0.558055928185681,-6.74395007254775,
124.170970173246));
#213797=CARTESIAN_POINT('Ctrl Pts',(-0.383380624247193,-6.75840430008827,
124.179179087675));
#213798=CARTESIAN_POINT('Ctrl Pts',(-0.208152740196801,-6.76606701879992,
124.187388002104));
#213799=CARTESIAN_POINT('Ctrl Pts',(-0.0329364771647726,-6.76691984498649,
124.195596916533));
#213800=CARTESIAN_POINT('Ctrl Pts',(0.142321442643743,-6.76777287392816,
124.20380778259));
#213801=CARTESIAN_POINT('Ctrl Pts',(0.31756737984478,-6.76181278307413,
124.212018648647));
#213802=CARTESIAN_POINT('Ctrl Pts',(0.492238098970516,-6.74907331816168,
124.220229514704));
#213803=CARTESIAN_POINT('Ctrl Pts',(0.666981480960584,-6.73632855364312,
124.228443796474));
#213804=CARTESIAN_POINT('Ctrl Pts',(0.841148813312677,-6.71679882248702,
124.236658078243));
#213805=CARTESIAN_POINT('Ctrl Pts',(1.01418285052883,-6.69056964284008,
124.244872360013));
#213806=CARTESIAN_POINT('Ctrl Pts',(1.1874116512138,-6.66431094018083,124.253095887606));
#213807=CARTESIAN_POINT('Ctrl Pts',(1.35950425674739,-6.6313377810379,124.261319415198));
#213808=CARTESIAN_POINT('Ctrl Pts',(1.52991350791545,-6.59178683349954,
124.269542942791));
#213809=CARTESIAN_POINT('Ctrl Pts',(1.70043198478499,-6.55221053534225,
124.277771741344));
#213810=CARTESIAN_POINT('Ctrl Pts',(1.86926461385819,-6.50604813791689,
124.286000539898));
#213811=CARTESIAN_POINT('Ctrl Pts',(2.03588028622283,-6.45348591539249,
124.294229338452));
#213812=CARTESIAN_POINT('Ctrl Pts',(2.20272529172712,-6.40085134517506,
124.302469463288));
#213813=CARTESIAN_POINT('Ctrl Pts',(2.36734691131735,-6.34179947487035,
124.310709588125));
#213814=CARTESIAN_POINT('Ctrl Pts',(2.52923392568352,-6.27656472516388,
124.318949712961));
#213815=CARTESIAN_POINT('Ctrl Pts',(2.60110507922975,-6.24760318843371,
124.322607988331));
#213816=CARTESIAN_POINT('Ctrl Pts',(2.67243756405475,-6.21742362024085,
124.326266263701));
#213817=CARTESIAN_POINT('Ctrl Pts',(2.74318828705647,-6.18604938727102,
124.329924539071));
#213818=CARTESIAN_POINT('Ctrl Pts',(2.90657230218699,-6.11359715022285,
124.338372561833));
#213819=CARTESIAN_POINT('Ctrl Pts',(3.06722604579447,-6.03460517790217,
124.346820584596));
#213820=CARTESIAN_POINT('Ctrl Pts',(3.22460929711039,-5.94930112542551,
124.355268607358));
#213821=CARTESIAN_POINT('Ctrl Pts',(3.38184842788281,-5.86407518841731,
124.363708894014));
#213822=CARTESIAN_POINT('Ctrl Pts',(3.53582274425704,-5.77254885098513,
124.37214918067));
#213823=CARTESIAN_POINT('Ctrl Pts',(3.68601381028946,-5.67499702117591,
124.380589467326));
#213824=CARTESIAN_POINT('Ctrl Pts',(3.83609046294761,-5.57751950493479,
124.389023324294));
#213825=CARTESIAN_POINT('Ctrl Pts',(3.98238933188045,-5.47402582778856,
124.397457181262));
#213826=CARTESIAN_POINT('Ctrl Pts',(4.12441797775684,-5.36483600352855,
124.405891038229));
#213827=CARTESIAN_POINT('Ctrl Pts',(4.26636026284292,-5.25571257235044,
124.414319766974));
#213828=CARTESIAN_POINT('Ctrl Pts',(4.40403723788053,-5.14090010222615,
124.422748495719));
#213829=CARTESIAN_POINT('Ctrl Pts',(4.53698645638378,-5.02076118677141,
124.431177224464));
#213830=CARTESIAN_POINT('Ctrl Pts',(4.66987525092612,-4.90067687313539,
124.439602122445));
#213831=CARTESIAN_POINT('Ctrl Pts',(4.79804032645077,-4.77527116451287,
124.448027020425));
#213832=CARTESIAN_POINT('Ctrl Pts',(4.9210529760274,-4.64494635137285,124.456451918405));
#213833=CARTESIAN_POINT('Ctrl Pts',(5.04403839040315,-4.51465039235862,
124.4648749511));
#213834=CARTESIAN_POINT('Ctrl Pts',(5.16187342264695,-4.37943774076962,
124.473297983794));
#213835=CARTESIAN_POINT('Ctrl Pts',(5.27416647872013,-4.23974727486733,
124.481721016488));
#213836=CARTESIAN_POINT('Ctrl Pts',(5.38644682896153,-4.10007261478262,
124.490143096125));
#213837=CARTESIAN_POINT('Ctrl Pts',(5.49318624423301,-3.95592141028999,
124.498565175763));
#213838=CARTESIAN_POINT('Ctrl Pts',(5.59403346747403,-3.80776556063796,
124.506987255401));
#213839=CARTESIAN_POINT('Ctrl Pts',(5.69488335748529,-3.65960579320218,
124.515409557749));
#213840=CARTESIAN_POINT('Ctrl Pts',(5.78984055749235,-3.50744144535963,
124.523831860097));
#213841=CARTESIAN_POINT('Ctrl Pts',(5.87859698863607,-3.35177362678314,
124.532254162445));
#213842=CARTESIAN_POINT('Ctrl Pts',(5.96736815728036,-3.19607996045076,
124.540677863269));
#213843=CARTESIAN_POINT('Ctrl Pts',(6.04993633971336,-3.03688195353878,
124.549101564093));
#213844=CARTESIAN_POINT('Ctrl Pts',(6.12603910961953,-2.87470586798232,
124.557525264916));
#213845=CARTESIAN_POINT('Ctrl Pts',(6.20219337896567,-2.71242003638648,
124.565954666135));
#213846=CARTESIAN_POINT('Ctrl Pts',(6.27187335126468,-2.54715240129741,
124.574384067354));
#213847=CARTESIAN_POINT('Ctrl Pts',(6.33486410868279,-2.37945071907839,
124.582813468573));
#213848=CARTESIAN_POINT('Ctrl Pts',(6.39787734111564,-2.21168920113211,
124.591245877391));
#213849=CARTESIAN_POINT('Ctrl Pts',(6.45419648821382,-2.04149221869552,
124.599678286209));
#213850=CARTESIAN_POINT('Ctrl Pts',(6.5036561652542,-1.86942383748336,124.608110695026));
#213851=CARTESIAN_POINT('Ctrl Pts',(6.55316160382688,-1.69719625359834,
124.616550905754));
#213852=CARTESIAN_POINT('Ctrl Pts',(6.59579480567521,-1.5230941337976,124.624991116481));
#213853=CARTESIAN_POINT('Ctrl Pts',(6.63144101104968,-1.34769399975232,
124.633431327209));
#213854=CARTESIAN_POINT('Ctrl Pts',(6.65171596439557,-1.24792939655625,
124.638231975046));
#213855=CARTESIAN_POINT('Ctrl Pts',(6.66973146463446,-1.14774503930318,
124.643032622883));
#213856=CARTESIAN_POINT('Ctrl Pts',(6.68547385807063,-1.04724796158993,
124.64783327072));
#213857=CARTESIAN_POINT('Ctrl Pts',(6.71216579650349,-0.876850631483663,
124.655972985753));
#213858=CARTESIAN_POINT('Ctrl Pts',(6.73237306386141,-0.705214189533114,
124.664112700786));
#213859=CARTESIAN_POINT('Ctrl Pts',(6.74598622680419,-0.532877873220674,
124.672252415819));
#213860=CARTESIAN_POINT('Ctrl Pts',(6.75958748375635,-0.360692281216413,
124.680385011906));
#213861=CARTESIAN_POINT('Ctrl Pts',(6.76660608715752,-0.187808395814929,
124.688517607993));
#213862=CARTESIAN_POINT('Ctrl Pts',(6.7669838716605,-0.0147743252546067,
124.69665020408));
#213863=CARTESIAN_POINT('Ctrl Pts',(6.76736139788972,0.15814144993203,124.704777240288));
#213864=CARTESIAN_POINT('Ctrl Pts',(6.76110714337227,0.331206841151615,
124.712904276496));
#213865=CARTESIAN_POINT('Ctrl Pts',(6.74821487702592,0.503869996612238,
124.721031312704));
#213866=CARTESIAN_POINT('Ctrl Pts',(6.73532877341621,0.676450615959723,
124.729154464041));
#213867=CARTESIAN_POINT('Ctrl Pts',(6.71581100385033,0.848629018016744,
124.737277615379));
#213868=CARTESIAN_POINT('Ctrl Pts',(6.68970741387236,1.01985475278647,124.745400766717));
#213869=CARTESIAN_POINT('Ctrl Pts',(6.66361115919718,1.1910323718522,124.753521635388));
#213870=CARTESIAN_POINT('Ctrl Pts',(6.63093282619393,1.36125749525762,124.76164250406));
#213871=CARTESIAN_POINT('Ctrl Pts',(6.59176995638125,1.52998622286268,124.769763372732));
#213872=CARTESIAN_POINT('Ctrl Pts',(6.55260497005717,1.69872406921404,124.777884680286));
#213873=CARTESIAN_POINT('Ctrl Pts',(6.50695482572185,1.86596500055958,124.786005987841));
#213874=CARTESIAN_POINT('Ctrl Pts',(6.45496792438712,2.03117652978107,124.794127295395));
#213875=CARTESIAN_POINT('Ctrl Pts',(6.42795372329491,2.11702618341604,124.798347409112));
#213876=CARTESIAN_POINT('Ctrl Pts',(6.39922929765506,2.20232807948675,124.802567522828));
#213877=CARTESIAN_POINT('Ctrl Pts',(6.36882075883247,2.28700921333182,124.806787636545));
#213878=CARTESIAN_POINT('Ctrl Pts',(6.30408230246524,2.46729166361793,124.815772075071));
#213879=CARTESIAN_POINT('Ctrl Pts',(6.23174008365757,2.64467017177402,124.824756513597));
#213880=CARTESIAN_POINT('Ctrl Pts',(6.15208292973967,2.81853944900649,124.833740952122));
#213881=CARTESIAN_POINT('Ctrl Pts',(6.07228829232828,2.99270881423443,124.842740897253));
#213882=CARTESIAN_POINT('Ctrl Pts',(5.98515358509819,3.16335662550598,124.851740842383));
#213883=CARTESIAN_POINT('Ctrl Pts',(5.89101378387091,3.32990174002822,124.860740787514));
#213884=CARTESIAN_POINT('Ctrl Pts',(5.79665213978569,3.49683932238764,124.869761941246));
#213885=CARTESIAN_POINT('Ctrl Pts',(5.6952524905742,3.65965465480885,124.878783094978));
#213886=CARTESIAN_POINT('Ctrl Pts',(5.58719490563032,3.81779282917482,124.88780424871));
#213887=CARTESIAN_POINT('Ctrl Pts',(5.47902737124187,3.97609191037989,124.896834581538));
#213888=CARTESIAN_POINT('Ctrl Pts',(5.36418850698005,4.12970413239017,124.905864914365));
#213889=CARTESIAN_POINT('Ctrl Pts',(5.24309999454458,4.27810605843365,124.914895247192));
#213890=CARTESIAN_POINT('Ctrl Pts',(5.12183981676803,4.42671837162896,124.923938382185));
#213891=CARTESIAN_POINT('Ctrl Pts',(4.99431242612214,4.5701054340135,124.932981517177));
#213892=CARTESIAN_POINT('Ctrl Pts',(4.86097937264908,4.70777745211902,124.94202465217));
#213893=CARTESIAN_POINT('Ctrl Pts',(4.74441556577524,4.82813451372058,124.94993043557));
#213894=CARTESIAN_POINT('Ctrl Pts',(4.62341526258758,4.94412416538557,124.95783621897));
#213895=CARTESIAN_POINT('Ctrl Pts',(4.49830907481142,5.05544305352847,124.96574200237));
#213896=CARTESIAN_POINT('Ctrl Pts',(4.3613729953246,5.17728812279391,124.974395347207));
#213897=CARTESIAN_POINT('Ctrl Pts',(4.2193959874644,5.29364401377653,124.983048692044));
#213898=CARTESIAN_POINT('Ctrl Pts',(4.07283576707601,5.40410009293188,124.991702036881));
#213899=CARTESIAN_POINT('Ctrl Pts',(3.91978829019922,5.51944533583362,125.000738408349));
#213900=CARTESIAN_POINT('Ctrl Pts',(3.76174285278105,5.62835634690295,125.009774779816));
#213901=CARTESIAN_POINT('Ctrl Pts',(3.59926106435887,5.73041087450021,125.018811151284));
#213902=CARTESIAN_POINT('Ctrl Pts',(3.43677927593659,5.83246540209754,125.027847522752));
#213903=CARTESIAN_POINT('Ctrl Pts',(3.26986143267321,5.92766320656322,125.03688389422));
#213904=CARTESIAN_POINT('Ctrl Pts',(3.09910619832122,6.01563211736946,125.045920265688));
#213905=CARTESIAN_POINT('Ctrl Pts',(3.09910619832137,6.01563211736939,123.045720569644));
#213906=CARTESIAN_POINT('Ctrl Pts',(3.02012383166216,6.05632189648086,123.049910250587));
#213907=CARTESIAN_POINT('Ctrl Pts',(2.9403707940658,6.09544007382996,123.05409993153));
#213908=CARTESIAN_POINT('Ctrl Pts',(2.85991315049611,6.13295897358032,123.058289612473));
#213909=CARTESIAN_POINT('Ctrl Pts',(2.70020941886589,6.20743180215135,123.066605884877));
#213910=CARTESIAN_POINT('Ctrl Pts',(2.53744008902743,6.275734827549,123.074922157281));
#213911=CARTESIAN_POINT('Ctrl Pts',(2.37211676705733,6.33761398662348,123.083238429685));
#213912=CARTESIAN_POINT('Ctrl Pts',(2.20693322615066,6.39944082679608,123.091547670671));
#213913=CARTESIAN_POINT('Ctrl Pts',(2.03920031965934,6.45485450061438,123.099856911657));
#213914=CARTESIAN_POINT('Ctrl Pts',(1.86945128349512,6.50364827605541,123.108166152643));
#213915=CARTESIAN_POINT('Ctrl Pts',(1.69981464746498,6.55240974246525,123.116469891626));
#213916=CARTESIAN_POINT('Ctrl Pts',(1.52816487515849,6.59455994910529,123.124773630608));
#213917=CARTESIAN_POINT('Ctrl Pts',(1.35505229717509,6.62994134754754,123.13307736959));
#213918=CARTESIAN_POINT('Ctrl Pts',(1.18202262106089,6.6653058021946,123.141377131996));
#213919=CARTESIAN_POINT('Ctrl Pts',(1.00753187552673,6.69390783910127,123.149676894402));
#213920=CARTESIAN_POINT('Ctrl Pts',(0.832142794086401,6.71564050335112,
123.157976656807));
#213921=CARTESIAN_POINT('Ctrl Pts',(0.656805572898131,6.73736674153706,
123.166273965082));
#213922=CARTESIAN_POINT('Ctrl Pts',(0.480570890164451,6.7522276130539,123.174571273356));
#213923=CARTESIAN_POINT('Ctrl Pts',(0.30400907717678,6.76016771101088,123.182868581631));
#213924=CARTESIAN_POINT('Ctrl Pts',(0.127429425179038,6.76810861119959,
123.191166728228));
#213925=CARTESIAN_POINT('Ctrl Pts',(-0.0494770758812695,6.76912731746488,
123.199464874825));
#213926=CARTESIAN_POINT('Ctrl Pts',(-0.226137003931016,6.76322046479731,
123.207763021422));
#213927=CARTESIAN_POINT('Ctrl Pts',(-0.402814696247761,6.75731301815855,
123.216062002451));
#213928=CARTESIAN_POINT('Ctrl Pts',(-0.579245418172349,6.74447863558347,
123.224360983479));
#213929=CARTESIAN_POINT('Ctrl Pts',(-0.754857874338941,6.72476606206852,
123.232659964507));
#213930=CARTESIAN_POINT('Ctrl Pts',(-0.930517174245742,6.70504823032364,
123.240961159246));
#213931=CARTESIAN_POINT('Ctrl Pts',(-1.1053574274804,6.67844858968281,123.249262353986));
#213932=CARTESIAN_POINT('Ctrl Pts',(-1.27881437867367,6.64506755307254,
123.257563548725));
#213933=CARTESIAN_POINT('Ctrl Pts',(-1.45234642861127,6.61167206403522,
123.265868337494));
#213934=CARTESIAN_POINT('Ctrl Pts',(-1.62449364134901,6.5714893932261,123.274173126262));
#213935=CARTESIAN_POINT('Ctrl Pts',(-1.79470364850953,6.52467070540932,
123.282477915031));
#213936=CARTESIAN_POINT('Ctrl Pts',(-1.96511543810503,6.47779651445858,
123.290792549052));
#213937=CARTESIAN_POINT('Ctrl Pts',(-2.13358509775705,6.42427068088018,
123.299107183073));
#213938=CARTESIAN_POINT('Ctrl Pts',(-2.29957594429869,6.36429410668637,
123.307421817094));
#213939=CARTESIAN_POINT('Ctrl Pts',(-2.46567174832421,6.30427960877296,
123.315741708532));
#213940=CARTESIAN_POINT('Ctrl Pts',(-2.62928529154253,6.23780636679659,
123.324061599969));
#213941=CARTESIAN_POINT('Ctrl Pts',(-2.78990134639432,6.16512282743719,
123.332381491407));
#213942=CARTESIAN_POINT('Ctrl Pts',(-2.95075757432773,6.09233060261888,
123.34071382378));
#213943=CARTESIAN_POINT('Ctrl Pts',(-3.10860704519385,6.01330967734598,
123.349046156154));
#213944=CARTESIAN_POINT('Ctrl Pts',(-3.26295933800925,5.92835435500428,
123.357378488527));
#213945=CARTESIAN_POINT('Ctrl Pts',(-3.37916881099805,5.86439279630733,
123.363651773725));
#213946=CARTESIAN_POINT('Ctrl Pts',(-3.49339649231599,5.79706835352984,
123.369925058924));
#213947=CARTESIAN_POINT('Ctrl Pts',(-3.60544469942284,5.72652228838793,
123.376198344122));
#213948=CARTESIAN_POINT('Ctrl Pts',(-3.74958158267289,5.63577304556057,
123.384268190125));
#213949=CARTESIAN_POINT('Ctrl Pts',(-3.89055611171987,5.53941070198235,
123.392338036128));
#213950=CARTESIAN_POINT('Ctrl Pts',(-4.02788897276636,5.43768327719326,
123.40040788213));
#213951=CARTESIAN_POINT('Ctrl Pts',(-4.16504905160565,5.33608383844372,
123.408467575241));
#213952=CARTESIAN_POINT('Ctrl Pts',(-4.29857628274578,5.22913296827748,
123.416527268351));
#213953=CARTESIAN_POINT('Ctrl Pts',(-4.42801627508799,5.11712427712635,
123.424586961461));
#213954=CARTESIAN_POINT('Ctrl Pts',(-4.5573218234387,5.00523192479176,123.432638283299));
#213955=CARTESIAN_POINT('Ctrl Pts',(-4.68254830134607,4.88829244775038,
123.440689605138));
#213956=CARTESIAN_POINT('Ctrl Pts',(-4.80327072619441,4.76664235399341,
123.448740926976));
#213957=CARTESIAN_POINT('Ctrl Pts',(-4.92389421602702,4.64509195549981,
123.456785650557));
#213958=CARTESIAN_POINT('Ctrl Pts',(-5.0400207379763,4.51883888733626,123.464830374139));
#213959=CARTESIAN_POINT('Ctrl Pts',(-5.15125890602972,4.38825941382794,
123.47287509772));
#213960=CARTESIAN_POINT('Ctrl Pts',(-5.26243026173404,4.25775836952715,
123.480914989444));
#213961=CARTESIAN_POINT('Ctrl Pts',(-5.36871886700291,4.12293637607806,
123.488954881168));
#213962=CARTESIAN_POINT('Ctrl Pts',(-5.46977077762932,3.98420589831805,
123.496994772893));
#213963=CARTESIAN_POINT('Ctrl Pts',(-5.57299861274131,3.84248817329489,
123.505207785513));
#213964=CARTESIAN_POINT('Ctrl Pts',(-5.6707613933312,3.69669201663191,123.513420798133));
#213965=CARTESIAN_POINT('Ctrl Pts',(-5.76272553304017,3.5472924084218,123.521633810753));
#213966=CARTESIAN_POINT('Ctrl Pts',(-5.85271976339828,3.4010930007046,123.529670897295));
#213967=CARTESIAN_POINT('Ctrl Pts',(-5.93716106226926,3.25144329030274,
123.537707983838));
#213968=CARTESIAN_POINT('Ctrl Pts',(-6.01578116995975,3.09881685731147,
123.54574507038));
#213969=CARTESIAN_POINT('Ctrl Pts',(-6.09440880196054,2.94617581726006,
123.55378292611));
#213970=CARTESIAN_POINT('Ctrl Pts',(-6.16721396225864,2.79055781946378,
123.561820781839));
#213971=CARTESIAN_POINT('Ctrl Pts',(-6.23397498433766,2.63245985622807,
123.569858637568));
#213972=CARTESIAN_POINT('Ctrl Pts',(-6.30075562334466,2.47431543779646,
123.577898855125));
#213973=CARTESIAN_POINT('Ctrl Pts',(-6.36148844380825,2.31368994745968,
123.585939072682));
#213974=CARTESIAN_POINT('Ctrl Pts',(-6.41600048956491,2.15109895586021,
123.593979290239));
#213975=CARTESIAN_POINT('Ctrl Pts',(-6.47257203533698,1.9823651724235,123.602323272366));
#213976=CARTESIAN_POINT('Ctrl Pts',(-6.52244343393842,1.81151489298898,
123.610667254494));
#213977=CARTESIAN_POINT('Ctrl Pts',(-6.56547887783275,1.63913883021911,
123.619011236622));
#213978=CARTESIAN_POINT('Ctrl Pts',(-6.60701979982183,1.47274899132513,
123.627065451457));
#213979=CARTESIAN_POINT('Ctrl Pts',(-6.6421915909967,1.30493794008595,123.635119666292));
#213980=CARTESIAN_POINT('Ctrl Pts',(-6.67092482339485,1.136244252181,123.643173881127));
#213981=CARTESIAN_POINT('Ctrl Pts',(-6.69967955786621,0.967424324945361,
123.65123412321));
#213982=CARTESIAN_POINT('Ctrl Pts',(-6.72198609155787,0.797720813758334,
123.659294365293));
#213983=CARTESIAN_POINT('Ctrl Pts',(-6.73782702997512,0.627675006780346,
123.667354607376));
#213984=CARTESIAN_POINT('Ctrl Pts',(-6.75369011511081,0.457391464100649,
123.675426118231));
#213985=CARTESIAN_POINT('Ctrl Pts',(-6.76306954960573,0.286765040342059,
123.683497629085));
#213986=CARTESIAN_POINT('Ctrl Pts',(-6.76599993523862,0.11633518965076,
123.691569139939));
#213987=CARTESIAN_POINT('Ctrl Pts',(-6.7663070702486,0.0984723618691296,
123.69241511855));
#213988=CARTESIAN_POINT('Ctrl Pts',(-6.766543407694,0.080611686774495,123.693261097161));
#213989=CARTESIAN_POINT('Ctrl Pts',(-6.7667090201264,0.0627537802848805,
123.694107075772));
#213990=CARTESIAN_POINT('Ctrl Pts',(-6.76690952899891,0.0411330079578402,
123.695131311784));
#213991=CARTESIAN_POINT('Ctrl Pts',(-6.76700640827308,0.0195120367193917,
123.696155547797));
#213992=CARTESIAN_POINT('Ctrl Pts',(-6.76699967149979,-0.00210853544012529,
123.69717978381));
#213993=CARTESIAN_POINT('',(-6.767,-9.58377703494387E-10,123.302820216235));
#213994=CARTESIAN_POINT('Ctrl Pts',(3.09910619832147,6.01563211736933,122.651395695404));
#213995=CARTESIAN_POINT('Ctrl Pts',(2.93375330764849,6.10081787314642,122.660145143307));
#213996=CARTESIAN_POINT('Ctrl Pts',(2.76488627843102,6.17918207037025,122.668894591209));
#213997=CARTESIAN_POINT('Ctrl Pts',(2.59307866646743,6.2504585455398,122.677644039111));
#213998=CARTESIAN_POINT('Ctrl Pts',(2.42127244185422,6.3217344451502,122.686393416362));
#213999=CARTESIAN_POINT('Ctrl Pts',(2.24652594672514,6.3859226274182,122.695142793612));
#214000=CARTESIAN_POINT('Ctrl Pts',(2.06943269687175,6.44280508110544,122.703892170862));
#214001=CARTESIAN_POINT('Ctrl Pts',(1.89234081822129,6.49968709436151,122.712641480368));
#214002=CARTESIAN_POINT('Ctrl Pts',(1.71290249405639,6.54926340459532,122.721390789873));
#214003=CARTESIAN_POINT('Ctrl Pts',(1.53172716625107,6.59136563150372,122.730140099378));
#214004=CARTESIAN_POINT('Ctrl Pts',(1.35055318107384,6.633467546407,122.738889344046));
#214005=CARTESIAN_POINT('Ctrl Pts',(1.16764249714472,6.66809542395767,122.747638588713));
#214006=CARTESIAN_POINT('Ctrl Pts',(0.983616340614894,6.6951316562466,122.75638783338));
#214007=CARTESIAN_POINT('Ctrl Pts',(0.799591486714353,6.72216769715955,
122.765137016116));
#214008=CARTESIAN_POINT('Ctrl Pts',(0.614451459527195,6.74161215869367,
122.773886198851));
#214009=CARTESIAN_POINT('Ctrl Pts',(0.428825047910737,6.75339900185709,
122.782635381587));
#214010=CARTESIAN_POINT('Ctrl Pts',(0.243199888597508,6.76518576550219,
122.791384505298));
#214011=CARTESIAN_POINT('Ctrl Pts',(0.057088637392387,6.76931499599834,
122.800133629008));
#214012=CARTESIAN_POINT('Ctrl Pts',(-0.128876626810673,6.76577266947848,
122.808882752719));
#214013=CARTESIAN_POINT('Ctrl Pts',(-0.314840698187782,6.76223036567995,
122.81763182031));
#214014=CARTESIAN_POINT('Ctrl Pts',(-0.500658497950976,6.75101660879225,
122.826380887902));
#214015=CARTESIAN_POINT('Ctrl Pts',(-0.68569895192604,6.7321694829622,122.835129955493));
#214016=CARTESIAN_POINT('Ctrl Pts',(-0.870738280459613,6.71332247176296,
122.843878969872));
#214017=CARTESIAN_POINT('Ctrl Pts',(-1.05499998761221,6.68684221356191,
122.85262798425));
#214018=CARTESIAN_POINT('Ctrl Pts',(-1.23785829161384,6.65281863948529,
122.861376998629));
#214019=CARTESIAN_POINT('Ctrl Pts',(-1.43007412917354,6.61705395368871,
122.870573732328));
#214020=CARTESIAN_POINT('Ctrl Pts',(-1.6207388253573,6.57295372727805,122.879770466027));
#214021=CARTESIAN_POINT('Ctrl Pts',(-1.80913696091439,6.520683434783,122.888967199726));
#214022=CARTESIAN_POINT('Ctrl Pts',(-1.98838356186041,6.4709521981522,122.89771719744));
#214023=CARTESIAN_POINT('Ctrl Pts',(-2.16557827572465,6.41382586850914,
122.906467195154));
#214024=CARTESIAN_POINT('Ctrl Pts',(-2.34011918621636,6.34949849943302,
122.915217192867));
#214025=CARTESIAN_POINT('Ctrl Pts',(-2.51465655691031,6.28517243495577,
122.923967013126));
#214026=CARTESIAN_POINT('Ctrl Pts',(-2.68653996295258,6.21364572242405,
122.932716833384));
#214027=CARTESIAN_POINT('Ctrl Pts',(-2.85518555379916,6.13516132252255,
122.941466653642));
#214028=CARTESIAN_POINT('Ctrl Pts',(-3.02382794858621,6.0566784100054,122.95021630808));
#214029=CARTESIAN_POINT('Ctrl Pts',(-3.18923239109218,5.97123819492115,
122.958965962517));
#214030=CARTESIAN_POINT('Ctrl Pts',(-3.3508370596764,5.87913088810746,122.967715616955));
#214031=CARTESIAN_POINT('Ctrl Pts',(-3.51243888042341,5.78702520443139,
122.976465117204));
#214032=CARTESIAN_POINT('Ctrl Pts',(-3.67024081223631,5.68825280605822,
122.985214617453));
#214033=CARTESIAN_POINT('Ctrl Pts',(-3.82370687544341,5.58314917682546,
122.993964117702));
#214034=CARTESIAN_POINT('Ctrl Pts',(-3.97717043817766,5.47804726008058,
123.002713475392));
#214035=CARTESIAN_POINT('Ctrl Pts',(-4.12629803722421,5.36661448084267,
123.011462833083));
#214036=CARTESIAN_POINT('Ctrl Pts',(-4.27058317206878,5.24922931204601,
123.020212190773));
#214037=CARTESIAN_POINT('Ctrl Pts',(-4.41486614774812,5.13184589986811,
123.028961417533));
#214038=CARTESIAN_POINT('Ctrl Pts',(-4.55430658194397,5.0085104572305,123.037710644293));
#214039=CARTESIAN_POINT('Ctrl Pts',(-4.68843089001835,4.87964187103129,
123.046459871053));
#214040=CARTESIAN_POINT('Ctrl Pts',(-4.82255336917826,4.75077504207971,
123.055208978509));
#214041=CARTESIAN_POINT('Ctrl Pts',(-4.95135966065125,4.61637541908104,
123.063958085965));
#214042=CARTESIAN_POINT('Ctrl Pts',(-5.07441230869235,4.47689945401855,
123.072707193421));
#214043=CARTESIAN_POINT('Ctrl Pts',(-5.19746344226408,4.33742520555527,
123.081456193197));
#214044=CARTESIAN_POINT('Ctrl Pts',(-5.31476088454758,4.19287495491348,
123.090205192974));
#214045=CARTESIAN_POINT('Ctrl Pts',(-5.42590627628844,4.04373961586719,
123.09895419275));
#214046=CARTESIAN_POINT('Ctrl Pts',(-5.53706380672662,3.89458798906743,
123.107704148045));
#214047=CARTESIAN_POINT('Ctrl Pts',(-5.64206777071861,3.74085050155288,
123.11645410334));
#214048=CARTESIAN_POINT('Ctrl Pts',(-5.74056148164008,3.58304938223161,
123.125204058634));
#214049=CARTESIAN_POINT('Ctrl Pts',(-5.83905138951875,3.42525435593296,
123.133953676075));
#214050=CARTESIAN_POINT('Ctrl Pts',(-5.93103139557637,3.26339625497211,
123.142703293517));
#214051=CARTESIAN_POINT('Ctrl Pts',(-6.01618907820824,3.09802485065047,
123.151452910958));
#214052=CARTESIAN_POINT('Ctrl Pts',(-6.10134392544964,2.9326589524968,123.160202237074));
#214053=CARTESIAN_POINT('Ctrl Pts',(-6.17967677261815,2.76378023986072,
123.168951563189));
#214054=CARTESIAN_POINT('Ctrl Pts',(-6.2509215700921,2.5919622922715,123.177700889305));
#214055=CARTESIAN_POINT('Ctrl Pts',(-6.32216437407743,2.42014915229118,
123.186449970608));
#214056=CARTESIAN_POINT('Ctrl Pts',(-6.38631941548914,2.24539720662871,
123.19519905191));
#214057=CARTESIAN_POINT('Ctrl Pts',(-6.44316881037533,2.06829994947699,
123.203948133213));
#214058=CARTESIAN_POINT('Ctrl Pts',(-6.50002334524571,1.89118668024453,
123.212698005555));
#214059=CARTESIAN_POINT('Ctrl Pts',(-6.54957082411098,1.71172794807696,
123.221447877897));
#214060=CARTESIAN_POINT('Ctrl Pts',(-6.59164294296087,1.53053334250324,
123.23019775024));
#214061=CARTESIAN_POINT('Ctrl Pts',(-6.63371214082135,1.34935131693592,
123.238947015095));
#214062=CARTESIAN_POINT('Ctrl Pts',(-6.66830695239689,1.16643393829764,
123.247696279949));
#214063=CARTESIAN_POINT('Ctrl Pts',(-6.69530988153987,0.982402458341086,
123.256445544804));
#214064=CARTESIAN_POINT('Ctrl Pts',(-6.72231419690482,0.79836153094714,
123.265195258811));
#214065=CARTESIAN_POINT('Ctrl Pts',(-6.74172580829277,0.613206671362544,
123.273944972818));
#214066=CARTESIAN_POINT('Ctrl Pts',(-6.75347878028179,0.42756679511345,
123.282694686825));
#214067=CARTESIAN_POINT('Ctrl Pts',(-6.76248992368205,0.285234494207005,
123.289403196614));
#214068=CARTESIAN_POINT('Ctrl Pts',(-6.76699999999986,0.142617266095549,
123.296111706402));
#214069=CARTESIAN_POINT('Ctrl Pts',(-6.767,6.54126883298573E-12,123.30282021619));
#214070=CARTESIAN_POINT('Ctrl Pts',(-6.767,-9.58186202505161E-10,123.302820216235));
#214071=CARTESIAN_POINT('Ctrl Pts',(-6.76699999997366,-0.186007250485151,
123.311569728047));
#214072=CARTESIAN_POINT('Ctrl Pts',(-6.75932637289252,-0.372014356707202,
123.320319239858));
#214073=CARTESIAN_POINT('Ctrl Pts',(-6.74400518256286,-0.557389538442699,
123.329068751669));
#214074=CARTESIAN_POINT('Ctrl Pts',(-6.72868405694564,-0.742763937204996,
123.337818226525));
#214075=CARTESIAN_POINT('Ctrl Pts',(-6.70571545632584,-0.92750613119238,
123.34656770138));
#214076=CARTESIAN_POINT('Ctrl Pts',(-6.67517739389057,-1.11098864084755,
123.355317176236));
#214077=CARTESIAN_POINT('Ctrl Pts',(-6.64463945790326,-1.29447039076273,
123.364066614863));
#214078=CARTESIAN_POINT('Ctrl Pts',(-6.60653216987388,-1.47669218407489,
123.37281605349));
#214079=CARTESIAN_POINT('Ctrl Pts',(-6.56098496069144,-1.65703510692464,
123.381565492117));
#214080=CARTESIAN_POINT('Ctrl Pts',(-6.515437936322,-1.83737729801239,123.390314895242));
#214081=CARTESIAN_POINT('Ctrl Pts',(-6.46245112138787,-2.01584035602721,
123.399064298367));
#214082=CARTESIAN_POINT('Ctrl Pts',(-6.40220448343118,-2.19181813851737,
123.407813701493));
#214083=CARTESIAN_POINT('Ctrl Pts',(-6.34195808492866,-2.3677952215724,
123.416563069843));
#214084=CARTESIAN_POINT('Ctrl Pts',(-6.27445201396999,-2.54128677773308,
123.425312438193));
#214085=CARTESIAN_POINT('Ctrl Pts',(-6.19991555033374,-2.71170355472901,
123.434061806543));
#214086=CARTESIAN_POINT('Ctrl Pts',(-6.12537937675744,-2.88211966854504,
123.442811140845));
#214087=CARTESIAN_POINT('Ctrl Pts',(-6.04381298009196,-3.0494607645765,
123.451560475146));
#214088=CARTESIAN_POINT('Ctrl Pts',(-5.95549339290184,-3.21315848459153,
123.460309809448));
#214089=CARTESIAN_POINT('Ctrl Pts',(-5.86717414207446,-3.37685558116826,
123.469059110428));
#214090=CARTESIAN_POINT('Ctrl Pts',(-5.77210188826372,-3.53690907728723,
123.477808411409));
#214091=CARTESIAN_POINT('Ctrl Pts',(-5.67059953294568,-3.69277537049796,
123.486557712389));
#214092=CARTESIAN_POINT('Ctrl Pts',(-5.56909755576737,-3.84864108303999,
123.495306980774));
#214093=CARTESIAN_POINT('Ctrl Pts',(-5.46116568140044,-4.00031938375068,
123.504056249159));
#214094=CARTESIAN_POINT('Ctrl Pts',(-5.34717048474704,-4.14729511935794,
123.512805517545));
#214095=CARTESIAN_POINT('Ctrl Pts',(-5.23317570330848,-4.29427031962239,
123.521554754062));
#214096=CARTESIAN_POINT('Ctrl Pts',(-5.11311781940504,-4.43654276262166,
123.530303990579));
#214097=CARTESIAN_POINT('Ctrl Pts',(-4.98740458919794,-4.57362924422688,
123.539053227096));
#214098=CARTESIAN_POINT('Ctrl Pts',(-4.86169180644861,-4.71071523789291,
123.547802432471));
#214099=CARTESIAN_POINT('Ctrl Pts',(-4.73032391135441,-4.84261509590373,
123.556551637847));
#214100=CARTESIAN_POINT('Ctrl Pts',(-4.59374706943103,-4.96888084603504,
123.565300843222));
#214101=CARTESIAN_POINT('Ctrl Pts',(-4.45717070229154,-5.09514615722703,
123.574050018182));
#214102=CARTESIAN_POINT('Ctrl Pts',(-4.31538563497034,-5.21577720520759,
123.582799193143));
#214103=CARTESIAN_POINT('Ctrl Pts',(-4.16887340953873,-5.33036429292041,
123.591548368103));
#214104=CARTESIAN_POINT('Ctrl Pts',(-4.02236168126448,-5.44495099180689,
123.600297513375));
#214105=CARTESIAN_POINT('Ctrl Pts',(-3.87112305269371,-5.55349359493526,
123.609046658647));
#214106=CARTESIAN_POINT('Ctrl Pts',(-3.71567116937521,-5.6556234635161,
123.617795803919));
#214107=CARTESIAN_POINT('Ctrl Pts',(-3.5602198006411,-5.75775299402168,
123.62654492023));
#214108=CARTESIAN_POINT('Ctrl Pts',(-3.40055544455261,-5.85346967512143,
123.63529403654));
#214109=CARTESIAN_POINT('Ctrl Pts',(-3.23722035902481,-5.94244843032864,
123.64404315285));
#214110=CARTESIAN_POINT('Ctrl Pts',(-3.07388580061552,-6.03142689838168,
123.652792240925));
#214111=CARTESIAN_POINT('Ctrl Pts',(-2.90688078809791,-6.11366734698046,
123.661541329));
#214112=CARTESIAN_POINT('Ctrl Pts',(-2.73677250633523,-6.188890469912,123.670290417074));
#214113=CARTESIAN_POINT('Ctrl Pts',(-2.56666475942524,-6.26411335632778,
123.679039477641));
#214114=CARTESIAN_POINT('Ctrl Pts',(-2.39345402485196,-6.33231884534564,
123.687788538207));
#214115=CARTESIAN_POINT('Ctrl Pts',(-2.21772855974711,-6.39327529794252,
123.696537598773));
#214116=CARTESIAN_POINT('Ctrl Pts',(-2.04200363256776,-6.45423156394135,
123.705286632556));
#214117=CARTESIAN_POINT('Ctrl Pts',(-1.86376426096788,-6.50793874402146,
123.71403566634));
#214118=CARTESIAN_POINT('Ctrl Pts',(-1.68361577660017,-6.55421443933467,
123.722784700124));
#214119=CARTESIAN_POINT('Ctrl Pts',(-1.50346782874008,-6.60048999683232,
123.731533707851));
#214120=CARTESIAN_POINT('Ctrl Pts',(-1.32141105700646,-6.63933404256489,
123.740282715579));
#214121=CARTESIAN_POINT('Ctrl Pts',(-1.1380637539224,-6.67061465623731,
123.749031723307));
#214122=CARTESIAN_POINT('Ctrl Pts',(-0.95471698165129,-6.70189517934853,
123.757780705705));
#214123=CARTESIAN_POINT('Ctrl Pts',(-0.770079967947586,-6.72561226603156,
123.766529688104));
#214124=CARTESIAN_POINT('Ctrl Pts',(-0.584779764601956,-6.74168536991397,
123.775278670502));
#214125=CARTESIAN_POINT('Ctrl Pts',(-0.39148982970262,-6.7584515101932,
123.784404889512));
#214126=CARTESIAN_POINT('Ctrl Pts',(-0.197478577298523,-6.76689983034339,
123.793531108521));
#214127=CARTESIAN_POINT('Ctrl Pts',(-0.00346287552154453,-6.76699911397165,
123.80265732753));
#214128=CARTESIAN_POINT('Ctrl Pts',(0.184489835574943,-6.76709529498653,
123.811498352196));
#214129=CARTESIAN_POINT('Ctrl Pts',(0.372446405159711,-6.75935639733125,
123.820339376861));
#214130=CARTESIAN_POINT('Ctrl Pts',(0.559755020386987,-6.74380925865727,
123.829180401527));
#214131=CARTESIAN_POINT('Ctrl Pts',(0.745134706418459,-6.72842222649875,
123.837930380136));
#214132=CARTESIAN_POINT('Ctrl Pts',(0.929879432122264,-6.7053870604513,
123.846680358746));
#214133=CARTESIAN_POINT('Ctrl Pts',(1.11336163715795,-6.67478200879287,
123.855430337356));
#214134=CARTESIAN_POINT('Ctrl Pts',(1.29684196389297,-6.64417727043724,
123.864180226392));
#214135=CARTESIAN_POINT('Ctrl Pts',(1.47905951305596,-6.60600284870869,
123.872930115429));
#214136=CARTESIAN_POINT('Ctrl Pts',(1.65939532154578,-6.560388415851,123.881680004465));
#214137=CARTESIAN_POINT('Ctrl Pts',(1.83972934387687,-6.51477443478721,
123.890429806838));
#214138=CARTESIAN_POINT('Ctrl Pts',(2.01818138492442,-6.46172066035225,
123.89917960921));
#214139=CARTESIAN_POINT('Ctrl Pts',(2.19414528439572,-6.40140730394216,
123.907929411582));
#214140=CARTESIAN_POINT('Ctrl Pts',(2.37010749948567,-6.34109452487033,
123.916679130198));
#214141=CARTESIAN_POINT('Ctrl Pts',(2.54358134950125,-6.27352239582582,
123.925428848814));
#214142=CARTESIAN_POINT('Ctrl Pts',(2.71397759518225,-6.19892043930625,
123.934178567431));
#214143=CARTESIAN_POINT('Ctrl Pts',(2.88437226639804,-6.12431917211046,
123.942928205199));
#214144=CARTESIAN_POINT('Ctrl Pts',(3.05168912761553,-6.04268832238096,
123.951677842968));
#214145=CARTESIAN_POINT('Ctrl Pts',(3.21535986353278,-5.95430516080445,
123.960427480737));
#214146=CARTESIAN_POINT('Ctrl Pts',(3.37902914151091,-5.86592278652365,
123.969177040566));
#214147=CARTESIAN_POINT('Ctrl Pts',(3.53905210698558,-5.77078835694729,
123.977926600395));
#214148=CARTESIAN_POINT('Ctrl Pts',(3.69488522907333,-5.66922500382334,
123.986676160224));
#214149=CARTESIAN_POINT('Ctrl Pts',(3.85071701481236,-5.56766252165709,
123.995425645021));
#214150=CARTESIAN_POINT('Ctrl Pts',(4.00235878895273,-5.45967138275952,
124.004175129818));
#214151=CARTESIAN_POINT('Ctrl Pts',(4.14929549682686,-5.34561838144216,
124.012924614616));
#214152=CARTESIAN_POINT('Ctrl Pts',(4.29623099345934,-5.23156632029659,
124.021674027288));
#214153=CARTESIAN_POINT('Ctrl Pts',(4.43846127504273,-5.11145267245704,
124.030423439961));
#214154=CARTESIAN_POINT('Ctrl Pts',(4.57550326121013,-4.98568539988791,
124.039172852633));
#214155=CARTESIAN_POINT('Ctrl Pts',(4.71254416322669,-4.85991912227439,
124.047922196089));
#214156=CARTESIAN_POINT('Ctrl Pts',(4.84439664081892,-4.7284995032074,124.056671539544));
#214157=CARTESIAN_POINT('Ctrl Pts',(4.97061286856049,-4.59187289794708,
124.065420882999));
#214158=CARTESIAN_POINT('Ctrl Pts',(5.09682813972158,-4.45524732816647,
124.074170160144));
#214159=CARTESIAN_POINT('Ctrl Pts',(5.21740705205413,-4.31341506166147,
124.082919437289));
#214160=CARTESIAN_POINT('Ctrl Pts',(5.33194007601308,-4.16685781204562,
124.091668714433));
#214161=CARTESIAN_POINT('Ctrl Pts',(5.44647226998129,-4.02030162449168,
124.100417928175));
#214162=CARTESIAN_POINT('Ctrl Pts',(5.55495848679725,-3.86902074813831,
124.109167141916));
#214163=CARTESIAN_POINT('Ctrl Pts',(5.65703027341314,-3.71352898005216,
124.117916355657));
#214164=CARTESIAN_POINT('Ctrl Pts',(5.75910135424448,-3.55803828712783,
124.126665508901));
#214165=CARTESIAN_POINT('Ctrl Pts',(5.85475793638072,-3.39833700028633,
124.135414662145));
#214166=CARTESIAN_POINT('Ctrl Pts',(5.94367514470539,-3.23496750744291,
124.144163815388));
#214167=CARTESIAN_POINT('Ctrl Pts',(6.032591767736,-3.0715990899728,124.152912911041));
#214168=CARTESIAN_POINT('Ctrl Pts',(6.11476896874655,-2.90456276649896,
124.161662006694));
#214169=CARTESIAN_POINT('Ctrl Pts',(6.18992765584347,-2.73442582920513,
124.170411102347));
#214170=CARTESIAN_POINT('Ctrl Pts',(6.2650858731725,-2.56428995532624,124.179160143315));
#214171=CARTESIAN_POINT('Ctrl Pts',(6.33322554859048,-2.3910537685074,124.187909184283));
#214172=CARTESIAN_POINT('Ctrl Pts',(6.39411526762577,-2.215305609688,124.196658225251));
#214173=CARTESIAN_POINT('Ctrl Pts',(6.45500462630047,-2.03955849099014,
124.20540721444));
#214174=CARTESIAN_POINT('Ctrl Pts',(6.5086440206556,-1.86129970077754,124.214156203629));
#214175=CARTESIAN_POINT('Ctrl Pts',(6.55485128391016,-1.6811346304866,124.222905192818));
#214176=CARTESIAN_POINT('Ctrl Pts',(6.6019980957382,-1.49730620030677,124.231832078289));
#214177=CARTESIAN_POINT('Ctrl Pts',(6.64140720724573,-1.31149343160855,
124.24075896376));
#214178=CARTESIAN_POINT('Ctrl Pts',(6.67293928736931,-1.12435326614156,
124.24968584923));
#214179=CARTESIAN_POINT('Ctrl Pts',(6.70384625888012,-0.940923066169056,
124.258435763408));
#214180=CARTESIAN_POINT('Ctrl Pts',(6.72718554589243,-0.75621789868124,
124.267185677585));
#214181=CARTESIAN_POINT('Ctrl Pts',(6.74287786822459,-0.570865180412135,
124.275935591762));
#214182=CARTESIAN_POINT('Ctrl Pts',(6.75856988195661,-0.385516107229694,
124.284685333867));
#214183=CARTESIAN_POINT('Ctrl Pts',(6.76661520775895,-0.199519794381159,
124.293435075971));
#214184=CARTESIAN_POINT('Ctrl Pts',(6.76698651789748,-0.0135080196104832,
124.302184818076));
#214185=CARTESIAN_POINT('Ctrl Pts',(6.76735782122748,0.172500344358102,
124.310934399741));
#214186=CARTESIAN_POINT('Ctrl Pts',(6.76005538990706,0.35852388305508,124.319683981406));
#214187=CARTESIAN_POINT('Ctrl Pts',(6.74510402735569,0.543930749406598,
124.328433563071));
#214188=CARTESIAN_POINT('Ctrl Pts',(6.73015291908924,0.729334462455587,
124.337182995927));
#214189=CARTESIAN_POINT('Ctrl Pts',(6.70755316295181,0.914121238472207,
124.345932428784));
#214190=CARTESIAN_POINT('Ctrl Pts',(6.67738151860868,1.09766345249497,124.354681861641));
#214191=CARTESIAN_POINT('Ctrl Pts',(6.64721034731574,1.28120278882651,124.363431157318));
#214192=CARTESIAN_POINT('Ctrl Pts',(6.60946757186873,1.46349731942832,124.372180452996));
#214193=CARTESIAN_POINT('Ctrl Pts',(6.56428138091005,1.64392790360088,124.380929748673));
#214194=CARTESIAN_POINT('Ctrl Pts',(6.51909583837082,1.82435589860415,124.389678918799));
#214195=CARTESIAN_POINT('Ctrl Pts',(6.4664671636788,2.00291972272963,124.398428088925));
#214196=CARTESIAN_POINT('Ctrl Pts',(6.40657409845692,2.1790129235461,124.40717725905));
#214197=CARTESIAN_POINT('Ctrl Pts',(6.34668181312688,2.35510383138174,124.415926315249));
#214198=CARTESIAN_POINT('Ctrl Pts',(6.27952541882496,2.52872390900938,124.424675371448));
#214199=CARTESIAN_POINT('Ctrl Pts',(6.20533299141835,2.69928350967715,124.433424427648));
#214200=CARTESIAN_POINT('Ctrl Pts',(6.12831602957061,2.87633638038868,124.442506563804));
#214201=CARTESIAN_POINT('Ctrl Pts',(6.04371690570292,3.05009086670547,124.451588699961));
#214202=CARTESIAN_POINT('Ctrl Pts',(5.95184520281472,3.21991112947724,124.460670836117));
#214203=CARTESIAN_POINT('Ctrl Pts',(5.86333549472327,3.38351691247043,124.469420616461));
#214204=CARTESIAN_POINT('Ctrl Pts',(5.76807618060673,3.54347103774993,124.478170396804));
#214205=CARTESIAN_POINT('Ctrl Pts',(5.66639083268618,3.69923018089576,124.486920177148));
#214206=CARTESIAN_POINT('Ctrl Pts',(5.56470914040105,3.85498372442815,124.495669642933));
#214207=CARTESIAN_POINT('Ctrl Pts',(5.45660203328321,4.00654234761577,124.504419108718));
#214208=CARTESIAN_POINT('Ctrl Pts',(5.34243669793871,4.15339128044996,124.513168574503));
#214209=CARTESIAN_POINT('Ctrl Pts',(5.22827486003637,4.30023571458367,124.521917772249));
#214210=CARTESIAN_POINT('Ctrl Pts',(5.10805534118599,4.44237052084252,124.530666969995));
#214211=CARTESIAN_POINT('Ctrl Pts',(4.98218644289937,4.57931296683135,124.539416167741));
#214212=CARTESIAN_POINT('Ctrl Pts',(4.85632073168066,4.71625194536412,124.548165143952));
#214213=CARTESIAN_POINT('Ctrl Pts',(4.72480612117347,4.84799861576135,124.556914120164));
#214214=CARTESIAN_POINT('Ctrl Pts',(4.58808925180949,4.97410554948628,124.565663096376));
#214215=CARTESIAN_POINT('Ctrl Pts',(4.45136349418311,5.10022068169853,124.574412641377));
#214216=CARTESIAN_POINT('Ctrl Pts',(4.30943501153029,5.22069514918927,124.583162186379));
#214217=CARTESIAN_POINT('Ctrl Pts',(4.16278587373484,5.33511975211744,124.591911731381));
#214218=CARTESIAN_POINT('Ctrl Pts',(4.01614535680894,5.44953762851731,124.600660762034));
#214219=CARTESIAN_POINT('Ctrl Pts',(3.8647849659718,5.55790617575023,124.609409792688));
#214220=CARTESIAN_POINT('Ctrl Pts',(3.70921874685333,5.65985735579898,124.618158823342));
#214221=CARTESIAN_POINT('Ctrl Pts',(3.55365041542928,5.76180992015885,124.626907972791));
#214222=CARTESIAN_POINT('Ctrl Pts',(3.39387638110511,5.85734478589903,124.635657122241));
#214223=CARTESIAN_POINT('Ctrl Pts',(3.23043927839561,5.94613749156533,124.644406271691));
#214224=CARTESIAN_POINT('Ctrl Pts',(3.18691767026854,5.96978206967205,124.646736079595));
#214225=CARTESIAN_POINT('Ctrl Pts',(3.1431364589772,5.99294880644713,124.6490658875));
#214226=CARTESIAN_POINT('Ctrl Pts',(3.09910619832142,6.01563211736936,124.651395695404));
#214227=CARTESIAN_POINT('Origin',(0.,0.,4.30282021618968));
#214228=CARTESIAN_POINT('',(3.09910619832142,6.01563211736936,127.045755263024));
#214229=CARTESIAN_POINT('',(3.0991061983215,6.01563211736932,126.651395695404));
#214230=CARTESIAN_POINT('',(3.09910619832133,6.0156321173694,4.30282021618968));
#214231=CARTESIAN_POINT('',(-6.7669980962981,0.00306854827779037,125.69717978381));
#214232=CARTESIAN_POINT('Ctrl Pts',(-6.767,6.53660624432471E-12,125.69717978381));
#214233=CARTESIAN_POINT('Ctrl Pts',(-6.76700000000018,-0.186007249520428,
125.705929295621));
#214234=CARTESIAN_POINT('Ctrl Pts',(-6.75932637294555,-0.372014355743573,
125.714678807432));
#214235=CARTESIAN_POINT('Ctrl Pts',(-6.74400518264232,-0.557389537481255,
125.723428319244));
#214236=CARTESIAN_POINT('Ctrl Pts',(-6.72868405705154,-0.742763936245608,
125.732177794099));
#214237=CARTESIAN_POINT('Ctrl Pts',(-6.7057154564581,-0.927506130236139,
125.740927268955));
#214238=CARTESIAN_POINT('Ctrl Pts',(-6.67517739404902,-1.11098863989554,
125.749676743811));
#214239=CARTESIAN_POINT('Ctrl Pts',(-6.6446394580879,-1.29447038981495,
125.758426182438));
#214240=CARTESIAN_POINT('Ctrl Pts',(-6.60653217008454,-1.47669218313241,
125.767175621065));
#214241=CARTESIAN_POINT('Ctrl Pts',(-6.56098496092786,-1.65703510598854,
125.775925059692));
#214242=CARTESIAN_POINT('Ctrl Pts',(-6.51543793658422,-1.83737729708254,
125.784674462817));
#214243=CARTESIAN_POINT('Ctrl Pts',(-6.46245112167563,-2.01584035510468,
125.793423865942));
#214244=CARTESIAN_POINT('Ctrl Pts',(-6.40220448374415,-2.1918181376032,
125.802173269067));
#214245=CARTESIAN_POINT('Ctrl Pts',(-6.34195808526676,-2.36779522066683,
125.810922637417));
#214246=CARTESIAN_POINT('Ctrl Pts',(-6.27445201433286,-2.54128677683716,
125.819672005767));
#214247=CARTESIAN_POINT('Ctrl Pts',(-6.19991555072094,-2.71170355384373,
125.828421374117));
#214248=CARTESIAN_POINT('Ctrl Pts',(-6.12537937716893,-2.88211966767052,
125.837170708419));
#214249=CARTESIAN_POINT('Ctrl Pts',(-6.04381298052728,-3.04946076371373,
125.845920042721));
#214250=CARTESIAN_POINT('Ctrl Pts',(-5.95549339336046,-3.21315848374148,
125.854669377023));
#214251=CARTESIAN_POINT('Ctrl Pts',(-5.86717414255645,-3.37685558033082,
125.863418678003));
#214252=CARTESIAN_POINT('Ctrl Pts',(-5.77210188876855,-3.53690907646335,
125.872167978983));
#214253=CARTESIAN_POINT('Ctrl Pts',(-5.67059953347276,-3.69277536968857,
125.880917279963));
#214254=CARTESIAN_POINT('Ctrl Pts',(-5.56909755631677,-3.84864108224499,
125.889666548349));
#214255=CARTESIAN_POINT('Ctrl Pts',(-5.46116568197157,-4.00031938297098,
125.898415816734));
#214256=CARTESIAN_POINT('Ctrl Pts',(-5.34717048533923,-4.14729511859441,
125.907165085119));
#214257=CARTESIAN_POINT('Ctrl Pts',(-5.23317570392174,-4.29427031887504,
125.915914321636));
#214258=CARTESIAN_POINT('Ctrl Pts',(-5.1131178200387,-4.43654276189137,
125.924663558153));
#214259=CARTESIAN_POINT('Ctrl Pts',(-4.98740458985127,-4.57362924351444,
125.93341279467));
#214260=CARTESIAN_POINT('Ctrl Pts',(-4.86169180712117,-4.71071523719882,
125.942162000046));
#214261=CARTESIAN_POINT('Ctrl Pts',(-4.73032391204544,-4.84261509522875,
125.950911205421));
#214262=CARTESIAN_POINT('Ctrl Pts',(-4.59374707013969,-4.96888084537988,
125.959660410797));
#214263=CARTESIAN_POINT('Ctrl Pts',(-4.4571707030184,-5.09514615659118,
125.968409585757));
#214264=CARTESIAN_POINT('Ctrl Pts',(-4.31538563571461,-5.21577720459179,
125.977158760717));
#214265=CARTESIAN_POINT('Ctrl Pts',(-4.16887341029955,-5.33036429232537,
125.985907935678));
#214266=CARTESIAN_POINT('Ctrl Pts',(-4.02236168204176,-5.44495099123268,
125.99465708095));
#214267=CARTESIAN_POINT('Ctrl Pts',(-3.87112305348659,-5.55349359438257,
126.003406226222));
#214268=CARTESIAN_POINT('Ctrl Pts',(-3.71567117018278,-5.65562346298554,
126.012155371494));
#214269=CARTESIAN_POINT('Ctrl Pts',(-3.56021980146347,-5.75775299351318,
126.020904487804));
#214270=CARTESIAN_POINT('Ctrl Pts',(-3.40055544538887,-5.8534696746356,
126.029653604114));
#214271=CARTESIAN_POINT('Ctrl Pts',(-3.23722035987401,-5.94244842986603,
126.038402720424));
#214272=CARTESIAN_POINT('Ctrl Pts',(-3.07388580147733,-6.03142689794247,
126.047151808499));
#214273=CARTESIAN_POINT('Ctrl Pts',(-2.90688078897135,-6.11366734656517,
126.055900896574));
#214274=CARTESIAN_POINT('Ctrl Pts',(-2.7367725072193,-6.18889046952106,
126.064649984649));
#214275=CARTESIAN_POINT('Ctrl Pts',(-2.56666476032041,-6.26411335596098,
126.073399045215));
#214276=CARTESIAN_POINT('Ctrl Pts',(-2.39345402575723,-6.33231884500346,
126.082148105781));
#214277=CARTESIAN_POINT('Ctrl Pts',(-2.21772856066146,-6.39327529762535,
126.090897166347));
#214278=CARTESIAN_POINT('Ctrl Pts',(-2.04200363349071,-6.45423156364935,
126.099646200131));
#214279=CARTESIAN_POINT('Ctrl Pts',(-1.86376426189839,-6.50793874375498,
126.108395233914));
#214280=CARTESIAN_POINT('Ctrl Pts',(-1.68361577753716,-6.55421443909398,
126.117144267698));
#214281=CARTESIAN_POINT('Ctrl Pts',(-1.50346782968394,-6.60048999661732,
126.125893275426));
#214282=CARTESIAN_POINT('Ctrl Pts',(-1.32141105795613,-6.63933404237587,
126.134642283154));
#214283=CARTESIAN_POINT('Ctrl Pts',(-1.1380637548768,-6.67061465607449,
126.143391290882));
#214284=CARTESIAN_POINT('Ctrl Pts',(-0.954716982609653,-6.70189517921202,
126.15214027328));
#214285=CARTESIAN_POINT('Ctrl Pts',(-0.770079968908832,-6.72561226592151,
126.160889255678));
#214286=CARTESIAN_POINT('Ctrl Pts',(-0.584779765564988,-6.74168536983044,
126.169638238077));
#214287=CARTESIAN_POINT('Ctrl Pts',(-0.391489830657955,-6.75845151013815,
126.178764457087));
#214288=CARTESIAN_POINT('Ctrl Pts',(-0.197478578244895,-6.76689983031606,
126.187890676097));
#214289=CARTESIAN_POINT('Ctrl Pts',(-0.00346287645780092,-6.76699911397117,
126.197016895106));
#214290=CARTESIAN_POINT('Ctrl Pts',(0.184489834648418,-6.76709529501206,
126.205857919772));
#214291=CARTESIAN_POINT('Ctrl Pts',(0.372446404243999,-6.75935639738198,
126.214698944438));
#214292=CARTESIAN_POINT('Ctrl Pts',(0.55975501948307,-6.7438092587323,126.223539969104));
#214293=CARTESIAN_POINT('Ctrl Pts',(0.745134705516604,-6.72842222659863,
126.232289947714));
#214294=CARTESIAN_POINT('Ctrl Pts',(0.929879431223498,-6.70538706057594,
126.241039926323));
#214295=CARTESIAN_POINT('Ctrl Pts',(1.11336163626329,-6.6747820089421,126.249789904933));
#214296=CARTESIAN_POINT('Ctrl Pts',(1.29684196300241,-6.64417727061106,
126.25853979397));
#214297=CARTESIAN_POINT('Ctrl Pts',(1.47905951217052,-6.60600284890693,
126.267289683006));
#214298=CARTESIAN_POINT('Ctrl Pts',(1.65939532066645,-6.56038841607342,
126.276039572043));
#214299=CARTESIAN_POINT('Ctrl Pts',(1.83972934300365,-6.5147744350338,126.284789374415));
#214300=CARTESIAN_POINT('Ctrl Pts',(2.01818138405831,-6.46172066062276,
126.293539176787));
#214301=CARTESIAN_POINT('Ctrl Pts',(2.1941452835377,-6.40140730423626,126.302288979159));
#214302=CARTESIAN_POINT('Ctrl Pts',(2.37010749863573,-6.34109452518802,
126.311038697775));
#214303=CARTESIAN_POINT('Ctrl Pts',(2.54358134866037,-6.27352239616675,
126.319788416392));
#214304=CARTESIAN_POINT('Ctrl Pts',(2.71397759435137,-6.19892043967002,
126.328538135008));
#214305=CARTESIAN_POINT('Ctrl Pts',(2.88437226557716,-6.12431917249707,
126.337287772777));
#214306=CARTESIAN_POINT('Ctrl Pts',(3.05168912680559,-6.04268832278999,
126.346037410546));
#214307=CARTESIAN_POINT('Ctrl Pts',(3.21535986273469,-5.95430516123542,
126.354787048314));
#214308=CARTESIAN_POINT('Ctrl Pts',(3.37902914072467,-5.86592278697657,
126.363536608143));
#214309=CARTESIAN_POINT('Ctrl Pts',(3.53905210621208,-5.77078835742165,
126.372286167972));
#214310=CARTESIAN_POINT('Ctrl Pts',(3.69488522831344,-5.66922500431859,
126.381035727801));
#214311=CARTESIAN_POINT('Ctrl Pts',(3.85071701406598,-5.5676625221733,126.389785212599));
#214312=CARTESIAN_POINT('Ctrl Pts',(4.00235878822073,-5.45967138329613,
126.398534697396));
#214313=CARTESIAN_POINT('Ctrl Pts',(4.14929549611005,-5.34561838199855,
126.407284182193));
#214314=CARTESIAN_POINT('Ctrl Pts',(4.29623099275782,-5.23156632087268,
126.416033594865));
#214315=CARTESIAN_POINT('Ctrl Pts',(4.43846127435732,-5.11145267305221,
126.424783007538));
#214316=CARTESIAN_POINT('Ctrl Pts',(4.57550326054159,-4.98568540050145,
126.433532420211));
#214317=CARTESIAN_POINT('Ctrl Pts',(4.71254416257501,-4.85991912290631,
126.442281763666));
#214318=CARTESIAN_POINT('Ctrl Pts',(4.84439664018486,-4.728499503857,126.451031107121));
#214319=CARTESIAN_POINT('Ctrl Pts',(4.97061286794475,-4.5918728986136,126.459780450576));
#214320=CARTESIAN_POINT('Ctrl Pts',(5.09682813912425,-4.45524732884982,
126.468529727721));
#214321=CARTESIAN_POINT('Ctrl Pts',(5.2174070514759,-4.31341506236089,126.477279004866));
#214322=CARTESIAN_POINT('Ctrl Pts',(5.33194007545457,-4.16685781276029,
126.486028282011));
#214323=CARTESIAN_POINT('Ctrl Pts',(5.44647226944242,-4.02030162522171,
126.494777495752));
#214324=CARTESIAN_POINT('Ctrl Pts',(5.55495848627867,-3.86902074888287,
126.503526709493));
#214325=CARTESIAN_POINT('Ctrl Pts',(5.6570302729154,-3.71352898081041,126.512275923234));
#214326=CARTESIAN_POINT('Ctrl Pts',(5.75910135376751,-3.55803828789986,
126.521025076478));
#214327=CARTESIAN_POINT('Ctrl Pts',(5.85475793592509,-3.3983370010713,126.529774229722));
#214328=CARTESIAN_POINT('Ctrl Pts',(5.9436751442716,-3.23496750823992,126.538523382966));
#214329=CARTESIAN_POINT('Ctrl Pts',(6.03259176732412,-3.07159909078173,
126.547272478619));
#214330=CARTESIAN_POINT('Ctrl Pts',(6.11476896835707,-2.90456276731891,
126.556021574272));
#214331=CARTESIAN_POINT('Ctrl Pts',(6.18992765547681,-2.73442583003515,
126.564770669925));
#214332=CARTESIAN_POINT('Ctrl Pts',(6.26508587282854,-2.56428995616658,
126.573519710893));
#214333=CARTESIAN_POINT('Ctrl Pts',(6.33322554826967,-2.39105376935712,
126.582268751861));
#214334=CARTESIAN_POINT('Ctrl Pts',(6.39411526732846,-2.21530561054613,
126.591017792829));
#214335=CARTESIAN_POINT('Ctrl Pts',(6.45500462602674,-2.03955849185645,
126.599766782018));
#214336=CARTESIAN_POINT('Ctrl Pts',(6.5086440204058,-1.86129970165104,126.608515771207));
#214337=CARTESIAN_POINT('Ctrl Pts',(6.55485128368454,-1.68113463136631,
126.617264760396));
#214338=CARTESIAN_POINT('Ctrl Pts',(6.60199809554197,-1.49730620117442,
126.626191645867));
#214339=CARTESIAN_POINT('Ctrl Pts',(6.6414072070776,-1.31149343246271,126.635118531339));
#214340=CARTESIAN_POINT('Ctrl Pts',(6.67293928722787,-1.12435326698098,
126.64404541681));
#214341=CARTESIAN_POINT('Ctrl Pts',(6.70384625876176,-0.94092306701236,
126.652795330987));
#214342=CARTESIAN_POINT('Ctrl Pts',(6.72718554579731,-0.75621789952748,
126.661545245165));
#214343=CARTESIAN_POINT('Ctrl Pts',(6.74287786815278,-0.570865181260349,
126.670295159342));
#214344=CARTESIAN_POINT('Ctrl Pts',(6.75856988190812,-0.385516108079882,
126.679044901447));
#214345=CARTESIAN_POINT('Ctrl Pts',(6.76661520773385,-0.19951979523236,
126.687794643551));
#214346=CARTESIAN_POINT('Ctrl Pts',(6.76698651789578,-0.0135080204617305,
126.696544385656));
#214347=CARTESIAN_POINT('Ctrl Pts',(6.76735782124918,0.172500343506936,
126.705293967321));
#214348=CARTESIAN_POINT('Ctrl Pts',(6.76005538995215,0.358523882204961,
126.714043548986));
#214349=CARTESIAN_POINT('Ctrl Pts',(6.74510402742409,0.543930748558488,
126.722793130651));
#214350=CARTESIAN_POINT('Ctrl Pts',(6.73015291918094,0.729334461609357,
126.731542563507));
#214351=CARTESIAN_POINT('Ctrl Pts',(6.70755316306675,0.91412123762882,126.740291996364));
#214352=CARTESIAN_POINT('Ctrl Pts',(6.6773815187467,1.09766345165538,126.749041429221));
#214353=CARTESIAN_POINT('Ctrl Pts',(6.64721034747681,1.28120278799083,126.757790724898));
#214354=CARTESIAN_POINT('Ctrl Pts',(6.6094675720527,1.46349731859751,126.766540020576));
#214355=CARTESIAN_POINT('Ctrl Pts',(6.56428138111666,1.64392790277588,126.775289316253));
#214356=CARTESIAN_POINT('Ctrl Pts',(6.5190958386001,1.82435589778482,126.784038486379));
#214357=CARTESIAN_POINT('Ctrl Pts',(6.46646716393053,2.00291972191692,126.792787656505));
#214358=CARTESIAN_POINT('Ctrl Pts',(6.40657409873078,2.17901292274092,126.80153682663));
#214359=CARTESIAN_POINT('Ctrl Pts',(6.34668181342287,2.35510383058409,126.810285882829));
#214360=CARTESIAN_POINT('Ctrl Pts',(6.27952541914277,2.52872390822016,126.819034939028));
#214361=CARTESIAN_POINT('Ctrl Pts',(6.2053329917576,2.69928350889726,126.827783995228));
#214362=CARTESIAN_POINT('Ctrl Pts',(6.12831602991799,2.87633637965092,126.836866131386));
#214363=CARTESIAN_POINT('Ctrl Pts',(6.04371690605525,3.05009086600959,126.845948267544));
#214364=CARTESIAN_POINT('Ctrl Pts',(5.95184520316888,3.21991112882259,126.855030403702));
#214365=CARTESIAN_POINT('Ctrl Pts',(5.86333549509543,3.38351691182551,126.863780184046));
#214366=CARTESIAN_POINT('Ctrl Pts',(5.76807618099648,3.54347103711549,126.872529964389));
#214367=CARTESIAN_POINT('Ctrl Pts',(5.66639083309306,3.69923018027251,126.881279744733));
#214368=CARTESIAN_POINT('Ctrl Pts',(5.56470914082492,3.85498372381629,126.890029210518));
#214369=CARTESIAN_POINT('Ctrl Pts',(5.45660203372359,4.006542347016,126.898778676303));
#214370=CARTESIAN_POINT('Ctrl Pts',(5.34243669839508,4.15339127986294,126.907528142088));
#214371=CARTESIAN_POINT('Ctrl Pts',(5.22827486050887,4.3002357140092,126.916277339834));
#214372=CARTESIAN_POINT('Ctrl Pts',(5.10805534167411,4.44237052028125,126.92502653758));
#214373=CARTESIAN_POINT('Ctrl Pts',(4.98218644340254,4.57931296628392,126.933775735326));
#214374=CARTESIAN_POINT('Ctrl Pts',(4.85632073219887,4.71625194483052,126.942524711537));
#214375=CARTESIAN_POINT('Ctrl Pts',(4.72480612170616,4.84799861524219,126.951273687749));
#214376=CARTESIAN_POINT('Ctrl Pts',(4.58808925235604,4.97410554898215,126.960022663961));
#214377=CARTESIAN_POINT('Ctrl Pts',(4.45136349474351,5.10022068120942,126.968772208962));
#214378=CARTESIAN_POINT('Ctrl Pts',(4.30943501210393,5.22069514871576,126.977521753964));
#214379=CARTESIAN_POINT('Ctrl Pts',(4.16278587432105,5.33511975166005,126.986271298966));
#214380=CARTESIAN_POINT('Ctrl Pts',(4.01614535740752,5.44953762807619,126.995020329619));
#214381=CARTESIAN_POINT('Ctrl Pts',(3.86478496658208,5.55790617532587,127.003769360273));
#214382=CARTESIAN_POINT('Ctrl Pts',(3.70921874747458,5.65985735539184,127.012518390927));
#214383=CARTESIAN_POINT('Ctrl Pts',(3.55365041606172,5.76180991976879,127.021267540377));
#214384=CARTESIAN_POINT('Ctrl Pts',(3.39387638174803,5.8573447855265,127.030016689826));
#214385=CARTESIAN_POINT('Ctrl Pts',(3.23043927904829,5.94613749121074,127.038765839276));
#214386=CARTESIAN_POINT('Ctrl Pts',(3.18691767070625,5.96978206944044,127.041095647192));
#214387=CARTESIAN_POINT('Ctrl Pts',(3.1431364591973,5.99294880633374,127.043425455108));
#214388=CARTESIAN_POINT('Ctrl Pts',(3.09910619832142,6.01563211736936,127.045755263024));
#214389=CARTESIAN_POINT('Ctrl Pts',(3.09910619832122,6.01563211736946,125.045920265688));
#214390=CARTESIAN_POINT('Ctrl Pts',(2.93605669788026,6.09963122296482,125.054548849515));
#214391=CARTESIAN_POINT('Ctrl Pts',(2.76950882349665,6.17703933309001,125.063177433343));
#214392=CARTESIAN_POINT('Ctrl Pts',(2.60001145328852,6.24757788609062,125.071806017171));
#214393=CARTESIAN_POINT('Ctrl Pts',(2.42685102922923,6.31964086698003,125.080621075675));
#214394=CARTESIAN_POINT('Ctrl Pts',(2.25061244904093,6.38453382912852,125.089436134179));
#214395=CARTESIAN_POINT('Ctrl Pts',(2.07190576960204,6.4420102050439,125.098251192682));
#214396=CARTESIAN_POINT('Ctrl Pts',(1.89319909016315,6.49948658095929,125.107066251186));
#214397=CARTESIAN_POINT('Ctrl Pts',(1.71202462495059,6.54954623780946,125.11588130969));
#214398=CARTESIAN_POINT('Ctrl Pts',(1.52901294840764,6.59199578303884,125.124696368194));
#214399=CARTESIAN_POINT('Ctrl Pts',(1.35410028661987,6.63256676237746,125.133121324327));
#214400=CARTESIAN_POINT('Ctrl Pts',(1.17758614510552,6.66616847679302,125.14154628046));
#214401=CARTESIAN_POINT('Ctrl Pts',(1.00005148439541,6.69269646917881,125.149971236594));
#214402=CARTESIAN_POINT('Ctrl Pts',(0.822475616185957,6.71923061896634,
125.15839814824));
#214403=CARTESIAN_POINT('Ctrl Pts',(0.643879084457784,6.73868772405462,
125.166825059886));
#214404=CARTESIAN_POINT('Ctrl Pts',(0.464849602483791,6.75101502346652,
125.175251971533));
#214405=CARTESIAN_POINT('Ctrl Pts',(0.285754284396154,6.76334685610656,
125.183681982083));
#214406=CARTESIAN_POINT('Ctrl Pts',(0.106226029271025,6.76854363246676,
125.192111992633));
#214407=CARTESIAN_POINT('Ctrl Pts',(-0.0731454130554328,6.76660466914899,
125.200542003183));
#214408=CARTESIAN_POINT('Ctrl Pts',(-0.252682088603254,6.76466391969877,
125.208979779282));
#214409=CARTESIAN_POINT('Ctrl Pts',(-0.432061330928625,6.75557430129622,
125.217417555382));
#214410=CARTESIAN_POINT('Ctrl Pts',(-0.610695349609868,6.739387226593,125.225855331481));
#214411=CARTESIAN_POINT('Ctrl Pts',(-0.789423137983143,6.72319165486878,
125.234297536791));
#214412=CARTESIAN_POINT('Ctrl Pts',(-0.967404593380288,6.69989123416269,
125.242739742101));
#214413=CARTESIAN_POINT('Ctrl Pts',(-1.14405953544785,6.66958895130359,
125.251181947411));
#214414=CARTESIAN_POINT('Ctrl Pts',(-1.32090083875935,6.63925470120336,
125.259633058783));
#214415=CARTESIAN_POINT('Ctrl Pts',(-1.49641250818432,6.60190389730576,
125.268084170155));
#214416=CARTESIAN_POINT('Ctrl Pts',(-1.67002593990945,6.55769032205925,
125.276535281527));
#214417=CARTESIAN_POINT('Ctrl Pts',(-1.7187508184487,6.5452817136799,125.278907099024));
#214418=CARTESIAN_POINT('Ctrl Pts',(-1.76732627885295,6.53233285720752,
125.281278916522));
#214419=CARTESIAN_POINT('Ctrl Pts',(-1.81573999407381,6.51884784865553,
125.283650734019));
#214420=CARTESIAN_POINT('Ctrl Pts',(-1.98549236513071,6.47156554104953,
125.291967006423));
#214421=CARTESIAN_POINT('Ctrl Pts',(-2.15356128852685,6.41760263709694,
125.300283278827));
#214422=CARTESIAN_POINT('Ctrl Pts',(-2.31939289326421,6.35709883568562,
125.308599551231));
#214423=CARTESIAN_POINT('Ctrl Pts',(-2.48508428718448,6.29664619030965,
125.316908792217));
#214424=CARTESIAN_POINT('Ctrl Pts',(-2.64854180610319,6.22966378459738,
125.325218033203));
#214425=CARTESIAN_POINT('Ctrl Pts',(-2.80922592743371,6.15634133951605,
125.333527274189));
#214426=CARTESIAN_POINT('Ctrl Pts',(-2.96980365100676,6.0830674452415,125.341831013172));
#214427=CARTESIAN_POINT('Ctrl Pts',(-3.1276113207775,6.00346202071407,125.350134752154));
#214428=CARTESIAN_POINT('Ctrl Pts',(-3.2821284124593,5.91776326698926,125.358438491137));
#214429=CARTESIAN_POINT('Ctrl Pts',(-3.43657150746257,5.83210555353424,
125.366738253542));
#214430=CARTESIAN_POINT('Ctrl Pts',(-3.58772686117721,5.74036049461802,
125.375038015948));
#214431=CARTESIAN_POINT('Ctrl Pts',(-3.7350974286931,5.64281279134531,125.383337778353));
#214432=CARTESIAN_POINT('Ctrl Pts',(-3.88242442066472,5.54529393164925,
125.391635086628));
#214433=CARTESIAN_POINT('Ctrl Pts',(-4.0259685673482,5.44197603942589,125.399932394903));
#214434=CARTESIAN_POINT('Ctrl Pts',(-4.16526057425219,5.33318791611362,
125.408229703177));
#214435=CARTESIAN_POINT('Ctrl Pts',(-4.30456665459266,5.22438880133976,
125.416527849774));
#214436=CARTESIAN_POINT('Ctrl Pts',(-4.4396194578643,5.11011855933301,125.424825996372));
#214437=CARTESIAN_POINT('Ctrl Pts',(-4.56998118497756,4.99074753608627,
125.433124142969));
#214438=CARTESIAN_POINT('Ctrl Pts',(-4.70035602078258,4.87136450933218,
125.441423123997));
#214439=CARTESIAN_POINT('Ctrl Pts',(-4.82603858307134,4.74687991369302,
125.449722105025));
#214440=CARTESIAN_POINT('Ctrl Pts',(-4.94662657602122,4.61770229848142,
125.458021086053));
#214441=CARTESIAN_POINT('Ctrl Pts',(-5.06724673521217,4.48849022579018,
125.466322280793));
#214442=CARTESIAN_POINT('Ctrl Pts',(-5.18276937903411,4.3545828929151,125.474623475532));
#214443=CARTESIAN_POINT('Ctrl Pts',(-5.29283115991687,4.21642352149462,
125.482924670272));
#214444=CARTESIAN_POINT('Ctrl Pts',(-5.40294059240145,4.07820433353017,
125.49122945904));
#214445=CARTESIAN_POINT('Ctrl Pts',(-5.50758423316813,3.93572971005687,
125.499534247809));
#214446=CARTESIAN_POINT('Ctrl Pts',(-5.60644076926536,3.78947369706128,
125.507839036577));
#214447=CARTESIAN_POINT('Ctrl Pts',(-5.7054144988983,3.6430442988758,125.516153670598));
#214448=CARTESIAN_POINT('Ctrl Pts',(-5.79858722147323,3.49282484324007,
125.524468304619));
#214449=CARTESIAN_POINT('Ctrl Pts',(-5.88568188424686,3.33931695971622,
125.53278293864));
#214450=CARTESIAN_POINT('Ctrl Pts',(-5.97283161774779,3.18571201179689,
125.541102830078));
#214451=CARTESIAN_POINT('Ctrl Pts',(-6.0538954676157,3.02881479809379,125.549422721516));
#214452=CARTESIAN_POINT('Ctrl Pts',(-6.12864359904791,2.86914911356121,
125.557742612954));
#214453=CARTESIAN_POINT('Ctrl Pts',(-6.20350350317373,2.70924467705857,
125.566074945327));
#214454=CARTESIAN_POINT('Ctrl Pts',(-6.27202868001501,2.54656381702103,
125.5744072777));
#214455=CARTESIAN_POINT('Ctrl Pts',(-6.33403796063636,2.38164903233401,
125.582739610073));
#214456=CARTESIAN_POINT('Ctrl Pts',(-6.38072379659001,2.25748722127797,
125.589012895272));
#214457=CARTESIAN_POINT('Ctrl Pts',(-6.42371720929835,2.1320595120651,125.59528618047));
#214458=CARTESIAN_POINT('Ctrl Pts',(-6.46295988947719,2.00560177179044,
125.601559465669));
#214459=CARTESIAN_POINT('Ctrl Pts',(-6.52335173577858,1.81099181193342,
125.611213629803));
#214460=CARTESIAN_POINT('Ctrl Pts',(-6.57501402000094,1.61344508945547,
125.620867793937));
#214461=CARTESIAN_POINT('Ctrl Pts',(-6.61768735554798,1.41368421658462,
125.630521958071));
#214462=CARTESIAN_POINT('Ctrl Pts',(-6.66011135209951,1.21509054038926,
125.640119713219));
#214463=CARTESIAN_POINT('Ctrl Pts',(-6.69365104287442,1.01430857789511,
125.649717468367));
#214464=CARTESIAN_POINT('Ctrl Pts',(-6.71809703750268,0.812072161016336,
125.659315223515));
#214465=CARTESIAN_POINT('Ctrl Pts',(-6.74230300623966,0.611821426330077,
125.668818741968));
#214466=CARTESIAN_POINT('Ctrl Pts',(-6.75759289335629,0.410144744707065,
125.678322260422));
#214467=CARTESIAN_POINT('Ctrl Pts',(-6.76380941444879,0.20777681539077,
125.687825778875));
#214468=CARTESIAN_POINT('Ctrl Pts',(-6.76584898780119,0.141382085947639,
125.69094378052));
#214469=CARTESIAN_POINT('Ctrl Pts',(-6.76691225805108,0.0749131229981565,
125.694061782165));
#214470=CARTESIAN_POINT('Ctrl Pts',(-6.76699479095664,0.00839637813163948,
125.69717978381));
#214471=CARTESIAN_POINT('',(-6.767,8.80633884406398E-10,125.302820216149));
#214472=CARTESIAN_POINT('Ctrl Pts',(3.09910619832142,6.01563211736936,124.651395695404));
#214473=CARTESIAN_POINT('Ctrl Pts',(2.93375330764834,6.10081787314649,124.660145143307));
#214474=CARTESIAN_POINT('Ctrl Pts',(2.76488627843078,6.17918207037036,124.668894591209));
#214475=CARTESIAN_POINT('Ctrl Pts',(2.5930786664671,6.25045854553994,124.677644039111));
#214476=CARTESIAN_POINT('Ctrl Pts',(2.42127244185391,6.32173444515031,124.686393416362));
#214477=CARTESIAN_POINT('Ctrl Pts',(2.24652594672486,6.38592262741831,124.695142793612));
#214478=CARTESIAN_POINT('Ctrl Pts',(2.06943269687149,6.44280508110553,124.703892170862));
#214479=CARTESIAN_POINT('Ctrl Pts',(1.89234081822105,6.49968709436158,124.712641480368));
#214480=CARTESIAN_POINT('Ctrl Pts',(1.71290249405618,6.54926340459537,124.721390789873));
#214481=CARTESIAN_POINT('Ctrl Pts',(1.53172716625088,6.59136563150377,124.730140099378));
#214482=CARTESIAN_POINT('Ctrl Pts',(1.35055318107369,6.63346754640703,124.738889344045));
#214483=CARTESIAN_POINT('Ctrl Pts',(1.16764249714459,6.66809542395769,124.747638588713));
#214484=CARTESIAN_POINT('Ctrl Pts',(0.983616340614793,6.69513165624662,
124.75638783338));
#214485=CARTESIAN_POINT('Ctrl Pts',(0.79959148671428,6.72216769715956,124.765137016116));
#214486=CARTESIAN_POINT('Ctrl Pts',(0.61445145952715,6.74161215869367,124.773886198851));
#214487=CARTESIAN_POINT('Ctrl Pts',(0.428825047910721,6.75339900185709,
124.782635381587));
#214488=CARTESIAN_POINT('Ctrl Pts',(0.243199888597392,6.7651857655022,124.791384505298));
#214489=CARTESIAN_POINT('Ctrl Pts',(0.0570886373921694,6.76931499599834,
124.800133629008));
#214490=CARTESIAN_POINT('Ctrl Pts',(-0.12887662681099,6.76577266947847,
124.808882752719));
#214491=CARTESIAN_POINT('Ctrl Pts',(-0.314840698187942,6.76223036567994,
124.81763182031));
#214492=CARTESIAN_POINT('Ctrl Pts',(-0.500658497950979,6.75101660879225,
124.826380887902));
#214493=CARTESIAN_POINT('Ctrl Pts',(-0.685698951925887,6.73216948296222,
124.835129955493));
#214494=CARTESIAN_POINT('Ctrl Pts',(-0.87073828045956,6.71332247176297,
124.843878969872));
#214495=CARTESIAN_POINT('Ctrl Pts',(-1.05499998761225,6.68684221356191,
124.85262798425));
#214496=CARTESIAN_POINT('Ctrl Pts',(-1.23785829161398,6.65281863948526,
124.861376998629));
#214497=CARTESIAN_POINT('Ctrl Pts',(-1.43007412915576,6.61705395369202,
124.870573732327));
#214498=CARTESIAN_POINT('Ctrl Pts',(-1.62073882532187,6.57295372728624,
124.879770466026));
#214499=CARTESIAN_POINT('Ctrl Pts',(-1.80913696086181,6.52068343479759,
124.888967199724));
#214500=CARTESIAN_POINT('Ctrl Pts',(-1.9883835618082,6.47095219816825,124.897717197438));
#214501=CARTESIAN_POINT('Ctrl Pts',(-2.16557827567288,6.41382586852662,
124.906467195151));
#214502=CARTESIAN_POINT('Ctrl Pts',(-2.34011918616508,6.34949849945192,
124.915217192865));
#214503=CARTESIAN_POINT('Ctrl Pts',(-2.51465655685964,6.28517243497605,
124.923967013123));
#214504=CARTESIAN_POINT('Ctrl Pts',(-2.68653996290258,6.21364572244567,
124.932716833381));
#214505=CARTESIAN_POINT('Ctrl Pts',(-2.85518555374987,6.13516132254548,
124.94146665364));
#214506=CARTESIAN_POINT('Ctrl Pts',(-3.02382794853742,6.05667841002976,
124.950216308077));
#214507=CARTESIAN_POINT('Ctrl Pts',(-3.18923239104394,5.97123819494691,
124.958965962515));
#214508=CARTESIAN_POINT('Ctrl Pts',(-3.35083705962877,5.87913088813461,
124.967715616952));
#214509=CARTESIAN_POINT('Ctrl Pts',(-3.51243888037639,5.78702520445992,
124.976465117201));
#214510=CARTESIAN_POINT('Ctrl Pts',(-3.67024081218995,5.68825280608812,
124.98521461745));
#214511=CARTESIAN_POINT('Ctrl Pts',(-3.82370687539778,5.58314917685671,
124.993964117699));
#214512=CARTESIAN_POINT('Ctrl Pts',(-3.97717043813265,5.47804726011324,
125.00271347539));
#214513=CARTESIAN_POINT('Ctrl Pts',(-4.1262980371799,5.36661448087672,125.01146283308));
#214514=CARTESIAN_POINT('Ctrl Pts',(-4.27058317202522,5.24922931208144,
125.020212190771));
#214515=CARTESIAN_POINT('Ctrl Pts',(-4.41486614770552,5.13184589990476,
125.028961417531));
#214516=CARTESIAN_POINT('Ctrl Pts',(-4.55430658190237,5.00851045726832,
125.037710644291));
#214517=CARTESIAN_POINT('Ctrl Pts',(-4.6884308899778,4.87964187107025,125.046459871051));
#214518=CARTESIAN_POINT('Ctrl Pts',(-4.82255336913904,4.75077504211953,
125.055208978507));
#214519=CARTESIAN_POINT('Ctrl Pts',(-4.95135966061338,4.61637541912167,
125.063958085963));
#214520=CARTESIAN_POINT('Ctrl Pts',(-5.07441230865585,4.47689945405992,
125.072707193419));
#214521=CARTESIAN_POINT('Ctrl Pts',(-5.19746344222887,4.33742520559747,
125.081456193195));
#214522=CARTESIAN_POINT('Ctrl Pts',(-5.31476088451368,4.19287495495646,
125.090205192971));
#214523=CARTESIAN_POINT('Ctrl Pts',(-5.42590627625588,4.04373961591088,
125.098954192748));
#214524=CARTESIAN_POINT('Ctrl Pts',(-5.53706380669524,3.89458798911204,
125.107704148042));
#214525=CARTESIAN_POINT('Ctrl Pts',(-5.64206777068846,3.74085050159836,
125.116454103337));
#214526=CARTESIAN_POINT('Ctrl Pts',(-5.74056148161118,3.5830493822779,125.125204058632));
#214527=CARTESIAN_POINT('Ctrl Pts',(-5.83905138949125,3.42525435597985,
125.133953676073));
#214528=CARTESIAN_POINT('Ctrl Pts',(-5.93103139555028,3.26339625501955,
125.142703293514));
#214529=CARTESIAN_POINT('Ctrl Pts',(-6.01618907818357,3.09802485069838,
125.151452910955));
#214530=CARTESIAN_POINT('Ctrl Pts',(-6.10134392542622,2.93265895254553,
125.160202237071));
#214531=CARTESIAN_POINT('Ctrl Pts',(-6.17967677259601,2.76378023991022,
125.168951563187));
#214532=CARTESIAN_POINT('Ctrl Pts',(-6.25092157007128,2.59196229232171,
125.177700889303));
#214533=CARTESIAN_POINT('Ctrl Pts',(-6.32216437405813,2.42014915234164,
125.186449970605));
#214534=CARTESIAN_POINT('Ctrl Pts',(-6.38631941547135,2.24539720667934,
125.195199051908));
#214535=CARTESIAN_POINT('Ctrl Pts',(-6.44316881035905,2.06829994952773,
125.20394813321));
#214536=CARTESIAN_POINT('Ctrl Pts',(-6.50002334523081,1.89118668029575,
125.212698005552));
#214537=CARTESIAN_POINT('Ctrl Pts',(-6.54957082409748,1.7117279481286,125.221447877895));
#214538=CARTESIAN_POINT('Ctrl Pts',(-6.5916429429488,1.53053334255523,125.230197750237));
#214539=CARTESIAN_POINT('Ctrl Pts',(-6.63371214081076,1.34935131698802,
125.238947015092));
#214540=CARTESIAN_POINT('Ctrl Pts',(-6.66830695238778,1.1664339383498,125.247696279947));
#214541=CARTESIAN_POINT('Ctrl Pts',(-6.69530988153222,0.982402458393223,
125.256445544802));
#214542=CARTESIAN_POINT('Ctrl Pts',(-6.7223141968986,0.798361530999515,
125.265195258809));
#214543=CARTESIAN_POINT('Ctrl Pts',(-6.74172580828799,0.613206671415098,
125.273944972816));
#214544=CARTESIAN_POINT('Ctrl Pts',(-6.75347878027846,0.427566795166124,
125.282694686823));
#214545=CARTESIAN_POINT('Ctrl Pts',(-6.76248992366252,0.285234494532973,
125.289403196598));
#214546=CARTESIAN_POINT('Ctrl Pts',(-6.76699999998144,0.142617266695871,
125.296111706374));
#214547=CARTESIAN_POINT('Ctrl Pts',(-6.767,8.80634713124887E-10,125.302820216149));
#214548=CARTESIAN_POINT('Ctrl Pts',(-6.767,6.68686382847748E-12,125.30282021619));
#214549=CARTESIAN_POINT('Ctrl Pts',(-6.76700000000019,-0.186007249520308,
125.311569728001));
#214550=CARTESIAN_POINT('Ctrl Pts',(-6.75932637294556,-0.372014355743486,
125.320319239812));
#214551=CARTESIAN_POINT('Ctrl Pts',(-6.74400518264232,-0.557389537481198,
125.329068751624));
#214552=CARTESIAN_POINT('Ctrl Pts',(-6.72868405705154,-0.742763936245582,
125.337818226479));
#214553=CARTESIAN_POINT('Ctrl Pts',(-6.7057154564581,-0.927506130236142,
125.346567701335));
#214554=CARTESIAN_POINT('Ctrl Pts',(-6.67517739404902,-1.11098863989558,
125.355317176191));
#214555=CARTESIAN_POINT('Ctrl Pts',(-6.64463945808789,-1.29447038981501,
125.364066614818));
#214556=CARTESIAN_POINT('Ctrl Pts',(-6.60653217008452,-1.47669218313251,
125.372816053445));
#214557=CARTESIAN_POINT('Ctrl Pts',(-6.56098496092783,-1.65703510598866,
125.381565492072));
#214558=CARTESIAN_POINT('Ctrl Pts',(-6.51543793658414,-1.83737729708282,
125.390314895197));
#214559=CARTESIAN_POINT('Ctrl Pts',(-6.4624511216755,-2.0158403551051,125.399064298322));
#214560=CARTESIAN_POINT('Ctrl Pts',(-6.40220448374395,-2.19181813760377,
125.407813701447));
#214561=CARTESIAN_POINT('Ctrl Pts',(-6.34195808526654,-2.36779522066742,
125.416563069797));
#214562=CARTESIAN_POINT('Ctrl Pts',(-6.27445201433262,-2.54128677683776,
125.425312438147));
#214563=CARTESIAN_POINT('Ctrl Pts',(-6.19991555072066,-2.71170355384435,
125.434061806497));
#214564=CARTESIAN_POINT('Ctrl Pts',(-6.12537937716873,-2.88211966767093,
125.442811140799));
#214565=CARTESIAN_POINT('Ctrl Pts',(-6.04381298052717,-3.04946076371394,
125.451560475101));
#214566=CARTESIAN_POINT('Ctrl Pts',(-5.95549339336046,-3.21315848374149,
125.460309809403));
#214567=CARTESIAN_POINT('Ctrl Pts',(-5.8671741425563,-3.37685558033108,
125.469059110383));
#214568=CARTESIAN_POINT('Ctrl Pts',(-5.77210188876825,-3.53690907646386,
125.477808411363));
#214569=CARTESIAN_POINT('Ctrl Pts',(-5.67059953347228,-3.6927753696893,
125.486557712343));
#214570=CARTESIAN_POINT('Ctrl Pts',(-5.56909755631612,-3.84864108224595,
125.495306980729));
#214571=CARTESIAN_POINT('Ctrl Pts',(-5.46116568197072,-4.00031938297215,
125.504056249114));
#214572=CARTESIAN_POINT('Ctrl Pts',(-5.34717048533817,-4.14729511859578,
125.512805517499));
#214573=CARTESIAN_POINT('Ctrl Pts',(-5.23317570392063,-4.2942703188764,
125.521554754016));
#214574=CARTESIAN_POINT('Ctrl Pts',(-5.11311782003753,-4.43654276189272,
125.530303990533));
#214575=CARTESIAN_POINT('Ctrl Pts',(-4.98740458985004,-4.57362924351579,
125.53905322705));
#214576=CARTESIAN_POINT('Ctrl Pts',(-4.86169180712014,-4.71071523719986,
125.547802432426));
#214577=CARTESIAN_POINT('Ctrl Pts',(-4.73032391204464,-4.84261509522952,
125.556551637801));
#214578=CARTESIAN_POINT('Ctrl Pts',(-4.59374707013913,-4.96888084538039,
125.565300843177));
#214579=CARTESIAN_POINT('Ctrl Pts',(-4.45717070301761,-5.09514615659187,
125.574050018137));
#214580=CARTESIAN_POINT('Ctrl Pts',(-4.31538563571359,-5.21577720459265,
125.582799193098));
#214581=CARTESIAN_POINT('Ctrl Pts',(-4.16887341029828,-5.33036429232637,
125.591548368058));
#214582=CARTESIAN_POINT('Ctrl Pts',(-4.02236168204043,-5.44495099123366,
125.60029751333));
#214583=CARTESIAN_POINT('Ctrl Pts',(-3.87112305348521,-5.55349359438353,
125.609046658602));
#214584=CARTESIAN_POINT('Ctrl Pts',(-3.71567117018136,-5.65562346298648,
125.617795803874));
#214585=CARTESIAN_POINT('Ctrl Pts',(-3.56021980146199,-5.75775299351409,
125.626544920184));
#214586=CARTESIAN_POINT('Ctrl Pts',(-3.40055544538734,-5.85346967463649,
125.635294036494));
#214587=CARTESIAN_POINT('Ctrl Pts',(-3.23722035987243,-5.94244842986689,
125.644043152805));
#214588=CARTESIAN_POINT('Ctrl Pts',(-3.07388580147592,-6.03142689794318,
125.652792240879));
#214589=CARTESIAN_POINT('Ctrl Pts',(-2.90688078897012,-6.11366734656575,
125.661541328954));
#214590=CARTESIAN_POINT('Ctrl Pts',(-2.73677250721827,-6.18889046952152,
125.670290417029));
#214591=CARTESIAN_POINT('Ctrl Pts',(-2.56666476031899,-6.26411335596158,
125.679039477595));
#214592=CARTESIAN_POINT('Ctrl Pts',(-2.3934540257554,-6.33231884500416,
125.687788538161));
#214593=CARTESIAN_POINT('Ctrl Pts',(-2.21772856065922,-6.39327529762612,
125.696537598727));
#214594=CARTESIAN_POINT('Ctrl Pts',(-2.04200363348842,-6.45423156365007,
125.705286632511));
#214595=CARTESIAN_POINT('Ctrl Pts',(-1.86376426189605,-6.50793874375565,
125.714035666295));
#214596=CARTESIAN_POINT('Ctrl Pts',(-1.68361577753478,-6.55421443909459,
125.722784700078));
#214597=CARTESIAN_POINT('Ctrl Pts',(-1.50346782968151,-6.60048999661787,
125.731533707806));
#214598=CARTESIAN_POINT('Ctrl Pts',(-1.32141105795366,-6.63933404237636,
125.740282715534));
#214599=CARTESIAN_POINT('Ctrl Pts',(-1.13806375487428,-6.67061465607492,
125.749031723262));
#214600=CARTESIAN_POINT('Ctrl Pts',(-0.954716982607099,-6.70189517921238,
125.75778070566));
#214601=CARTESIAN_POINT('Ctrl Pts',(-0.77007996890624,-6.72561226592181,
125.766529688059));
#214602=CARTESIAN_POINT('Ctrl Pts',(-0.584779765562359,-6.74168536983067,
125.775278670457));
#214603=CARTESIAN_POINT('Ctrl Pts',(-0.391489830655416,-6.75845151013829,
125.784404889467));
#214604=CARTESIAN_POINT('Ctrl Pts',(-0.197478578242453,-6.76689983031613,
125.793531108477));
#214605=CARTESIAN_POINT('Ctrl Pts',(-0.0034628764554554,-6.76699911397117,
125.802657327487));
#214606=CARTESIAN_POINT('Ctrl Pts',(0.184489834650666,-6.767095295012,125.811498352152));
#214607=CARTESIAN_POINT('Ctrl Pts',(0.372446404246149,-6.75935639738186,
125.820339376818));
#214608=CARTESIAN_POINT('Ctrl Pts',(0.559755019485118,-6.74380925873213,
125.829180401484));
#214609=CARTESIAN_POINT('Ctrl Pts',(0.74513470551855,-6.72842222659841,
125.837930380094));
#214610=CARTESIAN_POINT('Ctrl Pts',(0.929879431225341,-6.70538706057568,
125.846680358703));
#214611=CARTESIAN_POINT('Ctrl Pts',(1.11336163626503,-6.67478200894181,
125.855430337313));
#214612=CARTESIAN_POINT('Ctrl Pts',(1.29684196300417,-6.64417727061072,
125.86418022635));
#214613=CARTESIAN_POINT('Ctrl Pts',(1.4790595121723,-6.60600284890654,125.872930115386));
#214614=CARTESIAN_POINT('Ctrl Pts',(1.65939532066825,-6.56038841607296,
125.881680004423));
#214615=CARTESIAN_POINT('Ctrl Pts',(1.83972934300547,-6.51477443503329,
125.890429806795));
#214616=CARTESIAN_POINT('Ctrl Pts',(2.01818138406014,-6.46172066062219,
125.899179609167));
#214617=CARTESIAN_POINT('Ctrl Pts',(2.19414528353954,-6.40140730423563,
125.907929411539));
#214618=CARTESIAN_POINT('Ctrl Pts',(2.37010749863758,-6.34109452518732,
125.916679130156));
#214619=CARTESIAN_POINT('Ctrl Pts',(2.54358134866223,-6.273522396166,125.925428848772));
#214620=CARTESIAN_POINT('Ctrl Pts',(2.71397759435323,-6.1989204396692,125.934178567388));
#214621=CARTESIAN_POINT('Ctrl Pts',(2.88437226557891,-6.12431917249625,
125.942928205157));
#214622=CARTESIAN_POINT('Ctrl Pts',(3.05168912680723,-6.04268832278916,
125.951677842926));
#214623=CARTESIAN_POINT('Ctrl Pts',(3.21535986273622,-5.9543051612346,125.960427480694));
#214624=CARTESIAN_POINT('Ctrl Pts',(3.3790291407262,-5.86592278697568,125.969177040523));
#214625=CARTESIAN_POINT('Ctrl Pts',(3.53905210621362,-5.77078835742071,
125.977926600353));
#214626=CARTESIAN_POINT('Ctrl Pts',(3.69488522831498,-5.66922500431759,
125.986676160182));
#214627=CARTESIAN_POINT('Ctrl Pts',(3.85071701406762,-5.56766252217217,
125.995425644979));
#214628=CARTESIAN_POINT('Ctrl Pts',(4.00235878822247,-5.45967138329486,
126.004175129776));
#214629=CARTESIAN_POINT('Ctrl Pts',(4.14929549611188,-5.34561838199714,
126.012924614573));
#214630=CARTESIAN_POINT('Ctrl Pts',(4.29623099275953,-5.23156632087128,
126.021674027246));
#214631=CARTESIAN_POINT('Ctrl Pts',(4.43846127435892,-5.11145267305082,
126.030423439918));
#214632=CARTESIAN_POINT('Ctrl Pts',(4.57550326054307,-4.98568540050009,
126.039172852591));
#214633=CARTESIAN_POINT('Ctrl Pts',(4.71254416257657,-4.8599191229048,126.047922196046));
#214634=CARTESIAN_POINT('Ctrl Pts',(4.84439664018649,-4.72849950385534,
126.056671539501));
#214635=CARTESIAN_POINT('Ctrl Pts',(4.97061286794644,-4.59187289861178,
126.065420882956));
#214636=CARTESIAN_POINT('Ctrl Pts',(5.09682813912582,-4.45524732884802,
126.074170160101));
#214637=CARTESIAN_POINT('Ctrl Pts',(5.21740705147736,-4.31341506235912,
126.082919437246));
#214638=CARTESIAN_POINT('Ctrl Pts',(5.33194007545593,-4.16685781275856,
126.091668714391));
#214639=CARTESIAN_POINT('Ctrl Pts',(5.4464722694439,-4.02030162521971,126.100417928132));
#214640=CARTESIAN_POINT('Ctrl Pts',(5.55495848628026,-3.8690207488806,126.109167141873));
#214641=CARTESIAN_POINT('Ctrl Pts',(5.65703027291707,-3.71352898080785,
126.117916355614));
#214642=CARTESIAN_POINT('Ctrl Pts',(5.7591013537692,-3.55803828789713,126.126665508858));
#214643=CARTESIAN_POINT('Ctrl Pts',(5.85475793592679,-3.39833700106839,
126.135414662102));
#214644=CARTESIAN_POINT('Ctrl Pts',(5.94367514427329,-3.23496750823682,
126.144163815346));
#214645=CARTESIAN_POINT('Ctrl Pts',(6.03259176732568,-3.07159909077866,
126.152912910999));
#214646=CARTESIAN_POINT('Ctrl Pts',(6.1147689683585,-2.9045627673159,126.161662006652));
#214647=CARTESIAN_POINT('Ctrl Pts',(6.18992765547811,-2.73442583003219,
126.170411102305));
#214648=CARTESIAN_POINT('Ctrl Pts',(6.26508587282978,-2.56428995616356,
126.179160143273));
#214649=CARTESIAN_POINT('Ctrl Pts',(6.33322554827083,-2.39105376935404,
126.187909184241));
#214650=CARTESIAN_POINT('Ctrl Pts',(6.39411526732955,-2.21530561054298,
126.196658225209));
#214651=CARTESIAN_POINT('Ctrl Pts',(6.45500462602776,-2.03955849185324,
126.205407214398));
#214652=CARTESIAN_POINT('Ctrl Pts',(6.50864402040673,-1.86129970164778,
126.214156203587));
#214653=CARTESIAN_POINT('Ctrl Pts',(6.55485128368539,-1.681134631363,126.222905192776));
#214654=CARTESIAN_POINT('Ctrl Pts',(6.6019980955427,-1.49730620117118,126.231832078247));
#214655=CARTESIAN_POINT('Ctrl Pts',(6.64140720707823,-1.31149343245955,
126.240758963719));
#214656=CARTESIAN_POINT('Ctrl Pts',(6.67293928722839,-1.12435326697789,
126.24968584919));
#214657=CARTESIAN_POINT('Ctrl Pts',(6.70384625876218,-0.940923067009357,
126.258435763368));
#214658=CARTESIAN_POINT('Ctrl Pts',(6.72718554579763,-0.756217899524563,
126.267185677545));
#214659=CARTESIAN_POINT('Ctrl Pts',(6.74287786815302,-0.570865181257524,
126.275935591723));
#214660=CARTESIAN_POINT('Ctrl Pts',(6.75856988190828,-0.38551610807702,
126.284685333827));
#214661=CARTESIAN_POINT('Ctrl Pts',(6.76661520773394,-0.199519795229466,
126.293435075931));
#214662=CARTESIAN_POINT('Ctrl Pts',(6.76698651789578,-0.0135080204588065,
126.302184818036));
#214663=CARTESIAN_POINT('Ctrl Pts',(6.76735782124911,0.172500343509762,
126.310934399701));
#214664=CARTESIAN_POINT('Ctrl Pts',(6.76005538995201,0.358523882207686,
126.319683981366));
#214665=CARTESIAN_POINT('Ctrl Pts',(6.74510402742387,0.543930748561109,
126.328433563031));
#214666=CARTESIAN_POINT('Ctrl Pts',(6.73015291918067,0.729334461611875,
126.337182995888));
#214667=CARTESIAN_POINT('Ctrl Pts',(6.70755316306642,0.914121237631232,
126.345932428744));
#214668=CARTESIAN_POINT('Ctrl Pts',(6.67738151874632,1.09766345165769,126.354681861601));
#214669=CARTESIAN_POINT('Ctrl Pts',(6.64721034747636,1.28120278799316,126.363431157278));
#214670=CARTESIAN_POINT('Ctrl Pts',(6.60946757205218,1.46349731859985,126.372180452956));
#214671=CARTESIAN_POINT('Ctrl Pts',(6.56428138111607,1.64392790277824,126.380929748634));
#214672=CARTESIAN_POINT('Ctrl Pts',(6.51909583859944,1.82435589778719,126.389678918759));
#214673=CARTESIAN_POINT('Ctrl Pts',(6.46646716392979,2.0029197219193,126.398428088885));
#214674=CARTESIAN_POINT('Ctrl Pts',(6.40657409872997,2.17901292274331,126.40717725901));
#214675=CARTESIAN_POINT('Ctrl Pts',(6.34668181342194,2.3551038305866,126.415926315209));
#214676=CARTESIAN_POINT('Ctrl Pts',(6.27952541914172,2.5287239082228,126.424675371409));
#214677=CARTESIAN_POINT('Ctrl Pts',(6.2053329917564,2.69928350890001,126.433424427608));
#214678=CARTESIAN_POINT('Ctrl Pts',(6.12831602991675,2.87633637965354,126.442506563766));
#214679=CARTESIAN_POINT('Ctrl Pts',(6.04371690605398,3.05009086601209,126.451588699924));
#214680=CARTESIAN_POINT('Ctrl Pts',(5.9518452031676,3.21991112882497,126.460670836082));
#214681=CARTESIAN_POINT('Ctrl Pts',(5.86333549509407,3.38351691182788,126.469420616426));
#214682=CARTESIAN_POINT('Ctrl Pts',(5.76807618099504,3.54347103711784,126.478170396769));
#214683=CARTESIAN_POINT('Ctrl Pts',(5.66639083309153,3.69923018027485,126.486920177113));
#214684=CARTESIAN_POINT('Ctrl Pts',(5.56470914082346,3.8549837238184,126.495669642898));
#214685=CARTESIAN_POINT('Ctrl Pts',(5.4566020337222,4.00654234701789,126.504419108683));
#214686=CARTESIAN_POINT('Ctrl Pts',(5.34243669839378,4.15339127986461,126.513168574468));
#214687=CARTESIAN_POINT('Ctrl Pts',(5.22827486050759,4.30023571401076,126.521917772214));
#214688=CARTESIAN_POINT('Ctrl Pts',(5.10805534167284,4.4423705202827,126.53066696996));
#214689=CARTESIAN_POINT('Ctrl Pts',(4.9821864434013,4.57931296628526,126.539416167706));
#214690=CARTESIAN_POINT('Ctrl Pts',(4.85632073219784,4.71625194483157,126.548165143917));
#214691=CARTESIAN_POINT('Ctrl Pts',(4.72480612170535,4.84799861524297,126.556914120129));
#214692=CARTESIAN_POINT('Ctrl Pts',(4.58808925235548,4.97410554898267,126.565663096341));
#214693=CARTESIAN_POINT('Ctrl Pts',(4.45136349474291,5.10022068120994,126.574412641342));
#214694=CARTESIAN_POINT('Ctrl Pts',(4.3094350121033,5.22069514871628,126.583162186344));
#214695=CARTESIAN_POINT('Ctrl Pts',(4.16278587432038,5.33511975166057,126.591911731346));
#214696=CARTESIAN_POINT('Ctrl Pts',(4.01614535740682,5.44953762807671,126.600660761999));
#214697=CARTESIAN_POINT('Ctrl Pts',(3.86478496658133,5.55790617532639,126.609409792653));
#214698=CARTESIAN_POINT('Ctrl Pts',(3.70921874747379,5.65985735539236,126.618158823307));
#214699=CARTESIAN_POINT('Ctrl Pts',(3.5536504160609,5.7618099197693,126.626907972757));
#214700=CARTESIAN_POINT('Ctrl Pts',(3.39387638174717,5.85734478552701,126.635657122206));
#214701=CARTESIAN_POINT('Ctrl Pts',(3.23043927904738,5.94613749121124,126.644406271656));
#214702=CARTESIAN_POINT('Ctrl Pts',(3.18691767070567,5.96978206944075,126.646736079572));
#214703=CARTESIAN_POINT('Ctrl Pts',(3.14313645919705,5.99294880633387,126.649065887488));
#214704=CARTESIAN_POINT('Ctrl Pts',(3.0991061983215,6.01563211736932,126.651395695404));
#214705=CARTESIAN_POINT('Origin',(0.,0.,4.30282021618968));
#214706=CARTESIAN_POINT('',(3.09910619832118,6.01563211736948,129.045766611327));
#214707=CARTESIAN_POINT('',(3.09910619832144,6.01563211736935,128.651395695404));
#214708=CARTESIAN_POINT('',(3.09910619832133,6.0156321173694,4.30282021618968));
#214709=CARTESIAN_POINT('',(-6.76699890687685,-0.00271977263060589,127.69717978381));
#214710=CARTESIAN_POINT('Ctrl Pts',(-6.7669978137537,-0.00543954526750962,
127.69717978381));
#214711=CARTESIAN_POINT('Ctrl Pts',(-6.76683644173397,-0.206192374952252,
127.706596882396));
#214712=CARTESIAN_POINT('Ctrl Pts',(-6.7577377857915,-0.406590498140303,
127.716013980982));
#214713=CARTESIAN_POINT('Ctrl Pts',(-6.73981970767303,-0.60590371187369,
127.725431079567));
#214714=CARTESIAN_POINT('Ctrl Pts',(-6.72175068807275,-0.806895935578124,
127.734927507577));
#214715=CARTESIAN_POINT('Ctrl Pts',(-6.69471310070588,-1.00678476574515,
127.744423935587));
#214716=CARTESIAN_POINT('Ctrl Pts',(-6.65887750139783,-1.20483999824782,
127.753920363597));
#214717=CARTESIAN_POINT('Ctrl Pts',(-6.62290041652562,-1.40367718938511,
127.763454285258));
#214718=CARTESIAN_POINT('Ctrl Pts',(-6.57805580290485,-1.60066616659163,
127.772988206919));
#214719=CARTESIAN_POINT('Ctrl Pts',(-6.52456483723941,-1.79508848936734,
127.782522128581));
#214720=CARTESIAN_POINT('Ctrl Pts',(-6.47083000609436,-1.99039718412006,
127.792099515421));
#214721=CARTESIAN_POINT('Ctrl Pts',(-6.40836987881955,-2.18311565971218,
127.801676902261));
#214722=CARTESIAN_POINT('Ctrl Pts',(-6.33745636754904,-2.3725378372983,
127.811254289101));
#214723=CARTESIAN_POINT('Ctrl Pts',(-6.29879055934802,-2.47582085708316,
127.816476388472));
#214724=CARTESIAN_POINT('Ctrl Pts',(-6.25761237472158,-2.57812428063289,
127.821698487844));
#214725=CARTESIAN_POINT('Ctrl Pts',(-6.21397171263012,-2.67933658852946,
127.826920587215));
#214726=CARTESIAN_POINT('Ctrl Pts',(-6.14653266226067,-2.83574260079252,
127.834990433218));
#214727=CARTESIAN_POINT('Ctrl Pts',(-6.07306002673467,-2.9898895791241,
127.84306027922));
#214728=CARTESIAN_POINT('Ctrl Pts',(-5.99372495262846,-3.14126569908357,
127.851130125223));
#214729=CARTESIAN_POINT('Ctrl Pts',(-5.91448969213646,-3.29245136862991,
127.859189818333));
#214730=CARTESIAN_POINT('Ctrl Pts',(-5.82940683964584,-3.44087278991846,
127.867249511443));
#214731=CARTESIAN_POINT('Ctrl Pts',(-5.73869643029757,-3.58603573335374,
127.875309204553));
#214732=CARTESIAN_POINT('Ctrl Pts',(-5.64808023811702,-3.73104790201592,
127.883360526392));
#214733=CARTESIAN_POINT('Ctrl Pts',(-5.55184831694054,-3.87280801420068,
127.891411848231));
#214734=CARTESIAN_POINT('Ctrl Pts',(-5.45026762102806,-4.01084428258854,
127.899463170069));
#214735=CARTESIAN_POINT('Ctrl Pts',(-5.34877017301097,-4.14876742683674,
127.90750789365));
#214736=CARTESIAN_POINT('Ctrl Pts',(-5.24193289474739,-4.28297250235147,
127.915552617231));
#214737=CARTESIAN_POINT('Ctrl Pts',(-5.13006720173639,-4.41301478647745,
127.923597340812));
#214738=CARTESIAN_POINT('Ctrl Pts',(-5.01826869798149,-4.5429789640446,
127.931637232537));
#214739=CARTESIAN_POINT('Ctrl Pts',(-4.90144803443804,-4.66878504536288,
127.939677124261));
#214740=CARTESIAN_POINT('Ctrl Pts',(-4.77995816745076,-4.7900197199407,
127.947717015986));
#214741=CARTESIAN_POINT('Ctrl Pts',(-4.65585229078337,-4.91386490920691,
127.955930028606));
#214742=CARTESIAN_POINT('Ctrl Pts',(-4.52687408429014,-5.0329392675561,
127.964143041226));
#214743=CARTESIAN_POINT('Ctrl Pts',(-4.39344141097314,-5.14683995946507,
127.972356053845));
#214744=CARTESIAN_POINT('Ctrl Pts',(-4.2628669198969,-5.25830085213497,
127.980393140388));
#214745=CARTESIAN_POINT('Ctrl Pts',(-4.1280271659833,-5.36480723477413,
127.988430226931));
#214746=CARTESIAN_POINT('Ctrl Pts',(-3.98934870189478,-5.46602103313648,
127.996467313473));
#214747=CARTESIAN_POINT('Ctrl Pts',(-3.85065696563169,-5.56724451813051,
128.004505169202));
#214748=CARTESIAN_POINT('Ctrl Pts',(-3.70812608940294,-5.66317418989895,
128.012543024932));
#214749=CARTESIAN_POINT('Ctrl Pts',(-3.56221294243062,-5.75351440015403,
128.020580880661));
#214750=CARTESIAN_POINT('Ctrl Pts',(-3.41625692062508,-5.8438811557995,
128.028621098218));
#214751=CARTESIAN_POINT('Ctrl Pts',(-3.26691696736246,-5.92865498423049,
128.036661315775));
#214752=CARTESIAN_POINT('Ctrl Pts',(-3.1146758188146,-6.00758550032304,
128.044701533332));
#214753=CARTESIAN_POINT('Ctrl Pts',(-2.95668290213072,-6.08949806188589,
128.053045515459));
#214754=CARTESIAN_POINT('Ctrl Pts',(-2.79556568532968,-6.16511695391536,
128.061389497587));
#214755=CARTESIAN_POINT('Ctrl Pts',(-2.6318868760193,-6.23421690927075,
128.069733479715));
#214756=CARTESIAN_POINT('Ctrl Pts',(-2.47389225499252,-6.30091718223426,
128.07778769455));
#214757=CARTESIAN_POINT('Ctrl Pts',(-2.3135113428348,-6.36154363543611,
128.085841909385));
#214758=CARTESIAN_POINT('Ctrl Pts',(-2.15126556895633,-6.41594462661758,
128.09389612422));
#214759=CARTESIAN_POINT('Ctrl Pts',(-1.98889838094546,-6.47038632794507,
128.101956366303));
#214760=CARTESIAN_POINT('Ctrl Pts',(-1.82466390852764,-6.51859318662524,
128.110016608386));
#214761=CARTESIAN_POINT('Ctrl Pts',(-1.65909428435162,-6.56046455334009,
128.118076850469));
#214762=CARTESIAN_POINT('Ctrl Pts',(-1.49329318248335,-6.60239445909788,
128.126148361323));
#214763=CARTESIAN_POINT('Ctrl Pts',(-1.32615356655731,-6.63797112369992,
128.134219872178));
#214764=CARTESIAN_POINT('Ctrl Pts',(-1.15821377460314,-6.66714555505724,
128.142291383032));
#214765=CARTESIAN_POINT('Ctrl Pts',(-1.14061193097295,-6.67020334006922,
128.143137361643));
#214766=CARTESIAN_POINT('Ctrl Pts',(-1.12300129779593,-6.67319084227332,
128.143983340254));
#214767=CARTESIAN_POINT('Ctrl Pts',(-1.10538249481115,-6.67610803838322,
128.144829318865));
#214768=CARTESIAN_POINT('Ctrl Pts',(-0.933995738766564,-6.70448503870811,
128.153058568601));
#214769=CARTESIAN_POINT('Ctrl Pts',(-0.761263712658549,-6.72629982420718,
128.161287818337));
#214770=CARTESIAN_POINT('Ctrl Pts',(-0.587730201326801,-6.74142879591918,
128.169517068073));
#214771=CARTESIAN_POINT('Ctrl Pts',(-0.414403223103981,-6.75653976169367,
128.177736523663));
#214772=CARTESIAN_POINT('Ctrl Pts',(-0.240277012831369,-6.76498072728823,
128.185955979253));
#214773=CARTESIAN_POINT('Ctrl Pts',(-0.065905572641955,-6.76667905663441,
128.194175434843));
#214774=CARTESIAN_POINT('Ctrl Pts',(0.108293355242183,-6.7683757057587,
128.202386758613));
#214775=CARTESIAN_POINT('Ctrl Pts',(0.282736673728126,-6.76334299978061,
128.210598082382));
#214776=CARTESIAN_POINT('Ctrl Pts',(0.456865136902315,-6.75156006021447,
128.218809406152));
#214777=CARTESIAN_POINT('Ctrl Pts',(0.630856284795527,-6.73978641251037,
128.227014254586));
#214778=CARTESIAN_POINT('Ctrl Pts',(0.804532715698328,-6.72127315775058,
128.23521910302));
#214779=CARTESIAN_POINT('Ctrl Pts',(0.977334968178098,-6.69605147530814,
128.243423951454));
#214780=CARTESIAN_POINT('Ctrl Pts',(1.15003563266157,-6.67084462033552,
128.251623976374));
#214781=CARTESIAN_POINT('Ctrl Pts',(1.32186278856019,-6.63893724576152,
128.259824001294));
#214782=CARTESIAN_POINT('Ctrl Pts',(1.49226179257834,-6.60041239184423,
128.268024026214));
#214783=CARTESIAN_POINT('Ctrl Pts',(1.66261147926394,-6.56189868789253,
128.276221677861));
#214784=CARTESIAN_POINT('Ctrl Pts',(1.83153348713577,-6.51677139465191,
128.284419329508));
#214785=CARTESIAN_POINT('Ctrl Pts',(1.99848282142742,-6.46516476297855,
128.292616981155));
#214786=CARTESIAN_POINT('Ctrl Pts',(2.16540980017873,-6.41356504174986,
128.300813535086));
#214787=CARTESIAN_POINT('Ctrl Pts',(2.33036428856015,-6.35548781518088,
128.309010089017));
#214788=CARTESIAN_POINT('Ctrl Pts',(2.49281591947777,-6.29111737226371,
128.317206642948));
#214789=CARTESIAN_POINT('Ctrl Pts',(2.65527533505303,-6.22674384472461,
128.325403589657));
#214790=CARTESIAN_POINT('Ctrl Pts',(2.81523132065585,-6.15607663214782,
128.333600536365));
#214791=CARTESIAN_POINT('Ctrl Pts',(2.97217293169374,-6.07934840785648,
128.341797483074));
#214792=CARTESIAN_POINT('Ctrl Pts',(3.12915059934962,-6.00260255560621,
128.349996312994));
#214793=CARTESIAN_POINT('Ctrl Pts',(3.28311219088485,-5.91979307575749,
128.358195142914));
#214794=CARTESIAN_POINT('Ctrl Pts',(3.43357078995366,-5.83119890163052,
128.366393972833));
#214795=CARTESIAN_POINT('Ctrl Pts',(3.58417189255028,-5.74252081749486,
128.374600568093));
#214796=CARTESIAN_POINT('Ctrl Pts',(3.73126306451462,-5.64804727511739,
128.382807163353));
#214797=CARTESIAN_POINT('Ctrl Pts',(3.87438505941322,-5.54810142403648,
128.391013758613));
#214798=CARTESIAN_POINT('Ctrl Pts',(4.01757632617791,-5.44810719859063,
128.399224325912));
#214799=CARTESIAN_POINT('Ctrl Pts',(4.15679429987137,-5.34263560021629,
128.407434893211));
#214800=CARTESIAN_POINT('Ctrl Pts',(4.29161243240706,-5.23205043267065,
128.41564546051));
#214801=CARTESIAN_POINT('Ctrl Pts',(4.4266164984481,-5.12131275234759,128.423867351356));
#214802=CARTESIAN_POINT('Ctrl Pts',(4.55720832794847,-5.00544764684747,
128.432089242203));
#214803=CARTESIAN_POINT('Ctrl Pts',(4.68299700033132,-4.88485701887864,
128.44031113305));
#214804=CARTESIAN_POINT('Ctrl Pts',(4.79736858979085,-4.77521167853558,
128.447786772205));
#214805=CARTESIAN_POINT('Ctrl Pts',(4.90776969492203,-4.66166029872621,
128.455262411359));
#214806=CARTESIAN_POINT('Ctrl Pts',(5.01393570377541,-4.54452833178606,
128.462738050514));
#214807=CARTESIAN_POINT('Ctrl Pts',(5.14084036461515,-4.40451560362031,
128.471673993965));
#214808=CARTESIAN_POINT('Ctrl Pts',(5.26195793272095,-4.25909512080603,
128.480609937416));
#214809=CARTESIAN_POINT('Ctrl Pts',(5.37684636472458,-4.10874824857256,
128.489545880867));
#214810=CARTESIAN_POINT('Ctrl Pts',(5.49156208894257,-3.95862738756519,
128.498468391224));
#214811=CARTESIAN_POINT('Ctrl Pts',(5.60006720512561,-3.80359511868335,
128.507390901582));
#214812=CARTESIAN_POINT('Ctrl Pts',(5.70195934344626,-3.64416638556556,
128.516313411939));
#214813=CARTESIAN_POINT('Ctrl Pts',(5.80360181440798,-3.48512830231919,
128.525214059378));
#214814=CARTESIAN_POINT('Ctrl Pts',(5.89866350871404,-3.32171547240884,
128.534114706816));
#214815=CARTESIAN_POINT('Ctrl Pts',(5.98678516391366,-3.15447181016779,
128.543015354254));
#214816=CARTESIAN_POINT('Ctrl Pts',(6.07477063797122,-2.98748660236538,
128.551902246841));
#214817=CARTESIAN_POINT('Ctrl Pts',(6.15583734667113,-2.81668259853102,
128.560789139427));
#214818=CARTESIAN_POINT('Ctrl Pts',(6.22967022459886,-2.64263086577494,
128.569676032013));
#214819=CARTESIAN_POINT('Ctrl Pts',(6.30331332446926,-2.46902651094377,
128.578540081968));
#214820=CARTESIAN_POINT('Ctrl Pts',(6.36975959536808,-2.29219132178817,
128.587404131923));
#214821=CARTESIAN_POINT('Ctrl Pts',(6.42874095680524,-2.112718322516,128.596268181878));
#214822=CARTESIAN_POINT('Ctrl Pts',(6.48513188306158,-1.94112769760743,
128.604742926698));
#214823=CARTESIAN_POINT('Ctrl Pts',(6.53469939456372,-1.76712621777812,
128.613217671519));
#214824=CARTESIAN_POINT('Ctrl Pts',(6.57724914388337,-1.59125192828965,
128.621692416339));
#214825=CARTESIAN_POINT('Ctrl Pts',(6.6184642197997,-1.42089435136144,128.629901330768));
#214826=CARTESIAN_POINT('Ctrl Pts',(6.6530542122505,-1.24894359960696,128.638110245197));
#214827=CARTESIAN_POINT('Ctrl Pts',(6.68091396152673,-1.07595429209483,
128.646319159626));
#214828=CARTESIAN_POINT('Ctrl Pts',(6.70878033431683,-0.902923857253567,
128.654530025683));
#214829=CARTESIAN_POINT('Ctrl Pts',(6.72991321950296,-0.728854726296877,
128.66274089174));
#214830=CARTESIAN_POINT('Ctrl Pts',(6.74425911227886,-0.554308602173563,
128.670951757797));
#214831=CARTESIAN_POINT('Ctrl Pts',(6.75861097293342,-0.379689867017456,
128.679166039566));
#214832=CARTESIAN_POINT('Ctrl Pts',(6.76617018726055,-0.204594097975946,
128.687380321336));
#214833=CARTESIAN_POINT('Ctrl Pts',(6.7669353273155,-0.0295850626069757,
128.695594603106));
#214834=CARTESIAN_POINT('Ctrl Pts',(6.76770132859599,0.145620959247148,
128.703818130698));
#214835=CARTESIAN_POINT('Ctrl Pts',(6.76165797993374,0.320739696222828,
128.712041658291));
#214836=CARTESIAN_POINT('Ctrl Pts',(6.74885594684485,0.495209459458303,
128.720265185883));
#214837=CARTESIAN_POINT('Ctrl Pts',(6.73604570815073,0.669791051025288,
128.728493984437));
#214838=CARTESIAN_POINT('Ctrl Pts',(6.7164681890796,0.843722486719249,128.736722782991));
#214839=CARTESIAN_POINT('Ctrl Pts',(6.69022554282093,1.01645028712002,128.744951581544));
#214840=CARTESIAN_POINT('Ctrl Pts',(6.66394677565971,1.18941583351581,128.753191706381));
#214841=CARTESIAN_POINT('Ctrl Pts',(6.63098462397198,1.36117408682237,128.761431831217));
#214842=CARTESIAN_POINT('Ctrl Pts',(6.59149187850487,1.53118379550084,128.769671956054));
#214843=CARTESIAN_POINT('Ctrl Pts',(6.57395872932242,1.60666109011455,128.773330231424));
#214844=CARTESIAN_POINT('Ctrl Pts',(6.5551390564748,1.68179397001506,128.776988506794));
#214845=CARTESIAN_POINT('Ctrl Pts',(6.53504930254469,1.75653625448213,128.780646782164));
#214846=CARTESIAN_POINT('Ctrl Pts',(6.48865205642261,1.92915340948616,128.789095561742));
#214847=CARTESIAN_POINT('Ctrl Pts',(6.43537106265126,2.10008102358008,128.797544341319));
#214848=CARTESIAN_POINT('Ctrl Pts',(6.37534799585066,2.26875008138908,128.805993120897));
#214849=CARTESIAN_POINT('Ctrl Pts',(6.31538092067281,2.43726179878286,128.814434019157));
#214850=CARTESIAN_POINT('Ctrl Pts',(6.248684420805,2.60351884688755,128.822874917417));
#214851=CARTESIAN_POINT('Ctrl Pts',(6.1754502253491,2.76696648231159,128.831315815676));
#214852=CARTESIAN_POINT('Ctrl Pts',(6.10227306902599,2.93028681502789,128.839750139664));
#214853=CARTESIAN_POINT('Ctrl Pts',(6.02256850454503,3.09080179402754,128.848184463652));
#214854=CARTESIAN_POINT('Ctrl Pts',(5.93657683693599,3.24797544004802,128.85661878764));
#214855=CARTESIAN_POINT('Ctrl Pts',(5.85064623586848,3.40503747001023,128.865047122036));
#214856=CARTESIAN_POINT('Ctrl Pts',(5.75843759684971,3.55876260801143,128.873475456432));
#214857=CARTESIAN_POINT('Ctrl Pts',(5.66023783981895,3.70863810538069,128.881903790828));
#214858=CARTESIAN_POINT('Ctrl Pts',(5.56207889758102,3.85845130995453,128.890328622152));
#214859=CARTESIAN_POINT('Ctrl Pts',(5.45793398356232,4.0044177849552,128.898753453477));
#214860=CARTESIAN_POINT('Ctrl Pts',(5.34813447293877,4.14605193640455,128.907178284802));
#214861=CARTESIAN_POINT('Ctrl Pts',(5.23836526155172,4.28764700383043,128.91560079129));
#214862=CARTESIAN_POINT('Ctrl Pts',(5.12294476882755,4.42491186805172,128.924023297778));
#214863=CARTESIAN_POINT('Ctrl Pts',(5.00224617872701,4.55739203573832,128.932445804266));
#214864=CARTESIAN_POINT('Ctrl Pts',(4.88156404397508,4.68985414184407,128.940867162478));
#214865=CARTESIAN_POINT('Ctrl Pts',(4.75560547173743,4.81753260630425,128.94928852069));
#214866=CARTESIAN_POINT('Ctrl Pts',(4.62478245260127,4.94000771923601,128.957709878902));
#214867=CARTESIAN_POINT('Ctrl Pts',(4.49393193512466,5.06250857582034,128.966133007242));
#214868=CARTESIAN_POINT('Ctrl Pts',(4.35821516904719,5.17980366523237,128.974556135581));
#214869=CARTESIAN_POINT('Ctrl Pts',(4.21807990138325,5.29151121566861,128.98297926392));
#214870=CARTESIAN_POINT('Ctrl Pts',(4.07793088291443,5.40322972743354,128.991403218781));
#214871=CARTESIAN_POINT('Ctrl Pts',(3.9333627619541,5.5093594026608,128.999827173641));
#214872=CARTESIAN_POINT('Ctrl Pts',(3.7848550896124,5.60955978224987,129.008251128502));
#214873=CARTESIAN_POINT('Ctrl Pts',(3.63627224497738,5.70981088172569,129.016679347438));
#214874=CARTESIAN_POINT('Ctrl Pts',(3.48374614353515,5.8041265058107,129.025107566375));
#214875=CARTESIAN_POINT('Ctrl Pts',(3.32778464020283,5.8922099749101,129.033535785312));
#214876=CARTESIAN_POINT('Ctrl Pts',(3.25234212869507,5.934818169812,129.037612727317));
#214877=CARTESIAN_POINT('Ctrl Pts',(3.17609615240169,5.97596878037611,129.041689669322));
#214878=CARTESIAN_POINT('Ctrl Pts',(3.09910619832118,6.01563211736948,129.045766611327));
#214879=CARTESIAN_POINT('Ctrl Pts',(3.09910619832142,6.01563211736936,127.045755263024));
#214880=CARTESIAN_POINT('Ctrl Pts',(2.93375330764834,6.10081787314649,127.054504710927));
#214881=CARTESIAN_POINT('Ctrl Pts',(2.76488627843078,6.17918207037036,127.063254158829));
#214882=CARTESIAN_POINT('Ctrl Pts',(2.59307866646709,6.25045854553994,127.072003606731));
#214883=CARTESIAN_POINT('Ctrl Pts',(2.4212724418539,6.32173444515032,127.080752983982));
#214884=CARTESIAN_POINT('Ctrl Pts',(2.24652594672485,6.38592262741831,127.089502361232));
#214885=CARTESIAN_POINT('Ctrl Pts',(2.06943269687149,6.44280508110553,127.098251738482));
#214886=CARTESIAN_POINT('Ctrl Pts',(1.89234081822105,6.49968709436158,127.107001047988));
#214887=CARTESIAN_POINT('Ctrl Pts',(1.71290249405617,6.54926340459537,127.115750357493));
#214888=CARTESIAN_POINT('Ctrl Pts',(1.53172716625088,6.59136563150377,127.124499666998));
#214889=CARTESIAN_POINT('Ctrl Pts',(1.35055318107381,6.633467546407,127.133248911665));
#214890=CARTESIAN_POINT('Ctrl Pts',(1.16764249714483,6.66809542395764,127.141998156333));
#214891=CARTESIAN_POINT('Ctrl Pts',(0.983616340615169,6.69513165624656,
127.150747401));
#214892=CARTESIAN_POINT('Ctrl Pts',(0.799591486714658,6.72216769715951,
127.159496583736));
#214893=CARTESIAN_POINT('Ctrl Pts',(0.614451459527529,6.74161215869364,
127.168245766471));
#214894=CARTESIAN_POINT('Ctrl Pts',(0.4288250479111,6.75339900185707,127.176994949207));
#214895=CARTESIAN_POINT('Ctrl Pts',(0.243199888597772,6.76518576550218,
127.185744072918));
#214896=CARTESIAN_POINT('Ctrl Pts',(0.0570886373925512,6.76931499599834,
127.194493196628));
#214897=CARTESIAN_POINT('Ctrl Pts',(-0.128876626810609,6.76577266947848,
127.203242320339));
#214898=CARTESIAN_POINT('Ctrl Pts',(-0.314840698187433,6.76223036567996,
127.21199138793));
#214899=CARTESIAN_POINT('Ctrl Pts',(-0.500658497950342,6.75101660879229,
127.220740455522));
#214900=CARTESIAN_POINT('Ctrl Pts',(-0.685698951925125,6.73216948296229,
127.229489523113));
#214901=CARTESIAN_POINT('Ctrl Pts',(-0.870738280458545,6.7133224717631,
127.238238537492));
#214902=CARTESIAN_POINT('Ctrl Pts',(-1.05499998761099,6.6868422135621,127.24698755187));
#214903=CARTESIAN_POINT('Ctrl Pts',(-1.23785829161247,6.65281863948554,
127.255736566249));
#214904=CARTESIAN_POINT('Ctrl Pts',(-1.43007412917228,6.61705395368899,
127.264933299948));
#214905=CARTESIAN_POINT('Ctrl Pts',(-1.62073882535614,6.57295372727834,
127.274130033647));
#214906=CARTESIAN_POINT('Ctrl Pts',(-1.80913696091334,6.52068343478329,
127.283326767346));
#214907=CARTESIAN_POINT('Ctrl Pts',(-1.98838356185933,6.47095219815253,
127.29207676506));
#214908=CARTESIAN_POINT('Ctrl Pts',(-2.16557827572356,6.41382586850951,
127.300826762774));
#214909=CARTESIAN_POINT('Ctrl Pts',(-2.34011918621525,6.34949849943342,
127.309576760487));
#214910=CARTESIAN_POINT('Ctrl Pts',(-2.51465655690918,6.28517243495622,
127.318326580746));
#214911=CARTESIAN_POINT('Ctrl Pts',(-2.68653996295144,6.21364572242454,
127.327076401004));
#214912=CARTESIAN_POINT('Ctrl Pts',(-2.85518555379801,6.13516132252308,
127.335826221262));
#214913=CARTESIAN_POINT('Ctrl Pts',(-3.02382794858505,6.05667841000599,
127.3445758757));
#214914=CARTESIAN_POINT('Ctrl Pts',(-3.18923239109101,5.97123819492177,
127.353325530137));
#214915=CARTESIAN_POINT('Ctrl Pts',(-3.35083705967523,5.87913088810813,
127.362075184575));
#214916=CARTESIAN_POINT('Ctrl Pts',(-3.51243888042223,5.7870252044321,127.370824684824));
#214917=CARTESIAN_POINT('Ctrl Pts',(-3.67024081223512,5.68825280605898,
127.379574185073));
#214918=CARTESIAN_POINT('Ctrl Pts',(-3.82370687544222,5.58314917682628,
127.388323685322));
#214919=CARTESIAN_POINT('Ctrl Pts',(-3.97717043817636,5.47804726008151,
127.397073043012));
#214920=CARTESIAN_POINT('Ctrl Pts',(-4.12629803722282,5.36661448084373,
127.405822400703));
#214921=CARTESIAN_POINT('Ctrl Pts',(-4.2705831720673,5.24922931204721,127.414571758393));
#214922=CARTESIAN_POINT('Ctrl Pts',(-4.41486614774675,5.13184589986929,
127.423320985153));
#214923=CARTESIAN_POINT('Ctrl Pts',(-4.55430658194271,5.00851045723165,
127.432070211913));
#214924=CARTESIAN_POINT('Ctrl Pts',(-4.68843089001719,4.87964187103241,
127.440819438673));
#214925=CARTESIAN_POINT('Ctrl Pts',(-4.82255336917711,4.75077504208087,
127.449568546129));
#214926=CARTESIAN_POINT('Ctrl Pts',(-4.95135966065011,4.61637541908226,
127.458317653585));
#214927=CARTESIAN_POINT('Ctrl Pts',(-5.07441230869123,4.47689945401982,
127.467066761041));
#214928=CARTESIAN_POINT('Ctrl Pts',(-5.19746344226297,4.33742520555659,
127.475815760817));
#214929=CARTESIAN_POINT('Ctrl Pts',(-5.31476088454649,4.19287495491486,
127.484564760594));
#214930=CARTESIAN_POINT('Ctrl Pts',(-5.42590627628738,4.04373961586862,
127.49331376037));
#214931=CARTESIAN_POINT('Ctrl Pts',(-5.53706380672565,3.89458798906881,
127.502063715665));
#214932=CARTESIAN_POINT('Ctrl Pts',(-5.64206777071774,3.74085050155421,
127.51081367096));
#214933=CARTESIAN_POINT('Ctrl Pts',(-5.74056148163929,3.58304938223287,
127.519563626254));
#214934=CARTESIAN_POINT('Ctrl Pts',(-5.83905138951799,3.42525435593426,
127.528313243695));
#214935=CARTESIAN_POINT('Ctrl Pts',(-5.93103139557562,3.26339625497346,
127.537062861136));
#214936=CARTESIAN_POINT('Ctrl Pts',(-6.01618907820752,3.09802485065187,
127.545812478578));
#214937=CARTESIAN_POINT('Ctrl Pts',(-6.10134392544901,2.93265895249813,
127.554561804693));
#214938=CARTESIAN_POINT('Ctrl Pts',(-6.1796767726176,2.76378023986197,127.563311130809));
#214939=CARTESIAN_POINT('Ctrl Pts',(-6.25092157009161,2.59196229227267,
127.572060456925));
#214940=CARTESIAN_POINT('Ctrl Pts',(-6.32216437407696,2.4201491522924,127.580809538228));
#214941=CARTESIAN_POINT('Ctrl Pts',(-6.3863194154887,2.24539720662996,127.58955861953));
#214942=CARTESIAN_POINT('Ctrl Pts',(-6.44316881037492,2.06829994947828,
127.598307700833));
#214943=CARTESIAN_POINT('Ctrl Pts',(-6.50002334524528,1.89118668024599,
127.607057573175));
#214944=CARTESIAN_POINT('Ctrl Pts',(-6.54957082411055,1.71172794807858,
127.615807445517));
#214945=CARTESIAN_POINT('Ctrl Pts',(-6.59164294296046,1.53053334250502,
127.62455731786));
#214946=CARTESIAN_POINT('Ctrl Pts',(-6.63371214082104,1.34935131693749,
127.633306582715));
#214947=CARTESIAN_POINT('Ctrl Pts',(-6.66830695239666,1.166433938299,127.642055847569));
#214948=CARTESIAN_POINT('Ctrl Pts',(-6.6953098815397,0.982402458342219,
127.650805112424));
#214949=CARTESIAN_POINT('Ctrl Pts',(-6.72231419690468,0.798361530948305,
127.659554826431));
#214950=CARTESIAN_POINT('Ctrl Pts',(-6.74172580829266,0.61320667136374,
127.668304540438));
#214951=CARTESIAN_POINT('Ctrl Pts',(-6.75347878028171,0.427566795114677,
127.677054254445));
#214952=CARTESIAN_POINT('Ctrl Pts',(-6.76248992368202,0.285234494207743,
127.683762764234));
#214953=CARTESIAN_POINT('Ctrl Pts',(-6.76699999999987,0.142617266095797,
127.690471274022));
#214954=CARTESIAN_POINT('Ctrl Pts',(-6.767,6.29785154665824E-12,127.69717978381));
#214955=CARTESIAN_POINT('',(-6.767,6.9710326081884E-10,127.302820216158));
#214956=CARTESIAN_POINT('Ctrl Pts',(3.0991061983215,6.01563211736932,126.651395695404));
#214957=CARTESIAN_POINT('Ctrl Pts',(2.9337533076484,6.10081787314647,126.660145143307));
#214958=CARTESIAN_POINT('Ctrl Pts',(2.76488627843081,6.17918207037034,126.668894591209));
#214959=CARTESIAN_POINT('Ctrl Pts',(2.5930786664671,6.25045854553994,126.677644039111));
#214960=CARTESIAN_POINT('Ctrl Pts',(2.42127244185376,6.32173444515037,126.686393416362));
#214961=CARTESIAN_POINT('Ctrl Pts',(2.24652594672456,6.38592262741841,126.695142793612));
#214962=CARTESIAN_POINT('Ctrl Pts',(2.06943269687104,6.44280508110567,126.703892170862));
#214963=CARTESIAN_POINT('Ctrl Pts',(1.89234081822057,6.49968709436172,126.712641480368));
#214964=CARTESIAN_POINT('Ctrl Pts',(1.71290249405566,6.54926340459551,126.721390789873));
#214965=CARTESIAN_POINT('Ctrl Pts',(1.53172716625033,6.59136563150389,126.730140099378));
#214966=CARTESIAN_POINT('Ctrl Pts',(1.3505531810731,6.63346754640715,126.738889344046));
#214967=CARTESIAN_POINT('Ctrl Pts',(1.16764249714397,6.6680954239578,126.747638588713));
#214968=CARTESIAN_POINT('Ctrl Pts',(0.983616340614145,6.69513165624671,
126.75638783338));
#214969=CARTESIAN_POINT('Ctrl Pts',(0.799591486713599,6.72216769715964,
126.765137016116));
#214970=CARTESIAN_POINT('Ctrl Pts',(0.614451459526438,6.74161215869374,
126.773886198851));
#214971=CARTESIAN_POINT('Ctrl Pts',(0.428825047909977,6.75339900185714,
126.782635381587));
#214972=CARTESIAN_POINT('Ctrl Pts',(0.243199888596744,6.76518576550222,
126.791384505298));
#214973=CARTESIAN_POINT('Ctrl Pts',(0.0570886373916206,6.76931499599834,
126.800133629008));
#214974=CARTESIAN_POINT('Ctrl Pts',(-0.128876626811441,6.76577266947846,
126.808882752719));
#214975=CARTESIAN_POINT('Ctrl Pts',(-0.314840698188423,6.76223036567992,
126.81763182031));
#214976=CARTESIAN_POINT('Ctrl Pts',(-0.500658497951488,6.75101660879221,
126.826380887902));
#214977=CARTESIAN_POINT('Ctrl Pts',(-0.685698951926425,6.73216948296216,
126.835129955493));
#214978=CARTESIAN_POINT('Ctrl Pts',(-0.870738280459872,6.71332247176292,
126.843878969872));
#214979=CARTESIAN_POINT('Ctrl Pts',(-1.05499998761234,6.68684221356189,
126.85262798425));
#214980=CARTESIAN_POINT('Ctrl Pts',(-1.23785829161385,6.65281863948529,
126.861376998629));
#214981=CARTESIAN_POINT('Ctrl Pts',(-1.43007412915944,6.61705395369134,
126.870573732327));
#214982=CARTESIAN_POINT('Ctrl Pts',(-1.6207388253293,6.57295372728452,126.879770466026));
#214983=CARTESIAN_POINT('Ctrl Pts',(-1.80913696087289,6.52068343479452,
126.888967199724));
#214984=CARTESIAN_POINT('Ctrl Pts',(-1.98838356181923,6.47095219816486,
126.897717197438));
#214985=CARTESIAN_POINT('Ctrl Pts',(-2.16557827568384,6.41382586852292,
126.906467195152));
#214986=CARTESIAN_POINT('Ctrl Pts',(-2.34011918617595,6.34949849944791,
126.915217192865));
#214987=CARTESIAN_POINT('Ctrl Pts',(-2.51465655687044,6.28517243497173,
126.923967013124));
#214988=CARTESIAN_POINT('Ctrl Pts',(-2.68653996291328,6.21364572244104,
126.932716833382));
#214989=CARTESIAN_POINT('Ctrl Pts',(-2.85518555376046,6.13516132254055,
126.94146665364));
#214990=CARTESIAN_POINT('Ctrl Pts',(-3.0238279485479,6.05667841002453,126.950216308078));
#214991=CARTESIAN_POINT('Ctrl Pts',(-3.1892323910543,5.97123819494137,126.958965962515));
#214992=CARTESIAN_POINT('Ctrl Pts',(-3.350837059639,5.87913088812878,126.967715616953));
#214993=CARTESIAN_POINT('Ctrl Pts',(-3.51243888038659,5.78702520445373,
126.976465117202));
#214994=CARTESIAN_POINT('Ctrl Pts',(-3.67024081220012,5.68825280608157,
126.985214617451));
#214995=CARTESIAN_POINT('Ctrl Pts',(-3.82370687540789,5.58314917684979,
126.9939641177));
#214996=CARTESIAN_POINT('Ctrl Pts',(-3.9771704381427,5.47804726010595,127.00271347539));
#214997=CARTESIAN_POINT('Ctrl Pts',(-4.12629803718987,5.36661448086907,
127.011462833081));
#214998=CARTESIAN_POINT('Ctrl Pts',(-4.27058317203509,5.24922931207341,
127.020212190771));
#214999=CARTESIAN_POINT('Ctrl Pts',(-4.41486614771509,5.13184589989652,
127.028961417531));
#215000=CARTESIAN_POINT('Ctrl Pts',(-4.55430658191164,5.00851045725989,
127.037710644291));
#215001=CARTESIAN_POINT('Ctrl Pts',(-4.68843088998676,4.87964187106164,
127.046459871051));
#215002=CARTESIAN_POINT('Ctrl Pts',(-4.8225533691476,4.75077504211083,127.055208978507));
#215003=CARTESIAN_POINT('Ctrl Pts',(-4.95135966062154,4.6163754191129,127.063958085963));
#215004=CARTESIAN_POINT('Ctrl Pts',(-5.07441230866363,4.47689945405111,
127.072707193419));
#215005=CARTESIAN_POINT('Ctrl Pts',(-5.19746344223616,4.33742520558871,
127.081456193195));
#215006=CARTESIAN_POINT('Ctrl Pts',(-5.31476088452052,4.19287495494778,
127.090205192972));
#215007=CARTESIAN_POINT('Ctrl Pts',(-5.42590627626227,4.04373961590231,
127.098954192748));
#215008=CARTESIAN_POINT('Ctrl Pts',(-5.53706380670133,3.89458798910337,
127.107704148043));
#215009=CARTESIAN_POINT('Ctrl Pts',(-5.64206777069426,3.74085050158961,
127.116454103338));
#215010=CARTESIAN_POINT('Ctrl Pts',(-5.74056148161669,3.58304938226908,
127.125204058632));
#215011=CARTESIAN_POINT('Ctrl Pts',(-5.83905138949646,3.42525435597096,
127.133953676073));
#215012=CARTESIAN_POINT('Ctrl Pts',(-5.93103139555519,3.26339625501061,
127.142703293514));
#215013=CARTESIAN_POINT('Ctrl Pts',(-6.0161890781882,3.0980248506894,127.151452910956));
#215014=CARTESIAN_POINT('Ctrl Pts',(-6.10134392543061,2.9326589525364,127.160202237071));
#215015=CARTESIAN_POINT('Ctrl Pts',(-6.17967677260016,2.76378023990094,
127.168951563187));
#215016=CARTESIAN_POINT('Ctrl Pts',(-6.25092157007518,2.5919622923123,127.177700889303));
#215017=CARTESIAN_POINT('Ctrl Pts',(-6.32216437406154,2.42014915233269,
127.186449970606));
#215018=CARTESIAN_POINT('Ctrl Pts',(-6.38631941547431,2.24539720667087,
127.195199051908));
#215019=CARTESIAN_POINT('Ctrl Pts',(-6.4431688103616,2.06829994951977,127.20394813321));
#215020=CARTESIAN_POINT('Ctrl Pts',(-6.50002334523311,1.89118668028781,
127.212698005553));
#215021=CARTESIAN_POINT('Ctrl Pts',(-6.54957082409955,1.71172794812069,
127.221447877895));
#215022=CARTESIAN_POINT('Ctrl Pts',(-6.59164294295062,1.53053334254738,
127.230197750238));
#215023=CARTESIAN_POINT('Ctrl Pts',(-6.63371214081235,1.34935131698021,
127.238947015092));
#215024=CARTESIAN_POINT('Ctrl Pts',(-6.66830695238913,1.16643393834204,
127.247696279947));
#215025=CARTESIAN_POINT('Ctrl Pts',(-6.69530988153335,0.982402458385534,
127.256445544802));
#215026=CARTESIAN_POINT('Ctrl Pts',(-6.7223141968995,0.798361530991892,
127.265195258809));
#215027=CARTESIAN_POINT('Ctrl Pts',(-6.74172580828867,0.613206671407551,
127.273944972816));
#215028=CARTESIAN_POINT('Ctrl Pts',(-6.75347878027893,0.427566795158662,
127.282694686823));
#215029=CARTESIAN_POINT('Ctrl Pts',(-6.76248992366655,0.285234494466871,
127.289403196601));
#215030=CARTESIAN_POINT('Ctrl Pts',(-6.76699999998531,0.142617266570896,
127.296111706379));
#215031=CARTESIAN_POINT('Ctrl Pts',(-6.767,6.96911759829614E-10,127.302820216158));
#215032=CARTESIAN_POINT('Ctrl Pts',(-6.767,6.44645169383305E-12,127.30282021619));
#215033=CARTESIAN_POINT('Ctrl Pts',(-6.76700000000018,-0.186007249520387,
127.311569728001));
#215034=CARTESIAN_POINT('Ctrl Pts',(-6.75932637294556,-0.372014355743401,
127.320319239812));
#215035=CARTESIAN_POINT('Ctrl Pts',(-6.74400518264234,-0.557389537480952,
127.329068751624));
#215036=CARTESIAN_POINT('Ctrl Pts',(-6.72868405705156,-0.742763936245431,
127.337818226479));
#215037=CARTESIAN_POINT('Ctrl Pts',(-6.70571545645811,-0.92750613023609,
127.346567701335));
#215038=CARTESIAN_POINT('Ctrl Pts',(-6.67517739404901,-1.11098863989562,
127.355317176191));
#215039=CARTESIAN_POINT('Ctrl Pts',(-6.64463945808784,-1.29447038981527,
127.364066614818));
#215040=CARTESIAN_POINT('Ctrl Pts',(-6.60653217008442,-1.47669218313298,
127.372816053445));
#215041=CARTESIAN_POINT('Ctrl Pts',(-6.56098496092766,-1.65703510598935,
127.381565492072));
#215042=CARTESIAN_POINT('Ctrl Pts',(-6.51543793658396,-1.83737729708346,
127.390314895197));
#215043=CARTESIAN_POINT('Ctrl Pts',(-6.46245112167531,-2.01584035510571,
127.399064298322));
#215044=CARTESIAN_POINT('Ctrl Pts',(-6.40220448374376,-2.19181813760434,
127.407813701447));
#215045=CARTESIAN_POINT('Ctrl Pts',(-6.34195808526638,-2.36779522066783,
127.416563069797));
#215046=CARTESIAN_POINT('Ctrl Pts',(-6.27445201433251,-2.54128677683803,
127.425312438147));
#215047=CARTESIAN_POINT('Ctrl Pts',(-6.19991555072061,-2.71170355384447,
127.434061806497));
#215048=CARTESIAN_POINT('Ctrl Pts',(-6.12537937716864,-2.88211966767113,
127.442811140799));
#215049=CARTESIAN_POINT('Ctrl Pts',(-6.04381298052703,-3.04946076371422,
127.451560475101));
#215050=CARTESIAN_POINT('Ctrl Pts',(-5.95549339336027,-3.21315848374185,
127.460309809403));
#215051=CARTESIAN_POINT('Ctrl Pts',(-5.86717414255612,-3.37685558033141,
127.469059110383));
#215052=CARTESIAN_POINT('Ctrl Pts',(-5.77210188876808,-3.53690907646415,
127.477808411363));
#215053=CARTESIAN_POINT('Ctrl Pts',(-5.67059953347211,-3.69277536968956,
127.486557712343));
#215054=CARTESIAN_POINT('Ctrl Pts',(-5.56909755631596,-3.84864108224617,
127.495306980729));
#215055=CARTESIAN_POINT('Ctrl Pts',(-5.46116568197058,-4.00031938297234,
127.504056249114));
#215056=CARTESIAN_POINT('Ctrl Pts',(-5.34717048533805,-4.14729511859594,
127.512805517499));
#215057=CARTESIAN_POINT('Ctrl Pts',(-5.23317570392044,-4.29427031887663,
127.521554754016));
#215058=CARTESIAN_POINT('Ctrl Pts',(-5.11311782003727,-4.43654276189302,
127.530303990533));
#215059=CARTESIAN_POINT('Ctrl Pts',(-4.98740458984971,-4.57362924351615,
127.53905322705));
#215060=CARTESIAN_POINT('Ctrl Pts',(-4.86169180711974,-4.71071523720028,
127.547802432426));
#215061=CARTESIAN_POINT('Ctrl Pts',(-4.73032391204415,-4.84261509522999,
127.556551637801));
#215062=CARTESIAN_POINT('Ctrl Pts',(-4.59374707013856,-4.96888084538092,
127.565300843177));
#215063=CARTESIAN_POINT('Ctrl Pts',(-4.45717070301705,-5.09514615659236,
127.574050018137));
#215064=CARTESIAN_POINT('Ctrl Pts',(-4.31538563571304,-5.2157772045931,
127.582799193098));
#215065=CARTESIAN_POINT('Ctrl Pts',(-4.16887341029775,-5.33036429232679,
127.591548368058));
#215066=CARTESIAN_POINT('Ctrl Pts',(-4.02236168203971,-5.4449509912342,
127.60029751333));
#215067=CARTESIAN_POINT('Ctrl Pts',(-3.8711230534843,-5.55349359438418,
127.609046658602));
#215068=CARTESIAN_POINT('Ctrl Pts',(-3.71567117018023,-5.65562346298721,
127.617795803874));
#215069=CARTESIAN_POINT('Ctrl Pts',(-3.56021980146088,-5.75775299351478,
127.626544920184));
#215070=CARTESIAN_POINT('Ctrl Pts',(-3.40055544538624,-5.85346967463713,
127.635294036494));
#215071=CARTESIAN_POINT('Ctrl Pts',(-3.23722035987134,-5.94244842986748,
127.644043152805));
#215072=CARTESIAN_POINT('Ctrl Pts',(-3.07388580147439,-6.03142689794398,
127.652792240879));
#215073=CARTESIAN_POINT('Ctrl Pts',(-2.90688078896814,-6.1136673465667,
127.661541328954));
#215074=CARTESIAN_POINT('Ctrl Pts',(-2.73677250721582,-6.1888904695226,
127.670290417029));
#215075=CARTESIAN_POINT('Ctrl Pts',(-2.56666476031689,-6.26411335596242,
127.679039477595));
#215076=CARTESIAN_POINT('Ctrl Pts',(-2.39345402575367,-6.3323188450048,
127.687788538161));
#215077=CARTESIAN_POINT('Ctrl Pts',(-2.21772856065787,-6.39327529762659,
127.696537598727));
#215078=CARTESIAN_POINT('Ctrl Pts',(-2.04200363348673,-6.45423156365062,
127.705286632511));
#215079=CARTESIAN_POINT('Ctrl Pts',(-1.86376426189401,-6.50793874375624,
127.714035666295));
#215080=CARTESIAN_POINT('Ctrl Pts',(-1.68361577753238,-6.5542144390952,
127.722784700078));
#215081=CARTESIAN_POINT('Ctrl Pts',(-1.50346782967888,-6.60048999661848,
127.731533707806));
#215082=CARTESIAN_POINT('Ctrl Pts',(-1.32141105795079,-6.63933404237694,
127.740282715534));
#215083=CARTESIAN_POINT('Ctrl Pts',(-1.13806375487118,-6.67061465607545,
127.749031723262));
#215084=CARTESIAN_POINT('Ctrl Pts',(-0.954716982604014,-6.70189517921282,
127.75778070566));
#215085=CARTESIAN_POINT('Ctrl Pts',(-0.770079968903175,-6.72561226592216,
127.766529688059));
#215086=CARTESIAN_POINT('Ctrl Pts',(-0.58477976555932,-6.74168536983093,
127.775278670457));
#215087=CARTESIAN_POINT('Ctrl Pts',(-0.391489830652405,-6.75845151013846,
127.784404889467));
#215088=CARTESIAN_POINT('Ctrl Pts',(-0.197478578239474,-6.76689983031622,
127.793531108477));
#215089=CARTESIAN_POINT('Ctrl Pts',(-0.00346287645251185,-6.76699911397118,
127.802657327487));
#215090=CARTESIAN_POINT('Ctrl Pts',(0.184489834653576,-6.76709529501192,
127.811498352152));
#215091=CARTESIAN_POINT('Ctrl Pts',(0.372446404249023,-6.7593563973817,
127.820339376818));
#215092=CARTESIAN_POINT('Ctrl Pts',(0.559755019487951,-6.7438092587319,
127.829180401484));
#215093=CARTESIAN_POINT('Ctrl Pts',(0.745134705521472,-6.72842222659809,
127.837930380094));
#215094=CARTESIAN_POINT('Ctrl Pts',(0.929879431228346,-6.70538706057527,
127.846680358704));
#215095=CARTESIAN_POINT('Ctrl Pts',(1.11336163626811,-6.6747820089413,127.855430337313));
#215096=CARTESIAN_POINT('Ctrl Pts',(1.29684196300721,-6.64417727061013,
127.86418022635));
#215097=CARTESIAN_POINT('Ctrl Pts',(1.47905951217528,-6.60600284890587,
127.872930115386));
#215098=CARTESIAN_POINT('Ctrl Pts',(1.65939532067118,-6.56038841607222,
127.881680004423));
#215099=CARTESIAN_POINT('Ctrl Pts',(1.83972934300847,-6.51477443503244,
127.890429806795));
#215100=CARTESIAN_POINT('Ctrl Pts',(2.01818138406321,-6.46172066062124,
127.899179609167));
#215101=CARTESIAN_POINT('Ctrl Pts',(2.19414528354267,-6.40140730423455,
127.907929411539));
#215102=CARTESIAN_POINT('Ctrl Pts',(2.37010749864065,-6.34109452518618,
127.916679130156));
#215103=CARTESIAN_POINT('Ctrl Pts',(2.54358134866523,-6.27352239616478,
127.925428848772));
#215104=CARTESIAN_POINT('Ctrl Pts',(2.71397759435617,-6.19892043966792,
127.934178567388));
#215105=CARTESIAN_POINT('Ctrl Pts',(2.8843722655819,-6.12431917249484,127.942928205157));
#215106=CARTESIAN_POINT('Ctrl Pts',(3.05168912681027,-6.04268832278763,
127.951677842926));
#215107=CARTESIAN_POINT('Ctrl Pts',(3.21535986273929,-5.95430516123294,
127.960427480695));
#215108=CARTESIAN_POINT('Ctrl Pts',(3.37902914072932,-5.86592278697389,
127.969177040524));
#215109=CARTESIAN_POINT('Ctrl Pts',(3.53905210621676,-5.77078835741878,
127.977926600353));
#215110=CARTESIAN_POINT('Ctrl Pts',(3.69488522831815,-5.66922500431553,
127.986676160182));
#215111=CARTESIAN_POINT('Ctrl Pts',(3.8507170140707,-5.56766252217004,127.995425644979));
#215112=CARTESIAN_POINT('Ctrl Pts',(4.00235878822546,-5.45967138329266,
128.004175129776));
#215113=CARTESIAN_POINT('Ctrl Pts',(4.14929549611478,-5.34561838199488,
128.012924614573));
#215114=CARTESIAN_POINT('Ctrl Pts',(4.29623099276244,-5.23156632086889,
128.021674027246));
#215115=CARTESIAN_POINT('Ctrl Pts',(4.43846127436184,-5.11145267304829,
128.030423439918));
#215116=CARTESIAN_POINT('Ctrl Pts',(4.57550326054599,-4.98568540049741,
128.039172852591));
#215117=CARTESIAN_POINT('Ctrl Pts',(4.7125441625794,-4.85991912290207,128.047922196046));
#215118=CARTESIAN_POINT('Ctrl Pts',(4.84439664018921,-4.72849950385255,
128.056671539501));
#215119=CARTESIAN_POINT('Ctrl Pts',(4.97061286794906,-4.59187289860894,
128.065420882957));
#215120=CARTESIAN_POINT('Ctrl Pts',(5.09682813912843,-4.45524732884504,
128.074170160101));
#215121=CARTESIAN_POINT('Ctrl Pts',(5.21740705147994,-4.313415062356,128.082919437246));
#215122=CARTESIAN_POINT('Ctrl Pts',(5.33194007545848,-4.1668578127553,128.091668714391));
#215123=CARTESIAN_POINT('Ctrl Pts',(5.44647226944626,-4.0203016252165,128.100417928132));
#215124=CARTESIAN_POINT('Ctrl Pts',(5.55495848628244,-3.86902074887746,
128.109167141873));
#215125=CARTESIAN_POINT('Ctrl Pts',(5.65703027291908,-3.71352898080479,
128.117916355615));
#215126=CARTESIAN_POINT('Ctrl Pts',(5.75910135377118,-3.55803828789393,
128.126665508858));
#215127=CARTESIAN_POINT('Ctrl Pts',(5.85475793592873,-3.39833700106505,
128.135414662102));
#215128=CARTESIAN_POINT('Ctrl Pts',(5.94367514427518,-3.23496750823335,
128.144163815346));
#215129=CARTESIAN_POINT('Ctrl Pts',(6.03259176732757,-3.07159909077495,
128.152912910999));
#215130=CARTESIAN_POINT('Ctrl Pts',(6.11476896836039,-2.90456276731193,
128.161662006652));
#215131=CARTESIAN_POINT('Ctrl Pts',(6.18992765547998,-2.73442583002797,
128.170411102305));
#215132=CARTESIAN_POINT('Ctrl Pts',(6.26508587283162,-2.56428995615908,
128.179160143273));
#215133=CARTESIAN_POINT('Ctrl Pts',(6.33322554827263,-2.3910537693493,128.187909184241));
#215134=CARTESIAN_POINT('Ctrl Pts',(6.39411526733128,-2.21530561053799,
128.196658225209));
#215135=CARTESIAN_POINT('Ctrl Pts',(6.45500462602938,-2.03955849184812,
128.205407214398));
#215136=CARTESIAN_POINT('Ctrl Pts',(6.50864402040824,-1.86129970164252,
128.214156203587));
#215137=CARTESIAN_POINT('Ctrl Pts',(6.55485128368677,-1.68113463135761,
128.222905192776));
#215138=CARTESIAN_POINT('Ctrl Pts',(6.60199809554389,-1.4973062011659,128.231832078248));
#215139=CARTESIAN_POINT('Ctrl Pts',(6.64140720707924,-1.3114934324544,128.240758963719));
#215140=CARTESIAN_POINT('Ctrl Pts',(6.67293928722924,-1.12435326697288,
128.24968584919));
#215141=CARTESIAN_POINT('Ctrl Pts',(6.7038462587629,-0.940923067004233,
128.258435763368));
#215142=CARTESIAN_POINT('Ctrl Pts',(6.72718554579822,-0.756217899519327,
128.267185677545));
#215143=CARTESIAN_POINT('Ctrl Pts',(6.74287786815347,-0.570865181252181,
128.275935591723));
#215144=CARTESIAN_POINT('Ctrl Pts',(6.75856988190858,-0.385516108071698,
128.284685333827));
#215145=CARTESIAN_POINT('Ctrl Pts',(6.76661520773409,-0.19951979522417,
128.293435075932));
#215146=CARTESIAN_POINT('Ctrl Pts',(6.76698651789579,-0.013508020453543,
128.302184818036));
#215147=CARTESIAN_POINT('Ctrl Pts',(6.76735782124897,0.172500343514992,
128.310934399701));
#215148=CARTESIAN_POINT('Ctrl Pts',(6.76005538995173,0.358523882212877,
128.319683981366));
#215149=CARTESIAN_POINT('Ctrl Pts',(6.74510402742346,0.543930748566255,
128.328433563031));
#215150=CARTESIAN_POINT('Ctrl Pts',(6.7301529191801,0.729334461617104,128.337182995888));
#215151=CARTESIAN_POINT('Ctrl Pts',(6.70755316306569,0.914121237636537,
128.345932428745));
#215152=CARTESIAN_POINT('Ctrl Pts',(6.67738151874544,1.09766345166306,128.354681861601));
#215153=CARTESIAN_POINT('Ctrl Pts',(6.64721034747534,1.28120278799847,128.363431157279));
#215154=CARTESIAN_POINT('Ctrl Pts',(6.60946757205101,1.46349731860511,128.372180452956));
#215155=CARTESIAN_POINT('Ctrl Pts',(6.56428138111478,1.64392790278342,128.380929748634));
#215156=CARTESIAN_POINT('Ctrl Pts',(6.51909583859801,1.82435589779231,128.389678918759));
#215157=CARTESIAN_POINT('Ctrl Pts',(6.46646716392823,2.00291972192435,128.398428088885));
#215158=CARTESIAN_POINT('Ctrl Pts',(6.40657409872828,2.17901292274827,128.407177259011));
#215159=CARTESIAN_POINT('Ctrl Pts',(6.34668181342021,2.35510383059125,128.41592631521));
#215160=CARTESIAN_POINT('Ctrl Pts',(6.27952541913996,2.52872390822712,128.424675371409));
#215161=CARTESIAN_POINT('Ctrl Pts',(6.20533299175466,2.69928350890402,128.433424427608));
#215162=CARTESIAN_POINT('Ctrl Pts',(6.12831602991496,2.87633637965736,128.442506563766));
#215163=CARTESIAN_POINT('Ctrl Pts',(6.04371690605215,3.0500908660157,128.451588699924));
#215164=CARTESIAN_POINT('Ctrl Pts',(5.95184520316575,3.21991112882838,128.460670836082));
#215165=CARTESIAN_POINT('Ctrl Pts',(5.86333549509214,3.38351691183122,128.469420616426));
#215166=CARTESIAN_POINT('Ctrl Pts',(5.76807618099303,3.5434710371211,128.47817039677));
#215167=CARTESIAN_POINT('Ctrl Pts',(5.66639083308946,3.69923018027802,128.486920177113));
#215168=CARTESIAN_POINT('Ctrl Pts',(5.56470914082125,3.85498372382159,128.495669642898));
#215169=CARTESIAN_POINT('Ctrl Pts',(5.45660203371985,4.0065423470211,128.504419108683));
#215170=CARTESIAN_POINT('Ctrl Pts',(5.34243669839128,4.15339127986783,128.513168574468));
#215171=CARTESIAN_POINT('Ctrl Pts',(5.22827486050494,4.30023571401398,128.521917772214));
#215172=CARTESIAN_POINT('Ctrl Pts',(5.10805534167005,4.44237052028592,128.53066696996));
#215173=CARTESIAN_POINT('Ctrl Pts',(4.98218644339836,4.57931296628847,128.539416167706));
#215174=CARTESIAN_POINT('Ctrl Pts',(4.85632073219448,4.71625194483504,128.548165143918));
#215175=CARTESIAN_POINT('Ctrl Pts',(4.72480612170155,4.84799861524669,128.556914120129));
#215176=CARTESIAN_POINT('Ctrl Pts',(4.58808925235122,4.9741055489866,128.565663096341));
#215177=CARTESIAN_POINT('Ctrl Pts',(4.45136349473857,5.10022068121373,128.574412641343));
#215178=CARTESIAN_POINT('Ctrl Pts',(4.30943501209888,5.22069514871992,128.583162186344));
#215179=CARTESIAN_POINT('Ctrl Pts',(4.16278587431589,5.33511975166407,128.591911731346));
#215180=CARTESIAN_POINT('Ctrl Pts',(4.01614535740256,5.44953762807983,128.600660762));
#215181=CARTESIAN_POINT('Ctrl Pts',(3.86478496657733,5.55790617532915,128.609409792653));
#215182=CARTESIAN_POINT('Ctrl Pts',(3.70921874747008,5.65985735539479,128.618158823307));
#215183=CARTESIAN_POINT('Ctrl Pts',(3.55365041605714,5.76180991977161,128.626907972757));
#215184=CARTESIAN_POINT('Ctrl Pts',(3.39387638174338,5.8573447855292,128.635657122206));
#215185=CARTESIAN_POINT('Ctrl Pts',(3.23043927904357,5.94613749121331,128.644406271656));
#215186=CARTESIAN_POINT('Ctrl Pts',(3.1869176707031,5.96978206944211,128.646736079572));
#215187=CARTESIAN_POINT('Ctrl Pts',(3.14313645919572,5.99294880633455,128.649065887488));
#215188=CARTESIAN_POINT('Ctrl Pts',(3.09910619832143,6.01563211736935,128.651395695404));
#215189=CARTESIAN_POINT('Origin',(0.,0.,4.30282021618968));
#215190=CARTESIAN_POINT('',(3.09910619832127,6.01563211736944,131.045783168526));
#215191=CARTESIAN_POINT('',(3.0991061983213,6.01563211736942,130.651283639301));
#215192=CARTESIAN_POINT('',(3.09910619832133,6.0156321173694,4.30282021618968));
#215193=CARTESIAN_POINT('',(-6.76699967917944,-0.00208374312542183,129.697179783778));
#215194=CARTESIAN_POINT('Ctrl Pts',(-6.76699967917923,-0.00208374379854805,
129.69717978381));
#215195=CARTESIAN_POINT('Ctrl Pts',(-6.766929895115,-0.228708888680955,
129.707858586294));
#215196=CARTESIAN_POINT('Ctrl Pts',(-6.7554715143949,-0.455087020649597,
129.718537388777));
#215197=CARTESIAN_POINT('Ctrl Pts',(-6.7327234342321,-0.680238309816426,
129.729216191261));
#215198=CARTESIAN_POINT('Ctrl Pts',(-6.72906175718189,-0.716480107034841,
129.730935119878));
#215199=CARTESIAN_POINT('Ctrl Pts',(-6.72510766844374,-0.75269014195336,
129.732654048496));
#215200=CARTESIAN_POINT('Ctrl Pts',(-6.72086170282627,-0.788864355566378,
129.734372977113));
#215201=CARTESIAN_POINT('Ctrl Pts',(-6.70031948464487,-0.963877216132726,
129.742689249517));
#215202=CARTESIAN_POINT('Ctrl Pts',(-6.67291698920661,-1.13825686304642,
129.751005521921));
#215203=CARTESIAN_POINT('Ctrl Pts',(-6.63870684167096,-1.31143450860163,
129.759321794325));
#215204=CARTESIAN_POINT('Ctrl Pts',(-6.60452561885537,-1.48446573225344,
129.767631035311));
#215205=CARTESIAN_POINT('Ctrl Pts',(-6.56354827886101,-1.65629663975404,
129.775940276297));
#215206=CARTESIAN_POINT('Ctrl Pts',(-6.5158790831247,-1.82636490715793,
129.784249517283));
#215207=CARTESIAN_POINT('Ctrl Pts',(-6.46824145177365,-1.99632056304762,
129.792553256265));
#215208=CARTESIAN_POINT('Ctrl Pts',(-6.41392088762249,-2.1645155705911,
129.800856995247));
#215209=CARTESIAN_POINT('Ctrl Pts',(-6.35307248181565,-2.33039890164683,
129.80916073423));
#215210=CARTESIAN_POINT('Ctrl Pts',(-6.29225321569742,-2.49620279284627,
129.817460496635));
#215211=CARTESIAN_POINT('Ctrl Pts',(-6.22491245751344,-2.659696887782,129.825760259041));
#215212=CARTESIAN_POINT('Ctrl Pts',(-6.15125486270707,-2.82034618691086,
129.834060021446));
#215213=CARTESIAN_POINT('Ctrl Pts',(-6.07761904748579,-2.98094798414818,
129.842357329721));
#215214=CARTESIAN_POINT('Ctrl Pts',(-5.9976702635514,-3.13870634635862,
129.850654637995));
#215215=CARTESIAN_POINT('Ctrl Pts',(-5.91166101819438,-3.29310689258047,
129.85895194627));
#215216=CARTESIAN_POINT('Ctrl Pts',(-5.82564308285061,-3.44752303873809,
129.867250092867));
#215217=CARTESIAN_POINT('Ctrl Pts',(-5.73356362529532,-3.59858038339801,
129.875548239464));
#215218=CARTESIAN_POINT('Ctrl Pts',(-5.63572105690231,-3.74578925845915,
129.883846386061));
#215219=CARTESIAN_POINT('Ctrl Pts',(-5.53786864982352,-3.89301293629877,
129.892145367089));
#215220=CARTESIAN_POINT('Ctrl Pts',(-5.43425216905738,-4.03638708295056,
129.900444348117));
#215221=CARTESIAN_POINT('Ctrl Pts',(-5.32521324676965,-4.17545121830312,
129.908743329145));
#215222=CARTESIAN_POINT('Ctrl Pts',(-5.21614523889757,-4.31455244831467,
129.917044523884));
#215223=CARTESIAN_POINT('Ctrl Pts',(-5.10165212143132,-4.44934110171576,
129.925345718624));
#215224=CARTESIAN_POINT('Ctrl Pts',(-4.98211578975548,-4.57938983462526,
129.933646913363));
#215225=CARTESIAN_POINT('Ctrl Pts',(-4.86252770444059,-4.70949487255171,
129.941951702132));
#215226=CARTESIAN_POINT('Ctrl Pts',(-4.7378922885946,-4.83485564394035,
129.9502564909));
#215227=CARTESIAN_POINT('Ctrl Pts',(-4.60862837475821,-4.95508158392711,
129.958561279669));
#215228=CARTESIAN_POINT('Ctrl Pts',(-4.47921121971277,-5.07545005068607,
129.96687591369));
#215229=CARTESIAN_POINT('Ctrl Pts',(-4.34515485875983,-5.19067128645063,
129.975190547711));
#215230=CARTESIAN_POINT('Ctrl Pts',(-4.20691220275123,-5.30039420405151,
129.983505181732));
#215231=CARTESIAN_POINT('Ctrl Pts',(-4.06858213468563,-5.41018650042595,
129.991825073169));
#215232=CARTESIAN_POINT('Ctrl Pts',(-3.92606077318695,-5.51447334014883,
130.000144964607));
#215233=CARTESIAN_POINT('Ctrl Pts',(-3.77983021009384,-5.6129468715517,
130.008464856045));
#215234=CARTESIAN_POINT('Ctrl Pts',(-3.63338098489388,-5.7115676528139,
130.016797188418));
#215235=CARTESIAN_POINT('Ctrl Pts',(-3.48321176947096,-5.80435757049047,
130.025129520791));
#215236=CARTESIAN_POINT('Ctrl Pts',(-3.32983063984619,-5.89105397275747,
130.033461853164));
#215237=CARTESIAN_POINT('Ctrl Pts',(-3.21435234070656,-5.95632636382545,
130.039735138363));
#215238=CARTESIAN_POINT('Ctrl Pts',(-3.09705393676772,-6.01814568291422,
130.046008423563));
#215239=CARTESIAN_POINT('Ctrl Pts',(-2.97815948344666,-6.07641794901871,
130.052281708762));
#215240=CARTESIAN_POINT('Ctrl Pts',(-2.82521570702387,-6.15137838821319,
130.060351554765));
#215241=CARTESIAN_POINT('Ctrl Pts',(-2.6691574779838,-6.22069900745924,
130.068421400769));
#215242=CARTESIAN_POINT('Ctrl Pts',(-2.51044765573,-6.28410228814265,130.076491246772));
#215243=CARTESIAN_POINT('Ctrl Pts',(-2.35193751061973,-6.34742579943437,
130.084550939882));
#215244=CARTESIAN_POINT('Ctrl Pts',(-2.19078275215329,-6.40484664854533,
130.092610632993));
#215245=CARTESIAN_POINT('Ctrl Pts',(-2.02747193673638,-6.45613247585166,
130.100670326104));
#215246=CARTESIAN_POINT('Ctrl Pts',(-1.86433074554019,-6.50736503468052,
130.108721647943));
#215247=CARTESIAN_POINT('Ctrl Pts',(-1.69903830676271,-6.55247514160329,
130.116772969782));
#215248=CARTESIAN_POINT('Ctrl Pts',(-1.53210422535143,-6.59127799767695,
130.124824291621));
#215249=CARTESIAN_POINT('Ctrl Pts',(-1.3653069505528,-6.63004905384939,
130.132869015203));
#215250=CARTESIAN_POINT('Ctrl Pts',(-1.19687107238559,-6.66252306300127,
130.140913738784));
#215251=CARTESIAN_POINT('Ctrl Pts',(-1.02732237117795,-6.68856469996944,
130.148958462366));
#215252=CARTESIAN_POINT('Ctrl Pts',(-0.857875505044011,-6.71459069569708,
130.156998354091));
#215253=CARTESIAN_POINT('Ctrl Pts',(-0.687317514268115,-6.73419195365595,
130.165038245816));
#215254=CARTESIAN_POINT('Ctrl Pts',(-0.516185308803933,-6.74728402596,130.173078137541));
#215255=CARTESIAN_POINT('Ctrl Pts',(-0.341368158127535,-6.7606580064474,
130.18129115016));
#215256=CARTESIAN_POINT('Ctrl Pts',(-0.165952171610317,-6.76723920980045,
130.18950416278));
#215257=CARTESIAN_POINT('Ctrl Pts',(0.00948324521950484,-6.76699335510684,
130.197717175399));
#215258=CARTESIAN_POINT('Ctrl Pts',(0.18116076394389,-6.76675276672093,
130.205754261942));
#215259=CARTESIAN_POINT('Ctrl Pts',(0.352856500310551,-6.75997464784988,
130.213791348486));
#215260=CARTESIAN_POINT('Ctrl Pts',(0.524026562454356,-6.74667956567097,
130.221828435029));
#215261=CARTESIAN_POINT('Ctrl Pts',(0.695213006369794,-6.73338321109083,
130.229866290758));
#215262=CARTESIAN_POINT('Ctrl Pts',(0.865873303362873,-6.7135686801116,
130.237904146488));
#215263=CARTESIAN_POINT('Ctrl Pts',(1.03546812106564,-6.68730848475355,
130.245942002218));
#215264=CARTESIAN_POINT('Ctrl Pts',(1.20511277217761,-6.66104057315111,
130.253982219775));
#215265=CARTESIAN_POINT('Ctrl Pts',(1.37369095181014,-6.62832328440613,
130.262022437333));
#215266=CARTESIAN_POINT('Ctrl Pts',(1.54067311238569,-6.58928033709083,
130.27006265489));
#215267=CARTESIAN_POINT('Ctrl Pts',(1.71396396594366,-6.54876232221805,
130.278406637017));
#215268=CARTESIAN_POINT('Ctrl Pts',(1.88553541427208,-6.5014314391498,130.286750619144));
#215269=CARTESIAN_POINT('Ctrl Pts',(2.05481349248203,-6.44748249405253,
130.29509460127));
#215270=CARTESIAN_POINT('Ctrl Pts',(2.21821293271889,-6.39540707162642,
130.303148816106));
#215271=CARTESIAN_POINT('Ctrl Pts',(2.37947529598631,-6.33716572883949,
130.311203030942));
#215272=CARTESIAN_POINT('Ctrl Pts',(2.53810585416862,-6.27298235873775,
130.319257245777));
#215273=CARTESIAN_POINT('Ctrl Pts',(2.6968551210923,-6.20875095799696,130.327317487861));
#215274=CARTESIAN_POINT('Ctrl Pts',(2.85296832305128,-6.13856882827507,
130.335377729944));
#215275=CARTESIAN_POINT('Ctrl Pts',(3.0059757622498,-6.06270556078445,130.343437972028));
#215276=CARTESIAN_POINT('Ctrl Pts',(3.15919711634376,-5.98673623124209,
130.351509482883));
#215277=CARTESIAN_POINT('Ctrl Pts',(3.30930371942944,-5.90507009388891,
130.359580993738));
#215278=CARTESIAN_POINT('Ctrl Pts',(3.45585475290609,-5.8180200177394,130.367652504592));
#215279=CARTESIAN_POINT('Ctrl Pts',(3.47121483124572,-5.80889626093328,
130.368498483199));
#215280=CARTESIAN_POINT('Ctrl Pts',(3.48653588109474,-5.79971339654704,
130.369344461805));
#215281=CARTESIAN_POINT('Ctrl Pts',(3.50181741651349,-5.79047180991349,
130.370190440411));
#215282=CARTESIAN_POINT('Ctrl Pts',(3.65046842301036,-5.70057435412382,
130.378419690146));
#215283=CARTESIAN_POINT('Ctrl Pts',(3.7958739130941,-5.60481694627283,130.386648939882));
#215284=CARTESIAN_POINT('Ctrl Pts',(3.93754041277494,-5.5034593209875,130.394878189617));
#215285=CARTESIAN_POINT('Ctrl Pts',(4.07903830627505,-5.40222232776499,
130.403097645206));
#215286=CARTESIAN_POINT('Ctrl Pts',(4.21680578145831,-5.29539859547242,
130.411317100796));
#215287=CARTESIAN_POINT('Ctrl Pts',(4.35037474427182,-5.18329321806146,
130.419536556385));
#215288=CARTESIAN_POINT('Ctrl Pts',(4.48381156222443,-5.07129875076907,
130.427747880154));
#215289=CARTESIAN_POINT('Ctrl Pts',(4.61305786707213,-4.95403327344411,
130.435959203923));
#215290=CARTESIAN_POINT('Ctrl Pts',(4.73767523971573,-4.83184460873738,
130.444170527692));
#215291=CARTESIAN_POINT('Ctrl Pts',(4.86219434083499,-4.70975230030975,
130.452375376125));
#215292=CARTESIAN_POINT('Ctrl Pts',(4.98209152537206,-4.58274478719232,
130.460580224558));
#215293=CARTESIAN_POINT('Ctrl Pts',(5.09696206426688,-4.45120957891497,
130.468785072992));
#215294=CARTESIAN_POINT('Ctrl Pts',(5.21176507239897,-4.31975169832341,
130.476985097911));
#215295=CARTESIAN_POINT('Ctrl Pts',(5.32154708645066,-4.18377169449091,
130.48518512283));
#215296=CARTESIAN_POINT('Ctrl Pts',(5.42594076321777,-4.0436933407532,130.493385147749));
#215297=CARTESIAN_POINT('Ctrl Pts',(5.53030422608991,-3.90365552886437,
130.501582799396));
#215298=CARTESIAN_POINT('Ctrl Pts',(5.62928224079385,-3.75952201458261,
130.509780451042));
#215299=CARTESIAN_POINT('Ctrl Pts',(5.72254809659069,-3.61174919979313,
130.517978102688));
#215300=CARTESIAN_POINT('Ctrl Pts',(5.81580146351725,-3.46399617269014,
130.526174656619));
#215301=CARTESIAN_POINT('Ctrl Pts',(5.90334400279473,-3.31260511847879,
130.534371210549));
#215302=CARTESIAN_POINT('Ctrl Pts',(5.98489265618446,-3.1580609389227,130.542567764479));
#215303=CARTESIAN_POINT('Ctrl Pts',(6.06644521737349,-3.00350935363261,
130.550764711187));
#215304=CARTESIAN_POINT('Ctrl Pts',(6.14200315296424,-2.8458046592573,130.558961657895));
#215305=CARTESIAN_POINT('Ctrl Pts',(6.21132962421336,-2.68545588296838,
130.567158604603));
#215306=CARTESIAN_POINT('Ctrl Pts',(6.28067202290252,-2.5250702672807,130.575357434522));
#215307=CARTESIAN_POINT('Ctrl Pts',(6.34377996349516,-2.36203968901357,
130.583556264442));
#215308=CARTESIAN_POINT('Ctrl Pts',(6.40046494410733,-2.19689269179294,
130.591755094361));
#215309=CARTESIAN_POINT('Ctrl Pts',(6.45720361264282,-2.03158927925332,
130.59996168962));
#215310=CARTESIAN_POINT('Ctrl Pts',(6.50750705057403,-1.86416578267499,
130.608168284879));
#215311=CARTESIAN_POINT('Ctrl Pts',(6.55123653024521,-1.69516634133078,
130.616374880138));
#215312=CARTESIAN_POINT('Ctrl Pts',(6.59498717523529,-1.5260851032879,130.624585447437));
#215313=CARTESIAN_POINT('Ctrl Pts',(6.63215744184712,-1.35542675002679,
130.632796014735));
#215314=CARTESIAN_POINT('Ctrl Pts',(6.66265988019255,-1.18374504048491,
130.641006582033));
#215315=CARTESIAN_POINT('Ctrl Pts',(6.69320438576726,-1.01182655728721,
130.649228472879));
#215316=CARTESIAN_POINT('Ctrl Pts',(6.71706263598801,-0.838882252680426,
130.657450363725));
#215317=CARTESIAN_POINT('Ctrl Pts',(6.73419902221055,-0.665471659245134,
130.665672254571));
#215318=CARTESIAN_POINT('Ctrl Pts',(6.74978004151143,-0.507800504533539,
130.673147893735));
#215319=CARTESIAN_POINT('Ctrl Pts',(6.75980467048279,-0.349744100864699,
130.680623532898));
#215320=CARTESIAN_POINT('Ctrl Pts',(6.76428353672316,-0.191721764064525,
130.688099172061));
#215321=CARTESIAN_POINT('Ctrl Pts',(6.76963731244371,-0.00283107060319224,
130.697035115512));
#215322=CARTESIAN_POINT('Ctrl Pts',(6.76707809647515,0.186404318632308,
130.705971058963));
#215323=CARTESIAN_POINT('Ctrl Pts',(6.75658311908621,0.375331260194678,
130.714907002414));
#215324=CARTESIAN_POINT('Ctrl Pts',(6.74610391843197,0.563974194452848,
130.723829512771));
#215325=CARTESIAN_POINT('Ctrl Pts',(6.72771277420276,0.752309349020713,
130.732752023129));
#215326=CARTESIAN_POINT('Ctrl Pts',(6.70143889179924,0.939683872097727,
130.741674533487));
#215327=CARTESIAN_POINT('Ctrl Pts',(6.67522938856135,1.12659926944415,130.750575180925));
#215328=CARTESIAN_POINT('Ctrl Pts',(6.64117573255837,1.3125584779172,130.759475828363));
#215329=CARTESIAN_POINT('Ctrl Pts',(6.59935871645636,1.4969146707583,130.768376475802));
#215330=CARTESIAN_POINT('Ctrl Pts',(6.55760632339184,1.6809859638559,130.777263368388));
#215331=CARTESIAN_POINT('Ctrl Pts',(6.50811455855815,1.86345893226053,130.786150260974));
#215332=CARTESIAN_POINT('Ctrl Pts',(6.45101544745625,2.04369486388767,130.79503715356));
#215333=CARTESIAN_POINT('Ctrl Pts',(6.39406310238482,2.22346752188896,130.803901203515));
#215334=CARTESIAN_POINT('Ctrl Pts',(6.32954250688506,2.40101437146873,130.81276525347));
#215335=CARTESIAN_POINT('Ctrl Pts',(6.25763565836037,2.57571057520381,130.821629303425));
#215336=CARTESIAN_POINT('Ctrl Pts',(6.18888692666369,2.74273419931505,130.830104048245));
#215337=CARTESIAN_POINT('Ctrl Pts',(6.11338685668269,2.9071519374485,130.838578793066));
#215338=CARTESIAN_POINT('Ctrl Pts',(6.03133770514296,3.06842866733461,130.847053537886));
#215339=CARTESIAN_POINT('Ctrl Pts',(5.95186221903356,3.22464657166756,130.855262452319));
#215340=CARTESIAN_POINT('Ctrl Pts',(5.86631780649796,3.37776640094225,130.863471366751));
#215341=CARTESIAN_POINT('Ctrl Pts',(5.77498525549678,3.52729844198003,130.871680281184));
#215342=CARTESIAN_POINT('Ctrl Pts',(5.68363099064509,3.67686603350175,130.879891147244));
#215343=CARTESIAN_POINT('Ctrl Pts',(5.58648603136028,3.82284383352606,130.888102013305));
#215344=CARTESIAN_POINT('Ctrl Pts',(5.48387501293507,3.96477033918818,130.896312879365));
#215345=CARTESIAN_POINT('Ctrl Pts',(5.38122130841649,4.10675588615177,130.904527161138));
#215346=CARTESIAN_POINT('Ctrl Pts',(5.27309722317379,4.24468649288527,130.912741442912));
#215347=CARTESIAN_POINT('Ctrl Pts',(5.15986829629692,4.37813295422489,130.920955724685));
#215348=CARTESIAN_POINT('Ctrl Pts',(5.04651192132337,4.5117296200924,130.929179252281));
#215349=CARTESIAN_POINT('Ctrl Pts',(4.92803945872198,4.64083178790609,130.937402779877));
#215350=CARTESIAN_POINT('Ctrl Pts',(4.80485466955577,4.76504570853713,130.945626307473));
#215351=CARTESIAN_POINT('Ctrl Pts',(4.68159092373097,4.88933924546,130.953855106031));
#215352=CARTESIAN_POINT('Ctrl Pts',(4.55360909002018,5.00873804713577,130.962083904588));
#215353=CARTESIAN_POINT('Ctrl Pts',(4.42134670437477,5.12288808385605,130.970312703145));
#215354=CARTESIAN_POINT('Ctrl Pts',(4.28890227013917,5.23719523896758,130.978552827985));
#215355=CARTESIAN_POINT('Ctrl Pts',(4.15216579314281,5.34623897747476,130.986792952826));
#215356=CARTESIAN_POINT('Ctrl Pts',(4.01160532518633,5.4497074889334,130.995033077666));
#215357=CARTESIAN_POINT('Ctrl Pts',(3.94920227852705,5.49564323774093,130.998691353014));
#215358=CARTESIAN_POINT('Ctrl Pts',(3.88604587658117,5.54048070588965,131.002349628362));
#215359=CARTESIAN_POINT('Ctrl Pts',(3.82217864206139,5.58419550411424,131.006007903711));
#215360=CARTESIAN_POINT('Ctrl Pts',(3.67469067372378,5.68514565210346,131.014455922524));
#215361=CARTESIAN_POINT('Ctrl Pts',(3.5230728080901,5.78033677462241,131.022903941336));
#215362=CARTESIAN_POINT('Ctrl Pts',(3.3678025770459,5.86942883098884,131.031351960149));
#215363=CARTESIAN_POINT('Ctrl Pts',(3.27938985336079,5.92015891175893,131.036162362942));
#215364=CARTESIAN_POINT('Ctrl Pts',(3.1897935246329,5.96891222998303,131.040972765734));
#215365=CARTESIAN_POINT('Ctrl Pts',(3.09910619832127,6.01563211736944,131.045783168526));
#215366=CARTESIAN_POINT('Ctrl Pts',(3.09910619832118,6.01563211736948,129.045766611327));
#215367=CARTESIAN_POINT('Ctrl Pts',(2.93295980831911,6.10122666454888,129.054564761741));
#215368=CARTESIAN_POINT('Ctrl Pts',(2.76334723714547,6.17989107528915,129.063362912156));
#215369=CARTESIAN_POINT('Ctrl Pts',(2.59088386661367,6.25136863332511,129.07216106257));
#215370=CARTESIAN_POINT('Ctrl Pts',(2.41842049608198,6.32284619136102,129.080959212985));
#215371=CARTESIAN_POINT('Ctrl Pts',(2.24310672167691,6.38713678290893,129.089757363399));
#215372=CARTESIAN_POINT('Ctrl Pts',(2.06557696693954,6.44404227124938,129.098555513813));
#215373=CARTESIAN_POINT('Ctrl Pts',(1.90133317189418,6.49668907052971,129.106695228846));
#215374=CARTESIAN_POINT('Ctrl Pts',(1.73486519293263,6.54311981293916,129.114834943879));
#215375=CARTESIAN_POINT('Ctrl Pts',(1.56668894480396,6.58314322723037,129.122974658912));
#215376=CARTESIAN_POINT('Ctrl Pts',(1.39865978261292,6.62313163728356,129.131107254999));
#215377=CARTESIAN_POINT('Ctrl Pts',(1.22892567895543,6.65672378936519,129.139239851086));
#215378=CARTESIAN_POINT('Ctrl Pts',(1.05801921841487,6.6837776992854,129.147372447173));
#215379=CARTESIAN_POINT('Ctrl Pts',(0.887229598699516,6.7108131137014,129.155499483381));
#215380=CARTESIAN_POINT('Ctrl Pts',(0.715269578040404,6.73131912826273,
129.16362651959));
#215381=CARTESIAN_POINT('Ctrl Pts',(0.542683447704755,6.74520449471973,
129.171753555798));
#215382=CARTESIAN_POINT('Ctrl Pts',(0.370179816662838,6.75908322372027,
129.179876707135));
#215383=CARTESIAN_POINT('Ctrl Pts',(0.197051036185945,6.76634757744501,
129.187999858473));
#215384=CARTESIAN_POINT('Ctrl Pts',(0.023848042362166,6.76695797762004,
129.196123009811));
#215385=CARTESIAN_POINT('Ctrl Pts',(-0.149306280132994,6.76756820626809,
129.204243878482));
#215386=CARTESIAN_POINT('Ctrl Pts',(-0.322534408546306,6.76152820516158,
129.212364747154));
#215387=CARTESIAN_POINT('Ctrl Pts',(-0.495283907157348,6.74885048369802,
129.220485615826));
#215388=CARTESIAN_POINT('Ctrl Pts',(-0.668042741812549,6.73617207708186,
129.228606923381));
#215389=CARTESIAN_POINT('Ctrl Pts',(-0.840322529454317,6.71685525627807,
129.236728230935));
#215390=CARTESIAN_POINT('Ctrl Pts',(-1.0115742687147,6.69096454174391,129.24484953849));
#215391=CARTESIAN_POINT('Ctrl Pts',(-1.10056262544168,6.67751082646585,
129.249069652206));
#215392=CARTESIAN_POINT('Ctrl Pts',(-1.18927348003949,6.66228287926408,
129.253289765922));
#215393=CARTESIAN_POINT('Ctrl Pts',(-1.27763067473819,6.64529524242287,
129.257509879638));
#215394=CARTESIAN_POINT('Ctrl Pts',(-1.46573929868794,6.60912930255511,
129.266494318163));
#215395=CARTESIAN_POINT('Ctrl Pts',(-1.65215115647333,6.56500276800371,
129.275478756689));
#215396=CARTESIAN_POINT('Ctrl Pts',(-1.83622366294872,6.51310768064118,
129.284463195214));
#215397=CARTESIAN_POINT('Ctrl Pts',(-2.02061386758355,6.46112302545534,
129.293463140344));
#215398=CARTESIAN_POINT('Ctrl Pts',(-2.20265642084614,6.40134308321685,
129.302463085474));
#215399=CARTESIAN_POINT('Ctrl Pts',(-2.38172547904874,6.33400921553245,
129.311463030604));
#215400=CARTESIAN_POINT('Ctrl Pts',(-2.56121651808352,6.26651667386047,
129.320484184336));
#215401=CARTESIAN_POINT('Ctrl Pts',(-2.73771981737689,6.19143467424104,
129.329505338068));
#215402=CARTESIAN_POINT('Ctrl Pts',(-2.91062850105638,6.10905317777136,
129.3385264918));
#215403=CARTESIAN_POINT('Ctrl Pts',(-3.08371312068443,6.02658785747966,
129.347556824627));
#215404=CARTESIAN_POINT('Ctrl Pts',(-3.25319560486031,5.9368083105328,129.356587157453));
#215405=CARTESIAN_POINT('Ctrl Pts',(-3.41849375635632,5.84005046534299,
129.36561749028));
#215406=CARTESIAN_POINT('Ctrl Pts',(-3.58402624852605,5.7431554480286,129.374660625272));
#215407=CARTESIAN_POINT('Ctrl Pts',(-3.74536234037392,5.63926247190385,
129.383703760265));
#215408=CARTESIAN_POINT('Ctrl Pts',(-3.9019469282076,5.5287520444899,129.392746895257));
#215409=CARTESIAN_POINT('Ctrl Pts',(-4.03883793299568,5.43214047078686,
129.400652678659));
#215410=CARTESIAN_POINT('Ctrl Pts',(-4.17209783550899,5.33047203388531,
129.408558462061));
#215411=CARTESIAN_POINT('Ctrl Pts',(-4.30137593202846,5.2240266166403,129.416464245463));
#215412=CARTESIAN_POINT('Ctrl Pts',(-4.44287912048788,5.10751526365335,
129.425117633692));
#215413=CARTESIAN_POINT('Ctrl Pts',(-4.57973600641257,4.9851768166606,129.433771021921));
#215414=CARTESIAN_POINT('Ctrl Pts',(-4.71147028346091,4.85740020670161,
129.442424410149));
#215415=CARTESIAN_POINT('Ctrl Pts',(-4.8430828945598,4.72974160750577,129.45106980636));
#215416=CARTESIAN_POINT('Ctrl Pts',(-4.96958211557801,4.59665507382547,
129.459715202571));
#215417=CARTESIAN_POINT('Ctrl Pts',(-5.09052595749893,4.45856865776783,
129.468360598782));
#215418=CARTESIAN_POINT('Ctrl Pts',(-5.21533233830668,4.31607222675371,
129.477282099824));
#215419=CARTESIAN_POINT('Ctrl Pts',(-5.33422236960563,4.16825146843598,
129.486203600867));
#215420=CARTESIAN_POINT('Ctrl Pts',(-5.44675115624527,4.01561836358248,
129.495125101909));
#215421=CARTESIAN_POINT('Ctrl Pts',(-5.5555896865386,3.86799069156676,129.503754032251));
#215422=CARTESIAN_POINT('Ctrl Pts',(-5.65847736139182,3.71586155715784,
129.512382962594));
#215423=CARTESIAN_POINT('Ctrl Pts',(-5.75505186027942,3.55972851289174,
129.521011892936));
#215424=CARTESIAN_POINT('Ctrl Pts',(-5.85653801117727,3.39565474732168,
129.530079679328));
#215425=CARTESIAN_POINT('Ctrl Pts',(-5.95105186775873,3.22715944719311,
129.53914746572));
#215426=CARTESIAN_POINT('Ctrl Pts',(-6.03822362058705,3.05485588985547,
129.548215252112));
#215427=CARTESIAN_POINT('Ctrl Pts',(-6.12539537341537,2.88255233251783,
129.557283038504));
#215428=CARTESIAN_POINT('Ctrl Pts',(-6.20522481478602,2.70644085053473,
129.566350824896));
#215429=CARTESIAN_POINT('Ctrl Pts',(-6.27739733281653,2.52716673884965,
129.575418611288));
#215430=CARTESIAN_POINT('Ctrl Pts',(-6.34226712862127,2.36603234399354,
129.5835688805));
#215431=CARTESIAN_POINT('Ctrl Pts',(-6.40093863369382,2.2023738437227,129.591719149711));
#215432=CARTESIAN_POINT('Ctrl Pts',(-6.45322294622245,2.03671367804805,
129.599869418923));
#215433=CARTESIAN_POINT('Ctrl Pts',(-6.50552745197575,1.87098953117558,
129.608022835928));
#215434=CARTESIAN_POINT('Ctrl Pts',(-6.55143972202865,1.70326251997774,
129.616176252934));
#215435=CARTESIAN_POINT('Ctrl Pts',(-6.59082053962587,1.53407092875321,
129.624329669939));
#215436=CARTESIAN_POINT('Ctrl Pts',(-6.63020804405421,1.36485060893274,
129.632484471388));
#215437=CARTESIAN_POINT('Ctrl Pts',(-6.66306181120303,1.19416556972321,
129.640639272837));
#215438=CARTESIAN_POINT('Ctrl Pts',(-6.68929377653724,1.02256431151308,
129.648794074286));
#215439=CARTESIAN_POINT('Ctrl Pts',(-6.71554965728286,0.850806606211075,
129.656956310383));
#215440=CARTESIAN_POINT('Ctrl Pts',(-6.73517162464069,0.678131373831475,
129.66511854648));
#215441=CARTESIAN_POINT('Ctrl Pts',(-6.74812343557283,0.505093158014219,
129.673280782577));
#215442=CARTESIAN_POINT('Ctrl Pts',(-6.76076438924186,0.336208043756621,
129.681247116311));
#215443=CARTESIAN_POINT('Ctrl Pts',(-6.76705173772872,0.166977491905592,
129.689213450045));
#215444=CARTESIAN_POINT('Ctrl Pts',(-6.76699967917944,-0.00208374312541649,
129.697179783778));
#215445=CARTESIAN_POINT('',(-6.767,6.94095388803495E-12,129.30282021619));
#215446=CARTESIAN_POINT('Ctrl Pts',(3.09910619832143,6.01563211736935,128.651395695404));
#215447=CARTESIAN_POINT('Ctrl Pts',(2.93375330764824,6.10081787314654,128.660145143307));
#215448=CARTESIAN_POINT('Ctrl Pts',(2.76488627843057,6.17918207037046,128.668894591209));
#215449=CARTESIAN_POINT('Ctrl Pts',(2.59307866646676,6.25045854554008,128.677644039111));
#215450=CARTESIAN_POINT('Ctrl Pts',(2.42127244185333,6.32173444515054,128.686393416362));
#215451=CARTESIAN_POINT('Ctrl Pts',(2.24652594672404,6.3859226274186,128.695142793612));
#215452=CARTESIAN_POINT('Ctrl Pts',(2.06943269687042,6.44280508110587,128.703892170862));
#215453=CARTESIAN_POINT('Ctrl Pts',(1.89234081821986,6.49968709436193,128.712641480368));
#215454=CARTESIAN_POINT('Ctrl Pts',(1.71290249405485,6.54926340459572,128.721390789873));
#215455=CARTESIAN_POINT('Ctrl Pts',(1.53172716624943,6.59136563150411,128.730140099378));
#215456=CARTESIAN_POINT('Ctrl Pts',(1.3505531810721,6.63346754640735,128.738889344046));
#215457=CARTESIAN_POINT('Ctrl Pts',(1.16764249714286,6.66809542395799,128.747638588713));
#215458=CARTESIAN_POINT('Ctrl Pts',(0.983616340612941,6.69513165624689,
128.75638783338));
#215459=CARTESIAN_POINT('Ctrl Pts',(0.799591486712297,6.7221676971598,128.765137016116));
#215460=CARTESIAN_POINT('Ctrl Pts',(0.614451459525037,6.74161215869387,
128.773886198851));
#215461=CARTESIAN_POINT('Ctrl Pts',(0.428825047908479,6.75339900185724,
128.782635381587));
#215462=CARTESIAN_POINT('Ctrl Pts',(0.243199888595149,6.76518576550228,
128.791384505298));
#215463=CARTESIAN_POINT('Ctrl Pts',(0.0570886373899296,6.76931499599836,
128.800133629008));
#215464=CARTESIAN_POINT('Ctrl Pts',(-0.128876626813226,6.76577266947843,
128.808882752719));
#215465=CARTESIAN_POINT('Ctrl Pts',(-0.314840698190301,6.76223036567983,
128.81763182031));
#215466=CARTESIAN_POINT('Ctrl Pts',(-0.50065849795346,6.75101660879207,
128.826380887902));
#215467=CARTESIAN_POINT('Ctrl Pts',(-0.685698951928485,6.73216948296195,
128.835129955493));
#215468=CARTESIAN_POINT('Ctrl Pts',(-0.870738280462148,6.71332247176263,
128.843878969872));
#215469=CARTESIAN_POINT('Ctrl Pts',(-1.05499998761483,6.6868422135615,128.852627984251));
#215470=CARTESIAN_POINT('Ctrl Pts',(-1.23785829161654,6.65281863948479,
128.861376998629));
#215471=CARTESIAN_POINT('Ctrl Pts',(-1.4300741291762,6.61705395368814,128.870573732328));
#215472=CARTESIAN_POINT('Ctrl Pts',(-1.6207388253599,6.5729537272774,128.879770466027));
#215473=CARTESIAN_POINT('Ctrl Pts',(-1.80913696091694,6.52068343478229,
128.888967199727));
#215474=CARTESIAN_POINT('Ctrl Pts',(-1.98838356186291,6.47095219815144,
128.89771719744));
#215475=CARTESIAN_POINT('Ctrl Pts',(-2.1655782757271,6.41382586850831,128.906467195154));
#215476=CARTESIAN_POINT('Ctrl Pts',(-2.34011918621875,6.34949849943213,
128.915217192868));
#215477=CARTESIAN_POINT('Ctrl Pts',(-2.51465655691265,6.28517243495484,
128.923967013126));
#215478=CARTESIAN_POINT('Ctrl Pts',(-2.68653996295486,6.21364572242306,
128.932716833384));
#215479=CARTESIAN_POINT('Ctrl Pts',(-2.85518555380138,6.13516132252151,
128.941466653642));
#215480=CARTESIAN_POINT('Ctrl Pts',(-3.02382794858838,6.05667841000432,
128.95021630808));
#215481=CARTESIAN_POINT('Ctrl Pts',(-3.18923239109429,5.97123819492002,
128.958965962518));
#215482=CARTESIAN_POINT('Ctrl Pts',(-3.35083705967845,5.87913088810629,
128.967715616955));
#215483=CARTESIAN_POINT('Ctrl Pts',(-3.5124388804254,5.78702520443018,128.976465117204));
#215484=CARTESIAN_POINT('Ctrl Pts',(-3.67024081223823,5.68825280605697,
128.985214617453));
#215485=CARTESIAN_POINT('Ctrl Pts',(-3.82370687544528,5.58314917682418,
128.993964117702));
#215486=CARTESIAN_POINT('Ctrl Pts',(-3.97717043817946,5.47804726007926,
129.002713475392));
#215487=CARTESIAN_POINT('Ctrl Pts',(-4.12629803722595,5.36661448084132,
129.011462833083));
#215488=CARTESIAN_POINT('Ctrl Pts',(-4.27058317207046,5.24922931204464,
129.020212190773));
#215489=CARTESIAN_POINT('Ctrl Pts',(-4.41486614774964,5.13184589986679,
129.028961417533));
#215490=CARTESIAN_POINT('Ctrl Pts',(-4.55430658194534,5.00851045722925,
129.037710644293));
#215491=CARTESIAN_POINT('Ctrl Pts',(-4.68843089001957,4.87964187103012,
129.046459871053));
#215492=CARTESIAN_POINT('Ctrl Pts',(-4.82255336917943,4.75077504207853,
129.055208978509));
#215493=CARTESIAN_POINT('Ctrl Pts',(-4.95135966065236,4.61637541907985,
129.063958085965));
#215494=CARTESIAN_POINT('Ctrl Pts',(-5.0744123086934,4.47689945401736,129.072707193421));
#215495=CARTESIAN_POINT('Ctrl Pts',(-5.19746344226516,4.33742520555397,
129.081456193198));
#215496=CARTESIAN_POINT('Ctrl Pts',(-5.31476088454869,4.19287495491208,
129.090205192974));
#215497=CARTESIAN_POINT('Ctrl Pts',(-5.42590627628957,4.04373961586568,
129.09895419275));
#215498=CARTESIAN_POINT('Ctrl Pts',(-5.53706380672776,3.89458798906581,
129.107704148045));
#215499=CARTESIAN_POINT('Ctrl Pts',(-5.64206777071976,3.74085050155115,
129.11645410334));
#215500=CARTESIAN_POINT('Ctrl Pts',(-5.74056148164123,3.58304938222977,
129.125204058634));
#215501=CARTESIAN_POINT('Ctrl Pts',(-5.8390513895199,3.425254355931,129.133953676076));
#215502=CARTESIAN_POINT('Ctrl Pts',(-5.93103139557751,3.26339625497004,
129.142703293517));
#215503=CARTESIAN_POINT('Ctrl Pts',(-6.01618907820937,3.09802485064829,
129.151452910958));
#215504=CARTESIAN_POINT('Ctrl Pts',(-6.10134392545069,2.93265895249461,
129.160202237074));
#215505=CARTESIAN_POINT('Ctrl Pts',(-6.17967677261913,2.76378023985853,
129.16895156319));
#215506=CARTESIAN_POINT('Ctrl Pts',(-6.25092157009301,2.59196229226932,
129.177700889305));
#215507=CARTESIAN_POINT('Ctrl Pts',(-6.32216437407831,2.42014915228889,
129.186449970608));
#215508=CARTESIAN_POINT('Ctrl Pts',(-6.38631941548999,2.2453972066263,129.19519905191));
#215509=CARTESIAN_POINT('Ctrl Pts',(-6.44316881037614,2.06829994947446,
129.203948133213));
#215510=CARTESIAN_POINT('Ctrl Pts',(-6.5000233452464,1.89118668024214,129.212698005555));
#215511=CARTESIAN_POINT('Ctrl Pts',(-6.54957082411157,1.71172794807471,
129.221447877897));
#215512=CARTESIAN_POINT('Ctrl Pts',(-6.59164294296136,1.53053334250113,
129.23019775024));
#215513=CARTESIAN_POINT('Ctrl Pts',(-6.63371214082178,1.34935131693382,
129.238947015095));
#215514=CARTESIAN_POINT('Ctrl Pts',(-6.66830695239726,1.16643393829557,
129.24769627995));
#215515=CARTESIAN_POINT('Ctrl Pts',(-6.69530988154017,0.982402458339035,
129.256445544805));
#215516=CARTESIAN_POINT('Ctrl Pts',(-6.72231419690506,0.798361530945111,
129.265195258812));
#215517=CARTESIAN_POINT('Ctrl Pts',(-6.74172580829295,0.613206671360537,
129.273944972819));
#215518=CARTESIAN_POINT('Ctrl Pts',(-6.75347878028192,0.42756679511147,
129.282694686826));
#215519=CARTESIAN_POINT('Ctrl Pts',(-6.76248992368208,0.285234494205815,
129.289403196614));
#215520=CARTESIAN_POINT('Ctrl Pts',(-6.76699999999985,0.142617266095155,
129.296111706402));
#215521=CARTESIAN_POINT('Ctrl Pts',(-6.767,6.94095400683209E-12,129.30282021619));
#215522=CARTESIAN_POINT('Ctrl Pts',(-6.76699998027983,-0.000516616662484787,
129.30282021619));
#215523=CARTESIAN_POINT('Ctrl Pts',(-6.76698635528968,-0.17898609850718,
129.311175751275));
#215524=CARTESIAN_POINT('Ctrl Pts',(-6.75990811182994,-0.357370256202649,
129.319531286361));
#215525=CARTESIAN_POINT('Ctrl Pts',(-6.74581131082869,-0.535087617774603,
129.327886821446));
#215526=CARTESIAN_POINT('Ctrl Pts',(-6.7317049334655,-0.712925707856396,
129.336248032686));
#215527=CARTESIAN_POINT('Ctrl Pts',(-6.71057051792594,-0.890095762078785,
129.344609243927));
#215528=CARTESIAN_POINT('Ctrl Pts',(-6.68250576114816,-1.06602333568344,
129.352970455167));
#215529=CARTESIAN_POINT('Ctrl Pts',(-6.65440001357014,-1.24220786544432,
129.361343878619));
#215530=CARTESIAN_POINT('Ctrl Pts',(-6.61934375200373,-1.41714595444067,
129.36971730207));
#215531=CARTESIAN_POINT('Ctrl Pts',(-6.57748569718429,-1.59027384539146,
129.378090725522));
#215532=CARTESIAN_POINT('Ctrl Pts',(-6.53559356498376,-1.76354268281343,
129.386470965926));
#215533=CARTESIAN_POINT('Ctrl Pts',(-6.48688868596984,-1.93499805826365,
129.394851206329));
#215534=CARTESIAN_POINT('Ctrl Pts',(-6.43156917970343,-2.10409288927293,
129.403231446732));
#215535=CARTESIAN_POINT('Ctrl Pts',(-6.3761607646608,-2.27345948725024,
129.411625155747));
#215536=CARTESIAN_POINT('Ctrl Pts',(-6.31411659565488,-2.44045764319213,
129.420018864762));
#215537=CARTESIAN_POINT('Ctrl Pts',(-6.24568284109669,-2.60456039446783,
129.428412573776));
#215538=CARTESIAN_POINT('Ctrl Pts',(-6.21110627378886,-2.68747429947737,
129.43265354589));
#215539=CARTESIAN_POINT('Ctrl Pts',(-6.17489928125139,-2.76964944403422,
129.436894518003));
#215540=CARTESIAN_POINT('Ctrl Pts',(-6.13709797108201,-2.85102043018655,
129.441135490117));
#215541=CARTESIAN_POINT('Ctrl Pts',(-6.06179770496057,-3.0131115557158,
129.449583512879));
#215542=CARTESIAN_POINT('Ctrl Pts',(-5.98000648310577,-3.17235838630767,
129.458031535642));
#215543=CARTESIAN_POINT('Ctrl Pts',(-5.89196137931734,-3.32822476774525,
129.466479558404));
#215544=CARTESIAN_POINT('Ctrl Pts',(-5.80399690105999,-3.48394841768227,
129.47491984506));
#215545=CARTESIAN_POINT('Ctrl Pts',(-5.7097901194528,-3.63629749987733,
129.483360131716));
#215546=CARTESIAN_POINT('Ctrl Pts',(-5.60962497276874,-3.7847584685009,
129.491800418372));
#215547=CARTESIAN_POINT('Ctrl Pts',(-5.50953613043959,-3.93310634171341,
129.500234275339));
#215548=CARTESIAN_POINT('Ctrl Pts',(-5.40349815741405,-4.07757173042906,
129.508668132307));
#215549=CARTESIAN_POINT('Ctrl Pts',(-5.29183963587732,-4.21766787077383,
129.517101989275));
#215550=CARTESIAN_POINT('Ctrl Pts',(-5.1802490085182,-4.35767882539246,
129.52553071802));
#215551=CARTESIAN_POINT('Ctrl Pts',(-5.06304485375228,-4.49332556828457,
129.533959446765));
#215552=CARTESIAN_POINT('Ctrl Pts',(-4.94059780221203,-4.62415206895034,
129.54238817551));
#215553=CARTESIAN_POINT('Ctrl Pts',(-4.81820640151364,-4.75491911040652,
129.550813073491));
#215554=CARTESIAN_POINT('Ctrl Pts',(-4.69057708295744,-4.88087003491284,
129.559237971471));
#215555=CARTESIAN_POINT('Ctrl Pts',(-4.55811957752833,-5.00158324103008,
129.567662869451));
#215556=CARTESIAN_POINT('Ctrl Pts',(-4.42569139840627,-5.12226972104723,
129.576085902145));
#215557=CARTESIAN_POINT('Ctrl Pts',(-4.2884374082191,-5.23772056838595,
129.584508934839));
#215558=CARTESIAN_POINT('Ctrl Pts',(-4.14680327068804,-5.34755192908035,
129.592931967534));
#215559=CARTESIAN_POINT('Ctrl Pts',(-4.0051851588989,-5.45737086248094,
129.601354047171));
#215560=CARTESIAN_POINT('Ctrl Pts',(-3.85918815125639,-5.5615713725011,
129.609776126809));
#215561=CARTESIAN_POINT('Ctrl Pts',(-3.70929022153916,-5.65981051382411,
129.618198206446));
#215562=CARTESIAN_POINT('Ctrl Pts',(-3.55938832797121,-5.75805225295013,
129.626620508795));
#215563=CARTESIAN_POINT('Ctrl Pts',(-3.40558558578551,-5.85033212661465,
129.635042811143));
#215564=CARTESIAN_POINT('Ctrl Pts',(-3.24838841911922,-5.9363508722558,
129.643465113491));
#215565=CARTESIAN_POINT('Ctrl Pts',(-3.09116515075727,-6.02238390082052,
129.651888814315));
#215566=CARTESIAN_POINT('Ctrl Pts',(-2.93054662700452,-6.10215356913166,
129.660312515138));
#215567=CARTESIAN_POINT('Ctrl Pts',(-2.76706362151651,-6.17540670032994,
129.668736215962));
#215568=CARTESIAN_POINT('Ctrl Pts',(-2.60346998558457,-6.2487094025916,
129.677165617181));
#215569=CARTESIAN_POINT('Ctrl Pts',(-2.43700829911282,-6.31548661939793,
129.6855950184));
#215570=CARTESIAN_POINT('Ctrl Pts',(-2.26822999552332,-6.37553305123645,
129.694024419619));
#215571=CARTESIAN_POINT('Ctrl Pts',(-2.09939147206966,-6.43560090755839,
129.702456828436));
#215572=CARTESIAN_POINT('Ctrl Pts',(-1.92823499958499,-6.48893308440157,
129.710889237254));
#215573=CARTESIAN_POINT('Ctrl Pts',(-1.75532745154532,-6.5353740931833,
129.719321646072));
#215574=CARTESIAN_POINT('Ctrl Pts',(-1.58225992441111,-6.58185807053765,
129.727761856799));
#215575=CARTESIAN_POINT('Ctrl Pts',(-1.40743840847123,-6.6214380602208,
129.736202067527));
#215576=CARTESIAN_POINT('Ctrl Pts',(-1.2314413453438,-6.6540094088435,129.744642278255));
#215577=CARTESIAN_POINT('Ctrl Pts',(-1.13133721906875,-6.67253543613928,
129.749442926092));
#215578=CARTESIAN_POINT('Ctrl Pts',(-1.03085294210219,-6.68879501086256,
129.754243573929));
#215579=CARTESIAN_POINT('Ctrl Pts',(-0.930095770582873,-6.70277635443283,
129.759044221766));
#215580=CARTESIAN_POINT('Ctrl Pts',(-0.759257439694681,-6.72648235335184,
129.767183936799));
#215581=CARTESIAN_POINT('Ctrl Pts',(-0.587293664602942,-6.74368299044695,
129.775323651832));
#215582=CARTESIAN_POINT('Ctrl Pts',(-0.414745515237176,-6.75427828547141,
129.783463366865));
#215583=CARTESIAN_POINT('Ctrl Pts',(-0.242348275447631,-6.76486431391442,
129.791595962952));
#215584=CARTESIAN_POINT('Ctrl Pts',(-0.0693680417233102,-6.76885647706346,
129.799728559039));
#215585=CARTESIAN_POINT('Ctrl Pts',(0.103646143768112,-6.76620621004725,
129.807861155126));
#215586=CARTESIAN_POINT('Ctrl Pts',(0.27654204748035,-6.76355775489576,
129.815988191334));
#215587=CARTESIAN_POINT('Ctrl Pts',(0.449471492083241,-6.75427591630593,
129.824115227543));
#215588=CARTESIAN_POINT('Ctrl Pts',(0.621882601247664,-6.73836412122894,
129.832242263751));
#215589=CARTESIAN_POINT('Ctrl Pts',(0.794211294781642,-6.72245993227796,
129.840365415088));
#215590=CARTESIAN_POINT('Ctrl Pts',(0.966021782391835,-6.69993213141763,
129.848488566426));
#215591=CARTESIAN_POINT('Ctrl Pts',(1.13676450063965,-6.67083618972056,
129.856611717764));
#215592=CARTESIAN_POINT('Ctrl Pts',(1.30745923891445,-6.64174842419938,
129.864732586435));
#215593=CARTESIAN_POINT('Ctrl Pts',(1.47708644491182,-6.6060962563491,129.872853455107));
#215594=CARTESIAN_POINT('Ctrl Pts',(1.64510400869592,-6.56398673068225,
129.880974323779));
#215595=CARTESIAN_POINT('Ctrl Pts',(1.81313065279243,-6.52187492925541,
129.889095631334));
#215596=CARTESIAN_POINT('Ctrl Pts',(1.97954712467904,-6.47330515799107,
129.897216938888));
#215597=CARTESIAN_POINT('Ctrl Pts',(2.14382361570506,-6.41843511338592,
129.905338246443));
#215598=CARTESIAN_POINT('Ctrl Pts',(2.22918739097763,-6.38992273083127,
129.909558360159));
#215599=CARTESIAN_POINT('Ctrl Pts',(2.31397356464635,-6.35970997104257,
129.913778473875));
#215600=CARTESIAN_POINT('Ctrl Pts',(2.39810960016221,-6.32782421892469,
129.917998587591));
#215601=CARTESIAN_POINT('Ctrl Pts',(2.57723155983313,-6.25994083970533,
129.926983026116));
#215602=CARTESIAN_POINT('Ctrl Pts',(2.75331696070877,-6.18450567964859,
129.935967464642));
#215603=CARTESIAN_POINT('Ctrl Pts',(2.92576566098836,-6.10181811405268,
129.944951903167));
#215604=CARTESIAN_POINT('Ctrl Pts',(3.09851199743215,-6.01898783465369,
129.953951848297));
#215605=CARTESIAN_POINT('Ctrl Pts',(3.26760887229161,-5.92888023450163,
129.962951793427));
#215606=CARTESIAN_POINT('Ctrl Pts',(3.43248109364044,-5.83184040777874,
129.971951738557));
#215607=CARTESIAN_POINT('Ctrl Pts',(3.59774184061054,-5.73457190421353,
129.980972892289));
#215608=CARTESIAN_POINT('Ctrl Pts',(3.75875780795001,-5.63033861015721,
129.989994046021));
#215609=CARTESIAN_POINT('Ctrl Pts',(3.91498082350201,-5.51953024736812,
129.999015199753));
#215610=CARTESIAN_POINT('Ctrl Pts',(4.07136279720394,-5.40860913619631,
130.008045532579));
#215611=CARTESIAN_POINT('Ctrl Pts',(4.22294188507482,-5.29109973396594,
130.017075865406));
#215612=CARTESIAN_POINT('Ctrl Pts',(4.36920210967447,-5.16743281763935,
130.026106198233));
#215613=CARTESIAN_POINT('Ctrl Pts',(4.51566968516852,-5.04359058060764,
130.035149333225));
#215614=CARTESIAN_POINT('Ctrl Pts',(4.65680313746559,-4.91357352917454,
130.044192468217));
#215615=CARTESIAN_POINT('Ctrl Pts',(4.7921208249499,-4.77785171380208,130.05323560321));
#215616=CARTESIAN_POINT('Ctrl Pts',(4.91041965922102,-4.65919957865099,
130.061141386612));
#215617=CARTESIAN_POINT('Ctrl Pts',(5.02427411626289,-4.53618805361324,
130.069047170014));
#215618=CARTESIAN_POINT('Ctrl Pts',(5.1333866744504,-4.40915300829707,130.076952953416));
#215619=CARTESIAN_POINT('Ctrl Pts',(5.25281738467958,-4.27010498359552,
130.085606341645));
#215620=CARTESIAN_POINT('Ctrl Pts',(5.36667148794623,-4.12611281017222,
130.094259729874));
#215621=CARTESIAN_POINT('Ctrl Pts',(5.47454641738078,-3.977641326709,130.102913118103));
#215622=CARTESIAN_POINT('Ctrl Pts',(5.58232171666579,-3.82930696719271,
130.111558514314));
#215623=CARTESIAN_POINT('Ctrl Pts',(5.68412867816535,-3.67650179399611,
130.120203910524));
#215624=CARTESIAN_POINT('Ctrl Pts',(5.77960525181488,-3.519723303499,130.128849306735));
#215625=CARTESIAN_POINT('Ctrl Pts',(5.87813102559388,-3.35793783615668,
130.137770807778));
#215626=CARTESIAN_POINT('Ctrl Pts',(5.96991515749052,-3.19192130305316,
130.14669230882));
#215627=CARTESIAN_POINT('Ctrl Pts',(6.0546071247108,-3.02225438462768,130.155613809862));
#215628=CARTESIAN_POINT('Ctrl Pts',(6.13652171310393,-2.85815150400141,
130.164242740204));
#215629=CARTESIAN_POINT('Ctrl Pts',(6.21180175270025,-2.6906341532244,130.172871670547));
#215630=CARTESIAN_POINT('Ctrl Pts',(6.28017559863909,-2.52025463996361,
130.181500600889));
#215631=CARTESIAN_POINT('Ctrl Pts',(6.35202684846474,-2.3412098487225,130.190568387281));
#215632=CARTESIAN_POINT('Ctrl Pts',(6.4162509413252,-2.15900446694894,130.199636173673));
#215633=CARTESIAN_POINT('Ctrl Pts',(6.47258869647183,-1.97430609741881,
130.208703960065));
#215634=CARTESIAN_POINT('Ctrl Pts',(6.52892645161846,-1.78960772788868,
130.217771746457));
#215635=CARTESIAN_POINT('Ctrl Pts',(6.57737772144378,-1.60241673385363,
130.226839532849));
#215636=CARTESIAN_POINT('Ctrl Pts',(6.61774319506332,-1.41342279739403,
130.235907319241));
#215637=CARTESIAN_POINT('Ctrl Pts',(6.65524709401102,-1.23782695126286,
130.244332275374));
#215638=CARTESIAN_POINT('Ctrl Pts',(6.68575477026857,-1.06075182863909,
130.252757231506));
#215639=CARTESIAN_POINT('Ctrl Pts',(6.70917194918932,-0.882780129030567,
130.261182187639));
#215640=CARTESIAN_POINT('Ctrl Pts',(6.73259456346211,-0.704767120481909,
130.269609099285));
#215641=CARTESIAN_POINT('Ctrl Pts',(6.74892335571185,-0.525857448792384,
130.278036010931));
#215642=CARTESIAN_POINT('Ctrl Pts',(6.7581158576744,-0.346639660526275,
130.286462922577));
#215643=CARTESIAN_POINT('Ctrl Pts',(6.76731174007799,-0.167355966898705,
130.294892933127));
#215644=CARTESIAN_POINT('Ctrl Pts',(6.76936608262606,0.012235738216695,
130.303322943676));
#215645=CARTESIAN_POINT('Ctrl Pts',(6.76428852229768,0.191545783331,130.311752954226));
#215646=CARTESIAN_POINT('Ctrl Pts',(6.75920628462692,0.37102100510872,130.320190730325));
#215647=CARTESIAN_POINT('Ctrl Pts',(6.74697902767285,0.550213716802047,
130.328628506424));
#215648=CARTESIAN_POINT('Ctrl Pts',(6.72766844219846,0.728537117686494,
130.337066282523));
#215649=CARTESIAN_POINT('Ctrl Pts',(6.70834772009017,0.906954125211403,
130.345508487832));
#215650=CARTESIAN_POINT('Ctrl Pts',(6.68193629732504,1.08450058339776,130.353950693142));
#215651=CARTESIAN_POINT('Ctrl Pts',(6.6485472977742,1.26059820294153,130.362392898451));
#215652=CARTESIAN_POINT('Ctrl Pts',(6.61512307466596,1.43688159578465,130.370844009823));
#215653=CARTESIAN_POINT('Ctrl Pts',(6.57470663998523,1.611712772811,130.379295121194));
#215654=CARTESIAN_POINT('Ctrl Pts',(6.52746170286202,1.78452590837726,130.387746232566));
#215655=CARTESIAN_POINT('Ctrl Pts',(6.51420233806007,1.83302618261969,130.390118050066));
#215656=CARTESIAN_POINT('Ctrl Pts',(6.50040542261883,1.88136760758521,130.392489867566));
#215657=CARTESIAN_POINT('Ctrl Pts',(6.48607526764057,1.92953792979078,130.394861685066));
#215658=CARTESIAN_POINT('Ctrl Pts',(6.43582501806462,2.09845241233877,130.403178721519));
#215659=CARTESIAN_POINT('Ctrl Pts',(6.37892343167615,2.26556646756993,130.411495757971));
#215660=CARTESIAN_POINT('Ctrl Pts',(6.31551992189105,2.43032860251392,130.419812794424));
#215661=CARTESIAN_POINT('Ctrl Pts',(6.25217157846125,2.59494738062312,130.428122594359));
#215662=CARTESIAN_POINT('Ctrl Pts',(6.18233270841608,2.75721799274781,130.436432394295));
#215663=CARTESIAN_POINT('Ctrl Pts',(6.10620249139547,2.91660421279195,130.44474219423));
#215664=CARTESIAN_POINT('Ctrl Pts',(6.02735961331197,3.08166965995505,130.453348087775));
#215665=CARTESIAN_POINT('Ctrl Pts',(5.94176887260188,3.24364100646435,130.461953981319));
#215666=CARTESIAN_POINT('Ctrl Pts',(5.84970649809143,3.40194398633883,130.470559874864));
#215667=CARTESIAN_POINT('Ctrl Pts',(5.76091870473339,3.55461626249723,130.478859664021));
#215668=CARTESIAN_POINT('Ctrl Pts',(5.66611192138681,3.70387631016144,130.487159453177));
#215669=CARTESIAN_POINT('Ctrl Pts',(5.56558115943957,3.84923308695268,130.495459242334));
#215670=CARTESIAN_POINT('Ctrl Pts',(5.46507657711748,3.9945520107937,130.503756870109));
#215671=CARTESIAN_POINT('Ctrl Pts',(5.35885118393023,4.13596940317617,130.512054497884));
#215672=CARTESIAN_POINT('Ctrl Pts',(5.24724353377759,4.27302285241131,130.520352125658));
#215673=CARTESIAN_POINT('Ctrl Pts',(5.13564640125446,4.41006338606763,130.528648971485));
#215674=CARTESIAN_POINT('Ctrl Pts',(5.01866824256713,4.54274052676302,130.536945817312));
#215675=CARTESIAN_POINT('Ctrl Pts',(4.89668826116683,4.67062448425807,130.545242663139));
#215676=CARTESIAN_POINT('Ctrl Pts',(4.77469950614701,4.79851764002625,130.553540105731));
#215677=CARTESIAN_POINT('Ctrl Pts',(4.64770845244548,4.92161667474264,130.561837548322));
#215678=CARTESIAN_POINT('Ctrl Pts',(4.5161316871342,5.03952811128804,130.570134990914));
#215679=CARTESIAN_POINT('Ctrl Pts',(4.38448221110785,5.15750470694299,130.57843701876));
#215680=CARTESIAN_POINT('Ctrl Pts',(4.2482422204802,5.27028774542234,130.586739046607));
#215681=CARTESIAN_POINT('Ctrl Pts',(4.10786250804287,5.37752309293189,130.595041074453));
#215682=CARTESIAN_POINT('Ctrl Pts',(3.9674369825844,5.484793436775,130.603345811673));
#215683=CARTESIAN_POINT('Ctrl Pts',(3.82286932331226,5.58651227583874,130.611650548892));
#215684=CARTESIAN_POINT('Ctrl Pts',(3.67464010641463,5.68236826405409,130.619955286111));
#215685=CARTESIAN_POINT('Ctrl Pts',(3.52629000069492,5.77830242793378,130.628266796286));
#215686=CARTESIAN_POINT('Ctrl Pts',(3.37427267024646,5.86836401059003,130.636578306461));
#215687=CARTESIAN_POINT('Ctrl Pts',(3.21909476324528,5.95228677948625,130.644889816635));
#215688=CARTESIAN_POINT('Ctrl Pts',(3.17930335758787,5.97380662728918,130.647021090857));
#215689=CARTESIAN_POINT('Ctrl Pts',(3.13930424687303,5.9949230681795,130.649152365079));
#215690=CARTESIAN_POINT('Ctrl Pts',(3.0991061983213,6.01563211736942,130.651283639301));
#215691=CARTESIAN_POINT('Origin',(0.,0.,4.30282021618968));
#215692=CARTESIAN_POINT('',(3.09910619832141,6.01563211736936,133.045915245968));
#215693=CARTESIAN_POINT('',(3.09910619832128,6.01563211736943,132.651465380124));
#215694=CARTESIAN_POINT('',(3.09910619832133,6.0156321173694,4.30282021618968));
#215695=CARTESIAN_POINT('',(-6.76699907392669,0.00354026487730927,131.697179783784));
#215696=CARTESIAN_POINT('Ctrl Pts',(-6.76699907392698,0.00354026431528137,
131.69717978381));
#215697=CARTESIAN_POINT('Ctrl Pts',(-6.76709497084188,-0.179760833150435,
131.705813112895));
#215698=CARTESIAN_POINT('Ctrl Pts',(-6.75973839205797,-0.363203276888397,
131.714446441981));
#215699=CARTESIAN_POINT('Ctrl Pts',(-6.74492430186807,-0.546154888350881,
131.723079771066));
#215700=CARTESIAN_POINT('Ctrl Pts',(-6.73049099454992,-0.724403893098308,
131.731491188188));
#215701=CARTESIAN_POINT('Ctrl Pts',(-6.7089788469857,-0.90218662774764,
131.739902605309));
#215702=CARTESIAN_POINT('Ctrl Pts',(-6.6804358924897,-1.0789185726158,131.748314022431));
#215703=CARTESIAN_POINT('Ctrl Pts',(-6.65076339769416,-1.26264439241631,
131.757058307498));
#215704=CARTESIAN_POINT('Ctrl Pts',(-6.6134922718676,-1.44523418945677,
131.765802592566));
#215705=CARTESIAN_POINT('Ctrl Pts',(-6.56873593024028,-1.62603729316716,
131.774546877633));
#215706=CARTESIAN_POINT('Ctrl Pts',(-6.52397958861293,-1.80684039687767,
131.7832911627));
#215707=CARTESIAN_POINT('Ctrl Pts',(-6.47173810469297,-1.98585640656563,
131.792035447767));
#215708=CARTESIAN_POINT('Ctrl Pts',(-6.41218472486434,-2.16244677488636,
131.800779732834));
#215709=CARTESIAN_POINT('Ctrl Pts',(-6.35480615025228,-2.33258831267348,
131.809204688976));
#215710=CARTESIAN_POINT('Ctrl Pts',(-6.29065631498354,-2.500430846268,131.817629645118));
#215711=CARTESIAN_POINT('Ctrl Pts',(-6.21995157621256,-2.6654251798861,
131.82605460126));
#215712=CARTESIAN_POINT('Ctrl Pts',(-6.14923042618649,-2.83045781028806,
131.834481512916));
#215713=CARTESIAN_POINT('Ctrl Pts',(-6.0719514697138,-2.9926406177891,131.842908424571));
#215714=CARTESIAN_POINT('Ctrl Pts',(-5.9883785978316,-3.15144582200494,
131.851335336227));
#215715=CARTESIAN_POINT('Ctrl Pts',(-5.90477499294191,-3.3103094250938,
131.859765346787));
#215716=CARTESIAN_POINT('Ctrl Pts',(-5.81487301206899,-3.46579265500461,
131.868195357348));
#215717=CARTESIAN_POINT('Ctrl Pts',(-5.71898192682299,-3.61739335995853,
131.876625367908));
#215718=CARTESIAN_POINT('Ctrl Pts',(-5.62300250870327,-3.76913371632938,
131.885063144018));
#215719=CARTESIAN_POINT('Ctrl Pts',(-5.52102314104431,-3.91698412176279,
131.893500920129));
#215720=CARTESIAN_POINT('Ctrl Pts',(-5.41339639226867,-4.060471462795,131.90193869624));
#215721=CARTESIAN_POINT('Ctrl Pts',(-5.30571314737572,-4.20403412411464,
131.910380901561));
#215722=CARTESIAN_POINT('Ctrl Pts',(-5.19237681409164,-4.34322889305352,
131.918823106883));
#215723=CARTESIAN_POINT('Ctrl Pts',(-5.07377984477311,-4.47761622817032,
131.927265312205));
#215724=CARTESIAN_POINT('Ctrl Pts',(-4.95505776216699,-4.61214533454318,
131.935716423589));
#215725=CARTESIAN_POINT('Ctrl Pts',(-4.83106418257116,-4.74185663299263,
131.944167534974));
#215726=CARTESIAN_POINT('Ctrl Pts',(-4.70222869586103,-4.86634711994748,
131.952618646358));
#215727=CARTESIAN_POINT('Ctrl Pts',(-4.66607081797621,-4.90128556695519,
131.954990463792));
#215728=CARTESIAN_POINT('Ctrl Pts',(-4.62953177020199,-4.93581303554232,
131.957362281225));
#215729=CARTESIAN_POINT('Ctrl Pts',(-4.59262151425912,-4.96992118919046,
131.959734098659));
#215730=CARTESIAN_POINT('Ctrl Pts',(-4.46320356918836,-5.0895141598307,
131.968050370938));
#215731=CARTESIAN_POINT('Ctrl Pts',(-4.32898587182286,-5.2041647890652,
131.976366643218));
#215732=CARTESIAN_POINT('Ctrl Pts',(-4.19037828833678,-5.31347520937435,
131.984682915498));
#215733=CARTESIAN_POINT('Ctrl Pts',(-4.05188789774753,-5.42269320757722,
131.992992156358));
#215734=CARTESIAN_POINT('Ctrl Pts',(-3.90901528784766,-5.52657977833173,
132.001301397218));
#215735=CARTESIAN_POINT('Ctrl Pts',(-3.76220534782492,-5.62477554403708,
132.009610638078));
#215736=CARTESIAN_POINT('Ctrl Pts',(-3.6154926187237,-5.72290628893476,
132.017914376934));
#215737=CARTESIAN_POINT('Ctrl Pts',(-3.46484804272415,-5.81535354453606,
132.026218115789));
#215738=CARTESIAN_POINT('Ctrl Pts',(-3.31074777697401,-5.90179956939082,
132.034521854645));
#215739=CARTESIAN_POINT('Ctrl Pts',(-3.15672130830467,-5.9882041961062,
132.042821616923));
#215740=CARTESIAN_POINT('Ctrl Pts',(-2.99924275074094,-6.06861314962715,
132.051121379201));
#215741=CARTESIAN_POINT('Ctrl Pts',(-2.83881549031413,-6.1427530971017,
132.059421141479));
#215742=CARTESIAN_POINT('Ctrl Pts',(-2.67843566613839,-6.21687112235959,
132.067718449625));
#215743=CARTESIAN_POINT('Ctrl Pts',(-2.51510919250034,-6.28472369065521,
132.076015757772));
#215744=CARTESIAN_POINT('Ctrl Pts',(-2.34936239850547,-6.34608425097624,
132.084313065918));
#215745=CARTESIAN_POINT('Ctrl Pts',(-2.18359885820913,-6.40745101088893,
132.092611212386));
#215746=CARTESIAN_POINT('Ctrl Pts',(-2.01541483259486,-6.46232432432534,
132.100909358855));
#215747=CARTESIAN_POINT('Ctrl Pts',(-1.84535545163506,-6.51052626575769,
132.109207505323));
#215748=CARTESIAN_POINT('Ctrl Pts',(-1.67527897013812,-6.55873305419751,
132.117506486223));
#215749=CARTESIAN_POINT('Ctrl Pts',(-1.50332709221133,-6.6002670380266,
132.125805467122));
#215750=CARTESIAN_POINT('Ctrl Pts',(-1.33005880005892,-6.63500057184518,
132.134104448021));
#215751=CARTESIAN_POINT('Ctrl Pts',(-1.15674428946044,-6.66974337065933,
132.142405642632));
#215752=CARTESIAN_POINT('Ctrl Pts',(-0.982113006033505,-6.69768203560138,
132.150706837243));
#215753=CARTESIAN_POINT('Ctrl Pts',(-0.80673296985677,-6.71874027741407,
132.159008031853));
#215754=CARTESIAN_POINT('Ctrl Pts',(-0.631277002325003,-6.7398076364608,
132.167312820493));
#215755=CARTESIAN_POINT('Ctrl Pts',(-0.455071981281516,-6.75398859393647,
132.175617609133));
#215756=CARTESIAN_POINT('Ctrl Pts',(-0.278690069031756,-6.76125882106454,
132.183922397773));
#215757=CARTESIAN_POINT('Ctrl Pts',(-0.10209905758523,-6.76853766698257,
132.192237031666));
#215758=CARTESIAN_POINT('Ctrl Pts',(0.074668915954113,-6.76888939950066,
132.200551665559));
#215759=CARTESIAN_POINT('Ctrl Pts',(0.251041473807029,-6.76234184128759,
132.208866299452));
#215760=CARTESIAN_POINT('Ctrl Pts',(0.427525553601578,-6.75579014299505,
132.217186190763));
#215761=CARTESIAN_POINT('Ctrl Pts',(0.603613372588242,-6.74233048058884,
132.225506082073));
#215762=CARTESIAN_POINT('Ctrl Pts',(0.778738501598195,-6.72204249809004,
132.233825973384));
#215763=CARTESIAN_POINT('Ctrl Pts',(0.954125499504187,-6.70172417847395,
132.242158305631));
#215764=CARTESIAN_POINT('Ctrl Pts',(1.12854658684618,-6.67455718662064,
132.250490637879));
#215765=CARTESIAN_POINT('Ctrl Pts',(1.3014449890108,-6.6406724012391,132.258822970127));
#215766=CARTESIAN_POINT('Ctrl Pts',(1.43161757685582,-6.61516105962769,
132.265096256854));
#215767=CARTESIAN_POINT('Ctrl Pts',(1.56092727260945,-6.5858428926111,132.271369543581));
#215768=CARTESIAN_POINT('Ctrl Pts',(1.68914275140066,-6.55279221136995,
132.277642830309));
#215769=CARTESIAN_POINT('Ctrl Pts',(1.85407689834577,-6.51027639371783,
132.285712676513));
#215770=CARTESIAN_POINT('Ctrl Pts',(2.01770936421284,-6.46145082056711,
132.293782522718));
#215771=CARTESIAN_POINT('Ctrl Pts',(2.17950805597581,-6.4064056719768,132.301852368923));
#215772=CARTESIAN_POINT('Ctrl Pts',(2.34110318440282,-6.35142977718548,
132.309912062235));
#215773=CARTESIAN_POINT('Ctrl Pts',(2.50086878054943,-6.29024999521635,
132.317971755546));
#215774=CARTESIAN_POINT('Ctrl Pts',(2.65828259754013,-6.22300752302416,
132.326031448858));
#215775=CARTESIAN_POINT('Ctrl Pts',(2.81553291527486,-6.1558348928216,132.334082770898));
#215776=CARTESIAN_POINT('Ctrl Pts',(2.97043597466164,-6.08261224893743,
132.342134092938));
#215777=CARTESIAN_POINT('Ctrl Pts',(3.12248446810918,-6.0035306067694,132.350185414977));
#215778=CARTESIAN_POINT('Ctrl Pts',(3.2744083540449,-5.92451377396869,132.358230138759));
#215779=CARTESIAN_POINT('Ctrl Pts',(3.42348200086224,-5.83964767087949,
132.366274862541));
#215780=CARTESIAN_POINT('Ctrl Pts',(3.56921798634966,-5.74917141559704,
132.374319586322));
#215781=CARTESIAN_POINT('Ctrl Pts',(3.71486643925043,-5.65874950255978,
132.382359478247));
#215782=CARTESIAN_POINT('Ctrl Pts',(3.85718090534057,-5.56272434144218,
132.390399370171));
#215783=CARTESIAN_POINT('Ctrl Pts',(3.99569859359893,-5.46138093792326,
132.398439262096));
#215784=CARTESIAN_POINT('Ctrl Pts',(4.13719894149439,-5.35785533743756,
132.40665227459));
#215785=CARTESIAN_POINT('Ctrl Pts',(4.27473679332243,-5.24878004803285,
132.414865287084));
#215786=CARTESIAN_POINT('Ctrl Pts',(4.40784969965924,-5.13450582093486,
132.423078299578));
#215787=CARTESIAN_POINT('Ctrl Pts',(4.53811127849206,-5.02267938988977,
132.431115386319));
#215788=CARTESIAN_POINT('Ctrl Pts',(4.66413527302074,-4.9058747543783,132.439152473059));
#215789=CARTESIAN_POINT('Ctrl Pts',(4.78552188066206,-4.78446123714098,
132.447189559799));
#215790=CARTESIAN_POINT('Ctrl Pts',(4.90692010555167,-4.66303610008001,
132.455227415725));
#215791=CARTESIAN_POINT('Ctrl Pts',(5.0236797955743,-4.53700146714822,132.463265271651));
#215792=CARTESIAN_POINT('Ctrl Pts',(5.13543839212052,-4.40676315686861,
132.471303127577));
#215793=CARTESIAN_POINT('Ctrl Pts',(5.24722982757857,-4.27648657763682,
132.479343345329));
#215794=CARTESIAN_POINT('Ctrl Pts',(5.35401700137793,-4.14200414581877,
132.487383563082));
#215795=CARTESIAN_POINT('Ctrl Pts',(5.45547808825628,-4.00375421680148,
132.495423780835));
#215796=CARTESIAN_POINT('Ctrl Pts',(5.5607724328051,-3.86028112669699,132.503767762595));
#215797=CARTESIAN_POINT('Ctrl Pts',(5.66033012114379,-3.7127506613426,132.512111744355));
#215798=CARTESIAN_POINT('Ctrl Pts',(5.75384181462403,-3.56168406407476,
132.520455726115));
#215799=CARTESIAN_POINT('Ctrl Pts',(5.84410606836313,-3.41586365210489,
132.528509941142));
#215800=CARTESIAN_POINT('Ctrl Pts',(5.92873708984125,-3.26674894657301,
132.536564156169));
#215801=CARTESIAN_POINT('Ctrl Pts',(6.00750464953942,-3.11483175882138,
132.544618371196));
#215802=CARTESIAN_POINT('Ctrl Pts',(6.08633115371727,-2.96280088620225,
132.552678613469));
#215803=CARTESIAN_POINT('Ctrl Pts',(6.15928530123639,-2.80796369122435,
132.560738855743));
#215804=CARTESIAN_POINT('Ctrl Pts',(6.22618559531596,-2.65083042322213,
132.568799098016));
#215805=CARTESIAN_POINT('Ctrl Pts',(6.29317942057075,-2.49347747219124,
132.576870609058));
#215806=CARTESIAN_POINT('Ctrl Pts',(6.35410237390941,-2.33382238924736,
132.5849421201));
#215807=CARTESIAN_POINT('Ctrl Pts',(6.40882304117147,-2.17238952007914,
132.593013631142));
#215808=CARTESIAN_POINT('Ctrl Pts',(6.41455832695984,-2.15546970373476,
132.593859608081));
#215809=CARTESIAN_POINT('Ctrl Pts',(6.42022552602584,-2.1385303659194,132.594705585019));
#215810=CARTESIAN_POINT('Ctrl Pts',(6.42582451980291,-2.12157211536626,
132.595551561958));
#215811=CARTESIAN_POINT('Ctrl Pts',(6.480288792434,-1.95661054936942,132.603780811795));
#215812=CARTESIAN_POINT('Ctrl Pts',(6.52847676044186,-1.78930795410407,
132.612010061631));
#215813=CARTESIAN_POINT('Ctrl Pts',(6.57018245520745,-1.62018255307363,
132.620239311468));
#215814=CARTESIAN_POINT('Ctrl Pts',(6.6118385134206,-1.4512584387472,132.62845876716));
#215815=CARTESIAN_POINT('Ctrl Pts',(6.64702757545373,-1.28051618323012,
132.636678222852));
#215816=CARTESIAN_POINT('Ctrl Pts',(6.67559245066795,-1.10849196324786,
132.644897678545));
#215817=CARTESIAN_POINT('Ctrl Pts',(6.70412906556926,-0.93663793334162,
132.653109002418));
#215818=CARTESIAN_POINT('Ctrl Pts',(6.72605448654629,-0.763504816106835,
132.661320326292));
#215819=CARTESIAN_POINT('Ctrl Pts',(6.74126185300704,-0.589641949993522,
132.669531650165));
#215820=CARTESIAN_POINT('Ctrl Pts',(6.75645722715312,-0.415916189683682,
132.677736498705));
#215821=CARTESIAN_POINT('Ctrl Pts',(6.76494506755597,-0.241462182364821,
132.685941347244));
#215822=CARTESIAN_POINT('Ctrl Pts',(6.76666991567789,-0.0668375063847751,
132.694146195783));
#215823=CARTESIAN_POINT('Ctrl Pts',(6.76839374978632,0.1076845102499,132.70234622081));
#215824=CARTESIAN_POINT('Ctrl Pts',(6.76336250840278,0.282376638002501,
132.710546245836));
#215825=CARTESIAN_POINT('Ctrl Pts',(6.75157271658027,0.456678062456395,
132.718746270862));
#215826=CARTESIAN_POINT('Ctrl Pts',(6.73978633698824,0.630929040164369,
132.726943922617));
#215827=CARTESIAN_POINT('Ctrl Pts',(6.72124532343041,0.804789182163561,
132.735141574373));
#215828=CARTESIAN_POINT('Ctrl Pts',(6.69599828685307,0.977699310862392,
132.743339226128));
#215829=CARTESIAN_POINT('Ctrl Pts',(6.67075463100586,1.15058628585447,132.751535780168));
#215830=CARTESIAN_POINT('Ctrl Pts',(6.63880679155738,1.32252314591521,132.759732334208));
#215831=CARTESIAN_POINT('Ctrl Pts',(6.60025507465575,1.49295745065993,132.767928888248));
#215832=CARTESIAN_POINT('Ctrl Pts',(6.56170151035774,1.66339992260816,132.776125835067));
#215833=CARTESIAN_POINT('Ctrl Pts',(6.51654351724407,1.83233934584685,132.784322781885));
#215834=CARTESIAN_POINT('Ctrl Pts',(6.46493220196712,1.9992350096896,132.792519728704));
#215835=CARTESIAN_POINT('Ctrl Pts',(6.41330902922189,2.16616901706283,132.800718558734));
#215836=CARTESIAN_POINT('Ctrl Pts',(6.35522968734433,2.33105798718433,132.808917388765));
#215837=CARTESIAN_POINT('Ctrl Pts',(6.29089469473621,2.4933778172872,132.817116218795));
#215838=CARTESIAN_POINT('Ctrl Pts',(6.22649876866193,2.65585138502914,132.825322814166));
#215839=CARTESIAN_POINT('Ctrl Pts',(6.15583548680489,2.81575061728925,132.833529409537));
#215840=CARTESIAN_POINT('Ctrl Pts',(6.07915332149875,2.97257193247038,132.841736004908));
#215841=CARTESIAN_POINT('Ctrl Pts',(6.00243404158102,3.12946915007523,132.849946572319));
#215842=CARTESIAN_POINT('Ctrl Pts',(5.9196902398935,3.2832851646876,132.85815713973));
#215843=CARTESIAN_POINT('Ctrl Pts',(5.83121559865078,3.43354243341361,132.866367707141));
#215844=CARTESIAN_POINT('Ctrl Pts',(5.74261893821646,3.58400692841603,132.874589598099));
#215845=CARTESIAN_POINT('Ctrl Pts',(5.6482758366476,3.73090256688787,132.882811489057));
#215846=CARTESIAN_POINT('Ctrl Pts',(5.54852311298748,3.87378113277503,132.891033380015));
#215847=CARTESIAN_POINT('Ctrl Pts',(5.45782436231733,4.003691444474,132.898509017879));
#215848=CARTESIAN_POINT('Ctrl Pts',(5.36265406615867,4.1302810409493,132.905984655743));
#215849=CARTESIAN_POINT('Ctrl Pts',(5.26329298321657,4.2532382925041,132.913460293607));
#215850=CARTESIAN_POINT('Ctrl Pts',(5.14450120317043,4.40024062328876,132.922397840407));
#215851=CARTESIAN_POINT('Ctrl Pts',(5.01947177254576,4.54235715527166,132.931335387207));
#215852=CARTESIAN_POINT('Ctrl Pts',(4.888612363018,4.67907663584895,132.940272934007));
#215853=CARTESIAN_POINT('Ctrl Pts',(4.75804937042662,4.81548642551658,132.949190235871));
#215854=CARTESIAN_POINT('Ctrl Pts',(4.62168293609941,4.94652337913678,132.958107537736));
#215855=CARTESIAN_POINT('Ctrl Pts',(4.47995901652833,5.07171136897857,132.967024839601));
#215856=CARTESIAN_POINT('Ctrl Pts',(4.33843991738055,5.19671843624111,132.975929254117));
#215857=CARTESIAN_POINT('Ctrl Pts',(4.19157897124605,5.31589323208888,132.984833668633));
#215858=CARTESIAN_POINT('Ctrl Pts',(4.03985879706266,5.42879635829117,132.99373808315));
#215859=CARTESIAN_POINT('Ctrl Pts',(3.88850419997671,5.54142743895046,133.002621042048));
#215860=CARTESIAN_POINT('Ctrl Pts',(3.7323139469524,5.64781685353747,133.011504000947));
#215861=CARTESIAN_POINT('Ctrl Pts',(3.57180300349476,5.74756577206611,133.020386959846));
#215862=CARTESIAN_POINT('Ctrl Pts',(3.41804157718929,5.84312022869689,133.028896388553));
#215863=CARTESIAN_POINT('Ctrl Pts',(3.2603155590624,5.93258100663783,133.037405817261));
#215864=CARTESIAN_POINT('Ctrl Pts',(3.09910619832141,6.01563211736936,133.045915245968));
#215865=CARTESIAN_POINT('Ctrl Pts',(3.09910619832127,6.01563211736944,131.045783168526));
#215866=CARTESIAN_POINT('Ctrl Pts',(2.94005916857604,6.09756924817982,131.054219631559));
#215867=CARTESIAN_POINT('Ctrl Pts',(2.77765505604874,6.17324937003544,131.062656094593));
#215868=CARTESIAN_POINT('Ctrl Pts',(2.61241474863898,6.24240163567625,131.071092557626));
#215869=CARTESIAN_POINT('Ctrl Pts',(2.44728583965193,6.31150728161851,131.079523333132));
#215870=CARTESIAN_POINT('Ctrl Pts',(2.27932485447001,6.37409371657269,131.087954108638));
#215871=CARTESIAN_POINT('Ctrl Pts',(2.10907500319488,6.42993714050912,131.096384884145));
#215872=CARTESIAN_POINT('Ctrl Pts',(1.93891377186047,6.48575149633839,131.10481127119));
#215873=CARTESIAN_POINT('Ctrl Pts',(1.76646636625224,6.53482973579416,131.113237658236));
#215874=CARTESIAN_POINT('Ctrl Pts',(1.59229396690954,6.57699695324116,131.121664045281));
#215875=CARTESIAN_POINT('Ctrl Pts',(1.41810494468684,6.61916819509499,131.130091236534));
#215876=CARTESIAN_POINT('Ctrl Pts',(1.24219091916096,6.65442699955921,131.138518427788));
#215877=CARTESIAN_POINT('Ctrl Pts',(1.06512733873329,6.68264863301094,131.146945619041));
#215878=CARTESIAN_POINT('Ctrl Pts',(0.888165580687034,6.71085403729844,
131.155367964144));
#215879=CARTESIAN_POINT('Ctrl Pts',(0.710055918205982,6.7320303049067,131.163790309247));
#215880=CARTESIAN_POINT('Ctrl Pts',(0.531382030646969,6.74610421928875,
131.172212654351));
#215881=CARTESIAN_POINT('Ctrl Pts',(0.352714136698274,6.76017766156176,
131.180634716927));
#215882=CARTESIAN_POINT('Ctrl Pts',(0.173482387848984,6.76714919961372,
131.189056779503));
#215883=CARTESIAN_POINT('Ctrl Pts',(-0.00572532888578081,6.7669975779964,
131.197478842078));
#215884=CARTESIAN_POINT('Ctrl Pts',(-0.184952050309111,6.76684594029986,
131.2059017978));
#215885=CARTESIAN_POINT('Ctrl Pts',(-0.36415440107678,6.75956963771297,
131.214324753523));
#215886=CARTESIAN_POINT('Ctrl Pts',(-0.542745036850973,6.74519953930005,
131.222747709245));
#215887=CARTESIAN_POINT('Ctrl Pts',(-0.721500802956766,6.73081615385724,
131.231178453088));
#215888=CARTESIAN_POINT('Ctrl Pts',(-0.899643389640689,6.70932588122367,
131.239609196931));
#215889=CARTESIAN_POINT('Ctrl Pts',(-1.07658955657966,6.68081162185132,
131.248039940774));
#215890=CARTESIAN_POINT('Ctrl Pts',(-1.25354079277129,6.65229654558653,
131.256470926145));
#215891=CARTESIAN_POINT('Ctrl Pts',(-1.42929521484197,6.61675715479673,
131.264901911517));
#215892=CARTESIAN_POINT('Ctrl Pts',(-1.60328020808028,6.5743274617544,131.273332896888));
#215893=CARTESIAN_POINT('Ctrl Pts',(-1.77744048076064,6.531855023342,131.281772375972));
#215894=CARTESIAN_POINT('Ctrl Pts',(-1.94982743830728,6.4824784923953,131.290211855056));
#215895=CARTESIAN_POINT('Ctrl Pts',(-2.11988227947715,6.4263821953848,131.298651334139));
#215896=CARTESIAN_POINT('Ctrl Pts',(-2.28958022503889,6.37040362817192,
131.307073101213));
#215897=CARTESIAN_POINT('Ctrl Pts',(-2.45695553865008,6.30773362669709,
131.315494868287));
#215898=CARTESIAN_POINT('Ctrl Pts',(-2.62147298918131,6.23860307817326,
131.32391663536));
#215899=CARTESIAN_POINT('Ctrl Pts',(-2.78048061325775,6.17178776930249,
131.33205635044));
#215900=CARTESIAN_POINT('Ctrl Pts',(-2.93713551430113,6.09880390692183,
131.340196065519));
#215901=CARTESIAN_POINT('Ctrl Pts',(-3.09092138236668,6.01984169293748,
131.348335780599));
#215902=CARTESIAN_POINT('Ctrl Pts',(-3.24457275022895,5.94094853883469,
131.356468376732));
#215903=CARTESIAN_POINT('Ctrl Pts',(-3.39535975619418,5.85608760681051,
131.364600972865));
#215904=CARTESIAN_POINT('Ctrl Pts',(-3.54278547864823,5.7654973811701,131.372733568998));
#215905=CARTESIAN_POINT('Ctrl Pts',(-3.69011041296322,5.67496908787165,
131.380860605252));
#215906=CARTESIAN_POINT('Ctrl Pts',(-3.83407832814475,5.57871949014853,
131.388987641506));
#215907=CARTESIAN_POINT('Ctrl Pts',(-3.97421640348247,5.47703322778773,
131.39711467776));
#215908=CARTESIAN_POINT('Ctrl Pts',(-4.11428749027271,5.37539557330882,
131.405237829142));
#215909=CARTESIAN_POINT('Ctrl Pts',(-4.25053208703943,5.26832664391953,
131.413360980525));
#215910=CARTESIAN_POINT('Ctrl Pts',(-4.38250592672784,5.15615465266465,
131.421484131908));
#215911=CARTESIAN_POINT('Ctrl Pts',(-4.51444268078081,5.0440141825778,131.429605000624));
#215912=CARTESIAN_POINT('Ctrl Pts',(-4.64211078986738,4.92677374443147,
131.437725869341));
#215913=CARTESIAN_POINT('Ctrl Pts',(-4.76509872085858,4.8048020958695,131.445846738057));
#215914=CARTESIAN_POINT('Ctrl Pts',(-4.88809329857753,4.68282385550348,
131.453968045656));
#215915=CARTESIAN_POINT('Ctrl Pts',(-5.0064069300545,4.556114148958,131.462089353254));
#215916=CARTESIAN_POINT('Ctrl Pts',(-5.11966451445874,4.42507901165527,
131.470210660853));
#215917=CARTESIAN_POINT('Ctrl Pts',(-5.17851708823133,4.35698860406379,
131.474430774297));
#215918=CARTESIAN_POINT('Ctrl Pts',(-5.23600505119378,4.28773083069518,
131.478650887741));
#215919=CARTESIAN_POINT('Ctrl Pts',(-5.29208000568025,4.21736626503786,
131.482871001185));
#215920=CARTESIAN_POINT('Ctrl Pts',(-5.41146115058981,4.0675631579972,131.491855439589));
#215921=CARTESIAN_POINT('Ctrl Pts',(-5.52437645878455,3.91281606115083,
131.500839877993));
#215922=CARTESIAN_POINT('Ctrl Pts',(-5.63046266527174,3.75368874242139,
131.509824316397));
#215923=CARTESIAN_POINT('Ctrl Pts',(-5.73673197018465,3.5942867794897,131.518824261402));
#215924=CARTESIAN_POINT('Ctrl Pts',(-5.83614848254495,3.43048968312826,
131.527824206408));
#215925=CARTESIAN_POINT('Ctrl Pts',(-5.92839372845277,3.26288780077432,
131.536824151413));
#215926=CARTESIAN_POINT('Ctrl Pts',(-6.02085635263005,3.09489096031943,
131.545845305018));
#215927=CARTESIAN_POINT('Ctrl Pts',(-6.10611378196859,2.92307160440881,
131.554866458623));
#215928=CARTESIAN_POINT('Ctrl Pts',(-6.18389355657347,2.74804466502441,
131.563887612228));
#215929=CARTESIAN_POINT('Ctrl Pts',(-6.26175247270942,2.5728396343556,131.572917944928));
#215930=CARTESIAN_POINT('Ctrl Pts',(-6.33211844258303,2.39442072067031,
131.581948277627));
#215931=CARTESIAN_POINT('Ctrl Pts',(-6.39476764691178,2.21342172710273,
131.590978610327));
#215932=CARTESIAN_POINT('Ctrl Pts',(-6.45750566807776,2.03216613397694,
131.600021745193));
#215933=CARTESIAN_POINT('Ctrl Pts',(-6.51250497081679,1.84832337316261,
131.60906488006));
#215934=CARTESIAN_POINT('Ctrl Pts',(-6.5595913082107,1.66254349394134,131.618108014927));
#215935=CARTESIAN_POINT('Ctrl Pts',(-6.60075561899143,1.50012906316717,
131.626013798954));
#215936=CARTESIAN_POINT('Ctrl Pts',(-6.63587296388161,1.3362344347959,131.633919582982));
#215937=CARTESIAN_POINT('Ctrl Pts',(-6.66485893493869,1.17130029342092,
131.64182536701));
#215938=CARTESIAN_POINT('Ctrl Pts',(-6.69981997936319,0.972367167034594,
131.651360823526));
#215939=CARTESIAN_POINT('Ctrl Pts',(-6.72588152660799,0.771803127922735,
131.660896280042));
#215940=CARTESIAN_POINT('Ctrl Pts',(-6.74292139287532,0.570350847728295,
131.670431736559));
#215941=CARTESIAN_POINT('Ctrl Pts',(-6.75885431812254,0.381985277783969,
131.6793477523));
#215942=CARTESIAN_POINT('Ctrl Pts',(-6.7669000369816,0.192843308266294,
131.688263768042));
#215943=CARTESIAN_POINT('Ctrl Pts',(-6.76699907392669,0.00354026487731378,
131.697179783784));
#215944=CARTESIAN_POINT('',(-6.76699797440541,-0.00523587558187145,131.302820216153));
#215945=CARTESIAN_POINT('Ctrl Pts',(3.0991061983213,6.01563211736942,130.651283639301));
#215946=CARTESIAN_POINT('Ctrl Pts',(2.94215097151982,6.09649160258211,130.659605302688));
#215947=CARTESIAN_POINT('Ctrl Pts',(2.78216153052165,6.17113635103588,130.667926966075));
#215948=CARTESIAN_POINT('Ctrl Pts',(2.6196709735354,6.23935998243539,130.676248629462));
#215949=CARTESIAN_POINT('Ctrl Pts',(2.45695092246554,6.30767996970971,130.684582045979));
#215950=CARTESIAN_POINT('Ctrl Pts',(2.2917230233006,6.36956059997624,130.692915462495));
#215951=CARTESIAN_POINT('Ctrl Pts',(2.12453663340948,6.42484498593555,130.701248879011));
#215952=CARTESIAN_POINT('Ctrl Pts',(2.04748763072223,6.45032317710359,130.705089391579));
#215953=CARTESIAN_POINT('Ctrl Pts',(1.97002282961067,6.47440110779183,130.708929904147));
#215954=CARTESIAN_POINT('Ctrl Pts',(1.89219669411109,6.49706708221449,130.712770416715));
#215955=CARTESIAN_POINT('Ctrl Pts',(1.72866515570096,6.54469377783683,130.720840262718));
#215956=CARTESIAN_POINT('Ctrl Pts',(1.56303228692083,6.58623017011433,130.728910108722));
#215957=CARTESIAN_POINT('Ctrl Pts',(1.39580167597483,6.62148221181224,130.736979954725));
#215958=CARTESIAN_POINT('Ctrl Pts',(1.22878146240835,6.65668990195779,130.745039647836));
#215959=CARTESIAN_POINT('Ctrl Pts',(1.06016786676457,6.68562889732855,130.753099340946));
#215960=CARTESIAN_POINT('Ctrl Pts',(0.89048205076826,6.70815404692376,130.761159034057));
#215961=CARTESIAN_POINT('Ctrl Pts',(0.720972480443196,6.73065580057343,
130.769210355896));
#215962=CARTESIAN_POINT('Ctrl Pts',(0.550393272684829,6.74675691681266,
130.777261677735));
#215963=CARTESIAN_POINT('Ctrl Pts',(0.37927817132368,6.75636270997623,130.785312999574));
#215964=CARTESIAN_POINT('Ctrl Pts',(0.208303303024427,6.7659606309545,130.793357723156));
#215965=CARTESIAN_POINT('Ctrl Pts',(0.0367937858360792,6.76907380268978,
130.801402446737));
#215966=CARTESIAN_POINT('Ctrl Pts',(-0.134709183319342,6.76565905407075,
130.809447170319));
#215967=CARTESIAN_POINT('Ctrl Pts',(-0.306109143619822,6.76224635643279,
130.817487062044));
#215968=CARTESIAN_POINT('Ctrl Pts',(-0.477502191633343,6.75231355100528,
130.825526953769));
#215969=CARTESIAN_POINT('Ctrl Pts',(-0.648344889022779,6.73586949880103,
130.833566845494));
#215970=CARTESIAN_POINT('Ctrl Pts',(-0.822866297722585,6.71907136110319,
130.841779858113));
#215971=CARTESIAN_POINT('Ctrl Pts',(-0.9968129878807,6.69547836327735,130.849992870733));
#215972=CARTESIAN_POINT('Ctrl Pts',(-1.16960825650072,6.66515607666657,
130.858205883353));
#215973=CARTESIAN_POINT('Ctrl Pts',(-1.33870218006575,6.63548330578907,
130.866242969896));
#215974=CARTESIAN_POINT('Ctrl Pts',(-1.50669312963795,6.5993666940462,130.874280056439));
#215975=CARTESIAN_POINT('Ctrl Pts',(-1.67304879419528,6.55691975947866,
130.882317142982));
#215976=CARTESIAN_POINT('Ctrl Pts',(-1.83942037976398,6.51446876254193,
130.890354998712));
#215977=CARTESIAN_POINT('Ctrl Pts',(-2.00415600662239,6.46568632870257,
130.898392854441));
#215978=CARTESIAN_POINT('Ctrl Pts',(-2.16673676216277,6.41073636983244,
130.906430710171));
#215979=CARTESIAN_POINT('Ctrl Pts',(-2.32936529011382,6.35577026457406,
130.914470927729));
#215980=CARTESIAN_POINT('Ctrl Pts',(-2.48983733266218,6.29463314662318,
130.922511145286));
#215981=CARTESIAN_POINT('Ctrl Pts',(-2.64765239694011,6.22753769839872,
130.930551362844));
#215982=CARTESIAN_POINT('Ctrl Pts',(-2.81142981543061,6.15790734116419,
130.93889534497));
#215983=CARTESIAN_POINT('Ctrl Pts',(-2.97234515995403,6.08185981477191,
130.947239327097));
#215984=CARTESIAN_POINT('Ctrl Pts',(-3.12986636674479,5.99968545228163,
130.955583309224));
#215985=CARTESIAN_POINT('Ctrl Pts',(-3.2819172246423,5.92036481623276,130.963637524059));
#215986=CARTESIAN_POINT('Ctrl Pts',(-3.43080544743115,5.83533599211421,
130.971691738895));
#215987=CARTESIAN_POINT('Ctrl Pts',(-3.57608202193723,5.74490438322322,
130.979745953731));
#215988=CARTESIAN_POINT('Ctrl Pts',(-3.72146731193647,5.65440510122669,
130.987806195814));
#215989=CARTESIAN_POINT('Ctrl Pts',(-3.86323526487362,5.55849519204986,
130.995866437898));
#215990=CARTESIAN_POINT('Ctrl Pts',(-4.0009693626104,5.45752078873301,131.003926679981));
#215991=CARTESIAN_POINT('Ctrl Pts',(-4.13889602206308,5.35640521627442,
131.011998190836));
#215992=CARTESIAN_POINT('Ctrl Pts',(-4.27277728439513,5.25021125280951,
131.020069701691));
#215993=CARTESIAN_POINT('Ctrl Pts',(-4.4022325033873,5.1393227166739,131.028141212546));
#215994=CARTESIAN_POINT('Ctrl Pts',(-4.41580076188398,5.1277004403816,131.028987191152));
#215995=CARTESIAN_POINT('Ctrl Pts',(-4.42932043529909,5.11602662362992,
131.029833169758));
#215996=CARTESIAN_POINT('Ctrl Pts',(-4.44279111095812,5.10430172936431,
131.030679148365));
#215997=CARTESIAN_POINT('Ctrl Pts',(-4.57265722657723,4.99126608713964,
131.038834934924));
#215998=CARTESIAN_POINT('Ctrl Pts',(-4.69841388164103,4.87309066680269,
131.046990721484));
#215999=CARTESIAN_POINT('Ctrl Pts',(-4.81962338408803,4.75010730779336,
131.055146508044));
#216000=CARTESIAN_POINT('Ctrl Pts',(-4.94068725651242,4.62727171004854,
131.063292495642));
#216001=CARTESIAN_POINT('Ctrl Pts',(-5.05721459776948,4.49963993107349,
131.071438483239));
#216002=CARTESIAN_POINT('Ctrl Pts',(-5.16880017635472,4.36758442813822,
131.079584470836));
#216003=CARTESIAN_POINT('Ctrl Pts',(-5.28027520313374,4.23565975729215,
131.087722387914));
#216004=CARTESIAN_POINT('Ctrl Pts',(-5.38681798059027,4.09932036614932,
131.095860304991));
#216005=CARTESIAN_POINT('Ctrl Pts',(-5.48805961471042,3.95897596170835,
131.103998222068));
#216006=CARTESIAN_POINT('Ctrl Pts',(-5.59112173423524,3.81610794193725,
131.112282471822));
#216007=CARTESIAN_POINT('Ctrl Pts',(-5.68868996036298,3.66908975731962,
131.120566721575));
#216008=CARTESIAN_POINT('Ctrl Pts',(-5.78041677989208,3.51839037782081,
131.128850971329));
#216009=CARTESIAN_POINT('Ctrl Pts',(-5.87040026679604,3.37055514586596,
131.136977773098));
#216010=CARTESIAN_POINT('Ctrl Pts',(-5.95476219107801,3.2191777168747,131.145104574867));
#216011=CARTESIAN_POINT('Ctrl Pts',(-6.03321733768647,3.0647312371951,131.153231376636));
#216012=CARTESIAN_POINT('Ctrl Pts',(-6.11164946317512,2.9103300767975,131.161355793755));
#216013=CARTESIAN_POINT('Ctrl Pts',(-6.18417809602116,2.75286198456227,
131.169480210873));
#216014=CARTESIAN_POINT('Ctrl Pts',(-6.25056370359283,2.59282517484846,
131.177604627992));
#216015=CARTESIAN_POINT('Ctrl Pts',(-6.31694248689683,2.43280481650213,
131.185728209942));
#216016=CARTESIAN_POINT('Ctrl Pts',(-6.37717936281698,2.27021660475608,
131.193851791892));
#216017=CARTESIAN_POINT('Ctrl Pts',(-6.43108274969321,2.10557917604596,
131.201975373842));
#216018=CARTESIAN_POINT('Ctrl Pts',(-6.48684508236007,1.93526395837273,
131.210379110701));
#216019=CARTESIAN_POINT('Ctrl Pts',(-6.53582912103941,1.76275604363099,
131.21878284756));
#216020=CARTESIAN_POINT('Ctrl Pts',(-6.57787883692022,1.58864691067497,
131.22718658442));
#216021=CARTESIAN_POINT('Ctrl Pts',(-6.61855578425189,1.42022180047233,
131.235315970182));
#216022=CARTESIAN_POINT('Ctrl Pts',(-6.65274400306477,1.25029874997547,
131.243445355945));
#216023=CARTESIAN_POINT('Ctrl Pts',(-6.68035434969251,1.07942334722959,
131.251574741708));
#216024=CARTESIAN_POINT('Ctrl Pts',(-6.70936239027104,0.899897871379726,
131.260115654116));
#216025=CARTESIAN_POINT('Ctrl Pts',(-6.73110920848742,0.719321575123651,
131.268656566523));
#216026=CARTESIAN_POINT('Ctrl Pts',(-6.74555314380781,0.538332410379065,
131.277197478931));
#216027=CARTESIAN_POINT('Ctrl Pts',(-6.7599970791282,0.357343245634606,
131.285738391338));
#216028=CARTESIAN_POINT('Ctrl Pts',(-6.76713815815236,0.175941678540549,
131.294279303746));
#216029=CARTESIAN_POINT('Ctrl Pts',(-6.76699797440541,-0.00523587558206445,
131.302820216153));
#216030=CARTESIAN_POINT('Ctrl Pts',(-6.76699797440481,-0.0052358763600726,
131.30282021619));
#216031=CARTESIAN_POINT('Ctrl Pts',(-6.76680115043988,-0.259616858714105,
131.314812020025));
#216032=CARTESIAN_POINT('Ctrl Pts',(-6.75225713895637,-0.513482533726184,
131.326803823861));
#216033=CARTESIAN_POINT('Ctrl Pts',(-6.72355946680874,-0.765530597877477,
131.338795627696));
#216034=CARTESIAN_POINT('Ctrl Pts',(-6.71574816362024,-0.834136296521997,
131.342059711802));
#216035=CARTESIAN_POINT('Ctrl Pts',(-6.70688848524606,-0.902607492201805,
131.345323795908));
#216036=CARTESIAN_POINT('Ctrl Pts',(-6.69698490228259,-0.970918234764971,
131.348587880014));
#216037=CARTESIAN_POINT('Ctrl Pts',(-6.66987228678325,-1.1579296330053,
131.357523823465));
#216038=CARTESIAN_POINT('Ctrl Pts',(-6.63490476040764,-1.34392386470323,
131.366459766916));
#216039=CARTESIAN_POINT('Ctrl Pts',(-6.59217187828101,-1.52825355461753,
131.375395710367));
#216040=CARTESIAN_POINT('Ctrl Pts',(-6.54950323501061,-1.7123061481166,
131.384318220724));
#216041=CARTESIAN_POINT('Ctrl Pts',(-6.49909258658803,-1.8946989417192,
131.393240731082));
#216042=CARTESIAN_POINT('Ctrl Pts',(-6.44108064357375,-2.0747937591432,
131.40216324144));
#216043=CARTESIAN_POINT('Ctrl Pts',(-6.38321084782317,-2.25444728837425,
131.411063888878));
#216044=CARTESIAN_POINT('Ctrl Pts',(-6.31777700975614,-2.43181383409002,
131.419964536317));
#216045=CARTESIAN_POINT('Ctrl Pts',(-6.2449696302004,-2.60627000095437,
131.428865183755));
#216046=CARTESIAN_POINT('Ctrl Pts',(-6.17227476546436,-2.78045656734307,
131.437752076341));
#216047=CARTESIAN_POINT('Ctrl Pts',(-6.09222918802415,-2.95174148937959,
131.446638968927));
#216048=CARTESIAN_POINT('Ctrl Pts',(-6.00507248150573,-3.11951815059035,
131.455525861514));
#216049=CARTESIAN_POINT('Ctrl Pts',(-5.91813980025813,-3.28686356315181,
131.464389911468));
#216050=CARTESIAN_POINT('Ctrl Pts',(-5.82413258159977,-3.45071848031863,
131.473253961423));
#216051=CARTESIAN_POINT('Ctrl Pts',(-5.7233372620906,-3.61049852296954,
131.482118011378));
#216052=CARTESIAN_POINT('Ctrl Pts',(-5.62696882821723,-3.7632610971592,
131.490592756198));
#216053=CARTESIAN_POINT('Ctrl Pts',(-5.52439583947663,-3.91229879426962,
131.499067501019));
#216054=CARTESIAN_POINT('Ctrl Pts',(-5.41590930921664,-4.05711909541002,
131.507542245839));
#216055=CARTESIAN_POINT('Ctrl Pts',(-5.31082571521176,-4.19739676575517,
131.515751160272));
#216056=CARTESIAN_POINT('Ctrl Pts',(-5.20029426297779,-4.33358166469833,
131.523960074704));
#216057=CARTESIAN_POINT('Ctrl Pts',(-5.08467554832049,-4.46523947491193,
131.532168989137));
#216058=CARTESIAN_POINT('Ctrl Pts',(-4.96902934590067,-4.5969285861016,
131.540379855197));
#216059=CARTESIAN_POINT('Ctrl Pts',(-4.84829370641897,-4.72408819672218,
131.548590721257));
#216060=CARTESIAN_POINT('Ctrl Pts',(-4.7228675867584,-4.84631930004069,
131.556801587318));
#216061=CARTESIAN_POINT('Ctrl Pts',(-4.59738928994214,-4.9686012513909,
131.565015869091));
#216062=CARTESIAN_POINT('Ctrl Pts',(-4.46721688047966,-5.08595036258548,
131.573230150864));
#216063=CARTESIAN_POINT('Ctrl Pts',(-4.33278407556525,-5.19800645964664,
131.581444432638));
#216064=CARTESIAN_POINT('Ctrl Pts',(-4.19819995591528,-5.31018868469201,
131.589667960234));
#216065=CARTESIAN_POINT('Ctrl Pts',(-4.05934613642189,-5.41706576802213,
131.59789148783));
#216066=CARTESIAN_POINT('Ctrl Pts',(-3.91668791095474,-5.51831902015287,
131.606115015426));
#216067=CARTESIAN_POINT('Ctrl Pts',(-3.77393824711408,-5.61963717167976,
131.614343813983));
#216068=CARTESIAN_POINT('Ctrl Pts',(-3.62737961373741,-5.71532411219014,
131.622572612541));
#216069=CARTESIAN_POINT('Ctrl Pts',(-3.47750376914315,-5.80510607444819,
131.630801411098));
#216070=CARTESIAN_POINT('Ctrl Pts',(-3.32742163244156,-5.89501161439311,
131.639041535938));
#216071=CARTESIAN_POINT('Ctrl Pts',(-3.17401347602669,-5.97899577119909,
131.647281660778));
#216072=CARTESIAN_POINT('Ctrl Pts',(-3.01779388326723,-6.05683160390933,
131.655521785618));
#216073=CARTESIAN_POINT('Ctrl Pts',(-2.94843883146674,-6.09138750124716,
131.659180060967));
#216074=CARTESIAN_POINT('Ctrl Pts',(-2.87852989137046,-6.12473221224536,
131.662838336315));
#216075=CARTESIAN_POINT('Ctrl Pts',(-2.80811313775106,-6.15684899973923,
131.666496611664));
#216076=CARTESIAN_POINT('Ctrl Pts',(-2.64550035440514,-6.2310160116798,
131.674944634415));
#216077=CARTESIAN_POINT('Ctrl Pts',(-2.47980626960971,-6.29880116643513,
131.683392657166));
#216078=CARTESIAN_POINT('Ctrl Pts',(-2.31155964751762,-6.35995133597485,
131.691840679918));
#216079=CARTESIAN_POINT('Ctrl Pts',(-2.14346709388374,-6.42104550847746,
131.700280966562));
#216080=CARTESIAN_POINT('Ctrl Pts',(-1.97282697409764,-6.47551669336166,
131.708721253207));
#216081=CARTESIAN_POINT('Ctrl Pts',(-1.80018895131744,-6.52315941393085,
131.717161539851));
#216082=CARTESIAN_POINT('Ctrl Pts',(-1.62768244167816,-6.57076584096677,
131.725595396808));
#216083=CARTESIAN_POINT('Ctrl Pts',(-1.45318138346915,-6.61155408513223,
131.734029253764));
#216084=CARTESIAN_POINT('Ctrl Pts',(-1.27725193784871,-6.64536804753971,
131.742463110721));
#216085=CARTESIAN_POINT('Ctrl Pts',(-1.10142946646511,-6.67916144930249,
131.750891839454));
#216086=CARTESIAN_POINT('Ctrl Pts',(-0.924180666001446,-6.70598896138486,
131.759320568188));
#216087=CARTESIAN_POINT('Ctrl Pts',(-0.746083654274415,-6.7257451766198,
131.767749296922));
#216088=CARTESIAN_POINT('Ctrl Pts',(-0.568067585684722,-6.74549241287173,
131.776174194891));
#216089=CARTESIAN_POINT('Ctrl Pts',(-0.38920440544877,-6.75817472396021,
131.78459909286));
#216090=CARTESIAN_POINT('Ctrl Pts',(-0.210079545123407,-6.76373828475945,
131.793023990828));
#216091=CARTESIAN_POINT('Ctrl Pts',(-0.030994343332114,-6.76930061377733,
131.801447023511));
#216092=CARTESIAN_POINT('Ctrl Pts',(0.148352090080952,-6.76774732196723,
131.809870056194));
#216093=CARTESIAN_POINT('Ctrl Pts',(0.327371574155583,-6.75907662720544,
131.818293088877));
#216094=CARTESIAN_POINT('Ctrl Pts',(0.506370802380278,-6.75040691352285,
131.826715168504));
#216095=CARTESIAN_POINT('Ctrl Pts',(0.685042821999834,-6.7346214184739,
131.83513724813));
#216096=CARTESIAN_POINT('Ctrl Pts',(0.862801510431626,-6.71177044851781,
131.843559327756));
#216097=CARTESIAN_POINT('Ctrl Pts',(1.04056489945689,-6.68891887429802,
131.851981630093));
#216098=CARTESIAN_POINT('Ctrl Pts',(1.21741457844043,-6.65900149556442,
131.860403932431));
#216099=CARTESIAN_POINT('Ctrl Pts',(1.39277121929909,-6.6221203047583,131.868826234768));
#216100=CARTESIAN_POINT('Ctrl Pts',(1.56815697713251,-6.58523299003981,
131.87724993558));
#216101=CARTESIAN_POINT('Ctrl Pts',(1.74204887641515,-6.54137962714381,
131.885673636393));
#216102=CARTESIAN_POINT('Ctrl Pts',(1.91387906150491,-6.49071305311929,
131.894097337206));
#216103=CARTESIAN_POINT('Ctrl Pts',(2.08582552565676,-6.44001219255946,
131.902526738414));
#216104=CARTESIAN_POINT('Ctrl Pts',(2.25570716752529,-6.38248900226481,
131.910956139622));
#216105=CARTESIAN_POINT('Ctrl Pts',(2.42297157202295,-6.31834612546422,
131.91938554083));
#216106=CARTESIAN_POINT('Ctrl Pts',(2.59029565623062,-6.25418036257319,
131.927817949638));
#216107=CARTESIAN_POINT('Ctrl Pts',(2.75500033192922,-6.18339032881242,
131.936250358445));
#216108=CARTESIAN_POINT('Ctrl Pts',(2.91655384726697,-6.10622654804031,
131.944682767252));
#216109=CARTESIAN_POINT('Ctrl Pts',(3.0782568366238,-6.02899137309014,131.953122977969));
#216110=CARTESIAN_POINT('Ctrl Pts',(3.2368025420005,-5.94537081795523,131.961563188686));
#216111=CARTESIAN_POINT('Ctrl Pts',(3.39168348224042,-5.85566154728033,
131.970003399404));
#216112=CARTESIAN_POINT('Ctrl Pts',(3.4797771206816,-5.8046364434592,131.974804047373));
#216113=CARTESIAN_POINT('Ctrl Pts',(3.56668565016117,-5.75164237058268,
131.979604695343));
#216114=CARTESIAN_POINT('Ctrl Pts',(3.65231993181012,-5.69674013061001,
131.984405343313));
#216115=CARTESIAN_POINT('Ctrl Pts',(3.79751671734005,-5.60365090735823,
131.992545058392));
#216116=CARTESIAN_POINT('Ctrl Pts',(3.93933796368613,-5.50488787645263,
132.000684773471));
#216117=CARTESIAN_POINT('Ctrl Pts',(4.07730761878017,-5.4007269493872,132.008824488551));
#216118=CARTESIAN_POINT('Ctrl Pts',(4.21515660643658,-5.29665712084747,
132.016957084684));
#216119=CARTESIAN_POINT('Ctrl Pts',(4.34916041770699,-5.18719901234504,
132.025089680817));
#216120=CARTESIAN_POINT('Ctrl Pts',(4.47887038021226,-5.07267277845292,
132.03322227695));
#216121=CARTESIAN_POINT('Ctrl Pts',(4.60849166602303,-4.95822484084321,
132.041349313204));
#216122=CARTESIAN_POINT('Ctrl Pts',(4.73382467411888,-4.83871591755658,
132.049476349458));
#216123=CARTESIAN_POINT('Ctrl Pts',(4.85445238991508,-4.71450750280957,
132.057603385712));
#216124=CARTESIAN_POINT('Ctrl Pts',(4.97502244347042,-4.59035846194261,
132.065726537095));
#216125=CARTESIAN_POINT('Ctrl Pts',(5.09089142905951,-4.46151466516838,
132.073849688477));
#216126=CARTESIAN_POINT('Ctrl Pts',(5.20167793395675,-4.3283756388959,132.08197283986));
#216127=CARTESIAN_POINT('Ctrl Pts',(5.31243330701791,-4.19527402568509,
132.090093708577));
#216128=CARTESIAN_POINT('Ctrl Pts',(5.41810881068375,-4.05787986882479,
132.098214577293));
#216129=CARTESIAN_POINT('Ctrl Pts',(5.51836223316075,-3.91662702636147,
132.10633544601));
#216130=CARTESIAN_POINT('Ctrl Pts',(5.6186210737078,-3.77536655006606,132.114456753608));
#216131=CARTESIAN_POINT('Ctrl Pts',(5.71345703244159,-3.63024726789743,
132.122578061207));
#216132=CARTESIAN_POINT('Ctrl Pts',(5.80257018197704,-3.48173351697556,
132.130699368805));
#216133=CARTESIAN_POINT('Ctrl Pts',(5.84887646896811,-3.40456061479266,
132.13491948225));
#216134=CARTESIAN_POINT('Ctrl Pts',(5.89363819746646,-3.3264716096768,132.139139595694));
#216135=CARTESIAN_POINT('Ctrl Pts',(5.93681807242065,-3.24753447633425,
132.143359709138));
#216136=CARTESIAN_POINT('Ctrl Pts',(6.02874615254374,-3.07948074467572,
132.152344147542));
#216137=CARTESIAN_POINT('Ctrl Pts',(6.11345645332912,-2.9076648672125,132.161328585946));
#216138=CARTESIAN_POINT('Ctrl Pts',(6.19068775269391,-2.73270454836334,
132.17031302435));
#216139=CARTESIAN_POINT('Ctrl Pts',(6.26805234864637,-2.55744225850405,
132.179312969356));
#216140=CARTESIAN_POINT('Ctrl Pts',(6.33791204644033,-2.37902489855576,
132.188312914361));
#216141=CARTESIAN_POINT('Ctrl Pts',(6.40005430909273,-2.19808867898082,
132.197312859367));
#216142=CARTESIAN_POINT('Ctrl Pts',(6.46234301156852,-2.01672607859981,
132.206334012972));
#216143=CARTESIAN_POINT('Ctrl Pts',(6.51687781307106,-1.83283296902651,
132.215355166577));
#216144=CARTESIAN_POINT('Ctrl Pts',(6.56349572446274,-1.64706189166021,
132.224376320181));
#216145=CARTESIAN_POINT('Ctrl Pts',(6.61016106994521,-1.46110179076443,
132.233406652881));
#216146=CARTESIAN_POINT('Ctrl Pts',(6.64889338012126,-1.27326013770002,
132.242436985581));
#216147=CARTESIAN_POINT('Ctrl Pts',(6.67958082179362,-1.08419972566262,
132.25146731828));
#216148=CARTESIAN_POINT('Ctrl Pts',(6.71031176859167,-0.894871285515337,
132.260510453147));
#216149=CARTESIAN_POINT('Ctrl Pts',(6.73297500382871,-0.704320867581619,
132.269553588014));
#216150=CARTESIAN_POINT('Ctrl Pts',(6.74751031811957,-0.513218770964102,
132.278596722881));
#216151=CARTESIAN_POINT('Ctrl Pts',(6.76021753273533,-0.346151495592786,
132.286502506908));
#216152=CARTESIAN_POINT('Ctrl Pts',(6.76671353600646,-0.178662752507999,
132.294408290935));
#216153=CARTESIAN_POINT('Ctrl Pts',(6.76699072954348,-0.0112011728232508,
132.302314074962));
#216154=CARTESIAN_POINT('Ctrl Pts',(6.7672941356706,0.172096280214045,132.310967463275));
#216155=CARTESIAN_POINT('Ctrl Pts',(6.76014593713099,0.355523123183739,
132.319620851587));
#216156=CARTESIAN_POINT('Ctrl Pts',(6.74554260586999,0.538464439301936,
132.3282742399));
#216157=CARTESIAN_POINT('Ctrl Pts',(6.73095276182253,0.721236796122272,
132.336919636194));
#216158=CARTESIAN_POINT('Ctrl Pts',(6.70892154213067,0.903524218465778,
132.345565032488));
#216159=CARTESIAN_POINT('Ctrl Pts',(6.67949743572514,1.08471332901432,132.354210428782));
#216160=CARTESIAN_POINT('Ctrl Pts',(6.64913362291565,1.27168900671169,132.363131929782));
#216161=CARTESIAN_POINT('Ctrl Pts',(6.6108968903199,1.45749473334196,132.372053430783));
#216162=CARTESIAN_POINT('Ctrl Pts',(6.56489857922134,1.64146143559257,132.380974931783));
#216163=CARTESIAN_POINT('Ctrl Pts',(6.52040873093351,1.81939515701996,132.389603862205));
#216164=CARTESIAN_POINT('Ctrl Pts',(6.46865835845453,1.99560822897561,132.398232792628));
#216165=CARTESIAN_POINT('Ctrl Pts',(6.40980027306129,2.16950442715923,132.40686172305));
#216166=CARTESIAN_POINT('Ctrl Pts',(6.34794874411817,2.35224475354242,132.415929509339));
#216167=CARTESIAN_POINT('Ctrl Pts',(6.27824773848932,2.5324260628253,132.424997295629));
#216168=CARTESIAN_POINT('Ctrl Pts',(6.20093451363,2.70937265020379,132.434065081918));
#216169=CARTESIAN_POINT('Ctrl Pts',(6.12362128877068,2.88631923758228,132.443132868208));
#216170=CARTESIAN_POINT('Ctrl Pts',(6.03869596877439,3.06003073111488,132.452200654497));
#216171=CARTESIAN_POINT('Ctrl Pts',(5.94645565075196,3.22985358702838,132.461268440787));
#216172=CARTESIAN_POINT('Ctrl Pts',(5.86075439919666,3.38763742392869,132.469693396929));
#216173=CARTESIAN_POINT('Ctrl Pts',(5.76877634762448,3.54199530509277,132.478118353071));
#216174=CARTESIAN_POINT('Ctrl Pts',(5.67082881403919,3.6924232641807,132.486543309213));
#216175=CARTESIAN_POINT('Ctrl Pts',(5.57285854588218,3.84288613905569,132.494970220868));
#216176=CARTESIAN_POINT('Ctrl Pts',(5.46891621402277,3.98941699522619,132.503397132524));
#216177=CARTESIAN_POINT('Ctrl Pts',(5.35935229455184,4.13154111475149,132.51182404418));
#216178=CARTESIAN_POINT('Ctrl Pts',(5.24974808415041,4.27371749886397,132.52025405474));
#216179=CARTESIAN_POINT('Ctrl Pts',(5.13451836654412,4.41148365264945,132.5286840653));
#216180=CARTESIAN_POINT('Ctrl Pts',(5.01405393209504,4.54439788817422,132.537114075861));
#216181=CARTESIAN_POINT('Ctrl Pts',(4.89347852831402,4.67743456152877,132.545551851971));
#216182=CARTESIAN_POINT('Ctrl Pts',(4.76765899638341,4.80561014110518,132.553989628082));
#216183=CARTESIAN_POINT('Ctrl Pts',(4.63702380340669,4.92851897091203,132.562427404193));
#216184=CARTESIAN_POINT('Ctrl Pts',(4.5063200365742,5.051492318803,132.570869609514));
#216185=CARTESIAN_POINT('Ctrl Pts',(4.37079581374232,5.16919318187508,132.579311814836));
#216186=CARTESIAN_POINT('Ctrl Pts',(4.2309131390712,5.28125581747701,132.587754020158));
#216187=CARTESIAN_POINT('Ctrl Pts',(4.09088289586226,5.39343667300373,132.596205131542));
#216188=CARTESIAN_POINT('Ctrl Pts',(3.94648527943532,5.49996721837308,132.604656242927));
#216189=CARTESIAN_POINT('Ctrl Pts',(3.79821261674009,5.60052407530192,132.613107354311));
#216190=CARTESIAN_POINT('Ctrl Pts',(3.7565996654621,5.6287455121601,132.615479171745));
#216191=CARTESIAN_POINT('Ctrl Pts',(3.71468165514017,5.65649670150209,132.617850989178));
#216192=CARTESIAN_POINT('Ctrl Pts',(3.67246982934908,5.68377113829548,132.620222806612));
#216193=CARTESIAN_POINT('Ctrl Pts',(3.52444787496525,5.77941294869373,132.628539932094));
#216194=CARTESIAN_POINT('Ctrl Pts',(3.37254386156039,5.86936147603194,132.636857057577));
#216195=CARTESIAN_POINT('Ctrl Pts',(3.21722995071989,5.95329492333371,132.645174183059));
#216196=CARTESIAN_POINT('Ctrl Pts',(3.17806936885764,5.97445775811299,132.647271248747));
#216197=CARTESIAN_POINT('Ctrl Pts',(3.13869216104785,5.99523839979182,132.649368314435));
#216198=CARTESIAN_POINT('Ctrl Pts',(3.09910619832128,6.01563211736943,132.651465380124));
#216199=CARTESIAN_POINT('Origin',(0.,0.,4.30282021618968));
#216200=CARTESIAN_POINT('',(3.09910619832134,6.0156321173694,135.045755263024));
#216201=CARTESIAN_POINT('',(3.0991061983213,6.01563211736942,134.651530974814));
#216202=CARTESIAN_POINT('',(3.09910619832133,6.0156321173694,4.30282021618968));
#216203=CARTESIAN_POINT('',(-6.767,6.55463713633477E-12,133.69717978381));
#216204=CARTESIAN_POINT('Ctrl Pts',(-6.767,6.93929656985413E-12,133.69717978381));
#216205=CARTESIAN_POINT('Ctrl Pts',(-6.76700000000019,-0.186007249519898,
133.705929295621));
#216206=CARTESIAN_POINT('Ctrl Pts',(-6.75932637294559,-0.372014355742914,
133.714678807432));
#216207=CARTESIAN_POINT('Ctrl Pts',(-6.74400518264238,-0.55738953748047,
133.723428319244));
#216208=CARTESIAN_POINT('Ctrl Pts',(-6.72868405705164,-0.742763936244698,
133.732177794099));
#216209=CARTESIAN_POINT('Ctrl Pts',(-6.70571545645824,-0.927506130235109,
133.740927268955));
#216210=CARTESIAN_POINT('Ctrl Pts',(-6.67517739404921,-1.11098863989439,
133.749676743811));
#216211=CARTESIAN_POINT('Ctrl Pts',(-6.6446394580881,-1.29447038981393,
133.758426182438));
#216212=CARTESIAN_POINT('Ctrl Pts',(-6.60653217008474,-1.47669218313153,
133.767175621065));
#216213=CARTESIAN_POINT('Ctrl Pts',(-6.56098496092805,-1.65703510598779,
133.775925059692));
#216214=CARTESIAN_POINT('Ctrl Pts',(-6.51543793658437,-1.83737729708204,
133.784674462817));
#216215=CARTESIAN_POINT('Ctrl Pts',(-6.46245112167572,-2.01584035510443,
133.793423865942));
#216216=CARTESIAN_POINT('Ctrl Pts',(-6.40220448374415,-2.19181813760319,
133.802173269067));
#216217=CARTESIAN_POINT('Ctrl Pts',(-6.34195808526676,-2.36779522066682,
133.810922637417));
#216218=CARTESIAN_POINT('Ctrl Pts',(-6.27445201433287,-2.54128677683714,
133.819672005767));
#216219=CARTESIAN_POINT('Ctrl Pts',(-6.19991555072094,-2.71170355384371,
133.828421374117));
#216220=CARTESIAN_POINT('Ctrl Pts',(-6.12537937716898,-2.88211966767039,
133.837170708419));
#216221=CARTESIAN_POINT('Ctrl Pts',(-6.0438129805274,-3.0494607637135,133.845920042721));
#216222=CARTESIAN_POINT('Ctrl Pts',(-5.95549339336065,-3.21315848374114,
133.854669377023));
#216223=CARTESIAN_POINT('Ctrl Pts',(-5.86717414255658,-3.3768555803306,
133.863418678003));
#216224=CARTESIAN_POINT('Ctrl Pts',(-5.77210188876863,-3.53690907646324,
133.872167978983));
#216225=CARTESIAN_POINT('Ctrl Pts',(-5.67059953347276,-3.69277536968857,
133.880917279963));
#216226=CARTESIAN_POINT('Ctrl Pts',(-5.56909755631678,-3.84864108224498,
133.889666548349));
#216227=CARTESIAN_POINT('Ctrl Pts',(-5.46116568197157,-4.00031938297098,
133.898415816734));
#216228=CARTESIAN_POINT('Ctrl Pts',(-5.34717048533923,-4.14729511859441,
133.907165085119));
#216229=CARTESIAN_POINT('Ctrl Pts',(-5.23317570392182,-4.29427031887494,
133.915914321636));
#216230=CARTESIAN_POINT('Ctrl Pts',(-5.11311782003887,-4.43654276189117,
133.924663558153));
#216231=CARTESIAN_POINT('Ctrl Pts',(-4.98740458985153,-4.57362924351416,
133.93341279467));
#216232=CARTESIAN_POINT('Ctrl Pts',(-4.86169180712161,-4.71071523719835,
133.942162000046));
#216233=CARTESIAN_POINT('Ctrl Pts',(-4.73032391204608,-4.84261509522811,
133.950911205421));
#216234=CARTESIAN_POINT('Ctrl Pts',(-4.59374707014054,-4.9688808453791,
133.959660410797));
#216235=CARTESIAN_POINT('Ctrl Pts',(-4.45717070301936,-5.09514615659033,
133.968409585757));
#216236=CARTESIAN_POINT('Ctrl Pts',(-4.31538563571569,-5.21577720459089,
133.977158760717));
#216237=CARTESIAN_POINT('Ctrl Pts',(-4.16887341030076,-5.33036429232443,
133.985907935678));
#216238=CARTESIAN_POINT('Ctrl Pts',(-4.02236168204279,-5.44495099123193,
133.99465708095));
#216239=CARTESIAN_POINT('Ctrl Pts',(-3.87112305348743,-5.55349359438199,
134.003406226222));
#216240=CARTESIAN_POINT('Ctrl Pts',(-3.71567117018342,-5.65562346298512,
134.012155371494));
#216241=CARTESIAN_POINT('Ctrl Pts',(-3.56021980146412,-5.75775299351277,
134.020904487804));
#216242=CARTESIAN_POINT('Ctrl Pts',(-3.40055544538953,-5.85346967463522,
134.029653604114));
#216243=CARTESIAN_POINT('Ctrl Pts',(-3.23722035987468,-5.94244842986566,
134.038402720424));
#216244=CARTESIAN_POINT('Ctrl Pts',(-3.07388580147812,-6.03142689794207,
134.047151808499));
#216245=CARTESIAN_POINT('Ctrl Pts',(-2.90688078897226,-6.11366734656473,
134.055900896574));
#216246=CARTESIAN_POINT('Ctrl Pts',(-2.73677250722034,-6.1888904695206,
134.064649984649));
#216247=CARTESIAN_POINT('Ctrl Pts',(-2.56666476032147,-6.26411335596055,
134.073399045215));
#216248=CARTESIAN_POINT('Ctrl Pts',(-2.3934540257583,-6.33231884500305,
134.082148105781));
#216249=CARTESIAN_POINT('Ctrl Pts',(-2.21772856066254,-6.39327529762497,
134.090897166347));
#216250=CARTESIAN_POINT('Ctrl Pts',(-2.04200363349168,-6.45423156364905,
134.099646200131));
#216251=CARTESIAN_POINT('Ctrl Pts',(-1.86376426189924,-6.50793874375474,
134.108395233914));
#216252=CARTESIAN_POINT('Ctrl Pts',(-1.6836157775379,-6.55421443909379,
134.117144267698));
#216253=CARTESIAN_POINT('Ctrl Pts',(-1.5034678296848,-6.60048999661712,
134.125893275426));
#216254=CARTESIAN_POINT('Ctrl Pts',(-1.32141105795712,-6.63933404237567,
134.134642283154));
#216255=CARTESIAN_POINT('Ctrl Pts',(-1.13806375487792,-6.67061465607429,
134.143391290882));
#216256=CARTESIAN_POINT('Ctrl Pts',(-0.954716982610654,-6.70189517921188,
134.15214027328));
#216257=CARTESIAN_POINT('Ctrl Pts',(-0.770079968909707,-6.72561226592142,
134.160889255678));
#216258=CARTESIAN_POINT('Ctrl Pts',(-0.584779765565736,-6.74168536983037,
134.169638238077));
#216259=CARTESIAN_POINT('Ctrl Pts',(-0.391489830658705,-6.7584515101381,
134.178764457087));
#216260=CARTESIAN_POINT('Ctrl Pts',(-0.197478578245647,-6.76689983031604,
134.187890676096));
#216261=CARTESIAN_POINT('Ctrl Pts',(-0.00346287645855221,-6.76699911397117,
134.197016895106));
#216262=CARTESIAN_POINT('Ctrl Pts',(0.184489834647668,-6.76709529501208,
134.205857919772));
#216263=CARTESIAN_POINT('Ctrl Pts',(0.372446404243251,-6.75935639738202,
134.214698944438));
#216264=CARTESIAN_POINT('Ctrl Pts',(0.559755019482324,-6.74380925873236,
134.223539969104));
#216265=CARTESIAN_POINT('Ctrl Pts',(0.745134705515861,-6.72842222659871,
134.232289947714));
#216266=CARTESIAN_POINT('Ctrl Pts',(0.929879431222757,-6.70538706057604,
134.241039926323));
#216267=CARTESIAN_POINT('Ctrl Pts',(1.11336163626255,-6.67478200894222,
134.249789904933));
#216268=CARTESIAN_POINT('Ctrl Pts',(1.29684196300168,-6.64417727061121,
134.25853979397));
#216269=CARTESIAN_POINT('Ctrl Pts',(1.47905951216979,-6.6060028489071,134.267289683006));
#216270=CARTESIAN_POINT('Ctrl Pts',(1.65939532066573,-6.5603884160736,134.276039572043));
#216271=CARTESIAN_POINT('Ctrl Pts',(1.83972934300294,-6.514774435034,134.284789374415));
#216272=CARTESIAN_POINT('Ctrl Pts',(2.01818138405761,-6.46172066062299,
134.293539176787));
#216273=CARTESIAN_POINT('Ctrl Pts',(2.194145283537,-6.4014073042365,134.302288979159));
#216274=CARTESIAN_POINT('Ctrl Pts',(2.37010749863504,-6.34109452518828,
134.311038697775));
#216275=CARTESIAN_POINT('Ctrl Pts',(2.54358134865968,-6.27352239616703,
134.319788416392));
#216276=CARTESIAN_POINT('Ctrl Pts',(2.71397759435069,-6.19892043967032,
134.328538135008));
#216277=CARTESIAN_POINT('Ctrl Pts',(2.88437226557649,-6.12431917249739,
134.337287772777));
#216278=CARTESIAN_POINT('Ctrl Pts',(3.05168912680493,-6.04268832279033,
134.346037410546));
#216279=CARTESIAN_POINT('Ctrl Pts',(3.21535986273404,-5.95430516123577,
134.354787048314));
#216280=CARTESIAN_POINT('Ctrl Pts',(3.37902914072414,-5.86592278697687,
134.363536608143));
#216281=CARTESIAN_POINT('Ctrl Pts',(3.53905210621167,-5.7707883574219,134.372286167972));
#216282=CARTESIAN_POINT('Ctrl Pts',(3.69488522831315,-5.66922500431878,
134.381035727801));
#216283=CARTESIAN_POINT('Ctrl Pts',(3.85071701406569,-5.5676625221735,134.389785212599));
#216284=CARTESIAN_POINT('Ctrl Pts',(4.00235878822045,-5.45967138329633,
134.398534697396));
#216285=CARTESIAN_POINT('Ctrl Pts',(4.14929549610978,-5.34561838199877,
134.407284182193));
#216286=CARTESIAN_POINT('Ctrl Pts',(4.29623099275755,-5.23156632087291,
134.416033594865));
#216287=CARTESIAN_POINT('Ctrl Pts',(4.43846127435706,-5.11145267305244,
134.424783007538));
#216288=CARTESIAN_POINT('Ctrl Pts',(4.57550326054133,-4.98568540050169,
134.433532420211));
#216289=CARTESIAN_POINT('Ctrl Pts',(4.71254416257476,-4.85991912290656,
134.442281763666));
#216290=CARTESIAN_POINT('Ctrl Pts',(4.84439664018462,-4.72849950385725,
134.451031107121));
#216291=CARTESIAN_POINT('Ctrl Pts',(4.97061286794451,-4.59187289861386,
134.459780450576));
#216292=CARTESIAN_POINT('Ctrl Pts',(5.09682813912402,-4.45524732885008,
134.468529727721));
#216293=CARTESIAN_POINT('Ctrl Pts',(5.21740705147567,-4.31341506236116,
134.477279004866));
#216294=CARTESIAN_POINT('Ctrl Pts',(5.33194007545436,-4.16685781276057,
134.486028282011));
#216295=CARTESIAN_POINT('Ctrl Pts',(5.44647226944229,-4.02030162522188,
134.494777495752));
#216296=CARTESIAN_POINT('Ctrl Pts',(5.55495848627862,-3.86902074888294,
134.503526709493));
#216297=CARTESIAN_POINT('Ctrl Pts',(5.65703027291542,-3.71352898081037,
134.512275923234));
#216298=CARTESIAN_POINT('Ctrl Pts',(5.75910135376767,-3.55803828789961,
134.521025076478));
#216299=CARTESIAN_POINT('Ctrl Pts',(5.85475793592538,-3.39833700107082,
134.529774229722));
#216300=CARTESIAN_POINT('Ctrl Pts',(5.94367514427199,-3.2349675082392,134.538523382966));
#216301=CARTESIAN_POINT('Ctrl Pts',(6.03259176732455,-3.07159909078089,
134.547272478619));
#216302=CARTESIAN_POINT('Ctrl Pts',(6.11476896835753,-2.90456276731794,
134.556021574272));
#216303=CARTESIAN_POINT('Ctrl Pts',(6.18992765547729,-2.73442583003406,
134.564770669925));
#216304=CARTESIAN_POINT('Ctrl Pts',(6.26508587282905,-2.56428995616535,
134.573519710893));
#216305=CARTESIAN_POINT('Ctrl Pts',(6.33322554827019,-2.39105376935576,
134.582268751861));
#216306=CARTESIAN_POINT('Ctrl Pts',(6.39411526732898,-2.21530561054463,
134.591017792829));
#216307=CARTESIAN_POINT('Ctrl Pts',(6.45500462602718,-2.03955849185506,
134.599766782018));
#216308=CARTESIAN_POINT('Ctrl Pts',(6.50864402040616,-1.86129970164976,
134.608515771207));
#216309=CARTESIAN_POINT('Ctrl Pts',(6.55485128368484,-1.68113463136514,
134.617264760396));
#216310=CARTESIAN_POINT('Ctrl Pts',(6.6019980955422,-1.49730620117337,134.626191645867));
#216311=CARTESIAN_POINT('Ctrl Pts',(6.64140720707778,-1.31149343246178,
134.635118531339));
#216312=CARTESIAN_POINT('Ctrl Pts',(6.67293928722801,-1.12435326698016,
134.64404541681));
#216313=CARTESIAN_POINT('Ctrl Pts',(6.70384625876187,-0.940923067011545,
134.652795330988));
#216314=CARTESIAN_POINT('Ctrl Pts',(6.7271855457974,-0.756217899526663,
134.661545245165));
#216315=CARTESIAN_POINT('Ctrl Pts',(6.74287786815285,-0.570865181259529,
134.670295159342));
#216316=CARTESIAN_POINT('Ctrl Pts',(6.75856988190817,-0.38551610807906,
134.679044901447));
#216317=CARTESIAN_POINT('Ctrl Pts',(6.76661520773387,-0.199519795231536,
134.687794643551));
#216318=CARTESIAN_POINT('Ctrl Pts',(6.76698651789578,-0.0135080204609056,
134.696544385656));
#216319=CARTESIAN_POINT('Ctrl Pts',(6.76735782124916,0.172500343507633,
134.705293967321));
#216320=CARTESIAN_POINT('Ctrl Pts',(6.76005538995212,0.35852388220553,134.714043548986));
#216321=CARTESIAN_POINT('Ctrl Pts',(6.74510402742405,0.543930748558928,
134.722793130651));
#216322=CARTESIAN_POINT('Ctrl Pts',(6.73015291918089,0.729334461609797,
134.731542563507));
#216323=CARTESIAN_POINT('Ctrl Pts',(6.70755316306669,0.914121237629259,
134.740291996364));
#216324=CARTESIAN_POINT('Ctrl Pts',(6.67738151874663,1.09766345165582,134.749041429221));
#216325=CARTESIAN_POINT('Ctrl Pts',(6.64721034747673,1.28120278799127,134.757790724898));
#216326=CARTESIAN_POINT('Ctrl Pts',(6.6094675720526,1.46349731859795,134.766540020576));
#216327=CARTESIAN_POINT('Ctrl Pts',(6.56428138111656,1.64392790277631,134.775289316253));
#216328=CARTESIAN_POINT('Ctrl Pts',(6.51909583860002,1.82435589778513,134.784038486379));
#216329=CARTESIAN_POINT('Ctrl Pts',(6.46646716393047,2.0029197219171,134.792787656505));
#216330=CARTESIAN_POINT('Ctrl Pts',(6.40657409873076,2.17901292274098,134.80153682663));
#216331=CARTESIAN_POINT('Ctrl Pts',(6.34668181342285,2.35510383058415,134.810285882829));
#216332=CARTESIAN_POINT('Ctrl Pts',(6.27952541914275,2.52872390822022,134.819034939028));
#216333=CARTESIAN_POINT('Ctrl Pts',(6.20533299175757,2.69928350889732,134.827783995228));
#216334=CARTESIAN_POINT('Ctrl Pts',(6.12831602991791,2.8763363796511,134.836866131386));
#216335=CARTESIAN_POINT('Ctrl Pts',(6.04371690605511,3.05009086600988,134.845948267544));
#216336=CARTESIAN_POINT('Ctrl Pts',(5.95184520316867,3.21991112882299,134.855030403702));
#216337=CARTESIAN_POINT('Ctrl Pts',(5.86333549509521,3.38351691182591,134.863780184046));
#216338=CARTESIAN_POINT('Ctrl Pts',(5.76807618099625,3.54347103711587,134.872529964389));
#216339=CARTESIAN_POINT('Ctrl Pts',(5.66639083309281,3.69923018027288,134.881279744733));
#216340=CARTESIAN_POINT('Ctrl Pts',(5.56470914082474,3.85498372381656,134.890029210518));
#216341=CARTESIAN_POINT('Ctrl Pts',(5.45660203372347,4.00654234701616,134.898778676303));
#216342=CARTESIAN_POINT('Ctrl Pts',(5.34243669839503,4.153391279863,134.907528142088));
#216343=CARTESIAN_POINT('Ctrl Pts',(5.22827486050883,4.30023571400926,134.916277339834));
#216344=CARTESIAN_POINT('Ctrl Pts',(5.10805534167406,4.44237052028131,134.92502653758));
#216345=CARTESIAN_POINT('Ctrl Pts',(4.98218644340249,4.57931296628397,134.933775735326));
#216346=CARTESIAN_POINT('Ctrl Pts',(4.85632073219899,4.71625194483038,134.942524711537));
#216347=CARTESIAN_POINT('Ctrl Pts',(4.72480612170647,4.84799861524188,134.951273687749));
#216348=CARTESIAN_POINT('Ctrl Pts',(4.58808925235655,4.97410554898168,134.960022663961));
#216349=CARTESIAN_POINT('Ctrl Pts',(4.45136349474403,5.10022068120896,134.968772208962));
#216350=CARTESIAN_POINT('Ctrl Pts',(4.30943501210447,5.22069514871531,134.977521753964));
#216351=CARTESIAN_POINT('Ctrl Pts',(4.1627858743216,5.33511975165962,134.986271298966));
#216352=CARTESIAN_POINT('Ctrl Pts',(4.01614535740829,5.44953762807562,134.995020329619));
#216353=CARTESIAN_POINT('Ctrl Pts',(3.86478496658306,5.55790617532518,135.003769360273));
#216354=CARTESIAN_POINT('Ctrl Pts',(3.7092187474758,5.65985735539104,135.012518390927));
#216355=CARTESIAN_POINT('Ctrl Pts',(3.55365041606297,5.76180991976802,135.021267540376));
#216356=CARTESIAN_POINT('Ctrl Pts',(3.3938763817493,5.85734478552577,135.030016689826));
#216357=CARTESIAN_POINT('Ctrl Pts',(3.23043927904957,5.94613749121005,135.038765839276));
#216358=CARTESIAN_POINT('Ctrl Pts',(3.18691767070709,5.96978206944,135.041095647192));
#216359=CARTESIAN_POINT('Ctrl Pts',(3.14313645919769,5.99294880633354,135.043425455108));
#216360=CARTESIAN_POINT('Ctrl Pts',(3.09910619832134,6.0156321173694,135.045755263024));
#216361=CARTESIAN_POINT('Ctrl Pts',(3.09910619832141,6.01563211736936,133.045915245968));
#216362=CARTESIAN_POINT('Ctrl Pts',(2.93176423559343,6.10184259430862,133.05474838379));
#216363=CARTESIAN_POINT('Ctrl Pts',(2.76066887234771,6.18114604978671,133.063581521611));
#216364=CARTESIAN_POINT('Ctrl Pts',(2.58638754591484,6.25323024222974,133.072414659433));
#216365=CARTESIAN_POINT('Ctrl Pts',(2.4244223041923,6.32022040056955,133.080623578493));
#216366=CARTESIAN_POINT('Ctrl Pts',(2.25986139745912,6.38091035543149,133.088832497554));
#216367=CARTESIAN_POINT('Ctrl Pts',(2.0932365976775,6.4351106863941,133.097041416615));
#216368=CARTESIAN_POINT('Ctrl Pts',(1.92657218276064,6.48932390351437,133.10525228735));
#216369=CARTESIAN_POINT('Ctrl Pts',(1.75784323582365,6.53704431267304,133.113463158085));
#216370=CARTESIAN_POINT('Ctrl Pts',(1.58759649279234,6.57813243831967,133.121674028821));
#216371=CARTESIAN_POINT('Ctrl Pts',(1.41727892642892,6.61923765679237,133.129888315312));
#216372=CARTESIAN_POINT('Ctrl Pts',(1.24544265192892,6.65370501165978,133.138102601803));
#216373=CARTESIAN_POINT('Ctrl Pts',(1.07264447500648,6.6814461630876,133.146316888293));
#216374=CARTESIAN_POINT('Ctrl Pts',(0.899651799273974,6.70921853950309,
133.154540420651));
#216375=CARTESIAN_POINT('Ctrl Pts',(0.725695410321514,6.7302495344213,133.162763953009));
#216376=CARTESIAN_POINT('Ctrl Pts',(0.551338092464835,6.74450259899107,
133.170987485366));
#216377=CARTESIAN_POINT('Ctrl Pts',(0.376869017819126,6.75876479926417,
133.179216288713));
#216378=CARTESIAN_POINT('Ctrl Pts',(0.20199885682681,6.76624039371214,133.187445092061));
#216379=CARTESIAN_POINT('Ctrl Pts',(0.0272902215745766,6.76694497124119,
133.195673895408));
#216380=CARTESIAN_POINT('Ctrl Pts',(-0.147658886335797,6.76765051856564,
133.203914025054));
#216381=CARTESIAN_POINT('Ctrl Pts',(-0.322445669605848,6.7615664459333,
133.2121541547));
#216382=CARTESIAN_POINT('Ctrl Pts',(-0.496511789836325,6.74876025967389,
133.220394284346));
#216383=CARTESIAN_POINT('Ctrl Pts',(-0.573789318755462,6.74307488892112,
133.224052531316));
#216384=CARTESIAN_POINT('Ctrl Pts',(-0.650924926912838,6.73606529465226,
133.227710778287));
#216385=CARTESIAN_POINT('Ctrl Pts',(-0.727870451698626,6.72774060183239,
133.231369025257));
#216386=CARTESIAN_POINT('Ctrl Pts',(-0.905561349639612,6.70851632405453,
133.239817043396));
#216387=CARTESIAN_POINT('Ctrl Pts',(-1.08264444933174,6.68223138116163,
133.248265061535));
#216388=CARTESIAN_POINT('Ctrl Pts',(-1.2585358525355,6.64893799849891,133.256713079674));
#216389=CARTESIAN_POINT('Ctrl Pts',(-1.43426618613749,6.61567510369285,
133.265153361682));
#216390=CARTESIAN_POINT('Ctrl Pts',(-1.60880667236696,6.57541662354257,
133.27359364369));
#216391=CARTESIAN_POINT('Ctrl Pts',(-1.78157976401296,6.52826642719639,
133.282033925697));
#216392=CARTESIAN_POINT('Ctrl Pts',(-1.95422123926741,6.48115214928314,
133.290467778004));
#216393=CARTESIAN_POINT('Ctrl Pts',(-2.12509768333322,6.42715670861028,
133.29890163031));
#216394=CARTESIAN_POINT('Ctrl Pts',(-2.29364256579097,6.36643485636913,
133.307335482616));
#216395=CARTESIAN_POINT('Ctrl Pts',(-2.46208496408001,6.30574992621342,
133.315764206695));
#216396=CARTESIAN_POINT('Ctrl Pts',(-2.62819831430491,6.23834685164277,
133.324192930775));
#216397=CARTESIAN_POINT('Ctrl Pts',(-2.79143167869532,6.16443007772627,
133.332621654855));
#216398=CARTESIAN_POINT('Ctrl Pts',(-2.95459085539805,6.0905468981338,133.341046548176));
#216399=CARTESIAN_POINT('Ctrl Pts',(-3.11487235295816,6.01015605960155,
133.349471441497));
#216400=CARTESIAN_POINT('Ctrl Pts',(-3.27174527324697,5.92351009680798,
133.357896334819));
#216401=CARTESIAN_POINT('Ctrl Pts',(-3.42858346226766,5.83688331721162,
133.36631936289));
#216402=CARTESIAN_POINT('Ctrl Pts',(-3.58201428570271,5.74400433329873,
133.374742390961));
#216403=CARTESIAN_POINT('Ctrl Pts',(-3.7315310453231,5.64517183598426,133.383165419033));
#216404=CARTESIAN_POINT('Ctrl Pts',(-3.88103088779537,5.54635052112185,
133.391587494076));
#216405=CARTESIAN_POINT('Ctrl Pts',(-4.02661727117806,5.44157721958877,
133.40000956912));
#216406=CARTESIAN_POINT('Ctrl Pts',(-4.16781185472731,5.33119436370449,
133.408431644163));
#216407=CARTESIAN_POINT('Ctrl Pts',(-4.30901017261878,5.22080858839265,
133.416853941956));
#216408=CARTESIAN_POINT('Ctrl Pts',(-4.44581619661231,5.10481316862147,
133.425276239748));
#216409=CARTESIAN_POINT('Ctrl Pts',(-4.57778381064575,4.98359151445919,
133.43369853754));
#216410=CARTESIAN_POINT('Ctrl Pts',(-4.70977333790016,4.86234973144247,
133.442122233855));
#216411=CARTESIAN_POINT('Ctrl Pts',(-4.8369226082705,4.73588020987226,133.45054593017));
#216412=CARTESIAN_POINT('Ctrl Pts',(-4.95882132357918,4.60460422629529,
133.458969626484));
#216413=CARTESIAN_POINT('Ctrl Pts',(-5.08080253038164,4.47323940542455,
133.467399023296));
#216414=CARTESIAN_POINT('Ctrl Pts',(-5.19752585490095,4.33706186760948,
133.475828420108));
#216415=CARTESIAN_POINT('Ctrl Pts',(-5.30861969906324,4.19652783747681,
133.48425781692));
#216416=CARTESIAN_POINT('Ctrl Pts',(-5.41975318212811,4.05594366401915,
133.492690221388));
#216417=CARTESIAN_POINT('Ctrl Pts',(-5.52525297777009,3.91100016420562,
133.501122625856));
#216418=CARTESIAN_POINT('Ctrl Pts',(-5.62478969626702,3.76218418910722,
133.509555030324));
#216419=CARTESIAN_POINT('Ctrl Pts',(-5.72441851057413,3.61323052283314,
133.517995236828));
#216420=CARTESIAN_POINT('Ctrl Pts',(-5.81807304384533,3.46039750321733,
133.526435443332));
#216421=CARTESIAN_POINT('Ctrl Pts',(-5.90546832877107,3.30419927030467,
133.534875649837));
#216422=CARTESIAN_POINT('Ctrl Pts',(-5.95517786491757,3.21535532738957,
133.539676352193));
#216423=CARTESIAN_POINT('Ctrl Pts',(-6.00286323972515,3.12542311443387,
133.54447705455));
#216424=CARTESIAN_POINT('Ctrl Pts',(-6.04847883432461,3.03450041864014,
133.549277756907));
#216425=CARTESIAN_POINT('Ctrl Pts',(-6.12630417289266,2.87937606597523,
133.557468295462));
#216426=CARTESIAN_POINT('Ctrl Pts',(-6.19825425152646,2.72106392792542,
133.565658834017));
#216427=CARTESIAN_POINT('Ctrl Pts',(-6.26405876161416,2.56005016182201,
133.573849372572));
#216428=CARTESIAN_POINT('Ctrl Pts',(-6.32980308573432,2.39918366175382,
133.582032419916));
#216429=CARTESIAN_POINT('Ctrl Pts',(-6.38941289688081,2.23562078529211,
133.590215467259));
#216430=CARTESIAN_POINT('Ctrl Pts',(-6.44266407163697,2.06987165303508,
133.598398514603));
#216431=CARTESIAN_POINT('Ctrl Pts',(-6.49618067748921,1.90329634231249,
133.606622350441));
#216432=CARTESIAN_POINT('Ctrl Pts',(-6.54327490417465,1.73451324334587,
133.614846186279));
#216433=CARTESIAN_POINT('Ctrl Pts',(-6.58376808304185,1.56406100543408,
133.623070022117));
#216434=CARTESIAN_POINT('Ctrl Pts',(-6.62400730407458,1.39467777920355,
133.63124228118));
#216435=CARTESIAN_POINT('Ctrl Pts',(-6.65772795357341,1.22364664624818,
133.639414540244));
#216436=CARTESIAN_POINT('Ctrl Pts',(-6.68480458637177,1.05151159861551,
133.647586799308));
#216437=CARTESIAN_POINT('Ctrl Pts',(-6.71213754830078,0.87774698251167,
133.655836423533));
#216438=CARTESIAN_POINT('Ctrl Pts',(-6.7326999430227,0.702857800600873,
133.664086047758));
#216439=CARTESIAN_POINT('Ctrl Pts',(-6.74641559389651,0.52741410147062,
133.672335671983));
#216440=CARTESIAN_POINT('Ctrl Pts',(-6.76013124477032,0.351970402340238,
133.680585296208));
#216441=CARTESIAN_POINT('Ctrl Pts',(-6.76700011584166,0.175972563260165,
133.688834920433));
#216442=CARTESIAN_POINT('Ctrl Pts',(-6.76699999999853,-4.45461812127951E-6,
133.697084544658));
#216443=CARTESIAN_POINT('',(-6.76699895518313,0.00376039232056921,133.302820216217));
#216444=CARTESIAN_POINT('Ctrl Pts',(3.09910619832128,6.01563211736943,132.651465380124));
#216445=CARTESIAN_POINT('Ctrl Pts',(2.9422829664035,6.09642360205379,132.659773088112));
#216446=CARTESIAN_POINT('Ctrl Pts',(2.78218146133116,6.17113911591494,132.6680807961));
#216447=CARTESIAN_POINT('Ctrl Pts',(2.61930798531622,6.23951237502248,132.676388504088));
#216448=CARTESIAN_POINT('Ctrl Pts',(2.4565348215353,6.30784352368617,132.684691095437));
#216449=CARTESIAN_POINT('Ctrl Pts',(2.29099340863279,6.36984006698678,132.692993686786));
#216450=CARTESIAN_POINT('Ctrl Pts',(2.12321260920816,6.42528265651399,132.701296278135));
#216451=CARTESIAN_POINT('Ctrl Pts',(1.95550439899007,6.48070125918695,132.709595277426));
#216452=CARTESIAN_POINT('Ctrl Pts',(1.78555906292883,6.52957145023807,132.717894276716));
#216453=CARTESIAN_POINT('Ctrl Pts',(1.6139235213629,6.57172274728565,132.726193276006));
#216454=CARTESIAN_POINT('Ctrl Pts',(1.44233079473145,6.61386352958199,132.73449020509));
#216455=CARTESIAN_POINT('Ctrl Pts',(1.26904904063257,6.6492886760543,132.742787134173));
#216456=CARTESIAN_POINT('Ctrl Pts',(1.09463857049795,6.67787806117918,132.751084063256));
#216457=CARTESIAN_POINT('Ctrl Pts',(0.920200817714469,6.70647191847913,
132.75938229021));
#216458=CARTESIAN_POINT('Ctrl Pts',(0.744634338483491,6.72822781539155,
132.767680517163));
#216459=CARTESIAN_POINT('Ctrl Pts',(0.568508428552313,6.74307698062724,
132.775978744117));
#216460=CARTESIAN_POINT('Ctrl Pts',(0.392357421718683,6.75792826178132,
132.784278153519));
#216461=CARTESIAN_POINT('Ctrl Pts',(0.21564717217046,6.76587082003446,132.792577562921));
#216462=CARTESIAN_POINT('Ctrl Pts',(0.0389507607491826,6.76688789904466,
132.800876972323));
#216463=CARTESIAN_POINT('Ctrl Pts',(-0.137800194472367,6.76790529201344,
132.809178943641));
#216464=CARTESIAN_POINT('Ctrl Pts',(-0.314536955050337,6.76199294298867,
132.817480914959));
#216465=CARTESIAN_POINT('Ctrl Pts',(-0.490687586842416,6.74918622443616,
132.825782886277));
#216466=CARTESIAN_POINT('Ctrl Pts',(-0.666921872883159,6.73637342395021,
132.834088800216));
#216467=CARTESIAN_POINT('Ctrl Pts',(-0.842569128580576,6.71665975372667,
132.842394714155));
#216468=CARTESIAN_POINT('Ctrl Pts',(-1.01706348563162,6.69013235042438,
132.850700628094));
#216469=CARTESIAN_POINT('Ctrl Pts',(-1.19176641434726,6.6635732391359,132.859016470023));
#216470=CARTESIAN_POINT('Ctrl Pts',(-1.36531334720724,6.63018417696049,
132.867332311952));
#216471=CARTESIAN_POINT('Ctrl Pts',(-1.53714842304668,6.59010346849919,
132.875648153881));
#216472=CARTESIAN_POINT('Ctrl Pts',(-1.7090986528531,6.54999590025647,132.883969568609));
#216473=CARTESIAN_POINT('Ctrl Pts',(-1.87933440315601,6.50318783535335,
132.892290983336));
#216474=CARTESIAN_POINT('Ctrl Pts',(-2.04731575106779,6.44986722463569,
132.900612398063));
#216475=CARTESIAN_POINT('Ctrl Pts',(-2.21553622152306,6.39647071168119,
132.908945658379));
#216476=CARTESIAN_POINT('Ctrl Pts',(-2.38149555124351,6.3365432487563,132.917278918694));
#216477=CARTESIAN_POINT('Ctrl Pts',(-2.54467344291763,6.27032104990723,
132.92561217901));
#216478=CARTESIAN_POINT('Ctrl Pts',(-2.62638946484153,6.23715837941627,
132.92978529876));
#216479=CARTESIAN_POINT('Ctrl Pts',(-2.70740833253123,6.20241784780833,
132.933958418511));
#216480=CARTESIAN_POINT('Ctrl Pts',(-2.78766713701807,6.16613338593883,
132.938131538262));
#216481=CARTESIAN_POINT('Ctrl Pts',(-2.94286905967262,6.09596764797852,
132.946201384467));
#216482=CARTESIAN_POINT('Ctrl Pts',(-3.09570670996627,6.01980878026116,
132.954271230671));
#216483=CARTESIAN_POINT('Ctrl Pts',(-3.24567133678046,5.93783685980019,
132.962341076876));
#216484=CARTESIAN_POINT('Ctrl Pts',(-3.39544728901764,5.85596807044251,
132.970400770188));
#216485=CARTESIAN_POINT('Ctrl Pts',(-3.54235708668447,5.76830095697706,
132.978460463499));
#216486=CARTESIAN_POINT('Ctrl Pts',(-3.68591042633544,5.67506416959595,
132.986520156811));
#216487=CARTESIAN_POINT('Ctrl Pts',(-3.82931466303837,5.58192422343008,
132.994571478851));
#216488=CARTESIAN_POINT('Ctrl Pts',(-3.96936906909925,5.4832263170296,133.002622800891));
#216489=CARTESIAN_POINT('Ctrl Pts',(-4.10560660096983,5.37924561979401,
133.010674122931));
#216490=CARTESIAN_POINT('Ctrl Pts',(-4.24173248280347,5.27535013731919,
133.018718846712));
#216491=CARTESIAN_POINT('Ctrl Pts',(-4.37404742114997,5.16618070606974,
133.026763570494));
#216492=CARTESIAN_POINT('Ctrl Pts',(-4.50211221102706,5.05205647626004,
133.034808294276));
#216493=CARTESIAN_POINT('Ctrl Pts',(-4.63010008206802,4.93800079224611,
133.0428481862));
#216494=CARTESIAN_POINT('Ctrl Pts',(-4.75384260851946,4.81899648151168,
133.050888078124));
#216495=CARTESIAN_POINT('Ctrl Pts',(-4.87293271969347,4.69540367906113,
133.058927970049));
#216496=CARTESIAN_POINT('Ctrl Pts',(-4.99458716234243,4.56914959004131,
133.067140982543));
#216497=CARTESIAN_POINT('Ctrl Pts',(-5.11138624186292,4.43810740421035,
133.075353995037));
#216498=CARTESIAN_POINT('Ctrl Pts',(-5.22293449680575,4.3027019699343,133.083567007532));
#216499=CARTESIAN_POINT('Ctrl Pts',(-5.3320933470238,4.17019696995537,133.091604094272));
#216500=CARTESIAN_POINT('Ctrl Pts',(-5.43622380606403,4.03351406109677,
133.099641181012));
#216501=CARTESIAN_POINT('Ctrl Pts',(-5.53499531585419,3.89308564681953,
133.107678267752));
#216502=CARTESIAN_POINT('Ctrl Pts',(-5.63377627852553,3.75264379290652,
133.115716123678));
#216503=CARTESIAN_POINT('Ctrl Pts',(-5.72719705566639,3.60845602535668,
133.123753979604));
#216504=CARTESIAN_POINT('Ctrl Pts',(-5.81497003918787,3.46098431711954,
133.13179183553));
#216505=CARTESIAN_POINT('Ctrl Pts',(-5.90276881373872,3.313469276105,133.139832053283));
#216506=CARTESIAN_POINT('Ctrl Pts',(-5.98491630043968,3.16266869459248,
133.147872271035));
#216507=CARTESIAN_POINT('Ctrl Pts',(-6.06117060009071,3.00906961644226,
133.155912488788));
#216508=CARTESIAN_POINT('Ctrl Pts',(-6.1403058306289,2.84966747760555,133.164256470548));
#216509=CARTESIAN_POINT('Ctrl Pts',(-6.21309368252874,2.68725165285073,
133.172600452309));
#216510=CARTESIAN_POINT('Ctrl Pts',(-6.2793187702202,2.52238870556469,133.180944434069));
#216511=CARTESIAN_POINT('Ctrl Pts',(-6.34324401739305,2.36325105815218,
133.188998649096));
#216512=CARTESIAN_POINT('Ctrl Pts',(-6.4010546159101,2.201833773138,133.197052864122));
#216513=CARTESIAN_POINT('Ctrl Pts',(-6.452608071421,2.03866085375488,133.205107079149));
#216514=CARTESIAN_POINT('Ctrl Pts',(-6.50420010615967,1.87536582645173,
133.213167321423));
#216515=CARTESIAN_POINT('Ctrl Pts',(-6.54952557630775,1.71031290662024,
133.221227563696));
#216516=CARTESIAN_POINT('Ctrl Pts',(-6.58849315994731,1.54403590674815,
133.22928780597));
#216517=CARTESIAN_POINT('Ctrl Pts',(-6.62751522292725,1.37752644028642,
133.237359317012));
#216518=CARTESIAN_POINT('Ctrl Pts',(-6.66016159409174,1.20978984260038,
133.245430828054));
#216519=CARTESIAN_POINT('Ctrl Pts',(-6.6863927094321,1.0413652266392,133.253502339096));
#216520=CARTESIAN_POINT('Ctrl Pts',(-6.68914199869593,1.02371260369812,
133.254348316034));
#216521=CARTESIAN_POINT('Ctrl Pts',(-6.69182086238034,1.00605242249317,
133.255194292973));
#216522=CARTESIAN_POINT('Ctrl Pts',(-6.69442928804769,0.988385303072306,
133.256040269912));
#216523=CARTESIAN_POINT('Ctrl Pts',(-6.74250861780533,0.662739350751086,
133.271633585338));
#216524=CARTESIAN_POINT('Ctrl Pts',(-6.76681562166512,0.333677441931173,
133.287226900764));
#216525=CARTESIAN_POINT('Ctrl Pts',(-6.76699895518282,0.00376039288159187,
133.30282021619));
#216526=CARTESIAN_POINT('Ctrl Pts',(-6.76699895518313,0.00376039232075853,
133.302820216217));
#216527=CARTESIAN_POINT('Ctrl Pts',(-6.76709367130421,-0.166685624388963,
133.31087623669));
#216528=CARTESIAN_POINT('Ctrl Pts',(-6.76074448764723,-0.337402547659519,
133.318932257163));
#216529=CARTESIAN_POINT('Ctrl Pts',(-6.74791638606985,-0.50785179591102,
133.326988277637));
#216530=CARTESIAN_POINT('Ctrl Pts',(-6.73510162204312,-0.6781238257745,
133.335035922157));
#216531=CARTESIAN_POINT('Ctrl Pts',(-6.71582137301528,-0.8481283643743,
133.343083566677));
#216532=CARTESIAN_POINT('Ctrl Pts',(-6.69009260406261,-1.01732489847972,
133.351131211197));
#216533=CARTESIAN_POINT('Ctrl Pts',(-6.66438491642342,-1.18638279846776,
133.35917226174));
#216534=CARTESIAN_POINT('Ctrl Pts',(-6.63223928122514,-1.35463364351775,
133.367213312282));
#216535=CARTESIAN_POINT('Ctrl Pts',(-6.59372461489781,-1.52154024031268,
133.375254362825));
#216536=CARTESIAN_POINT('Ctrl Pts',(-6.55407050051306,-1.69338473260621,
133.383533306106));
#216537=CARTESIAN_POINT('Ctrl Pts',(-6.50766470528992,-1.86380380860883,
133.391812249386));
#216538=CARTESIAN_POINT('Ctrl Pts',(-6.45463959831345,-2.03221963770749,
133.400091192667));
#216539=CARTESIAN_POINT('Ctrl Pts',(-6.40318384022079,-2.19565097533634,
133.408125109561));
#216540=CARTESIAN_POINT('Ctrl Pts',(-6.34549514090866,-2.35719557670721,
133.416159026454));
#216541=CARTESIAN_POINT('Ctrl Pts',(-6.28174561715427,-2.51633880893712,
133.424192943347));
#216542=CARTESIAN_POINT('Ctrl Pts',(-6.21800263890322,-2.67546570108328,
133.432226035356));
#216543=CARTESIAN_POINT('Ctrl Pts',(-6.14820021359972,-2.83219136695208,
133.440259127364));
#216544=CARTESIAN_POINT('Ctrl Pts',(-6.07255909613137,-2.98601993027377,
133.448292219372));
#216545=CARTESIAN_POINT('Ctrl Pts',(-5.99691068375431,-3.13986332898346,
133.4563260861));
#216546=CARTESIAN_POINT('Ctrl Pts',(-5.91542262429346,-3.29080873312182,
133.464359952829));
#216547=CARTESIAN_POINT('Ctrl Pts',(-5.82836215843078,-3.43838385730449,
133.472393819557));
#216548=CARTESIAN_POINT('Ctrl Pts',(-5.741275957439,-3.58600260478777,133.480430061101));
#216549=CARTESIAN_POINT('Ctrl Pts',(-5.64861426273166,-3.73024876760867,
133.488466302645));
#216550=CARTESIAN_POINT('Ctrl Pts',(-5.55068815627169,-3.87067823408575,
133.49650254419));
#216551=CARTESIAN_POINT('Ctrl Pts',(-5.45266859848319,-4.01124171304105,
133.504546454756));
#216552=CARTESIAN_POINT('Ctrl Pts',(-5.34937481495106,-4.14798091798835,
133.512590365322));
#216553=CARTESIAN_POINT('Ctrl Pts',(-5.24115911562539,-4.28048363210244,
133.520634275888));
#216554=CARTESIAN_POINT('Ctrl Pts',(-5.13288128729715,-4.4130624189261,
133.528682804639));
#216555=CARTESIAN_POINT('Ctrl Pts',(-5.01967616295562,-4.5413995915947,
133.53673133339));
#216556=CARTESIAN_POINT('Ctrl Pts',(-4.90193317647914,-4.6651195197265,
133.544779862142));
#216557=CARTESIAN_POINT('Ctrl Pts',(-4.78404786584367,-4.78898899676348,
133.552838119711));
#216558=CARTESIAN_POINT('Ctrl Pts',(-4.66161401386229,-4.90822983192578,
133.56089637728));
#216559=CARTESIAN_POINT('Ctrl Pts',(-4.53505477822122,-5.02250606356358,
133.56895463485));
#216560=CARTESIAN_POINT('Ctrl Pts',(-4.50890838002663,-5.04611486493982,
133.570619423753));
#216561=CARTESIAN_POINT('Ctrl Pts',(-4.48258600667227,-5.06951191744136,
133.572284212657));
#216562=CARTESIAN_POINT('Ctrl Pts',(-4.45609154241186,-5.09269448972207,
133.573949001561));
#216563=CARTESIAN_POINT('Ctrl Pts',(-4.3138795473748,-5.21712953478379,
133.582884941876));
#216564=CARTESIAN_POINT('Ctrl Pts',(-4.16636189976131,-5.33568374524025,
133.591820882191));
#216565=CARTESIAN_POINT('Ctrl Pts',(-4.01402762616934,-5.4479235692463,
133.600756822507));
#216566=CARTESIAN_POINT('Ctrl Pts',(-3.86192235100635,-5.55999466731326,
133.609679329756));
#216567=CARTESIAN_POINT('Ctrl Pts',(-3.7050151048525,-5.66577016628138,
133.618601837006));
#216568=CARTESIAN_POINT('Ctrl Pts',(-3.5438277933209,-5.76485676936438,
133.627524344256));
#216569=CARTESIAN_POINT('Ctrl Pts',(-3.38303543922898,-5.8637005804392,
133.636424988676));
#216570=CARTESIAN_POINT('Ctrl Pts',(-3.21798417041297,-5.95588807180147,
133.645325633097));
#216571=CARTESIAN_POINT('Ctrl Pts',(-3.04922410440849,-6.04106955439964,
133.654226277518));
#216572=CARTESIAN_POINT('Ctrl Pts',(-2.88072483506674,-6.12611940013066,
133.663113167154));
#216573=CARTESIAN_POINT('Ctrl Pts',(-2.70852843065635,-6.20418471810273,
133.67200005679));
#216574=CARTESIAN_POINT('Ctrl Pts',(-2.53321138391679,-6.27496048468788,
133.680886946426));
#216575=CARTESIAN_POINT('Ctrl Pts',(-2.35834496471864,-6.34555433222819,
133.689750993576));
#216576=CARTESIAN_POINT('Ctrl Pts',(-2.18037414758836,-6.4088959199107,
133.698615040725));
#216577=CARTESIAN_POINT('Ctrl Pts',(-1.99989655680842,-6.46472758606779,
133.707479087875));
#216578=CARTESIAN_POINT('Ctrl Pts',(-1.82734510126143,-6.51810726173493,
133.715953847712));
#216579=CARTESIAN_POINT('Ctrl Pts',(-1.6525025570652,-6.5646223548235,133.724428607549));
#216580=CARTESIAN_POINT('Ctrl Pts',(-1.47591029112629,-6.60408796220549,
133.732903367385));
#216581=CARTESIAN_POINT('Ctrl Pts',(-1.30485746535172,-6.64231559141512,
133.741112286446));
#216582=CARTESIAN_POINT('Ctrl Pts',(-1.13232764321828,-6.67389126433614,
133.749321205506));
#216583=CARTESIAN_POINT('Ctrl Pts',(-0.958877199700067,-6.69871954300935,
133.757530124567));
#216584=CARTESIAN_POINT('Ctrl Pts',(-0.785385518245537,-6.72355372461917,
133.765740995302));
#216585=CARTESIAN_POINT('Ctrl Pts',(-0.610973131834763,-6.74163726551333,
133.773951866038));
#216586=CARTESIAN_POINT('Ctrl Pts',(-0.436202594282811,-6.75292649869232,
133.782162736773));
#216587=CARTESIAN_POINT('Ctrl Pts',(-0.261359351486093,-6.76422042823761,
133.790377023264));
#216588=CARTESIAN_POINT('Ctrl Pts',(-0.0861580157723752,-6.76871439623117,
133.798591309754));
#216589=CARTESIAN_POINT('Ctrl Pts',(0.0888377060821969,-6.76641684069036,
133.806805596245));
#216590=CARTESIAN_POINT('Ctrl Pts',(0.264030400271302,-6.76411669905845,
133.815029128603));
#216591=CARTESIAN_POINT('Ctrl Pts',(0.43901666216046,-6.75500977012508,
133.823252660961));
#216592=CARTESIAN_POINT('Ctrl Pts',(0.613235774965258,-6.73915654101482,
133.831476193318));
#216593=CARTESIAN_POINT('Ctrl Pts',(0.787566555974475,-6.72329315055314,
133.839704996665));
#216594=CARTESIAN_POINT('Ctrl Pts',(0.961128855517095,-6.7006748859166,
133.847933800013));
#216595=CARTESIAN_POINT('Ctrl Pts',(1.13337106600222,-6.67141357035741,
133.85616260336));
#216596=CARTESIAN_POINT('Ctrl Pts',(1.30585035430655,-6.64211197890498,
133.864402733006));
#216597=CARTESIAN_POINT('Ctrl Pts',(1.47700557681594,-6.60614914596039,
133.872642862652));
#216598=CARTESIAN_POINT('Ctrl Pts',(1.6462982380752,-6.5636873105984,133.880882992298));
#216599=CARTESIAN_POINT('Ctrl Pts',(1.7214565659004,-6.54483616537771,133.884541239269));
#216600=CARTESIAN_POINT('Ctrl Pts',(1.79624802391357,-6.52470474051377,
133.88819948624));
#216601=CARTESIAN_POINT('Ctrl Pts',(1.87062672729915,-6.50331028377965,
133.89185773321));
#216602=CARTESIAN_POINT('Ctrl Pts',(2.04239004463055,-6.45390389870048,
133.900305751349));
#216603=CARTESIAN_POINT('Ctrl Pts',(2.21234394623014,-6.39764562152587,
133.908753769488));
#216604=CARTESIAN_POINT('Ctrl Pts',(2.37992213524361,-6.33468701911764,
133.917201787627));
#216605=CARTESIAN_POINT('Ctrl Pts',(2.54734686734116,-6.27178606999361,
133.925642069635));
#216606=CARTESIAN_POINT('Ctrl Pts',(2.71239991259888,-6.20219714265404,
133.934082351643));
#216607=CARTESIAN_POINT('Ctrl Pts',(2.87453008596152,-6.12612159403501,
133.942522633651));
#216608=CARTESIAN_POINT('Ctrl Pts',(3.03653675057568,-6.05010399882222,
133.950956485957));
#216609=CARTESIAN_POINT('Ctrl Pts',(3.19562468117761,-5.96760977425559,
133.959390338263));
#216610=CARTESIAN_POINT('Ctrl Pts',(3.35126227056852,-5.87888851687663,
133.967824190569));
#216611=CARTESIAN_POINT('Ctrl Pts',(3.50680522410583,-5.79022120669615,
133.976252914649));
#216612=CARTESIAN_POINT('Ctrl Pts',(3.65890173023552,-5.69533457745867,
133.984681638728));
#216613=CARTESIAN_POINT('Ctrl Pts',(3.80704406398739,-5.59452451016692,
133.993110362808));
#216614=CARTESIAN_POINT('Ctrl Pts',(3.95511906875269,-5.4937602598911,134.001535256129));
#216615=CARTESIAN_POINT('Ctrl Pts',(4.09924320935774,-5.38707812701131,
134.009960149451));
#216616=CARTESIAN_POINT('Ctrl Pts',(4.23893674913172,-5.27481793400119,
134.018385042772));
#216617=CARTESIAN_POINT('Ctrl Pts',(4.37859936110751,-5.16258259511533,
134.026808070844));
#216618=CARTESIAN_POINT('Ctrl Pts',(4.51383306664667,-5.04477186504803,
134.035231098915));
#216619=CARTESIAN_POINT('Ctrl Pts',(4.64418988453205,-4.92176688968608,
134.043654126986));
#216620=CARTESIAN_POINT('Ctrl Pts',(4.77453195313025,-4.79877583178342,
134.05207620203));
#216621=CARTESIAN_POINT('Ctrl Pts',(4.89999799161701,-4.67059192902208,
134.060498277073));
#216622=CARTESIAN_POINT('Ctrl Pts',(5.02017545619937,-4.53763455877327,
134.068920352117));
#216623=CARTESIAN_POINT('Ctrl Pts',(5.14035609925841,-4.40467367204237,
134.077342649909));
#216624=CARTESIAN_POINT('Ctrl Pts',(5.25524766621523,-4.26693931376235,
134.085764947701));
#216625=CARTESIAN_POINT('Ctrl Pts',(5.36447638677372,-4.12488570699204,
134.094187245494));
#216626=CARTESIAN_POINT('Ctrl Pts',(5.47372324476179,-3.98280851221963,
134.102610941809));
#216627=CARTESIAN_POINT('Ctrl Pts',(5.57730517887522,-3.83641090374199,
134.111034638123));
#216628=CARTESIAN_POINT('Ctrl Pts',(5.6748901988497,-3.68617826902059,134.119458334438));
#216629=CARTESIAN_POINT('Ctrl Pts',(5.77254125671401,-3.53584396863183,
134.12788773125));
#216630=CARTESIAN_POINT('Ctrl Pts',(5.86418710925702,-3.38166973601207,
134.136317128062));
#216631=CARTESIAN_POINT('Ctrl Pts',(5.94953988539577,-3.22416875366116,
134.144746524874));
#216632=CARTESIAN_POINT('Ctrl Pts',(6.03492311588055,-3.06661157408229,
134.153178929342));
#216633=CARTESIAN_POINT('Ctrl Pts',(6.11400863927412,-2.9057255740443,134.16161133381));
#216634=CARTESIAN_POINT('Ctrl Pts',(6.18655541898425,-2.74204687192554,
134.170043738277));
#216635=CARTESIAN_POINT('Ctrl Pts',(6.25916932220979,-2.57821672697324,
134.178483944782));
#216636=CARTESIAN_POINT('Ctrl Pts',(6.32523226446926,-2.41158902475306,
134.186924151286));
#216637=CARTESIAN_POINT('Ctrl Pts',(6.38455165269328,-2.24271915185374,
134.19536435779));
#216638=CARTESIAN_POINT('Ctrl Pts',(6.41829190853671,-2.14666771089225,
134.200165060147));
#216639=CARTESIAN_POINT('Ctrl Pts',(6.44985138425098,-2.04989117763733,
134.204965762503));
#216640=CARTESIAN_POINT('Ctrl Pts',(6.47920190307621,-1.95249371296647,
134.20976646486));
#216641=CARTESIAN_POINT('Ctrl Pts',(6.52896652431803,-1.78735360187953,
134.217906189267));
#216642=CARTESIAN_POINT('Ctrl Pts',(6.57247710501642,-1.62009842067415,
134.226045913675));
#216643=CARTESIAN_POINT('Ctrl Pts',(6.6095514310584,-1.45124735320821,134.234185638083));
#216644=CARTESIAN_POINT('Ctrl Pts',(6.64659333170785,-1.28254396373748,
134.242318243447));
#216645=CARTESIAN_POINT('Ctrl Pts',(6.6772101045517,-1.11224782151601,134.25045084881));
#216646=CARTESIAN_POINT('Ctrl Pts',(6.70126910669482,-0.940893915198506,
134.258583454174));
#216647=CARTESIAN_POINT('Ctrl Pts',(6.72531166052328,-0.769657157670257,
134.266710499555));
#216648=CARTESIAN_POINT('Ctrl Pts',(6.74280531900876,-0.597364436978038,
134.274837544935));
#216649=CARTESIAN_POINT('Ctrl Pts',(6.75366837228143,-0.42456155884102,
134.282964590315));
#216650=CARTESIAN_POINT('Ctrl Pts',(6.76452623258499,-0.251841287314305,
134.291087750647));
#216651=CARTESIAN_POINT('Ctrl Pts',(6.76875977664518,-0.078611708688447,
134.299210910978));
#216652=CARTESIAN_POINT('Ctrl Pts',(6.76633907293236,0.0945756316865812,
134.307334071309));
#216653=CARTESIAN_POINT('Ctrl Pts',(6.76391904948411,0.267714303068407,
134.315454948875));
#216654=CARTESIAN_POINT('Ctrl Pts',(6.75484850878356,0.440810393999221,
134.323575826441));
#216655=CARTESIAN_POINT('Ctrl Pts',(6.73914962523719,0.613311771177977,
134.331696704007));
#216656=CARTESIAN_POINT('Ctrl Pts',(6.72344989360934,0.785822467186494,
134.339818020277));
#216657=CARTESIAN_POINT('Ctrl Pts',(6.7011211330024,0.957738020181045,134.347939336548));
#216658=CARTESIAN_POINT('Ctrl Pts',(6.67223746082235,1.12851064080003,134.356060652818));
#216659=CARTESIAN_POINT('Ctrl Pts',(6.65722871038969,1.21724879111642,134.360280712107));
#216660=CARTESIAN_POINT('Ctrl Pts',(6.64045090130213,1.30567844182336,134.364500771396));
#216661=CARTESIAN_POINT('Ctrl Pts',(6.62191990559178,1.3937237042999,134.368720830685));
#216662=CARTESIAN_POINT('Ctrl Pts',(6.58246773098609,1.58117057022766,134.377705265117));
#216663=CARTESIAN_POINT('Ctrl Pts',(6.53508587936941,1.76678162433251,134.386689699548));
#216664=CARTESIAN_POINT('Ctrl Pts',(6.4799776082147,1.94991774109476,134.39567413398));
#216665=CARTESIAN_POINT('Ctrl Pts',(6.42477422283632,2.13336994198028,134.404674075113));
#216666=CARTESIAN_POINT('Ctrl Pts',(6.3618178328622,2.31433843884362,134.413674016247));
#216667=CARTESIAN_POINT('Ctrl Pts',(6.29136071496936,2.49220170815692,134.42267395738));
#216668=CARTESIAN_POINT('Ctrl Pts',(6.22073756119818,2.67048412155427,134.431695107344));
#216669=CARTESIAN_POINT('Ctrl Pts',(6.14257840135267,2.84564644294452,134.440716257309));
#216670=CARTESIAN_POINT('Ctrl Pts',(6.05718377222747,3.01708696418651,134.449737407274));
#216671=CARTESIAN_POINT('Ctrl Pts',(5.9717022519301,3.18870193044924,134.458767736484));
#216672=CARTESIAN_POINT('Ctrl Pts',(5.87897066616139,3.35658731998988,134.467798065694));
#216673=CARTESIAN_POINT('Ctrl Pts',(5.77933508011031,3.52016690397008,134.476828394905));
#216674=CARTESIAN_POINT('Ctrl Pts',(5.6795582386698,3.68397839804141,134.485871526596));
#216675=CARTESIAN_POINT('Ctrl Pts',(5.57285795009395,3.84347167641061,134.494914658287));
#216676=CARTESIAN_POINT('Ctrl Pts',(5.45962437772617,3.99809837974732,134.503957789978));
#216677=CARTESIAN_POINT('Ctrl Pts',(5.36063187673157,4.1332781127874,134.511863592155));
#216678=CARTESIAN_POINT('Ctrl Pts',(5.25664680599319,4.26473878927251,134.519769394332));
#216679=CARTESIAN_POINT('Ctrl Pts',(5.14795514502898,4.39213465467188,134.527675196509));
#216680=CARTESIAN_POINT('Ctrl Pts',(5.02897023659875,4.53159508102349,134.536329688857));
#216681=CARTESIAN_POINT('Ctrl Pts',(4.90423896087291,4.66630674144622,134.544984181205));
#216682=CARTESIAN_POINT('Ctrl Pts',(4.7741586796986,4.79580002721742,134.553638673553));
#216683=CARTESIAN_POINT('Ctrl Pts',(4.64424148225365,4.92513096518477,134.562282315625));
#216684=CARTESIAN_POINT('Ctrl Pts',(4.508988877527,5.04925637129254,134.570925957698));
#216685=CARTESIAN_POINT('Ctrl Pts',(4.36883632402047,5.16774207695385,134.57956959977));
#216686=CARTESIAN_POINT('Ctrl Pts',(4.22879280700214,5.28613560259473,134.588206517224));
#216687=CARTESIAN_POINT('Ctrl Pts',(4.08385717428778,5.39889798157439,134.596843434679));
#216688=CARTESIAN_POINT('Ctrl Pts',(3.93450038150467,5.50563309238271,134.605480352133));
#216689=CARTESIAN_POINT('Ctrl Pts',(3.78528659056306,5.61226600953039,134.614109000161));
#216690=CARTESIAN_POINT('Ctrl Pts',(3.6316603333524,5.71288299806633,134.622737648188));
#216691=CARTESIAN_POINT('Ctrl Pts',(3.47412434380166,5.80712915680414,134.631366296216));
#216692=CARTESIAN_POINT('Ctrl Pts',(3.35140667946281,5.88054519656873,134.638087855748));
#216693=CARTESIAN_POINT('Ctrl Pts',(3.22631723720771,5.95009610861492,134.644809415281));
#216694=CARTESIAN_POINT('Ctrl Pts',(3.09910619832129,6.01563211736943,134.651530974814));
#216695=CARTESIAN_POINT('Origin',(0.,0.,4.30282021618968));
#216696=CARTESIAN_POINT('',(3.0991061983214,6.01563211736937,137.045755263024));
#216697=CARTESIAN_POINT('',(3.09910619832118,6.01563211736948,136.651395695404));
#216698=CARTESIAN_POINT('',(3.09910619832133,6.0156321173694,4.30282021618968));
#216699=CARTESIAN_POINT('',(-6.767,-5.66010073996262E-10,135.697179783837));
#216700=CARTESIAN_POINT('Ctrl Pts',(-6.767,-5.65818573007036E-10,135.697179783837));
#216701=CARTESIAN_POINT('Ctrl Pts',(-6.76699999998445,-0.186007250092783,
135.705929295648));
#216702=CARTESIAN_POINT('Ctrl Pts',(-6.75932637291409,-0.372014356315282,
135.714678807459));
#216703=CARTESIAN_POINT('Ctrl Pts',(-6.74400518259517,-0.557389538051668,
135.72342831927));
#216704=CARTESIAN_POINT('Ctrl Pts',(-6.72868405698871,-0.742763936814854,
135.732177794126));
#216705=CARTESIAN_POINT('Ctrl Pts',(-6.70571545637962,-0.927506130803568,
135.740927268982));
#216706=CARTESIAN_POINT('Ctrl Pts',(-6.67517739395499,-1.11098864046051,
135.749676743838));
#216707=CARTESIAN_POINT('Ctrl Pts',(-6.64463945797831,-1.29447039037746,
135.758426182465));
#216708=CARTESIAN_POINT('Ctrl Pts',(-6.6065321699595,-1.47669218369183,
135.767175621092));
#216709=CARTESIAN_POINT('Ctrl Pts',(-6.56098496078752,-1.65703510654422,
135.775925059719));
#216710=CARTESIAN_POINT('Ctrl Pts',(-6.51543793642857,-1.83737729763449,
135.784674462844));
#216711=CARTESIAN_POINT('Ctrl Pts',(-6.46245112150483,-2.01584035565226,
135.793423865969));
#216712=CARTESIAN_POINT('Ctrl Pts',(-6.40220448355839,-2.1918181381458,
135.802173269094));
#216713=CARTESIAN_POINT('Ctrl Pts',(-6.34195808506609,-2.36779522120432,
135.810922637444));
#216714=CARTESIAN_POINT('Ctrl Pts',(-6.27445201411749,-2.54128677736892,
135.819672005794));
#216715=CARTESIAN_POINT('Ctrl Pts',(-6.19991555049112,-2.71170355436917,
135.828421374144));
#216716=CARTESIAN_POINT('Ctrl Pts',(-6.12537937692472,-2.88211966818953,
135.837170708446));
#216717=CARTESIAN_POINT('Ctrl Pts',(-6.04381298026895,-3.04946076422573,
135.845920042748));
#216718=CARTESIAN_POINT('Ctrl Pts',(-5.95549339308833,-3.21315848424588,
135.85466937705));
#216719=CARTESIAN_POINT('Ctrl Pts',(-5.86717414227038,-3.37685558082785,
135.86341867803));
#216720=CARTESIAN_POINT('Ctrl Pts',(-5.77210188846886,-3.53690907695245,
135.87216797901));
#216721=CARTESIAN_POINT('Ctrl Pts',(-5.67059953315979,-3.69277537016916,
135.88091727999));
#216722=CARTESIAN_POINT('Ctrl Pts',(-5.56909755599059,-3.84864108271698,
135.889666548376));
#216723=CARTESIAN_POINT('Ctrl Pts',(-5.46116568163254,-4.00031938343382,
135.898415816761));
#216724=CARTESIAN_POINT('Ctrl Pts',(-5.34717048498774,-4.14729511904759,
135.907165085146));
#216725=CARTESIAN_POINT('Ctrl Pts',(-5.23317570355772,-4.29427031931866,
135.915914321663));
#216726=CARTESIAN_POINT('Ctrl Pts',(-5.11311781966253,-4.43654276232491,
135.92466355818));
#216727=CARTESIAN_POINT('Ctrl Pts',(-4.98740458946339,-4.57362924393742,
135.933412794697));
#216728=CARTESIAN_POINT('Ctrl Pts',(-4.86169180672201,-4.71071523761075,
135.942162000073));
#216729=CARTESIAN_POINT('Ctrl Pts',(-4.73032391163547,-4.84261509562919,
135.950911205448));
#216730=CARTESIAN_POINT('Ctrl Pts',(-4.59374706971941,-4.96888084576842,
135.959660410824));
#216731=CARTESIAN_POINT('Ctrl Pts',(-4.45717070258735,-5.09514615696826,
135.968409585784));
#216732=CARTESIAN_POINT('Ctrl Pts',(-4.31538563527325,-5.21577720495696,
135.977158760744));
#216733=CARTESIAN_POINT('Ctrl Pts',(-4.1688734098484,-5.33036429267822,
135.985907935705));
#216734=CARTESIAN_POINT('Ctrl Pts',(-4.0223616815807,-5.44495099157329,
135.994657080977));
#216735=CARTESIAN_POINT('Ctrl Pts',(-3.87112305301613,-5.55349359471052,
136.003406226249));
#216736=CARTESIAN_POINT('Ctrl Pts',(-3.71567116970346,-5.65562346330045,
136.012155371521));
#216737=CARTESIAN_POINT('Ctrl Pts',(-3.56021980097516,-5.75775299381512,
136.020904487831));
#216738=CARTESIAN_POINT('Ctrl Pts',(-3.40055544489212,-5.8534696749242,
136.029653604141));
#216739=CARTESIAN_POINT('Ctrl Pts',(-3.23722035936936,-5.94244843014094,
136.038402720452));
#216740=CARTESIAN_POINT('Ctrl Pts',(-3.07388580096523,-6.03142689820346,
136.047151808526));
#216741=CARTESIAN_POINT('Ctrl Pts',(-2.90688078845238,-6.11366734681192,
136.055900896601));
#216742=CARTESIAN_POINT('Ctrl Pts',(-2.73677250669407,-6.18889046975332,
136.064649984676));
#216743=CARTESIAN_POINT('Ctrl Pts',(-2.56666475978868,-6.26411335617886,
136.073399045242));
#216744=CARTESIAN_POINT('Ctrl Pts',(-2.39345402521959,-6.33231884520667,
136.082148105808));
#216745=CARTESIAN_POINT('Ctrl Pts',(-2.21772856011852,-6.39327529781368,
136.090897166374));
#216746=CARTESIAN_POINT('Ctrl Pts',(-2.04200363294235,-6.45423156382285,
136.099646200158));
#216747=CARTESIAN_POINT('Ctrl Pts',(-1.86376426134522,-6.5079387439134,
136.108395233942));
#216748=CARTESIAN_POINT('Ctrl Pts',(-1.68361577697981,-6.55421443923714,
136.117144267725));
#216749=CARTESIAN_POINT('Ctrl Pts',(-1.5034678291224,-6.60048999674524,
136.125893275453));
#216750=CARTESIAN_POINT('Ctrl Pts',(-1.32141105739104,-6.63933404248835,
136.134642283181));
#216751=CARTESIAN_POINT('Ctrl Pts',(-1.13806375430879,-6.67061465617139,
136.143391290909));
#216752=CARTESIAN_POINT('Ctrl Pts',(-0.954716982039362,-6.70189517929325,
136.152140273307));
#216753=CARTESIAN_POINT('Ctrl Pts',(-0.770079968336905,-6.72561226598699,
136.160889255705));
#216754=CARTESIAN_POINT('Ctrl Pts',(-0.584779764992078,-6.74168536988013,
136.169638238104));
#216755=CARTESIAN_POINT('Ctrl Pts',(-0.391489830089624,-6.7584515101709,
136.178764457113));
#216756=CARTESIAN_POINT('Ctrl Pts',(-0.197478577681895,-6.76689983033232,
136.187890676123));
#216757=CARTESIAN_POINT('Ctrl Pts',(-0.00346287590081867,-6.76699911397146,
136.197016895133));
#216758=CARTESIAN_POINT('Ctrl Pts',(0.184489835199639,-6.76709529499687,
136.205857919798));
#216759=CARTESIAN_POINT('Ctrl Pts',(0.372446404788815,-6.7593563973518,
136.214698944464));
#216760=CARTESIAN_POINT('Ctrl Pts',(0.559755020020896,-6.74380925868766,
136.223539969129));
#216761=CARTESIAN_POINT('Ctrl Pts',(0.745134706053204,-6.72842222653921,
136.232289947739));
#216762=CARTESIAN_POINT('Ctrl Pts',(0.92987943175826,-6.70538706050178,
136.241039926349));
#216763=CARTESIAN_POINT('Ctrl Pts',(1.11336163679561,-6.67478200885331,
136.249789904959));
#216764=CARTESIAN_POINT('Ctrl Pts',(1.29684196353216,-6.64417727050766,
136.258539793995));
#216765=CARTESIAN_POINT('Ctrl Pts',(1.4790595126971,-6.60600284878903,136.267289683032));
#216766=CARTESIAN_POINT('Ctrl Pts',(1.65939532118928,-6.56038841594117,
136.276039572068));
#216767=CARTESIAN_POINT('Ctrl Pts',(1.83972934352284,-6.51477443488718,
136.28478937444));
#216768=CARTESIAN_POINT('Ctrl Pts',(2.01818138457328,-6.46172066046193,
136.293539176812));
#216769=CARTESIAN_POINT('Ctrl Pts',(2.19414528404785,-6.4014073040614,136.302288979185));
#216770=CARTESIAN_POINT('Ctrl Pts',(2.37010749914096,-6.34109452499917,
136.311038697801));
#216771=CARTESIAN_POINT('Ctrl Pts',(2.5435813491601,-6.27352239596414,136.319788416417));
#216772=CARTESIAN_POINT('Ctrl Pts',(2.71397759484504,-6.19892043945389,
136.328538135033));
#216773=CARTESIAN_POINT('Ctrl Pts',(2.88437226606477,-6.12431917226742,
136.337287772802));
#216774=CARTESIAN_POINT('Ctrl Pts',(3.05168912728658,-6.04268832254707,
136.346037410571));
#216775=CARTESIAN_POINT('Ctrl Pts',(3.21535986320854,-5.95430516097954,
136.35478704834));
#216776=CARTESIAN_POINT('Ctrl Pts',(3.3790291411916,-5.8659227867076,136.363536608169));
#216777=CARTESIAN_POINT('Ctrl Pts',(3.53905210667155,-5.77078835713988,
136.372286167998));
#216778=CARTESIAN_POINT('Ctrl Pts',(3.69488522876493,-5.66922500402434,
136.381035727827));
#216779=CARTESIAN_POINT('Ctrl Pts',(3.85071701450938,-5.56766252186664,
136.389785212624));
#216780=CARTESIAN_POINT('Ctrl Pts',(4.00235878865553,-5.45967138297739,
136.398534697421));
#216781=CARTESIAN_POINT('Ctrl Pts',(4.14929549653577,-5.34561838166811,
136.407284182218));
#216782=CARTESIAN_POINT('Ctrl Pts',(4.29623099317445,-5.23156632053054,
136.416033594891));
#216783=CARTESIAN_POINT('Ctrl Pts',(4.43846127476439,-5.11145267269874,
136.424783007563));
#216784=CARTESIAN_POINT('Ctrl Pts',(4.57550326093864,-4.98568540013707,
136.433532420236));
#216785=CARTESIAN_POINT('Ctrl Pts',(4.71254416296205,-4.85991912253102,
136.442281763691));
#216786=CARTESIAN_POINT('Ctrl Pts',(4.84439664056143,-4.72849950347121,
136.451031107146));
#216787=CARTESIAN_POINT('Ctrl Pts',(4.97061286831044,-4.59187289821775,
136.459780450602));
#216788=CARTESIAN_POINT('Ctrl Pts',(5.09682813947888,-4.45524732844411,
136.468529727747));
#216789=CARTESIAN_POINT('Ctrl Pts',(5.21740705181908,-4.31341506194578,
136.477279004891));
#216790=CARTESIAN_POINT('Ctrl Pts',(5.33194007578594,-4.16685781233627,
136.486028282036));
#216791=CARTESIAN_POINT('Ctrl Pts',(5.44647226976221,-4.02030162478847,
136.494777495777));
#216792=CARTESIAN_POINT('Ctrl Pts',(5.5549584865865,-3.86902074844091,136.503526709518));
#216793=CARTESIAN_POINT('Ctrl Pts',(5.65703027321092,-3.71352898036021,
136.512275923259));
#216794=CARTESIAN_POINT('Ctrl Pts',(5.75910135405073,-3.55803828744144,
136.521025076503));
#216795=CARTESIAN_POINT('Ctrl Pts',(5.85475793619567,-3.39833700060515,
136.529774229747));
#216796=CARTESIAN_POINT('Ctrl Pts',(5.94367514452923,-3.23496750776657,
136.538523382991));
#216797=CARTESIAN_POINT('Ctrl Pts',(6.0325917675688,-3.07159909030118,136.547272478644));
#216798=CARTESIAN_POINT('Ctrl Pts',(6.1147689685885,-2.90456276683171,136.556021574297));
#216799=CARTESIAN_POINT('Ctrl Pts',(6.18992765569473,-2.73442582954184,
136.56477066995));
#216800=CARTESIAN_POINT('Ctrl Pts',(6.26508587303301,-2.56428995566705,
136.573519710918));
#216801=CARTESIAN_POINT('Ctrl Pts',(6.33322554846041,-2.39105376885192,
136.582268751886));
#216802=CARTESIAN_POINT('Ctrl Pts',(6.39411526750526,-2.21530561003582,
136.591017792854));
#216803=CARTESIAN_POINT('Ctrl Pts',(6.45500462618948,-2.0395584913414,136.599766782043));
#216804=CARTESIAN_POINT('Ctrl Pts',(6.50864402055428,-1.86129970113184,
136.608515771232));
#216805=CARTESIAN_POINT('Ctrl Pts',(6.55485128381862,-1.68113463084354,
136.617264760421));
#216806=CARTESIAN_POINT('Ctrl Pts',(6.60199809565858,-1.49730620065882,
136.626191645892));
#216807=CARTESIAN_POINT('Ctrl Pts',(6.64140720717751,-1.31149343195513,
136.635118531363));
#216808=CARTESIAN_POINT('Ctrl Pts',(6.67293928731192,-1.12435326648217,
136.644045416834));
#216809=CARTESIAN_POINT('Ctrl Pts',(6.70384625883209,-0.940923066511241,
136.652795331011));
#216810=CARTESIAN_POINT('Ctrl Pts',(6.72718554585383,-0.756217899024617,
136.661545245189));
#216811=CARTESIAN_POINT('Ctrl Pts',(6.74287786819546,-0.570865180756313,
136.670295159366));
#216812=CARTESIAN_POINT('Ctrl Pts',(6.75856988193694,-0.385516107574673,
136.679044901471));
#216813=CARTESIAN_POINT('Ctrl Pts',(6.76661520774876,-0.199519794726551,
136.687794643575));
#216814=CARTESIAN_POINT('Ctrl Pts',(6.76698651789679,-0.0135080199558931,
136.69654438568));
#216815=CARTESIAN_POINT('Ctrl Pts',(6.76735782123629,0.172500344012673,
136.705293967345));
#216816=CARTESIAN_POINT('Ctrl Pts',(6.76005538992536,0.358523882710025,
136.71404354901));
#216817=CARTESIAN_POINT('Ctrl Pts',(6.74510402738346,0.543930749062307,
136.722793130675));
#216818=CARTESIAN_POINT('Ctrl Pts',(6.73015291912646,0.729334462112059,
136.731542563531));
#216819=CARTESIAN_POINT('Ctrl Pts',(6.70755316299847,0.914121238129835,
136.740291996388));
#216820=CARTESIAN_POINT('Ctrl Pts',(6.67738151866471,1.09766345215414,136.749041429245));
#216821=CARTESIAN_POINT('Ctrl Pts',(6.64721034738111,1.28120278848734,136.757790724922));
#216822=CARTESIAN_POINT('Ctrl Pts',(6.60946757194338,1.4634973190912,136.7665400206));
#216823=CARTESIAN_POINT('Ctrl Pts',(6.56428138099387,1.6439279032662,136.775289316277));
#216824=CARTESIAN_POINT('Ctrl Pts',(6.51909583846384,1.82435589827176,136.784038486403));
#216825=CARTESIAN_POINT('Ctrl Pts',(6.46646716378092,2.00291972239993,136.792787656528));
#216826=CARTESIAN_POINT('Ctrl Pts',(6.40657409856802,2.17901292321946,136.801536826654));
#216827=CARTESIAN_POINT('Ctrl Pts',(6.34668181324704,2.35510383105791,136.810285882853));
#216828=CARTESIAN_POINT('Ctrl Pts',(6.27952541895408,2.52872390868873,136.819034939052));
#216829=CARTESIAN_POINT('Ctrl Pts',(6.20533299155628,2.69928350936006,136.827783995251));
#216830=CARTESIAN_POINT('Ctrl Pts',(6.12831602971186,2.8763363800887,136.836866131408));
#216831=CARTESIAN_POINT('Ctrl Pts',(6.0437169058462,3.05009086642249,136.845948267566));
#216832=CARTESIAN_POINT('Ctrl Pts',(5.95184520295876,3.219911129211,136.855030403723));
#216833=CARTESIAN_POINT('Ctrl Pts',(5.86333549487463,3.38351691220815,136.863780184066));
#216834=CARTESIAN_POINT('Ctrl Pts',(5.76807618076524,3.54347103749191,136.87252996441));
#216835=CARTESIAN_POINT('Ctrl Pts',(5.66639083285165,3.69923018064229,136.881279744754));
#216836=CARTESIAN_POINT('Ctrl Pts',(5.56470914057342,3.85498372417933,136.890029210539));
#216837=CARTESIAN_POINT('Ctrl Pts',(5.45660203346228,4.00654234737189,136.898778676323));
#216838=CARTESIAN_POINT('Ctrl Pts',(5.34243669812427,4.15339128021128,136.907528142108));
#216839=CARTESIAN_POINT('Ctrl Pts',(5.22827486022857,4.30023571434999,136.916277339854));
#216840=CARTESIAN_POINT('Ctrl Pts',(5.10805534138462,4.44237052061411,136.9250265376));
#216841=CARTESIAN_POINT('Ctrl Pts',(4.98218644310422,4.57931296660848,136.933775735346));
#216842=CARTESIAN_POINT('Ctrl Pts',(4.85632073189171,4.71625194514679,136.942524711558));
#216843=CARTESIAN_POINT('Ctrl Pts',(4.72480612139051,4.84799861554981,136.95127368777));
#216844=CARTESIAN_POINT('Ctrl Pts',(4.58808925203228,4.97410554928079,136.960022663981));
#216845=CARTESIAN_POINT('Ctrl Pts',(4.45136349441154,5.10022068149915,136.968772208983));
#216846=CARTESIAN_POINT('Ctrl Pts',(4.30943501176412,5.22069514899625,136.977521753985));
#216847=CARTESIAN_POINT('Ctrl Pts',(4.16278587397379,5.335119751931,136.986271298986));
#216848=CARTESIAN_POINT('Ctrl Pts',(4.01614535705282,5.44953762833759,136.99502032964));
#216849=CARTESIAN_POINT('Ctrl Pts',(3.86478496622032,5.55790617557742,137.003769360294));
#216850=CARTESIAN_POINT('Ctrl Pts',(3.70921874710619,5.65985735563327,137.012518390948));
#216851=CARTESIAN_POINT('Ctrl Pts',(3.55365041568669,5.76180992000009,137.021267540397));
#216852=CARTESIAN_POINT('Ctrl Pts',(3.39387638136678,5.85734478574741,137.030016689847));
#216853=CARTESIAN_POINT('Ctrl Pts',(3.23043927866126,5.94613749142101,137.038765839296));
#216854=CARTESIAN_POINT('Ctrl Pts',(3.18691767044669,5.96978206957779,137.041095647206));
#216855=CARTESIAN_POINT('Ctrl Pts',(3.14313645906677,5.99294880640099,137.043425455115));
#216856=CARTESIAN_POINT('Ctrl Pts',(3.0991061983214,6.01563211736937,137.045755263024));
#216857=CARTESIAN_POINT('Ctrl Pts',(3.09910619832134,6.0156321173694,135.045755263024));
#216858=CARTESIAN_POINT('Ctrl Pts',(2.93375330764826,6.10081787314653,135.054504710927));
#216859=CARTESIAN_POINT('Ctrl Pts',(2.7648862784307,6.17918207037039,135.063254158829));
#216860=CARTESIAN_POINT('Ctrl Pts',(2.59307866646702,6.25045854553997,135.072003606731));
#216861=CARTESIAN_POINT('Ctrl Pts',(2.42127244185382,6.32173444515035,135.080752983982));
#216862=CARTESIAN_POINT('Ctrl Pts',(2.24652594672477,6.38592262741833,135.089502361232));
#216863=CARTESIAN_POINT('Ctrl Pts',(2.06943269687141,6.44280508110556,135.098251738482));
#216864=CARTESIAN_POINT('Ctrl Pts',(1.89234081822097,6.49968709436161,135.107001047988));
#216865=CARTESIAN_POINT('Ctrl Pts',(1.71290249405609,6.54926340459539,135.115750357493));
#216866=CARTESIAN_POINT('Ctrl Pts',(1.5317271662508,6.59136563150379,135.124499666998));
#216867=CARTESIAN_POINT('Ctrl Pts',(1.3505531810736,6.63346754640705,135.133248911666));
#216868=CARTESIAN_POINT('Ctrl Pts',(1.16764249714449,6.66809542395771,135.141998156333));
#216869=CARTESIAN_POINT('Ctrl Pts',(0.983616340614701,6.69513165624663,
135.150747401));
#216870=CARTESIAN_POINT('Ctrl Pts',(0.79959148671406,6.72216769715959,135.159496583736));
#216871=CARTESIAN_POINT('Ctrl Pts',(0.614451459526801,6.74161215869371,
135.168245766471));
#216872=CARTESIAN_POINT('Ctrl Pts',(0.428825047910242,6.75339900185712,
135.176994949207));
#216873=CARTESIAN_POINT('Ctrl Pts',(0.243199888596912,6.76518576550222,
135.185744072918));
#216874=CARTESIAN_POINT('Ctrl Pts',(0.057088637391689,6.76931499599835,
135.194493196628));
#216875=CARTESIAN_POINT('Ctrl Pts',(-0.128876626811471,6.76577266947846,
135.203242320339));
#216876=CARTESIAN_POINT('Ctrl Pts',(-0.314840698188552,6.76223036567991,
135.21199138793));
#216877=CARTESIAN_POINT('Ctrl Pts',(-0.500658497951714,6.7510166087922,
135.220740455522));
#216878=CARTESIAN_POINT('Ctrl Pts',(-0.685698951926748,6.73216948296213,
135.229489523113));
#216879=CARTESIAN_POINT('Ctrl Pts',(-0.870738280460292,6.71332247176287,
135.238238537492));
#216880=CARTESIAN_POINT('Ctrl Pts',(-1.05499998761286,6.68684221356181,
135.24698755187));
#216881=CARTESIAN_POINT('Ctrl Pts',(-1.23785829161446,6.65281863948517,
135.255736566249));
#216882=CARTESIAN_POINT('Ctrl Pts',(-1.43007412917413,6.61705395368859,
135.264933299948));
#216883=CARTESIAN_POINT('Ctrl Pts',(-1.62073882535785,6.57295372727791,
135.274130033647));
#216884=CARTESIAN_POINT('Ctrl Pts',(-1.80913696091492,6.52068343478286,
135.283326767346));
#216885=CARTESIAN_POINT('Ctrl Pts',(-1.9883835618609,6.47095219815205,135.29207676506));
#216886=CARTESIAN_POINT('Ctrl Pts',(-2.16557827572511,6.41382586850898,
135.300826762774));
#216887=CARTESIAN_POINT('Ctrl Pts',(-2.34011918621679,6.34949849943286,
135.309576760487));
#216888=CARTESIAN_POINT('Ctrl Pts',(-2.51465655691083,6.28517243495557,
135.318326580746));
#216889=CARTESIAN_POINT('Ctrl Pts',(-2.68653996295318,6.21364572242379,
135.327076401004));
#216890=CARTESIAN_POINT('Ctrl Pts',(-2.85518555379984,6.13516132252223,
135.335826221262));
#216891=CARTESIAN_POINT('Ctrl Pts',(-3.02382794858663,6.05667841000519,
135.3445758757));
#216892=CARTESIAN_POINT('Ctrl Pts',(-3.18923239109234,5.97123819492105,
135.353325530137));
#216893=CARTESIAN_POINT('Ctrl Pts',(-3.35083705967632,5.87913088810751,
135.362075184575));
#216894=CARTESIAN_POINT('Ctrl Pts',(-3.5124388804233,5.78702520443145,135.370824684824));
#216895=CARTESIAN_POINT('Ctrl Pts',(-3.67024081223617,5.6882528060583,135.379574185073));
#216896=CARTESIAN_POINT('Ctrl Pts',(-3.82370687544326,5.58314917682556,
135.388323685322));
#216897=CARTESIAN_POINT('Ctrl Pts',(-3.97717043817738,5.47804726008077,
135.397073043012));
#216898=CARTESIAN_POINT('Ctrl Pts',(-4.12629803722382,5.36661448084296,
135.405822400703));
#216899=CARTESIAN_POINT('Ctrl Pts',(-4.27058317206828,5.24922931204642,
135.414571758393));
#216900=CARTESIAN_POINT('Ctrl Pts',(-4.41486614774761,5.13184589986855,
135.423320985153));
#216901=CARTESIAN_POINT('Ctrl Pts',(-4.55430658194345,5.00851045723097,
135.432070211913));
#216902=CARTESIAN_POINT('Ctrl Pts',(-4.68843089001782,4.8796418710318,135.440819438673));
#216903=CARTESIAN_POINT('Ctrl Pts',(-4.82255336917773,4.75077504208025,
135.449568546129));
#216904=CARTESIAN_POINT('Ctrl Pts',(-4.95135966065071,4.61637541908161,
135.458317653585));
#216905=CARTESIAN_POINT('Ctrl Pts',(-5.07441230869181,4.47689945401916,
135.467066761041));
#216906=CARTESIAN_POINT('Ctrl Pts',(-5.1974634422637,4.33742520555572,135.475815760817));
#216907=CARTESIAN_POINT('Ctrl Pts',(-5.31476088454736,4.19287495491377,
135.484564760594));
#216908=CARTESIAN_POINT('Ctrl Pts',(-5.42590627628836,4.04373961586729,
135.49331376037));
#216909=CARTESIAN_POINT('Ctrl Pts',(-5.53706380672645,3.89458798906766,
135.502063715665));
#216910=CARTESIAN_POINT('Ctrl Pts',(-5.64206777071836,3.74085050155325,
135.51081367096));
#216911=CARTESIAN_POINT('Ctrl Pts',(-5.74056148163976,3.58304938223212,
135.519563626254));
#216912=CARTESIAN_POINT('Ctrl Pts',(-5.8390513895185,3.42525435593339,135.528313243695));
#216913=CARTESIAN_POINT('Ctrl Pts',(-5.93103139557618,3.26339625497246,
135.537062861137));
#216914=CARTESIAN_POINT('Ctrl Pts',(-6.0161890782081,3.09802485065074,135.545812478578));
#216915=CARTESIAN_POINT('Ctrl Pts',(-6.1013439254495,2.9326589524971,135.554561804693));
#216916=CARTESIAN_POINT('Ctrl Pts',(-6.17967677261801,2.76378023986105,
135.563311130809));
#216917=CARTESIAN_POINT('Ctrl Pts',(-6.25092157009195,2.59196229227185,
135.572060456925));
#216918=CARTESIAN_POINT('Ctrl Pts',(-6.32216437407728,2.42014915229157,
135.580809538228));
#216919=CARTESIAN_POINT('Ctrl Pts',(-6.386319415489,2.24539720662912,135.58955861953));
#216920=CARTESIAN_POINT('Ctrl Pts',(-6.44316881037519,2.06829994947743,
135.598307700833));
#216921=CARTESIAN_POINT('Ctrl Pts',(-6.50002334524557,1.89118668024501,
135.607057573175));
#216922=CARTESIAN_POINT('Ctrl Pts',(-6.54957082411085,1.71172794807747,
135.615807445517));
#216923=CARTESIAN_POINT('Ctrl Pts',(-6.59164294296075,1.53053334250378,
135.62455731786));
#216924=CARTESIAN_POINT('Ctrl Pts',(-6.63371214082129,1.34935131693624,
135.633306582715));
#216925=CARTESIAN_POINT('Ctrl Pts',(-6.66830695239688,1.16643393829774,
135.642055847569));
#216926=CARTESIAN_POINT('Ctrl Pts',(-6.69530988153989,0.982402458340958,
135.650805112424));
#216927=CARTESIAN_POINT('Ctrl Pts',(-6.72231419690481,0.798361530947166,
135.659554826431));
#216928=CARTESIAN_POINT('Ctrl Pts',(-6.74172580829275,0.613206671362721,
135.668304540438));
#216929=CARTESIAN_POINT('Ctrl Pts',(-6.75347878028177,0.427566795113783,
135.677054254445));
#216930=CARTESIAN_POINT('Ctrl Pts',(-6.76248992368203,0.285234494207359,
135.683762764234));
#216931=CARTESIAN_POINT('Ctrl Pts',(-6.76699999999985,0.142617266095927,
135.690471274022));
#216932=CARTESIAN_POINT('Ctrl Pts',(-6.767,6.94095400683209E-12,135.69717978381));
#216933=CARTESIAN_POINT('',(-6.767,6.93929614291322E-12,135.30282021619));
#216934=CARTESIAN_POINT('Ctrl Pts',(3.09910619832129,6.01563211736943,134.651530974814));
#216935=CARTESIAN_POINT('Ctrl Pts',(2.93600378292275,6.09965848345377,134.660148958007));
#216936=CARTESIAN_POINT('Ctrl Pts',(2.76941303260316,6.17708323365079,134.668766941199));
#216937=CARTESIAN_POINT('Ctrl Pts',(2.59988462643395,6.24763066523882,134.677384924392));
#216938=CARTESIAN_POINT('Ctrl Pts',(2.53926608414269,6.27285642274986,134.680466470373));
#216939=CARTESIAN_POINT('Ctrl Pts',(2.47827216835747,6.2972032914136,134.683548016353));
#216940=CARTESIAN_POINT('Ctrl Pts',(2.4169287797121,6.32066011376971,134.686629562334));
#216941=CARTESIAN_POINT('Ctrl Pts',(2.24921401483504,6.3847918080418,134.695054606516));
#216942=CARTESIAN_POINT('Ctrl Pts',(2.07895886568387,6.44223889516753,134.703479650697));
#216943=CARTESIAN_POINT('Ctrl Pts',(1.90672453923883,6.49281838121662,134.711904694879));
#216944=CARTESIAN_POINT('Ctrl Pts',(1.73445021098399,6.54340961446514,134.720331695797));
#216945=CARTESIAN_POINT('Ctrl Pts',(1.56019610708374,6.587129972977,134.728758696714));
#216946=CARTESIAN_POINT('Ctrl Pts',(1.38453719934345,6.62384674819958,134.737185697631));
#216947=CARTESIAN_POINT('Ctrl Pts',(1.20881367420903,6.66057702995233,134.745615798481));
#216948=CARTESIAN_POINT('Ctrl Pts',(1.03168463927251,6.6902985236657,134.754045899331));
#216949=CARTESIAN_POINT('Ctrl Pts',(0.853734211707432,6.71292982949772,
134.762476000182));
#216950=CARTESIAN_POINT('Ctrl Pts',(0.675619840749096,6.73558198525476,
134.770913867573));
#216951=CARTESIAN_POINT('Ctrl Pts',(0.496682894442441,6.75113086071185,
134.779351734965));
#216952=CARTESIAN_POINT('Ctrl Pts',(0.317512679657415,6.75954692995446,
134.787789602356));
#216953=CARTESIAN_POINT('Ctrl Pts',(0.138248403430535,6.76796741749622,
134.79623189949));
#216954=CARTESIAN_POINT('Ctrl Pts',(-0.0412490543095359,6.76924762290726,
134.804674196625));
#216955=CARTESIAN_POINT('Ctrl Pts',(-0.220390865830408,6.76341015067536,
134.813116493759));
#216956=CARTESIAN_POINT('Ctrl Pts',(-0.399721664706716,6.75756652014669,
134.821567697175));
#216957=CARTESIAN_POINT('Ctrl Pts',(-0.578695737101644,6.74459023095583,
134.830018900591));
#216958=CARTESIAN_POINT('Ctrl Pts',(-0.756728770012883,6.72455578968863,
134.838470104007));
#216959=CARTESIAN_POINT('Ctrl Pts',(-0.806682038090416,6.71893444066682,
134.840841378724));
#216960=CARTESIAN_POINT('Ctrl Pts',(-0.856561275549977,6.71275773118605,
134.843212653441));
#216961=CARTESIAN_POINT('Ctrl Pts',(-0.906353719630754,6.7060280296843,
134.845583928159));
#216962=CARTESIAN_POINT('Ctrl Pts',(-1.08097882032073,6.68242656114724,
134.853900131429));
#216963=CARTESIAN_POINT('Ctrl Pts',(-1.25485079803176,6.65197705904537,
134.862216334699));
#216964=CARTESIAN_POINT('Ctrl Pts',(-1.42740188091235,6.61474208645869,
134.870532537969));
#216965=CARTESIAN_POINT('Ctrl Pts',(-1.59980705750844,6.57753859913663,
134.878841709198));
#216966=CARTESIAN_POINT('Ctrl Pts',(-1.77089322619723,6.53356114592075,
134.887150880427));
#216967=CARTESIAN_POINT('Ctrl Pts',(-1.9400999808047,6.48292380523492,134.895460051656));
#216968=CARTESIAN_POINT('Ctrl Pts',(-2.10919468280949,6.43231999776016,
134.903763720361));
#216969=CARTESIAN_POINT('Ctrl Pts',(-2.27641211849353,6.37506519031083,
134.912067389066));
#216970=CARTESIAN_POINT('Ctrl Pts',(-2.44120406465513,6.31132408569797,
134.920371057771));
#216971=CARTESIAN_POINT('Ctrl Pts',(-2.60591708464302,6.24761350952787,
134.92867074948));
#216972=CARTESIAN_POINT('Ctrl Pts',(-2.76820660635052,6.17742295252512,
134.93697044119));
#216973=CARTESIAN_POINT('Ctrl Pts',(-2.92754129958098,6.10096639387956,
134.945270132899));
#216974=CARTESIAN_POINT('Ctrl Pts',(-3.08682887315697,6.02453244554285,
134.953567370161));
#216975=CARTESIAN_POINT('Ctrl Pts',(-3.24316304670243,5.94183633952596,
134.961864607423));
#216976=CARTESIAN_POINT('Ctrl Pts',(-3.39603394244471,5.85313953889393,
134.970161844686));
#216977=CARTESIAN_POINT('Ctrl Pts',(-3.54892028053974,5.76443377849702,
134.978459920099));
#216978=CARTESIAN_POINT('Ctrl Pts',(-3.69834233705561,5.66972628035997,
134.986757995512));
#216979=CARTESIAN_POINT('Ctrl Pts',(-3.84381574630596,5.56932397230134,
134.995056070925));
#216980=CARTESIAN_POINT('Ctrl Pts',(-3.98930378271827,5.46891156892131,
135.003354980698));
#216981=CARTESIAN_POINT('Ctrl Pts',(-4.13084209365886,5.36280341159873,
135.011653890472));
#216982=CARTESIAN_POINT('Ctrl Pts',(-4.26797625311067,5.2513491316883,135.019952800246));
#216983=CARTESIAN_POINT('Ctrl Pts',(-4.40514699306072,5.13986512138022,
135.028253923751));
#216984=CARTESIAN_POINT('Ctrl Pts',(-4.53791096991338,5.02303236570051,
135.036555047257));
#216985=CARTESIAN_POINT('Ctrl Pts',(-4.66584759328945,4.90124017328217,
135.044856170762));
#216986=CARTESIAN_POINT('Ctrl Pts',(-4.79383960942083,4.77939524846451,
135.053160888407));
#216987=CARTESIAN_POINT('Ctrl Pts',(-4.91699985457346,4.65258684715798,
135.061465606053));
#216988=CARTESIAN_POINT('Ctrl Pts',(-5.03494515810745,4.52124056591223,
135.069770323698));
#216989=CARTESIAN_POINT('Ctrl Pts',(-5.15303029447224,4.38973856399113,
135.078084887197));
#216990=CARTESIAN_POINT('Ctrl Pts',(-5.26588790351228,4.25368819222075,
135.086399450695));
#216991=CARTESIAN_POINT('Ctrl Pts',(-5.37317488258129,4.11354842942168,
135.094714014194));
#216992=CARTESIAN_POINT('Ctrl Pts',(-5.48052970397372,3.97332005002445,
135.103033835361));
#216993=CARTESIAN_POINT('Ctrl Pts',(-5.58230667026415,3.82899740668009,
135.111353656527));
#216994=CARTESIAN_POINT('Ctrl Pts',(-5.67820641843379,3.68106789799609,
135.119673477694));
#216995=CARTESIAN_POINT('Ctrl Pts',(-5.77424958151963,3.53291716560194,
135.128005740879));
#216996=CARTESIAN_POINT('Ctrl Pts',(-5.86439778375524,3.38114908719061,
135.136338004065));
#216997=CARTESIAN_POINT('Ctrl Pts',(-5.94839730981834,3.22627625050087,
135.14467026725));
#216998=CARTESIAN_POINT('Ctrl Pts',(-6.01164831454297,3.10965818151534,
135.150944398103));
#216999=CARTESIAN_POINT('Ctrl Pts',(-6.07141399149068,2.99128022710502,
135.157218528956));
#217000=CARTESIAN_POINT('Ctrl Pts',(-6.12760425966692,2.87136814722735,
135.163492659808));
#217001=CARTESIAN_POINT('Ctrl Pts',(-6.20546860883635,2.70520278870045,
135.172186889812));
#217002=CARTESIAN_POINT('Ctrl Pts',(-6.27668004813401,2.53563375665815,
135.180881119815));
#217003=CARTESIAN_POINT('Ctrl Pts',(-6.34094305750286,2.3632033643989,135.189575349818));
#217004=CARTESIAN_POINT('Ctrl Pts',(-6.40506363778926,2.19115513759997,
135.198250310397));
#217005=CARTESIAN_POINT('Ctrl Pts',(-6.46226638485983,2.01625846582904,
135.206925270975));
#217006=CARTESIAN_POINT('Ctrl Pts',(-6.51230193574305,1.83907925270158,
135.215600231554));
#217007=CARTESIAN_POINT('Ctrl Pts',(-6.56218337877673,1.66244574571772,
135.22424847354));
#217008=CARTESIAN_POINT('Ctrl Pts',(-6.60494156714428,1.48354399855786,
135.232896715525));
#217009=CARTESIAN_POINT('Ctrl Pts',(-6.64037571162132,1.30295794579476,
135.241544957511));
#217010=CARTESIAN_POINT('Ctrl Pts',(-6.67574416231199,1.12270669387829,
135.250177165929));
#217011=CARTESIAN_POINT('Ctrl Pts',(-6.70381557493082,0.940777645910259,
135.258809374347));
#217012=CARTESIAN_POINT('Ctrl Pts',(-6.72443845616014,0.757770710251219,
135.267441582765));
#217013=CARTESIAN_POINT('Ctrl Pts',(-6.74500929652179,0.575225583958943,
135.276052008212));
#217014=CARTESIAN_POINT('Ctrl Pts',(-6.75816905394779,0.391608284783801,
135.284662433659));
#217015=CARTESIAN_POINT('Ctrl Pts',(-6.76381701651168,0.207529195890568,
135.293272859106));
#217016=CARTESIAN_POINT('Ctrl Pts',(-6.76590452913319,0.139492728390334,
135.296455311468));
#217017=CARTESIAN_POINT('Ctrl Pts',(-6.76696637000047,0.0713933033251629,
135.299637763829));
#217018=CARTESIAN_POINT('Ctrl Pts',(-6.76699921371665,0.00326214013017339,
135.30282021619));
#217019=CARTESIAN_POINT('Ctrl Pts',(-6.767,6.93929656985413E-12,135.30282021619));
#217020=CARTESIAN_POINT('Ctrl Pts',(-6.76700000000019,-0.186007249520054,
135.311569728001));
#217021=CARTESIAN_POINT('Ctrl Pts',(-6.75932637294557,-0.372014355743232,
135.320319239812));
#217022=CARTESIAN_POINT('Ctrl Pts',(-6.74400518264234,-0.557389537480943,
135.329068751624));
#217023=CARTESIAN_POINT('Ctrl Pts',(-6.72868405705156,-0.742763936245454,
135.337818226479));
#217024=CARTESIAN_POINT('Ctrl Pts',(-6.7057154564581,-0.927506130236138,
135.346567701335));
#217025=CARTESIAN_POINT('Ctrl Pts',(-6.67517739404899,-1.1109886398957,
135.355317176191));
#217026=CARTESIAN_POINT('Ctrl Pts',(-6.64463945808786,-1.29447038981513,
135.364066614818));
#217027=CARTESIAN_POINT('Ctrl Pts',(-6.60653217008449,-1.47669218313263,
135.372816053445));
#217028=CARTESIAN_POINT('Ctrl Pts',(-6.5609849609278,-1.65703510598878,
135.381565492072));
#217029=CARTESIAN_POINT('Ctrl Pts',(-6.51543793658408,-1.83737729708305,
135.390314895197));
#217030=CARTESIAN_POINT('Ctrl Pts',(-6.46245112167539,-2.01584035510546,
135.399064298322));
#217031=CARTESIAN_POINT('Ctrl Pts',(-6.40220448374379,-2.19181813760425,
135.407813701447));
#217032=CARTESIAN_POINT('Ctrl Pts',(-6.34195808526632,-2.36779522066801,
135.416563069797));
#217033=CARTESIAN_POINT('Ctrl Pts',(-6.27445201433233,-2.54128677683847,
135.425312438147));
#217034=CARTESIAN_POINT('Ctrl Pts',(-6.19991555072031,-2.71170355384517,
135.434061806498));
#217035=CARTESIAN_POINT('Ctrl Pts',(-6.12537937716824,-2.88211966767197,
135.442811140799));
#217036=CARTESIAN_POINT('Ctrl Pts',(-6.04381298052655,-3.04946076371519,
135.451560475101));
#217037=CARTESIAN_POINT('Ctrl Pts',(-5.95549339335968,-3.21315848374295,
135.460309809403));
#217038=CARTESIAN_POINT('Ctrl Pts',(-5.8671741425556,-3.37685558033229,
135.469059110383));
#217039=CARTESIAN_POINT('Ctrl Pts',(-5.77210188876765,-3.53690907646483,
135.477808411363));
#217040=CARTESIAN_POINT('Ctrl Pts',(-5.6705995334718,-3.69277536969004,
135.486557712343));
#217041=CARTESIAN_POINT('Ctrl Pts',(-5.5690975563159,-3.84864108224624,
135.495306980729));
#217042=CARTESIAN_POINT('Ctrl Pts',(-5.4611656819708,-4.00031938297202,
135.504056249114));
#217043=CARTESIAN_POINT('Ctrl Pts',(-5.34717048533858,-4.14729511859525,
135.512805517499));
#217044=CARTESIAN_POINT('Ctrl Pts',(-5.23317570392105,-4.29427031887589,
135.521554754016));
#217045=CARTESIAN_POINT('Ctrl Pts',(-5.11311782003796,-4.43654276189222,
135.530303990533));
#217046=CARTESIAN_POINT('Ctrl Pts',(-4.98740458985049,-4.57362924351529,
135.53905322705));
#217047=CARTESIAN_POINT('Ctrl Pts',(-4.86169180712061,-4.71071523719938,
135.547802432426));
#217048=CARTESIAN_POINT('Ctrl Pts',(-4.73032391204511,-4.84261509522905,
135.556551637801));
#217049=CARTESIAN_POINT('Ctrl Pts',(-4.59374707013962,-4.96888084537994,
135.565300843177));
#217050=CARTESIAN_POINT('Ctrl Pts',(-4.45717070301812,-5.09514615659143,
135.574050018137));
#217051=CARTESIAN_POINT('Ctrl Pts',(-4.31538563571411,-5.21577720459222,
135.582799193098));
#217052=CARTESIAN_POINT('Ctrl Pts',(-4.16887341029881,-5.33036429232596,
135.591548368058));
#217053=CARTESIAN_POINT('Ctrl Pts',(-4.02236168204108,-5.44495099123318,
135.60029751333));
#217054=CARTESIAN_POINT('Ctrl Pts',(-3.87112305348597,-5.553493594383,135.609046658602));
#217055=CARTESIAN_POINT('Ctrl Pts',(-3.71567117018224,-5.65562346298589,
135.617795803874));
#217056=CARTESIAN_POINT('Ctrl Pts',(-3.560219801463,-5.75775299351346,135.626544920184));
#217057=CARTESIAN_POINT('Ctrl Pts',(-3.40055544538848,-5.85346967463583,
135.635294036494));
#217058=CARTESIAN_POINT('Ctrl Pts',(-3.2372203598737,-5.94244842986619,
135.644043152804));
#217059=CARTESIAN_POINT('Ctrl Pts',(-3.07388580147699,-6.03142689794265,
135.652792240879));
#217060=CARTESIAN_POINT('Ctrl Pts',(-2.90688078897097,-6.11366734656535,
135.661541328954));
#217061=CARTESIAN_POINT('Ctrl Pts',(-2.73677250721889,-6.18889046952124,
135.670290417029));
#217062=CARTESIAN_POINT('Ctrl Pts',(-2.56666476032021,-6.26411335596106,
135.679039477595));
#217063=CARTESIAN_POINT('Ctrl Pts',(-2.39345402575724,-6.33231884500344,
135.687788538161));
#217064=CARTESIAN_POINT('Ctrl Pts',(-2.21772856066169,-6.39327529762527,
135.696537598727));
#217065=CARTESIAN_POINT('Ctrl Pts',(-2.04200363349079,-6.45423156364933,
135.705286632511));
#217066=CARTESIAN_POINT('Ctrl Pts',(-1.86376426189832,-6.507938743755,135.714035666294));
#217067=CARTESIAN_POINT('Ctrl Pts',(-1.68361577753694,-6.55421443909403,
135.722784700078));
#217068=CARTESIAN_POINT('Ctrl Pts',(-1.50346782968356,-6.60048999661741,
135.731533707806));
#217069=CARTESIAN_POINT('Ctrl Pts',(-1.3214110579556,-6.63933404237598,
135.740282715534));
#217070=CARTESIAN_POINT('Ctrl Pts',(-1.13806375487611,-6.6706146560746,
135.749031723262));
#217071=CARTESIAN_POINT('Ctrl Pts',(-0.954716982609564,-6.70189517921201,
135.75778070566));
#217072=CARTESIAN_POINT('Ctrl Pts',(-0.770079968909347,-6.72561226592144,
135.766529688058));
#217073=CARTESIAN_POINT('Ctrl Pts',(-0.584779765566115,-6.74168536983034,
135.775278670457));
#217074=CARTESIAN_POINT('Ctrl Pts',(-0.391489830659183,-6.75845151013807,
135.784404889467));
#217075=CARTESIAN_POINT('Ctrl Pts',(-0.197478578246223,-6.76689983031602,
135.793531108477));
#217076=CARTESIAN_POINT('Ctrl Pts',(-0.00346287645922686,-6.76699911397117,
135.802657327486));
#217077=CARTESIAN_POINT('Ctrl Pts',(0.184489834647022,-6.7670952950121,
135.811498352152));
#217078=CARTESIAN_POINT('Ctrl Pts',(0.372446404242634,-6.75935639738206,
135.820339376818));
#217079=CARTESIAN_POINT('Ctrl Pts',(0.559755019481737,-6.74380925873241,
135.829180401484));
#217080=CARTESIAN_POINT('Ctrl Pts',(0.745134705515176,-6.72842222659879,
135.837930380094));
#217081=CARTESIAN_POINT('Ctrl Pts',(0.929879431221979,-6.70538706057615,
135.846680358703));
#217082=CARTESIAN_POINT('Ctrl Pts',(1.11336163626168,-6.67478200894237,
135.855430337313));
#217083=CARTESIAN_POINT('Ctrl Pts',(1.29684196300084,-6.64417727061137,
135.86418022635));
#217084=CARTESIAN_POINT('Ctrl Pts',(1.47905951216898,-6.60600284890728,
135.872930115386));
#217085=CARTESIAN_POINT('Ctrl Pts',(1.65939532066495,-6.5603884160738,135.881680004423));
#217086=CARTESIAN_POINT('Ctrl Pts',(1.83972934300219,-6.51477443503421,
135.890429806795));
#217087=CARTESIAN_POINT('Ctrl Pts',(2.01818138405689,-6.46172066062321,
135.899179609167));
#217088=CARTESIAN_POINT('Ctrl Pts',(2.19414528353632,-6.40140730423673,
135.907929411539));
#217089=CARTESIAN_POINT('Ctrl Pts',(2.37010749863427,-6.34109452518856,
135.916679130155));
#217090=CARTESIAN_POINT('Ctrl Pts',(2.54358134865883,-6.27352239616737,
135.925428848772));
#217091=CARTESIAN_POINT('Ctrl Pts',(2.71397759434976,-6.19892043967073,
135.934178567388));
#217092=CARTESIAN_POINT('Ctrl Pts',(2.88437226557548,-6.12431917249786,
135.942928205157));
#217093=CARTESIAN_POINT('Ctrl Pts',(3.05168912680384,-6.04268832279087,
135.951677842925));
#217094=CARTESIAN_POINT('Ctrl Pts',(3.21535986273288,-5.9543051612364,135.960427480694));
#217095=CARTESIAN_POINT('Ctrl Pts',(3.3790291407228,-5.86592278697764,135.969177040523));
#217096=CARTESIAN_POINT('Ctrl Pts',(3.53905210621016,-5.77078835742282,
135.977926600352));
#217097=CARTESIAN_POINT('Ctrl Pts',(3.69488522831148,-5.66922500431987,
135.986676160181));
#217098=CARTESIAN_POINT('Ctrl Pts',(3.85071701406418,-5.56766252217455,
135.995425644979));
#217099=CARTESIAN_POINT('Ctrl Pts',(4.00235878821909,-5.45967138329733,
136.004175129776));
#217100=CARTESIAN_POINT('Ctrl Pts',(4.14929549610857,-5.3456183819997,136.012924614573));
#217101=CARTESIAN_POINT('Ctrl Pts',(4.29623099275649,-5.23156632087378,
136.021674027245));
#217102=CARTESIAN_POINT('Ctrl Pts',(4.43846127435614,-5.11145267305324,
136.030423439918));
#217103=CARTESIAN_POINT('Ctrl Pts',(4.57550326054055,-4.9856854005024,136.039172852591));
#217104=CARTESIAN_POINT('Ctrl Pts',(4.71254416257393,-4.85991912290736,
136.047922196046));
#217105=CARTESIAN_POINT('Ctrl Pts',(4.84439664018374,-4.72849950385815,
136.056671539501));
#217106=CARTESIAN_POINT('Ctrl Pts',(4.97061286794359,-4.59187289861485,
136.065420882956));
#217107=CARTESIAN_POINT('Ctrl Pts',(5.09682813912306,-4.45524732885118,
136.074170160101));
#217108=CARTESIAN_POINT('Ctrl Pts',(5.21740705147468,-4.31341506236236,
136.082919437246));
#217109=CARTESIAN_POINT('Ctrl Pts',(5.33194007545334,-4.16685781276187,
136.091668714391));
#217110=CARTESIAN_POINT('Ctrl Pts',(5.44647226944125,-4.02030162522329,
136.100417928132));
#217111=CARTESIAN_POINT('Ctrl Pts',(5.55495848627756,-3.86902074888446,
136.109167141873));
#217112=CARTESIAN_POINT('Ctrl Pts',(5.65703027291435,-3.713528980812,136.117916355614));
#217113=CARTESIAN_POINT('Ctrl Pts',(5.75910135376652,-3.55803828790146,
136.126665508858));
#217114=CARTESIAN_POINT('Ctrl Pts',(5.85475793592416,-3.39833700107291,
136.135414662102));
#217115=CARTESIAN_POINT('Ctrl Pts',(5.94367514427073,-3.23496750824152,
136.144163815346));
#217116=CARTESIAN_POINT('Ctrl Pts',(6.03259176732325,-3.07159909078344,
136.152912910999));
#217117=CARTESIAN_POINT('Ctrl Pts',(6.1147689683562,-2.90456276732074,136.161662006652));
#217118=CARTESIAN_POINT('Ctrl Pts',(6.18992765547595,-2.73442583003709,
136.170411102304));
#217119=CARTESIAN_POINT('Ctrl Pts',(6.2650858728278,-2.5642899561684,136.179160143273));
#217120=CARTESIAN_POINT('Ctrl Pts',(6.33322554826903,-2.39105376935882,
136.187909184241));
#217121=CARTESIAN_POINT('Ctrl Pts',(6.39411526732792,-2.21530561054769,
136.196658225209));
#217122=CARTESIAN_POINT('Ctrl Pts',(6.45500462602617,-2.03955849185824,
136.205407214398));
#217123=CARTESIAN_POINT('Ctrl Pts',(6.50864402040522,-1.86129970165306,
136.214156203587));
#217124=CARTESIAN_POINT('Ctrl Pts',(6.55485128368396,-1.68113463136857,
136.222905192776));
#217125=CARTESIAN_POINT('Ctrl Pts',(6.60199809554146,-1.49730620117666,
136.231832078247));
#217126=CARTESIAN_POINT('Ctrl Pts',(6.64140720707716,-1.31149343246494,
136.240758963719));
#217127=CARTESIAN_POINT('Ctrl Pts',(6.6729392872275,-1.12435326698318,136.24968584919));
#217128=CARTESIAN_POINT('Ctrl Pts',(6.70384625876143,-0.940923067014677,
136.258435763367));
#217129=CARTESIAN_POINT('Ctrl Pts',(6.72718554579703,-0.756217899529902,
136.267185677545));
#217130=CARTESIAN_POINT('Ctrl Pts',(6.74287786815257,-0.570865181262876,
136.275935591722));
#217131=CARTESIAN_POINT('Ctrl Pts',(6.75856988190798,-0.385516108082386,
136.284685333827));
#217132=CARTESIAN_POINT('Ctrl Pts',(6.76661520773378,-0.199519795234839,
136.293435075931));
#217133=CARTESIAN_POINT('Ctrl Pts',(6.76698651789577,-0.0135080204641805,
136.302184818036));
#217134=CARTESIAN_POINT('Ctrl Pts',(6.76735782124925,0.172500343504387,
136.310934399701));
#217135=CARTESIAN_POINT('Ctrl Pts',(6.76005538995229,0.358523882202315,
136.319683981366));
#217136=CARTESIAN_POINT('Ctrl Pts',(6.74510402742431,0.543930748555749,
136.328433563031));
#217137=CARTESIAN_POINT('Ctrl Pts',(6.73015291918125,0.729334461606526,
136.337182995887));
#217138=CARTESIAN_POINT('Ctrl Pts',(6.70755316306714,0.914121237625899,
136.345932428744));
#217139=CARTESIAN_POINT('Ctrl Pts',(6.6773815187472,1.09766345165238,136.354681861601));
#217140=CARTESIAN_POINT('Ctrl Pts',(6.64721034747738,1.28120278798787,136.363431157278));
#217141=CARTESIAN_POINT('Ctrl Pts',(6.60946757205334,1.4634973185946,136.372180452956));
#217142=CARTESIAN_POINT('Ctrl Pts',(6.56428138111738,1.64392790277301,136.380929748633));
#217143=CARTESIAN_POINT('Ctrl Pts',(6.51909583860089,1.82435589778201,136.389678918759));
#217144=CARTESIAN_POINT('Ctrl Pts',(6.46646716393138,2.00291972191416,136.398428088885));
#217145=CARTESIAN_POINT('Ctrl Pts',(6.4065740987317,2.17901292273821,136.40717725901));
#217146=CARTESIAN_POINT('Ctrl Pts',(6.3466818134239,2.35510383058131,136.415926315209));
#217147=CARTESIAN_POINT('Ctrl Pts',(6.27952541914391,2.52872390821732,136.424675371408));
#217148=CARTESIAN_POINT('Ctrl Pts',(6.20533299175886,2.69928350889436,136.433424427607));
#217149=CARTESIAN_POINT('Ctrl Pts',(6.12831602991927,2.8763363796482,136.442506563766));
#217150=CARTESIAN_POINT('Ctrl Pts',(6.04371690605653,3.05009086600705,136.451588699924));
#217151=CARTESIAN_POINT('Ctrl Pts',(5.95184520317016,3.21991112882022,136.460670836082));
#217152=CARTESIAN_POINT('Ctrl Pts',(5.86333549509676,3.38351691182321,136.469420616426));
#217153=CARTESIAN_POINT('Ctrl Pts',(5.76807618099786,3.54347103711324,136.478170396769));
#217154=CARTESIAN_POINT('Ctrl Pts',(5.66639083309448,3.69923018027033,136.486920177113));
#217155=CARTESIAN_POINT('Ctrl Pts',(5.56470914082653,3.85498372381396,136.495669642898));
#217156=CARTESIAN_POINT('Ctrl Pts',(5.4566020337254,4.00654234701354,136.504419108683));
#217157=CARTESIAN_POINT('Ctrl Pts',(5.34243669839709,4.15339127986035,136.513168574467));
#217158=CARTESIAN_POINT('Ctrl Pts',(5.22827486051102,4.30023571400659,136.521917772213));
#217159=CARTESIAN_POINT('Ctrl Pts',(5.10805534167639,4.44237052027862,136.53066696996));
#217160=CARTESIAN_POINT('Ctrl Pts',(4.98218644340496,4.57931296628128,136.539416167706));
#217161=CARTESIAN_POINT('Ctrl Pts',(4.85632073220169,4.71625194482759,136.548165143917));
#217162=CARTESIAN_POINT('Ctrl Pts',(4.72480612170941,4.84799861523901,136.556914120129));
#217163=CARTESIAN_POINT('Ctrl Pts',(4.58808925235973,4.97410554897874,136.56566309634));
#217164=CARTESIAN_POINT('Ctrl Pts',(4.45136349474737,5.10022068120604,136.574412641342));
#217165=CARTESIAN_POINT('Ctrl Pts',(4.30943501210796,5.22069514871242,136.583162186344));
#217166=CARTESIAN_POINT('Ctrl Pts',(4.16278587432525,5.33511975165677,136.591911731345));
#217167=CARTESIAN_POINT('Ctrl Pts',(4.016145357412,5.44953762807288,136.600660761999));
#217168=CARTESIAN_POINT('Ctrl Pts',(3.86478496658682,5.55790617532256,136.609409792653));
#217169=CARTESIAN_POINT('Ctrl Pts',(3.70921874747961,5.65985735538855,136.618158823307));
#217170=CARTESIAN_POINT('Ctrl Pts',(3.55365041606682,5.76180991976565,136.626907972756));
#217171=CARTESIAN_POINT('Ctrl Pts',(3.39387638175318,5.85734478552352,136.635657122206));
#217172=CARTESIAN_POINT('Ctrl Pts',(3.23043927905349,5.94613749120792,136.644406271655));
#217173=CARTESIAN_POINT('Ctrl Pts',(3.18691767070967,5.96978206943863,136.646736079572));
#217174=CARTESIAN_POINT('Ctrl Pts',(3.14313645919891,5.99294880633292,136.649065887488));
#217175=CARTESIAN_POINT('Ctrl Pts',(3.09910619832119,6.01563211736948,136.651395695404));
#217176=CARTESIAN_POINT('Origin',(0.,0.,8.));
#217177=CARTESIAN_POINT('',(-7.91099969351913,0.00214482957247683,8.64224520787028));
#217178=CARTESIAN_POINT('',(3.42067962509756,7.13322310757503,8.));
#217179=CARTESIAN_POINT('Ctrl Pts',(-7.91099969351913,0.00214482957247683,
8.64224520787028));
#217180=CARTESIAN_POINT('Ctrl Pts',(-7.91037070257867,2.20309451064308,
8.55368653892647));
#217181=CARTESIAN_POINT('Ctrl Pts',(-6.94161582034834,4.38658408256068,
8.46512786998266));
#217182=CARTESIAN_POINT('Ctrl Pts',(-3.67820201488298,7.34180684107625,
8.28798176530613));
#217183=CARTESIAN_POINT('Ctrl Pts',(-1.4086817587176,8.08992666571333,8.1993943295734));
#217184=CARTESIAN_POINT('Ctrl Pts',(1.69567364519642,7.78146992497721,8.07387126256046));
#217185=CARTESIAN_POINT('Ctrl Pts',(2.59296389908063,7.53014751000291,8.03693563128023));
#217186=CARTESIAN_POINT('Ctrl Pts',(3.42067962509756,7.13322310757503,8.));
#217187=CARTESIAN_POINT('',(-3.42067962509656,7.13322310757551,8.));
#217188=CARTESIAN_POINT('Origin',(0.,0.,8.));
#217189=CARTESIAN_POINT('',(-7.911,-6.54698517621455E-12,10.3576684917633));
#217190=CARTESIAN_POINT('Ctrl Pts',(-3.42067962509657,7.13322310757551,
7.99999999999995));
#217191=CARTESIAN_POINT('Ctrl Pts',(-3.44489616196924,7.12161026257943,
8.00108062834697));
#217192=CARTESIAN_POINT('Ctrl Pts',(-3.46905336347038,7.109874194047,8.00216253476664));
#217193=CARTESIAN_POINT('Ctrl Pts',(-3.52825103437878,7.08074121098439,
8.004823170029));
#217194=CARTESIAN_POINT('Ctrl Pts',(-3.56322308571844,7.06320696896667,
8.00640312738629));
#217195=CARTESIAN_POINT('Ctrl Pts',(-3.73207987925261,6.97697250955979,
8.01406979255727));
#217196=CARTESIAN_POINT('Ctrl Pts',(-3.86411558107353,6.90472128607229,
8.02018090088184));
#217197=CARTESIAN_POINT('Ctrl Pts',(-4.1228934846205,6.75336685075825,8.0323662050104));
#217198=CARTESIAN_POINT('Ctrl Pts',(-4.24961771503789,6.67435119686245,
8.03843788348709));
#217199=CARTESIAN_POINT('Ctrl Pts',(-4.47947890501097,6.52182529976682,
8.04963551657544));
#217200=CARTESIAN_POINT('Ctrl Pts',(-4.58323415501454,6.44933340920085,
8.05476307079416));
#217201=CARTESIAN_POINT('Ctrl Pts',(-4.72079991078508,6.34822184255562,
8.06166188123683));
#217202=CARTESIAN_POINT('Ctrl Pts',(-4.75617411126229,6.32176242800932,
8.06344512348087));
#217203=CARTESIAN_POINT('Ctrl Pts',(-4.82371178017375,6.27035742417348,
8.06686785533001));
#217204=CARTESIAN_POINT('Ctrl Pts',(-4.85590799614451,6.2454571577027,8.06850757265641));
#217205=CARTESIAN_POINT('Ctrl Pts',(-4.91919182907623,6.19572880863505,
8.07174681245983));
#217206=CARTESIAN_POINT('Ctrl Pts',(-4.95028717324043,6.1709124636523,8.07334636169313));
#217207=CARTESIAN_POINT('Ctrl Pts',(-5.03093952164691,6.10554409710508,
8.07751629300772));
#217208=CARTESIAN_POINT('Ctrl Pts',(-5.08019376990848,6.06462302989733,
8.08008398698963));
#217209=CARTESIAN_POINT('Ctrl Pts',(-5.26858972302629,5.90419545879211,
8.08999106706074));
#217210=CARTESIAN_POINT('Ctrl Pts',(-5.40405659601133,5.78046146870616,
8.09729751661436));
#217211=CARTESIAN_POINT('Ctrl Pts',(-5.7305208338707,5.46075679401348,8.11545169826978));
#217212=CARTESIAN_POINT('Ctrl Pts',(-5.91588381712733,5.25937752987953,
8.12626051285213));
#217213=CARTESIAN_POINT('Ctrl Pts',(-6.16201694618838,4.96246365723223,
8.14159012515508));
#217214=CARTESIAN_POINT('Ctrl Pts',(-6.231746020937,4.87461174296043,8.14605752741075));
#217215=CARTESIAN_POINT('Ctrl Pts',(-6.30121186644715,4.78316393843605,
8.1506538525498));
#217216=CARTESIAN_POINT('Ctrl Pts',(-6.30283924957226,4.78101930992288,
8.15076161551514));
#217217=CARTESIAN_POINT('Ctrl Pts',(-6.3052682769726,4.77781484794909,8.15092258868417));
#217218=CARTESIAN_POINT('Ctrl Pts',(-6.30607074968009,4.77675564226476,
8.15097578969882));
#217219=CARTESIAN_POINT('Ctrl Pts',(-6.30725841110619,4.7751871945745,8.15105455793406));
#217220=CARTESIAN_POINT('Ctrl Pts',(-6.30764380502466,4.77467810816932,
8.15108012285505));
#217221=CARTESIAN_POINT('Ctrl Pts',(-6.3098237178123,4.77179782608195,8.15122475336233));
#217222=CARTESIAN_POINT('Ctrl Pts',(-6.31161696088066,4.76942566584106,
8.15134383319784));
#217223=CARTESIAN_POINT('Ctrl Pts',(-6.31475886559297,4.76526457697446,
8.15155265297687));
#217224=CARTESIAN_POINT('Ctrl Pts',(-6.31610810579078,4.76347608528831,
8.15164238635198));
#217225=CARTESIAN_POINT('Ctrl Pts',(-6.31845356152026,4.76036430690394,
8.1517984776924));
#217226=CARTESIAN_POINT('Ctrl Pts',(-6.31945012162097,4.75904127990884,
8.15186483170955));
#217227=CARTESIAN_POINT('Ctrl Pts',(-6.32117176135778,4.7567541473838,8.15197951986239));
#217228=CARTESIAN_POINT('Ctrl Pts',(-6.32189703617846,4.7557901887276,8.15202785174711));
#217229=CARTESIAN_POINT('Ctrl Pts',(-6.32314405624532,4.75413199208373,
8.15211098210216));
#217230=CARTESIAN_POINT('Ctrl Pts',(-6.32366590774386,4.75343783397053,
8.15214577934082));
#217231=CARTESIAN_POINT('Ctrl Pts',(-6.32455997956009,4.75224814682945,
8.15220541170329));
#217232=CARTESIAN_POINT('Ctrl Pts',(-6.32493225598301,4.75175265994797,
8.15223024617435));
#217233=CARTESIAN_POINT('Ctrl Pts',(-6.32556840365334,4.75090576246467,
8.15227269123428));
#217234=CARTESIAN_POINT('Ctrl Pts',(-6.32583230384371,4.7505543736247,8.15229030148437));
#217235=CARTESIAN_POINT('Ctrl Pts',(-6.32628240796313,4.74995494619594,
8.15232034117433));
#217236=CARTESIAN_POINT('Ctrl Pts',(-6.32646862661027,4.74970691861204,
8.15233277044376));
#217237=CARTESIAN_POINT('Ctrl Pts',(-6.32746906980883,4.74837424915331,
8.15239955174269));
#217238=CARTESIAN_POINT('Ctrl Pts',(-6.32828302993814,4.74728940895812,
8.15245390686309));
#217239=CARTESIAN_POINT('Ctrl Pts',(-6.32981681244675,4.7452440992548,8.15255637203748));
#217240=CARTESIAN_POINT('Ctrl Pts',(-6.33053669530587,4.74428367512224,
8.152604481378));
#217241=CARTESIAN_POINT('Ctrl Pts',(-6.33189056223415,4.74247657102205,
8.15269499184989));
#217242=CARTESIAN_POINT('Ctrl Pts',(-6.33252459513822,4.74162992764851,
8.15273739240259));
#217243=CARTESIAN_POINT('Ctrl Pts',(-6.33371478693054,4.74003996393019,
8.15281701085052));
#217244=CARTESIAN_POINT('Ctrl Pts',(-6.33427098691357,4.73929666999183,
8.15285422842171));
#217245=CARTESIAN_POINT('Ctrl Pts',(-6.34690696063237,4.72240402291306,
8.15369998657488));
#217246=CARTESIAN_POINT('Ctrl Pts',(-6.35892504913736,4.706208658729,8.15450925886066));
#217247=CARTESIAN_POINT('Ctrl Pts',(-6.38185619673594,4.67505884530564,
8.15606295834953));
#217248=CARTESIAN_POINT('Ctrl Pts',(-6.3927789522268,4.66011169273404,8.15680725374525));
#217249=CARTESIAN_POINT('Ctrl Pts',(-6.41586478693557,4.62828616771946,
8.15838952923648));
#217250=CARTESIAN_POINT('Ctrl Pts',(-6.42801392534389,4.61139792103343,
8.15922772072681));
#217251=CARTESIAN_POINT('Ctrl Pts',(-6.46234659646926,4.56327352471234,
8.16161206849807));
#217252=CARTESIAN_POINT('Ctrl Pts',(-6.48436997999502,4.53192395569455,
8.16316030432853));
#217253=CARTESIAN_POINT('Ctrl Pts',(-6.59396487541828,4.37348471773237,
8.1709576194927));
#217254=CARTESIAN_POINT('Ctrl Pts',(-6.67803133589984,4.24401206271492,
8.17724056167673));
#217255=CARTESIAN_POINT('Ctrl Pts',(-6.84900707012616,3.96301699898009,
8.19063853914678));
#217256=CARTESIAN_POINT('Ctrl Pts',(-6.93479615302133,3.810905977909,8.19775058869798));
#217257=CARTESIAN_POINT('Ctrl Pts',(-7.04809404058325,3.59350397157942,
8.20769640499898));
#217258=CARTESIAN_POINT('Ctrl Pts',(-7.0798670713997,3.53049326770188,8.21055424082725));
#217259=CARTESIAN_POINT('Ctrl Pts',(-7.12892538659613,3.42987691122489,
8.2150781158383));
#217260=CARTESIAN_POINT('Ctrl Pts',(-7.14676585079713,3.39254634196463,
8.21674805274142));
#217261=CARTESIAN_POINT('Ctrl Pts',(-7.17719440879838,3.3275702850262,8.21964002157895));
#217262=CARTESIAN_POINT('Ctrl Pts',(-7.18991762787208,3.29998910514304,
8.22086307439478));
#217263=CARTESIAN_POINT('Ctrl Pts',(-7.21424617641942,3.24644143645658,
8.22322887644935));
#217264=CARTESIAN_POINT('Ctrl Pts',(-7.22587094006779,3.22048428920485,
8.22437176550019));
#217265=CARTESIAN_POINT('Ctrl Pts',(-7.24859866089076,3.16899253822501,
8.22663125844302));
#217266=CARTESIAN_POINT('Ctrl Pts',(-7.25970729108622,3.14346088041579,
8.22774789415815));
#217267=CARTESIAN_POINT('Ctrl Pts',(-7.28825882046671,3.07688049422375,
8.23065030612765));
#217268=CARTESIAN_POINT('Ctrl Pts',(-7.30548980830494,3.03574190125326,
8.23243428890514));
#217269=CARTESIAN_POINT('Ctrl Pts',(-7.36594846086816,2.88790195944531,
8.23881298128726));
#217270=CARTESIAN_POINT('Ctrl Pts',(-7.40719394056845,2.78040513357046,
8.24339067858313));
#217271=CARTESIAN_POINT('Ctrl Pts',(-7.55974311846658,2.35530268793264,
8.26128696507654));
#217272=CARTESIAN_POINT('Ctrl Pts',(-7.65308059558276,2.03163092083539,
8.27444842044223));
#217273=CARTESIAN_POINT('Ctrl Pts',(-7.74957012589917,1.59391405026631,
8.29211198302982));
#217274=CARTESIAN_POINT('Ctrl Pts',(-7.77130362350533,1.48433108845941,
8.29652511896635));
#217275=CARTESIAN_POINT('Ctrl Pts',(-7.80185086684639,1.31116637868868,
8.30351442441401));
#217276=CARTESIAN_POINT('Ctrl Pts',(-7.81222398254457,1.24787441711603,
8.30607233169107));
#217277=CARTESIAN_POINT('Ctrl Pts',(-7.82476727290191,1.16504247183047,
8.30942941745381));
#217278=CARTESIAN_POINT('Ctrl Pts',(-7.82763590111199,1.14561033173175,
8.31021766186169));
#217279=CARTESIAN_POINT('Ctrl Pts',(-7.83221168575533,1.11379413843461,
8.31150956172022));
#217280=CARTESIAN_POINT('Ctrl Pts',(-7.83396191720569,1.10141633910341,
8.31201248749622));
#217281=CARTESIAN_POINT('Ctrl Pts',(-7.83730150803856,1.07738773824884,
8.31298948906482));
#217282=CARTESIAN_POINT('Ctrl Pts',(-7.83889424480481,1.06573743685103,
8.31346350363929));
#217283=CARTESIAN_POINT('Ctrl Pts',(-7.84252165388203,1.03875612518575,
8.31456207680034));
#217284=CARTESIAN_POINT('Ctrl Pts',(-7.8445373542177,1.02342262792947,8.31518698476303));
#217285=CARTESIAN_POINT('Ctrl Pts',(-7.85014022691805,0.979812160872172,
8.31696614771628));
#217286=CARTESIAN_POINT('Ctrl Pts',(-7.85361952585118,0.951521820256821,
8.318122584369));
#217287=CARTESIAN_POINT('Ctrl Pts',(-7.8937873969268,0.609675840819445,
8.33212312057686));
#217288=CARTESIAN_POINT('Ctrl Pts',(-7.91182712553228,0.294221168223732,
8.34530284940324));
#217289=CARTESIAN_POINT('Ctrl Pts',(-7.90979792715798,-0.453916304909866,
8.37668785241045));
#217290=CARTESIAN_POINT('Ctrl Pts',(-7.87316573965032,-0.885560802343966,
8.39487570545381));
#217291=CARTESIAN_POINT('Ctrl Pts',(-7.76783241553769,-1.51187307472053,
8.42111027935031));
#217292=CARTESIAN_POINT('Ctrl Pts',(-7.7265602089607,-1.71033637076335,
8.4294061156004));
#217293=CARTESIAN_POINT('Ctrl Pts',(-7.66662143851645,-1.95165412892429,
8.43949037576807));
#217294=CARTESIAN_POINT('Ctrl Pts',(-7.65514048357083,-1.996211994601,8.44135233994781));
#217295=CARTESIAN_POINT('Ctrl Pts',(-7.63732356179955,-2.06294485578655,
8.44414139215461));
#217296=CARTESIAN_POINT('Ctrl Pts',(-7.63127833121435,-2.08519632190923,
8.44507145248801));
#217297=CARTESIAN_POINT('Ctrl Pts',(-7.61932656067252,-2.128440586409,8.44687920414763));
#217298=CARTESIAN_POINT('Ctrl Pts',(-7.61343032938801,-2.14943601689064,
8.44775699248032));
#217299=CARTESIAN_POINT('Ctrl Pts',(-7.60096872045207,-2.19311494033233,
8.44958346471322));
#217300=CARTESIAN_POINT('Ctrl Pts',(-7.59438843737883,-2.2157939653495,
8.45053198828996));
#217301=CARTESIAN_POINT('Ctrl Pts',(-7.57594732406781,-2.27830426595978,
8.4531470672118));
#217302=CARTESIAN_POINT('Ctrl Pts',(-7.56387399234706,-2.31807213727665,
8.45481146952113));
#217303=CARTESIAN_POINT('Ctrl Pts',(-7.51306425492964,-2.4808078936581,
8.46162689420654));
#217304=CARTESIAN_POINT('Ctrl Pts',(-7.47163781704315,-2.60291589587731,
8.46675105322172));
#217305=CARTESIAN_POINT('Ctrl Pts',(-7.34475073858618,-2.9488909578239,
8.48133476395445));
#217306=CARTESIAN_POINT('Ctrl Pts',(-7.25207831476744,-3.16996615482062,
8.49074969533208));
#217307=CARTESIAN_POINT('Ctrl Pts',(-6.92549199415194,-3.85944990412971,
8.52039672915874));
#217308=CARTESIAN_POINT('Ctrl Pts',(-6.65509131412303,-4.30901099874273,
8.54002080608389));
#217309=CARTESIAN_POINT('Ctrl Pts',(-6.12000715349156,-5.02669967795899,
8.5733643409996));
#217310=CARTESIAN_POINT('Ctrl Pts',(-5.87700617083448,-5.30876403512616,
8.58714527828322));
#217311=CARTESIAN_POINT('Ctrl Pts',(-5.5301472547523,-5.65826214385748,
8.60618930549681));
#217312=CARTESIAN_POINT('Ctrl Pts',(-5.4432687188775,-5.74188847932049,
8.61091576102426));
#217313=CARTESIAN_POINT('Ctrl Pts',(-5.34282275833126,-5.83424530474291,
8.61636969928414));
#217314=CARTESIAN_POINT('Ctrl Pts',(-5.33109779227009,-5.84496104588815,
8.61700617691609));
#217315=CARTESIAN_POINT('Ctrl Pts',(-5.31337811782222,-5.86105782835972,
8.61796795665845));
#217316=CARTESIAN_POINT('Ctrl Pts',(-5.30740729686589,-5.86646517716934,
8.61829201846961));
#217317=CARTESIAN_POINT('Ctrl Pts',(-5.29714895474028,-5.87572694997919,
8.61884876678747));
#217318=CARTESIAN_POINT('Ctrl Pts',(-5.29286545322486,-5.87958583008033,
8.61908123953142));
#217319=CARTESIAN_POINT('Ctrl Pts',(-5.28405732787018,-5.88750338436385,
8.61955926953376));
#217320=CARTESIAN_POINT('Ctrl Pts',(-5.27953223832777,-5.89156153233657,
8.61980485198002));
#217321=CARTESIAN_POINT('Ctrl Pts',(-5.26739156119237,-5.90242420026434,
8.6204637519577));
#217322=CARTESIAN_POINT('Ctrl Pts',(-5.25976748102481,-5.90921918218692,
8.62087753703051));
#217323=CARTESIAN_POINT('Ctrl Pts',(-5.23208151202193,-5.93379834581175,
8.62238026485478));
#217324=CARTESIAN_POINT('Ctrl Pts',(-5.21194254755674,-5.9514951579442,
8.62347357727135));
#217325=CARTESIAN_POINT('Ctrl Pts',(-4.88789553212716,-6.23334042000821,
8.6410753294484));
#217326=CARTESIAN_POINT('Ctrl Pts',(-4.56440662098179,-6.47395701534081,
8.65899822507158));
#217327=CARTESIAN_POINT('Ctrl Pts',(-3.86466130504848,-6.91585285960687,
8.696577733721));
#217328=CARTESIAN_POINT('Ctrl Pts',(-3.48750813687489,-7.1135040855648,
8.71616210765956));
#217329=CARTESIAN_POINT('Ctrl Pts',(-2.82386912088756,-7.39576409731374,
8.74824627365588));
#217330=CARTESIAN_POINT('Ctrl Pts',(-2.54513820613614,-7.49625619154637,
8.76107714788845));
#217331=CARTESIAN_POINT('Ctrl Pts',(-2.15302756136409,-7.61322439324809,
8.77813941959008));
#217332=CARTESIAN_POINT('Ctrl Pts',(-2.04396038013496,-7.64322841792792,
8.78278446980245));
#217333=CARTESIAN_POINT('Ctrl Pts',(-1.9172706737058,-7.67517439757066,
8.78806561117108));
#217334=CARTESIAN_POINT('Ctrl Pts',(-1.90024273767793,-7.67940794672888,
8.78877306735934));
#217335=CARTESIAN_POINT('Ctrl Pts',(-1.87438460940062,-7.6857456196566,
8.78984382309759));
#217336=CARTESIAN_POINT('Ctrl Pts',(-1.86556470013447,-7.68789124170809,
8.7902084169985));
#217337=CARTESIAN_POINT('Ctrl Pts',(-1.84960236412615,-7.69174531735599,
8.79086712840494));
#217338=CARTESIAN_POINT('Ctrl Pts',(-1.84246122076305,-7.69345901287549,
8.79116140926346));
#217339=CARTESIAN_POINT('Ctrl Pts',(-1.82820648524223,-7.69685880688339,
8.7917480200298));
#217340=CARTESIAN_POINT('Ctrl Pts',(-1.82109292155917,-7.69854499351601,
8.79204035245549));
#217341=CARTESIAN_POINT('Ctrl Pts',(-1.80114541562527,-7.70324412044258,
8.79285896504975));
#217342=CARTESIAN_POINT('Ctrl Pts',(-1.78830623842805,-7.70623485153833,
8.7933845513515));
#217343=CARTESIAN_POINT('Ctrl Pts',(-1.73604959542368,-7.71826977568501,
8.79551842901275));
#217344=CARTESIAN_POINT('Ctrl Pts',(-1.69657021646568,-7.72704381304776,
8.79711827669385));
#217345=CARTESIAN_POINT('Ctrl Pts',(-1.08097459703194,-7.85891057407248,
8.82187726823715));
#217346=CARTESIAN_POINT('Ctrl Pts',(-0.492939563608088,-7.91758073475562,
8.8427895216776));
#217347=CARTESIAN_POINT('Ctrl Pts',(0.498700126488024,-7.90551948604952,
8.87683658463479));
#217348=CARTESIAN_POINT('Ctrl Pts',(0.900212089266585,-7.86991355186963,
8.89034209444207));
#217349=CARTESIAN_POINT('Ctrl Pts',(1.60335781328868,-7.75302857782367,
8.91555906642412));
#217350=CARTESIAN_POINT('Ctrl Pts',(1.90617520529572,-7.68418315985583,
8.92696273711215));
#217351=CARTESIAN_POINT('Ctrl Pts',(2.21931325853927,-7.59334045926619,
8.93999892752131));
#217352=CARTESIAN_POINT('Ctrl Pts',(2.23447519837941,-7.58889262350306,
8.94063325872745));
#217353=CARTESIAN_POINT('Ctrl Pts',(2.2553982569527,-7.58268659400234,8.941513059558));
#217354=CARTESIAN_POINT('Ctrl Pts',(2.2611709305597,-7.58096717462512,8.94175626436494));
#217355=CARTESIAN_POINT('Ctrl Pts',(2.27090358374208,-7.57805615014655,
8.94216710155076));
#217356=CARTESIAN_POINT('Ctrl Pts',(2.27486461068765,-7.57686802738072,
8.94233452824279));
#217357=CARTESIAN_POINT('Ctrl Pts',(2.28269272720289,-7.57451326678125,
8.94266585464807));
#217358=CARTESIAN_POINT('Ctrl Pts',(2.28655985908946,-7.57334677181498,
8.94282974583779));
#217359=CARTESIAN_POINT('Ctrl Pts',(2.29506930743921,-7.57077284073997,
8.94319085555833));
#217360=CARTESIAN_POINT('Ctrl Pts',(2.29971122277883,-7.56936409638567,
8.94338815246656));
#217361=CARTESIAN_POINT('Ctrl Pts',(2.31585486381004,-7.56444854813234,
8.94407540219058));
#217362=CARTESIAN_POINT('Ctrl Pts',(2.32734983343493,-7.56091980761333,
8.94456668127522));
#217363=CARTESIAN_POINT('Ctrl Pts',(2.45647386626368,-7.52095878618009,
8.9501073689217));
#217364=CARTESIAN_POINT('Ctrl Pts',(2.57323747096091,-7.48181327451927,
8.95532581378026));
#217365=CARTESIAN_POINT('Ctrl Pts',(2.99794759519844,-7.32830990784588,
8.9749363266347));
#217366=CARTESIAN_POINT('Ctrl Pts',(3.29959143545574,-7.1975332729554,8.99008272993728));
#217367=CARTESIAN_POINT('Ctrl Pts',(3.91938148001642,-6.88165767235397,
9.02251466157164));
#217368=CARTESIAN_POINT('Ctrl Pts',(4.23455881289234,-6.69233105866938,
9.03979261809929));
#217369=CARTESIAN_POINT('Ctrl Pts',(4.72427383600306,-6.34966685206859,
9.06703758044295));
#217370=CARTESIAN_POINT('Ctrl Pts',(4.90724289830053,-6.20934865775254,
9.07732509576453));
#217371=CARTESIAN_POINT('Ctrl Pts',(5.20430401176946,-5.96018988961546,
9.09410929961352));
#217372=CARTESIAN_POINT('Ctrl Pts',(5.32173892719841,-5.8555736394445,9.10076921216874));
#217373=CARTESIAN_POINT('Ctrl Pts',(5.49568602894485,-5.69105517716831,
9.11066798351163));
#217374=CARTESIAN_POINT('Ctrl Pts',(5.55450678978714,-5.6336603436928,9.11402177596556));
#217375=CARTESIAN_POINT('Ctrl Pts',(5.62280848796092,-5.56490456551562,
9.11792517107459));
#217376=CARTESIAN_POINT('Ctrl Pts',(5.63316383217025,-5.55442196442253,
9.11851722446226));
#217377=CARTESIAN_POINT('Ctrl Pts',(5.64899794935275,-5.53830343569123,
9.11942292278793));
#217378=CARTESIAN_POINT('Ctrl Pts',(5.65449768162376,-5.53268820254622,
9.11973757794163));
#217379=CARTESIAN_POINT('Ctrl Pts',(5.66407845598095,-5.52287701339287,
9.12028585489125));
#217380=CARTESIAN_POINT('Ctrl Pts',(5.6681632216031,-5.51868471232471,9.12051965553829));
#217381=CARTESIAN_POINT('Ctrl Pts',(5.6766979757651,-5.50990580057034,9.12100825188447));
#217382=CARTESIAN_POINT('Ctrl Pts',(5.68114706824986,-5.5053183221685,9.12126300462157));
#217383=CARTESIAN_POINT('Ctrl Pts',(5.69344541874112,-5.49260665592771,
9.12196734778831));
#217384=CARTESIAN_POINT('Ctrl Pts',(5.70128285663692,-5.48447102308259,
9.12241637344519));
#217385=CARTESIAN_POINT('Ctrl Pts',(5.73201339647766,-5.45243420681422,
9.12417767104035));
#217386=CARTESIAN_POINT('Ctrl Pts',(5.75477400728524,-5.42840607537118,
9.12548364528953));
#217387=CARTESIAN_POINT('Ctrl Pts',(6.12187832434344,-5.03595420531949,
9.14657409822095));
#217388=CARTESIAN_POINT('Ctrl Pts',(6.43038966284449,-4.63555747130408,
9.16456425362355));
#217389=CARTESIAN_POINT('Ctrl Pts',(7.08646316922651,-3.59127621927101,
9.2067079651504));
#217390=CARTESIAN_POINT('Ctrl Pts',(7.38699512295196,-2.92355531425107,
9.22973078807729));
#217391=CARTESIAN_POINT('Ctrl Pts',(7.6038522267635,-2.18338470808729,9.25998610153256));
#217392=CARTESIAN_POINT('Ctrl Pts',(7.61550460888024,-2.14238814548624,
9.26167744732356));
#217393=CARTESIAN_POINT('Ctrl Pts',(7.62891588902088,-2.09371089685046,
9.26370627919391));
#217394=CARTESIAN_POINT('Ctrl Pts',(7.63099537570652,-2.08611901300698,
9.26402328938701));
#217395=CARTESIAN_POINT('Ctrl Pts',(7.63436342753745,-2.0737503548789,9.2645407001706));
#217396=CARTESIAN_POINT('Ctrl Pts',(7.63565885283248,-2.06897543750131,
9.26474067426841));
#217397=CARTESIAN_POINT('Ctrl Pts',(7.63795803150873,-2.06046913099128,
9.26509732101109));
#217398=CARTESIAN_POINT('Ctrl Pts',(7.63896353359213,-2.0567382096906,9.26525388610885));
#217399=CARTESIAN_POINT('Ctrl Pts',(7.64107401745293,-2.04888434994692,
9.26558375412748));
#217400=CARTESIAN_POINT('Ctrl Pts',(7.64217839629818,-2.04476125224057,
9.26575709378419));
#217401=CARTESIAN_POINT('Ctrl Pts',(7.6450777929925,-2.0339014588578,9.26621408614928));
#217402=CARTESIAN_POINT('Ctrl Pts',(7.64686723993238,-2.02716329374114,
9.26649807578861));
#217403=CARTESIAN_POINT('Ctrl Pts',(7.65482219121028,-1.99704849768258,
9.26776924458624));
#217404=CARTESIAN_POINT('Ctrl Pts',(7.66088936497753,-1.97364626868803,
9.26876228375342));
#217405=CARTESIAN_POINT('Ctrl Pts',(7.70474513229622,-1.80123695377259,
9.2761146287747));
#217406=CARTESIAN_POINT('Ctrl Pts',(7.73828859033302,-1.6511924094569,9.28271278229449));
#217407=CARTESIAN_POINT('Ctrl Pts',(7.79736812662115,-1.34531744521089,
9.29643359665464));
#217408=CARTESIAN_POINT('Ctrl Pts',(7.82265325323392,-1.18950447270505,
9.30356245239264));
#217409=CARTESIAN_POINT('Ctrl Pts',(7.89758369537892,-0.620605514863718,
9.32985966080013));
#217410=CARTESIAN_POINT('Ctrl Pts',(7.91928986533777,-0.2045248942233,9.349568273859));
#217411=CARTESIAN_POINT('Ctrl Pts',(7.89264723839935,0.792453647545537,
9.39578604552791));
#217412=CARTESIAN_POINT('Ctrl Pts',(7.81311147433822,1.37016149131502,9.42163842289761));
#217413=CARTESIAN_POINT('Ctrl Pts',(7.66160148988842,1.97110300776564,9.44690877800006));
#217414=CARTESIAN_POINT('Ctrl Pts',(7.6519801942013,2.00812938300014,9.44845986946134));
#217415=CARTESIAN_POINT('Ctrl Pts',(7.6388787103723,2.05708711986375,9.45050317920551));
#217416=CARTESIAN_POINT('Ctrl Pts',(7.6356385296699,2.06908182935054,9.45100318645236));
#217417=CARTESIAN_POINT('Ctrl Pts',(7.63032679423929,2.08856274649633,9.45181428706856));
#217418=CARTESIAN_POINT('Ctrl Pts',(7.62827245397738,2.09605360171813,9.45212593929718));
#217419=CARTESIAN_POINT('Ctrl Pts',(7.6243394656068,2.11031231005066,9.45271872080262));
#217420=CARTESIAN_POINT('Ctrl Pts',(7.62246283093478,2.11708070798162,9.45299991515602));
#217421=CARTESIAN_POINT('Ctrl Pts',(7.61820010234857,2.13237581077174,9.45363492606483));
#217422=CARTESIAN_POINT('Ctrl Pts',(7.61580870054306,2.14090103348527,9.45398856976115));
#217423=CARTESIAN_POINT('Ctrl Pts',(7.60857340135766,2.16652896612847,9.45505077443395));
#217424=CARTESIAN_POINT('Ctrl Pts',(7.60368615428648,2.18361943509198,9.4557579263014));
#217425=CARTESIAN_POINT('Ctrl Pts',(7.56250933965201,2.32579824513729,9.46163107417658));
#217426=CARTESIAN_POINT('Ctrl Pts',(7.52319240390765,2.44999244817969,9.46669771973346));
#217427=CARTESIAN_POINT('Ctrl Pts',(7.38863419824306,2.84118665214395,9.48249621903437));
#217428=CARTESIAN_POINT('Ctrl Pts',(7.28210197882458,3.10407183805344,9.49286343175283));
#217429=CARTESIAN_POINT('Ctrl Pts',(7.07471645379601,3.54601451104537,9.51024887179538));
#217430=CARTESIAN_POINT('Ctrl Pts',(6.98058610601986,3.72790180133291,9.5173934847611));
#217431=CARTESIAN_POINT('Ctrl Pts',(6.57523560630917,4.44184372847885,9.54588894983493));
#217432=CARTESIAN_POINT('Ctrl Pts',(6.20937960948001,4.94037819754794,9.56679781001265));
#217433=CARTESIAN_POINT('Ctrl Pts',(5.76071160169085,5.42216672155814,9.59278744616902));
#217434=CARTESIAN_POINT('Ctrl Pts',(5.73180223121717,5.45271796575667,9.59446081963003));
#217435=CARTESIAN_POINT('Ctrl Pts',(5.69381543785865,5.49222625818714,9.59665663435051));
#217436=CARTESIAN_POINT('Ctrl Pts',(5.68495775314304,5.50139426457833,9.5971684412104));
#217437=CARTESIAN_POINT('Ctrl Pts',(5.67076897038288,5.51600927976661,9.59798790558535));
#217438=CARTESIAN_POINT('Ctrl Pts',(5.66545207416039,5.52147008367058,9.5982948950159));
#217439=CARTESIAN_POINT('Ctrl Pts',(5.65586163453775,5.53129166203543,9.59884846903116));
#217440=CARTESIAN_POINT('Ctrl Pts',(5.6515909145629,5.53565519281628,9.59909492306821));
#217441=CARTESIAN_POINT('Ctrl Pts',(5.64156153664911,5.54587882406283,9.59967355339112));
#217442=CARTESIAN_POINT('Ctrl Pts',(5.63579879814406,5.55173490084542,9.60000591557709));
#217443=CARTESIAN_POINT('Ctrl Pts',(5.61916621858536,5.56858429176758,9.60096484867161));
#217444=CARTESIAN_POINT('Ctrl Pts',(5.60827328947805,5.57955470567329,9.60159245127284));
#217445=CARTESIAN_POINT('Ctrl Pts',(5.53470338399272,5.6532148248611,9.60582808725772));
#217446=CARTESIAN_POINT('Ctrl Pts',(5.47100971574863,5.71487808433386,9.6094797680974));
#217447=CARTESIAN_POINT('Ctrl Pts',(5.25727196141003,5.91495390594267,9.62165454972014));
#217448=CARTESIAN_POINT('Ctrl Pts',(5.10290932243144,6.04862799950733,9.6303200133286));
#217449=CARTESIAN_POINT('Ctrl Pts',(4.42223601261422,6.5934544330793,9.66762994998348));
#217450=CARTESIAN_POINT('Ctrl Pts',(3.85013693435381,6.94307877578777,9.69649600156466));
#217451=CARTESIAN_POINT('Ctrl Pts',(3.14231015407456,7.26095700003366,9.72889892547154));
#217452=CARTESIAN_POINT('Ctrl Pts',(3.04278682675111,7.30322246066215,9.73339336601753));
#217453=CARTESIAN_POINT('Ctrl Pts',(2.91367789026081,7.35495488883782,9.73915505654857));
#217454=CARTESIAN_POINT('Ctrl Pts',(2.88486048458015,7.36630574005381,9.74043674199395));
#217455=CARTESIAN_POINT('Ctrl Pts',(2.84214898383273,7.38284024120973,9.74233030508017));
#217456=CARTESIAN_POINT('Ctrl Pts',(2.82830581752351,7.38815451088679,9.74294308565485));
#217457=CARTESIAN_POINT('Ctrl Pts',(2.81206961885348,7.39433512453511,9.74366072600313));
#217458=CARTESIAN_POINT('Ctrl Pts',(2.80969101912654,7.39523926943917,9.74376583329986));
#217459=CARTESIAN_POINT('Ctrl Pts',(2.53833544134911,7.49823617482062,9.7557536423545));
#217460=CARTESIAN_POINT('Ctrl Pts',(2.26398198238071,7.58558402445757,9.76755953217075));
#217461=CARTESIAN_POINT('Ctrl Pts',(1.95635801204336,7.66534339291514,9.7804277693657));
#217462=CARTESIAN_POINT('Ctrl Pts',(1.92719472409004,7.67272744901626,9.78164411088452));
#217463=CARTESIAN_POINT('Ctrl Pts',(1.87252058520879,7.6862393903802,9.78391776903705));
#217464=CARTESIAN_POINT('Ctrl Pts',(1.84702000553859,7.69240706238575,9.78497551309459));
#217465=CARTESIAN_POINT('Ctrl Pts',(1.80340324981471,7.70272699311088,9.78678009964377));
#217466=CARTESIAN_POINT('Ctrl Pts',(1.78530228686225,7.70694246498242,9.78752765334314));
#217467=CARTESIAN_POINT('Ctrl Pts',(1.74817532058392,7.71545102117662,9.78905821625662));
#217468=CARTESIAN_POINT('Ctrl Pts',(1.72914795375515,7.71973761006485,9.78984114592412));
#217469=CARTESIAN_POINT('Ctrl Pts',(1.68516052862311,7.72947654858285,9.79164774327979));
#217470=CARTESIAN_POINT('Ctrl Pts',(1.66018949870662,7.73487844484264,9.79267081545002));
#217471=CARTESIAN_POINT('Ctrl Pts',(1.58133026134982,7.7515383148923,9.79589391045869));
#217472=CARTESIAN_POINT('Ctrl Pts',(1.52735028119158,7.76235485013393,9.79808867987738));
#217473=CARTESIAN_POINT('Ctrl Pts',(1.15567060102562,7.83280500539108,9.81312519086709));
#217474=CARTESIAN_POINT('Ctrl Pts',(0.834683732020157,7.87348213233303,
9.82571745476222));
#217475=CARTESIAN_POINT('Ctrl Pts',(-0.0336831296969686,7.9298121911959,
9.85927095986215));
#217476=CARTESIAN_POINT('Ctrl Pts',(-0.581643712634404,7.908520471578,9.87984168800481));
#217477=CARTESIAN_POINT('Ctrl Pts',(-1.16169251647472,7.82533833442156,
9.90316819721011));
#217478=CARTESIAN_POINT('Ctrl Pts',(-1.20035142683879,7.81950164489381,
9.90473083611415));
#217479=CARTESIAN_POINT('Ctrl Pts',(-1.2522571329176,7.81127097136814,9.90684093613767));
#217480=CARTESIAN_POINT('Ctrl Pts',(-1.26554353129027,7.80912938064962,
9.90738211366105));
#217481=CARTESIAN_POINT('Ctrl Pts',(-1.28832949067893,7.80539690823245,
9.90831198862464));
#217482=CARTESIAN_POINT('Ctrl Pts',(-1.2978317463643,7.80382255879118,9.90870029426351));
#217483=CARTESIAN_POINT('Ctrl Pts',(-1.31635524007655,7.80071878762672,
9.90945826015159));
#217484=CARTESIAN_POINT('Ctrl Pts',(-1.32537674897428,7.79919106026147,
9.90982788088646));
#217485=CARTESIAN_POINT('Ctrl Pts',(-1.34702906569414,7.79548574338497,
9.91071610593231));
#217486=CARTESIAN_POINT('Ctrl Pts',(-1.35965725901217,7.79329310469952,
9.91123504670571));
#217487=CARTESIAN_POINT('Ctrl Pts',(-1.39784794995567,7.78656638753121,
9.91280712745014));
#217488=CARTESIAN_POINT('Ctrl Pts',(-1.42339343266007,7.78193717036247,
9.91386231549853));
#217489=CARTESIAN_POINT('Ctrl Pts',(-1.70902205249713,7.72872358544662,
9.9256994715271));
#217490=CARTESIAN_POINT('Ctrl Pts',(-1.96652822247709,7.66724755259749,
9.93672809268633));
#217491=CARTESIAN_POINT('Ctrl Pts',(-2.78182758172099,7.42882468809274,
9.97234953166494));
#217492=CARTESIAN_POINT('Ctrl Pts',(-3.32328334586225,7.20290471528132,
9.99697633622257));
#217493=CARTESIAN_POINT('Ctrl Pts',(-3.92288690088566,6.87058973624737,
10.0249691290664));
#217494=CARTESIAN_POINT('Ctrl Pts',(-4.00995457972157,6.82013999539848,
10.029057264785));
#217495=CARTESIAN_POINT('Ctrl Pts',(-4.12866891743919,6.74829377258149,
10.0346680884985));
#217496=CARTESIAN_POINT('Ctrl Pts',(-4.16115777523213,6.7283089894796,10.0362075068509));
#217497=CARTESIAN_POINT('Ctrl Pts',(-4.21298763673543,6.69590802686731,
10.0386699752365));
#217498=CARTESIAN_POINT('Ctrl Pts',(-4.23242120734334,6.68364121261004,
10.0395947820479));
#217499=CARTESIAN_POINT('Ctrl Pts',(-4.27252132323462,6.65808427841552,
10.0415063061666));
#217500=CARTESIAN_POINT('Ctrl Pts',(-4.29317996488126,6.64478220181507,
10.0424928710688));
#217501=CARTESIAN_POINT('Ctrl Pts',(-4.34147536410036,6.61336560038426,
10.0448036249742));
#217502=CARTESIAN_POINT('Ctrl Pts',(-4.36906129055225,6.59517371653357,
10.0461268964245));
#217503=CARTESIAN_POINT('Ctrl Pts',(-4.45972194159991,6.53456796249722,
10.0504876425986));
#217504=CARTESIAN_POINT('Ctrl Pts',(-4.52229963154844,6.49141775047207,
10.0535166375223));
#217505=CARTESIAN_POINT('Ctrl Pts',(-5.16806420843812,6.03226266903351,
10.0850011382433));
#217506=CARTESIAN_POINT('Ctrl Pts',(-5.69283409008161,5.53975028330331,
10.1124983806052));
#217507=CARTESIAN_POINT('Ctrl Pts',(-6.41964869114742,4.64363384768455,
10.1554422904928));
#217508=CARTESIAN_POINT('Ctrl Pts',(-6.66650918132427,4.28168792692901,
10.1714367569983));
#217509=CARTESIAN_POINT('Ctrl Pts',(-6.89831648685216,3.8727536663235,10.1894478531826));
#217510=CARTESIAN_POINT('Ctrl Pts',(-6.91427301630708,3.84419301607496,
10.1907058099702));
#217511=CARTESIAN_POINT('Ctrl Pts',(-6.98701317872356,3.7120770274598,10.1965280651845));
#217512=CARTESIAN_POINT('Ctrl Pts',(-7.04164921538346,3.60735967999222,
10.2011516576573));
#217513=CARTESIAN_POINT('Ctrl Pts',(-7.10127255207553,3.48656351853141,
10.2065326914923));
#217514=CARTESIAN_POINT('Ctrl Pts',(-7.10857907143045,3.47164235021424,
10.2071981955016));
#217515=CARTESIAN_POINT('Ctrl Pts',(-7.11925442818967,3.44966643359212,
10.2081796956698));
#217516=CARTESIAN_POINT('Ctrl Pts',(-7.12265992404065,3.44262947792414,
10.2084941861709));
#217517=CARTESIAN_POINT('Ctrl Pts',(-7.12870009848692,3.43010101950255,
10.2090544763789));
#217518=CARTESIAN_POINT('Ctrl Pts',(-7.13133887937239,3.42461149408941,
10.2093001043395));
#217519=CARTESIAN_POINT('Ctrl Pts',(-7.13682958475998,3.41315516997417,
10.2098129940607));
#217520=CARTESIAN_POINT('Ctrl Pts',(-7.13968037130188,3.40718783332111,
10.2100803037653));
#217521=CARTESIAN_POINT('Ctrl Pts',(-7.14706152367414,3.39168748258723,
10.2107750732467));
#217522=CARTESIAN_POINT('Ctrl Pts',(-7.15158029105656,3.38214898280205,
10.2112030313548));
#217523=CARTESIAN_POINT('Ctrl Pts',(-7.17077326217329,3.34142480128834,
10.2130320570353));
#217524=CARTESIAN_POINT('Ctrl Pts',(-7.18526252518813,3.3101527565099,10.2144412536191));
#217525=CARTESIAN_POINT('Ctrl Pts',(-7.28015388339508,3.10179073269101,
10.2238675213317));
#217526=CARTESIAN_POINT('Ctrl Pts',(-7.35419520899954,2.92190698075219,
10.2322134055462));
#217527=CARTESIAN_POINT('Ctrl Pts',(-7.74520097764315,1.86263999763756,
10.2820008873398));
#217528=CARTESIAN_POINT('Ctrl Pts',(-7.91095464617904,0.935317427441046,
10.327041855684));
#217529=CARTESIAN_POINT('Ctrl Pts',(-7.91099999069558,0.000383685446136151,
10.3667112445445));
#217530=CARTESIAN_POINT('',(-7.91258408968956,-0.00269315930910046,12.3576684917633));
#217531=CARTESIAN_POINT('Ctrl Pts',(-7.911,-6.54698517621455E-12,10.3576684917633));
#217532=CARTESIAN_POINT('Ctrl Pts',(-7.91099999999818,-2.20167589667329,
10.446255927496));
#217533=CARTESIAN_POINT('Ctrl Pts',(-6.9421457667201,-4.38610418339253,
10.5348433632287));
#217534=CARTESIAN_POINT('Ctrl Pts',(-3.67820201487687,-7.34180684107932,
10.7120182346942));
#217535=CARTESIAN_POINT('Ctrl Pts',(-1.40868175871086,-8.0899266657145,
10.8006056704269));
#217536=CARTESIAN_POINT('Ctrl Pts',(2.97309270521891,-7.65454228025016,
10.9777805418924));
#217537=CARTESIAN_POINT('Ctrl Pts',(5.05102072676122,-6.47444880833819,
11.0663679776251));
#217538=CARTESIAN_POINT('Ctrl Pts',(7.66951518848105,-2.93425195367096,
11.2435428490905));
#217539=CARTESIAN_POINT('Ctrl Pts',(8.18956872247118,-0.601881960092681,
11.3321302848233));
#217540=CARTESIAN_POINT('Ctrl Pts',(7.3230668976105,3.71537198233024,11.5093051562887));
#217541=CARTESIAN_POINT('Ctrl Pts',(5.94329958849758,5.66643518936975,11.5978925920214));
#217542=CARTESIAN_POINT('Ctrl Pts',(2.16154501637234,7.92205913233164,11.7750674634869));
#217543=CARTESIAN_POINT('Ctrl Pts',(-0.210816529306694,8.20894963712986,
11.8636548992196));
#217544=CARTESIAN_POINT('Ctrl Pts',(-4.42123908576965,6.91982244717493,
12.0408297706851));
#217545=CARTESIAN_POINT('Ctrl Pts',(-6.22631625634594,5.35390358803047,
12.1294172064178));
#217546=CARTESIAN_POINT('Ctrl Pts',(-7.65317280859671,2.31334857513923,
12.2645592586881));
#217547=CARTESIAN_POINT('Ctrl Pts',(-7.91100000000096,1.15702837835884,
12.3111138752257));
#217548=CARTESIAN_POINT('Ctrl Pts',(-7.911,-6.53810339201755E-12,12.3576684917633));
#217549=CARTESIAN_POINT('',(-7.91331685262984,-0.000560519916223401,14.3576684617817));
#217550=CARTESIAN_POINT('Ctrl Pts',(-7.91258408968956,-0.00269315930910046,
12.3576684917633));
#217551=CARTESIAN_POINT('Ctrl Pts',(-7.91593504939377,-0.776264288801357,
12.3886864088733));
#217552=CARTESIAN_POINT('Ctrl Pts',(-7.43681856913235,-4.19026845229773,
12.5256739031998));
#217553=CARTESIAN_POINT('Ctrl Pts',(-3.65584480504754,-7.92457769675913,
12.7156461861345));
#217554=CARTESIAN_POINT('Ctrl Pts',(1.79759080058233,-8.02852789826421,
12.9275853405675));
#217555=CARTESIAN_POINT('Ctrl Pts',(6.66378542679534,-5.62439576614873,
13.1395244950005));
#217556=CARTESIAN_POINT('Ctrl Pts',(9.26557616308506,1.35890735276843,13.4044484380419));
#217557=CARTESIAN_POINT('Ctrl Pts',(3.84357001655874,8.53192481528771,13.7223571696913));
#217558=CARTESIAN_POINT('Ctrl Pts',(-3.5690748421245,7.95640288263857,13.9872811127326));
#217559=CARTESIAN_POINT('Ctrl Pts',(-7.23560627100123,3.93118237953513,
14.1990515434295));
#217560=CARTESIAN_POINT('Ctrl Pts',(-7.91285669218149,1.3077251098878,14.3048523969097));
#217561=CARTESIAN_POINT('Ctrl Pts',(-7.91331685262984,-0.000560519916223401,
14.3576684617817));
#217562=CARTESIAN_POINT('',(-7.91099988478435,0.00135016367355217,18.3664967938599));
#217563=CARTESIAN_POINT('Ctrl Pts',(-7.91099997617816,-0.000613929265750893,
14.3563333568247));
#217564=CARTESIAN_POINT('Ctrl Pts',(-7.91099935780322,-0.00858221555712144,
14.3566531921185));
#217565=CARTESIAN_POINT('Ctrl Pts',(-7.91098670047397,-0.0165504911307802,
14.3569733132972));
#217566=CARTESIAN_POINT('Ctrl Pts',(-7.91092601335387,-0.0361311553618632,
14.3577606644224));
#217567=CARTESIAN_POINT('Ctrl Pts',(-7.91086445415868,-0.047743438954302,
14.3582282105699));
#217568=CARTESIAN_POINT('Ctrl Pts',(-7.91070448295947,-0.069064059512712,
14.3590877341926));
#217569=CARTESIAN_POINT('Ctrl Pts',(-7.91061376652499,-0.0787724397538128,
14.3594795347212));
#217570=CARTESIAN_POINT('Ctrl Pts',(-7.91039648001536,-0.0981986849055518,
14.3602643315667));
#217571=CARTESIAN_POINT('Ctrl Pts',(-7.91026987364833,-0.107916533444963,
14.3606573280512));
#217572=CARTESIAN_POINT('Ctrl Pts',(-7.9098819762533,-0.134000099461685,
14.3617132350183));
#217573=CARTESIAN_POINT('Ctrl Pts',(-7.9095878016966,-0.150365253041726,
14.3623768544412));
#217574=CARTESIAN_POINT('Ctrl Pts',(-7.90832284448457,-0.210371813784779,
14.3648141611594));
#217575=CARTESIAN_POINT('Ctrl Pts',(-7.90704164589483,-0.254005656347762,
14.3665941987198));
#217576=CARTESIAN_POINT('Ctrl Pts',(-7.8880309044882,-0.758959250380348,
14.387274724489));
#217577=CARTESIAN_POINT('Ctrl Pts',(-7.83031338981521,-1.21788090148529,
14.4068061599072));
#217578=CARTESIAN_POINT('Ctrl Pts',(-7.6498456347303,-2.05396554232061,
14.4426578333511));
#217579=CARTESIAN_POINT('Ctrl Pts',(-7.53816870490578,-2.43206548002689,
14.4589848871743));
#217580=CARTESIAN_POINT('Ctrl Pts',(-7.38111865470644,-2.84701684970282,
14.4770303286938));
#217581=CARTESIAN_POINT('Ctrl Pts',(-7.3629898367631,-2.89357879468404,
14.4790575499912));
#217582=CARTESIAN_POINT('Ctrl Pts',(-7.33274298028933,-2.9691394119104,
14.482351778737));
#217583=CARTESIAN_POINT('Ctrl Pts',(-7.32089115934277,-2.99824300302658,
14.4836217013238));
#217584=CARTESIAN_POINT('Ctrl Pts',(-7.29972140117194,-3.04935395798992,
14.4858540321543));
#217585=CARTESIAN_POINT('Ctrl Pts',(-7.29047657110277,-3.071391128832,14.4868172319709));
#217586=CARTESIAN_POINT('Ctrl Pts',(-7.27155223407225,-3.11593474258506,
14.488765678678));
#217587=CARTESIAN_POINT('Ctrl Pts',(-7.26186774619344,-3.13843879248177,
14.489750859617));
#217588=CARTESIAN_POINT('Ctrl Pts',(-7.24286345297947,-3.18204053268,14.4916613357138));
#217589=CARTESIAN_POINT('Ctrl Pts',(-7.23355561343504,-3.20314316587706,
14.4925867487731));
#217590=CARTESIAN_POINT('Ctrl Pts',(-7.21103171141795,-3.25361023657898,
14.4948018678875));
#217591=CARTESIAN_POINT('Ctrl Pts',(-7.19772837024615,-3.28293530736774,
14.4960906347056));
#217592=CARTESIAN_POINT('Ctrl Pts',(-7.14783907237772,-3.39114717316062,
14.5008529398403));
#217593=CARTESIAN_POINT('Ctrl Pts',(-7.11013207420096,-3.4695107164351,
14.5043147400745));
#217594=CARTESIAN_POINT('Ctrl Pts',(-6.78352051358068,-4.12058540043313,
14.533220115032));
#217595=CARTESIAN_POINT('Ctrl Pts',(-6.4272157762679,-4.65686164785477,
14.5579956243139));
#217596=CARTESIAN_POINT('Ctrl Pts',(-5.84158268048582,-5.34106383559166,
14.5916886329292));
#217597=CARTESIAN_POINT('Ctrl Pts',(-5.66353512370756,-5.52950463140723,
14.6012702853086));
#217598=CARTESIAN_POINT('Ctrl Pts',(-5.39514515349256,-5.78697319181438,
14.6150946386616));
#217599=CARTESIAN_POINT('Ctrl Pts',(-5.31206715749001,-5.86332603058683,
14.6192972339497));
#217600=CARTESIAN_POINT('Ctrl Pts',(-5.08087514394196,-6.06685501192869,
14.6308463942725));
#217601=CARTESIAN_POINT('Ctrl Pts',(-4.92964530888855,-6.19036467326444,
14.6382427404057));
#217602=CARTESIAN_POINT('Ctrl Pts',(-4.72463625103934,-6.34551549907018,
14.6482424482844));
#217603=CARTESIAN_POINT('Ctrl Pts',(-4.67482835626658,-6.38229851091883,
14.6506701163304));
#217604=CARTESIAN_POINT('Ctrl Pts',(-4.60446564743442,-6.43299561740641,
14.6541037678996));
#217605=CARTESIAN_POINT('Ctrl Pts',(-4.58426876575193,-6.44740384804727,
14.6550898334904));
#217606=CARTESIAN_POINT('Ctrl Pts',(-4.55358742627076,-6.46907452462936,
14.6565889659631));
#217607=CARTESIAN_POINT('Ctrl Pts',(-4.5431525378649,-6.47640708026922,
14.6570990356698));
#217608=CARTESIAN_POINT('Ctrl Pts',(-4.52614570638438,-6.48829638645187,
14.6579307558024));
#217609=CARTESIAN_POINT('Ctrl Pts',(-4.51958448315963,-6.49286847648109,
14.6582517307959));
#217610=CARTESIAN_POINT('Ctrl Pts',(-4.50688230306024,-6.50169121735234,
14.6588733313664));
#217611=CARTESIAN_POINT('Ctrl Pts',(-4.50074223523536,-6.50594313769646,
14.6591738995724));
#217612=CARTESIAN_POINT('Ctrl Pts',(-4.49007953178265,-6.51330460840188,
14.6596960387613));
#217613=CARTESIAN_POINT('Ctrl Pts',(-4.48555965819528,-6.51641816308199,
14.6599174270253));
#217614=CARTESIAN_POINT('Ctrl Pts',(-4.47615573060957,-6.52288172144017,
14.6603781645653));
#217615=CARTESIAN_POINT('Ctrl Pts',(-4.47127114907023,-6.52623094808969,
14.6606175494134));
#217616=CARTESIAN_POINT('Ctrl Pts',(-4.45935524150135,-6.53438170942558,
14.6612017058356));
#217617=CARTESIAN_POINT('Ctrl Pts',(-4.45231992534214,-6.53917737762496,
14.6615467510764));
#217618=CARTESIAN_POINT('Ctrl Pts',(-4.425636199398,-6.55730348480021,14.662856069622));
#217619=CARTESIAN_POINT('Ctrl Pts',(-4.40593567894893,-6.57055671441549,
14.6638240112931));
#217620=CARTESIAN_POINT('Ctrl Pts',(-4.1492163636711,-6.74158706222824,
14.6764576097869));
#217621=CARTESIAN_POINT('Ctrl Pts',(-3.90395243243347,-6.88651522203738,
14.688847716405));
#217622=CARTESIAN_POINT('Ctrl Pts',(-3.56053577122835,-7.06519708512882,
14.7062216485793));
#217623=CARTESIAN_POINT('Ctrl Pts',(-3.46870868321951,-7.11073021656714,
14.7108675043172));
#217624=CARTESIAN_POINT('Ctrl Pts',(-3.13091958769764,-7.27012496742601,
14.7279041342482));
#217625=CARTESIAN_POINT('Ctrl Pts',(-2.88003456556343,-7.37311156524941,
14.7404508563278));
#217626=CARTESIAN_POINT('Ctrl Pts',(-2.54472868876093,-7.49102144994287,
14.7567850368745));
#217627=CARTESIAN_POINT('Ctrl Pts',(-2.46465267895177,-7.51774792305902,
14.7606549118307));
#217628=CARTESIAN_POINT('Ctrl Pts',(-2.33620160230442,-7.55834725622247,
14.7668051339396));
#217629=CARTESIAN_POINT('Ctrl Pts',(-2.28809569355128,-7.57304887933787,
14.7690957269753));
#217630=CARTESIAN_POINT('Ctrl Pts',(-2.09890582629606,-7.62889983071797,
14.7780506426993));
#217631=CARTESIAN_POINT('Ctrl Pts',(-1.95682394954797,-7.66657422640383,
14.7846591121127));
#217632=CARTESIAN_POINT('Ctrl Pts',(-1.59098126353183,-7.7527471952586,
14.8013317641483));
#217633=CARTESIAN_POINT('Ctrl Pts',(-1.36600895248158,-7.79553335477924,
14.8112584957362));
#217634=CARTESIAN_POINT('Ctrl Pts',(-0.993698764179286,-7.84972534608339,
14.8271094233152));
#217635=CARTESIAN_POINT('Ctrl Pts',(-0.847342739479785,-7.86686967410458,
14.8331970902977));
#217636=CARTESIAN_POINT('Ctrl Pts',(-0.681702320304589,-7.88159643953867,
14.8399301348295));
#217637=CARTESIAN_POINT('Ctrl Pts',(-0.662810557941004,-7.88320763774275,
14.8406957762589));
#217638=CARTESIAN_POINT('Ctrl Pts',(-0.63446610460771,-7.88552240521146,
14.8418411223026));
#217639=CARTESIAN_POINT('Ctrl Pts',(-0.625017706542182,-7.88627692312939,
14.8422223493299));
#217640=CARTESIAN_POINT('Ctrl Pts',(-0.60878270693865,-7.88754403701043,
14.8428764383968));
#217641=CARTESIAN_POINT('Ctrl Pts',(-0.601996768830469,-7.88806485841931,
14.8431495460385));
#217642=CARTESIAN_POINT('Ctrl Pts',(-0.588036471191368,-7.88911819300989,
14.8437107997456));
#217643=CARTESIAN_POINT('Ctrl Pts',(-0.580862038931829,-7.889649678332,
14.8439989148573));
#217644=CARTESIAN_POINT('Ctrl Pts',(-0.561591662599399,-7.89105080912434,
14.8447719230641));
#217645=CARTESIAN_POINT('Ctrl Pts',(-0.549494406323064,-7.8919024301312,
14.8452562770622));
#217646=CARTESIAN_POINT('Ctrl Pts',(-0.50539440390847,-7.89490508462575,
14.8470186635983));
#217647=CARTESIAN_POINT('Ctrl Pts',(-0.47338042335452,-7.89688931181057,
14.8482917096749));
#217648=CARTESIAN_POINT('Ctrl Pts',(0.0441231675576322,-7.92580589618363,
14.8687700964924));
#217649=CARTESIAN_POINT('Ctrl Pts',(0.531083640545139,-7.90811999269952,
14.8865299364146));
#217650=CARTESIAN_POINT('Ctrl Pts',(1.27672076557734,-7.81181222259129,
14.9129498992756));
#217651=CARTESIAN_POINT('Ctrl Pts',(1.53818401177015,-7.76456167768514,
14.922082101914));
#217652=CARTESIAN_POINT('Ctrl Pts',(1.99430598686077,-7.65818547896182,
14.9382718556132));
#217653=CARTESIAN_POINT('Ctrl Pts',(2.18998775985691,-7.60453891413295,
14.9453058626977));
#217654=CARTESIAN_POINT('Ctrl Pts',(2.57078817304305,-7.48422300014504,
14.9594632038919));
#217655=CARTESIAN_POINT('Ctrl Pts',(2.75591001522079,-7.41805228471244,
14.9665725272052));
#217656=CARTESIAN_POINT('Ctrl Pts',(3.00606832804269,-7.31797725100345,
14.976696363252));
#217657=CARTESIAN_POINT('Ctrl Pts',(3.0733895327388,-7.28995981916303,14.9794735726764));
#217658=CARTESIAN_POINT('Ctrl Pts',(3.18663915665525,-7.24098056157631,
14.9842482637425));
#217659=CARTESIAN_POINT('Ctrl Pts',(3.23277234797359,-7.22050215554365,
14.9862225570641));
#217660=CARTESIAN_POINT('Ctrl Pts',(3.29759265087358,-7.19098285421745,
14.9890416794821));
#217661=CARTESIAN_POINT('Ctrl Pts',(3.31644553315007,-7.18230747782314,
14.9898670654784));
#217662=CARTESIAN_POINT('Ctrl Pts',(3.34506773786834,-7.16899991090405,
14.9911282151428));
#217663=CARTESIAN_POINT('Ctrl Pts',(3.35486223508288,-7.1644216288049,14.9915612199923));
#217664=CARTESIAN_POINT('Ctrl Pts',(3.37079127199088,-7.15693602637745,
14.9922677360995));
#217665=CARTESIAN_POINT('Ctrl Pts',(3.37693153256675,-7.15404085178162,
14.9925406409231));
#217666=CARTESIAN_POINT('Ctrl Pts',(3.38882855512097,-7.14841259540262,
14.9930704809727));
#217667=CARTESIAN_POINT('Ctrl Pts',(3.39458575694009,-7.14568045385069,
14.9933273698755));
#217668=CARTESIAN_POINT('Ctrl Pts',(3.40452756648217,-7.14094773558511,
14.9937718150547));
#217669=CARTESIAN_POINT('Ctrl Pts',(3.40871373362139,-7.13895042673583,
14.9939592130585));
#217670=CARTESIAN_POINT('Ctrl Pts',(3.41737395675531,-7.13480909721746,
14.9943474247741));
#217671=CARTESIAN_POINT('Ctrl Pts',(3.42184775607711,-7.13266454756814,
14.9945482637732));
#217672=CARTESIAN_POINT('Ctrl Pts',(3.43268559855492,-7.12745680209742,
14.9950355019325));
#217673=CARTESIAN_POINT('Ctrl Pts',(3.43904755451075,-7.12438929323911,
14.9953221051187));
#217674=CARTESIAN_POINT('Ctrl Pts',(3.46272973022396,-7.1129314774667,14.9963911443719));
#217675=CARTESIAN_POINT('Ctrl Pts',(3.48002333404723,-7.10448653832251,
14.9971761210625));
#217676=CARTESIAN_POINT('Ctrl Pts',(3.79688969567079,-6.94831748844125,
15.0116362581684));
#217677=CARTESIAN_POINT('Ctrl Pts',(4.08682696422884,-6.78183671496138,
15.0261195463624));
#217678=CARTESIAN_POINT('Ctrl Pts',(4.74915053093661,-6.34360107586198,
15.0609632208406));
#217679=CARTESIAN_POINT('Ctrl Pts',(5.110074959318,-6.05663886299537,15.0813670405938));
#217680=CARTESIAN_POINT('Ctrl Pts',(5.55323229247072,-5.63632807981863,
15.1075152519499));
#217681=CARTESIAN_POINT('Ctrl Pts',(5.65948087184041,-5.52963482973197,
15.1138876136051));
#217682=CARTESIAN_POINT('Ctrl Pts',(5.89212397978899,-5.28228403897193,
15.1280783354445));
#217683=CARTESIAN_POINT('Ctrl Pts',(6.01665189889842,-5.13999548233371,
15.1358445528358));
#217684=CARTESIAN_POINT('Ctrl Pts',(6.15539185589763,-4.96950894769468,
15.1447314757485));
#217685=CARTESIAN_POINT('Ctrl Pts',(6.17467729091905,-4.94552610446243,
15.1459724325339));
#217686=CARTESIAN_POINT('Ctrl Pts',(6.20178913010534,-4.91140474664761,
15.147725285661));
#217687=CARTESIAN_POINT('Ctrl Pts',(6.20973154220032,-4.90135891101773,
15.1482398055005));
#217688=CARTESIAN_POINT('Ctrl Pts',(6.22569404247316,-4.88106791313544,
15.1492759707693));
#217689=CARTESIAN_POINT('Ctrl Pts',(6.23371331941065,-4.87082216219094,
15.1497975970903));
#217690=CARTESIAN_POINT('Ctrl Pts',(6.24904800145695,-4.85113005620534,
15.1507971634151));
#217691=CARTESIAN_POINT('Ctrl Pts',(6.25636735234919,-4.8416868238327,15.1512751886229));
#217692=CARTESIAN_POINT('Ctrl Pts',(6.27351846519045,-4.81945508067404,
15.1523975333499));
#217693=CARTESIAN_POINT('Ctrl Pts',(6.28333256928127,-4.8066529970093,15.1530414731178));
#217694=CARTESIAN_POINT('Ctrl Pts',(6.31734106974931,-4.76200820319867,
15.1552790086126));
#217695=CARTESIAN_POINT('Ctrl Pts',(6.34133325569627,-4.7300119333516,15.1568684242194));
#217696=CARTESIAN_POINT('Ctrl Pts',(6.59392817457237,-4.38777187464092,
15.1737224558768));
#217697=CARTESIAN_POINT('Ctrl Pts',(6.79981909854397,-4.0613932197315,15.188483521749));
#217698=CARTESIAN_POINT('Ctrl Pts',(7.24808073288946,-3.22045898664596,
15.2241405309309));
#217699=CARTESIAN_POINT('Ctrl Pts',(7.46037061939149,-2.6923709677696,15.2444708611561));
#217700=CARTESIAN_POINT('Ctrl Pts',(7.66784334268925,-1.95627512409909,
15.2733511331224));
#217701=CARTESIAN_POINT('Ctrl Pts',(7.71423582310269,-1.7644810656686,15.2809369771586));
#217702=CARTESIAN_POINT('Ctrl Pts',(7.75764765228021,-1.5502513117995,15.2896280626817));
#217703=CARTESIAN_POINT('Ctrl Pts',(7.76180045457719,-1.52932335350084,
15.290479383311));
#217704=CARTESIAN_POINT('Ctrl Pts',(7.76802995338839,-1.49725086403733,
15.2917878356465));
#217705=CARTESIAN_POINT('Ctrl Pts',(7.77016745819575,-1.4861181570062,15.2922427112589));
#217706=CARTESIAN_POINT('Ctrl Pts',(7.77364420962375,-1.46779772411631,
15.2929924650061));
#217707=CARTESIAN_POINT('Ctrl Pts',(7.7749974372309,-1.46061264793973,15.2932868116689));
#217708=CARTESIAN_POINT('Ctrl Pts',(7.77739026520432,-1.44781017356194,
15.29381183258));
#217709=CARTESIAN_POINT('Ctrl Pts',(7.77843374614193,-1.44219350040737,
15.294042356937));
#217710=CARTESIAN_POINT('Ctrl Pts',(7.78043901039287,-1.43133441706998,
15.2944884156002));
#217711=CARTESIAN_POINT('Ctrl Pts',(7.78140158182625,-1.42609215344736,
15.2947039190429));
#217712=CARTESIAN_POINT('Ctrl Pts',(7.78336422694018,-1.41534223608281,
15.2951461838447));
#217713=CARTESIAN_POINT('Ctrl Pts',(7.78436375420205,-1.40983448550887,
15.2953729666738));
#217714=CARTESIAN_POINT('Ctrl Pts',(7.78674145841359,-1.39665287292741,
15.2959161782196));
#217715=CARTESIAN_POINT('Ctrl Pts',(7.78811413658624,-1.3889780352934,15.29623282615));
#217716=CARTESIAN_POINT('Ctrl Pts',(7.79301373355582,-1.36134808000553,
15.29737414253));
#217717=CARTESIAN_POINT('Ctrl Pts',(7.79647530163153,-1.3413815664667,15.2982014584043));
#217718=CARTESIAN_POINT('Ctrl Pts',(7.84291546799194,-1.0672584969498,15.309596987744));
#217719=CARTESIAN_POINT('Ctrl Pts',(7.87351566128646,-0.811215330371204,
15.3207660863788));
#217720=CARTESIAN_POINT('Ctrl Pts',(7.92935416494666,-0.0160561983133679,
15.3564238601709));
#217721=CARTESIAN_POINT('Ctrl Pts',(7.91200567443565,0.524513016241022,
15.3818093515221));
#217722=CARTESIAN_POINT('Ctrl Pts',(7.81310333305847,1.25660080367556,15.4151070653646));
#217723=CARTESIAN_POINT('Ctrl Pts',(7.77897249047789,1.4530046783481,15.4239453393603));
#217724=CARTESIAN_POINT('Ctrl Pts',(7.70306049268923,1.80943378647634,15.4397320284595));
#217725=CARTESIAN_POINT('Ctrl Pts',(7.66361099261169,1.9698381816982,15.4467414340259));
#217726=CARTESIAN_POINT('Ctrl Pts',(7.59496313033157,2.21552389567352,15.4573181082936));
#217727=CARTESIAN_POINT('Ctrl Pts',(7.5692823240326,2.30173345635525,15.460998802241));
#217728=CARTESIAN_POINT('Ctrl Pts',(7.53737181940608,2.40253955129851,15.4652674404652));
#217729=CARTESIAN_POINT('Ctrl Pts',(7.53256224607572,2.41757652462369,15.465903256478));
#217730=CARTESIAN_POINT('Ctrl Pts',(7.52513019238944,2.44057510606064,15.4668743123657));
#217731=CARTESIAN_POINT('Ctrl Pts',(7.52254003104011,2.44854706769303,15.4672106490127));
#217732=CARTESIAN_POINT('Ctrl Pts',(7.5180040542434,2.46243269910159,15.4677960341189));
#217733=CARTESIAN_POINT('Ctrl Pts',(7.51606392170615,2.46834820928785,15.4680452757413));
#217734=CARTESIAN_POINT('Ctrl Pts',(7.51168939453167,2.48163326790347,15.4686047046561));
#217735=CARTESIAN_POINT('Ctrl Pts',(7.50925113202372,2.48900154137041,15.4689147597458));
#217736=CARTESIAN_POINT('Ctrl Pts',(7.50271309900235,2.50866200583322,15.4697414824283));
#217737=CARTESIAN_POINT('Ctrl Pts',(7.49859395594341,2.52094775659288,15.4702574874924));
#217738=CARTESIAN_POINT('Ctrl Pts',(7.48082533053159,2.57351555653326,15.4724627594869));
#217739=CARTESIAN_POINT('Ctrl Pts',(7.46688118240589,2.61369765427672,15.4741419105012));
#217740=CARTESIAN_POINT('Ctrl Pts',(7.24909110562212,3.22532106457252,15.4996049523723));
#217741=CARTESIAN_POINT('Ctrl Pts',(6.98050048350745,3.77156892159659,15.5208431908311));
#217742=CARTESIAN_POINT('Ctrl Pts',(6.42534607497203,4.63404020483107,15.5554990138076));
#217743=CARTESIAN_POINT('Ctrl Pts',(6.17100647544183,4.96770107539512,15.5693129568213));
#217744=CARTESIAN_POINT('Ctrl Pts',(5.77644295054215,5.40798752966261,15.5900967330713));
#217745=CARTESIAN_POINT('Ctrl Pts',(5.65726780721133,5.53253450743778,15.5963088547547));
#217746=CARTESIAN_POINT('Ctrl Pts',(5.47009263877204,5.71577093920366,15.6061399436221));
#217747=CARTESIAN_POINT('Ctrl Pts',(5.40500041976233,5.77736274836877,15.6095717231991));
#217748=CARTESIAN_POINT('Ctrl Pts',(5.30605143347067,5.86785463765291,15.6148316812426));
#217749=CARTESIAN_POINT('Ctrl Pts',(5.27297264923195,5.89759774427823,15.6165970970495));
#217750=CARTESIAN_POINT('Ctrl Pts',(5.23341999206203,5.93256312482076,15.6187186238196));
#217751=CARTESIAN_POINT('Ctrl Pts',(5.22718592842097,5.93805669491063,15.6190533160584));
#217752=CARTESIAN_POINT('Ctrl Pts',(5.21758360611871,5.94649159671674,15.6195693371526));
#217753=CARTESIAN_POINT('Ctrl Pts',(5.2142214726166,5.949439925825,15.6197501085775));
#217754=CARTESIAN_POINT('Ctrl Pts',(5.20809330059185,5.9548046703826,15.6200797743035));
#217755=CARTESIAN_POINT('Ctrl Pts',(5.20532807369477,5.95722201493172,15.6202285940524));
#217756=CARTESIAN_POINT('Ctrl Pts',(5.19973089346847,5.96210816326705,15.6205299563838));
#217757=CARTESIAN_POINT('Ctrl Pts',(5.19689886287909,5.96457687718906,15.6206825061414));
#217758=CARTESIAN_POINT('Ctrl Pts',(5.18874628218923,5.97167336210418,15.6211218511035));
#217759=CARTESIAN_POINT('Ctrl Pts',(5.18342131667848,5.97629602493524,15.6214090590183));
#217760=CARTESIAN_POINT('Ctrl Pts',(5.1597443012597,5.99679486036049,15.6226871549473));
#217761=CARTESIAN_POINT('Ctrl Pts',(5.14132562358707,6.01259350511214,15.6236841994389));
#217762=CARTESIAN_POINT('Ctrl Pts',(4.84418429220112,6.26510319729904,15.639809123811));
#217763=CARTESIAN_POINT('Ctrl Pts',(4.54947520658831,6.48227297364153,15.6563479640861));
#217764=CARTESIAN_POINT('Ctrl Pts',(3.80204896278301,6.95690486373847,15.6973266159132));
#217765=CARTESIAN_POINT('Ctrl Pts',(3.33681832060663,7.19164918488398,15.721982862257));
#217766=CARTESIAN_POINT('Ctrl Pts',(2.49373938090724,7.51748878293906,15.762540644776));
#217767=CARTESIAN_POINT('Ctrl Pts',(2.1259339179929,7.6296682377762,15.7790206789024));
#217768=CARTESIAN_POINT('Ctrl Pts',(1.73093870865515,7.71934013293631,15.7953853349192));
#217769=CARTESIAN_POINT('Ctrl Pts',(1.71046684005026,7.72390212908402,15.7962299024903));
#217770=CARTESIAN_POINT('Ctrl Pts',(1.68100955061902,7.73034359846533,15.7974400597501));
#217771=CARTESIAN_POINT('Ctrl Pts',(1.67203871523932,7.73228891048045,15.7978079180774));
#217772=CARTESIAN_POINT('Ctrl Pts',(1.65646525765424,7.73563762166319,15.7984453498401));
#217773=CARTESIAN_POINT('Ctrl Pts',(1.64986419762829,7.73704818992347,15.7987151698813));
#217774=CARTESIAN_POINT('Ctrl Pts',(1.63716982817361,7.73974384158282,15.7992333548886));
#217775=CARTESIAN_POINT('Ctrl Pts',(1.63107679318099,7.74103018173803,15.7994817628994));
#217776=CARTESIAN_POINT('Ctrl Pts',(1.61672289272429,7.7440428272254,15.8000662315986));
#217777=CARTESIAN_POINT('Ctrl Pts',(1.60846076273674,7.74576311263946,15.8004020852574));
#217778=CARTESIAN_POINT('Ctrl Pts',(1.57990902781709,7.75166031101287,15.8015607548397));
#217779=CARTESIAN_POINT('Ctrl Pts',(1.55960569444343,7.75577076764853,15.8023812895051));
#217780=CARTESIAN_POINT('Ctrl Pts',(1.33140725767735,7.80103774250884,15.8115658896232));
#217781=CARTESIAN_POINT('Ctrl Pts',(1.12194745549349,7.83390564206428,15.8196409511701));
#217782=CARTESIAN_POINT('Ctrl Pts',(0.697165307759898,7.88317190650409,
15.8354368125971));
#217783=CARTESIAN_POINT('Ctrl Pts',(0.481989061022481,7.89924880160957,
15.8431420523301));
#217784=CARTESIAN_POINT('Ctrl Pts',(-0.22293209331493,7.92300174743003,
15.8677952867758));
#217785=CARTESIAN_POINT('Ctrl Pts',(-0.712731552397718,7.89402586215829,
15.8839332829613));
#217786=CARTESIAN_POINT('Ctrl Pts',(-1.47347829990967,7.77760783059701,
15.910780307215));
#217787=CARTESIAN_POINT('Ctrl Pts',(-1.74779483160068,7.72059012346852,
15.9208573336582));
#217788=CARTESIAN_POINT('Ctrl Pts',(-2.0813502115402,7.63257027744579,15.9342350781325));
#217789=CARTESIAN_POINT('Ctrl Pts',(-2.1440032104375,7.61520830425879,15.936797960387));
#217790=CARTESIAN_POINT('Ctrl Pts',(-2.21531496627557,7.5944970957119,15.9397801197608));
#217791=CARTESIAN_POINT('Ctrl Pts',(-2.22419192706759,7.59190205450382,
15.9401525038197));
#217792=CARTESIAN_POINT('Ctrl Pts',(-2.2376779540179,7.58793394166489,15.9407199868228));
#217793=CARTESIAN_POINT('Ctrl Pts',(-2.24229039053542,7.58657221235515,
15.9409143863981));
#217794=CARTESIAN_POINT('Ctrl Pts',(-2.25028725570714,7.58420336854743,
15.9412519654746));
#217795=CARTESIAN_POINT('Ctrl Pts',(-2.25367226177303,7.5831981910749,15.9413950267111));
#217796=CARTESIAN_POINT('Ctrl Pts',(-2.26070450327306,7.58110484265696,
15.9416925769256));
#217797=CARTESIAN_POINT('Ctrl Pts',(-2.2643516277544,7.58001630554069,15.9418470880913));
#217798=CARTESIAN_POINT('Ctrl Pts',(-2.27431983246404,7.57703331421637,
15.9422699180735));
#217799=CARTESIAN_POINT('Ctrl Pts',(-2.28063931794703,7.57513358601745,
15.9425385545351));
#217800=CARTESIAN_POINT('Ctrl Pts',(-2.30468803971605,7.56787137325946,
15.9435630262013));
#217801=CARTESIAN_POINT('Ctrl Pts',(-2.32240067627104,7.56245457311464,
15.9443220930826));
#217802=CARTESIAN_POINT('Ctrl Pts',(-2.63231164295717,7.4664875062857,15.9576802792473));
#217803=CARTESIAN_POINT('Ctrl Pts',(-2.91900929989047,7.35913379099867,
15.971234298508));
#217804=CARTESIAN_POINT('Ctrl Pts',(-3.84836935432984,6.94827102071024,
16.0176047654335));
#217805=CARTESIAN_POINT('Ctrl Pts',(-4.45647569220624,6.57483498169648,
16.0516697229704));
#217806=CARTESIAN_POINT('Ctrl Pts',(-5.17696207090427,5.9859362614302,16.0926696676948));
#217807=CARTESIAN_POINT('Ctrl Pts',(-5.34150562403159,5.83958021296413,
16.1021181678034));
#217808=CARTESIAN_POINT('Ctrl Pts',(-5.5736475534076,5.61506416284713,16.115563637908));
#217809=CARTESIAN_POINT('Ctrl Pts',(-5.64615601095024,5.54214903764875,
16.1197817764979));
#217810=CARTESIAN_POINT('Ctrl Pts',(-5.72889932244715,5.45563184961359,
16.1246203158833));
#217811=CARTESIAN_POINT('Ctrl Pts',(-5.74053517558061,5.44338701800336,
16.1253013359021));
#217812=CARTESIAN_POINT('Ctrl Pts',(-5.75820091399726,5.4246770766829,16.1263362088741));
#217813=CARTESIAN_POINT('Ctrl Pts',(-5.76425929329439,5.41823900843915,
16.1266912826983));
#217814=CARTESIAN_POINT('Ctrl Pts',(-5.77523485326303,5.40653634813208,
16.1273348585507));
#217815=CARTESIAN_POINT('Ctrl Pts',(-5.78015565456969,5.40127517381916,
16.127623514948));
#217816=CARTESIAN_POINT('Ctrl Pts',(-5.78999005917396,5.39073169065454,
16.1282006380164));
#217817=CARTESIAN_POINT('Ctrl Pts',(-5.79490363677673,5.38544936721038,
16.1284891035195));
#217818=CARTESIAN_POINT('Ctrl Pts',(-5.80873863779206,5.37053524340787,
16.1293016603914));
#217819=CARTESIAN_POINT('Ctrl Pts',(-5.8176433387451,5.36088792534746,16.1298250437338));
#217820=CARTESIAN_POINT('Ctrl Pts',(-5.85435966784315,5.32091038100809,
16.1319847542219));
#217821=CARTESIAN_POINT('Ctrl Pts',(-5.88195867339734,5.29038530087749,
16.1336121420364));
#217822=CARTESIAN_POINT('Ctrl Pts',(-6.33282587472184,4.7838268908701,16.1602693941614));
#217823=CARTESIAN_POINT('Ctrl Pts',(-6.6973134961961,4.25860960472822,16.1826227163787));
#217824=CARTESIAN_POINT('Ctrl Pts',(-7.16693673194111,3.36965827644062,
16.2174630859276));
#217825=CARTESIAN_POINT('Ctrl Pts',(-7.31602226416854,3.03238776846265,
16.2301529459766));
#217826=CARTESIAN_POINT('Ctrl Pts',(-7.51222838259756,2.48883037003805,
16.2512651639963));
#217827=CARTESIAN_POINT('Ctrl Pts',(-7.57552572331831,2.28894341957907,
16.2591846793608));
#217828=CARTESIAN_POINT('Ctrl Pts',(-7.6374228804733,2.06260044129216,16.268466281304));
#217829=CARTESIAN_POINT('Ctrl Pts',(-7.64391743189899,2.03840013547349,
16.2694619393055));
#217830=CARTESIAN_POINT('Ctrl Pts',(-7.655237853753,1.99540247054524,16.2712363700641));
#217831=CARTESIAN_POINT('Ctrl Pts',(-7.66010975199435,1.97661736221219,
16.2720134202061));
#217832=CARTESIAN_POINT('Ctrl Pts',(-7.66713534470493,1.94911192190456,
16.2731537021131));
#217833=CARTESIAN_POINT('Ctrl Pts',(-7.66934340716722,1.94040546802124,
16.2735150097861));
#217834=CARTESIAN_POINT('Ctrl Pts',(-7.67319969644353,1.92509059690481,
16.2741511872963));
#217835=CARTESIAN_POINT('Ctrl Pts',(-7.67485422805534,1.91848376735113,
16.2744258393873));
#217836=CARTESIAN_POINT('Ctrl Pts',(-7.67805613474756,1.90562757134092,
16.2749606741889));
#217837=CARTESIAN_POINT('Ctrl Pts',(-7.67960441740908,1.89937843538817,
16.2752208259352));
#217838=CARTESIAN_POINT('Ctrl Pts',(-7.68329221046285,1.88441564259427,
16.2758441478943));
#217839=CARTESIAN_POINT('Ctrl Pts',(-7.68542452632376,1.87570023055054,
16.2762075566575));
#217840=CARTESIAN_POINT('Ctrl Pts',(-7.69186412951485,1.84918431316404,
16.2773142037854));
#217841=CARTESIAN_POINT('Ctrl Pts',(-7.69612442105751,1.83137251829451,
16.2780589603471));
#217842=CARTESIAN_POINT('Ctrl Pts',(-7.7460963144361,1.61919169996095,16.2869461670382));
#217843=CARTESIAN_POINT('Ctrl Pts',(-7.78449384303411,1.42317964181873,
16.2953075273668));
#217844=CARTESIAN_POINT('Ctrl Pts',(-7.87892463966614,0.821174561950701,
16.3211556837578));
#217845=CARTESIAN_POINT('Ctrl Pts',(-7.91087598531184,0.412096929851135,
16.3389141450628));
#217846=CARTESIAN_POINT('Ctrl Pts',(-7.91122481811769,-0.743705493900177,
16.3884127477905));
#217847=CARTESIAN_POINT('Ctrl Pts',(-7.80590345515495,-1.48610707923397,
16.4193039870618));
#217848=CARTESIAN_POINT('Ctrl Pts',(-7.57736574926858,-2.27442753535988,
16.4526704896892));
#217849=CARTESIAN_POINT('Ctrl Pts',(-7.55556898687502,-2.34581962696523,
16.4556948906204));
#217850=CARTESIAN_POINT('Ctrl Pts',(-7.52445344597799,-2.44279788095363,
16.459806860129));
#217851=CARTESIAN_POINT('Ctrl Pts',(-7.51600824186062,-2.46865981103749,
16.4609037928098));
#217852=CARTESIAN_POINT('Ctrl Pts',(-7.50136310499068,-2.51273610639126,
16.4627739369616));
#217853=CARTESIAN_POINT('Ctrl Pts',(-7.49522983234375,-2.53097233014358,
16.4635478854462));
#217854=CARTESIAN_POINT('Ctrl Pts',(-7.482531161884,-2.56827864051784,16.465131581671));
#217855=CARTESIAN_POINT('Ctrl Pts',(-7.47595924021528,-2.58734636360536,
16.4659412488633));
#217856=CARTESIAN_POINT('Ctrl Pts',(-7.46061969837214,-2.63130598417239,
16.4678084326599));
#217857=CARTESIAN_POINT('Ctrl Pts',(-7.45180028644896,-2.65617958035703,
16.4688653381997));
#217858=CARTESIAN_POINT('Ctrl Pts',(-7.42360445770979,-2.73445516146129,
16.4721927296461));
#217859=CARTESIAN_POINT('Ctrl Pts',(-7.40377713792021,-2.7876930118315,
16.4744578189848));
#217860=CARTESIAN_POINT('Ctrl Pts',(-7.21371737448243,-3.28168276449015,
16.4954988710632));
#217861=CARTESIAN_POINT('Ctrl Pts',(-7.00489181316891,-3.70657094219149,
16.5137046890007));
#217862=CARTESIAN_POINT('Ctrl Pts',(-6.66297360762328,-4.2688575725084,
16.5389885353465));
#217863=CARTESIAN_POINT('Ctrl Pts',(-6.56100128272182,-4.42398277906825,
16.5461116421576));
#217864=CARTESIAN_POINT('Ctrl Pts',(-6.32360704237753,-4.7588325223663,
16.5619922547787));
#217865=CARTESIAN_POINT('Ctrl Pts',(-6.1857848884082,-4.93665401812913,
16.5707686658607));
#217866=CARTESIAN_POINT('Ctrl Pts',(-6.0246139863263,-5.12723694194316,
16.5807519238626));
#217867=CARTESIAN_POINT('Ctrl Pts',(-6.00855975003395,-5.14604139796238,
16.5817434987504));
#217868=CARTESIAN_POINT('Ctrl Pts',(-5.9843328493046,-5.1741506262578,16.583235894038));
#217869=CARTESIAN_POINT('Ctrl Pts',(-5.97622607926751,-5.18351195644496,
16.5837346077011));
#217870=CARTESIAN_POINT('Ctrl Pts',(-5.96145852556676,-5.2004841638832,
16.5846418345552));
#217871=CARTESIAN_POINT('Ctrl Pts',(-5.95480505686396,-5.20810138389114,
16.5850501261238));
#217872=CARTESIAN_POINT('Ctrl Pts',(-5.94044435150669,-5.22447873455879,
16.5859303723319));
#217873=CARTESIAN_POINT('Ctrl Pts',(-5.93273230772726,-5.23323461207253,
16.5864024680483));
#217874=CARTESIAN_POINT('Ctrl Pts',(-5.91153828586117,-5.25719020862571,
16.5876981383882));
#217875=CARTESIAN_POINT('Ctrl Pts',(-5.89801710776141,-5.27235507018253,
16.5885228302435));
#217876=CARTESIAN_POINT('Ctrl Pts',(-5.82583403600294,-5.35268781529885,
16.5929149493199));
#217877=CARTESIAN_POINT('Ctrl Pts',(-5.76615077945662,-5.41692845538449,
16.5965097636945));
#217878=CARTESIAN_POINT('Ctrl Pts',(-5.429971643884,-5.76692548361496,16.6165261898275));
#217879=CARTESIAN_POINT('Ctrl Pts',(-5.13330539865589,-6.03251126805825,
16.6333168935519));
#217880=CARTESIAN_POINT('Ctrl Pts',(-4.55191783805583,-6.47892374906174,
16.6640542837353));
#217881=CARTESIAN_POINT('Ctrl Pts',(-4.27317332956748,-6.66606394778776,
16.6780083589665));
#217882=CARTESIAN_POINT('Ctrl Pts',(-3.87686666090794,-6.89703028231194,
16.6967917186288));
#217883=CARTESIAN_POINT('Ctrl Pts',(-3.76890742286182,-6.95661262827356,
16.7018100248811));
#217884=CARTESIAN_POINT('Ctrl Pts',(-3.62296231759696,-7.03276422915456,
16.7084709861178));
#217885=CARTESIAN_POINT('Ctrl Pts',(-3.58617656520798,-7.05159317622081,
16.7101396966647));
#217886=CARTESIAN_POINT('Ctrl Pts',(-3.5281740140914,-7.08071076897187,
16.7127553417805));
#217887=CARTESIAN_POINT('Ctrl Pts',(-3.50705595473638,-7.09119421549831,
16.7137044643006));
#217888=CARTESIAN_POINT('Ctrl Pts',(-3.46628106917132,-7.1112090230155,
16.7155309870954));
#217889=CARTESIAN_POINT('Ctrl Pts',(-3.44663101121033,-7.12075367466183,
16.71640852752));
#217890=CARTESIAN_POINT('Ctrl Pts',(-3.40000197813141,-7.14316463058394,
16.7184846639398));
#217891=CARTESIAN_POINT('Ctrl Pts',(-3.37298909631384,-7.15595968091379,
16.7196824751856));
#217892=CARTESIAN_POINT('Ctrl Pts',(-3.29255097656199,-7.19350372005637,
16.7232350890006));
#217893=CARTESIAN_POINT('Ctrl Pts',(-3.23892110823703,-7.21780976571606,
16.7255851924293));
#217894=CARTESIAN_POINT('Ctrl Pts',(-2.8741555315789,-7.37824406385046,
16.7414526427757));
#217895=CARTESIAN_POINT('Ctrl Pts',(-2.55479248996414,-7.49481831616603,
16.7548217308199));
#217896=CARTESIAN_POINT('Ctrl Pts',(-1.78270437262863,-7.72153931382124,
16.7860242710609));
#217897=CARTESIAN_POINT('Ctrl Pts',(-1.32579321320553,-7.81296982832797,
16.8034911819049));
#217898=CARTESIAN_POINT('Ctrl Pts',(-0.479143300877044,-7.90593724794838,
16.8351401251896));
#217899=CARTESIAN_POINT('Ctrl Pts',(-0.0922365345026519,-7.91990494120669,
16.8493601012997));
#217900=CARTESIAN_POINT('Ctrl Pts',(0.299619445892115,-7.90532601685582,
16.8643922488431));
#217901=CARTESIAN_POINT('Ctrl Pts',(0.305114962567271,-7.90511581853389,
16.8646031977026));
#217902=CARTESIAN_POINT('Ctrl Pts',(0.328325148613027,-7.90420381182826,
16.8654947105307));
#217903=CARTESIAN_POINT('Ctrl Pts',(0.346037604667464,-7.90344818889555,
16.8661764685522));
#217904=CARTESIAN_POINT('Ctrl Pts',(0.391746202730702,-7.90134428506339,
16.8679397301249));
#217905=CARTESIAN_POINT('Ctrl Pts',(0.419737900728484,-7.89990675116246,
16.869023341465));
#217906=CARTESIAN_POINT('Ctrl Pts',(0.54744049651709,-7.89266784992797,
16.8739862156299));
#217907=CARTESIAN_POINT('Ctrl Pts',(0.647041611770897,-7.88512733702743,
16.8779105055205));
#217908=CARTESIAN_POINT('Ctrl Pts',(0.762125053221456,-7.87421955888687,
16.8825299855726));
#217909=CARTESIAN_POINT('Ctrl Pts',(0.777774819086329,-7.87268915840396,
16.8831600017052));
#217910=CARTESIAN_POINT('Ctrl Pts',(0.801244543784525,-7.87032337512253,
16.8841076961318));
#217911=CARTESIAN_POINT('Ctrl Pts',(0.809068039735018,-7.86952296867311,
16.8844240830014));
#217912=CARTESIAN_POINT('Ctrl Pts',(0.82296900940171,-7.86807983934883,
16.8849871151419));
#217913=CARTESIAN_POINT('Ctrl Pts',(0.829046963173051,-7.86744173676509,
16.8852335862202));
#217914=CARTESIAN_POINT('Ctrl Pts',(0.841808454551067,-7.86608700111764,
16.8857517159136));
#217915=CARTESIAN_POINT('Ctrl Pts',(0.848491828173234,-7.86536889156965,
16.8860234308248));
#217916=CARTESIAN_POINT('Ctrl Pts',(0.866028876139057,-7.86346197303484,
16.886737375529));
#217917=CARTESIAN_POINT('Ctrl Pts',(0.876880996434796,-7.86225921298665,
16.8871801476474));
#217918=CARTESIAN_POINT('Ctrl Pts',(0.924883247016807,-7.85683841660979,
16.889143102701));
#217919=CARTESIAN_POINT('Ctrl Pts',(0.962005287176125,-7.85237955560534,
16.8906728980387));
#217920=CARTESIAN_POINT('Ctrl Pts',(1.22096365756672,-7.81941128320379,
16.9014346404006));
#217921=CARTESIAN_POINT('Ctrl Pts',(1.44150350079323,-7.78177267628682,
16.9111032630698));
#217922=CARTESIAN_POINT('Ctrl Pts',(1.91642753726304,-7.67984005746852,
16.932694518889));
#217923=CARTESIAN_POINT('Ctrl Pts',(2.16982890755309,-7.61212659798136,
16.9446948969209));
#217924=CARTESIAN_POINT('Ctrl Pts',(2.98366944528276,-7.35070748181602,
16.9840364504983));
#217925=CARTESIAN_POINT('Ctrl Pts',(3.52585681112428,-7.10659258770302,
17.0113709298823));
#217926=CARTESIAN_POINT('Ctrl Pts',(4.22060749972608,-6.69452057109854,
17.0460336058856));
#217927=CARTESIAN_POINT('Ctrl Pts',(4.40096281659593,-6.57736031714092,
17.0550151134507));
#217928=CARTESIAN_POINT('Ctrl Pts',(4.59335558223891,-6.44091927325026,
17.064582227223));
#217929=CARTESIAN_POINT('Ctrl Pts',(4.61033208552855,-6.42877862885907,
17.0654263272162));
#217930=CARTESIAN_POINT('Ctrl Pts',(4.63546481340481,-6.41065435669106,
17.066675870371));
#217931=CARTESIAN_POINT('Ctrl Pts',(4.64365786261525,-6.40472208399058,
17.0670831950191));
#217932=CARTESIAN_POINT('Ctrl Pts',(4.65766222512379,-6.39454106398617,
17.0677794130459));
#217933=CARTESIAN_POINT('Ctrl Pts',(4.66347914934097,-6.39030007483029,
17.0680685914856));
#217934=CARTESIAN_POINT('Ctrl Pts',(4.67527099950436,-6.38167822539996,
17.0686547928282));
#217935=CARTESIAN_POINT('Ctrl Pts',(4.68124557704735,-6.37729689908686,
17.06895179811));
#217936=CARTESIAN_POINT('Ctrl Pts',(4.69494013283534,-6.36722468058036,
17.0696325658985));
#217937=CARTESIAN_POINT('Ctrl Pts',(4.70265594125082,-6.36152812482307,
17.0700161183778));
#217938=CARTESIAN_POINT('Ctrl Pts',(4.71880916420298,-6.34955680607217,
17.0708190865432));
#217939=CARTESIAN_POINT('Ctrl Pts',(4.72724446956772,-6.34327922195496,
17.0712383966277));
#217940=CARTESIAN_POINT('Ctrl Pts',(4.74947858396878,-6.32666353319766,
17.0723436303306));
#217941=CARTESIAN_POINT('Ctrl Pts',(4.76325618685626,-6.31629707857646,
17.0730284993763));
#217942=CARTESIAN_POINT('Ctrl Pts',(4.80440400848555,-6.28512570168122,
17.0750739696588));
#217943=CARTESIAN_POINT('Ctrl Pts',(4.8316727570022,-6.26418720727239,17.0764295835561));
#217944=CARTESIAN_POINT('Ctrl Pts',(5.13399232002024,-6.02890051874563,
17.0914616902129));
#217945=CARTESIAN_POINT('Ctrl Pts',(5.39472961595636,-5.79676114851014,
17.10443041916));
#217946=CARTESIAN_POINT('Ctrl Pts',(5.92997317058396,-5.25272328977008,
17.1318029862695));
#217947=CARTESIAN_POINT('Ctrl Pts',(6.19697061040851,-4.93490084494681,
17.1459677397571));
#217948=CARTESIAN_POINT('Ctrl Pts',(6.72055578030378,-4.2017496353388,17.177168162694));
#217949=CARTESIAN_POINT('Ctrl Pts',(6.96613100122361,-3.78067411618811,
17.1942237944322));
#217950=CARTESIAN_POINT('Ctrl Pts',(7.18488433895395,-3.31094684236518,
17.2147237232296));
#217951=CARTESIAN_POINT('Ctrl Pts',(7.1981332490866,-3.28204351145843,17.2159909447991));
#217952=CARTESIAN_POINT('Ctrl Pts',(7.21517264154306,-3.24427152714235,
17.2176538161701));
#217953=CARTESIAN_POINT('Ctrl Pts',(7.21912186127115,-3.23547423726308,
17.2180415868109));
#217954=CARTESIAN_POINT('Ctrl Pts',(7.22517070706325,-3.22193360599626,
17.2186391480001));
#217955=CARTESIAN_POINT('Ctrl Pts',(7.22728177850907,-3.21719536265559,
17.218848385048));
#217956=CARTESIAN_POINT('Ctrl Pts',(7.23125601214119,-3.20825164914942,
17.21924357984));
#217957=CARTESIAN_POINT('Ctrl Pts',(7.2331201706971,-3.20404662162282,17.2194294900012));
#217958=CARTESIAN_POINT('Ctrl Pts',(7.2373928035448,-3.19438600851786,17.2198568319446));
#217959=CARTESIAN_POINT('Ctrl Pts',(7.23979877639917,-3.18892932520966,
17.2200983812559));
#217960=CARTESIAN_POINT('Ctrl Pts',(7.24643837090136,-3.17382465553584,
17.2207674753057));
#217961=CARTESIAN_POINT('Ctrl Pts',(7.25065888258752,-3.16417094579374,
17.2211956263255));
#217962=CARTESIAN_POINT('Ctrl Pts',(7.27350018835718,-3.11163963760719,
17.2235281450474));
#217963=CARTESIAN_POINT('Ctrl Pts',(7.29175969894736,-3.06860662094485,
17.2254487014873));
#217964=CARTESIAN_POINT('Ctrl Pts',(7.57347273159961,-2.38796614461766,
17.2559511480148));
#217965=CARTESIAN_POINT('Ctrl Pts',(7.75279829534976,-1.71873934032661,
17.2873092424353));
#217966=CARTESIAN_POINT('Ctrl Pts',(7.89553649078866,-0.636803331712192,
17.3344857316866));
#217967=CARTESIAN_POINT('Ctrl Pts',(7.91767744205785,-0.235450646987964,
17.3513312488676));
#217968=CARTESIAN_POINT('Ctrl Pts',(7.9084831315777,0.202956362386627,17.3690919653084));
#217969=CARTESIAN_POINT('Ctrl Pts',(7.90744464334923,0.240033264658368,
17.3705894331964));
#217970=CARTESIAN_POINT('Ctrl Pts',(7.9055463365649,0.294194932724599,17.3727706581365));
#217971=CARTESIAN_POINT('Ctrl Pts',(7.90489180339208,0.311286230616918,
17.3734580557675));
#217972=CARTESIAN_POINT('Ctrl Pts',(7.90364830890303,0.341217855308203,
17.3746603411717));
#217973=CARTESIAN_POINT('Ctrl Pts',(7.90308347224003,0.354059101752278,
17.3751756484989));
#217974=CARTESIAN_POINT('Ctrl Pts',(7.90185818923262,0.380449975351676,
17.3762336993426));
#217975=CARTESIAN_POINT('Ctrl Pts',(7.90119418207741,0.393999397063265,
17.3767763797474));
#217976=CARTESIAN_POINT('Ctrl Pts',(7.89943473111563,0.428107197611385,
17.3781411559915));
#217977=CARTESIAN_POINT('Ctrl Pts',(7.89829388006276,0.448663161362323,
17.3789624785136));
#217978=CARTESIAN_POINT('Ctrl Pts',(7.89364320146484,0.526935994223997,
17.3820855982453));
#217979=CARTESIAN_POINT('Ctrl Pts',(7.88958081721388,0.584618826696907,
17.3843784221275));
#217980=CARTESIAN_POINT('Ctrl Pts',(7.83701258015053,1.22999547795197,17.4099390275444));
#217981=CARTESIAN_POINT('Ctrl Pts',(7.72357520639323,1.8105501972467,17.4318915575522));
#217982=CARTESIAN_POINT('Ctrl Pts',(7.42953922400908,2.74560134478082,17.4679417549818));
#217983=CARTESIAN_POINT('Ctrl Pts',(7.28499846947608,3.10888346147995,17.4821866086519));
#217984=CARTESIAN_POINT('Ctrl Pts',(7.04644150997162,3.59939031107713,17.5030062044131));
#217985=CARTESIAN_POINT('Ctrl Pts',(6.9745661320557,3.73675963987432,17.5090255027129));
#217986=CARTESIAN_POINT('Ctrl Pts',(6.88668389597182,3.89334164130696,17.5161861656357));
#217987=CARTESIAN_POINT('Ctrl Pts',(6.87456351411343,3.91470314238978,17.5171696564554));
#217988=CARTESIAN_POINT('Ctrl Pts',(6.85813575004615,3.94334459217472,17.5184975953473));
#217989=CARTESIAN_POINT('Ctrl Pts',(6.85391580880677,3.95067470488548,17.5188382709899));
#217990=CARTESIAN_POINT('Ctrl Pts',(6.84679248991659,3.96300227153346,17.5194126108909));
#217991=CARTESIAN_POINT('Ctrl Pts',(6.84389537152192,3.96800334520582,17.5196459995112));
#217992=CARTESIAN_POINT('Ctrl Pts',(6.83834117374544,3.97756695333956,17.5200930632562));
#217993=CARTESIAN_POINT('Ctrl Pts',(6.83568500140166,3.98213001272897,17.5203066978421));
#217994=CARTESIAN_POINT('Ctrl Pts',(6.82946160269699,3.99279666352969,17.520806866718));
#217995=CARTESIAN_POINT('Ctrl Pts',(6.82589076238279,3.99889813305984,17.5210935642522));
#217996=CARTESIAN_POINT('Ctrl Pts',(6.81563160724507,4.0163740995185,17.5219164532698));
#217997=CARTESIAN_POINT('Ctrl Pts',(6.80892302612491,4.02773662674448,17.5224535756714));
#217998=CARTESIAN_POINT('Ctrl Pts',(6.76523935690617,4.10130394393699,17.5259450988667));
#217999=CARTESIAN_POINT('Ctrl Pts',(6.72744154484847,4.16301421287914,17.5289384189671));
#218000=CARTESIAN_POINT('Ctrl Pts',(6.6147590512869,4.34144132807819,17.5378040425662));
#218001=CARTESIAN_POINT('Ctrl Pts',(6.53764835196612,4.45671406129018,17.5438005936128));
#218002=CARTESIAN_POINT('Ctrl Pts',(6.38079462798303,4.67835837220955,17.5557737039828));
#218003=CARTESIAN_POINT('Ctrl Pts',(6.30131830144144,4.78486811140937,17.5617388441873));
#218004=CARTESIAN_POINT('Ctrl Pts',(6.16331763153661,4.96040444154811,17.5718674407996));
#218005=CARTESIAN_POINT('Ctrl Pts',(6.10622152199834,5.03052232104846,17.5759969880647));
#218006=CARTESIAN_POINT('Ctrl Pts',(5.99692643556687,5.16014109508985,17.5837693013283));
#218007=CARTESIAN_POINT('Ctrl Pts',(5.945011512419,5.21986789194586,17.5874080889248));
#218008=CARTESIAN_POINT('Ctrl Pts',(5.60126735627597,5.60355556308885,17.6111186084839));
#218009=CARTESIAN_POINT('Ctrl Pts',(5.28395479734401,5.90371929368651,17.6311947158881));
#218010=CARTESIAN_POINT('Ctrl Pts',(4.70845083775999,6.36435864889453,17.6635551836821));
#218011=CARTESIAN_POINT('Ctrl Pts',(4.46283140566761,6.53893972216612,17.6763151063948));
#218012=CARTESIAN_POINT('Ctrl Pts',(4.18814210735458,6.711477303161,17.6894589220539));
#218013=CARTESIAN_POINT('Ctrl Pts',(4.16839304281629,6.72376095316463,17.69039798765));
#218014=CARTESIAN_POINT('Ctrl Pts',(4.14085334878118,6.74072229835736,17.6916993178132));
#218015=CARTESIAN_POINT('Ctrl Pts',(4.13310849644529,6.74547386897397,17.6920643893391));
#218016=CARTESIAN_POINT('Ctrl Pts',(4.11974958857148,6.75363809295936,17.6926925546024));
#218017=CARTESIAN_POINT('Ctrl Pts',(4.11413944430297,6.75705711063139,17.6929558898508));
#218018=CARTESIAN_POINT('Ctrl Pts',(4.10266703726978,6.76402921131861,17.6934934443249));
#218019=CARTESIAN_POINT('Ctrl Pts',(4.09680440141934,6.76758167199382,17.693767639835));
#218020=CARTESIAN_POINT('Ctrl Pts',(4.08321038898621,6.77579481796083,17.6944022626615));
#218021=CARTESIAN_POINT('Ctrl Pts',(4.07547563025945,6.78044990275075,17.6947624776017));
#218022=CARTESIAN_POINT('Ctrl Pts',(4.05919965605398,6.79020751816177,17.695518632824));
#218023=CARTESIAN_POINT('Ctrl Pts',(4.05065674522095,6.79530719841064,17.6959144650043));
#218024=CARTESIAN_POINT('Ctrl Pts',(4.02791270393648,6.80882609583634,17.6969654992531));
#218025=CARTESIAN_POINT('Ctrl Pts',(4.0136947656629,6.81721701916115,17.6976196330092));
#218026=CARTESIAN_POINT('Ctrl Pts',(3.97067786158824,6.84242284802061,17.6995900501004));
#218027=CARTESIAN_POINT('Ctrl Pts',(3.941798574629,6.85910031595811,17.7009011647227));
#218028=CARTESIAN_POINT('Ctrl Pts',(3.8384166002455,6.91793369623867,17.7055535399807));
#218029=CARTESIAN_POINT('Ctrl Pts',(3.7633350893431,6.95906302673103,17.7088565295266));
#218030=CARTESIAN_POINT('Ctrl Pts',(3.40329239908198,7.14876148495397,17.7243533920744));
#218031=CARTESIAN_POINT('Ctrl Pts',(3.1101104504096,7.28110057494453,17.7359504514779));
#218032=CARTESIAN_POINT('Ctrl Pts',(2.08862568196925,7.66919295046357,17.7740200046964));
#218033=CARTESIAN_POINT('Ctrl Pts',(1.33150665333911,7.83617718435891,17.7980517133665));
#218034=CARTESIAN_POINT('Ctrl Pts',(0.538504565817504,7.89268671613492,
17.8277355579075));
#218035=CARTESIAN_POINT('Ctrl Pts',(0.514687785514003,7.89427559896378,
17.8286315431259));
#218036=CARTESIAN_POINT('Ctrl Pts',(0.483124760025503,7.89623781298593,
17.8298252641054));
#218037=CARTESIAN_POINT('Ctrl Pts',(0.475384473094035,7.89670758829863,
17.8301185071108));
#218038=CARTESIAN_POINT('Ctrl Pts',(0.359055861748371,7.90359617622608,
17.834533373592));
#218039=CARTESIAN_POINT('Ctrl Pts',(0.250351708259917,7.90778576104458,
17.8387599924468));
#218040=CARTESIAN_POINT('Ctrl Pts',(0.131133523855111,7.909920011679,17.8435378505872));
#218041=CARTESIAN_POINT('Ctrl Pts',(0.1206662575226,7.91008661422039,17.8439585460098));
#218042=CARTESIAN_POINT('Ctrl Pts',(0.105154395058921,7.91030271251114,
17.8445838124572));
#218043=CARTESIAN_POINT('Ctrl Pts',(0.100109994754808,7.91036816077997,
17.8447874321589));
#218044=CARTESIAN_POINT('Ctrl Pts',(0.091488194108342,7.91047177541537,
17.8451359480434));
#218045=CARTESIAN_POINT('Ctrl Pts',(0.0879108186967583,7.91051234037162,
17.8452806999385));
#218046=CARTESIAN_POINT('Ctrl Pts',(0.0809624521533742,7.91058641606786,
17.8455621363214));
#218047=CARTESIAN_POINT('Ctrl Pts',(0.0775914646616999,7.91062019877506,
17.8456988042998));
#218048=CARTESIAN_POINT('Ctrl Pts',(0.0695428551312033,7.91069571360369,
17.8460254259222));
#218049=CARTESIAN_POINT('Ctrl Pts',(0.0648652464374623,7.91073545137829,
17.8462155001267));
#218050=CARTESIAN_POINT('Ctrl Pts',(0.0507019376084755,7.91084321017827,
17.8467917898599));
#218051=CARTESIAN_POINT('Ctrl Pts',(0.0412162212705007,7.91089831839667,
17.8471787896223));
#218052=CARTESIAN_POINT('Ctrl Pts',(-0.0493513180513969,7.91126158142155,
17.8508835022615));
#218053=CARTESIAN_POINT('Ctrl Pts',(-0.130430537977473,7.91034021487243,
17.8542744756896));
#218054=CARTESIAN_POINT('Ctrl Pts',(-0.468429134589048,7.90130154356842,
17.8686752118965));
#218055=CARTESIAN_POINT('Ctrl Pts',(-0.724875649511695,7.8819114770744,
17.8802352980139));
#218056=CARTESIAN_POINT('Ctrl Pts',(-1.18498850829019,7.82447690145656,
17.9015486843676));
#218057=CARTESIAN_POINT('Ctrl Pts',(-1.38898920206389,7.79084995150255,
17.9112052138981));
#218058=CARTESIAN_POINT('Ctrl Pts',(-1.87779738768121,7.69046550426202,
17.9345216740625));
#218059=CARTESIAN_POINT('Ctrl Pts',(-2.16068967225937,7.61582660293843,
17.9481577013894));
#218060=CARTESIAN_POINT('Ctrl Pts',(-2.61111143578272,7.46986103314748,
17.969683821983));
#218061=CARTESIAN_POINT('Ctrl Pts',(-2.78145116834839,7.40812131488053,
17.9777827967962));
#218062=CARTESIAN_POINT('Ctrl Pts',(-3.19882536764348,7.24041575186159,
17.9974450563588));
#218063=CARTESIAN_POINT('Ctrl Pts',(-3.44287123018338,7.12760562098013,
18.0087729044886));
#218064=CARTESIAN_POINT('Ctrl Pts',(-3.70021990464694,6.99233715146218,
18.0205271646795));
#218065=CARTESIAN_POINT('Ctrl Pts',(-3.71967465505053,6.98200735133162,
18.0214145976387));
#218066=CARTESIAN_POINT('Ctrl Pts',(-3.74740066349827,6.96713702209471,
18.0226777236157));
#218067=CARTESIAN_POINT('Ctrl Pts',(-3.75570724207176,6.96266279020748,
18.023055943862));
#218068=CARTESIAN_POINT('Ctrl Pts',(-3.76991834605047,6.95497533077351,
18.0237026640499));
#218069=CARTESIAN_POINT('Ctrl Pts',(-3.77582680645159,6.95176942335889,
18.0239714433805));
#218070=CARTESIAN_POINT('Ctrl Pts',(-3.78720482388141,6.94557697079396,
18.0244888387639));
#218071=CARTESIAN_POINT('Ctrl Pts',(-3.79267495083239,6.94259148681735,
18.0247374951372));
#218072=CARTESIAN_POINT('Ctrl Pts',(-3.80640154267989,6.93507872781798,
18.025361247898));
#218073=CARTESIAN_POINT('Ctrl Pts',(-3.8146534737496,6.93054316350501,18.025736026294));
#218074=CARTESIAN_POINT('Ctrl Pts',(-3.84244160334208,6.91520512203659,
18.0269974201178));
#218075=CARTESIAN_POINT('Ctrl Pts',(-3.86194025680446,6.90433463984726,
18.027881423695));
#218076=CARTESIAN_POINT('Ctrl Pts',(-4.21647187341269,6.70471179813409,
18.0439354013687));
#218077=CARTESIAN_POINT('Ctrl Pts',(-4.53736164708381,6.49185541262765,
18.0581116042004));
#218078=CARTESIAN_POINT('Ctrl Pts',(-5.50449033298963,5.74345105556112,
18.1012394415903));
#218079=CARTESIAN_POINT('Ctrl Pts',(-6.08154747687998,5.12843857623232,
18.1271523554186));
#218080=CARTESIAN_POINT('Ctrl Pts',(-6.57384695119827,4.40114530004626,
18.1616701216648));
#218081=CARTESIAN_POINT('Ctrl Pts',(-6.59617182633263,4.36761500298037,
18.1632702885342));
#218082=CARTESIAN_POINT('Ctrl Pts',(-6.62250875064856,4.3273963979237,18.1652020020667));
#218083=CARTESIAN_POINT('Ctrl Pts',(-6.62676857489583,4.32087028158809,
18.1655158413832));
#218084=CARTESIAN_POINT('Ctrl Pts',(-6.63372543031743,4.31017778613808,
18.1660306621788));
#218085=CARTESIAN_POINT('Ctrl Pts',(-6.63642821456398,4.30601511674972,
18.1662312395067));
#218086=CARTESIAN_POINT('Ctrl Pts',(-6.64125779764992,4.29856152900336,
18.1665906599341));
#218087=CARTESIAN_POINT('Ctrl Pts',(-6.64338607446431,4.29527156521906,
18.1667494000091));
#218088=CARTESIAN_POINT('Ctrl Pts',(-6.64788389208938,4.2883073434912,18.1670856193968));
#218089=CARTESIAN_POINT('Ctrl Pts',(-6.6502528321763,4.28463270105201,18.1672631400872));
#218090=CARTESIAN_POINT('Ctrl Pts',(-6.65653732615097,4.27486657842691,
18.167735241838));
#218091=CARTESIAN_POINT('Ctrl Pts',(-6.66044755655857,4.26877169493221,
18.1680301866821));
#218092=CARTESIAN_POINT('Ctrl Pts',(-6.67842522718944,4.24066503005928,
18.169391741989));
#218093=CARTESIAN_POINT('Ctrl Pts',(-6.69239180785445,4.21858925136638,
18.170465130678));
#218094=CARTESIAN_POINT('Ctrl Pts',(-6.79808284028377,4.04968668031033,
18.1787055074252));
#218095=CARTESIAN_POINT('Ctrl Pts',(-6.88506936362933,3.89996217116627,
18.1861696038195));
#218096=CARTESIAN_POINT('Ctrl Pts',(-7.03269744742566,3.62550428521574,
18.1999697160386));
#218097=CARTESIAN_POINT('Ctrl Pts',(-7.09510734782595,3.50179438647836,
18.2062311853947));
#218098=CARTESIAN_POINT('Ctrl Pts',(-7.54810672283103,2.54196902095565,
18.2547946016206));
#218099=CARTESIAN_POINT('Ctrl Pts',(-7.79304169727483,1.64462231686705,
18.2990276855453));
#218100=CARTESIAN_POINT('Ctrl Pts',(-7.88149309390995,0.683896519358582,
18.3391263512647));
#218101=CARTESIAN_POINT('Ctrl Pts',(-7.88497679169827,0.642486500084795,
18.3408433137367));
#218102=CARTESIAN_POINT('Ctrl Pts',(-7.89257334162507,0.542790049007174,
18.3449498826676));
#218103=CARTESIAN_POINT('Ctrl Pts',(-7.89636707329895,0.484481399242725,
18.3473294003498));
#218104=CARTESIAN_POINT('Ctrl Pts',(-7.90024278748618,0.412635049269635,
18.3502347043649));
#218105=CARTESIAN_POINT('Ctrl Pts',(-7.90093644115714,0.399132985684674,
18.3507795393431));
#218106=CARTESIAN_POINT('Ctrl Pts',(-7.90202878927546,0.376750620175531,
18.3516808078834));
#218107=CARTESIAN_POINT('Ctrl Pts',(-7.90244713368098,0.367871331287926,
18.3520378527977));
#218108=CARTESIAN_POINT('Ctrl Pts',(-7.90315779313715,0.352226843907147,
18.3526660630081));
#218109=CARTESIAN_POINT('Ctrl Pts',(-7.90345638917552,0.345461947958117,
18.3529374233963));
#218110=CARTESIAN_POINT('Ctrl Pts',(-7.90403589271197,0.331938788771921,
18.3534793078982));
#218111=CARTESIAN_POINT('Ctrl Pts',(-7.90431681896681,0.325180532104748,
18.3537498323726));
#218112=CARTESIAN_POINT('Ctrl Pts',(-7.90490883545092,0.310484159625379,
18.3543374935094));
#218113=CARTESIAN_POINT('Ctrl Pts',(-7.90521663713799,0.302545914787239,
18.354654527851));
#218114=CARTESIAN_POINT('Ctrl Pts',(-7.90593743813165,0.283203885276079,
18.3554260549983));
#218115=CARTESIAN_POINT('Ctrl Pts',(-7.90633772230234,0.271799629455422,
18.3558801533904));
#218116=CARTESIAN_POINT('Ctrl Pts',(-7.90777074649013,0.228286764508202,
18.3576097295215));
#218117=CARTESIAN_POINT('Ctrl Pts',(-7.90863258422699,0.196172638484583,
18.3588799192196));
#218118=CARTESIAN_POINT('Ctrl Pts',(-7.91042368178897,0.109820990047875,
18.362278829094));
#218119=CARTESIAN_POINT('Ctrl Pts',(-7.91099075449839,0.0555774990504133,
18.3643964145847));
#218120=CARTESIAN_POINT('Ctrl Pts',(-7.91099988786644,0.00133198240303771,
18.3664974980729));
#218121=CARTESIAN_POINT('',(-7.91099433110756,0.00947064855683299,22.3535317449623));
#218122=CARTESIAN_POINT('Ctrl Pts',(-7.91099988478435,0.00135016367355217,
18.3664967938599));
#218123=CARTESIAN_POINT('Ctrl Pts',(-7.91115913952513,-0.93176947257981,
18.402639240933));
#218124=CARTESIAN_POINT('Ctrl Pts',(-7.74625062688717,-1.85749765228585,
18.4325732657663));
#218125=CARTESIAN_POINT('Ctrl Pts',(-7.33513467715508,-2.97416559759076,
18.475745801834));
#218126=CARTESIAN_POINT('Ctrl Pts',(-7.23475610488461,-3.21063296551924,
18.4854408182715));
#218127=CARTESIAN_POINT('Ctrl Pts',(-7.1142579140074,-3.4600090221591,18.4964894798939));
#218128=CARTESIAN_POINT('Ctrl Pts',(-7.10541019306603,-3.47814233175404,
18.4972971599541));
#218129=CARTESIAN_POINT('Ctrl Pts',(-7.09245985157269,-3.5044282765506,
18.4984740239186));
#218130=CARTESIAN_POINT('Ctrl Pts',(-7.0884123018454,-3.51260805241907,
18.4988411003412));
#218131=CARTESIAN_POINT('Ctrl Pts',(-7.08130936149064,-3.52690025716869,
18.4994839558376));
#218132=CARTESIAN_POINT('Ctrl Pts',(-7.07826018428449,-3.53301577415346,
18.499759502394));
#218133=CARTESIAN_POINT('Ctrl Pts',(-7.07234163031472,-3.5448477789195,
18.5002935259715));
#218134=CARTESIAN_POINT('Ctrl Pts',(-7.06947323642752,-3.55056475377522,
18.5005519667374));
#218135=CARTESIAN_POINT('Ctrl Pts',(-7.06263574176736,-3.5641513806774,
18.5011671331627));
#218136=CARTESIAN_POINT('Ctrl Pts',(-7.05866041999558,-3.57201788346468,
18.5015240835875));
#218137=CARTESIAN_POINT('Ctrl Pts',(-7.04667269843559,-3.59564143994581,
18.5025983319648));
#218138=CARTESIAN_POINT('Ctrl Pts',(-7.03862064736651,-3.61137824947899,
18.5033170300506));
#218139=CARTESIAN_POINT('Ctrl Pts',(-6.95315121321176,-3.77704675309989,
18.51091491882));
#218140=CARTESIAN_POINT('Ctrl Pts',(-6.87101047988283,-3.92448794007304,
18.5179512888794));
#218141=CARTESIAN_POINT('Ctrl Pts',(-6.71256541137726,-4.18865051896204,
18.5309603610538));
#218142=CARTESIAN_POINT('Ctrl Pts',(-6.63776753007232,-4.30620120436085,
18.5369025949031));
#218143=CARTESIAN_POINT('Ctrl Pts',(-6.52916878006164,-4.46731465751185,
18.5452282556834));
#218144=CARTESIAN_POINT('Ctrl Pts',(-6.49795694959084,-4.51259356235029,
18.5475887696759));
#218145=CARTESIAN_POINT('Ctrl Pts',(-6.28527527934746,-4.8143478705476,
18.5634513492042));
#218146=CARTESIAN_POINT('Ctrl Pts',(-6.08913477802393,-5.0601455121102,
18.5769993967422));
#218147=CARTESIAN_POINT('Ctrl Pts',(-5.64215614832003,-5.55654257192806,
18.6054902147358));
#218148=CARTESIAN_POINT('Ctrl Pts',(-5.38804073534318,-5.80328534622556,
18.6203555815865));
#218149=CARTESIAN_POINT('Ctrl Pts',(-4.83845037421414,-6.26960727931723,
18.6502432655373));
#218150=CARTESIAN_POINT('Ctrl Pts',(-4.54245300336523,-6.48727296774719,
18.6653107839227));
#218151=CARTESIAN_POINT('Ctrl Pts',(-4.19253084360786,-6.70886241736414,
18.6820841447806));
#218152=CARTESIAN_POINT('Ctrl Pts',(-4.1524198290262,-6.73376264849548,
18.6839918036046));
#218153=CARTESIAN_POINT('Ctrl Pts',(-4.09116656238656,-6.77103219012437,
18.6868823373086));
#218154=CARTESIAN_POINT('Ctrl Pts',(-4.07018590320014,-6.78366475284956,
18.6878684239068));
#218155=CARTESIAN_POINT('Ctrl Pts',(-4.0319917807993,-6.80642064851768,
18.689656349691));
#218156=CARTESIAN_POINT('Ctrl Pts',(-4.01479801417763,-6.81657660948537,
18.6904585905905));
#218157=CARTESIAN_POINT('Ctrl Pts',(-3.97765771143759,-6.83832526097283,
18.6921858919366));
#218158=CARTESIAN_POINT('Ctrl Pts',(-3.95769853468321,-6.84989602526038,
18.6931106690872));
#218159=CARTESIAN_POINT('Ctrl Pts',(-3.90412178559349,-6.88064327951778,
18.6955838471163));
#218160=CARTESIAN_POINT('Ctrl Pts',(-3.87041356194284,-6.89966069714503,
18.6971302014744));
#218161=CARTESIAN_POINT('Ctrl Pts',(-3.70600453535699,-6.99083257379868,
18.704626328575));
#218162=CARTESIAN_POINT('Ctrl Pts',(-3.57341725905485,-7.05952547009614,
18.7105303120116));
#218163=CARTESIAN_POINT('Ctrl Pts',(-2.97324397932429,-7.34922940900218,
18.7366930187995));
#218164=CARTESIAN_POINT('Ctrl Pts',(-2.48660803953748,-7.52782393940463,
18.7563310566229));
#218165=CARTESIAN_POINT('Ctrl Pts',(-1.81910216947437,-7.70094331671891,
18.7829684336073));
#218166=CARTESIAN_POINT('Ctrl Pts',(-1.65080460185735,-7.738766237814,18.7896693023064));
#218167=CARTESIAN_POINT('Ctrl Pts',(-1.39977847187603,-7.78661973499417,
18.7997488734291));
#218168=CARTESIAN_POINT('Ctrl Pts',(-1.31790901964077,-7.80089367498487,
18.8030495767753));
#218169=CARTESIAN_POINT('Ctrl Pts',(-1.21752849416448,-7.81676971183015,
18.8071237155196));
#218170=CARTESIAN_POINT('Ctrl Pts',(-1.19921601069593,-7.81960007400795,
18.8078680844331));
#218171=CARTESIAN_POINT('Ctrl Pts',(-1.16980652823982,-7.8240398397127,
18.8090653669125));
#218172=CARTESIAN_POINT('Ctrl Pts',(-1.15871582910239,-7.82569002410157,
18.8095172896549));
#218173=CARTESIAN_POINT('Ctrl Pts',(-1.13754706035839,-7.82879373628687,
18.8103806325824));
#218174=CARTESIAN_POINT('Ctrl Pts',(-1.1274696145841,-7.83025139745363,
18.8107919575086));
#218175=CARTESIAN_POINT('Ctrl Pts',(-1.10442226384094,-7.83353968730601,
18.8117333947354));
#218176=CARTESIAN_POINT('Ctrl Pts',(-1.09145058039057,-7.83535756673221,
18.8122637880096));
#218177=CARTESIAN_POINT('Ctrl Pts',(-1.05760186042179,-7.84001551151188,
18.8136491308801));
#218178=CARTESIAN_POINT('Ctrl Pts',(-1.03671792768029,-7.84280439947771,
18.8145051643668));
#218179=CARTESIAN_POINT('Ctrl Pts',(-0.899734372558705,-7.86054079557132,
18.8201281243445));
#218180=CARTESIAN_POINT('Ctrl Pts',(-0.783327871189056,-7.87299308963963,
18.8249439046932));
#218181=CARTESIAN_POINT('Ctrl Pts',(-0.213703552831976,-7.92116885966793,
18.8486252761663));
#218182=CARTESIAN_POINT('Ctrl Pts',(0.24174137508306,-7.92036287116089,
18.8678721906608));
#218183=CARTESIAN_POINT('Ctrl Pts',(1.00541812397437,-7.85305160507057,
18.8998826604197));
#218184=CARTESIAN_POINT('Ctrl Pts',(1.31435854628966,-7.80728862433748,
18.9127700839643));
#218185=CARTESIAN_POINT('Ctrl Pts',(1.69253212656578,-7.72818079147799,
18.9284874713727));
#218186=CARTESIAN_POINT('Ctrl Pts',(1.76505262311285,-7.71194091742455,
18.9314994482547));
#218187=CARTESIAN_POINT('Ctrl Pts',(1.86927515056508,-7.68705469088483,
18.9358270746457));
#218188=CARTESIAN_POINT('Ctrl Pts',(1.90116861851135,-7.67922895245231,
18.937151252008));
#218189=CARTESIAN_POINT('Ctrl Pts',(1.9567910150461,-7.66521305913183,18.9394606444427));
#218190=CARTESIAN_POINT('Ctrl Pts',(1.98054157131064,-7.65911074520033,
18.9404467529206));
#218191=CARTESIAN_POINT('Ctrl Pts',(2.02653558668333,-7.6470650964517,18.9423565368898));
#218192=CARTESIAN_POINT('Ctrl Pts',(2.04878222678175,-7.64113489373845,
18.9432803358976));
#218193=CARTESIAN_POINT('Ctrl Pts',(2.10192917437701,-7.62671892516321,
18.9454875741516));
#218194=CARTESIAN_POINT('Ctrl Pts',(2.13280446483298,-7.61814235504656,
18.9467700891275));
#218195=CARTESIAN_POINT('Ctrl Pts',(2.24590940118031,-7.58598245111726,
18.9514698040529));
#218196=CARTESIAN_POINT('Ctrl Pts',(2.32780747633226,-7.56125328908962,
18.9548756841669));
#218197=CARTESIAN_POINT('Ctrl Pts',(2.93191664336227,-7.36809672603653,
18.980047653073));
#218198=CARTESIAN_POINT('Ctrl Pts',(3.43577363822072,-7.14706256497588,
19.0013884629811));
#218199=CARTESIAN_POINT('Ctrl Pts',(4.23830843990542,-6.69036722695345,
19.0362271313472));
#218200=CARTESIAN_POINT('Ctrl Pts',(4.55033791160038,-6.48218312783275,
19.0500429369366));
#218201=CARTESIAN_POINT('Ctrl Pts',(5.11648357670775,-6.0433641097861,19.0766947732885));
#218202=CARTESIAN_POINT('Ctrl Pts',(5.37266927478679,-5.81679072891381,
19.0894903356786));
#218203=CARTESIAN_POINT('Ctrl Pts',(5.63364305523964,-5.55399071943741,
19.1041214108656));
#218204=CARTESIAN_POINT('Ctrl Pts',(5.65378287549411,-5.53348770293115,
19.1052617436981));
#218205=CARTESIAN_POINT('Ctrl Pts',(5.68824582176904,-5.49801869579115,
19.1072333252215));
#218206=CARTESIAN_POINT('Ctrl Pts',(5.70262277772041,-5.4831052838322,19.1080619644604));
#218207=CARTESIAN_POINT('Ctrl Pts',(5.72294106811683,-5.46186249235418,
19.1092420701152));
#218208=CARTESIAN_POINT('Ctrl Pts',(5.72893088045403,-5.45557946700145,
19.1095910859627));
#218209=CARTESIAN_POINT('Ctrl Pts',(5.73921145993667,-5.44476003216063,
19.1101920730499));
#218210=CARTESIAN_POINT('Ctrl Pts',(5.74350722721105,-5.44022837024231,
19.1104437866939));
#218211=CARTESIAN_POINT('Ctrl Pts',(5.75168961905515,-5.43157616266721,
19.1109243756278));
#218212=CARTESIAN_POINT('Ctrl Pts',(5.75557719420145,-5.42745651720956,
19.111153201165));
#218213=CARTESIAN_POINT('Ctrl Pts',(5.76462564571406,-5.41784726024587,
19.1116869532443));
#218214=CARTESIAN_POINT('Ctrl Pts',(5.76978310471141,-5.41235445020171,
19.1119920595269));
#218215=CARTESIAN_POINT('Ctrl Pts',(5.78737933147483,-5.39356033817725,
19.1130360537816));
#218216=CARTESIAN_POINT('Ctrl Pts',(5.79977995511999,-5.38022351883813,
19.1137769817191));
#218217=CARTESIAN_POINT('Ctrl Pts',(5.96965556164268,-5.19625323140725,
19.1240003535394));
#218218=CARTESIAN_POINT('Ctrl Pts',(6.11956056867999,-5.01884264982179,
19.1339570344492));
#218219=CARTESIAN_POINT('Ctrl Pts',(6.66922081269003,-4.3070379026706,19.1737745401103));
#218220=CARTESIAN_POINT('Ctrl Pts',(7.00857184624998,-3.72948711151417,
19.2054363194764));
#218221=CARTESIAN_POINT('Ctrl Pts',(7.42077676716266,-2.7676321216702,19.2522662244487));
#218222=CARTESIAN_POINT('Ctrl Pts',(7.54490312634706,-2.40877573281266,
19.2686423991422));
#218223=CARTESIAN_POINT('Ctrl Pts',(7.65206670126215,-2.00775489843252,
19.285667207868));
#218224=CARTESIAN_POINT('Ctrl Pts',(7.66108078447154,-1.97308027937703,
19.2871293770324));
#218225=CARTESIAN_POINT('Ctrl Pts',(7.67421383668803,-1.92111396659172,
19.2893060728995));
#218226=CARTESIAN_POINT('Ctrl Pts',(7.67851052542316,-1.90386790506852,
19.2900260504147));
#218227=CARTESIAN_POINT('Ctrl Pts',(7.6853094652972,-1.8761808791694,19.2911780834312));
#218228=CARTESIAN_POINT('Ctrl Pts',(7.68784863244946,-1.86574909203476,
19.2916112711375));
#218229=CARTESIAN_POINT('Ctrl Pts',(7.69265147859991,-1.84584104174467,
19.2924363161049));
#218230=CARTESIAN_POINT('Ctrl Pts',(7.6949189022797,-1.83636570725299,19.2928282876486));
#218231=CARTESIAN_POINT('Ctrl Pts',(7.69888555652324,-1.819653113123,19.2935183961487));
#218232=CARTESIAN_POINT('Ctrl Pts',(7.70059209853602,-1.81241761105669,
19.2938167568333));
#218233=CARTESIAN_POINT('Ctrl Pts',(7.70391879305557,-1.79822336728175,
19.2944012589736));
#218234=CARTESIAN_POINT('Ctrl Pts',(7.7055397218824,-1.79126481666798,19.2946874239375));
#218235=CARTESIAN_POINT('Ctrl Pts',(7.70938724769102,-1.77464575281496,
19.2953699661643));
#218236=CARTESIAN_POINT('Ctrl Pts',(7.7116051192622,-1.76498322040901,19.2957660761962));
#218237=CARTESIAN_POINT('Ctrl Pts',(7.71947487864257,-1.73039926526118,
19.2971812326588));
#218238=CARTESIAN_POINT('Ctrl Pts',(7.72502419679118,-1.70545454149892,
19.2981971426909));
#218239=CARTESIAN_POINT('Ctrl Pts',(7.80439777401764,-1.34032523417243,
19.3129981917866));
#218240=CARTESIAN_POINT('Ctrl Pts',(7.85581443988878,-0.995643531176569,
19.3260684634179));
#218241=CARTESIAN_POINT('Ctrl Pts',(7.90742131691975,-0.368379645686695,
19.3488064406817));
#218242=CARTESIAN_POINT('Ctrl Pts',(7.91551921976296,-0.0870530682486353,
19.3586347939389));
#218243=CARTESIAN_POINT('Ctrl Pts',(7.89800906097888,0.626353289272118,
19.3833479612142));
#218244=CARTESIAN_POINT('Ctrl Pts',(7.85198267404627,1.05697837594131,19.3980564830445));
#218245=CARTESIAN_POINT('Ctrl Pts',(7.72969810845085,1.69833483242862,19.4217884829383));
#218246=CARTESIAN_POINT('Ctrl Pts',(7.67934506566328,1.91317056795507,19.430063907437));
#218247=CARTESIAN_POINT('Ctrl Pts',(7.61129410602145,2.15712626801572,19.4400823283802));
#218248=CARTESIAN_POINT('Ctrl Pts',(7.60230684550761,2.18858909984918,19.4413865434531));
#218249=CARTESIAN_POINT('Ctrl Pts',(7.5905058137588,2.22895257780103,19.4430745568355));
#218250=CARTESIAN_POINT('Ctrl Pts',(7.5878709656063,2.23790578688966,19.4434499235521));
#218251=CARTESIAN_POINT('Ctrl Pts',(7.58360268418897,2.25231520143772,19.444055535564));
#218252=CARTESIAN_POINT('Ctrl Pts',(7.5819791859609,2.25777436022152,19.4442853232697));
#218253=CARTESIAN_POINT('Ctrl Pts',(7.57887799549317,2.26816132502367,19.4447231837878));
#218254=CARTESIAN_POINT('Ctrl Pts',(7.57740138831986,2.2730894542476,19.4449312072538));
#218255=CARTESIAN_POINT('Ctrl Pts',(7.57402734311617,2.2843104004534,19.4454054899613));
#218256=CARTESIAN_POINT('Ctrl Pts',(7.57212686931596,2.29060229514045,19.4456718852432));
#218257=CARTESIAN_POINT('Ctrl Pts',(7.56644911008027,2.30931535700076,19.4464655155457));
#218258=CARTESIAN_POINT('Ctrl Pts',(7.56264909809753,2.32172956430267,19.4469937527857));
#218259=CARTESIAN_POINT('Ctrl Pts',(7.53601424635286,2.40798338908755,19.4506758101268));
#218260=CARTESIAN_POINT('Ctrl Pts',(7.51212938856055,2.48149274529982,19.453874324933));
#218261=CARTESIAN_POINT('Ctrl Pts',(7.33940042586255,2.98772929277415,19.476267391495));
#218262=CARTESIAN_POINT('Ctrl Pts',(7.15433387048857,3.40717106135049,19.4966171699505));
#218263=CARTESIAN_POINT('Ctrl Pts',(6.76768100932711,4.11118799554153,19.5319333696045));
#218264=CARTESIAN_POINT('Ctrl Pts',(6.58162534955884,4.40290818516588,19.5469758080647));
#218265=CARTESIAN_POINT('Ctrl Pts',(6.27446864134037,4.82131002998187,19.5689359944092));
#218266=CARTESIAN_POINT('Ctrl Pts',(6.16728727745257,4.95767666270367,19.5761659469251));
#218267=CARTESIAN_POINT('Ctrl Pts',(5.99111129211771,5.167260839965,19.587409994742));
#218268=CARTESIAN_POINT('Ctrl Pts',(5.92505672531264,5.24287158785245,19.5914956734813));
#218269=CARTESIAN_POINT('Ctrl Pts',(5.84092050011597,5.33555836502391,19.5965472277717));
#218270=CARTESIAN_POINT('Ctrl Pts',(5.82417478916609,5.35383258879095,19.5975453546343));
#218271=CARTESIAN_POINT('Ctrl Pts',(5.79749993295642,5.38266900851745,19.5991239664494));
#218272=CARTESIAN_POINT('Ctrl Pts',(5.78762720404809,5.39328308884937,19.599705797346));
#218273=CARTESIAN_POINT('Ctrl Pts',(5.76991758882429,5.41221790643816,19.6007451749863));
#218274=CARTESIAN_POINT('Ctrl Pts',(5.76209174468442,5.42054889980848,19.6012029815743));
#218275=CARTESIAN_POINT('Ctrl Pts',(5.74410208738454,5.43961678725398,19.6022519735008));
#218276=CARTESIAN_POINT('Ctrl Pts',(5.73392616880704,5.45034221630158,19.6028428718792));
#218277=CARTESIAN_POINT('Ctrl Pts',(5.70561494860836,5.48001523298295,19.6044800958982));
#218278=CARTESIAN_POINT('Ctrl Pts',(5.68741535867653,5.49890129410917,19.6055249214135));
#218279=CARTESIAN_POINT('Ctrl Pts',(5.60063599962763,5.58806219285022,19.610471430596));
#218280=CARTESIAN_POINT('Ctrl Pts',(5.53084484656556,5.65714755327642,19.6143455111531));
#218281=CARTESIAN_POINT('Ctrl Pts',(5.20900942805888,5.96407816705975,19.6317566789819));
#218282=CARTESIAN_POINT('Ctrl Pts',(4.94278493607555,6.18650958866493,19.6449139702574));
#218283=CARTESIAN_POINT('Ctrl Pts',(4.24926817039201,6.69251178863727,19.6769018021472));
#218284=CARTESIAN_POINT('Ctrl Pts',(3.80741566888015,6.95338434965661,19.6953251887285));
#218285=CARTESIAN_POINT('Ctrl Pts',(3.19331518712385,7.23975903988982,19.7208282012629));
#218286=CARTESIAN_POINT('Ctrl Pts',(3.04099545569801,7.30504731325001,19.7271542022879));
#218287=CARTESIAN_POINT('Ctrl Pts',(2.81638952548769,7.39307655842408,19.7365983951208));
#218288=CARTESIAN_POINT('Ctrl Pts',(2.74564559993629,7.41964020427929,19.7395895001563));
#218289=CARTESIAN_POINT('Ctrl Pts',(2.66197343911482,7.44969774688287,19.7431558737268));
#218290=CARTESIAN_POINT('Ctrl Pts',(2.64940211145755,7.45417785939972,19.7436924599653));
#218291=CARTESIAN_POINT('Ctrl Pts',(2.63012397104017,7.46099318662085,19.7445165412959));
#218292=CARTESIAN_POINT('Ctrl Pts',(2.62342521601794,7.46335122913246,19.7448031188863));
#218293=CARTESIAN_POINT('Ctrl Pts',(2.61173978571683,7.46744696521154,19.7453034363137));
#218294=CARTESIAN_POINT('Ctrl Pts',(2.60675452299177,7.46918869377547,19.7455170115554));
#218295=CARTESIAN_POINT('Ctrl Pts',(2.59554004676288,7.47309416176346,19.7459977502483));
#218296=CARTESIAN_POINT('Ctrl Pts',(2.58930986876329,7.47525510521967,19.7462650285767));
#218297=CARTESIAN_POINT('Ctrl Pts',(2.57264826612155,7.48101086995242,19.7469803833945));
#218298=CARTESIAN_POINT('Ctrl Pts',(2.56221203357467,7.4845916542505,19.7474290446012));
#218299=CARTESIAN_POINT('Ctrl Pts',(2.51732314565953,7.49988862825384,19.7493614872902));
#218300=CARTESIAN_POINT('Ctrl Pts',(2.48279773600636,7.51138872613442,19.7508544559496));
#218301=CARTESIAN_POINT('Ctrl Pts',(1.94822871550004,7.68536053016548,19.7740875340796));
#218302=CARTESIAN_POINT('Ctrl Pts',(1.43338396258432,7.79779192508504,19.7983356054488));
#218303=CARTESIAN_POINT('Ctrl Pts',(0.750881799979827,7.87693980052665,
19.8299691452143));
#218304=CARTESIAN_POINT('Ctrl Pts',(0.589920483933854,7.89062729225981,
19.8373972286174));
#218305=CARTESIAN_POINT('Ctrl Pts',(0.0926095563395046,7.9176133539248,
19.8601090107858));
#218306=CARTESIAN_POINT('Ctrl Pts',(-0.244273348460455,7.91438809406514,
19.8751423896768));
#218307=CARTESIAN_POINT('Ctrl Pts',(-0.739068114120515,7.87801718912681,
19.8963783846863));
#218308=CARTESIAN_POINT('Ctrl Pts',(-0.897801805706668,7.86150954990597,
19.9030656575271));
#218309=CARTESIAN_POINT('Ctrl Pts',(-1.10706140818153,7.83332607715578,
19.9117114817328));
#218310=CARTESIAN_POINT('Ctrl Pts',(-1.15812052083219,7.82594015999699,
19.9138076758021));
#218311=CARTESIAN_POINT('Ctrl Pts',(-1.22224268985226,7.81602332073487,
19.9164235814831));
#218312=CARTESIAN_POINT('Ctrl Pts',(-1.23537587429331,7.81395829235747,
19.9169584822217));
#218313=CARTESIAN_POINT('Ctrl Pts',(-1.25624212914935,7.81062341453613,
19.9178069580068));
#218314=CARTESIAN_POINT('Ctrl Pts',(-1.26397859693608,7.80937516820079,
19.9181212399443));
#218315=CARTESIAN_POINT('Ctrl Pts',(-1.27852982873629,7.8070051989157,19.9187117934291));
#218316=CARTESIAN_POINT('Ctrl Pts',(-1.28534499998096,7.80588604389105,
19.9189881488892));
#218317=CARTESIAN_POINT('Ctrl Pts',(-1.30063800741792,7.80335412774052,
19.9196077566529));
#218318=CARTESIAN_POINT('Ctrl Pts',(-1.30911503066057,7.80193647156822,
19.9199508478283));
#218319=CARTESIAN_POINT('Ctrl Pts',(-1.33061856793118,7.79830429132077,
19.9208202481394));
#218320=CARTESIAN_POINT('Ctrl Pts',(-1.34364189862826,7.79607093630254,
19.9213459372932));
#218321=CARTESIAN_POINT('Ctrl Pts',(-1.41493531726343,7.78366096422403,
19.9242190814441));
#218322=CARTESIAN_POINT('Ctrl Pts',(-1.47309619834195,7.77286354876746,
19.9265460185952));
#218323=CARTESIAN_POINT('Ctrl Pts',(-2.44844572863632,7.58045168564622,
19.9652958194041));
#218324=CARTESIAN_POINT('Ctrl Pts',(-3.32625998410969,7.23836562082014,
19.9949453023875));
#218325=CARTESIAN_POINT('Ctrl Pts',(-4.293346126716,6.64758972347121,20.0340323555139));
#218326=CARTESIAN_POINT('Ctrl Pts',(-4.45866952752661,6.53785359401399,
20.0410243303857));
#218327=CARTESIAN_POINT('Ctrl Pts',(-4.74865554143482,6.32925204963865,
20.0541620798706));
#218328=CARTESIAN_POINT('Ctrl Pts',(-4.8747934221936,6.23261938609712,20.0601966652247));
#218329=CARTESIAN_POINT('Ctrl Pts',(-5.01682577456608,6.11685984872732,
20.0674725081515));
#218330=CARTESIAN_POINT('Ctrl Pts',(-5.0356506361448,6.10137180530029,20.0684469015648));
#218331=CARTESIAN_POINT('Ctrl Pts',(-5.05966581824736,6.08142660914316,
20.0697032978819));
#218332=CARTESIAN_POINT('Ctrl Pts',(-5.06492253958996,6.07704923973013,
20.069979136338));
#218333=CARTESIAN_POINT('Ctrl Pts',(-5.07335737880369,6.07000684594348,
20.0704230780638));
#218334=CARTESIAN_POINT('Ctrl Pts',(-5.07653910021436,6.06734612221237,
20.0705908443267));
#218335=CARTESIAN_POINT('Ctrl Pts',(-5.08257698970345,6.0622888453903,20.0709097958613));
#218336=CARTESIAN_POINT('Ctrl Pts',(-5.08543356001441,6.05989277197123,
20.071060943235));
#218337=CARTESIAN_POINT('Ctrl Pts',(-5.09192095375131,6.05444336884073,
20.0714047742904));
#218338=CARTESIAN_POINT('Ctrl Pts',(-5.09555070241924,6.05138881123872,
20.0715975564809));
#218339=CARTESIAN_POINT('Ctrl Pts',(-5.10499414418457,6.04342731109227,
20.0721001739626));
#218340=CARTESIAN_POINT('Ctrl Pts',(-5.11080346560196,6.03851528206595,
20.0724104152236));
#218341=CARTESIAN_POINT('Ctrl Pts',(-5.14703864484835,6.00778714623434,
20.0743520040089));
#218342=CARTESIAN_POINT('Ctrl Pts',(-5.17727538420419,5.98174996867785,
20.0760007739786));
#218343=CARTESIAN_POINT('Ctrl Pts',(-5.7095678509391,5.51632803470183,20.1055127140682));
#218344=CARTESIAN_POINT('Ctrl Pts',(-6.15423095249231,5.01542018242688,
20.1376510456358));
#218345=CARTESIAN_POINT('Ctrl Pts',(-6.83867378485568,4.01424623852371,
20.193830262923));
#218346=CARTESIAN_POINT('Ctrl Pts',(-7.09921848528766,3.53311406394057,
20.2181572790312));
#218347=CARTESIAN_POINT('Ctrl Pts',(-7.32813036484757,2.98079524870643,
20.2426123867452));
#218348=CARTESIAN_POINT('Ctrl Pts',(-7.34760086507924,2.93247278468919,
20.2447259042483));
#218349=CARTESIAN_POINT('Ctrl Pts',(-7.37132186341728,2.87188148432562,
20.2473440655732));
#218350=CARTESIAN_POINT('Ctrl Pts',(-7.37602113180862,2.85979047125106,
20.2478649406148));
#218351=CARTESIAN_POINT('Ctrl Pts',(-7.38341292886023,2.84063227376752,
20.2486877794603));
#218352=CARTESIAN_POINT('Ctrl Pts',(-7.38612508911111,2.83357272030832,
20.2489904516954));
#218353=CARTESIAN_POINT('Ctrl Pts',(-7.3911902850637,2.82033170334348,20.2495571521993));
#218354=CARTESIAN_POINT('Ctrl Pts',(-7.39354569841451,2.81415116023561,
20.2498212660011));
#218355=CARTESIAN_POINT('Ctrl Pts',(-7.39879151309521,2.80033423259518,
20.2504108008889));
#218356=CARTESIAN_POINT('Ctrl Pts',(-7.40167785063667,2.79269630723452,
20.2507360755296));
#218357=CARTESIAN_POINT('Ctrl Pts',(-7.40892907955581,2.77341764838255,
20.2515555408771));
#218358=CARTESIAN_POINT('Ctrl Pts',(-7.41327837291874,2.76177104876626,
20.2520491710258));
#218359=CARTESIAN_POINT('Ctrl Pts',(-7.43633450594891,2.69958411244033,
20.2546773562784));
#218360=CARTESIAN_POINT('Ctrl Pts',(-7.45455222123624,2.64886326568902,
20.2567943716127));
#218361=CARTESIAN_POINT('Ctrl Pts',(-7.76383412578447,1.75930673492556,
20.2934736017286));
#218362=CARTESIAN_POINT('Ctrl Pts',(-7.91212168501964,0.877724371696439,
20.3218504654584));
#218363=CARTESIAN_POINT('Ctrl Pts',(-7.9109860860975,-0.0159761828078189,
20.3531105060327));
#218364=CARTESIAN_POINT('Ctrl Pts',(-7.91097190483238,-0.0219000838148015,
20.3533178653847));
#218365=CARTESIAN_POINT('Ctrl Pts',(-7.91093271805898,-0.0330417282952556,
20.3537081602693));
#218366=CARTESIAN_POINT('Ctrl Pts',(-7.91090920425387,-0.0382594749948222,
20.3538910608219));
#218367=CARTESIAN_POINT('Ctrl Pts',(-7.91085671392213,-0.0478103392606033,
20.354226080611));
#218368=CARTESIAN_POINT('Ctrl Pts',(-7.91082933931471,-0.0521434649049955,
20.3543781614645));
#218369=CARTESIAN_POINT('Ctrl Pts',(-7.91077500806176,-0.0597537649582373,
20.3546454162844));
#218370=CARTESIAN_POINT('Ctrl Pts',(-7.91074957509471,-0.0630309504684151,
20.3547605530863));
#218371=CARTESIAN_POINT('Ctrl Pts',(-7.91070375574369,-0.0684973121570124,
20.3549526868767));
#218372=CARTESIAN_POINT('Ctrl Pts',(-7.91068449704923,-0.0706864983443649,
20.355029655987));
#218373=CARTESIAN_POINT('Ctrl Pts',(-7.91065244772581,-0.0741654566928713,
20.3551520084347));
#218374=CARTESIAN_POINT('Ctrl Pts',(-7.91064025039873,-0.0754552347215277,
20.3551973769727));
#218375=CARTESIAN_POINT('Ctrl Pts',(-7.9106210391236,-0.0774354709228726,
20.3552670450185));
#218376=CARTESIAN_POINT('Ctrl Pts',(-7.91061425020951,-0.0781259314439278,
20.355291338883));
#218377=CARTESIAN_POINT('Ctrl Pts',(-7.91060389694048,-0.0791650635999006,
20.3553279042374));
#218378=CARTESIAN_POINT('Ctrl Pts',(-7.91060039993006,-0.0795137359895382,
20.3553401740347));
#218379=CARTESIAN_POINT('Ctrl Pts',(-7.91059515665141,-0.0800330975359515,
20.3553584512692));
#218380=CARTESIAN_POINT('Ctrl Pts',(-7.91059342791128,-0.0802037868481622,
20.3553644582636));
#218381=CARTESIAN_POINT('Ctrl Pts',(-7.91021163026892,-0.117780955681033,
20.3566869262875));
#218382=CARTESIAN_POINT('Ctrl Pts',(-7.90956625051917,-0.155184018494225,
20.3580100540781));
#218383=CARTESIAN_POINT('Ctrl Pts',(-7.90225486069639,-0.455438532159219,
20.3686955101006));
#218384=CARTESIAN_POINT('Ctrl Pts',(-7.88275371481392,-0.717793124483094,
20.3784232310423));
#218385=CARTESIAN_POINT('Ctrl Pts',(-7.84826578401422,-0.994433342120351,
20.3895559488599));
#218386=CARTESIAN_POINT('Ctrl Pts',(-7.84625256633663,-1.01019510695341,
20.3901932917789));
#218387=CARTESIAN_POINT('Ctrl Pts',(-7.8434751755752,-1.0314304192876,20.3910561723516));
#218388=CARTESIAN_POINT('Ctrl Pts',(-7.84275275217372,-1.03690925719923,
20.3912791757272));
#218389=CARTESIAN_POINT('Ctrl Pts',(-7.84152088491908,-1.04617676565502,
20.3916570174797));
#218390=CARTESIAN_POINT('Ctrl Pts',(-7.84101443374242,-1.04996583913891,
20.3918116782628));
#218391=CARTESIAN_POINT('Ctrl Pts',(-7.84003558043433,-1.05724903860938,
20.3921093011222));
#218392=CARTESIAN_POINT('Ctrl Pts',(-7.83956358819452,-1.06074321996108,
20.3922522390309));
#218393=CARTESIAN_POINT('Ctrl Pts',(-7.83844739542212,-1.06896501090112,
20.3925889238262));
#218394=CARTESIAN_POINT('Ctrl Pts',(-7.83780125421114,-1.07369235101253,
20.3927827842399));
#218395=CARTESIAN_POINT('Ctrl Pts',(-7.83591556603223,-1.08739613535713,
20.3933455438195));
#218396=CARTESIAN_POINT('Ctrl Pts',(-7.83466487574452,-1.0963710123131,
20.3937150890883));
#218397=CARTESIAN_POINT('Ctrl Pts',(-7.82594405801734,-1.15817409114814,
20.3962665429619));
#218398=CARTESIAN_POINT('Ctrl Pts',(-7.8179552469144,-1.21092655710541,
20.3984779802046));
#218399=CARTESIAN_POINT('Ctrl Pts',(-7.79289516786784,-1.36580635467497,
20.4050616970903));
#218400=CARTESIAN_POINT('Ctrl Pts',(-7.77435217207518,-1.46768143170529,
20.4095089520627));
#218401=CARTESIAN_POINT('Ctrl Pts',(-7.71617226515173,-1.75517060488679,
20.4223354572617));
#218402=CARTESIAN_POINT('Ctrl Pts',(-7.67184895997818,-1.93975904408205,
20.4308992465233));
#218403=CARTESIAN_POINT('Ctrl Pts',(-7.46998374039145,-2.6645429696049,
20.4653957543712));
#218404=CARTESIAN_POINT('Ctrl Pts',(-7.26163172780135,-3.18892108742889,
20.4921743115637));
#218405=CARTESIAN_POINT('Ctrl Pts',(-6.94841175843544,-3.78357927309295,
20.522525732552));
#218406=CARTESIAN_POINT('Ctrl Pts',(-6.89540485111491,-3.87934157881735,
20.5274182978205));
#218407=CARTESIAN_POINT('Ctrl Pts',(-6.79349329571786,-4.05476252758364,
20.5363789912569));
#218408=CARTESIAN_POINT('Ctrl Pts',(-6.74513128574468,-4.13471341118438,
20.5404623431943));
#218409=CARTESIAN_POINT('Ctrl Pts',(-6.57236464952416,-4.40922524714831,
20.5544735784253));
#218410=CARTESIAN_POINT('Ctrl Pts',(-6.44086245243957,-4.59918984167382,
20.5641494735474));
#218411=CARTESIAN_POINT('Ctrl Pts',(-6.2875931070313,-4.80110430606929,
20.5744235808924));
#218412=CARTESIAN_POINT('Ctrl Pts',(-6.27388031458407,-4.819009799386,20.5753346260514));
#218413=CARTESIAN_POINT('Ctrl Pts',(-6.25447069753839,-4.84413065424665,
20.5766127819941));
#218414=CARTESIAN_POINT('Ctrl Pts',(-6.24883764349203,-4.85139501666961,
20.5769823933357));
#218415=CARTESIAN_POINT('Ctrl Pts',(-6.23902481984364,-4.86400414614803,
20.5776239495327));
#218416=CARTESIAN_POINT('Ctrl Pts',(-6.2348508175237,-4.86935337800691,
20.5778961208588));
#218417=CARTESIAN_POINT('Ctrl Pts',(-6.22613685514385,-4.88049126425749,
20.578462825857));
#218418=CARTESIAN_POINT('Ctrl Pts',(-6.22159569073457,-4.8862789708418,
20.5787573116687));
#218419=CARTESIAN_POINT('Ctrl Pts',(-6.21085777022427,-4.89992519470359,
20.57945165837));
#218420=CARTESIAN_POINT('Ctrl Pts',(-6.20465415569413,-4.9077783125172,
20.5798512479867));
#218421=CARTESIAN_POINT('Ctrl Pts',(-6.18421541467847,-4.93355089657461,
20.5811626713572));
#218422=CARTESIAN_POINT('Ctrl Pts',(-6.16991737192236,-4.95142044054334,
20.5820720145653));
#218423=CARTESIAN_POINT('Ctrl Pts',(-5.96280030440594,-5.20798299811566,
20.5951296223955));
#218424=CARTESIAN_POINT('Ctrl Pts',(-5.75632365626615,-5.43533201902799,
20.6067072602713));
#218425=CARTESIAN_POINT('Ctrl Pts',(-4.98117247113122,-6.19498330335456,
20.6462154594106));
#218426=CARTESIAN_POINT('Ctrl Pts',(-4.34789877793545,-6.65473250382228,
20.6713744183327));
#218427=CARTESIAN_POINT('Ctrl Pts',(-3.49770058106296,-7.09807048669171,
20.7070399331822));
#218428=CARTESIAN_POINT('Ctrl Pts',(-3.33483808871978,-7.17602698948031,
20.713991219408));
#218429=CARTESIAN_POINT('Ctrl Pts',(-3.15171630375763,-7.25609946828432,
20.7219676330616));
#218430=CARTESIAN_POINT('Ctrl Pts',(-3.13396522925643,-7.26378393725362,
20.7227421536145));
#218431=CARTESIAN_POINT('Ctrl Pts',(-3.10803096318952,-7.27489816116355,
20.7238754961013));
#218432=CARTESIAN_POINT('Ctrl Pts',(-3.09986982759641,-7.2783794057937,
20.7242323974466));
#218433=CARTESIAN_POINT('Ctrl Pts',(-3.08542729228833,-7.28451137045385,
20.7248644289317));
#218434=CARTESIAN_POINT('Ctrl Pts',(-3.07914828203073,-7.28716771724208,
20.7251393542828));
#218435=CARTESIAN_POINT('Ctrl Pts',(-3.06613143930582,-7.29265468864227,
20.7257095844235));
#218436=CARTESIAN_POINT('Ctrl Pts',(-3.05939310369036,-7.29548409960426,
20.7260049321062));
#218437=CARTESIAN_POINT('Ctrl Pts',(-3.04207255060414,-7.3027287416812,
20.7267645071582));
#218438=CARTESIAN_POINT('Ctrl Pts',(-3.03148465404137,-7.30713030324215,
20.7272292102662));
#218439=CARTESIAN_POINT('Ctrl Pts',(-2.98773973354293,-7.32520433913742,
20.7291506646386));
#218440=CARTESIAN_POINT('Ctrl Pts',(-2.95449972592711,-7.3386741754066,
20.7306142234757));
#218441=CARTESIAN_POINT('Ctrl Pts',(-2.71248951032243,-7.43483315481171,
20.7412909332252));
#218442=CARTESIAN_POINT('Ctrl Pts',(-2.50037975844424,-7.50882401135501,
20.7507580701854));
#218443=CARTESIAN_POINT('Ctrl Pts',(-1.85276467728768,-7.7042467763377,
20.779600183233));
#218444=CARTESIAN_POINT('Ctrl Pts',(-1.40971695344449,-7.79749093084379,
20.7991934325331));
#218445=CARTESIAN_POINT('Ctrl Pts',(-0.305814160610344,-7.93260803441085,
20.8465594412363));
#218446=CARTESIAN_POINT('Ctrl Pts',(0.356984446419582,-7.93047287432116,
20.8738100242726));
#218447=CARTESIAN_POINT('Ctrl Pts',(1.08411208581547,-7.83670451579456,
20.9036081091696));
#218448=CARTESIAN_POINT('Ctrl Pts',(1.15629005288069,-7.82638039668823,
20.9065618969188));
#218449=CARTESIAN_POINT('Ctrl Pts',(1.25495293821127,-7.81087326812838,
20.9105939419744));
#218450=CARTESIAN_POINT('Ctrl Pts',(1.28156897182594,-7.80655039467753,
20.9116811003882));
#218451=CARTESIAN_POINT('Ctrl Pts',(1.32707409424849,-7.79892063387666,
20.9135388799059));
#218452=CARTESIAN_POINT('Ctrl Pts',(1.34597418553832,-7.79568099650728,
20.9143102170922));
#218453=CARTESIAN_POINT('Ctrl Pts',(1.38475611839659,-7.78888820028072,
20.9158924160856));
#218454=CARTESIAN_POINT('Ctrl Pts',(1.40463651240967,-7.78532755731211,
20.9167031899448));
#218455=CARTESIAN_POINT('Ctrl Pts',(1.45065575160813,-7.77690335365144,
20.9185793249096));
#218456=CARTESIAN_POINT('Ctrl Pts',(1.47678417343494,-7.7719840705631,20.9196440554137));
#218457=CARTESIAN_POINT('Ctrl Pts',(1.55970026469578,-7.75593995857618,
20.9230214518708));
#218458=CARTESIAN_POINT('Ctrl Pts',(1.61639110852671,-7.74432368939628,
20.9253284824738));
#218459=CARTESIAN_POINT('Ctrl Pts',(1.71449273955713,-7.7230979706777,20.9293179100728));
#218460=CARTESIAN_POINT('Ctrl Pts',(1.75596283485193,-7.71377483252006,
20.9310034712683));
#218461=CARTESIAN_POINT('Ctrl Pts',(1.87030507303023,-7.68709900773947,
20.9356492737567));
#218462=CARTESIAN_POINT('Ctrl Pts',(1.94300922772652,-7.66904475770914,
20.9386013895525));
#218463=CARTESIAN_POINT('Ctrl Pts',(2.28569722099213,-7.57876072461122,
20.9525160476721));
#218464=CARTESIAN_POINT('Ctrl Pts',(2.55198792470274,-7.49328952122857,
20.9633209280324));
#218465=CARTESIAN_POINT('Ctrl Pts',(3.24401850819709,-7.22998877782816,
20.991810314466));
#218466=CARTESIAN_POINT('Ctrl Pts',(3.65967048777963,-7.02873921173164,
21.0093232520307));
#218467=CARTESIAN_POINT('Ctrl Pts',(4.09051295773349,-6.77150615721725,
21.029296334435));
#218468=CARTESIAN_POINT('Ctrl Pts',(4.12544680429371,-6.7502800322146,21.0309299765678));
#218469=CARTESIAN_POINT('Ctrl Pts',(4.1718124884069,-6.72161345953944,21.0331186328309));
#218470=CARTESIAN_POINT('Ctrl Pts',(4.18339203115805,-6.7144127106195,21.0336669567953));
#218471=CARTESIAN_POINT('Ctrl Pts',(4.20318470605052,-6.70203354195451,
21.0346071169437));
#218472=CARTESIAN_POINT('Ctrl Pts',(4.21140704806293,-6.69686986177469,
21.0349985469051));
#218473=CARTESIAN_POINT('Ctrl Pts',(4.22739850344639,-6.68678603365406,
21.0357615004399));
#218474=CARTESIAN_POINT('Ctrl Pts',(4.23516858712259,-6.68186744891962,
21.0361329819323));
#218475=CARTESIAN_POINT('Ctrl Pts',(4.25376519610399,-6.67005003458364,
21.0370239007636));
#218476=CARTESIAN_POINT('Ctrl Pts',(4.26458352875971,-6.66313838459529,
21.037543671038));
#218477=CARTESIAN_POINT('Ctrl Pts',(4.29712739648824,-6.64223493315225,
21.0391116879193));
#218478=CARTESIAN_POINT('Ctrl Pts',(4.31880118173396,-6.62816302686519,
21.0401619414964));
#218479=CARTESIAN_POINT('Ctrl Pts',(4.54743948071369,-6.47811991304877,
21.0513028943962));
#218480=CARTESIAN_POINT('Ctrl Pts',(4.74797559055538,-6.33261129572139,
21.0616086205743));
#218481=CARTESIAN_POINT('Ctrl Pts',(5.32898445241308,-5.86789840132567,
21.0927710499984));
#218482=CARTESIAN_POINT('Ctrl Pts',(5.68658896414178,-5.52204992429265,
21.1137025848621));
#218483=CARTESIAN_POINT('Ctrl Pts',(6.03013007694855,-5.12078763435865,
21.135467962359));
#218484=CARTESIAN_POINT('Ctrl Pts',(6.05069083617393,-5.0964767394766,21.1367780052267));
#218485=CARTESIAN_POINT('Ctrl Pts',(6.16874585856948,-4.95516791145632,
21.1443432367032));
#218486=CARTESIAN_POINT('Ctrl Pts',(6.26299321364288,-4.8354970408097,21.1505546318638));
#218487=CARTESIAN_POINT('Ctrl Pts',(6.38034049097667,-4.67730386373611,
21.1585295972884));
#218488=CARTESIAN_POINT('Ctrl Pts',(6.40664825261346,-4.64120398279059,
21.1603341951164));
#218489=CARTESIAN_POINT('Ctrl Pts',(6.44832737073148,-4.58298162851746,
21.1632208448287));
#218490=CARTESIAN_POINT('Ctrl Pts',(6.46389386310364,-4.56100017759178,
21.1643053084913));
#218491=CARTESIAN_POINT('Ctrl Pts',(6.49188557198494,-4.52104194207126,
21.16626712286));
#218492=CARTESIAN_POINT('Ctrl Pts',(6.50434913068953,-4.50309237202046,
21.1671449315492));
#218493=CARTESIAN_POINT('Ctrl Pts',(6.53371666520347,-4.46042199634498,
21.1692236400733));
#218494=CARTESIAN_POINT('Ctrl Pts',(6.55055497209323,-4.43565636767066,
21.1704237493483));
#218495=CARTESIAN_POINT('Ctrl Pts',(6.60024287218715,-4.36167584358126,
21.1739902911522));
#218496=CARTESIAN_POINT('Ctrl Pts',(6.63268146300191,-4.31218724120532,
21.176351968782));
#218497=CARTESIAN_POINT('Ctrl Pts',(6.84538586891979,-3.97960421005094,
21.1920713162999));
#218498=CARTESIAN_POINT('Ctrl Pts',(7.00804105708511,-3.68563810160182,
21.2052842386913));
#218499=CARTESIAN_POINT('Ctrl Pts',(7.34758256731569,-2.96769679575803,
21.236090889135));
#218500=CARTESIAN_POINT('Ctrl Pts',(7.50722048829168,-2.53689874396757,
21.2533323760965));
#218501=CARTESIAN_POINT('Ctrl Pts',(7.72951205768504,-1.72733523885317,
21.2845384645283));
#218502=CARTESIAN_POINT('Ctrl Pts',(7.80371114555069,-1.35318819759569,
21.2985448294476));
#218503=CARTESIAN_POINT('Ctrl Pts',(7.86847397019705,-0.831809383643287,
21.3186192712006));
#218504=CARTESIAN_POINT('Ctrl Pts',(7.88235054647267,-0.687994848071836,
21.3242182200834));
#218505=CARTESIAN_POINT('Ctrl Pts',(7.89450002917865,-0.511694709694051,
21.3312287551038));
#218506=CARTESIAN_POINT('Ctrl Pts',(7.89652144218214,-0.479490630347162,
21.3325153472307));
#218507=CARTESIAN_POINT('Ctrl Pts',(7.89893019141788,-0.436955011831059,
21.3342235400982));
#218508=CARTESIAN_POINT('Ctrl Pts',(7.89949439281172,-0.426633552315023,
21.3346387280268));
#218509=CARTESIAN_POINT('Ctrl Pts',(7.90035066610369,-0.410384663632813,
21.3352934691067));
#218510=CARTESIAN_POINT('Ctrl Pts',(7.9006563014503,-0.404457940554016,
21.3355325176555));
#218511=CARTESIAN_POINT('Ctrl Pts',(7.90125331601707,-0.392622006344857,
21.3360103847259));
#218512=CARTESIAN_POINT('Ctrl Pts',(7.90154473584647,-0.386712801573303,
21.3362492015308));
#218513=CARTESIAN_POINT('Ctrl Pts',(7.90219083537574,-0.373305962584931,
21.3367915782132));
#218514=CARTESIAN_POINT('Ctrl Pts',(7.90254147350319,-0.365808145697425,
21.3370952926291));
#218515=CARTESIAN_POINT('Ctrl Pts',(7.9035418490985,-0.343743863763675,
21.3379902212282));
#218516=CARTESIAN_POINT('Ctrl Pts',(7.90416198416795,-0.32917613608675,
21.3385825890612));
#218517=CARTESIAN_POINT('Ctrl Pts',(7.90547124123999,-0.296280032940708,
21.3399237800177));
#218518=CARTESIAN_POINT('Ctrl Pts',(7.90613690255562,-0.277950848421,21.3406735479447));
#218519=CARTESIAN_POINT('Ctrl Pts',(7.91115296726171,-0.125186150170402,
21.346944248329));
#218520=CARTESIAN_POINT('Ctrl Pts',(7.91213750945838,0.00932024328144952,
21.3526193068265));
#218521=CARTESIAN_POINT('Ctrl Pts',(7.90614283229866,0.339098544217776,
21.3668687812909));
#218522=CARTESIAN_POINT('Ctrl Pts',(7.89535918553394,0.534208544160177,
21.3755744605981));
#218523=CARTESIAN_POINT('Ctrl Pts',(7.82008525248643,1.34792127042609,21.4125761989884));
#218524=CARTESIAN_POINT('Ctrl Pts',(7.68998299482453,1.95828654873776,21.4418430210699));
#218525=CARTESIAN_POINT('Ctrl Pts',(7.44215809221688,2.68701369387939,21.4758850093446));
#218526=CARTESIAN_POINT('Ctrl Pts',(7.39066539022854,2.82556674690524,21.4823255384689));
#218527=CARTESIAN_POINT('Ctrl Pts',(7.25795223941161,3.15416098080264,21.4975009748971));
#218528=CARTESIAN_POINT('Ctrl Pts',(7.17310728029139,3.3426250522858,21.5061217722289));
#218529=CARTESIAN_POINT('Ctrl Pts',(7.07074562706712,3.54809861074902,21.5154322621857));
#218530=CARTESIAN_POINT('Ctrl Pts',(7.06042495053649,3.56859173949286,21.5163598899398));
#218531=CARTESIAN_POINT('Ctrl Pts',(7.04583066941112,3.59725954760483,21.5176562390892));
#218532=CARTESIAN_POINT('Ctrl Pts',(7.04163175115944,3.60547200191611,21.5180274526292));
#218533=CARTESIAN_POINT('Ctrl Pts',(7.03391631379916,3.62049735136443,21.5187063454141));
#218534=CARTESIAN_POINT('Ctrl Pts',(7.03040423742139,3.62731250923441,21.5190141729184));
#218535=CARTESIAN_POINT('Ctrl Pts',(7.02328139103339,3.64108513302807,21.5196360504375));
#218536=CARTESIAN_POINT('Ctrl Pts',(7.01967017629657,3.64804235995725,21.5199500850606));
#218537=CARTESIAN_POINT('Ctrl Pts',(7.01078166414746,3.66510455749891,21.5207199800449));
#218538=CARTESIAN_POINT('Ctrl Pts',(7.00549284638322,3.67520352366444,21.5211754526882));
#218539=CARTESIAN_POINT('Ctrl Pts',(6.98628572076714,3.71168731209647,21.522820122082));
#218540=CARTESIAN_POINT('Ctrl Pts',(6.97223995610578,3.73800493487893,21.5240050211915));
#218541=CARTESIAN_POINT('Ctrl Pts',(6.77323418734576,4.1058587991568,21.5405475024166));
#218542=CARTESIAN_POINT('Ctrl Pts',(6.56350895449849,4.43341489518475,21.5550076613076));
#218543=CARTESIAN_POINT('Ctrl Pts',(6.22168789434987,4.88952689931979,21.5754020176109));
#218544=CARTESIAN_POINT('Ctrl Pts',(6.10785520898122,5.03100193704645,21.5817745184293));
#218545=CARTESIAN_POINT('Ctrl Pts',(5.59836509279022,5.62140586373309,21.6089026258922));
#218546=CARTESIAN_POINT('Ctrl Pts',(5.15738317849322,6.02853070226537,21.6289019173298));
#218547=CARTESIAN_POINT('Ctrl Pts',(4.56738087035909,6.46070259543378,21.6565169059394));
#218548=CARTESIAN_POINT('Ctrl Pts',(4.4580095466773,6.53665028697409,21.6616741747669));
#218549=CARTESIAN_POINT('Ctrl Pts',(4.3358291913977,6.61699915025736,21.667521513679));
#218550=CARTESIAN_POINT('Ctrl Pts',(4.32486857210806,6.62416820154599,21.6680467173917));
#218551=CARTESIAN_POINT('Ctrl Pts',(4.30833723629718,6.63492239170158,21.668839766944));
#218552=CARTESIAN_POINT('Ctrl Pts',(4.30277969889074,6.63852782987389,21.6691065306222));
#218553=CARTESIAN_POINT('Ctrl Pts',(4.29315080803214,6.64475737716687,21.6695689791331));
#218554=CARTESIAN_POINT('Ctrl Pts',(4.28908155587205,6.64738473904073,21.6697644936162));
#218555=CARTESIAN_POINT('Ctrl Pts',(4.28088084104161,6.65266896461637,21.6701586680266));
#218556=CARTESIAN_POINT('Ctrl Pts',(4.27674931113416,6.65532572136908,21.6703573333893));
#218557=CARTESIAN_POINT('Ctrl Pts',(4.2669854063907,6.66159149831317,21.670827015911));
#218558=CARTESIAN_POINT('Ctrl Pts',(4.26135092825651,6.66519722248379,21.6710982005692));
#218559=CARTESIAN_POINT('Ctrl Pts',(4.24379508170847,6.67640053825089,21.6719435858687));
#218560=CARTESIAN_POINT('Ctrl Pts',(4.23185795831254,6.6839732988507,21.67251902463));
#218561=CARTESIAN_POINT('Ctrl Pts',(4.20409311340327,6.70148277240838,21.673858767274));
#218562=CARTESIAN_POINT('Ctrl Pts',(4.18825038624189,6.71139545468534,21.674624218095));
#218563=CARTESIAN_POINT('Ctrl Pts',(4.13464737154508,6.74467076771323,21.677217023411));
#218564=CARTESIAN_POINT('Ctrl Pts',(4.096725928947,6.76777136253398,21.679056210811));
#218565=CARTESIAN_POINT('Ctrl Pts',(3.93306181694111,6.86559099389532,21.6870084533196));
#218566=CARTESIAN_POINT('Ctrl Pts',(3.80545767316003,6.93713227803034,21.693244583989));
#218567=CARTESIAN_POINT('Ctrl Pts',(3.39165803013796,7.15427515994618,21.7134246878212));
#218568=CARTESIAN_POINT('Ctrl Pts',(3.09855336687518,7.28601129607747,21.7276409876623));
#218569=CARTESIAN_POINT('Ctrl Pts',(2.67733648573444,7.44530078542147,21.7474436822204));
#218570=CARTESIAN_POINT('Ctrl Pts',(2.55530986901585,7.48805892963322,21.7531121436162));
#218571=CARTESIAN_POINT('Ctrl Pts',(1.98449402256463,7.67249366139754,21.7792481226111));
#218572=CARTESIAN_POINT('Ctrl Pts',(1.52465808512055,7.77694379217276,21.7991410679494));
#218573=CARTESIAN_POINT('Ctrl Pts',(1.0201489788642,7.84504263121774,21.819763603688));
#218574=CARTESIAN_POINT('Ctrl Pts',(0.982027729137657,7.84990569340666,
21.8213151656408));
#218575=CARTESIAN_POINT('Ctrl Pts',(0.928442124823705,7.85634506313133,
21.8234872101291));
#218576=CARTESIAN_POINT('Ctrl Pts',(0.913006435558643,7.85815384048847,
21.8241118438224));
#218577=CARTESIAN_POINT('Ctrl Pts',(0.884662989579706,7.86139052840842,
21.8252569536541));
#218578=CARTESIAN_POINT('Ctrl Pts',(0.871756864853068,7.86283216246031,
21.8257776695716));
#218579=CARTESIAN_POINT('Ctrl Pts',(0.845566530484154,7.86569238675135,
21.8268329516179));
#218580=CARTESIAN_POINT('Ctrl Pts',(0.832282159000866,7.8671091189533,21.827367483916));
#218581=CARTESIAN_POINT('Ctrl Pts',(0.79948112043046,7.8705232243456,21.8286855563566));
#218582=CARTESIAN_POINT('Ctrl Pts',(0.779960466390587,7.87248166473394,
21.8294684297796));
#218583=CARTESIAN_POINT('Ctrl Pts',(0.709111220382261,7.87932362152865,
21.8323044430253));
#218584=CARTESIAN_POINT('Ctrl Pts',(0.657742007341309,7.88377796384483,
21.8343505708884));
#218585=CARTESIAN_POINT('Ctrl Pts',(0.376724601058868,7.90537987640605,
21.845491071166));
#218586=CARTESIAN_POINT('Ctrl Pts',(0.146450258908566,7.91299629948024,
21.8544215671859));
#218587=CARTESIAN_POINT('Ctrl Pts',(-0.200421085763858,7.90932021747925,
21.8676476024266));
#218588=CARTESIAN_POINT('Ctrl Pts',(-0.316967106070901,7.90550740842303,
21.8720537432554));
#218589=CARTESIAN_POINT('Ctrl Pts',(-0.517151172562729,7.89452424920726,
21.8795761263049));
#218590=CARTESIAN_POINT('Ctrl Pts',(-0.600836856155371,7.88859643479536,
21.8827070833749));
#218591=CARTESIAN_POINT('Ctrl Pts',(-1.25053454501037,7.83217689350823,
21.9069477716208));
#218592=CARTESIAN_POINT('Ctrl Pts',(-1.80968104960947,7.72216471960022,
21.9272913244381));
#218593=CARTESIAN_POINT('Ctrl Pts',(-2.50004311591564,7.50717574209895,
21.9549589576368));
#218594=CARTESIAN_POINT('Ctrl Pts',(-2.64651248707179,7.45680035530527,
21.9609908293334));
#218595=CARTESIAN_POINT('Ctrl Pts',(-2.80616993862786,7.3965924809871,21.9678198912855));
#218596=CARTESIAN_POINT('Ctrl Pts',(-2.82091956015657,7.39097983253615,
21.9684532046756));
#218597=CARTESIAN_POINT('Ctrl Pts',(-2.8429067380082,7.38253768467095,21.9694010138659));
#218598=CARTESIAN_POINT('Ctrl Pts',(-2.85015712998586,7.37974157545378,
21.9697141662333));
#218599=CARTESIAN_POINT('Ctrl Pts',(-2.86261719516203,7.3749152575768,21.9702533897646));
#218600=CARTESIAN_POINT('Ctrl Pts',(-2.86782886427353,7.37289019770988,
21.970479249917));
#218601=CARTESIAN_POINT('Ctrl Pts',(-2.8782718849754,7.36881968208915,21.9709324699893));
#218602=CARTESIAN_POINT('Ctrl Pts',(-2.88350321315181,7.36677417670083,
21.9711598318736));
#218603=CARTESIAN_POINT('Ctrl Pts',(-2.8957210378762,7.36198186814832,21.9716916073191));
#218604=CARTESIAN_POINT('Ctrl Pts',(-2.90270580484743,7.35923069118881,
21.9719962045549));
#218605=CARTESIAN_POINT('Ctrl Pts',(-2.92395406329744,7.3508264188931,21.9729246314419));
#218606=CARTESIAN_POINT('Ctrl Pts',(-2.93820498218206,7.34514178781756,
21.9735498083944));
#218607=CARTESIAN_POINT('Ctrl Pts',(-2.97071983690408,7.33206198215857,
21.9749820690807));
#218608=CARTESIAN_POINT('Ctrl Pts',(-2.98897281342758,7.32463997546764,
21.9757903374959));
#218609=CARTESIAN_POINT('Ctrl Pts',(-3.04801954040579,7.30037298803718,
21.9784192259412));
#218610=CARTESIAN_POINT('Ctrl Pts',(-3.08869958878179,7.2832550149435,21.9802524329248));
#218611=CARTESIAN_POINT('Ctrl Pts',(-3.23355635479727,7.22086810637651,
21.9868651796408));
#218612=CARTESIAN_POINT('Ctrl Pts',(-3.33689326115389,7.17369941602656,
21.9917432591517));
#218613=CARTESIAN_POINT('Ctrl Pts',(-3.57433433654651,7.05907790442507,
22.0032688331088));
#218614=CARTESIAN_POINT('Ctrl Pts',(-3.70760718041908,6.98999948138854,
22.009978359212));
#218615=CARTESIAN_POINT('Ctrl Pts',(-4.44805180757511,6.57907438202911,
22.0483145514951));
#218616=CARTESIAN_POINT('Ctrl Pts',(-5.01004795484847,6.16190158004555,
22.081180602425));
#218617=CARTESIAN_POINT('Ctrl Pts',(-5.67190883575128,5.51943960109531,
22.1209469098375));
#218618=CARTESIAN_POINT('Ctrl Pts',(-5.8269214456974,5.35553555400147,22.1303892209941));
#218619=CARTESIAN_POINT('Ctrl Pts',(-5.98893532557489,5.16885330000307,
22.1403979110106));
#218620=CARTESIAN_POINT('Ctrl Pts',(-6.00307430571377,5.15242560946019,
22.1412726493189));
#218621=CARTESIAN_POINT('Ctrl Pts',(-6.02286875612673,5.12923489982746,
22.1424991108452));
#218622=CARTESIAN_POINT('Ctrl Pts',(-6.02858064147224,5.12252029386454,
22.1428532354283));
#218623=CARTESIAN_POINT('Ctrl Pts',(-6.03848439037269,5.11083843532389,
22.1434676269019));
#218624=CARTESIAN_POINT('Ctrl Pts',(-6.042681372483,5.10587554447732,22.143728111207));
#218625=CARTESIAN_POINT('Ctrl Pts',(-6.05141168865918,5.09552618865137,
22.1442702056203));
#218626=CARTESIAN_POINT('Ctrl Pts',(-6.05594395947538,5.09013883159554,
22.1445517705512));
#218627=CARTESIAN_POINT('Ctrl Pts',(-6.06661712052576,5.07741757286198,
22.1452151706438));
#218628=CARTESIAN_POINT('Ctrl Pts',(-6.07275191935543,5.07007856182593,
22.1455967477419));
#218629=CARTESIAN_POINT('Ctrl Pts',(-6.09283736237928,5.04596175064919,
22.1468469112061));
#218630=CARTESIAN_POINT('Ctrl Pts',(-6.10673196254756,5.02913728796018,
22.1477131299382));
#218631=CARTESIAN_POINT('Ctrl Pts',(-6.36585216210786,4.71272087137329,
22.1638939762135));
#218632=CARTESIAN_POINT('Ctrl Pts',(-6.58883964426354,4.39557145677893,
22.1782317250367));
#218633=CARTESIAN_POINT('Ctrl Pts',(-6.93729561032466,3.81348254277342,
22.2021811773027));
#218634=CARTESIAN_POINT('Ctrl Pts',(-7.07295952013767,3.55555495991087,
22.2120748894831));
#218635=CARTESIAN_POINT('Ctrl Pts',(-7.2474591786569,3.17406896853133,22.2262007549969));
#218636=CARTESIAN_POINT('Ctrl Pts',(-7.29797665220492,3.05612747356098,
22.2305031063275));
#218637=CARTESIAN_POINT('Ctrl Pts',(-7.36995885857173,2.87609649184549,
22.2370292144113));
#218638=CARTESIAN_POINT('Ctrl Pts',(-7.39355527722465,2.81488275302091,
22.2392412197324));
#218639=CARTESIAN_POINT('Ctrl Pts',(-7.4412165755555,2.68650443489874,22.2438768850733));
#218640=CARTESIAN_POINT('Ctrl Pts',(-7.46513970607562,2.61929365303851,
22.2463019169655));
#218641=CARTESIAN_POINT('Ctrl Pts',(-7.59503562179923,2.23811488765928,
22.260085018354));
#218642=CARTESIAN_POINT('Ctrl Pts',(-7.68210037590923,1.91807806255168,
22.2717634104519));
#218643=CARTESIAN_POINT('Ctrl Pts',(-7.7651139198809,1.514415685093,22.2876004533614));
#218644=CARTESIAN_POINT('Ctrl Pts',(-7.78017528097231,1.43503337894554,
22.2907674527641));
#218645=CARTESIAN_POINT('Ctrl Pts',(-7.7958270788906,1.34503259471773,22.2944307451041));
#218646=CARTESIAN_POINT('Ctrl Pts',(-7.79761563129311,1.33462466233148,
22.2948554731086));
#218647=CARTESIAN_POINT('Ctrl Pts',(-7.80021236821219,1.31933033798389,
22.2954812524248));
#218648=CARTESIAN_POINT('Ctrl Pts',(-7.8010368192283,1.31444668007342,22.2956813176428));
#218649=CARTESIAN_POINT('Ctrl Pts',(-7.80248090540606,1.3058433828348,22.2960342015207));
#218650=CARTESIAN_POINT('Ctrl Pts',(-7.8031024689808,1.30212406406063,22.2961869023084));
#218651=CARTESIAN_POINT('Ctrl Pts',(-7.80437912373904,1.29445106270511,
22.2965022263383));
#218652=CARTESIAN_POINT('Ctrl Pts',(-7.80503387022686,1.29049732478725,
22.2966648707077));
#218653=CARTESIAN_POINT('Ctrl Pts',(-7.80634767573858,1.2825262332704,22.2969931107874));
#218654=CARTESIAN_POINT('Ctrl Pts',(-7.80700663630438,1.27850887911462,
22.2971587121941));
#218655=CARTESIAN_POINT('Ctrl Pts',(-7.80861084098274,1.26868135705134,
22.2975642343431));
#218656=CARTESIAN_POINT('Ctrl Pts',(-7.80955270070102,1.26287064509135,
22.2978043632079));
#218657=CARTESIAN_POINT('Ctrl Pts',(-7.81212187000328,1.24690761731703,
22.2984650047925));
#218658=CARTESIAN_POINT('Ctrl Pts',(-7.81373586890071,1.23675320373788,
22.2988863256342));
#218659=CARTESIAN_POINT('Ctrl Pts',(-7.8785311275676,0.823906228856935,
22.3160586058685));
#218660=CARTESIAN_POINT('Ctrl Pts',(-7.91050707665273,0.416979381960712,
22.3346078413317));
#218661=CARTESIAN_POINT('Ctrl Pts',(-7.91099434492025,0.00945910354153937,
22.35353228109));
#218662=CARTESIAN_POINT('',(-7.91099777923565,-0.00592764106740733,26.3576684917633));
#218663=CARTESIAN_POINT('Ctrl Pts',(-7.91099433110756,0.00947064855683299,
22.3535317449623));
#218664=CARTESIAN_POINT('Ctrl Pts',(-7.91132738906062,-0.268738342389904,
22.3664512181225));
#218665=CARTESIAN_POINT('Ctrl Pts',(-7.89698450830174,-0.546774875940983,
22.3795297055049));
#218666=CARTESIAN_POINT('Ctrl Pts',(-7.81067683996992,-1.37140734219466,
22.4179794102181));
#218667=CARTESIAN_POINT('Ctrl Pts',(-7.69624630752847,-1.91190848755121,
22.4426006476018));
#218668=CARTESIAN_POINT('Ctrl Pts',(-7.50905049898906,-2.49024260815374,
22.4675066381919));
#218669=CARTESIAN_POINT('Ctrl Pts',(-7.4909759876114,-2.5440964185709,22.4698133677065));
#218670=CARTESIAN_POINT('Ctrl Pts',(-7.46793898366663,-2.61036138445217,
22.4726367973827));
#218671=CARTESIAN_POINT('Ctrl Pts',(-7.46352330562275,-2.62295998636552,
22.4731729327037));
#218672=CARTESIAN_POINT('Ctrl Pts',(-7.4565282840326,-2.6427571624589,22.4740143648846));
#218673=CARTESIAN_POINT('Ctrl Pts',(-7.4539703687289,-2.64996324745637,
22.4743204254822));
#218674=CARTESIAN_POINT('Ctrl Pts',(-7.44940625728032,-2.66276223478934,
22.4748636477076));
#218675=CARTESIAN_POINT('Ctrl Pts',(-7.44740420235687,-2.66835660134912,
22.4751009569242));
#218676=CARTESIAN_POINT('Ctrl Pts',(-7.44276857606013,-2.68126413116127,
22.4756481866518));
#218677=CARTESIAN_POINT('Ctrl Pts',(-7.44013052332249,-2.68857568505004,
22.4759579467845));
#218678=CARTESIAN_POINT('Ctrl Pts',(-7.43286433995909,-2.70862184382663,
22.4768066156558));
#218679=CARTESIAN_POINT('Ctrl Pts',(-7.42821425161995,-2.72134849360274,
22.477344738817));
#218680=CARTESIAN_POINT('Ctrl Pts',(-7.40526974948067,-2.7836474321062,
22.4799757048829));
#218681=CARTESIAN_POINT('Ctrl Pts',(-7.38651147292415,-2.83304809266183,
22.4820519086078));
#218682=CARTESIAN_POINT('Ctrl Pts',(-7.06340291774898,-3.65893693661997,
22.5166048658313));
#218683=CARTESIAN_POINT('Ctrl Pts',(-6.63870925191398,-4.38257078431541,
22.5437330007848));
#218684=CARTESIAN_POINT('Ctrl Pts',(-6.01865014138278,-5.13613824041793,
22.5774624884684));
#218685=CARTESIAN_POINT('Ctrl Pts',(-5.92553770890973,-5.24328775650253,
22.582432497387));
#218686=CARTESIAN_POINT('Ctrl Pts',(-5.67722987213511,-5.51396260092418,
22.5956129595548));
#218687=CARTESIAN_POINT('Ctrl Pts',(-5.51784570028461,-5.67345456356453,
22.6040033871958));
#218688=CARTESIAN_POINT('Ctrl Pts',(-5.33339807097235,-5.84289449826277,
22.6139436891075));
#218689=CARTESIAN_POINT('Ctrl Pts',(-5.31483166165228,-5.8597880081408,
22.6149467645789));
#218690=CARTESIAN_POINT('Ctrl Pts',(-5.29232173829739,-5.88007471621918,
22.6161663415352));
#218691=CARTESIAN_POINT('Ctrl Pts',(-5.28845484371562,-5.88355278855391,
22.6163759682639));
#218692=CARTESIAN_POINT('Ctrl Pts',(-5.28166968987759,-5.88964359105746,
22.6167440017176));
#218693=CARTESIAN_POINT('Ctrl Pts',(-5.27875291078135,-5.89225797546792,
22.6169022773221));
#218694=CARTESIAN_POINT('Ctrl Pts',(-5.27286611912393,-5.89752657948172,
22.6172218492687));
#218695=CARTESIAN_POINT('Ctrl Pts',(-5.2698960413717,-5.90018072425938,
22.6173831513823));
#218696=CARTESIAN_POINT('Ctrl Pts',(-5.26417790232757,-5.9052828515783,
22.6176938260265));
#218697=CARTESIAN_POINT('Ctrl Pts',(-5.26143013410749,-5.90773116249542,
22.6178431729129));
#218698=CARTESIAN_POINT('Ctrl Pts',(-5.25494853323093,-5.91349827674835,
22.6181955928357));
#218699=CARTESIAN_POINT('Ctrl Pts',(-5.25121326738718,-5.91681545902874,
22.6183987907697));
#218700=CARTESIAN_POINT('Ctrl Pts',(-5.24015968957158,-5.92661311223877,
22.6190004006471));
#218701=CARTESIAN_POINT('Ctrl Pts',(-5.23283252833325,-5.933083539202,22.6193995779622));
#218702=CARTESIAN_POINT('Ctrl Pts',(-5.16887711538896,-5.98935028218625,
22.6228870068242));
#218703=CARTESIAN_POINT('Ctrl Pts',(-5.1115532387619,-6.03834664623039,
22.6260345904189));
#218704=CARTESIAN_POINT('Ctrl Pts',(-4.85634511740895,-6.25024203055892,
22.6401085514726));
#218705=CARTESIAN_POINT('Ctrl Pts',(-4.65132340335551,-6.40427867530036,
22.6515696164034));
#218706=CARTESIAN_POINT('Ctrl Pts',(-4.31640458046204,-6.63133343766325,
22.6700839250487));
#218707=CARTESIAN_POINT('Ctrl Pts',(-4.19128877325705,-6.71111231781684,
22.6769582579013));
#218708=CARTESIAN_POINT('Ctrl Pts',(-3.95980540012706,-6.84971625345231,
22.6895168430201));
#218709=CARTESIAN_POINT('Ctrl Pts',(-3.85418175622888,-6.90970002493307,
22.6951893485242));
#218710=CARTESIAN_POINT('Ctrl Pts',(-3.53040945581009,-7.08383610865673,
22.7123384211577));
#218711=CARTESIAN_POINT('Ctrl Pts',(-3.30826906055341,-7.19026336747525,
22.7237795881239));
#218712=CARTESIAN_POINT('Ctrl Pts',(-2.6264404055016,-7.47862786741661,
22.757540212062));
#218713=CARTESIAN_POINT('Ctrl Pts',(-2.15428626939292,-7.62805549178081,
22.779061854378));
#218714=CARTESIAN_POINT('Ctrl Pts',(-1.64987825024774,-7.73707304235151,
22.7999665991115));
#218715=CARTESIAN_POINT('Ctrl Pts',(-1.6285228339128,-7.74159614631759,
22.8008480398433));
#218716=CARTESIAN_POINT('Ctrl Pts',(-1.59753759557242,-7.74802497309539,
22.8021217653868));
#218717=CARTESIAN_POINT('Ctrl Pts',(-1.58792260845171,-7.75000123506068,
22.8025162910012));
#218718=CARTESIAN_POINT('Ctrl Pts',(-1.57112729135953,-7.75342077239019,
22.8032041878312));
#218719=CARTESIAN_POINT('Ctrl Pts',(-1.56394859953637,-7.75487197945635,
22.8034978103725));
#218720=CARTESIAN_POINT('Ctrl Pts',(-1.55006863493017,-7.7576578240465,
22.804064758424));
#218721=CARTESIAN_POINT('Ctrl Pts',(-1.54336763030362,-7.758993752156,22.8043381245707));
#218722=CARTESIAN_POINT('Ctrl Pts',(-1.52746527297408,-7.76214266754479,
22.8049860393772));
#218723=CARTESIAN_POINT('Ctrl Pts',(-1.51826240065996,-7.76394797992649,
22.8053603450488));
#218724=CARTESIAN_POINT('Ctrl Pts',(-1.48586203468725,-7.77024409547664,
22.806675881429));
#218725=CARTESIAN_POINT('Ctrl Pts',(-1.46264754907615,-7.77464735205636,
22.8076143475751));
#218726=CARTESIAN_POINT('Ctrl Pts',(-1.162051151145,-7.83026960456698,22.819714006432));
#218727=CARTESIAN_POINT('Ctrl Pts',(-0.88213145939188,-7.86672399444468,
22.8303965263708));
#218728=CARTESIAN_POINT('Ctrl Pts',(-0.0333197098617335,-7.93137844934754,
22.8615555816639));
#218729=CARTESIAN_POINT('Ctrl Pts',(0.537192307667847,-7.91323538274013,
22.8807452602072));
#218730=CARTESIAN_POINT('Ctrl Pts',(1.32534613161184,-7.80248588546917,
22.9086659873577));
#218731=CARTESIAN_POINT('Ctrl Pts',(1.54840399341934,-7.76129922206249,
22.9167483955407));
#218732=CARTESIAN_POINT('Ctrl Pts',(1.86762787828406,-7.68804585092992,
22.9289110069963));
#218733=CARTESIAN_POINT('Ctrl Pts',(1.96543774556981,-7.66362422208288,
22.9327201808654));
#218734=CARTESIAN_POINT('Ctrl Pts',(2.11932888064962,-7.62206012935536,
22.9388780328626));
#218735=CARTESIAN_POINT('Ctrl Pts',(2.17573375164834,-7.6061513192077,22.9411704718224));
#218736=CARTESIAN_POINT('Ctrl Pts',(2.2562860410519,-7.58246249392462,22.9444908655487));
#218737=CARTESIAN_POINT('Ctrl Pts',(2.28058185956919,-7.57519046191902,
22.9454984528267));
#218738=CARTESIAN_POINT('Ctrl Pts',(2.31774374827146,-7.56387247439887,
22.9470486152508));
#218739=CARTESIAN_POINT('Ctrl Pts',(2.33063526652272,-7.55991019413761,
22.9475880329004));
#218740=CARTESIAN_POINT('Ctrl Pts',(2.35456108315577,-7.55248944533344,
22.9485921839809));
#218741=CARTESIAN_POINT('Ctrl Pts',(2.36559806693217,-7.54903970716123,
22.9490565981438));
#218742=CARTESIAN_POINT('Ctrl Pts',(2.38355792865656,-7.54338288819076,
22.9498142311254));
#218743=CARTESIAN_POINT('Ctrl Pts',(2.39048542004355,-7.5411904400617,22.950106931292));
#218744=CARTESIAN_POINT('Ctrl Pts',(2.40387369609309,-7.53693294778547,
22.9506735021079));
#218745=CARTESIAN_POINT('Ctrl Pts',(2.41033486692504,-7.53486913191958,
22.950947329886));
#218746=CARTESIAN_POINT('Ctrl Pts',(2.42515992144219,-7.53011271895305,
22.9515765346064));
#218747=CARTESIAN_POINT('Ctrl Pts',(2.43352198247945,-7.52741449402307,
22.9519321035013));
#218748=CARTESIAN_POINT('Ctrl Pts',(2.45937478231427,-7.51902487017744,
22.9530334414548));
#218749=CARTESIAN_POINT('Ctrl Pts',(2.47685012242444,-7.51328641696531,
22.9537807788884));
#218750=CARTESIAN_POINT('Ctrl Pts',(2.61736879920439,-7.46660016049683,
22.9598126372424));
#218751=CARTESIAN_POINT('Ctrl Pts',(2.73940562435025,-7.4226944269035,22.9651901254188));
#218752=CARTESIAN_POINT('Ctrl Pts',(3.45187544104198,-7.1464019590393,22.997249073056));
#218753=CARTESIAN_POINT('Ctrl Pts',(4.01370845633387,-6.8466557446557,23.0249985431122));
#218754=CARTESIAN_POINT('Ctrl Pts',(4.90355710499443,-6.22436658576277,
23.0710227064924));
#218755=CARTESIAN_POINT('Ctrl Pts',(5.25060485734947,-5.93454101434495,
23.0897136441153));
#218756=CARTESIAN_POINT('Ctrl Pts',(5.70374150398613,-5.48508733076998,
23.1159220734153));
#218757=CARTESIAN_POINT('Ctrl Pts',(5.83172914427766,-5.3488117412613,23.1235548263573));
#218758=CARTESIAN_POINT('Ctrl Pts',(5.98510689699571,-5.17344562679096,
23.1329881348284));
#218759=CARTESIAN_POINT('Ctrl Pts',(6.01513867865191,-5.13849695233709,
23.1348498216447));
#218760=CARTESIAN_POINT('Ctrl Pts',(6.06051113683805,-5.0847531053173,23.1376851059365));
#218761=CARTESIAN_POINT('Ctrl Pts',(6.07607345793738,-5.06614653559885,
23.1386617317339));
#218762=CARTESIAN_POINT('Ctrl Pts',(6.10304677416558,-5.03359372238583,
23.1403617644181));
#218763=CARTESIAN_POINT('Ctrl Pts',(6.11449613974235,-5.01967953645452,
23.1410857019816));
#218764=CARTESIAN_POINT('Ctrl Pts',(6.14017397110136,-4.98825557072307,
23.1427145744411));
#218765=CARTESIAN_POINT('Ctrl Pts',(6.15437528153048,-4.97072378353024,
23.143619122286));
#218766=CARTESIAN_POINT('Ctrl Pts',(6.19237580854727,-4.92339891292325,
23.1460495831962));
#218767=CARTESIAN_POINT('Ctrl Pts',(6.21603498600845,-4.89349405654072,
23.14757349581));
#218768=CARTESIAN_POINT('Ctrl Pts',(6.3223519721031,-4.75709569759269,23.1544710592942));
#218769=CARTESIAN_POINT('Ctrl Pts',(6.40249642874486,-4.64867015571946,
23.1598080732728));
#218770=CARTESIAN_POINT('Ctrl Pts',(6.70804842033338,-4.21239488764495,
23.1807536819333));
#218771=CARTESIAN_POINT('Ctrl Pts',(6.9113618840989,-3.86978930538546,23.196027616382));
#218772=CARTESIAN_POINT('Ctrl Pts',(7.25369617879374,-3.17914186783272,
23.2256442515566));
#218773=CARTESIAN_POINT('Ctrl Pts',(7.39550028729147,-2.83365618355761,
23.2399565835744));
#218774=CARTESIAN_POINT('Ctrl Pts',(7.52190510346137,-2.45067023357923,
23.2560595967062));
#218775=CARTESIAN_POINT('Ctrl Pts',(7.53124576320613,-2.42181300279579,
23.2572744662538));
#218776=CARTESIAN_POINT('Ctrl Pts',(7.54444376636864,-2.38022398091136,
23.2590281694345));
#218777=CARTESIAN_POINT('Ctrl Pts',(7.54843533335873,-2.36753499649502,
23.2595636027704));
#218778=CARTESIAN_POINT('Ctrl Pts',(7.55526946954872,-2.34561665725087,
23.2604890854947));
#218779=CARTESIAN_POINT('Ctrl Pts',(7.55812718220442,-2.33639203843616,
23.2608787703606));
#218780=CARTESIAN_POINT('Ctrl Pts',(7.56407399149598,-2.31707080925271,
23.2616953422492));
#218781=CARTESIAN_POINT('Ctrl Pts',(7.5671597793045,-2.30697320261887,23.2621223054978));
#218782=CARTESIAN_POINT('Ctrl Pts',(7.57491374088395,-2.2814170109135,23.2632034130755));
#218783=CARTESIAN_POINT('Ctrl Pts',(7.57955480890161,-2.26595027651699,
23.2638581664163));
#218784=CARTESIAN_POINT('Ctrl Pts',(7.59676134431879,-2.20796374506986,
23.2663144912943));
#218785=CARTESIAN_POINT('Ctrl Pts',(7.60901656982578,-2.16535299909108,
23.2681226697767));
#218786=CARTESIAN_POINT('Ctrl Pts',(7.71692618155002,-1.77792552160713,
23.2845846814515));
#218787=CARTESIAN_POINT('Ctrl Pts',(7.78943845978878,-1.42709787813032,
23.2996300913183));
#218788=CARTESIAN_POINT('Ctrl Pts',(7.89177819041648,-0.679240925806107,
23.3313399115327));
#218789=CARTESIAN_POINT('Ctrl Pts',(7.9159203528083,-0.282401844542897,
23.3479481870861));
#218790=CARTESIAN_POINT('Ctrl Pts',(7.90874449395551,0.213007664597464,
23.3682922702164));
#218791=CARTESIAN_POINT('Ctrl Pts',(7.90548160012989,0.31140441566165,23.3723155235435));
#218792=CARTESIAN_POINT('Ctrl Pts',(7.89657317702969,0.483182091164209,
23.3793122201177));
#218793=CARTESIAN_POINT('Ctrl Pts',(7.89173857881504,0.556592493744786,
23.3822937120554));
#218794=CARTESIAN_POINT('Ctrl Pts',(7.88327634409368,0.662529156606506,
23.3865857192254));
#218795=CARTESIAN_POINT('Ctrl Pts',(7.88046975434703,0.695116725743285,
23.3879045656946));
#218796=CARTESIAN_POINT('Ctrl Pts',(7.87520742344474,0.752083336704774,
23.3902077937332));
#218797=CARTESIAN_POINT('Ctrl Pts',(7.87284037199482,0.776470082609166,
23.3911930542105));
#218798=CARTESIAN_POINT('Ctrl Pts',(7.86802560638372,0.823787498717093,
23.3931034680931));
#218799=CARTESIAN_POINT('Ctrl Pts',(7.86559084400334,0.846719235709332,
23.3940287398877));
#218800=CARTESIAN_POINT('Ctrl Pts',(7.85951754555579,0.90163239837388,23.3962431703346));
#218801=CARTESIAN_POINT('Ctrl Pts',(7.85578402149688,0.933602939070093,
23.3975313910599));
#218802=CARTESIAN_POINT('Ctrl Pts',(7.84125686170906,1.05173786091209,23.402288366475));
#218803=CARTESIAN_POINT('Ctrl Pts',(7.82923981079504,1.13774595282398,23.4057454188129));
#218804=CARTESIAN_POINT('Ctrl Pts',(7.71935605519007,1.83966906679815,23.4339394987534));
#218805=CARTESIAN_POINT('Ctrl Pts',(7.55037928510078,2.44227265188441,23.458062001236));
#218806=CARTESIAN_POINT('Ctrl Pts',(7.19784249574146,3.29622182712517,23.4926743723737));
#218807=CARTESIAN_POINT('Ctrl Pts',(7.06760844407218,3.5669210739248,23.5037563358507));
#218808=CARTESIAN_POINT('Ctrl Pts',(6.74681534517606,4.14678552794455,23.5284160059575));
#218809=CARTESIAN_POINT('Ctrl Pts',(6.54973407530411,4.45155026875225,23.5419993385837));
#218810=CARTESIAN_POINT('Ctrl Pts',(6.32232909439529,4.75524572731487,23.5570954889225));
#218811=CARTESIAN_POINT('Ctrl Pts',(6.31214742211871,4.76875266933936,23.5577703565172));
#218812=CARTESIAN_POINT('Ctrl Pts',(6.29382758189763,4.79289418736283,23.558982972903));
#218813=CARTESIAN_POINT('Ctrl Pts',(6.28570556507965,4.80354097186587,23.5595199990598));
#218814=CARTESIAN_POINT('Ctrl Pts',(6.27313985677971,4.81992634947665,23.5603500247477));
#218815=CARTESIAN_POINT('Ctrl Pts',(6.26871521381598,4.8256795629979,23.5606421387505));
#218816=CARTESIAN_POINT('Ctrl Pts',(6.26057668873738,4.83623173011331,23.5611791731473));
#218817=CARTESIAN_POINT('Ctrl Pts',(6.25686518756732,4.84103251871604,23.5614239804994));
#218818=CARTESIAN_POINT('Ctrl Pts',(6.24885271431672,4.85137196367426,23.5619522660716));
#218819=CARTESIAN_POINT('Ctrl Pts',(6.24454989634671,4.85690917835383,23.5622358333464));
#218820=CARTESIAN_POINT('Ctrl Pts',(6.23292294590525,4.87183068861322,23.5630017503862));
#218821=CARTESIAN_POINT('Ctrl Pts',(6.22558500218917,4.88120416358291,23.563484779959));
#218822=CARTESIAN_POINT('Ctrl Pts',(6.19155479585651,4.92447271948966,23.5657234046176));
#218823=CARTESIAN_POINT('Ctrl Pts',(6.16460703934914,4.95816521511221,23.5674919902993));
#218824=CARTESIAN_POINT('Ctrl Pts',(5.58340269139946,5.6727757620947,23.6055864171149));
#218825=CARTESIAN_POINT('Ctrl Pts',(4.91994584182078,6.25689846845801,23.6481654894897));
#218826=CARTESIAN_POINT('Ctrl Pts',(3.82910546589323,6.93447208857148,23.7055327940616));
#218827=CARTESIAN_POINT('Ctrl Pts',(3.46799611524375,7.12193899185499,23.7229781519623));
#218828=CARTESIAN_POINT('Ctrl Pts',(3.07089608888263,7.29068933387601,23.740493399286));
#218829=CARTESIAN_POINT('Ctrl Pts',(3.04769828864377,7.30041703656497,23.7415109537161));
#218830=CARTESIAN_POINT('Ctrl Pts',(3.0146217872346,7.3141021122818,23.7429538649886));
#218831=CARTESIAN_POINT('Ctrl Pts',(3.00478100220456,7.31815040559034,23.7433821545098));
#218832=CARTESIAN_POINT('Ctrl Pts',(2.98781577873539,7.32508955480979,23.7441187990631));
#218833=CARTESIAN_POINT('Ctrl Pts',(2.98069525068141,7.32798989741475,23.7444274594668));
#218834=CARTESIAN_POINT('Ctrl Pts',(2.96708430414006,7.33351080483567,23.7450164781509));
#218835=CARTESIAN_POINT('Ctrl Pts',(2.96059461652865,7.33613314419733,23.7452968933152));
#218836=CARTESIAN_POINT('Ctrl Pts',(2.9454310857152,7.34223699395543,23.745951102279));
#218837=CARTESIAN_POINT('Ctrl Pts',(2.93675452747391,7.34571175599954,23.7463246789888));
#218838=CARTESIAN_POINT('Ctrl Pts',(2.90693582103706,7.3575921860718,23.7476059472233));
#218839=CARTESIAN_POINT('Ctrl Pts',(2.8857634934038,7.36592205462879,23.7485112059678));
#218840=CARTESIAN_POINT('Ctrl Pts',(2.66855034729262,7.45030035004233,23.7577531097291));
#218841=CARTESIAN_POINT('Ctrl Pts',(2.46958072402386,7.51859793258854,23.7658376899532));
#218842=CARTESIAN_POINT('Ctrl Pts',(1.52842406226246,7.8002557065653,23.8025865928719));
#218843=CARTESIAN_POINT('Ctrl Pts',(0.760377522155833,7.91213087908242,
23.8279140890067));
#218844=CARTESIAN_POINT('Ctrl Pts',(-0.169589144134691,7.91075831512624,
23.8609782525965));
#218845=CARTESIAN_POINT('Ctrl Pts',(-0.327455181626436,7.90579709125895,
23.8666904079398));
#218846=CARTESIAN_POINT('Ctrl Pts',(-0.598038368836354,7.88917505253697,
23.8767828271517));
#218847=CARTESIAN_POINT('Ctrl Pts',(-0.710849436313869,7.87981118448368,
23.8810811160126));
#218848=CARTESIAN_POINT('Ctrl Pts',(-0.886189323553663,7.86146125168594,
23.8879480214623));
#218849=CARTESIAN_POINT('Ctrl Pts',(-0.9488761648537,7.85414147724108,23.8904412671906));
#218850=CARTESIAN_POINT('Ctrl Pts',(-1.02277277304069,7.8446151397523,23.893427198762));
#218851=CARTESIAN_POINT('Ctrl Pts',(-1.03407061448032,7.84313386334491,
23.8938849600546));
#218852=CARTESIAN_POINT('Ctrl Pts',(-1.051462083779,7.84081541163407,23.8945915055022));
#218853=CARTESIAN_POINT('Ctrl Pts',(-1.05755803322652,7.83999552544475,
23.8948395162447));
#218854=CARTESIAN_POINT('Ctrl Pts',(-1.06822465264976,7.83854823141273,
23.8952740997024));
#218855=CARTESIAN_POINT('Ctrl Pts',(-1.0727957469833,7.83792393238386,23.8954605354177));
#218856=CARTESIAN_POINT('Ctrl Pts',(-1.082388951832,7.8366051872511,23.895852214784));
#218857=CARTESIAN_POINT('Ctrl Pts',(-1.08741094490711,7.8359099114665,23.896057494488));
#218858=CARTESIAN_POINT('Ctrl Pts',(-1.10139481637611,7.8339601956773,23.8966297564365));
#218859=CARTESIAN_POINT('Ctrl Pts',(-1.11035519838549,7.83269520800184,
23.8969971917991));
#218860=CARTESIAN_POINT('Ctrl Pts',(-1.14619299851865,7.82757305199663,
23.8984697273036));
#218861=CARTESIAN_POINT('Ctrl Pts',(-1.17305245260442,7.82359292095127,
23.8995799857741));
#218862=CARTESIAN_POINT('Ctrl Pts',(-1.22570373306422,7.81551363400674,
23.9017687031059));
#218863=CARTESIAN_POINT('Ctrl Pts',(-1.251496848543,7.81142487782648,23.9028467441788));
#218864=CARTESIAN_POINT('Ctrl Pts',(-1.30055829169142,7.80339836456902,
23.9049078037622));
#218865=CARTESIAN_POINT('Ctrl Pts',(-1.32383022493121,7.79948404879771,
23.9058899611385));
#218866=CARTESIAN_POINT('Ctrl Pts',(-1.63020491389335,7.7465414150172,23.9188765796201));
#218867=CARTESIAN_POINT('Ctrl Pts',(-1.9104399982384,7.68223131036253,23.9313818707812));
#218868=CARTESIAN_POINT('Ctrl Pts',(-2.50861976885112,7.51019717499976,
23.9587146320488));
#218869=CARTESIAN_POINT('Ctrl Pts',(-2.82449353229944,7.3971940140238,23.973547315303));
#218870=CARTESIAN_POINT('Ctrl Pts',(-3.53457856870992,7.09102509063753,
24.0071303848532));
#218871=CARTESIAN_POINT('Ctrl Pts',(-3.92182102906554,6.88442095650999,
24.0255959998223));
#218872=CARTESIAN_POINT('Ctrl Pts',(-4.32328892044129,6.62530488812017,
24.0449582223639));
#218873=CARTESIAN_POINT('Ctrl Pts',(-4.35642848561461,6.60356137508039,
24.0465587818311));
#218874=CARTESIAN_POINT('Ctrl Pts',(-4.40395512192688,6.5718647445142,24.0488580404523));
#218875=CARTESIAN_POINT('Ctrl Pts',(-4.41847462132928,6.56211162353109,
24.0495609913981));
#218876=CARTESIAN_POINT('Ctrl Pts',(-4.44368807215542,6.54505347844184,
24.0507826534891));
#218877=CARTESIAN_POINT('Ctrl Pts',(-4.45439663674166,6.53777021024828,
24.0513018200204));
#218878=CARTESIAN_POINT('Ctrl Pts',(-4.47501688372335,6.52367148010543,
24.0523021403465));
#218879=CARTESIAN_POINT('Ctrl Pts',(-4.48493099847679,6.51685964477934,
24.0527833678447));
#218880=CARTESIAN_POINT('Ctrl Pts',(-4.50836697485973,6.50067833736237,
24.0539216309815));
#218881=CARTESIAN_POINT('Ctrl Pts',(-4.52187523571779,6.49128923871956,
24.0545782598247));
#218882=CARTESIAN_POINT('Ctrl Pts',(-4.56882156385422,6.45844090697395,
24.0568623133264));
#218883=CARTESIAN_POINT('Ctrl Pts',(-4.60210736080558,6.43476474350345,
24.058485385381));
#218884=CARTESIAN_POINT('Ctrl Pts',(-5.06245282324008,6.10192226358925,
24.0809878398833));
#218885=CARTESIAN_POINT('Ctrl Pts',(-5.45775693711108,5.75107127150145,
24.1008530284542));
#218886=CARTESIAN_POINT('Ctrl Pts',(-6.09593885443711,5.05913775650199,
24.1356063278963));
#218887=CARTESIAN_POINT('Ctrl Pts',(-6.35231153515151,4.73323008413558,
24.1506263207329));
#218888=CARTESIAN_POINT('Ctrl Pts',(-6.67058944218628,4.25589724918746,
24.172251464074));
#218889=CARTESIAN_POINT('Ctrl Pts',(-6.7551394000578,4.12037785277874,24.1783576106507));
#218890=CARTESIAN_POINT('Ctrl Pts',(-6.87257444266999,3.91880817894615,
24.1874961017926));
#218891=CARTESIAN_POINT('Ctrl Pts',(-6.90873163945283,3.85470669998232,
24.1904103737995));
#218892=CARTESIAN_POINT('Ctrl Pts',(-6.95033606793557,3.77848184844983,
24.1938940179655));
#218893=CARTESIAN_POINT('Ctrl Pts',(-6.95665433903014,3.76683646325639,
24.1944267344584));
#218894=CARTESIAN_POINT('Ctrl Pts',(-6.96630449608345,3.74894289212901,
24.1952461012844));
#218895=CARTESIAN_POINT('Ctrl Pts',(-6.96965731386259,3.74270598197403,
24.1955318503646));
#218896=CARTESIAN_POINT('Ctrl Pts',(-6.97573747076955,3.7313591743994,24.1960520052883));
#218897=CARTESIAN_POINT('Ctrl Pts',(-6.97846758255995,3.72625076295222,
24.1962862899482));
#218898=CARTESIAN_POINT('Ctrl Pts',(-6.98438646242607,3.71514641206537,
24.1967958044797));
#218899=CARTESIAN_POINT('Ctrl Pts',(-6.98757312319085,3.70914935898864,
24.1970711269789));
#218900=CARTESIAN_POINT('Ctrl Pts',(-6.99618478085933,3.69289239062106,
24.1978179068998));
#218901=CARTESIAN_POINT('Ctrl Pts',(-7.00159491556002,3.68262465275913,
24.1982900272373));
#218902=CARTESIAN_POINT('Ctrl Pts',(-7.02684730614991,3.63444207383412,
24.2005078078407));
#218903=CARTESIAN_POINT('Ctrl Pts',(-7.04640404639417,3.59637903504548,
24.2022664615881));
#218904=CARTESIAN_POINT('Ctrl Pts',(-7.43354843992086,2.8276032463904,24.2379501882632));
#218905=CARTESIAN_POINT('Ctrl Pts',(-7.68588528680803,2.04449707151529,
24.2775250345033));
#218906=CARTESIAN_POINT('Ctrl Pts',(-7.84264991007195,1.05402552909513,
24.3223631292469));
#218907=CARTESIAN_POINT('Ctrl Pts',(-7.86514854992047,0.870385593894323,
24.3304927693579));
#218908=CARTESIAN_POINT('Ctrl Pts',(-7.89796965140514,0.493381558045493,
24.3467494714145));
#218909=CARTESIAN_POINT('Ctrl Pts',(-7.90767381607238,0.300086478573789,
24.3548534681929));
#218910=CARTESIAN_POINT('Ctrl Pts',(-7.91075720999831,0.0713253403884549,
24.3641665519708));
#218911=CARTESIAN_POINT('Ctrl Pts',(-7.91099671319619,0.0360275876546984,
24.3655958226027));
#218912=CARTESIAN_POINT('Ctrl Pts',(-7.9110010339876,-0.0108545984166303,
24.3674840000062));
#218913=CARTESIAN_POINT('Ctrl Pts',(-7.91097665939552,-0.0224383175062282,
24.3679497094544));
#218914=CARTESIAN_POINT('Ctrl Pts',(-7.91089798963952,-0.0407309266759933,
24.3686838457705));
#218915=CARTESIAN_POINT('Ctrl Pts',(-7.91086060247442,-0.0474398501254188,
24.3689528193622));
#218916=CARTESIAN_POINT('Ctrl Pts',(-7.91077194961176,-0.0603915182460814,
24.3694715465466));
#218917=CARTESIAN_POINT('Ctrl Pts',(-7.91072182858753,-0.0666342644040845,
24.3697213370205));
#218918=CARTESIAN_POINT('Ctrl Pts',(-7.9105857155312,-0.0814090955993259,
24.3703119599698));
#218919=CARTESIAN_POINT('Ctrl Pts',(-7.91049330944747,-0.0899411219108776,
24.3706525843056));
#218920=CARTESIAN_POINT('Ctrl Pts',(-7.91018172436542,-0.114970912963646,
24.3716505551158));
#218921=CARTESIAN_POINT('Ctrl Pts',(-7.90992473654661,-0.131468208588591,
24.3723066743381));
#218922=CARTESIAN_POINT('Ctrl Pts',(-7.90762753838329,-0.254267512867061,
24.3771783845604));
#218923=CARTESIAN_POINT('Ctrl Pts',(-7.9034960842377,-0.360521898386537,
24.3813255566221));
#218924=CARTESIAN_POINT('Ctrl Pts',(-7.88314449914637,-0.704926385295538,
24.3945633691707));
#218925=CARTESIAN_POINT('Ctrl Pts',(-7.85828919467957,-0.942438342881225,
24.4033702667052));
#218926=CARTESIAN_POINT('Ctrl Pts',(-7.71671606965057,-1.88220173239001,
24.4373544792518));
#218927=CARTESIAN_POINT('Ctrl Pts',(-7.51624662197628,-2.56832884594178,
24.4599268898903));
#218928=CARTESIAN_POINT('Ctrl Pts',(-7.17719781653705,-3.32965359525488,
24.4891771430719));
#218929=CARTESIAN_POINT('Ctrl Pts',(-7.12507541791424,-3.43977618596408,
24.4935282994109));
#218930=CARTESIAN_POINT('Ctrl Pts',(-7.05036059614297,-3.58864023334215,
24.4996299904059));
#218931=CARTESIAN_POINT('Ctrl Pts',(-7.02994985643906,-3.62846085429612,
24.5012841251903));
#218932=CARTESIAN_POINT('Ctrl Pts',(-6.9961428240933,-3.69306104968029,
24.5040067631413));
#218933=CARTESIAN_POINT('Ctrl Pts',(-6.98294991928229,-3.71794630510182,
24.5050651435584));
#218934=CARTESIAN_POINT('Ctrl Pts',(-6.91670089662859,-3.84131268985399,
24.5103621487923));
#218935=CARTESIAN_POINT('Ctrl Pts',(-6.86169517737788,-3.9387271538288,
24.5147045104919));
#218936=CARTESIAN_POINT('Ctrl Pts',(-6.7987475960701,-4.04488390688901,
24.5196494793193));
#218937=CARTESIAN_POINT('Ctrl Pts',(-6.79282838898946,-4.05481653965159,
24.5201142466962));
#218938=CARTESIAN_POINT('Ctrl Pts',(-6.78448037250994,-4.0687552177949,
24.5207694511315));
#218939=CARTESIAN_POINT('Ctrl Pts',(-6.78206972209699,-4.07277218019092,
24.5209586226559));
#218940=CARTESIAN_POINT('Ctrl Pts',(-6.7778604288556,-4.07977219225579,
24.5212888889154));
#218941=CARTESIAN_POINT('Ctrl Pts',(-6.77606337913362,-4.08275620330591,
24.5214298716049));
#218942=CARTESIAN_POINT('Ctrl Pts',(-6.77230116043796,-4.08899406233144,
24.5217249948599));
#218943=CARTESIAN_POINT('Ctrl Pts',(-6.77033561655297,-4.09224768172471,
24.5218791619662));
#218944=CARTESIAN_POINT('Ctrl Pts',(-6.76565839999338,-4.09997741498914,
24.522245979107));
#218945=CARTESIAN_POINT('Ctrl Pts',(-6.76294465005449,-4.10445222273462,
24.522458778058));
#218946=CARTESIAN_POINT('Ctrl Pts',(-6.7537128175157,-4.11964093720143,
24.5231825865886));
#218947=CARTESIAN_POINT('Ctrl Pts',(-6.74717374176657,-4.13034196740307,
24.5236950902292));
#218948=CARTESIAN_POINT('Ctrl Pts',(-6.60494299565158,-4.36185985154354,
24.5348376621657));
#218949=CARTESIAN_POINT('Ctrl Pts',(-6.4585175107822,-4.57587379775202,
24.5462101414511));
#218950=CARTESIAN_POINT('Ctrl Pts',(-5.93362054323009,-5.26755675728417,
24.5855297558398));
#218951=CARTESIAN_POINT('Ctrl Pts',(-5.51055126598146,-5.7086709607868,
24.6147994608072));
#218952=CARTESIAN_POINT('Ctrl Pts',(-4.87736048201414,-6.23220413840931,
24.6519098357519));
#218953=CARTESIAN_POINT('Ctrl Pts',(-4.70831640251503,-6.36087882075856,
24.6612975136818));
#218954=CARTESIAN_POINT('Ctrl Pts',(-4.3667788710594,-6.59976904046135,
24.6791993648328));
#218955=CARTESIAN_POINT('Ctrl Pts',(-4.19478175087233,-6.71040416655264,
24.6877264794834));
#218956=CARTESIAN_POINT('Ctrl Pts',(-4.00099582124599,-6.82468863831104,
24.6968158363949));
#218957=CARTESIAN_POINT('Ctrl Pts',(-3.98326946681432,-6.83504988534656,
24.6976426710025));
#218958=CARTESIAN_POINT('Ctrl Pts',(-3.95822819708615,-6.84955627909286,
24.6988042682525));
#218959=CARTESIAN_POINT('Ctrl Pts',(-3.95094678555921,-6.85375890872563,
24.699141269475));
#218960=CARTESIAN_POINT('Ctrl Pts',(-3.93826734533509,-6.86105021077644,
24.6997267802067));
#218961=CARTESIAN_POINT('Ctrl Pts',(-3.93287235493141,-6.86414413588494,
24.6999754937399));
#218962=CARTESIAN_POINT('Ctrl Pts',(-3.92160884169991,-6.87058590952261,
24.7004938852152));
#218963=CARTESIAN_POINT('Ctrl Pts',(-3.91573966552925,-6.87393260947116,
24.7007635185039));
#218964=CARTESIAN_POINT('Ctrl Pts',(-3.90185570940555,-6.88182591547928,
24.7014002019519));
#218965=CARTESIAN_POINT('Ctrl Pts',(-3.89383725048185,-6.88636605006852,
24.7017670014679));
#218966=CARTESIAN_POINT('Ctrl Pts',(-3.86736958884071,-6.90129130566539,
24.7029747709186));
#218967=CARTESIAN_POINT('Ctrl Pts',(-3.84888655231765,-6.91161642014936,
24.7038134246));
#218968=CARTESIAN_POINT('Ctrl Pts',(-3.51538507314411,-7.09616654320072,
24.7188609830471));
#218969=CARTESIAN_POINT('Ctrl Pts',(-3.18886624465887,-7.2487709143762,
24.7322040924546));
#218970=CARTESIAN_POINT('Ctrl Pts',(-2.29074197388234,-7.59604483954615,
24.7663726598042));
#218971=CARTESIAN_POINT('Ctrl Pts',(-1.70546352257685,-7.74846582425057,
24.7859460246541));
#218972=CARTESIAN_POINT('Ctrl Pts',(-0.823835515641905,-7.87324068167831,
24.8173742432762));
#218973=CARTESIAN_POINT('Ctrl Pts',(-0.537129896616979,-7.89797987771685,
24.8279251577688));
#218974=CARTESIAN_POINT('Ctrl Pts',(-0.23228753765349,-7.90760826633078,
24.8400905462782));
#218975=CARTESIAN_POINT('Ctrl Pts',(-0.214830469100922,-7.90810178640301,
24.8407905137678));
#218976=CARTESIAN_POINT('Ctrl Pts',(-0.190997205769173,-7.9086965884587,
24.8417508054288));
#218977=CARTESIAN_POINT('Ctrl Pts',(-0.184622428222553,-7.90884797043401,
24.8420081098077));
#218978=CARTESIAN_POINT('Ctrl Pts',(-0.17448734722532,-7.90907638802005,
24.842417900949));
#218979=CARTESIAN_POINT('Ctrl Pts',(-0.170727147818328,-7.90915844997314,
24.8425700922576));
#218980=CARTESIAN_POINT('Ctrl Pts',(-0.163423864046552,-7.90931262495937,
24.8428659872182));
#218981=CARTESIAN_POINT('Ctrl Pts',(-0.159880786254882,-7.9093850388499,
24.8430096732791));
#218982=CARTESIAN_POINT('Ctrl Pts',(-0.151426390271033,-7.90955214777615,
24.8433528582454));
#218983=CARTESIAN_POINT('Ctrl Pts',(-0.146515034872999,-7.90964464906047,
24.8435524842301));
#218984=CARTESIAN_POINT('Ctrl Pts',(-0.131868276137306,-7.90990686195429,
24.8441485879744));
#218985=CARTESIAN_POINT('Ctrl Pts',(-0.122132673431918,-7.91006317392594,
24.8445458345057));
#218986=CARTESIAN_POINT('Ctrl Pts',(-0.0413583157847655,-7.91121090489695,
24.8478500366152));
#218987=CARTESIAN_POINT('Ctrl Pts',(0.0296885311668372,-7.91126326767768,
24.8508097437689));
#218988=CARTESIAN_POINT('Ctrl Pts',(0.371648363382786,-7.906909019316,24.8652814699334));
#218989=CARTESIAN_POINT('Ctrl Pts',(0.642197525837218,-7.88954328864179,
24.8774108105545));
#218990=CARTESIAN_POINT('Ctrl Pts',(1.37625939628521,-7.8044170626596,24.9112730609767));
#218991=CARTESIAN_POINT('Ctrl Pts',(1.83551795534609,-7.7093390018141,24.9334554800228));
#218992=CARTESIAN_POINT('Ctrl Pts',(2.77853646681446,-7.42501143978334,
24.9786338293376));
#218993=CARTESIAN_POINT('Ctrl Pts',(3.25762435748081,-7.22766042612521,
25.0013312415204));
#218994=CARTESIAN_POINT('Ctrl Pts',(3.74370540033309,-6.96919765749632,
25.0237430468356));
#218995=CARTESIAN_POINT('Ctrl Pts',(3.77322141090087,-6.95326156089598,
25.0251018893287));
#218996=CARTESIAN_POINT('Ctrl Pts',(3.81322953016855,-6.93133086134579,
25.0269411233938));
#218997=CARTESIAN_POINT('Ctrl Pts',(3.82381035852238,-6.92549935404854,
25.0274272878759));
#218998=CARTESIAN_POINT('Ctrl Pts',(3.84050402086261,-6.91624890530693,
25.0281939342265));
#218999=CARTESIAN_POINT('Ctrl Pts',(3.8466257233662,-6.91284605637047,25.0284749869321));
#219000=CARTESIAN_POINT('Ctrl Pts',(3.85843899920075,-6.90625890210985,
25.0290171873585));
#219001=CARTESIAN_POINT('Ctrl Pts',(3.86413116851248,-6.90307568018211,
25.0292783732753));
#219002=CARTESIAN_POINT('Ctrl Pts',(3.8775999230906,-6.89552169273847,25.0298962239147));
#219003=CARTESIAN_POINT('Ctrl Pts',(3.88537307210499,-6.89114480110596,
25.0302526703099));
#219004=CARTESIAN_POINT('Ctrl Pts',(3.9081764265212,-6.87825387826642,25.0312979690574));
#219005=CARTESIAN_POINT('Ctrl Pts',(3.9231862116198,-6.86970373076358,25.0319855342826));
#219006=CARTESIAN_POINT('Ctrl Pts',(4.03552598466638,-6.80522243701821,
25.037128148783));
#219007=CARTESIAN_POINT('Ctrl Pts',(4.13168575574991,-6.74727326121044,
25.0415105145102));
#219008=CARTESIAN_POINT('Ctrl Pts',(4.44411880129165,-6.54980570291558,
25.055710864306));
#219009=CARTESIAN_POINT('Ctrl Pts',(4.65482492530766,-6.40177812230887,
25.0652199786224));
#219010=CARTESIAN_POINT('Ctrl Pts',(5.37701547321621,-5.83987644079141,
25.0981283335534));
#219011=CARTESIAN_POINT('Ctrl Pts',(5.84365389425602,-5.37290148949582,
25.1198194011806));
#219012=CARTESIAN_POINT('Ctrl Pts',(6.3976392482897,-4.6598637118227,25.1526893801091));
#219013=CARTESIAN_POINT('Ctrl Pts',(6.53904646526501,-4.45925850621323,
25.1619795408695));
#219014=CARTESIAN_POINT('Ctrl Pts',(6.68068157045178,-4.23706787199869,
25.172490887677));
#219015=CARTESIAN_POINT('Ctrl Pts',(6.69038456697445,-4.22173006447441,
25.1732171561989));
#219016=CARTESIAN_POINT('Ctrl Pts',(6.70479050270604,-4.19878379033217,
25.1743045679438));
#219017=CARTESIAN_POINT('Ctrl Pts',(6.70953349436633,-4.1912004593394,25.1746640793592));
#219018=CARTESIAN_POINT('Ctrl Pts',(6.71766400599599,-4.17815182196231,
25.1752829159307));
#219019=CARTESIAN_POINT('Ctrl Pts',(6.72105774780615,-4.17269039052995,
25.1755419940517));
#219020=CARTESIAN_POINT('Ctrl Pts',(6.72767359490597,-4.1620147249433,25.1760485485514));
#219021=CARTESIAN_POINT('Ctrl Pts',(6.73089630644967,-4.1568008710797,25.1762960010598));
#219022=CARTESIAN_POINT('Ctrl Pts',(6.7386333945356,-4.14425085787144,25.1768917635437));
#219023=CARTESIAN_POINT('Ctrl Pts',(6.74314185086959,-4.13691106713021,
25.1772402992153));
#219024=CARTESIAN_POINT('Ctrl Pts',(6.75599510237946,-4.11590906949252,
25.1782378783861));
#219025=CARTESIAN_POINT('Ctrl Pts',(6.76431040387185,-4.10222891217102,
25.1788880171649));
#219026=CARTESIAN_POINT('Ctrl Pts',(6.78353065928454,-4.07039081930573,
25.1804017587042));
#219027=CARTESIAN_POINT('Ctrl Pts',(6.79440430851134,-4.05221417390089,
25.1812664640886));
#219028=CARTESIAN_POINT('Ctrl Pts',(6.89620295312634,-3.88048347883253,
25.1894395623873));
#219029=CARTESIAN_POINT('Ctrl Pts',(6.98197836194144,-3.72394168540918,
25.1969144766021));
#219030=CARTESIAN_POINT('Ctrl Pts',(7.22370856312189,-3.24501754425016,
25.2196534681444));
#219031=CARTESIAN_POINT('Ctrl Pts',(7.36314826699406,-2.91481557483264,
25.2351396661347));
#219032=CARTESIAN_POINT('Ctrl Pts',(7.6246787059487,-2.15551973768225,25.2696227997907));
#219033=CARTESIAN_POINT('Ctrl Pts',(7.73385175208269,-1.72323901142584,
25.2884709061032));
#219034=CARTESIAN_POINT('Ctrl Pts',(7.81128592684167,-1.25250003537469,
25.3083014889854));
#219035=CARTESIAN_POINT('Ctrl Pts',(7.81628638783297,-1.22090592641171,
25.3096294948078));
#219036=CARTESIAN_POINT('Ctrl Pts',(7.83278128558146,-1.11243028148906,
25.3141797041729));
#219037=CARTESIAN_POINT('Ctrl Pts',(7.84333412809913,-1.03540989707081,
25.3173942729427));
#219038=CARTESIAN_POINT('Ctrl Pts',(7.85505517872804,-0.939356833106798,
25.3213873915063));
#219039=CARTESIAN_POINT('Ctrl Pts',(7.85729202517308,-0.920459207756815,
25.3221722474698));
#219040=CARTESIAN_POINT('Ctrl Pts',(7.89079523881774,-0.62838875677535,
25.3342917221045));
#219041=CARTESIAN_POINT('Ctrl Pts',(7.90786791627459,-0.353769153556332,
25.3455618527819));
#219042=CARTESIAN_POINT('Ctrl Pts',(7.9110116725741,-0.0382375612866903,
25.3583364229323));
#219043=CARTESIAN_POINT('Ctrl Pts',(7.91110373604007,0.00234377887646953,
25.3599761443587));
#219044=CARTESIAN_POINT('Ctrl Pts',(7.9107452451188,0.0684133312128098,
25.3626405031876));
#219045=CARTESIAN_POINT('Ctrl Pts',(7.91048375170222,0.0939017384435331,
25.3636670958938));
#219046=CARTESIAN_POINT('Ctrl Pts',(7.90979642597227,0.139440589538119,
25.3654990239649));
#219047=CARTESIAN_POINT('Ctrl Pts',(7.90941752865496,0.159491499452698,
25.3663048544668));
#219048=CARTESIAN_POINT('Ctrl Pts',(7.90853838875326,0.198218546501772,
25.3678597925179));
#219049=CARTESIAN_POINT('Ctrl Pts',(7.90804822296554,0.216894776292699,
25.3686090045103));
#219050=CARTESIAN_POINT('Ctrl Pts',(7.90651131759177,0.268485012838611,
25.3706767930177));
#219051=CARTESIAN_POINT('Ctrl Pts',(7.90532521507062,0.301394547522225,
25.3719938198419));
#219052=CARTESIAN_POINT('Ctrl Pts',(7.89979268774025,0.43220303528134,25.377221003294));
#219053=CARTESIAN_POINT('Ctrl Pts',(7.89383285467975,0.530025611400865,
25.3811127331075));
#219054=CARTESIAN_POINT('Ctrl Pts',(7.87390853319274,0.780337998346133,
25.3910346037837));
#219055=CARTESIAN_POINT('Ctrl Pts',(7.85733155752323,0.932579664573326,
25.3970339355675));
#219056=CARTESIAN_POINT('Ctrl Pts',(7.79026180895559,1.41732372848122,25.4160852667382));
#219057=CARTESIAN_POINT('Ctrl Pts',(7.72298793484054,1.74712495566934,25.4289571672772));
#219058=CARTESIAN_POINT('Ctrl Pts',(7.60799596606838,2.17092139138167,25.4458421632243));
#219059=CARTESIAN_POINT('Ctrl Pts',(7.57912505558121,2.26966198404375,25.4498026946971));
#219060=CARTESIAN_POINT('Ctrl Pts',(7.47861211052378,2.59008687786884,25.4627866038761));
#219061=CARTESIAN_POINT('Ctrl Pts',(7.3991049333707,2.80916880410323,25.4718697677481));
#219062=CARTESIAN_POINT('Ctrl Pts',(7.30055450654627,3.04736636713169,25.4821799840283));
#219063=CARTESIAN_POINT('Ctrl Pts',(7.29095117871762,3.07027177693828,25.4831760112892));
#219064=CARTESIAN_POINT('Ctrl Pts',(7.27639059424223,3.10454743237777,25.4846736650364));
#219065=CARTESIAN_POINT('Ctrl Pts',(7.27151421404099,3.11595184069142,25.4851731616243));
#219066=CARTESIAN_POINT('Ctrl Pts',(7.26270688693184,3.13641630061166,25.4860715784433));
#219067=CARTESIAN_POINT('Ctrl Pts',(7.25878575188677,3.14548055847955,25.4864702544068));
#219068=CARTESIAN_POINT('Ctrl Pts',(7.25042886510551,3.1646998392054,25.4873171404528));
#219069=CARTESIAN_POINT('Ctrl Pts',(7.24598873004309,3.1748529294128,25.4877654557867));
#219070=CARTESIAN_POINT('Ctrl Pts',(7.2367136458911,3.1959411070766,25.4886985151989));
#219071=CARTESIAN_POINT('Ctrl Pts',(7.23187521101558,3.20687462862538,25.4891833400564));
#219072=CARTESIAN_POINT('Ctrl Pts',(7.21968788403927,3.23424675784679,25.4903997320156));
#219073=CARTESIAN_POINT('Ctrl Pts',(7.21230762943266,3.25067129811652,25.4911320063211));
#219074=CARTESIAN_POINT('Ctrl Pts',(7.19122012396466,3.29717557984885,25.4932119767452));
#219075=CARTESIAN_POINT('Ctrl Pts',(7.17738037253587,3.32719471070576,25.4945624994365));
#219076=CARTESIAN_POINT('Ctrl Pts',(7.13040926050307,3.42742051297302,25.4990968945706));
#219077=CARTESIAN_POINT('Ctrl Pts',(7.09643293789722,3.49722560515425,25.5022968751233));
#219078=CARTESIAN_POINT('Ctrl Pts',(6.89905909328302,3.88801077382679,25.5204268912399));
#219079=CARTESIAN_POINT('Ctrl Pts',(6.71491863070724,4.19803628041317,25.5356224760104));
#219080=CARTESIAN_POINT('Ctrl Pts',(6.26102576116218,4.85551158733953,25.5691307109213));
#219081=CARTESIAN_POINT('Ctrl Pts',(5.98213724346328,5.19523767141024,25.5873250646001));
#219082=CARTESIAN_POINT('Ctrl Pts',(5.64180254628225,5.54585147478261,25.6071460179521));
#219083=CARTESIAN_POINT('Ctrl Pts',(5.60675453475713,5.58128194753369,25.6091625982154));
#219084=CARTESIAN_POINT('Ctrl Pts',(5.54932589252839,5.63825040348392,25.612428075788));
#219085=CARTESIAN_POINT('Ctrl Pts',(5.52714918811681,5.65999181408121,25.613679874725));
#219086=CARTESIAN_POINT('Ctrl Pts',(5.48741104182905,5.69849368914344,25.6159068792057));
#219087=CARTESIAN_POINT('Ctrl Pts',(5.46989941444212,5.71530494964329,25.6168827838942));
#219088=CARTESIAN_POINT('Ctrl Pts',(5.43580929070604,5.74773146706245,25.6187721389096));
#219089=CARTESIAN_POINT('Ctrl Pts',(5.41924019706674,5.76335625763105,25.6196857115009));
#219090=CARTESIAN_POINT('Ctrl Pts',(5.37344623946958,5.80616824823389,25.6221978623551));
#219091=CARTESIAN_POINT('Ctrl Pts',(5.3440826764968,5.83320620071678,25.6237944544804));
#219092=CARTESIAN_POINT('Ctrl Pts',(5.21856725896904,5.94703747714062,25.6305605916497));
#219093=CARTESIAN_POINT('Ctrl Pts',(5.12049551279392,6.03168510548819,25.63570283005));
#219094=CARTESIAN_POINT('Ctrl Pts',(4.84751173979438,6.25584441242179,25.6496685255382));
#219095=CARTESIAN_POINT('Ctrl Pts',(4.66868724654889,6.39040860716263,25.6584572578504));
#219096=CARTESIAN_POINT('Ctrl Pts',(4.12999990742665,6.76107143248479,25.6838643756109));
#219097=CARTESIAN_POINT('Ctrl Pts',(3.75629536910645,6.97561832569681,25.7001173469114));
#219098=CARTESIAN_POINT('Ctrl Pts',(2.97448813217734,7.34332891031433,25.7322979591062));
#219099=CARTESIAN_POINT('Ctrl Pts',(2.56748357372203,7.49533592773626,25.7481729311362));
#219100=CARTESIAN_POINT('Ctrl Pts',(2.12909288786566,7.61914434672653,25.765608404051));
#219101=CARTESIAN_POINT('Ctrl Pts',(2.10807011184755,7.62498770477838,25.766445447061));
#219102=CARTESIAN_POINT('Ctrl Pts',(2.07485610043199,7.63407180229317,25.7677696747495));
#219103=CARTESIAN_POINT('Ctrl Pts',(2.0626807793214,7.63737049784182,25.7682554755917));
#219104=CARTESIAN_POINT('Ctrl Pts',(1.93201888412045,7.67243587284948,25.7734733836137));
#219105=CARTESIAN_POINT('Ctrl Pts',(1.81281960381764,7.70147080990682,25.7782723792714));
#219106=CARTESIAN_POINT('Ctrl Pts',(1.67816650034748,7.7309707475096,25.7837782190235));
#219107=CARTESIAN_POINT('Ctrl Pts',(1.66332669103334,7.73417712603138,25.7843861573076));
#219108=CARTESIAN_POINT('Ctrl Pts',(1.6408891442759,7.7389575537035,25.7853072005107));
#219109=CARTESIAN_POINT('Ctrl Pts',(1.6332981248773,7.74056318600747,25.7856191254138));
#219110=CARTESIAN_POINT('Ctrl Pts',(1.62010578458997,7.74333332471392,25.7861617881929));
#219111=CARTESIAN_POINT('Ctrl Pts',(1.61450553184268,7.74450292906741,25.7863923318706));
#219112=CARTESIAN_POINT('Ctrl Pts',(1.60283515662178,7.74692706051798,25.786873143356));
#219113=CARTESIAN_POINT('Ctrl Pts',(1.59676482068339,7.74818053012619,25.7871234517536));
#219114=CARTESIAN_POINT('Ctrl Pts',(1.58473221214955,7.75065041426796,25.7876200479722));
#219115=CARTESIAN_POINT('Ctrl Pts',(1.57876999645954,7.75186708647838,25.7878663254889));
#219116=CARTESIAN_POINT('Ctrl Pts',(1.55850792793213,7.75597749469947,25.7887040134404));
#219117=CARTESIAN_POINT('Ctrl Pts',(1.54420152863638,7.75883854032758,25.7892967219912));
#219118=CARTESIAN_POINT('Ctrl Pts',(1.43303820497962,7.78074975059871,25.7939123453743));
#219119=CARTESIAN_POINT('Ctrl Pts',(1.33585056127449,7.79802332907676,25.7980108877753));
#219120=CARTESIAN_POINT('Ctrl Pts',(1.15757886474194,7.8262776171013,25.8056603166599));
#219121=CARTESIAN_POINT('Ctrl Pts',(1.07660814816163,7.8378265084089,25.8091802656747));
#219122=CARTESIAN_POINT('Ctrl Pts',(0.672199605143743,7.88912271075981,
25.8269452543213));
#219123=CARTESIAN_POINT('Ctrl Pts',(0.346714494306063,7.91011236524295,
25.8418212189034));
#219124=CARTESIAN_POINT('Ctrl Pts',(-0.762587769734756,7.91304050343044,
25.8928548188322));
#219125=CARTESIAN_POINT('Ctrl Pts',(-1.54218521638967,7.79870718468197,
25.928803940738));
#219126=CARTESIAN_POINT('Ctrl Pts',(-2.33945362149577,7.55733450619418,
25.9629217045627));
#219127=CARTESIAN_POINT('Ctrl Pts',(-2.38647167787547,7.54261898322933,
25.9649257826575));
#219128=CARTESIAN_POINT('Ctrl Pts',(-2.44707373976049,7.52302858842245,
25.9674988724865));
#219129=CARTESIAN_POINT('Ctrl Pts',(-2.46078561606207,7.51855459410687,
25.9680803986936));
#219130=CARTESIAN_POINT('Ctrl Pts',(-2.48256298439458,7.51138298550722,
25.9690029442039));
#219131=CARTESIAN_POINT('Ctrl Pts',(-2.49063646393958,7.50870983135632,
25.9693447296601));
#219132=CARTESIAN_POINT('Ctrl Pts',(-2.50510756887577,7.50389249623141,
25.9699569488164));
#219133=CARTESIAN_POINT('Ctrl Pts',(-2.51150678521652,7.50175314141431,
25.9702275336683));
#219134=CARTESIAN_POINT('Ctrl Pts',(-2.52642560573334,7.49674432509508,
25.9708580320195));
#219135=CARTESIAN_POINT('Ctrl Pts',(-2.53494307892034,7.49386852062725,
25.9712177457458));
#219136=CARTESIAN_POINT('Ctrl Pts',(-2.55920276136945,7.48563148872873,
25.9722415821931));
#219137=CARTESIAN_POINT('Ctrl Pts',(-2.57493303335665,7.48023511907965,
25.972904597896));
#219138=CARTESIAN_POINT('Ctrl Pts',(-2.6736230633045,7.44603068221338,25.9770590351514));
#219139=CARTESIAN_POINT('Ctrl Pts',(-2.75611674817165,7.41589200748601,
25.9805082406233));
#219140=CARTESIAN_POINT('Ctrl Pts',(-2.99817894961433,7.32285852699981,
25.990569059474));
#219141=CARTESIAN_POINT('Ctrl Pts',(-3.15622612659897,7.25614047146743,
25.9970587151788));
#219142=CARTESIAN_POINT('Ctrl Pts',(-3.63297433729236,7.03635909971397,
26.0164988608652));
#219143=CARTESIAN_POINT('Ctrl Pts',(-3.94369551238686,6.86703249493978,
26.028961394301));
#219144=CARTESIAN_POINT('Ctrl Pts',(-4.36300585777615,6.60065392374823,
26.046204784009));
#219145=CARTESIAN_POINT('Ctrl Pts',(-4.48184204138811,6.52054786404915,
26.0511465462194));
#219146=CARTESIAN_POINT('Ctrl Pts',(-4.72759217015259,6.34499696529504,
26.0615801299753));
#219147=CARTESIAN_POINT('Ctrl Pts',(-4.85394016042886,6.24887015542638,
26.0670714218476));
#219148=CARTESIAN_POINT('Ctrl Pts',(-5.27998823258973,5.90400593195878,
26.0862774113004));
#219149=CARTESIAN_POINT('Ctrl Pts',(-5.56414345744967,5.63700504895694,
26.1003112359413));
#219150=CARTESIAN_POINT('Ctrl Pts',(-5.84507556421056,5.33101217609701,
26.1168001978018));
#219151=CARTESIAN_POINT('Ctrl Pts',(-5.86259256903854,5.31174241822961,
26.1178400730554));
#219152=CARTESIAN_POINT('Ctrl Pts',(-5.88597098729484,5.28576823434068,
26.1192433036034));
#219153=CARTESIAN_POINT('Ctrl Pts',(-5.89191683180774,5.27913973451568,
26.1196015370934));
#219154=CARTESIAN_POINT('Ctrl Pts',(-5.90120952902763,5.26874486774975,
26.1201635129317));
#219155=CARTESIAN_POINT('Ctrl Pts',(-5.9045640087252,5.26498530421748,26.1203668045862));
#219156=CARTESIAN_POINT('Ctrl Pts',(-5.9109851508513,5.25777489620911,26.1207567647896));
#219157=CARTESIAN_POINT('Ctrl Pts',(-5.91405238963775,5.25432456603907,
26.1209433996392));
#219158=CARTESIAN_POINT('Ctrl Pts',(-5.92123335290712,5.24623246237463,
26.1213811846904));
#219159=CARTESIAN_POINT('Ctrl Pts',(-5.92534463861371,5.24158853613927,
26.1216324746744));
#219160=CARTESIAN_POINT('Ctrl Pts',(-5.93382148014275,5.23199075311297,
26.1221519244846));
#219161=CARTESIAN_POINT('Ctrl Pts',(-5.93818630295439,5.22703625679943,
26.1224201253125));
#219162=CARTESIAN_POINT('Ctrl Pts',(-5.94941777341498,5.21425522611201,
26.1231121250301));
#219163=CARTESIAN_POINT('Ctrl Pts',(-5.9562751689613,5.20642060496903,26.1235364346771));
#219164=CARTESIAN_POINT('Ctrl Pts',(-6.03733137419294,5.11344361171303,
26.1285731150626));
#219165=CARTESIAN_POINT('Ctrl Pts',(-6.10971212216422,5.02673770224553,
26.1332818418867));
#219166=CARTESIAN_POINT('Ctrl Pts',(-6.33177819953746,4.74883738029606,
26.1483337765984));
#219167=CARTESIAN_POINT('Ctrl Pts',(-6.47453002333946,4.55228792647149,
26.1589176161616));
#219168=CARTESIAN_POINT('Ctrl Pts',(-6.66606623623699,4.26129453619557,
26.1742173467374));
#219169=CARTESIAN_POINT('Ctrl Pts',(-6.72234803544436,4.17194282919486,
26.1788688094947));
#219170=CARTESIAN_POINT('Ctrl Pts',(-6.83269232072961,3.98872946052635,
26.188288692328));
#219171=CARTESIAN_POINT('Ctrl Pts',(-6.8866500855219,3.89482962872367,26.1930560808351));
#219172=CARTESIAN_POINT('Ctrl Pts',(-7.20699677688648,3.30986522013551,
26.2223230969753));
#219173=CARTESIAN_POINT('Ctrl Pts',(-7.42269418079283,2.79279882790139,
26.2461706717191));
#219174=CARTESIAN_POINT('Ctrl Pts',(-7.59215920201566,2.22357298943364,
26.2702337829383));
#219175=CARTESIAN_POINT('Ctrl Pts',(-7.60197058740697,2.18979483068414,
26.271654539089));
#219176=CARTESIAN_POINT('Ctrl Pts',(-7.61621293849822,2.13951242682499,
26.2737592458376));
#219177=CARTESIAN_POINT('Ctrl Pts',(-7.62081619405549,2.12305758004906,
26.2744463853379));
#219178=CARTESIAN_POINT('Ctrl Pts',(-7.6286135052345,2.0948330981062,26.2756222905566));
#219179=CARTESIAN_POINT('Ctrl Pts',(-7.63183371639946,2.08307077348754,
26.2761115307317));
#219180=CARTESIAN_POINT('Ctrl Pts',(-7.63839210264199,2.05889589331696,
26.2771154216151));
#219181=CARTESIAN_POINT('Ctrl Pts',(-7.64172725101118,2.04648255196108,
26.2776300167359));
#219182=CARTESIAN_POINT('Ctrl Pts',(-7.64827046578289,2.02188983603875,
26.2786477888843));
#219183=CARTESIAN_POINT('Ctrl Pts',(-7.65147972925777,2.00971082014847,
26.2791509856662));
#219184=CARTESIAN_POINT('Ctrl Pts',(-7.65881483943904,1.98160213714104,
26.2803104571856));
#219185=CARTESIAN_POINT('Ctrl Pts',(-7.66292009964485,1.96566714461528,
26.2809663736341));
#219186=CARTESIAN_POINT('Ctrl Pts',(-7.67339531350322,1.92447495656088,
26.2826584137667));
#219187=CARTESIAN_POINT('Ctrl Pts',(-7.67969031752528,1.89919881307823,
26.2836932852363));
#219188=CARTESIAN_POINT('Ctrl Pts',(-7.68648670856122,1.87132308026282,
26.2848309425881));
#219189=CARTESIAN_POINT('Ctrl Pts',(-7.68711174881307,1.86875385026542,
26.2849357631341));
#219190=CARTESIAN_POINT('Ctrl Pts',(-7.83651897519375,1.25327164182394,
26.3100382812323));
#219191=CARTESIAN_POINT('Ctrl Pts',(-7.91147323817745,0.624771831188963,
26.3334951089523));
#219192=CARTESIAN_POINT('Ctrl Pts',(-7.91099775207325,-0.00596378169342535,
26.3566855201154));
#219193=CARTESIAN_POINT('',(-7.91915402201384,0.00415711932536667,28.3576688734072));
#219194=CARTESIAN_POINT('Ctrl Pts',(-7.91099777923565,-0.00592764106740734,
26.3576684917633));
#219195=CARTESIAN_POINT('Ctrl Pts',(-7.91081234552831,-0.253406466168664,
26.367633558589));
#219196=CARTESIAN_POINT('Ctrl Pts',(-7.89901033771747,-0.500480502849058,
26.3775986254146));
#219197=CARTESIAN_POINT('Ctrl Pts',(-7.87572819848802,-0.74620797606343,
26.3875636922403));
#219198=CARTESIAN_POINT('Ctrl Pts',(-7.85216115441233,-0.994942430177823,
26.3976507021487));
#219199=CARTESIAN_POINT('Ctrl Pts',(-7.81683130210497,-1.24229732251291,
26.4077377120572));
#219200=CARTESIAN_POINT('Ctrl Pts',(-7.76993023616728,-1.48731473639357,
26.4178247219656));
#219201=CARTESIAN_POINT('Ctrl Pts',(-7.73756601590349,-1.65638973272377,
26.4247852932011));
#219202=CARTESIAN_POINT('Ctrl Pts',(-7.69969293076519,-1.82435207936941,
26.4317458644366));
#219203=CARTESIAN_POINT('Ctrl Pts',(-7.65638765302037,-1.99089153563854,
26.4387064356721));
#219204=CARTESIAN_POINT('Ctrl Pts',(-7.60718904108376,-2.18009503479169,
26.4466142580186));
#219205=CARTESIAN_POINT('Ctrl Pts',(-7.55090996100215,-2.36771584605453,
26.4545220803651));
#219206=CARTESIAN_POINT('Ctrl Pts',(-7.48766754116812,-2.55318542079053,
26.4624299027117));
#219207=CARTESIAN_POINT('Ctrl Pts',(-7.42448973161223,-2.73846551446555,
26.470329646199));
#219208=CARTESIAN_POINT('Ctrl Pts',(-7.35436286296112,-2.92159842557277,
26.4782293896864));
#219209=CARTESIAN_POINT('Ctrl Pts',(-7.2774547056937,-3.10202740261537,
26.4861291331738));
#219210=CARTESIAN_POINT('Ctrl Pts',(-7.20061083918178,-3.28230555150578,
26.4940222729342));
#219211=CARTESIAN_POINT('Ctrl Pts',(-7.11699711146742,-3.45988395371757,
26.5019154126945));
#219212=CARTESIAN_POINT('Ctrl Pts',(-7.02683065685917,-3.63422232669165,
26.5098085524549));
#219213=CARTESIAN_POINT('Ctrl Pts',(-6.93672283807322,-3.80844732630642,
26.5176965592559));
#219214=CARTESIAN_POINT('Ctrl Pts',(-6.8400709403987,-3.97943618940445,
26.525584566057));
#219215=CARTESIAN_POINT('Ctrl Pts',(-6.73713974615048,-4.14666963246887,
26.5334725728581));
#219216=CARTESIAN_POINT('Ctrl Pts',(-6.63425638483063,-4.31382536084861,
26.5413569140409));
#219217=CARTESIAN_POINT('Ctrl Pts',(-6.52509972210309,-4.4772288536476,
26.5492412552237));
#219218=CARTESIAN_POINT('Ctrl Pts',(-6.40998005051429,-4.63638617373584,
26.5571255964065));
#219219=CARTESIAN_POINT('Ctrl Pts',(-6.29489251299128,-4.79549906725715,
26.5650077367844));
#219220=CARTESIAN_POINT('Ctrl Pts',(-6.17384548610093,-4.95036787126117,
26.5728898771623));
#219221=CARTESIAN_POINT('Ctrl Pts',(-6.04719223232534,-5.10052812023462,
26.5807720175402));
#219222=CARTESIAN_POINT('Ctrl Pts',(-5.92052512983102,-5.25070478826553,
26.5886550197795));
#219223=CARTESIAN_POINT('Ctrl Pts',(-5.78825079265693,-5.39617160433021,
26.5965380220188));
#219224=CARTESIAN_POINT('Ctrl Pts',(-5.65076277685022,-5.53649718141028,
26.604421024258));
#219225=CARTESIAN_POINT('Ctrl Pts',(-5.51325817951605,-5.67683968223746,
26.6123049772145));
#219226=CARTESIAN_POINT('Ctrl Pts',(-5.3705388916713,-5.81203946154334,
26.6201889301709));
#219227=CARTESIAN_POINT('Ctrl Pts',(-5.22303531337968,-5.94170203857353,
26.6280728831274));
#219228=CARTESIAN_POINT('Ctrl Pts',(-5.07548913974285,-6.07140205891387,
26.6359591127723));
#219229=CARTESIAN_POINT('Ctrl Pts',(-4.92315618161962,-6.1955614627831,
26.6438453424172));
#219230=CARTESIAN_POINT('Ctrl Pts',(-4.76650006527091,-6.31382595006961,
26.6517315720621));
#219231=CARTESIAN_POINT('Ctrl Pts',(-4.6097723648779,-6.43214447833769,
26.6596214053213));
#219232=CARTESIAN_POINT('Ctrl Pts',(-4.44871784480252,-6.54456251467399,
26.6675112385805));
#219233=CARTESIAN_POINT('Ctrl Pts',(-4.2838294423279,-6.65076885097089,
26.6754010718397));
#219234=CARTESIAN_POINT('Ctrl Pts',(-4.11875088072907,-6.75709767073899,
26.6833000041244));
#219235=CARTESIAN_POINT('Ctrl Pts',(-3.94982989526002,-6.85720029469113,
26.6911989364091));
#219236=CARTESIAN_POINT('Ctrl Pts',(-3.77758538490002,-6.950810719606,26.6990978686937));
#219237=CARTESIAN_POINT('Ctrl Pts',(-3.60522710960576,-7.04448297281262,
26.7070020181056));
#219238=CARTESIAN_POINT('Ctrl Pts',(-3.42954124134811,-7.13165432588132,
26.7149061675174));
#219239=CARTESIAN_POINT('Ctrl Pts',(-3.25106724206579,-7.21210668165459,
26.7228103169293));
#219240=CARTESIAN_POINT('Ctrl Pts',(-3.07234865061488,-7.29266929447507,
26.7307252986924));
#219241=CARTESIAN_POINT('Ctrl Pts',(-2.8908346144224,-7.36649438832649,
26.7386402804554));
#219242=CARTESIAN_POINT('Ctrl Pts',(-2.7070814610296,-7.43341314359358,
26.7465552622185));
#219243=CARTESIAN_POINT('Ctrl Pts',(-2.62923165918707,-7.46176428609592,
26.7499085639196));
#219244=CARTESIAN_POINT('Ctrl Pts',(-2.55098010369695,-7.48887641831373,
26.7532618656206));
#219245=CARTESIAN_POINT('Ctrl Pts',(-2.47236966538338,-7.51473946572282,
26.7566151673216));
#219246=CARTESIAN_POINT('Ctrl Pts',(-2.29044769764609,-7.57459228650951,
26.7643754502682));
#219247=CARTESIAN_POINT('Ctrl Pts',(-2.10603030035296,-7.62794040411383,
26.7721357332148));
#219248=CARTESIAN_POINT('Ctrl Pts',(-1.91963366571878,-7.67456367420579,
26.7798960161614));
#219249=CARTESIAN_POINT('Ctrl Pts',(-1.73346136875843,-7.72113083085998,
26.7876469592193));
#219250=CARTESIAN_POINT('Ctrl Pts',(-1.54531491949835,-7.76098916388463,
26.7953979022772));
#219251=CARTESIAN_POINT('Ctrl Pts',(-1.35572989318385,-7.79396673438678,
26.8031488453351));
#219252=CARTESIAN_POINT('Ctrl Pts',(-1.16633456185022,-7.82691130819226,
26.8108920329545));
#219253=CARTESIAN_POINT('Ctrl Pts',(-0.975503869297573,-7.85298876381602,
26.818635220574));
#219254=CARTESIAN_POINT('Ctrl Pts',(-0.783788036871119,-7.87207706474331,
26.8263784081935));
#219255=CARTESIAN_POINT('Ctrl Pts',(-0.592225175822845,-7.89115013498432,
26.8341154174704));
#219256=CARTESIAN_POINT('Ctrl Pts',(-0.399778936164906,-7.90324511807012,
26.8418524267473));
#219257=CARTESIAN_POINT('Ctrl Pts',(-0.207009301238635,-7.90829110169831,
26.8495894360243));
#219258=CARTESIAN_POINT('Ctrl Pts',(-0.0143544498463088,-7.91333408072552,
26.857321838345));
#219259=CARTESIAN_POINT('Ctrl Pts',(0.178623055672807,-7.91133640881237,
26.8650542406657));
#219260=CARTESIAN_POINT('Ctrl Pts',(0.371358452897015,-7.9022790319921,
26.8727866429865));
#219261=CARTESIAN_POINT('Ctrl Pts',(0.564018081156201,-7.8932252158466,
26.8805160055121));
#219262=CARTESIAN_POINT('Ctrl Pts',(0.756435432608975,-7.87711723920013,
26.8882453680377));
#219263=CARTESIAN_POINT('Ctrl Pts',(0.948045998137956,-7.85398814523008,
26.8959747305633));
#219264=CARTESIAN_POINT('Ctrl Pts',(1.139656488908,-7.83085906028409,26.9037040900732));
#219265=CARTESIAN_POINT('Ctrl Pts',(1.33045983660178,-7.80070889512595,
26.9114334495831));
#219266=CARTESIAN_POINT('Ctrl Pts',(1.51989649849299,-7.76362258445558,
26.919162809093));
#219267=CARTESIAN_POINT('Ctrl Pts',(1.70934265562977,-7.72653441488618,
26.9268925560261));
#219268=CARTESIAN_POINT('Ctrl Pts',(1.89742163769622,-7.6825094755353,26.9346223029593));
#219269=CARTESIAN_POINT('Ctrl Pts',(2.08358411429359,-7.63168384032406,
26.9423520498924));
#219270=CARTESIAN_POINT('Ctrl Pts',(2.26979003381491,-7.58084634442937,
26.9500836006413));
#219271=CARTESIAN_POINT('Ctrl Pts',(2.45407821066096,-7.52320508683273,
26.9578151513902));
#219272=CARTESIAN_POINT('Ctrl Pts',(2.63591444857681,-7.45894603947394,
26.9655467021391));
#219273=CARTESIAN_POINT('Ctrl Pts',(2.81782644965242,-7.39466021819744,
26.9732814742851));
#219274=CARTESIAN_POINT('Ctrl Pts',(2.99728413916984,-7.32375123608585,
26.981016246431));
#219275=CARTESIAN_POINT('Ctrl Pts',(3.17377322716514,-7.24645323606865,
26.9887510185769));
#219276=CARTESIAN_POINT('Ctrl Pts',(3.35047277848795,-7.16906305814698,
26.9964950144426));
#219277=CARTESIAN_POINT('Ctrl Pts',(3.52419632934816,-7.08526879055788,
27.0042390103082));
#219278=CARTESIAN_POINT('Ctrl Pts',(3.69445320748985,-6.9953510632182,27.0119830061739));
#219279=CARTESIAN_POINT('Ctrl Pts',(3.86482059088637,-6.90537497476276,
27.0197320282813));
#219280=CARTESIAN_POINT('Ctrl Pts',(4.03171650970528,-6.80926768825034,
27.0274810503888));
#219281=CARTESIAN_POINT('Ctrl Pts',(4.19467935553526,-6.70735313698677,
27.0352300724962));
#219282=CARTESIAN_POINT('Ctrl Pts',(4.35789124698183,-6.60528283628148,
27.0429909369348));
#219283=CARTESIAN_POINT('Ctrl Pts',(4.51715776493355,-6.49738774639976,
27.0507518013734));
#219284=CARTESIAN_POINT('Ctrl Pts',(4.6720495024886,-6.38403277296538,27.0585126658121));
#219285=CARTESIAN_POINT('Ctrl Pts',(4.7785671781947,-6.30607956196428,27.0638497435318));
#219286=CARTESIAN_POINT('Ctrl Pts',(4.88301665375285,-6.22554509245537,
27.0691868212515));
#219287=CARTESIAN_POINT('Ctrl Pts',(4.98526863013735,-6.14255791062392,
27.0745238989712));
#219288=CARTESIAN_POINT('Ctrl Pts',(5.13880338537601,-6.01794988737626,
27.0825376992942));
#219289=CARTESIAN_POINT('Ctrl Pts',(5.28785309562113,-5.88742820012953,
27.0905514996173));
#219290=CARTESIAN_POINT('Ctrl Pts',(5.43194002709184,-5.7513431946005,27.0985652999404));
#219291=CARTESIAN_POINT('Ctrl Pts',(5.5758627164689,-5.6154133099141,27.106569965477));
#219292=CARTESIAN_POINT('Ctrl Pts',(5.71483365802107,-5.47393297085151,
27.1145746310137));
#219293=CARTESIAN_POINT('Ctrl Pts',(5.84840691621087,-5.3272936414672,27.1225792965504));
#219294=CARTESIAN_POINT('Ctrl Pts',(5.98185059292036,-5.18079656916062,
27.1305761966374));
#219295=CARTESIAN_POINT('Ctrl Pts',(6.1099067975314,-5.02915072602463,27.1385730967244));
#219296=CARTESIAN_POINT('Ctrl Pts',(6.23216501251044,-4.87278567729392,
27.1465699968114));
#219297=CARTESIAN_POINT('Ctrl Pts',(6.35432536491272,-4.71654579223084,
27.1545604957151));
#219298=CARTESIAN_POINT('Ctrl Pts',(6.47069677235522,-4.55559449279696,
27.1625509946188));
#219299=CARTESIAN_POINT('Ctrl Pts',(6.58090746171654,-4.3903961074513,27.1705414935225));
#219300=CARTESIAN_POINT('Ctrl Pts',(6.69104862015278,-4.22530194426977,
27.1785269512928));
#219301=CARTESIAN_POINT('Ctrl Pts',(6.79503662284419,-4.0559663136662,27.1865124090632));
#219302=CARTESIAN_POINT('Ctrl Pts',(6.89254144589137,-3.88288467723028,
27.1944978668335));
#219303=CARTESIAN_POINT('Ctrl Pts',(6.9932432187942,-3.70412810805434,27.202745148658));
#219304=CARTESIAN_POINT('Ctrl Pts',(7.08702923843833,-3.52137600817342,
27.2109924304824));
#219305=CARTESIAN_POINT('Ctrl Pts',(7.17358526280352,-3.33520546252973,
27.2192397123069));
#219306=CARTESIAN_POINT('Ctrl Pts',(7.25733666092416,-3.15506729651651,
27.2272197620904));
#219307=CARTESIAN_POINT('Ctrl Pts',(7.33431911353444,-2.97172907265719,
27.2351998118739));
#219308=CARTESIAN_POINT('Ctrl Pts',(7.40429523026887,-2.78573745048194,
27.2431798616573));
#219309=CARTESIAN_POINT('Ctrl Pts',(7.47426579002794,-2.5997605983584,27.2511592777254));
#219310=CARTESIAN_POINT('Ctrl Pts',(7.53723100496438,-2.41113108097571,
27.2591386937935));
#219311=CARTESIAN_POINT('Ctrl Pts',(7.59300213145897,-2.22041429279753,
27.2671181098617));
#219312=CARTESIAN_POINT('Ctrl Pts',(7.64877740018541,-2.02968333970634,
27.2750981185768));
#219313=CARTESIAN_POINT('Ctrl Pts',(7.6973574218759,-1.83686512805803,27.2830781272919));
#219314=CARTESIAN_POINT('Ctrl Pts',(7.73860360030138,-1.64253928945476,
27.291058136007));
#219315=CARTESIAN_POINT('Ctrl Pts',(7.77985918114683,-1.44816915261064,
27.2990399638336));
#219316=CARTESIAN_POINT('Ctrl Pts',(7.81377751748777,-1.25229103108626,
27.3070217916601));
#219317=CARTESIAN_POINT('Ctrl Pts',(7.84027123541226,-1.05549417580919,
27.3150036194866));
#219318=CARTESIAN_POINT('Ctrl Pts',(7.86678465260723,-0.858550993221867,
27.322991382161));
#219319=CARTESIAN_POINT('Ctrl Pts',(7.88586237907792,-0.660688044086383,
27.3309791448354));
#219320=CARTESIAN_POINT('Ctrl Pts',(7.89746887389976,-0.46250014679399,
27.3389669075098));
#219321=CARTESIAN_POINT('Ctrl Pts',(7.90908048063459,-0.264224960504955,
27.3469581882789));
#219322=CARTESIAN_POINT('Ctrl Pts',(7.91321428347661,-0.0656248747359486,
27.3549494690479));
#219323=CARTESIAN_POINT('Ctrl Pts',(7.90988687085329,0.13270527609249,27.362940749817));
#219324=CARTESIAN_POINT('Ctrl Pts',(7.90655632757708,0.331222029224147,
27.3709395493188));
#219325=CARTESIAN_POINT('Ctrl Pts',(7.89575056311862,0.529468006427327,
27.3789383488207));
#219326=CARTESIAN_POINT('Ctrl Pts',(7.87753809705243,0.726852481241957,
27.3869371483225));
#219327=CARTESIAN_POINT('Ctrl Pts',(7.87336720928981,0.772056051562621,
27.3887689757552));
#219328=CARTESIAN_POINT('Ctrl Pts',(7.86880807626953,0.817214474545574,
27.390600803188));
#219329=CARTESIAN_POINT('Ctrl Pts',(7.86386189895736,0.86232072578982,27.3924326306207));
#219330=CARTESIAN_POINT('Ctrl Pts',(7.84191885665016,1.06242846898338,27.4005592836538));
#219331=CARTESIAN_POINT('Ctrl Pts',(7.81231554044796,1.26186151973571,27.4086859366868));
#219332=CARTESIAN_POINT('Ctrl Pts',(7.77510704393797,1.46001077232541,27.4168125897199));
#219333=CARTESIAN_POINT('Ctrl Pts',(7.73793022096867,1.65799135138606,27.4249323249815));
#219334=CARTESIAN_POINT('Ctrl Pts',(7.69316118279052,1.85468999905893,27.4330520602431));
#219335=CARTESIAN_POINT('Ctrl Pts',(7.64090667989423,2.04950386902485,27.4411717955047));
#219336=CARTESIAN_POINT('Ctrl Pts',(7.58869007803003,2.24417643735494,27.4492856413916));
#219337=CARTESIAN_POINT('Ctrl Pts',(7.52899891914404,2.43696664675881,27.4573994872786));
#219338=CARTESIAN_POINT('Ctrl Pts',(7.46199089884747,2.62728240307689,27.4655133331655));
#219339=CARTESIAN_POINT('Ctrl Pts',(7.39503049024378,2.81746293296538,27.4736214138628));
#219340=CARTESIAN_POINT('Ctrl Pts',(7.32076369783073,3.00517221739098,27.4817294945602));
#219341=CARTESIAN_POINT('Ctrl Pts',(7.23939798117092,3.18983351763356,27.4898375752576));
#219342=CARTESIAN_POINT('Ctrl Pts',(7.15806721149645,3.37441550491707,27.4979421734934));
#219343=CARTESIAN_POINT('Ctrl Pts',(7.06964372535775,3.5559518270448,27.5060467717293));
#219344=CARTESIAN_POINT('Ctrl Pts',(6.97438333418001,3.73388512248464,27.5141513699651));
#219345=CARTESIAN_POINT('Ctrl Pts',(6.87915271862058,3.91176280116894,27.52225343494));
#219346=CARTESIAN_POINT('Ctrl Pts',(6.77708961036011,4.08603941845193,27.530355499915));
#219347=CARTESIAN_POINT('Ctrl Pts',(6.66849630597499,4.25618115418011,27.5384575648899));
#219348=CARTESIAN_POINT('Ctrl Pts',(6.61073120943118,4.34668630867486,27.5427673754085));
#219349=CARTESIAN_POINT('Ctrl Pts',(6.55111910721999,4.43602187306296,27.547077185927));
#219350=CARTESIAN_POINT('Ctrl Pts',(6.48971066688954,4.52411057115761,27.5513869964456));
#219351=CARTESIAN_POINT('Ctrl Pts',(6.37160875429003,4.69352447692362,27.559675708265));
#219352=CARTESIAN_POINT('Ctrl Pts',(6.2469109124311,4.85825186655254,27.5679644200845));
#219353=CARTESIAN_POINT('Ctrl Pts',(6.11601819192606,5.01779258997714,27.5762531319039));
#219354=CARTESIAN_POINT('Ctrl Pts',(5.98505001304714,5.17742528706926,27.5845466220847));
#219355=CARTESIAN_POINT('Ctrl Pts',(5.84788001260705,5.33186512346555,27.5928401122655));
#219356=CARTESIAN_POINT('Ctrl Pts',(5.7049483526403,5.48064643027688,27.6011336024463));
#219357=CARTESIAN_POINT('Ctrl Pts',(5.56192567655974,5.62952247814388,27.609432373761));
#219358=CARTESIAN_POINT('Ctrl Pts',(5.41313421994016,5.77273259311984,27.6177311450758));
#219359=CARTESIAN_POINT('Ctrl Pts',(5.25905028154673,5.90984865594401,27.6260299163906));
#219360=CARTESIAN_POINT('Ctrl Pts',(5.10478698055674,6.04712432977836,27.6343383479541));
#219361=CARTESIAN_POINT('Ctrl Pts',(4.9452191019751,6.17829157707465,27.6426467795176));
#219362=CARTESIAN_POINT('Ctrl Pts',(4.78085658491677,6.30296210637966,27.6509552110811));
#219363=CARTESIAN_POINT('Ctrl Pts',(4.61639267790957,6.42770954092328,27.6592687678487));
#219364=CARTESIAN_POINT('Ctrl Pts',(4.44712846544184,6.54595208638212,27.6675823246164));
#219365=CARTESIAN_POINT('Ctrl Pts',(4.27360319432333,6.65734457103351,27.675895881384));
#219366=CARTESIAN_POINT('Ctrl Pts',(4.09988820943162,6.768858840186,27.6842185272959));
#219367=CARTESIAN_POINT('Ctrl Pts',(3.92190310444567,6.87350792750676,27.6925411732078));
#219368=CARTESIAN_POINT('Ctrl Pts',(3.74021347826065,6.97099161791473,27.7008638191197));
#219369=CARTESIAN_POINT('Ctrl Pts',(3.67124617746068,7.00799531009367,27.7040230001699));
#219370=CARTESIAN_POINT('Ctrl Pts',(3.60174533351802,7.04396704201864,27.7071821812201));
#219371=CARTESIAN_POINT('Ctrl Pts',(3.53174268526238,7.0788921877011,27.7103413622702));
#219372=CARTESIAN_POINT('Ctrl Pts',(3.3390033883788,7.17505209293512,27.7190395808307));
#219373=CARTESIAN_POINT('Ctrl Pts',(3.14228745469956,7.26336011798245,27.7277377993912));
#219374=CARTESIAN_POINT('Ctrl Pts',(2.9422257820067,7.34351608207506,27.7364360179517));
#219375=CARTESIAN_POINT('Ctrl Pts',(2.74233989031145,7.42360161840836,27.7451265939612));
#219376=CARTESIAN_POINT('Ctrl Pts',(2.5391143416163,7.4955493109218,27.7538171699706));
#219377=CARTESIAN_POINT('Ctrl Pts',(2.33320040946053,7.55910688172176,27.7625077459801));
#219378=CARTESIAN_POINT('Ctrl Pts',(2.12234812839698,7.62418872752853,27.7714067444897));
#219379=CARTESIAN_POINT('Ctrl Pts',(1.90867711533581,7.6804728782617,27.7803057429993));
#219380=CARTESIAN_POINT('Ctrl Pts',(1.6929071988585,7.72774133987759,27.7892047415089));
#219381=CARTESIAN_POINT('Ctrl Pts',(1.48281167866957,7.77376671817802,27.7978697108964));
#219382=CARTESIAN_POINT('Ctrl Pts',(1.27072649096759,7.81124450237042,27.806534680284));
#219383=CARTESIAN_POINT('Ctrl Pts',(1.05733189541374,7.8400236136724,27.8151996496715));
#219384=CARTESIAN_POINT('Ctrl Pts',(0.835292050071472,7.86996865237403,
27.8242156627421));
#219385=CARTESIAN_POINT('Ctrl Pts',(0.611834712781352,7.8904954553862,27.8332316758127));
#219386=CARTESIAN_POINT('Ctrl Pts',(0.387740269425987,7.90149216815821,
27.8422476888833));
#219387=CARTESIAN_POINT('Ctrl Pts',(0.163645826070641,7.91248888093021,
27.8512637019539));
#219388=CARTESIAN_POINT('Ctrl Pts',(-0.0610854473386478,7.91395542263523,
27.8602797150245));
#219389=CARTESIAN_POINT('Ctrl Pts',(-0.285662862010668,7.90584073513171,
27.8692957280951));
#219390=CARTESIAN_POINT('Ctrl Pts',(-0.480211015268739,7.8988110991802,
27.8771061692972));
#219391=CARTESIAN_POINT('Ctrl Pts',(-0.674559784868564,7.88459373706153,
27.8849166104994));
#219392=CARTESIAN_POINT('Ctrl Pts',(-0.868135493372626,7.86322209816985,
27.8927270517016));
#219393=CARTESIAN_POINT('Ctrl Pts',(-1.06169724545758,7.84185200013034,
27.9005369297867));
#219394=CARTESIAN_POINT('Ctrl Pts',(-1.25448569742344,7.81332869140897,
27.9083468078717));
#219395=CARTESIAN_POINT('Ctrl Pts',(-1.44593247985462,7.77773747716529,
27.9161566859568));
#219396=CARTESIAN_POINT('Ctrl Pts',(-1.63739925074674,7.74214254693544,
27.923967379451));
#219397=CARTESIAN_POINT('Ctrl Pts',(-1.82752372698342,7.69947830650449,
27.9317780729451));
#219398=CARTESIAN_POINT('Ctrl Pts',(-2.01574776697818,7.64988117162106,
27.9395887664393));
#219399=CARTESIAN_POINT('Ctrl Pts',(-2.20410538122401,7.60024883985127,
27.9474050028361));
#219400=CARTESIAN_POINT('Ctrl Pts',(-2.39055952383616,7.54367387406576,
27.9552212392329));
#219401=CARTESIAN_POINT('Ctrl Pts',(-2.57456640881466,7.48034282680969,
27.9630374756298));
#219402=CARTESIAN_POINT('Ctrl Pts',(-2.75864132380225,7.41698836514866,
27.9708566018023));
#219403=CARTESIAN_POINT('Ctrl Pts',(-2.94026684866335,7.34687296844819,
27.9786757279749));
#219404=CARTESIAN_POINT('Ctrl Pts',(-3.11891909844799,7.27023140328672,
27.9864948541474));
#219405=CARTESIAN_POINT('Ctrl Pts',(-3.29777000429548,7.19350461495227,
27.994322674959));
#219406=CARTESIAN_POINT('Ctrl Pts',(-3.47364071051776,7.11023730843021,
28.0021504957706));
#219407=CARTESIAN_POINT('Ctrl Pts',(-3.64603087473383,7.02071078029053,
28.0099783165822));
#219408=CARTESIAN_POINT('Ctrl Pts',(-3.7801624877571,6.95105287560464,28.016068909028));
#219409=CARTESIAN_POINT('Ctrl Pts',(-3.91218747058962,6.87760662874013,
28.0221595014739));
#219410=CARTESIAN_POINT('Ctrl Pts',(-4.04188246519154,6.80052256356651,
28.0282500939197));
#219411=CARTESIAN_POINT('Ctrl Pts',(-4.21472797360549,6.69779204203449,
28.0363670729217));
#219412=CARTESIAN_POINT('Ctrl Pts',(-4.38377786317178,6.58839489746363,
28.0444840519237));
#219413=CARTESIAN_POINT('Ctrl Pts',(-4.54850427346319,6.47263701085478,
28.0526010309257));
#219414=CARTESIAN_POINT('Ctrl Pts',(-4.71311019210323,6.35696379712196,
28.0607120726393));
#219415=CARTESIAN_POINT('Ctrl Pts',(-4.87339867558365,6.23493930186843,
28.0688231143529));
#219416=CARTESIAN_POINT('Ctrl Pts',(-5.02886943702191,6.10691355640367,
28.0769341560665));
#219417=CARTESIAN_POINT('Ctrl Pts',(-5.18424858218529,5.97896325433277,
28.0850404180811));
#219418=CARTESIAN_POINT('Ctrl Pts',(-5.33481541949327,5.84501895723589,
28.0931466800958));
#219419=CARTESIAN_POINT('Ctrl Pts',(-5.48010099593342,5.70547229196405,
28.1012529421105));
#219420=CARTESIAN_POINT('Ctrl Pts',(-5.62532159301977,5.565988039303,28.1093555785783));
#219421=CARTESIAN_POINT('Ctrl Pts',(-5.76526540890448,5.42090663721578,
28.1174582150462));
#219422=CARTESIAN_POINT('Ctrl Pts',(-5.89949834397028,5.27065843035687,
28.125560851514));
#219423=CARTESIAN_POINT('Ctrl Pts',(-6.03369029242549,5.12045610020283,
28.1336610139272));
#219424=CARTESIAN_POINT('Ctrl Pts',(-6.16217462460431,4.96509035080169,
28.1417611763405));
#219425=CARTESIAN_POINT('Ctrl Pts',(-6.28455534534605,4.8050270666545,28.1498613387537));
#219426=CARTESIAN_POINT('Ctrl Pts',(-6.40812811406901,4.64340468795731,
28.1580404007044));
#219427=CARTESIAN_POINT('Ctrl Pts',(-6.52547751237483,4.47699302135058,
28.166219462655));
#219428=CARTESIAN_POINT('Ctrl Pts',(-6.63623817174748,4.30630513640658,
28.1743985246057));
#219429=CARTESIAN_POINT('Ctrl Pts',(-6.74592977371789,4.13726472402103,
28.1824986425814));
#219430=CARTESIAN_POINT('Ctrl Pts',(-6.8491591054058,3.96403056200219,28.190598760557));
#219431=CARTESIAN_POINT('Ctrl Pts',(-6.94561521639302,3.78712955492808,
28.1986988785327));
#219432=CARTESIAN_POINT('Ctrl Pts',(-7.04208430867657,3.61020474008927,
28.2068000866418));
#219433=CARTESIAN_POINT('Ctrl Pts',(-7.13177820871898,3.42961237766244,
28.2149012947509));
#219434=CARTESIAN_POINT('Ctrl Pts',(-7.21443201372118,3.24590383705294,
28.22300250286));
#219435=CARTESIAN_POINT('Ctrl Pts',(-7.29710761715152,3.06214684667854,
28.2311058475145));
#219436=CARTESIAN_POINT('Ctrl Pts',(-7.37273929120307,2.87527233165193,
28.239209192169));
#219437=CARTESIAN_POINT('Ctrl Pts',(-7.44111013701217,2.68585199310289,
28.2473125368234));
#219438=CARTESIAN_POINT('Ctrl Pts',(-7.51061029049638,2.49330292564002,
28.2555497275523));
#219439=CARTESIAN_POINT('Ctrl Pts',(-7.57260753909675,2.29812352187236,
28.2637869182811));
#219440=CARTESIAN_POINT('Ctrl Pts',(-7.62692677239108,2.100930510175,28.2720241090099));
#219441=CARTESIAN_POINT('Ctrl Pts',(-7.68043295853602,1.90668907209746,
28.2801380059432));
#219442=CARTESIAN_POINT('Ctrl Pts',(-7.72648932949952,1.71049420536543,
28.2882519028766));
#219443=CARTESIAN_POINT('Ctrl Pts',(-7.76498004321694,1.51294610890233,
28.2963657998099));
#219444=CARTESIAN_POINT('Ctrl Pts',(-7.80434807881021,1.31089528308394,
28.3046646374365));
#219445=CARTESIAN_POINT('Ctrl Pts',(-7.83580140239664,1.10742915874967,
28.312963475063));
#219446=CARTESIAN_POINT('Ctrl Pts',(-7.85927207572049,0.903196235488287,
28.3212623126896));
#219447=CARTESIAN_POINT('Ctrl Pts',(-7.88274274904433,0.698963312226884,
28.3295611503162));
#219448=CARTESIAN_POINT('Ctrl Pts',(-7.898230780354,0.493963947803846,28.3378599879427));
#219449=CARTESIAN_POINT('Ctrl Pts',(-7.90572501483226,0.288847693180128,
28.3461588255693));
#219450=CARTESIAN_POINT('Ctrl Pts',(-7.9091896019269,0.194022380370513,
28.3499953809673));
#219451=CARTESIAN_POINT('Ctrl Pts',(-7.91094894867227,0.0991112522795639,
28.3538319363653));
#219452=CARTESIAN_POINT('Ctrl Pts',(-7.9109989050297,0.00416228529412779,
28.3576684917633));
#219453=CARTESIAN_POINT('',(-7.90357832657621,0.00116160200912298,30.3576684917633));
#219454=CARTESIAN_POINT('Ctrl Pts',(-7.92069697714534,0.00415614191964403,
28.3576689456146));
#219455=CARTESIAN_POINT('Ctrl Pts',(-7.91973006024624,-1.21367684137233,
28.4068170275411));
#219456=CARTESIAN_POINT('Ctrl Pts',(-7.29458056008006,-3.75569163334529,
28.5089498980758));
#219457=CARTESIAN_POINT('Ctrl Pts',(-3.85135548505637,-7.82348539955324,
28.717052345827));
#219458=CARTESIAN_POINT('Ctrl Pts',(3.55328581504252,-8.66439214142531,
28.9819762888683));
#219459=CARTESIAN_POINT('Ctrl Pts',(9.20702352837811,-1.6725696989809,29.2998850205178));
#219460=CARTESIAN_POINT('Ctrl Pts',(6.86085464277753,5.38250085615541,29.5648089635592));
#219461=CARTESIAN_POINT('Ctrl Pts',(2.06639954247995,7.97215553854543,29.776748117992));
#219462=CARTESIAN_POINT('Ctrl Pts',(-2.00486737260903,8.00605902378823,
29.9357024838169));
#219463=CARTESIAN_POINT('Ctrl Pts',(-5.57344547750851,6.06317035785365,
30.0946568496417));
#219464=CARTESIAN_POINT('Ctrl Pts',(-7.57769228948297,3.04117976839579,
30.2353121856238));
#219465=CARTESIAN_POINT('Ctrl Pts',(-7.90592795537224,0.863866818058979,
30.3229827329977));
#219466=CARTESIAN_POINT('Ctrl Pts',(-7.89949422726844,0.0018008241519719,
30.3576684917633));
#219467=CARTESIAN_POINT('',(-7.911,-6.8273164899324E-12,32.3576684917633));
#219468=CARTESIAN_POINT('Ctrl Pts',(-7.911,-6.88560319872522E-12,30.3576684917633));
#219469=CARTESIAN_POINT('Ctrl Pts',(-7.91099999999808,-2.20167589667365,
30.446255927496));
#219470=CARTESIAN_POINT('Ctrl Pts',(-6.9421457667199,-4.38610418339286,
30.5348433632287));
#219471=CARTESIAN_POINT('Ctrl Pts',(-3.6782020148765,-7.34180684107951,
30.7120182346942));
#219472=CARTESIAN_POINT('Ctrl Pts',(-1.40868175871044,-8.08992666571458,
30.8006056704269));
#219473=CARTESIAN_POINT('Ctrl Pts',(2.97309270521935,-7.65454228025,30.9777805418924));
#219474=CARTESIAN_POINT('Ctrl Pts',(5.05102072676161,-6.4744488083379,31.0663679776251));
#219475=CARTESIAN_POINT('Ctrl Pts',(7.66951518848124,-2.93425195367047,
31.2435428490906));
#219476=CARTESIAN_POINT('Ctrl Pts',(8.18956872247123,-0.601881960092137,
31.3321302848233));
#219477=CARTESIAN_POINT('Ctrl Pts',(7.32306689761024,3.71537198233077,31.5093051562887));
#219478=CARTESIAN_POINT('Ctrl Pts',(5.94329958849717,5.66643518937019,31.5978925920215));
#219479=CARTESIAN_POINT('Ctrl Pts',(2.16154501637172,7.92205913233182,31.7750674634869));
#219480=CARTESIAN_POINT('Ctrl Pts',(-0.210816529307356,8.20894963712984,
31.8636548992196));
#219481=CARTESIAN_POINT('Ctrl Pts',(-4.42123908577025,6.91982244717456,
32.0408297706851));
#219482=CARTESIAN_POINT('Ctrl Pts',(-6.22631625634641,5.35390358802993,
32.1294172064178));
#219483=CARTESIAN_POINT('Ctrl Pts',(-7.65317280859686,2.31334857513867,
32.2645592586881));
#219484=CARTESIAN_POINT('Ctrl Pts',(-7.911000000001,1.15702837835841,32.3111138752257));
#219485=CARTESIAN_POINT('Ctrl Pts',(-7.911,-6.8273164899324E-12,32.3576684917633));
#219486=CARTESIAN_POINT('',(-7.91204594914714,-0.00281928559808421,34.3576684917633));
#219487=CARTESIAN_POINT('Ctrl Pts',(-7.91099999939128,-9.81387723526022E-5,
32.3576684917633));
#219488=CARTESIAN_POINT('Ctrl Pts',(-7.91099751585164,-0.200297118282624,
32.3656923392676));
#219489=CARTESIAN_POINT('Ctrl Pts',(-7.90339122720327,-0.40042256281032,
32.373716186772));
#219490=CARTESIAN_POINT('Ctrl Pts',(-7.88822379333303,-0.599871974920195,
32.3817400342763));
#219491=CARTESIAN_POINT('Ctrl Pts',(-7.87290732035448,-0.801281228278693,
32.389842726171));
#219492=CARTESIAN_POINT('Ctrl Pts',(-7.84988034736886,-1.00200075216182,
32.3979454180657));
#219493=CARTESIAN_POINT('Ctrl Pts',(-7.81924013616528,-1.20141778452877,
32.4060481099605));
#219494=CARTESIAN_POINT('Ctrl Pts',(-7.78884737466464,-1.39922432912552,
32.4140853646854));
#219495=CARTESIAN_POINT('Ctrl Pts',(-7.75096400576114,-1.59574903115637,
32.4221226194104));
#219496=CARTESIAN_POINT('Ctrl Pts',(-7.70573595741653,-1.79040619820696,
32.4301598741354));
#219497=CARTESIAN_POINT('Ctrl Pts',(-7.65995555713476,-1.9874406348334,
32.438295284615));
#219498=CARTESIAN_POINT('Ctrl Pts',(-7.60665000850472,-2.18256128921893,
32.4464306950946));
#219499=CARTESIAN_POINT('Ctrl Pts',(-7.54602201322522,-2.37517847243538,
32.4545661055742));
#219500=CARTESIAN_POINT('Ctrl Pts',(-7.48539401794571,-2.56779565565183,
32.4627015160538));
#219501=CARTESIAN_POINT('Ctrl Pts',(-7.41744373511158,-2.75790905979931,
32.4708369265334));
#219502=CARTESIAN_POINT('Ctrl Pts',(-7.34242339731225,-2.94495155386327,
32.4789723370131));
#219503=CARTESIAN_POINT('Ctrl Pts',(-7.26757302459109,-3.13157028694375,
32.487089316015));
#219504=CARTESIAN_POINT('Ctrl Pts',(-7.18555049878641,-3.31546674058872,
32.495206295017));
#219505=CARTESIAN_POINT('Ctrl Pts',(-7.09657665040477,-3.49607220247663,
32.503323274019));
#219506=CARTESIAN_POINT('Ctrl Pts',(-7.00766788330481,-3.67654555773826,
32.5114343157326));
#219507=CARTESIAN_POINT('Ctrl Pts',(-6.91181807296472,-3.85373243432938,
32.5195453574462));
#219508=CARTESIAN_POINT('Ctrl Pts',(-6.80929592384273,-4.02708455604533,
32.5276563991598));
#219509=CARTESIAN_POINT('Ctrl Pts',(-6.70683418927916,-4.20033452430493,
32.5357626611745));
#219510=CARTESIAN_POINT('Ctrl Pts',(-6.59770811918204,-4.36975396842767,
32.5438689231892));
#219511=CARTESIAN_POINT('Ctrl Pts',(-6.48223234756314,-4.53481915760773,
32.5519751852039));
#219512=CARTESIAN_POINT('Ctrl Pts',(-6.36680822278493,-4.69981052095046,
32.5600778216717));
#219513=CARTESIAN_POINT('Ctrl Pts',(-6.24504024355459,-4.86045125074867,
32.5681804581395));
#219514=CARTESIAN_POINT('Ctrl Pts',(-6.11728667280101,-5.01624608275662,
32.5762830946073));
#219515=CARTESIAN_POINT('Ctrl Pts',(-5.98957211025251,-5.1719933444562,
32.5843832570206));
#219516=CARTESIAN_POINT('Ctrl Pts',(-5.85587580458666,-5.32289741184233,
32.5924834194338));
#219517=CARTESIAN_POINT('Ctrl Pts',(-5.71659700898962,-5.46849518942926,
32.600583581847));
#219518=CARTESIAN_POINT('Ctrl Pts',(-5.57596156991047,-5.61551116046858,
32.6087626437977));
#219519=CARTESIAN_POINT('Ctrl Pts',(-5.42963451903887,-5.75711666265266,
32.6169417057483));
#219520=CARTESIAN_POINT('Ctrl Pts',(-5.27806645274836,-5.89287158526065,
32.625120767699));
#219521=CARTESIAN_POINT('Ctrl Pts',(-5.12796131530042,-6.02731620684901,
32.6332208856746));
#219522=CARTESIAN_POINT('Ctrl Pts',(-4.97271614545482,-6.15602248894394,
32.6413210036503));
#219523=CARTESIAN_POINT('Ctrl Pts',(-4.81280360002459,-6.27860195486147,
32.649421121626));
#219524=CARTESIAN_POINT('Ctrl Pts',(-4.65286953317809,-6.40119791781935,
32.6575223297351));
#219525=CARTESIAN_POINT('Ctrl Pts',(-4.48826709261825,-6.51766522496317,
32.6656235378442));
#219526=CARTESIAN_POINT('Ctrl Pts',(-4.31950020762517,-6.62765712422769,
32.6737247459533));
#219527=CARTESIAN_POINT('Ctrl Pts',(-4.15068881345533,-6.73767803184233,
32.6818280906077));
#219528=CARTESIAN_POINT('Ctrl Pts',(-3.97771105325729,-6.84121995071108,
32.6899314352621));
#219529=CARTESIAN_POINT('Ctrl Pts',(-3.80109834675442,-6.93798042360317,
32.6980347799166));
#219530=CARTESIAN_POINT('Ctrl Pts',(-3.62156845994399,-7.03633912660939,
32.7062719706454));
#219531=CARTESIAN_POINT('Ctrl Pts',(-3.43828279823117,-7.12769023333335,
32.7145091613742));
#219532=CARTESIAN_POINT('Ctrl Pts',(-3.25182371357782,-7.21176563234087,
32.7227463521031));
#219533=CARTESIAN_POINT('Ctrl Pts',(-3.06815553774374,-7.29458259562771,
32.7308602490364));
#219534=CARTESIAN_POINT('Ctrl Pts',(-2.88140858540826,-7.37034004299627,
32.7389741459697));
#219535=CARTESIAN_POINT('Ctrl Pts',(-2.69215801552766,-7.43883097129046,
32.7470880429031));
#219536=CARTESIAN_POINT('Ctrl Pts',(-2.49859384247002,-7.50888301871932,
32.7553868805296));
#219537=CARTESIAN_POINT('Ctrl Pts',(-2.30241090357604,-7.57133323731986,
32.7636857181562));
#219538=CARTESIAN_POINT('Ctrl Pts',(-2.10423946725972,-7.62601450722634,
32.7719845557828));
#219539=CARTESIAN_POINT('Ctrl Pts',(-1.90606803094339,-7.68069577713281,
32.7802833934094));
#219540=CARTESIAN_POINT('Ctrl Pts',(-1.70590845196345,-7.72760805133005,
32.788582231036));
#219541=CARTESIAN_POINT('Ctrl Pts',(-1.50440079314152,-7.76664015218905,
32.7968810686625));
#219542=CARTESIAN_POINT('Ctrl Pts',(-1.31199505282891,-7.80390920839087,
32.8048050553071));
#219543=CARTESIAN_POINT('Ctrl Pts',(-1.11794724197646,-7.83407388985267,
32.8127290419516));
#219544=CARTESIAN_POINT('Ctrl Pts',(-0.922822870368844,-7.85699172393125,
32.8206530285961));
#219545=CARTESIAN_POINT('Ctrl Pts',(-0.72790742030301,-7.87988501966442,
32.8285685309519));
#219546=CARTESIAN_POINT('Ctrl Pts',(-0.531918042238157,-7.89554688301356,
32.8364840333077));
#219547=CARTESIAN_POINT('Ctrl Pts',(-0.33543177697902,-7.90388553326734,
32.8443995356635));
#219548=CARTESIAN_POINT('Ctrl Pts',(-0.13912347375537,-7.91221663101779,
32.8523078687706));
#219549=CARTESIAN_POINT('Ctrl Pts',(0.0576804802670977,-7.91323771422012,
32.8602162018777));
#219550=CARTESIAN_POINT('Ctrl Pts',(0.254396269709758,-7.90690859552314,
32.8681245349847));
#219551=CARTESIAN_POINT('Ctrl Pts',(0.450938590661315,-7.90058505798807,
32.8760258943424));
#219552=CARTESIAN_POINT('Ctrl Pts',(0.647392561310094,-7.88692425101804,
32.8839272537001));
#219553=CARTESIAN_POINT('Ctrl Pts',(0.843172661556533,-7.86593801544378,
32.8918286130578));
#219554=CARTESIAN_POINT('Ctrl Pts',(1.03885195967599,-7.84496258514126,
32.8997259042092));
#219555=CARTESIAN_POINT('Ctrl Pts',(1.23385773914795,-7.81666927600717,
32.9076231953607));
#219556=CARTESIAN_POINT('Ctrl Pts',(1.42760726097397,-7.78112193121367,
32.9155204865121));
#219557=CARTESIAN_POINT('Ctrl Pts',(1.62129091441759,-7.7455866713331,32.9234150928477));
#219558=CARTESIAN_POINT('Ctrl Pts',(1.81371882481146,-7.70280235050061,
32.9313096991832));
#219559=CARTESIAN_POINT('Ctrl Pts',(2.00431583579567,-7.65288436018595,
32.9392043055188));
#219560=CARTESIAN_POINT('Ctrl Pts',(2.13815588371267,-7.61783120703767,
32.944748015175));
#219561=CARTESIAN_POINT('Ctrl Pts',(2.27109324457853,-7.57926148210648,
32.9502917248312));
#219562=CARTESIAN_POINT('Ctrl Pts',(2.40293217908638,-7.53723012403835,
32.9558354344874));
#219563=CARTESIAN_POINT('Ctrl Pts',(2.60554771556565,-7.47263459165091,
32.9643552371562));
#219564=CARTESIAN_POINT('Ctrl Pts',(2.80536580397596,-7.39992595719343,
32.972875039825));
#219565=CARTESIAN_POINT('Ctrl Pts',(3.00176547501411,-7.31938009895738,
32.9813948424938));
#219566=CARTESIAN_POINT('Ctrl Pts',(3.1985203517524,-7.23868856660783,32.9899300539587));
#219567=CARTESIAN_POINT('Ctrl Pts',(3.39184422391902,-7.15013157600585,
32.9984652654236));
#219568=CARTESIAN_POINT('Ctrl Pts',(3.58113923516166,-7.05403166837134,
33.0070004768884));
#219569=CARTESIAN_POINT('Ctrl Pts',(3.78035301829711,-6.95289627112467,
33.0159829205071));
#219570=CARTESIAN_POINT('Ctrl Pts',(3.97510414562345,-6.84340654501848,
33.0249653641257));
#219571=CARTESIAN_POINT('Ctrl Pts',(4.16473106960945,-6.72598960137687,
33.0339478077443));
#219572=CARTESIAN_POINT('Ctrl Pts',(4.34567291235788,-6.61395045785329,
33.0425188474816));
#219573=CARTESIAN_POINT('Ctrl Pts',(4.52194926412814,-6.49469414161851,
33.0510898872189));
#219574=CARTESIAN_POINT('Ctrl Pts',(4.69301903899192,-6.36863355042974,
33.0596609269561));
#219575=CARTESIAN_POINT('Ctrl Pts',(4.86430347557559,-6.24241477593048,
33.0682427218027));
#219576=CARTESIAN_POINT('Ctrl Pts',(5.03036808583398,-6.10937482078115,
33.0768245166493));
#219577=CARTESIAN_POINT('Ctrl Pts',(5.1907054161778,-5.96996635522031,33.0854063114959));
#219578=CARTESIAN_POINT('Ctrl Pts',(5.35131094072339,-5.83032470290213,
33.094002461001));
#219579=CARTESIAN_POINT('Ctrl Pts',(5.50616984471472,-5.68429340668538,
33.1025986105061));
#219580=CARTESIAN_POINT('Ctrl Pts',(5.65481044660595,-5.53236295021904,
33.1111947600111));
#219581=CARTESIAN_POINT('Ctrl Pts',(5.67553169914019,-5.51118307529908,
33.1123931067781));
#219582=CARTESIAN_POINT('Ctrl Pts',(5.69613216964715,-5.48988861109374,
33.1135914535451));
#219583=CARTESIAN_POINT('Ctrl Pts',(5.71661064203229,-5.46848093782937,
33.114789800312));
#219584=CARTESIAN_POINT('Ctrl Pts',(5.8517469197889,-5.32721291617385,33.1226976226586));
#219585=CARTESIAN_POINT('Ctrl Pts',(5.98181649645736,-5.180751969505,33.1306054450051));
#219586=CARTESIAN_POINT('Ctrl Pts',(6.10639715746423,-5.02949647134908,
33.1385132673516));
#219587=CARTESIAN_POINT('Ctrl Pts',(6.23085054327868,-4.8783955001677,33.146413010839));
#219588=CARTESIAN_POINT('Ctrl Pts',(6.34982596579197,-4.72250999835522,
33.1543127543264));
#219589=CARTESIAN_POINT('Ctrl Pts',(6.46293785533335,-4.56227523041948,
33.1622124978138));
#219590=CARTESIAN_POINT('Ctrl Pts',(6.57595518990039,-4.40217440944928,
33.1701056375742));
#219591=CARTESIAN_POINT('Ctrl Pts',(6.68311855829631,-4.23773184540781,
33.1779987773345));
#219592=CARTESIAN_POINT('Ctrl Pts',(6.78408233919181,-4.06941615162,33.1858919170949));
#219593=CARTESIAN_POINT('Ctrl Pts',(6.88498046269459,-3.90120991460482,
33.193779923896));
#219594=CARTESIAN_POINT('Ctrl Pts',(6.97968685448573,-3.7291358608326,33.2016679306971));
#219595=CARTESIAN_POINT('Ctrl Pts',(7.0678987945588,-3.55369211241974,33.2095559374981));
#219596=CARTESIAN_POINT('Ctrl Pts',(7.1560697418556,-3.37832989408455,33.217440278681));
#219597=CARTESIAN_POINT('Ctrl Pts',(7.2377520967932,-3.19960140903364,33.2253246198638));
#219598=CARTESIAN_POINT('Ctrl Pts',(7.31268861647481,-3.01803018515052,
33.2332089610466));
#219599=CARTESIAN_POINT('Ctrl Pts',(7.38760421866241,-2.83650964436564,
33.2410911014245));
#219600=CARTESIAN_POINT('Ctrl Pts',(7.45577760722682,-2.65214826482966,
33.2489732418025));
#219601=CARTESIAN_POINT('Ctrl Pts',(7.51699919169613,-2.46549065137951,
33.2568553821804));
#219602=CARTESIAN_POINT('Ctrl Pts',(7.57822747035189,-2.27881262812,33.2647383844197));
#219603=CARTESIAN_POINT('Ctrl Pts',(7.63250231191321,-2.08983819486411,
33.2726213866589));
#219604=CARTESIAN_POINT('Ctrl Pts',(7.67966344111192,-1.89912886114897,
33.2805043888982));
#219605=CARTESIAN_POINT('Ctrl Pts',(7.72683025810499,-1.70839652723239,
33.2883883418546));
#219606=CARTESIAN_POINT('Ctrl Pts',(7.76688156967074,-1.51592921081426,
33.2962722948111));
#219607=CARTESIAN_POINT('Ctrl Pts',(7.79970786024444,-1.32230037995951,
33.3041562477676));
#219608=CARTESIAN_POINT('Ctrl Pts',(7.83254363023004,-1.12861563394007,
33.3120424774125));
#219609=CARTESIAN_POINT('Ctrl Pts',(7.85815016386974,-0.933769045222951,
33.3199287070574));
#219610=CARTESIAN_POINT('Ctrl Pts',(7.87646959053683,-0.738341241803896,
33.3278149367023));
#219611=CARTESIAN_POINT('Ctrl Pts',(7.8947973882697,-0.542824137609977,
33.3357047699615));
#219612=CARTESIAN_POINT('Ctrl Pts',(7.90583141148543,-0.34672563261261,
33.3435946032207));
#219613=CARTESIAN_POINT('Ctrl Pts',(7.9095658546241,-0.150628653862828,
33.3514844364799));
#219614=CARTESIAN_POINT('Ctrl Pts',(7.91330460454496,0.0456944755994065,
33.3593833687646));
#219615=CARTESIAN_POINT('Ctrl Pts',(7.90972695288974,0.242015730339113,
33.3672823010493));
#219616=CARTESIAN_POINT('Ctrl Pts',(7.89887919719827,0.437753844150282,
33.375181233334));
#219617=CARTESIAN_POINT('Ctrl Pts',(7.88802427672569,0.633621240071249,
33.3830853827458));
#219618=CARTESIAN_POINT('Ctrl Pts',(7.86988971147021,0.828904384874831,
33.3909895321577));
#219619=CARTESIAN_POINT('Ctrl Pts',(7.84457336390429,1.02302968594434,33.3988936815696));
#219620=CARTESIAN_POINT('Ctrl Pts',(7.81922232119861,1.21742102872598,33.4068086633326));
#219621=CARTESIAN_POINT('Ctrl Pts',(7.78666989428001,1.41065101945937,33.4147236450957));
#219622=CARTESIAN_POINT('Ctrl Pts',(7.74706473490351,1.60215760561012,33.4226386268588));
#219623=CARTESIAN_POINT('Ctrl Pts',(7.73028541029121,1.68329226647263,33.4259919285598));
#219624=CARTESIAN_POINT('Ctrl Pts',(7.71224078485991,1.76411778931457,33.4293452302607));
#219625=CARTESIAN_POINT('Ctrl Pts',(7.69294481085428,1.8445924040693,33.4326985319616));
#219626=CARTESIAN_POINT('Ctrl Pts',(7.6482896526346,2.03082848904188,33.4404588149082));
#219627=CARTESIAN_POINT('Ctrl Pts',(7.59678883034721,2.21577027280105,33.4482190978548));
#219628=CARTESIAN_POINT('Ctrl Pts',(7.5385262387593,2.39886288635627,33.4559793808014));
#219629=CARTESIAN_POINT('Ctrl Pts',(7.48033376911482,2.5817351387923,33.4637303238593));
#219630=CARTESIAN_POINT('Ctrl Pts',(7.41539583586916,2.76276231328958,33.4714812669172));
#219631=CARTESIAN_POINT('Ctrl Pts',(7.34384753351423,2.94139837568748,33.4792322099751));
#219632=CARTESIAN_POINT('Ctrl Pts',(7.27237082095791,3.11985569841846,33.4869753975945));
#219633=CARTESIAN_POINT('Ctrl Pts',(7.1942970382658,3.29592634153664,33.494718585214));
#219634=CARTESIAN_POINT('Ctrl Pts',(7.10981143473723,3.46907802773011,33.5024617728334));
#219635=CARTESIAN_POINT('Ctrl Pts',(7.02539324285138,3.64209155500512,33.5101987821104));
#219636=CARTESIAN_POINT('Ctrl Pts',(6.93457357238678,3.81219044163001,33.5179357913873));
#219637=CARTESIAN_POINT('Ctrl Pts',(6.83758630096032,3.97886096476362,33.5256728006642));
#219638=CARTESIAN_POINT('Ctrl Pts',(6.7406567800286,4.14543224492414,33.533405202985));
#219639=CARTESIAN_POINT('Ctrl Pts',(6.63756715092253,4.30857891727795,33.5411376053057));
#219640=CARTESIAN_POINT('Ctrl Pts',(6.52859792619909,4.46781043890953,33.5488700076264));
#219641=CARTESIAN_POINT('Ctrl Pts',(6.41967153992414,4.62697936276311,33.556599370152));
#219642=CARTESIAN_POINT('Ctrl Pts',(6.30487036406361,4.78223590553231,33.5643287326775));
#219643=CARTESIAN_POINT('Ctrl Pts',(6.18451910530415,4.93311711153586,33.5720580952031));
#219644=CARTESIAN_POINT('Ctrl Pts',(6.06416789350083,5.08399825867174,33.579787454713));
#219645=CARTESIAN_POINT('Ctrl Pts',(5.93826681802207,5.23050378465456,33.5875168142229));
#219646=CARTESIAN_POINT('Ctrl Pts',(5.80718212848568,5.37220222316664,33.5952461737328));
#219647=CARTESIAN_POINT('Ctrl Pts',(5.67609086851405,5.51390776411316,33.602975920666));
#219648=CARTESIAN_POINT('Ctrl Pts',(5.53981572038103,5.65080547330261,33.6107056675991));
#219649=CARTESIAN_POINT('Ctrl Pts',(5.39876108033296,5.78249944206501,33.6184354145323));
#219650=CARTESIAN_POINT('Ctrl Pts',(5.25767352373744,5.91422414296617,33.6261669652812));
#219651=CARTESIAN_POINT('Ctrl Pts',(5.11180451665938,6.04074243996941,33.6338985160301));
#219652=CARTESIAN_POINT('Ctrl Pts',(4.96159295997803,6.16169751768913,33.641630066779));
#219653=CARTESIAN_POINT('Ctrl Pts',(4.81131881675027,6.28270299206776,33.6493648389249));
#219654=CARTESIAN_POINT('Ctrl Pts',(4.65669880047748,6.39814040644776,33.6570996110708));
#219655=CARTESIAN_POINT('Ctrl Pts',(4.49820233994311,6.5076951917657,33.6648343832167));
#219656=CARTESIAN_POINT('Ctrl Pts',(4.33951687229848,6.61738062122115,33.6725783790824));
#219657=CARTESIAN_POINT('Ctrl Pts',(4.17694602386429,6.72116920750912,33.680322374948));
#219658=CARTESIAN_POINT('Ctrl Pts',(4.01098636851405,6.8187909010025,33.6880663708137));
#219659=CARTESIAN_POINT('Ctrl Pts',(3.84491899702214,6.91647595587214,33.6958153929211));
#219660=CARTESIAN_POINT('Ctrl Pts',(3.67545875205341,7.00798597507403,33.7035644150286));
#219661=CARTESIAN_POINT('Ctrl Pts',(3.50312378239829,7.09309838964578,33.711313437136));
#219662=CARTESIAN_POINT('Ctrl Pts',(3.33052544431363,7.17834087603641,33.7190743015746));
#219663=CARTESIAN_POINT('Ctrl Pts',(3.15504393341909,7.25716608453744,33.7268351660132));
#219664=CARTESIAN_POINT('Ctrl Pts',(2.97721534149284,7.32940037181621,33.7345960304519));
#219665=CARTESIAN_POINT('Ctrl Pts',(2.85492419423598,7.37907525124317,33.7399331081716));
#219666=CARTESIAN_POINT('Ctrl Pts',(2.73152339249698,7.42563420155241,33.7452701858914));
#219667=CARTESIAN_POINT('Ctrl Pts',(2.60719024406889,7.46903474561687,33.7506072636111));
#219668=CARTESIAN_POINT('Ctrl Pts',(2.42049987204106,7.53420211103824,33.7586210639342));
#219669=CARTESIAN_POINT('Ctrl Pts',(2.23113424949472,7.59244632073761,33.7666348642572));
#219670=CARTESIAN_POINT('Ctrl Pts',(2.03964247063132,7.64354496238473,33.7746486645803));
#219671=CARTESIAN_POINT('Ctrl Pts',(1.8483689697918,7.69458535761214,33.782653330117));
#219672=CARTESIAN_POINT('Ctrl Pts',(1.65497446234548,7.73849632921086,33.7906579956536));
#219673=CARTESIAN_POINT('Ctrl Pts',(1.4600263215984,7.77510412407704,33.7986626611903));
#219674=CARTESIAN_POINT('Ctrl Pts',(1.26526730305292,7.81167640515615,33.8066595612773));
#219675=CARTESIAN_POINT('Ctrl Pts',(1.06895798155994,7.84095956712274,33.8146564613643));
#219676=CARTESIAN_POINT('Ctrl Pts',(0.87167954054783,7.86283001079067,33.8226533614514));
#219677=CARTESIAN_POINT('Ctrl Pts',(0.674559012659043,7.8846829480851,33.830643860355));
#219678=CARTESIAN_POINT('Ctrl Pts',(0.476471242419789,7.89913495629219,
33.8386343592587));
#219679=CARTESIAN_POINT('Ctrl Pts',(0.278006635571342,7.90611366668721,
33.8466248581624));
#219680=CARTESIAN_POINT('Ctrl Pts',(0.0796672382447334,7.91308797427709,
33.8546103159327));
#219681=CARTESIAN_POINT('Ctrl Pts',(-0.119048188392748,7.91259837046145,
33.8625957737031));
#219682=CARTESIAN_POINT('Ctrl Pts',(-0.317544683696693,7.90462436639819,
33.8705812314734));
#219683=CARTESIAN_POINT('Ctrl Pts',(-0.522549404154987,7.89638891382046,
33.8788285132979));
#219684=CARTESIAN_POINT('Ctrl Pts',(-0.727320230152651,7.88016990300526,
33.8870757951224));
#219685=CARTESIAN_POINT('Ctrl Pts',(-0.931201043011376,7.85600315793563,
33.8953230769468));
#219686=CARTESIAN_POINT('Ctrl Pts',(-1.12847562039773,7.83261947433359,
33.9033031267303));
#219687=CARTESIAN_POINT('Ctrl Pts',(-1.32491660216615,7.80179508432112,
33.9112831765138));
#219688=CARTESIAN_POINT('Ctrl Pts',(-1.51993413497656,7.76361521620779,
33.9192632262972));
#219689=CARTESIAN_POINT('Ctrl Pts',(-1.71493618096541,7.72543838005161,
33.9272426423654));
#219690=CARTESIAN_POINT('Ctrl Pts',(-1.90851467496671,7.67990729418527,
33.9352220584335));
#219691=CARTESIAN_POINT('Ctrl Pts',(-2.10008938177088,7.62715842162553,
33.9432014745016));
#219692=CARTESIAN_POINT('Ctrl Pts',(-2.2916783172079,7.57440563130256,33.9511814832167));
#219693=CARTESIAN_POINT('Ctrl Pts',(-2.48126284631228,7.51443407491835,
33.9591614919319));
#219694=CARTESIAN_POINT('Ctrl Pts',(-2.66827696741949,7.44743036389993,
33.967141500647));
#219695=CARTESIAN_POINT('Ctrl Pts',(-2.8553337199984,7.38041137881133,33.9751233284735));
#219696=CARTESIAN_POINT('Ctrl Pts',(-3.03981858195051,7.30635715717243,
33.9831051563001));
#219697=CARTESIAN_POINT('Ctrl Pts',(-3.22118427901842,7.22550294724212,
33.9910869841266));
#219698=CARTESIAN_POINT('Ctrl Pts',(-3.40268482963671,7.14458861857134,
33.999074746801));
#219699=CARTESIAN_POINT('Ctrl Pts',(-3.58106127676926,7.05686433803137,
34.0070625094754));
#219700=CARTESIAN_POINT('Ctrl Pts',(-3.75578884196494,6.96261238146801,
34.0150502721498));
#219701=CARTESIAN_POINT('Ctrl Pts',(-3.93059336339302,6.86831891299172,
34.0230415529188));
#219702=CARTESIAN_POINT('Ctrl Pts',(-4.10174550842667,6.76749220202758,
34.0310328336879));
#219703=CARTESIAN_POINT('Ctrl Pts',(-4.26874787360661,6.66045888746256,
34.039024114457));
#219704=CARTESIAN_POINT('Ctrl Pts',(-4.43590736580849,6.55332486877909,
34.0470229139588));
#219705=CARTESIAN_POINT('Ctrl Pts',(-4.59890900402786,6.43997277148666,
34.0550217134607));
#219706=CARTESIAN_POINT('Ctrl Pts',(-4.75728616458605,6.32077126213551,
34.0630205129625));
#219707=CARTESIAN_POINT('Ctrl Pts',(-4.79355656083256,6.29347259127849,
34.0648523403952));
#219708=CARTESIAN_POINT('Ctrl Pts',(-4.82958456007265,6.26586729955871,
34.0666841678279));
#219709=CARTESIAN_POINT('Ctrl Pts',(-4.86536481653062,6.23796009942882,
34.0685159952606));
#219710=CARTESIAN_POINT('Ctrl Pts',(-5.02409905343179,6.11415360514417,
34.0766426482937));
#219711=CARTESIAN_POINT('Ctrl Pts',(-5.17823453496432,5.98418379559127,
34.0847693013268));
#219712=CARTESIAN_POINT('Ctrl Pts',(-5.32728194534809,5.84841757014393,
34.0928959543598));
#219713=CARTESIAN_POINT('Ctrl Pts',(-5.47620247989274,5.71276691499556,
34.1010156896214));
#219714=CARTESIAN_POINT('Ctrl Pts',(-5.62004334347727,5.57132989459795,
34.109135424883));
#219715=CARTESIAN_POINT('Ctrl Pts',(-5.75834768658442,5.42451407228407,
34.1172551601446));
#219716=CARTESIAN_POINT('Ctrl Pts',(-5.89655171532517,5.27780473784946,
34.1253690060315));
#219717=CARTESIAN_POINT('Ctrl Pts',(-6.02922701250107,5.12572461156609,
34.1334828519184));
#219718=CARTESIAN_POINT('Ctrl Pts',(-6.15595264358235,4.96871895461712,
34.1415966978053));
#219719=CARTESIAN_POINT('Ctrl Pts',(-6.28258823138525,4.81182485603212,
34.1497047785027));
#219720=CARTESIAN_POINT('Ctrl Pts',(-6.40328238722698,4.65001245644391,
34.1578128592001));
#219721=CARTESIAN_POINT('Ctrl Pts',(-6.51765338771445,4.48376129132834,
34.1659209398974));
#219722=CARTESIAN_POINT('Ctrl Pts',(-6.63197526528062,4.31758153192632,
34.1740255381332));
#219723=CARTESIAN_POINT('Ctrl Pts',(-6.73997922220622,4.14696707052053,
34.1821301363691));
#219724=CARTESIAN_POINT('Ctrl Pts',(-6.84132542625956,3.97242840237738,
34.1902347346049));
#219725=CARTESIAN_POINT('Ctrl Pts',(-6.94263995244727,3.79794428992803,
34.1983367995798));
#219726=CARTESIAN_POINT('Ctrl Pts',(-7.03730071617164,3.61953869245295,
34.2064388645547));
#219727=CARTESIAN_POINT('Ctrl Pts',(-7.12501233872718,3.43774928884954,
34.2145409295297));
#219728=CARTESIAN_POINT('Ctrl Pts',(-7.17166963839849,3.34104827667042,
34.2188507400483));
#219729=CARTESIAN_POINT('Ctrl Pts',(-7.21636137211169,3.24339022665641,
34.2231605505669));
#219730=CARTESIAN_POINT('Ctrl Pts',(-7.25904840949159,3.14485885035522,
34.2274703610855));
#219731=CARTESIAN_POINT('Ctrl Pts',(-7.3397234526633,2.95864252978646,34.2356155538885));
#219732=CARTESIAN_POINT('Ctrl Pts',(-7.41321019089491,2.76936358343293,
34.2437607466915));
#219733=CARTESIAN_POINT('Ctrl Pts',(-7.47929653081031,2.57760439249488,
34.2519059394945));
#219734=CARTESIAN_POINT('Ctrl Pts',(-7.54540914024934,2.38576897668789,
34.2600543700367));
#219735=CARTESIAN_POINT('Ctrl Pts',(-7.60411538130517,2.19145164546105,
34.268202800579));
#219736=CARTESIAN_POINT('Ctrl Pts',(-7.65525293737596,1.99525022611117,
34.2763512311212));
#219737=CARTESIAN_POINT('Ctrl Pts',(-7.70643729736452,1.79886923237797,
34.2845071195575));
#219738=CARTESIAN_POINT('Ctrl Pts',(-7.75003905080395,1.60060100786197,
34.2926630079937));
#219739=CARTESIAN_POINT('Ctrl Pts',(-7.7859466513297,1.40105522469594,34.30081889643));
#219740=CARTESIAN_POINT('Ctrl Pts',(-7.82187261808719,1.20140737667341,
34.3089789564882));
#219741=CARTESIAN_POINT('Ctrl Pts',(-7.85009653171284,1.00048097534893,
34.3171390165465));
#219742=CARTESIAN_POINT('Ctrl Pts',(-7.87055857554369,0.798892176038643,
34.3252990766047));
#219743=CARTESIAN_POINT('Ctrl Pts',(-7.89104121973609,0.597100425244778,
34.3334673518828));
#219744=CARTESIAN_POINT('Ctrl Pts',(-7.90374635618476,0.394645255978008,
34.3416356271609));
#219745=CARTESIAN_POINT('Ctrl Pts',(-7.90866620186477,0.192145537241679,
34.3498039024389));
#219746=CARTESIAN_POINT('Ctrl Pts',(-7.91024517924965,0.127155190567017,
34.3524254322137));
#219747=CARTESIAN_POINT('Ctrl Pts',(-7.91102265168034,0.0621602421645904,
34.3550469619885));
#219748=CARTESIAN_POINT('Ctrl Pts',(-7.91099949777088,-0.00281891271787961,
34.3576684917633));
#219749=CARTESIAN_POINT('',(-7.91647471845545,0.00302621288097889,36.3576684917633));
#219750=CARTESIAN_POINT('Ctrl Pts',(-7.91204594914714,-0.00281928559808421,
34.3576684917633));
#219751=CARTESIAN_POINT('Ctrl Pts',(-7.91263194564264,-0.240441980020169,
34.3672539034789));
#219752=CARTESIAN_POINT('Ctrl Pts',(-7.84556028379859,-1.79088486701073,
34.4298241038026));
#219753=CARTESIAN_POINT('Ctrl Pts',(-6.85004567783285,-4.57189276894299,
34.5453790927351));
#219754=CARTESIAN_POINT('Ctrl Pts',(-2.81663569969601,-8.25789292523349,
34.7573182471679));
#219755=CARTESIAN_POINT('Ctrl Pts',(3.1111528735023,-8.15382484340564,34.969257401601));
#219756=CARTESIAN_POINT('Ctrl Pts',(6.99765226366875,-4.32682987995013,
35.1811965560339));
#219757=CARTESIAN_POINT('Ctrl Pts',(8.68015910443019,0.833487127119469,
35.3931357104671));
#219758=CARTESIAN_POINT('Ctrl Pts',(5.50527049693975,7.57558763524673,35.6580596535081));
#219759=CARTESIAN_POINT('Ctrl Pts',(-3.41422952378675,8.71262350896433,
35.9759683851579));
#219760=CARTESIAN_POINT('Ctrl Pts',(-7.61324989218557,3.69250539781279,
36.2091713312427));
#219761=CARTESIAN_POINT('Ctrl Pts',(-7.91879245460977,0.531856155555196,
36.3364047001113));
#219762=CARTESIAN_POINT('Ctrl Pts',(-7.91647471845545,0.00302621288097889,
36.3576684917633));
#219763=CARTESIAN_POINT('',(-7.91099900736828,0.00390977488672659,38.3579590976759));
#219764=CARTESIAN_POINT('Ctrl Pts',(-7.91099942198829,0.00302411985178654,
36.3576684917633));
#219765=CARTESIAN_POINT('Ctrl Pts',(-7.91107476249638,-0.194064205058786,
36.3655987410024));
#219766=CARTESIAN_POINT('Ctrl Pts',(-7.90378024015271,-0.391324740971317,
36.3735289902414));
#219767=CARTESIAN_POINT('Ctrl Pts',(-7.88910633031748,-0.588151603708371,
36.3814592394805));
#219768=CARTESIAN_POINT('Ctrl Pts',(-7.87478977333831,-0.780185153528796,
36.3891963638301));
#219769=CARTESIAN_POINT('Ctrl Pts',(-7.85344908612159,-0.971805523534133,
36.3969334881797));
#219770=CARTESIAN_POINT('Ctrl Pts',(-7.82512812677067,-1.16245034286313,
36.4046706125293));
#219771=CARTESIAN_POINT('Ctrl Pts',(-7.79574679629921,-1.36023313581051,
36.4126974242131));
#219772=CARTESIAN_POINT('Ctrl Pts',(-7.75885239555156,-1.55696551137542,
36.4207242358969));
#219773=CARTESIAN_POINT('Ctrl Pts',(-7.71455283276676,-1.75202613863217,
36.4287510475807));
#219774=CARTESIAN_POINT('Ctrl Pts',(-7.67025326998196,-1.94708676588892,
36.4367778592645));
#219775=CARTESIAN_POINT('Ctrl Pts',(-7.61854863814548,-2.14047522170225,
36.4448046709482));
#219776=CARTESIAN_POINT('Ctrl Pts',(-7.55960584956221,-2.33158323875963,
36.452831482632));
#219777=CARTESIAN_POINT('Ctrl Pts',(-7.49873986595021,-2.52892675972155,
36.4611201944515));
#219778=CARTESIAN_POINT('Ctrl Pts',(-7.43016362405057,-2.72381637900719,
36.469408906271));
#219779=CARTESIAN_POINT('Ctrl Pts',(-7.35410670943481,-2.91565352987044,
36.4776976180904));
#219780=CARTESIAN_POINT('Ctrl Pts',(-7.27800594875152,-3.10760127297521,
36.4859911082712));
#219781=CARTESIAN_POINT('Ctrl Pts',(-7.19441601513058,-3.29649276321212,
36.494284598452));
#219782=CARTESIAN_POINT('Ctrl Pts',(-7.10361425212294,-3.48175035823016,
36.5025780886328));
#219783=CARTESIAN_POINT('Ctrl Pts',(-7.01275466831001,-3.66712592169922,
36.5108768599476));
#219784=CARTESIAN_POINT('Ctrl Pts',(-6.91467421693679,-3.84886270843548,
36.5191756312624));
#219785=CARTESIAN_POINT('Ctrl Pts',(-6.80969610124306,-4.02640782940763,
36.5274744025772));
#219786=CARTESIAN_POINT('Ctrl Pts',(-6.70459578496448,-4.20415962314656,
36.5357828341408));
#219787=CARTESIAN_POINT('Ctrl Pts',(-6.59258190386947,-4.3777097458219,
36.5440912657043));
#219788=CARTESIAN_POINT('Ctrl Pts',(-6.47402183736757,-4.54653299221372,
36.5523996972678));
#219789=CARTESIAN_POINT('Ctrl Pts',(-6.35538863497532,-4.71546038023435,
36.5607132540355));
#219790=CARTESIAN_POINT('Ctrl Pts',(-6.23020135994754,-4.87965483613968,
36.5690268108031));
#219791=CARTESIAN_POINT('Ctrl Pts',(-6.09886844427265,-5.03862329406112,
36.5773403675708));
#219792=CARTESIAN_POINT('Ctrl Pts',(-5.9673919433846,-5.19776555091025,
36.5856630134827));
#219793=CARTESIAN_POINT('Ctrl Pts',(-5.82975656394132,-5.35167016877368,
36.5939856593946));
#219794=CARTESIAN_POINT('Ctrl Pts',(-5.68640953514584,-5.49987887126639,
36.6023083053066));
#219795=CARTESIAN_POINT('Ctrl Pts',(-5.63199664509257,-5.55613719696339,
36.6054674863567));
#219796=CARTESIAN_POINT('Ctrl Pts',(-5.57676114621976,-5.61157520261264,
36.6086266674068));
#219797=CARTESIAN_POINT('Ctrl Pts',(-5.52072881163643,-5.66616928694929,
36.6117858484569));
#219798=CARTESIAN_POINT('Ctrl Pts',(-5.36645418003708,-5.8164839634869,
36.6204840670173));
#219799=CARTESIAN_POINT('Ctrl Pts',(-5.20599955280558,-5.9605317973859,
36.6291822855778));
#219800=CARTESIAN_POINT('Ctrl Pts',(-5.03987436346181,-6.09783464850601,
36.6378805041383));
#219801=CARTESIAN_POINT('Ctrl Pts',(-4.87389513736593,-6.235016860666,36.6465710801477));
#219802=CARTESIAN_POINT('Ctrl Pts',(-4.70225547389765,-6.36546577796639,
36.6552616561572));
#219803=CARTESIAN_POINT('Ctrl Pts',(-4.52549880935453,-6.48874267686204,
36.6639522321667));
#219804=CARTESIAN_POINT('Ctrl Pts',(-4.34450306262691,-6.61497607477977,
36.6728512306762));
#219805=CARTESIAN_POINT('Ctrl Pts',(-4.158141977721,-6.73368897837097,36.6817502291858));
#219806=CARTESIAN_POINT('Ctrl Pts',(-3.96703473233668,-6.84445442912979,
36.6906492276954));
#219807=CARTESIAN_POINT('Ctrl Pts',(-3.78095329528384,-6.9523069294971,
36.6993141970829));
#219808=CARTESIAN_POINT('Ctrl Pts',(-3.5903723669704,-7.05262452971617,
36.7079791664705));
#219809=CARTESIAN_POINT('Ctrl Pts',(-3.39589382665893,-7.14505606122582,
36.716644135858));
#219810=CARTESIAN_POINT('Ctrl Pts',(-3.19353638222078,-7.24123226900607,
36.7256601489286));
#219811=CARTESIAN_POINT('Ctrl Pts',(-2.98695913188559,-7.328869994186,36.7346761619992));
#219812=CARTESIAN_POINT('Ctrl Pts',(-2.77687127158161,-7.40762491903206,
36.7436921750698));
#219813=CARTESIAN_POINT('Ctrl Pts',(-2.56678341127766,-7.48637984387811,
36.7527081881404));
#219814=CARTESIAN_POINT('Ctrl Pts',(-2.35318517926386,-7.55625180730678,
36.761724201211));
#219815=CARTESIAN_POINT('Ctrl Pts',(-2.13681410900475,-7.61695125779063,
36.7707402142816));
#219816=CARTESIAN_POINT('Ctrl Pts',(-1.94937499274797,-7.66953431033245,
36.7785506554837));
#219817=CARTESIAN_POINT('Ctrl Pts',(-1.75993569387107,-7.7152106682391,
36.7863610966859));
#219818=CARTESIAN_POINT('Ctrl Pts',(-1.56905280285689,-7.75383739201738,
36.7941715378881));
#219819=CARTESIAN_POINT('Ctrl Pts',(-1.37818367411464,-7.7924613308867,
36.8019814159732));
#219820=CARTESIAN_POINT('Ctrl Pts',(-1.18587150572844,-7.82403657819518,
36.8097912940583));
#219821=CARTESIAN_POINT('Ctrl Pts',(-0.992683632905888,-7.84847120176667,
36.8176011721434));
#219822=CARTESIAN_POINT('Ctrl Pts',(-0.799475589840243,-7.87290837649363,
36.8254118656376));
#219823=CARTESIAN_POINT('Ctrl Pts',(-0.605392009731172,-7.89020339912567,
36.8332225591317));
#219824=CARTESIAN_POINT('Ctrl Pts',(-0.411006059591829,-7.90031613411633,
36.8410332526259));
#219825=CARTESIAN_POINT('Ctrl Pts',(-0.216482162367165,-7.91043604566639,
36.8488494890227));
#219826=CARTESIAN_POINT('Ctrl Pts',(-0.0216558185432678,-7.91336346825983,
36.8566657254195));
#219827=CARTESIAN_POINT('Ctrl Pts',(0.172898201252367,-7.90911039321134,
36.8644819618164));
#219828=CARTESIAN_POINT('Ctrl Pts',(0.367524150485898,-7.90485574573944,
36.8723010879889));
#219829=CARTESIAN_POINT('Ctrl Pts',(0.56187722347289,-7.89341532808239,
36.8801202141615));
#219830=CARTESIAN_POINT('Ctrl Pts',(0.755386913604808,-7.87485311677333,
36.8879393403341));
#219831=CARTESIAN_POINT('Ctrl Pts',(0.94911178083699,-7.85627026482968,
36.8957671611457));
#219832=CARTESIAN_POINT('Ctrl Pts',(1.14199104226654,-7.83054984195504,
36.9035949819573));
#219833=CARTESIAN_POINT('Ctrl Pts',(1.33346243678921,-7.79780731550044,
36.9114228027688));
#219834=CARTESIAN_POINT('Ctrl Pts',(1.48244058245026,-7.77233133833098,
36.9175133952147));
#219835=CARTESIAN_POINT('Ctrl Pts',(1.63056657029824,-7.74260527242311,
36.9236039876605));
#219836=CARTESIAN_POINT('Ctrl Pts',(1.77758179887016,-7.70870442735519,
36.9296945801064));
#219837=CARTESIAN_POINT('Ctrl Pts',(1.97351011518767,-7.66352451259113,
36.9378115591084));
#219838=CARTESIAN_POINT('Ctrl Pts',(2.16785460434091,-7.61083846189088,
36.9459285381104));
#219839=CARTESIAN_POINT('Ctrl Pts',(2.3600193048635,-7.55077677333078,36.9540455171123));
#219840=CARTESIAN_POINT('Ctrl Pts',(2.55204344357796,-7.49075901781104,
36.9621565588259));
#219841=CARTESIAN_POINT('Ctrl Pts',(2.74189066777335,-7.42337647672146,
36.9702676005396));
#219842=CARTESIAN_POINT('Ctrl Pts',(2.92897782587097,-7.34881010065957,
36.9783786422531));
#219843=CARTESIAN_POINT('Ctrl Pts',(3.11595473668884,-7.27428766529466,
36.9864849042678));
#219844=CARTESIAN_POINT('Ctrl Pts',(3.30017452750588,-7.1925899548432,36.9945911662825));
#219845=CARTESIAN_POINT('Ctrl Pts',(3.48107121658169,-7.10394708490192,
37.0026974282972));
#219846=CARTESIAN_POINT('Ctrl Pts',(3.66188699914079,-7.01534386071576,
37.010800064765));
#219847=CARTESIAN_POINT('Ctrl Pts',(3.83938235647035,-6.91980181257708,
37.0189027012329));
#219848=CARTESIAN_POINT('Ctrl Pts',(4.01301270567736,-6.81759855257495,
37.0270053377007));
#219849=CARTESIAN_POINT('Ctrl Pts',(4.18659003868975,-6.7154264992596,37.035105500114));
#219850=CARTESIAN_POINT('Ctrl Pts',(4.35630444132757,-6.60659745331978,
37.0432056625273));
#219851=CARTESIAN_POINT('Ctrl Pts',(4.52163679433242,-6.49143448708675,
37.0513058249406));
#219852=CARTESIAN_POINT('Ctrl Pts',(4.68857956518987,-6.37514977732676,
37.0594848868912));
#219853=CARTESIAN_POINT('Ctrl Pts',(4.85105417908993,-6.25240726674657,
37.0676639488419));
#219854=CARTESIAN_POINT('Ctrl Pts',(5.00855630989813,-6.12358430092864,
37.0758430107925));
#219855=CARTESIAN_POINT('Ctrl Pts',(5.16453823651368,-5.99600472916347,
37.0839431287682));
#219856=CARTESIAN_POINT('Ctrl Pts',(5.31564300693685,-5.86246178413592,
37.0920432467439));
#219857=CARTESIAN_POINT('Ctrl Pts',(5.46141391000008,-5.72336256964886,
37.1001433647196));
#219858=CARTESIAN_POINT('Ctrl Pts',(5.60720443126282,-5.58424463485422,
37.1082445728287));
#219859=CARTESIAN_POINT('Ctrl Pts',(5.74765942143414,-5.43956916074917,
37.1163457809378));
#219860=CARTESIAN_POINT('Ctrl Pts',(5.8823585729742,-5.28978058325267,37.1244469890468));
#219861=CARTESIAN_POINT('Ctrl Pts',(6.01709324894984,-5.1399525017607,37.1325503337013));
#219862=CARTESIAN_POINT('Ctrl Pts',(6.14606884454866,-4.98500886611857,
37.1406536783557));
#219863=CARTESIAN_POINT('Ctrl Pts',(6.26890457849805,-4.82542810387702,
37.1487570230102));
#219864=CARTESIAN_POINT('Ctrl Pts',(6.39376923772251,-4.6632114845317,37.156994213739));
#219865=CARTESIAN_POINT('Ctrl Pts',(6.51228922050543,-4.49620348421384,
37.1652314044678));
#219866=CARTESIAN_POINT('Ctrl Pts',(6.62410982722577,-4.32493814948271,
37.1734685951966));
#219867=CARTESIAN_POINT('Ctrl Pts',(6.73425670955768,-4.15623630439844,
37.1815824921299));
#219868=CARTESIAN_POINT('Ctrl Pts',(6.83790322831374,-3.98340397470245,
37.1896963890633));
#219869=CARTESIAN_POINT('Ctrl Pts',(6.93475617045278,-3.80697752244048,
37.1978102859966));
#219870=CARTESIAN_POINT('Ctrl Pts',(7.03381668934642,-3.6265297681271,37.2061091236232));
#219871=CARTESIAN_POINT('Ctrl Pts',(7.12577008698459,-3.44232241762529,
37.2144079612497));
#219872=CARTESIAN_POINT('Ctrl Pts',(7.21035405914917,-3.254952433095,37.2227067988763));
#219873=CARTESIAN_POINT('Ctrl Pts',(7.29493803131375,-3.06758244856471,
37.2310056365028));
#219874=CARTESIAN_POINT('Ctrl Pts',(7.37215247685052,-2.87705017327259,
37.2393044741294));
#219875=CARTESIAN_POINT('Ctrl Pts',(7.44178885452159,-2.683970872554,37.2476033117559));
#219876=CARTESIAN_POINT('Ctrl Pts',(7.50827982006027,-2.49961278903974,
37.2555272984004));
#219877=CARTESIAN_POINT('Ctrl Pts',(7.56800456966879,-2.31253682802811,
37.263451285045));
#219878=CARTESIAN_POINT('Ctrl Pts',(7.62073513691692,-2.12327976794391,
37.2713752716895));
#219879=CARTESIAN_POINT('Ctrl Pts',(7.6734092450396,-1.93422534721395,37.2792907740453));
#219880=CARTESIAN_POINT('Ctrl Pts',(7.71910399549655,-1.74299480556682,
37.2872062764011));
#219881=CARTESIAN_POINT('Ctrl Pts',(7.75763972954911,-1.55014413088628,
37.2951217787569));
#219882=CARTESIAN_POINT('Ctrl Pts',(7.79614056091922,-1.35746812540629,
37.3030301118639));
#219883=CARTESIAN_POINT('Ctrl Pts',(7.82749522594396,-1.16317524362569,
37.310938444971));
#219884=CARTESIAN_POINT('Ctrl Pts',(7.85157399763482,-0.967836122318609,
37.318846778078));
#219885=CARTESIAN_POINT('Ctrl Pts',(7.8756315361131,-0.772669255524447,
37.3267481374357));
#219886=CARTESIAN_POINT('Ctrl Pts',(7.892425930422,-0.576458326801188,37.3346494967933));
#219887=CARTESIAN_POINT('Ctrl Pts',(7.90187859668068,-0.379783679638453,
37.342550856151));
#219888=CARTESIAN_POINT('Ctrl Pts',(7.91132639600518,-0.183210295181699,
37.3504481473024));
#219889=CARTESIAN_POINT('Ctrl Pts',(7.91343998100059,0.013825991140516,
37.3583454384539));
#219890=CARTESIAN_POINT('Ctrl Pts',(7.90819257704468,0.210739565282478,
37.3662427296053));
#219891=CARTESIAN_POINT('Ctrl Pts',(7.90294695703129,0.407586195369699,
37.3741373359408));
#219892=CARTESIAN_POINT('Ctrl Pts',(7.89034534262739,0.604309854653562,
37.3820319422764));
#219893=CARTESIAN_POINT('Ctrl Pts',(7.870413060219,0.800324472657258,37.3899265486119));
#219894=CARTESIAN_POINT('Ctrl Pts',(7.85641631588982,0.937968844574584,
37.3954702582682));
#219895=CARTESIAN_POINT('Ctrl Pts',(7.838805867321,1.0752635556771,37.4010139679244));
#219896=CARTESIAN_POINT('Ctrl Pts',(7.81760581450124,1.21200673639894,37.4065576775806));
#219897=CARTESIAN_POINT('Ctrl Pts',(7.7850246950356,1.42215932163486,37.4150774802494));
#219898=CARTESIAN_POINT('Ctrl Pts',(7.74399615321713,1.63079889778628,37.4235972829182));
#219899=CARTESIAN_POINT('Ctrl Pts',(7.69469701891557,1.83726938337627,37.4321170855871));
#219900=CARTESIAN_POINT('Ctrl Pts',(7.64530872288838,2.04411328860228,37.440652297052));
#219901=CARTESIAN_POINT('Ctrl Pts',(7.58761999670923,2.24878002015923,37.4491875085169));
#219902=CARTESIAN_POINT('Ctrl Pts',(7.52185733897788,2.4506291380102,37.4577227199818));
#219903=CARTESIAN_POINT('Ctrl Pts',(7.4526488175824,2.66305484392548,37.4667051636004));
#219904=CARTESIAN_POINT('Ctrl Pts',(7.37449776855023,2.87235944314116,37.475687607219));
#219905=CARTESIAN_POINT('Ctrl Pts',(7.28772418927061,3.0778234421617,37.4846700508377));
#219906=CARTESIAN_POINT('Ctrl Pts',(7.20492491685308,3.27387700786832,37.493241090575));
#219907=CARTESIAN_POINT('Ctrl Pts',(7.11427539764419,3.46643371593889,37.5018121303123));
#219908=CARTESIAN_POINT('Ctrl Pts',(7.01610015978658,3.65489528548257,37.5103831700496));
#219909=CARTESIAN_POINT('Ctrl Pts',(6.91780172970799,3.84359334031346,37.5189649648963));
#219910=CARTESIAN_POINT('Ctrl Pts',(6.81195883449633,4.02818577239186,37.527546759743));
#219911=CARTESIAN_POINT('Ctrl Pts',(6.69894048499784,4.20810139830981,37.5361285545897));
#219912=CARTESIAN_POINT('Ctrl Pts',(6.58573309115283,4.38831796679222,37.5447247040947));
#219913=CARTESIAN_POINT('Ctrl Pts',(6.46532638008344,4.5638418784101,37.5533208535998));
#219914=CARTESIAN_POINT('Ctrl Pts',(6.33813223962513,4.7341314634286,37.5619170031049));
#219915=CARTESIAN_POINT('Ctrl Pts',(6.32040073240938,4.75787069382586,37.5631153498717));
#219916=CARTESIAN_POINT('Ctrl Pts',(6.30253738256674,4.78150825552507,37.5643136966385));
#219917=CARTESIAN_POINT('Ctrl Pts',(6.28454336630384,4.80504273415403,37.5655120434053));
#219918=CARTESIAN_POINT('Ctrl Pts',(6.16580187356797,4.96034542380006,37.5734198657519));
#219919=CARTESIAN_POINT('Ctrl Pts',(6.04114830945474,5.11144271903652,37.5813276880984));
#219920=CARTESIAN_POINT('Ctrl Pts',(5.91091118070632,5.25785602824963,37.589235510445));
#219921=CARTESIAN_POINT('Ctrl Pts',(5.78080710596087,5.40411975740776,37.5971352539323));
#219922=CARTESIAN_POINT('Ctrl Pts',(5.64513105637164,5.54570877677501,37.6050349974197));
#219923=CARTESIAN_POINT('Ctrl Pts',(5.50425363886146,5.68217501306325,37.6129347409071));
#219924=CARTESIAN_POINT('Ctrl Pts',(5.3634939866952,5.81852717149903,37.6208278806675));
#219925=CARTESIAN_POINT('Ctrl Pts',(5.21754187482366,5.94976483924279,37.6287210204279));
#219926=CARTESIAN_POINT('Ctrl Pts',(5.06680701991465,6.07547427144117,37.6366141601883));
#219927=CARTESIAN_POINT('Ctrl Pts',(4.9161701888471,6.20110195399076,37.6445021669893));
#219928=CARTESIAN_POINT('Ctrl Pts',(4.76075707549972,6.32120834360865,37.6523901737904));
#219929=CARTESIAN_POINT('Ctrl Pts',(4.60101316751264,6.43541753364732,37.6602781805914));
#219930=CARTESIAN_POINT('Ctrl Pts',(4.44134349376458,6.54957364978527,37.6681625217742));
#219931=CARTESIAN_POINT('Ctrl Pts',(4.27734731577844,6.65783782706723,37.676046862957));
#219932=CARTESIAN_POINT('Ctrl Pts',(4.10950223537964,6.75987517469145,37.6839312041398));
#219933=CARTESIAN_POINT('Ctrl Pts',(3.94170400661599,6.86188403999989,37.6918133445177));
#219934=CARTESIAN_POINT('Ctrl Pts',(3.77005931122769,6.95766936099216,37.6996954848956));
#219935=CARTESIAN_POINT('Ctrl Pts',(3.59507392359959,7.04694007948516,37.7075776252735));
#219936=CARTESIAN_POINT('Ctrl Pts',(3.42006940244416,7.13622055915739,37.7154606275128));
#219937=CARTESIAN_POINT('Ctrl Pts',(3.24172376327543,7.21898485001104,37.7233436297521));
#219938=CARTESIAN_POINT('Ctrl Pts',(3.06056708707034,7.2949880127072,37.7312266319914));
#219939=CARTESIAN_POINT('Ctrl Pts',(2.87938856274774,7.3710003416459,37.7391105849478));
#219940=CARTESIAN_POINT('Ctrl Pts',(2.69539864384964,7.44024978345649,37.7469945379042));
#219941=CARTESIAN_POINT('Ctrl Pts',(2.50914705365698,7.50253970753401,37.7548784908607));
#219942=CARTESIAN_POINT('Ctrl Pts',(2.3228416786623,7.56484761938404,37.7627647205056));
#219943=CARTESIAN_POINT('Ctrl Pts',(2.13427365805966,7.62019189917519,37.7706509501505));
#219944=CARTESIAN_POINT('Ctrl Pts',(1.94400775272161,7.66842583959435,37.7785371797954));
#219945=CARTESIAN_POINT('Ctrl Pts',(1.75365490533875,7.71668182052256,37.7864270130546));
#219946=CARTESIAN_POINT('Ctrl Pts',(1.56160296125589,7.75782090296864,37.7943168463138));
#219947=CARTESIAN_POINT('Ctrl Pts',(1.36842698097498,7.79174746752869,37.802206679573));
#219948=CARTESIAN_POINT('Ctrl Pts',(1.17502821865124,7.82571315822309,37.8101056118577));
#219949=CARTESIAN_POINT('Ctrl Pts',(0.9805031706794,7.85244965697262,37.8180045441423));
#219950=CARTESIAN_POINT('Ctrl Pts',(0.78543329051248,7.87191308044968,37.825903476427));
#219951=CARTESIAN_POINT('Ctrl Pts',(0.590234569593391,7.89138935922822,
37.8338076258389));
#219952=CARTESIAN_POINT('Ctrl Pts',(0.39449064227463,7.90358296490442,37.8417117752508));
#219953=CARTESIAN_POINT('Ctrl Pts',(0.198783331142212,7.90850214561898,
37.8496159246627));
#219954=CARTESIAN_POINT('Ctrl Pts',(0.00280781021079834,7.91342806789298,
37.8575309064257));
#219955=CARTESIAN_POINT('Ctrl Pts',(-0.193130650653157,7.91105965676954,
37.8654458881888));
#219956=CARTESIAN_POINT('Ctrl Pts',(-0.388453799583046,7.90145712167,37.8733608699519));
#219957=CARTESIAN_POINT('Ctrl Pts',(-0.471205404976599,7.89738886248163,
37.8767141716529));
#219958=CARTESIAN_POINT('Ctrl Pts',(-0.553846669945976,7.89202276760672,
37.8800674733539));
#219959=CARTESIAN_POINT('Ctrl Pts',(-0.636334172624782,7.88536618177938,
37.8834207750549));
#219960=CARTESIAN_POINT('Ctrl Pts',(-0.827228526136434,7.86996136763375,
37.8911810580015));
#219961=CARTESIAN_POINT('Ctrl Pts',(-1.01789961082983,7.84759318625714,
37.8989413409481));
#219962=CARTESIAN_POINT('Ctrl Pts',(-1.20778625754698,7.81825897218049,
37.9067016238947));
#219963=CARTESIAN_POINT('Ctrl Pts',(-1.3974443661861,7.78896006329786,37.9144525669526));
#219964=CARTESIAN_POINT('Ctrl Pts',(-1.58631956594894,7.75271186340924,
37.9222035100104));
#219965=CARTESIAN_POINT('Ctrl Pts',(-1.77385152220997,7.70956365672879,
37.9299544530683));
#219966=CARTESIAN_POINT('Ctrl Pts',(-1.9611958377506,7.66645862327997,37.9376976406878));
#219967=CARTESIAN_POINT('Ctrl Pts',(-2.14719923865808,7.61646740642545,
37.9454408283072));
#219968=CARTESIAN_POINT('Ctrl Pts',(-2.33130724911348,7.55969096658263,
37.9531840159267));
#219969=CARTESIAN_POINT('Ctrl Pts',(-2.51526835852451,7.50295982905059,
37.9609210252036));
#219970=CARTESIAN_POINT('Ctrl Pts',(-2.69733674743482,7.43945435264161,
37.9686580344805));
#219971=CARTESIAN_POINT('Ctrl Pts',(-2.87696877445214,7.36932640550189,
37.9763950437574));
#219972=CARTESIAN_POINT('Ctrl Pts',(-3.056493840646,7.29924021563173,37.9841274460782));
#219973=CARTESIAN_POINT('Ctrl Pts',(-3.23358510038085,7.22253953731047,
37.9918598483989));
#219974=CARTESIAN_POINT('Ctrl Pts',(-3.40771462419382,7.13942589008777,
37.9995922507196));
#219975=CARTESIAN_POINT('Ctrl Pts',(-3.58177569346296,7.05634491685787,
38.0073216132452));
#219976=CARTESIAN_POINT('Ctrl Pts',(-3.75287702226877,6.96685615034051,
38.0150509757708));
#219977=CARTESIAN_POINT('Ctrl Pts',(-3.92051112403433,6.87120902944475,
38.0227803382964));
#219978=CARTESIAN_POINT('Ctrl Pts',(-4.08814516039471,6.77556194586727,
38.0305096978063));
#219979=CARTESIAN_POINT('Ctrl Pts',(-4.25231165492579,6.67375668066268,
38.0382390573162));
#219980=CARTESIAN_POINT('Ctrl Pts',(-4.41252782819546,6.5660885742884,38.0459684168261));
#219981=CARTESIAN_POINT('Ctrl Pts',(-4.57275203207569,6.45841507120158,
38.0536981637593));
#219982=CARTESIAN_POINT('Ctrl Pts',(-4.72902522157414,6.34487834135559,
38.0614279106924));
#219983=CARTESIAN_POINT('Ctrl Pts',(-4.88089386772019,6.22581689837176,
38.0691576576256));
#219984=CARTESIAN_POINT('Ctrl Pts',(-5.03279795397306,6.1067276711786,38.0768892083745));
#219985=CARTESIAN_POINT('Ctrl Pts',(-5.18029516725317,5.98211138501453,
38.0846207591234));
#219986=CARTESIAN_POINT('Ctrl Pts',(-5.32296528397476,5.85234667339517,
38.0923523098723));
#219987=CARTESIAN_POINT('Ctrl Pts',(-5.46569484505672,5.72252789452993,
38.1000870820183));
#219988=CARTESIAN_POINT('Ctrl Pts',(-5.60359303920781,5.58755666010915,
38.1078218541642));
#219989=CARTESIAN_POINT('Ctrl Pts',(-5.73627667674065,5.44784828054905,
38.1155566263102));
#219990=CARTESIAN_POINT('Ctrl Pts',(-5.86911853957823,5.3079732986758,38.1233006221758));
#219991=CARTESIAN_POINT('Ctrl Pts',(-5.99673317963242,5.16335015029389,
38.1310446180414));
#219992=CARTESIAN_POINT('Ctrl Pts',(-6.11877720864985,5.01442783086038,
38.1387886139071));
#219993=CARTESIAN_POINT('Ctrl Pts',(-6.2409004503644,4.86540885337093,38.1465376360145));
#219994=CARTESIAN_POINT('Ctrl Pts',(-6.35744566258698,4.71208543132804,
38.1542866581219));
#219995=CARTESIAN_POINT('Ctrl Pts',(-6.46811304319438,4.55493519827217,
38.1620356802293));
#219996=CARTESIAN_POINT('Ctrl Pts',(-6.57894954962902,4.39754480264065,
38.169796544668));
#219997=CARTESIAN_POINT('Ctrl Pts',(-6.68389008910803,4.23631621542687,
38.1775574091066));
#219998=CARTESIAN_POINT('Ctrl Pts',(-6.78268043334072,4.07175234256418,
38.1853182735452));
#219999=CARTESIAN_POINT('Ctrl Pts',(-6.85061767787057,3.95858322509337,
38.1906553512649));
#220000=CARTESIAN_POINT('Ctrl Pts',(-6.9156473584285,3.84383726930316,38.1959924289847));
#220001=CARTESIAN_POINT('Ctrl Pts',(-6.97770016626062,3.72768311284188,
38.2013295067044));
#220002=CARTESIAN_POINT('Ctrl Pts',(-7.07871441134965,3.53859860822715,
38.2100176047241));
#220003=CARTESIAN_POINT('Ctrl Pts',(-7.17210872623232,3.34527559886758,
38.2187057027438));
#220004=CARTESIAN_POINT('Ctrl Pts',(-7.25754798714799,3.14831990341581,
38.2273938007634));
#220005=CARTESIAN_POINT('Ctrl Pts',(-7.34282980133001,2.95172715622213,
38.2360658884309));
#220006=CARTESIAN_POINT('Ctrl Pts',(-7.42018572299943,2.75151529464273,
38.2447379760985));
#220007=CARTESIAN_POINT('Ctrl Pts',(-7.48932709473185,2.54831329865765,
38.253410063766));
#220008=CARTESIAN_POINT('Ctrl Pts',(-7.55859694649434,2.3447337082179,38.2620982660991));
#220009=CARTESIAN_POINT('Ctrl Pts',(-7.61962154043449,2.13815305182341,
38.2707864684322));
#220010=CARTESIAN_POINT('Ctrl Pts',(-7.67215758315153,1.929227570633,38.2794746707653));
#220011=CARTESIAN_POINT('Ctrl Pts',(-7.72432902666704,1.72175202856402,
38.2881025771289));
#220012=CARTESIAN_POINT('Ctrl Pts',(-7.76812926263982,1.51196432347098,
38.2967304834924));
#220013=CARTESIAN_POINT('Ctrl Pts',(-7.80336783994071,1.30052733711331,
38.3053583898559));
#220014=CARTESIAN_POINT('Ctrl Pts',(-7.83897581349406,1.08687391534949,
38.3140767401738));
#220015=CARTESIAN_POINT('Ctrl Pts',(-7.86584148296301,0.87153664402298,
38.3227950904917));
#220016=CARTESIAN_POINT('Ctrl Pts',(-7.88381960402942,0.655217102280911,
38.3315134408096));
#220017=CARTESIAN_POINT('Ctrl Pts',(-7.90179772509583,0.438897560538843,
38.3402317911275));
#220018=CARTESIAN_POINT('Ctrl Pts',(-7.91088819026632,0.221595984180793,
38.3489501414454));
#220019=CARTESIAN_POINT('Ctrl Pts',(-7.91099897442464,0.00402823191254809,
38.3576684917633));
#220020=CARTESIAN_POINT('',(-7.92439853970512,0.00241054887052533,42.3578451112103));
#220021=CARTESIAN_POINT('Ctrl Pts',(-7.91099999125534,0.000371964958585618,
38.3666382661385));
#220022=CARTESIAN_POINT('Ctrl Pts',(-7.91100271520357,-0.0575613265987164,
38.3690406849655));
#220023=CARTESIAN_POINT('Ctrl Pts',(-7.9103690600493,-0.115493823804628,
38.3714232920843));
#220024=CARTESIAN_POINT('Ctrl Pts',(-7.90838440824614,-0.206009619986472,
38.3751157245008));
#220025=CARTESIAN_POINT('Ctrl Pts',(-7.90746825211672,-0.238599637850203,
38.3764390523976));
#220026=CARTESIAN_POINT('Ctrl Pts',(-7.90596219549245,-0.282508723941569,
38.3782138863615));
#220027=CARTESIAN_POINT('Ctrl Pts',(-7.90554940551862,-0.293833309801218,
38.3786709066768));
#220028=CARTESIAN_POINT('Ctrl Pts',(-7.90480709229007,-0.313062983095493,
38.3794457228368));
#220029=CARTESIAN_POINT('Ctrl Pts',(-7.90449004101174,-0.320968518269954,
38.379763906663));
#220030=CARTESIAN_POINT('Ctrl Pts',(-7.90388018161711,-0.335625904036209,
38.3803531916325));
#220031=CARTESIAN_POINT('Ctrl Pts',(-7.90359058040864,-0.342377876603587,
38.3806243923135));
#220032=CARTESIAN_POINT('Ctrl Pts',(-7.90299231014186,-0.355921003355959,
38.3811678576104));
#220033=CARTESIAN_POINT('Ctrl Pts',(-7.90268353872469,-0.362712147380527,
38.3814401188041));
#220034=CARTESIAN_POINT('Ctrl Pts',(-7.90194822328956,-0.378437955671679,
38.3820699835571));
#220035=CARTESIAN_POINT('Ctrl Pts',(-7.90151527853552,-0.387372319072966,
38.3824273878951));
#220036=CARTESIAN_POINT('Ctrl Pts',(-7.90038089752371,-0.409988231430878,
38.3833309855707));
#220037=CARTESIAN_POINT('Ctrl Pts',(-7.89965907279563,-0.423668752526804,
38.3838765454769));
#220038=CARTESIAN_POINT('Ctrl Pts',(-7.89555229742595,-0.497840948260592,
38.3868288902424));
#220039=CARTESIAN_POINT('Ctrl Pts',(-7.8915080159501,-0.558294839597717,
38.3892151939417));
#220040=CARTESIAN_POINT('Ctrl Pts',(-7.88350108713109,-0.6603622260029,
38.393212241086));
#220041=CARTESIAN_POINT('Ctrl Pts',(-7.87990242229589,-0.702001096365646,
38.3948338789408));
#220042=CARTESIAN_POINT('Ctrl Pts',(-7.78940110074119,-1.66054947662174,
38.4319683124899));
#220043=CARTESIAN_POINT('Ctrl Pts',(-7.54340726935622,-2.55517792037413,
38.4615223651022));
#220044=CARTESIAN_POINT('Ctrl Pts',(-7.11896055711377,-3.45098212916863,
38.4975134515376));
#220045=CARTESIAN_POINT('Ctrl Pts',(-7.08796926483968,-3.51419528037316,
38.5000954516352));
#220046=CARTESIAN_POINT('Ctrl Pts',(-6.98097220032684,-3.72526300089221,
38.5088835234331));
#220047=CARTESIAN_POINT('Ctrl Pts',(-6.90116232317098,-3.87111269627868,
38.515250026745));
#220048=CARTESIAN_POINT('Ctrl Pts',(-6.80002871001735,-4.0428484989135,
38.523151571807));
#220049=CARTESIAN_POINT('Ctrl Pts',(-6.78307074601405,-4.07123637943482,
38.5244703690638));
#220050=CARTESIAN_POINT('Ctrl Pts',(-6.76017316436285,-4.10902706686521,
38.5262422827698));
#220051=CARTESIAN_POINT('Ctrl Pts',(-6.7543908401765,-4.11852510312975,
38.5266890071502));
#220052=CARTESIAN_POINT('Ctrl Pts',(-6.74481490552963,-4.13418011093671,
38.5274275699904));
#220053=CARTESIAN_POINT('Ctrl Pts',(-6.741032833677,-4.14034414444287,38.5277189519936));
#220054=CARTESIAN_POINT('Ctrl Pts',(-6.73365166125648,-4.1523370810343,
38.5282869916163));
#220055=CARTESIAN_POINT('Ctrl Pts',(-6.73005343015131,-4.15816651382083,
38.528563615347));
#220056=CARTESIAN_POINT('Ctrl Pts',(-6.72167408808717,-4.17170237453172,
38.5292071201259));
#220057=CARTESIAN_POINT('Ctrl Pts',(-6.71688729251227,-4.17940526236564,
38.5295742180452));
#220058=CARTESIAN_POINT('Ctrl Pts',(-6.70128749956797,-4.20441234950533,
38.530768869808));
#220059=CARTESIAN_POINT('Ctrl Pts',(-6.690420837446,-4.22168288320633,38.5315984245083));
#220060=CARTESIAN_POINT('Ctrl Pts',(-6.57057832438846,-4.41052538393717,
38.5407172316674));
#220061=CARTESIAN_POINT('Ctrl Pts',(-6.4550989127875,-4.57787355432885,
38.5492327207875));
#220062=CARTESIAN_POINT('Ctrl Pts',(-6.04559034718836,-5.12496746765744,
38.5782338796753));
#220063=CARTESIAN_POINT('Ctrl Pts',(-5.72347520198491,-5.48236237008008,
38.5990891690844));
#220064=CARTESIAN_POINT('Ctrl Pts',(-4.87310576715638,-6.26869387387898,
38.6484651614694));
#220065=CARTESIAN_POINT('Ctrl Pts',(-4.31813371183424,-6.66314139238969,
38.6764608749002));
#220066=CARTESIAN_POINT('Ctrl Pts',(-3.6565655008636,-7.01559423391413,
38.7069170972005));
#220067=CARTESIAN_POINT('Ctrl Pts',(-3.59300596085827,-7.04835739684581,
38.7098130697934));
#220068=CARTESIAN_POINT('Ctrl Pts',(-3.50316297181426,-7.09313782991565,
38.7138647255688));
#220069=CARTESIAN_POINT('Ctrl Pts',(-3.47724487160706,-7.10587948053701,
38.715028728308));
#220070=CARTESIAN_POINT('Ctrl Pts',(-3.432733747905,-7.12745984222853,38.7170195510794));
#220071=CARTESIAN_POINT('Ctrl Pts',(-3.41417496050453,-7.13636841317174,
38.7178471910449));
#220072=CARTESIAN_POINT('Ctrl Pts',(-3.37877152905703,-7.15319301776245,
38.719421435893));
#220073=CARTESIAN_POINT('Ctrl Pts',(-3.3619333131652,-7.16112224409712,
38.7201681945741));
#220074=CARTESIAN_POINT('Ctrl Pts',(-3.32264080803551,-7.17945621241007,
38.721906228771));
#220075=CARTESIAN_POINT('Ctrl Pts',(-3.30016534542252,-7.18981516751878,
38.7228969428637));
#220076=CARTESIAN_POINT('Ctrl Pts',(-3.26052548909528,-7.20786016832306,
38.7246382596247));
#220077=CARTESIAN_POINT('Ctrl Pts',(-3.24338162372294,-7.21559078082115,
38.7253893981968));
#220078=CARTESIAN_POINT('Ctrl Pts',(-3.12052734476668,-7.27046264375817,
38.7307581977238));
#220079=CARTESIAN_POINT('Ctrl Pts',(-3.01382024168068,-7.31534045871677,
38.7353475410548));
#220080=CARTESIAN_POINT('Ctrl Pts',(-2.23422058661147,-7.6232622653596,
38.7683875594053));
#220081=CARTESIAN_POINT('Ctrl Pts',(-1.52911817523031,-7.79535729482972,
38.7953257885712));
#220082=CARTESIAN_POINT('Ctrl Pts',(-0.720756914736055,-7.87861481531954,
38.8273359660099));
#220083=CARTESIAN_POINT('Ctrl Pts',(-0.630854176453375,-7.88632262198436,
38.830916309755));
#220084=CARTESIAN_POINT('Ctrl Pts',(-0.521912899122263,-7.89378792888539,
38.8352930736138));
#220085=CARTESIAN_POINT('Ctrl Pts',(-0.502980753681077,-7.89501686495704,
38.8360550966044));
#220086=CARTESIAN_POINT('Ctrl Pts',(-0.472764132041824,-7.89686917682917,
38.8372736385121));
#220087=CARTESIAN_POINT('Ctrl Pts',(-0.461482510633819,-7.8975364900623,
38.8377290975011));
#220088=CARTESIAN_POINT('Ctrl Pts',(-0.440053325420325,-7.89875796252408,
38.8385951670821));
#220089=CARTESIAN_POINT('Ctrl Pts',(-0.429906042740363,-7.89931674725418,
38.8390056720697));
#220090=CARTESIAN_POINT('Ctrl Pts',(-0.406840797752764,-7.90054231578217,
38.8399396514505));
#220091=CARTESIAN_POINT('Ctrl Pts',(-0.393922229818125,-7.90119697220654,
38.8404633910863));
#220092=CARTESIAN_POINT('Ctrl Pts',(-0.360495683730597,-7.90280870036098,
38.8418201318137));
#220093=CARTESIAN_POINT('Ctrl Pts',(-0.339985519612715,-7.90371762738879,
38.8426541459414));
#220094=CARTESIAN_POINT('Ctrl Pts',(-0.212138288763526,-7.9088847327349,
38.8478619099687));
#220095=CARTESIAN_POINT('Ctrl Pts',(-0.104728643885638,-7.91103606682353,
38.8522768196841));
#220096=CARTESIAN_POINT('Ctrl Pts',(0.269888492743345,-7.91090869061913,
38.8677759941054));
#220097=CARTESIAN_POINT('Ctrl Pts',(0.536907991786122,-7.89728071512809,
38.878998287945));
#220098=CARTESIAN_POINT('Ctrl Pts',(1.17548499987085,-7.83214875715672,
38.9059645797674));
#220099=CARTESIAN_POINT('Ctrl Pts',(1.54508422159397,-7.76769239284312,
38.9216646679157));
#220100=CARTESIAN_POINT('Ctrl Pts',(2.08565917721932,-7.63329463885581,
38.9446156192098));
#220101=CARTESIAN_POINT('Ctrl Pts',(2.26102071893566,-7.58320173009643,
38.9520632859458));
#220102=CARTESIAN_POINT('Ctrl Pts',(2.47767115759562,-7.51313021395045,
38.9612838798034));
#220103=CARTESIAN_POINT('Ctrl Pts',(2.52072430977822,-7.49879516725812,
38.9631172610841));
#220104=CARTESIAN_POINT('Ctrl Pts',(2.58927957279897,-7.47531177522488,
38.9660388729488));
#220105=CARTESIAN_POINT('Ctrl Pts',(2.61486203976945,-7.46640150018851,
38.9671296217264));
#220106=CARTESIAN_POINT('Ctrl Pts',(2.66326573892189,-7.44926339170212,
38.9691945080094));
#220107=CARTESIAN_POINT('Ctrl Pts',(2.68609586863034,-7.44106164897747,
38.9701689080954));
#220108=CARTESIAN_POINT('Ctrl Pts',(2.73794074019937,-7.42216664331352,
38.9723829014106));
#220109=CARTESIAN_POINT('Ctrl Pts',(2.76693126057956,-7.41140800292276,
38.9736217986367));
#220110=CARTESIAN_POINT('Ctrl Pts',(2.85592775459304,-7.37778564684661,
38.9774281968979));
#220111=CARTESIAN_POINT('Ctrl Pts',(2.91571920133957,-7.35436101920162,
38.9799899307979));
#220112=CARTESIAN_POINT('Ctrl Pts',(3.0604552529429,-7.29561489774216,38.986205572551));
#220113=CARTESIAN_POINT('Ctrl Pts',(3.1450819346465,-7.25953461951917,38.9898520929798));
#220114=CARTESIAN_POINT('Ctrl Pts',(3.41976419997844,-7.13671998058995,
39.0017453460508));
#220115=CARTESIAN_POINT('Ctrl Pts',(3.60701978363886,-7.04393144972072,
39.0099542913002));
#220116=CARTESIAN_POINT('Ctrl Pts',(4.31233168883667,-6.65892784241672,
39.0412100602678));
#220117=CARTESIAN_POINT('Ctrl Pts',(4.8004908165499,-6.31607764594432,39.0633350943303));
#220118=CARTESIAN_POINT('Ctrl Pts',(5.46689748272606,-5.72576036371308,
39.0963879917825));
#220119=CARTESIAN_POINT('Ctrl Pts',(5.677001770324,-5.51751216030138,39.1073702202544));
#220120=CARTESIAN_POINT('Ctrl Pts',(5.97080660544676,-5.19171217778812,
39.1242178287143));
#220121=CARTESIAN_POINT('Ctrl Pts',(6.06375507665267,-5.08284159513783,
39.1297998753315));
#220122=CARTESIAN_POINT('Ctrl Pts',(6.16368103374691,-4.9591541183792,39.1361541653297));
#220123=CARTESIAN_POINT('Ctrl Pts',(6.17362877195611,-4.94676472427187,
39.1367907973691));
#220124=CARTESIAN_POINT('Ctrl Pts',(6.18839703962758,-4.92825767805735,
39.1377421230619));
#220125=CARTESIAN_POINT('Ctrl Pts',(6.19324600090646,-4.92216269876513,
39.138055480075));
#220126=CARTESIAN_POINT('Ctrl Pts',(6.20152423659714,-4.91172563937437,
39.1385921830369));
#220127=CARTESIAN_POINT('Ctrl Pts',(6.20495797692332,-4.90738709681956,
39.138815315389));
#220128=CARTESIAN_POINT('Ctrl Pts',(6.21197910980657,-4.89849672123536,
39.1392726230588));
#220129=CARTESIAN_POINT('Ctrl Pts',(6.21556605670109,-4.89394454230649,
39.1395068196496));
#220130=CARTESIAN_POINT('Ctrl Pts',(6.22412194577437,-4.88306172105563,
39.1400668133257));
#220131=CARTESIAN_POINT('Ctrl Pts',(6.22908623061827,-4.87672743737101,
39.1403928380221));
#220132=CARTESIAN_POINT('Ctrl Pts',(6.24406681195771,-4.8575524554928,39.1413800576716));
#220133=CARTESIAN_POINT('Ctrl Pts',(6.25405309401799,-4.84468844219225,
39.1420427453491));
#220134=CARTESIAN_POINT('Ctrl Pts',(6.39114836767435,-4.66695636702513,
39.1512051820283));
#220135=CARTESIAN_POINT('Ctrl Pts',(6.51171854436379,-4.49719444148638,
39.1600827168072));
#220136=CARTESIAN_POINT('Ctrl Pts',(7.05173089917422,-3.6695488224066,39.2035578025975));
#220137=CARTESIAN_POINT('Ctrl Pts',(7.379054417748,-2.95672873120676,39.2409017257229));
#220138=CARTESIAN_POINT('Ctrl Pts',(7.68024011589105,-1.9202371514314,39.2884241153686));
#220139=CARTESIAN_POINT('Ctrl Pts',(7.74735464126035,-1.62847140738848,
39.301174309276));
#220140=CARTESIAN_POINT('Ctrl Pts',(7.80310647979635,-1.30247694968702,
39.314709516951));
#220141=CARTESIAN_POINT('Ctrl Pts',(7.80824025664181,-1.27133829603604,
39.3159954471475));
#220142=CARTESIAN_POINT('Ctrl Pts',(7.81572572646455,-1.2241791143627,39.3179325925056));
#220143=CARTESIAN_POINT('Ctrl Pts',(7.81821476286821,-1.20818088915252,
39.3185879432793));
#220144=CARTESIAN_POINT('Ctrl Pts',(7.82217286480417,-1.18221578633447,
39.319648669934));
#220145=CARTESIAN_POINT('Ctrl Pts',(7.82367202981318,-1.17225358314323,
39.3200549525274));
#220146=CARTESIAN_POINT('Ctrl Pts',(7.82651310842613,-1.15312591211613,
39.3208337000043));
#220147=CARTESIAN_POINT('Ctrl Pts',(7.82785796130529,-1.14396090139137,
39.321206252941));
#220148=CARTESIAN_POINT('Ctrl Pts',(7.83024356812774,-1.12750208245547,
39.3218742526899));
#220149=CARTESIAN_POINT('Ctrl Pts',(7.83129023488242,-1.12020914990784,
39.3221698772805));
#220150=CARTESIAN_POINT('Ctrl Pts',(7.83335681930409,-1.10566521083275,
39.3227586973428));
#220151=CARTESIAN_POINT('Ctrl Pts',(7.83437686073325,-1.098414230298,39.3230518962471));
#220152=CARTESIAN_POINT('Ctrl Pts',(7.83684417182053,-1.08069702626316,
39.323767425465));
#220153=CARTESIAN_POINT('Ctrl Pts',(7.83828054565859,-1.07022928600295,
39.3241894275831));
#220154=CARTESIAN_POINT('Ctrl Pts',(7.84367300623051,-1.03033789156443,
39.3257947926687));
#220155=CARTESIAN_POINT('Ctrl Pts',(7.84748444372987,-1.00089476382841,
39.3269738031868));
#220156=CARTESIAN_POINT('Ctrl Pts',(7.90924919453521,-0.501710311019217,
39.3468651678445));
#220157=CARTESIAN_POINT('Ctrl Pts',(7.92510132197997,-0.027706405577548,
39.3642113656409));
#220158=CARTESIAN_POINT('Ctrl Pts',(7.86938845878505,0.961356924089496,
39.3991103625044));
#220159=CARTESIAN_POINT('Ctrl Pts',(7.78971844561418,1.4736817027025,39.4164568344321));
#220160=CARTESIAN_POINT('Ctrl Pts',(7.64562512745606,2.03271899099538,39.4370736695871));
#220161=CARTESIAN_POINT('Ctrl Pts',(7.6299685321875,2.09072000372798,39.4392345089688));
#220162=CARTESIAN_POINT('Ctrl Pts',(7.55235467016894,2.36575607206893,39.4496049411629));
#220163=CARTESIAN_POINT('Ctrl Pts',(7.48179207598633,2.58023984417568,39.4580605834728));
#220164=CARTESIAN_POINT('Ctrl Pts',(7.3904863048398,2.82236216501128,39.4682943514352));
#220165=CARTESIAN_POINT('Ctrl Pts',(7.37861624582227,2.85325046568614,39.4696131354601));
#220166=CARTESIAN_POINT('Ctrl Pts',(7.36313698551467,2.89278802037589,39.4713174113298));
#220167=CARTESIAN_POINT('Ctrl Pts',(7.35970550930436,2.90150712793873,39.4716942651444));
#220168=CARTESIAN_POINT('Ctrl Pts',(7.35416030718162,2.91552391681494,39.4723017025418));
#220169=CARTESIAN_POINT('Ctrl Pts',(7.35205632132558,2.92082546227149,39.4725318234672));
#220170=CARTESIAN_POINT('Ctrl Pts',(7.34804438438703,2.93090279155142,39.4729699432471));
#220171=CARTESIAN_POINT('Ctrl Pts',(7.34613750542787,2.93567900145971,39.4731778918163));
#220172=CARTESIAN_POINT('Ctrl Pts',(7.34178859231193,2.94654106827947,39.4736514840893));
#220173=CARTESIAN_POINT('Ctrl Pts',(7.33934364775402,2.95262575025401,39.4739172623778));
#220174=CARTESIAN_POINT('Ctrl Pts',(7.33206199778297,2.97068251169752,39.4747073987852));
#220175=CARTESIAN_POINT('Ctrl Pts',(7.32720355836226,2.98264576109962,39.4752327462041));
#220176=CARTESIAN_POINT('Ctrl Pts',(7.29357638235363,3.06487011503149,39.478856003977));
#220177=CARTESIAN_POINT('Ctrl Pts',(7.2638273512309,3.13472438617163,39.4819970277138));
#220178=CARTESIAN_POINT('Ctrl Pts',(7.22201098502701,3.22912139496021,39.4863174093829));
#220179=CARTESIAN_POINT('Ctrl Pts',(7.21081446849818,3.2540470696945,39.4874654820911));
#220180=CARTESIAN_POINT('Ctrl Pts',(7.18864687072568,3.30272031208883,39.4897209708892));
#220181=CARTESIAN_POINT('Ctrl Pts',(7.17768667474293,3.32647249719887,39.4908280191946));
#220182=CARTESIAN_POINT('Ctrl Pts',(7.15174932842089,3.38195709427862,39.4934283779987));
#220183=CARTESIAN_POINT('Ctrl Pts',(7.13667849656462,3.41364500864425,39.494924501378));
#220184=CARTESIAN_POINT('Ctrl Pts',(7.11700818813409,3.45430413118417,39.4968575736647));
#220185=CARTESIAN_POINT('Ctrl Pts',(7.1126015894661,3.46336847727902,39.4972893838175));
#220186=CARTESIAN_POINT('Ctrl Pts',(7.05330795713899,3.58474467753427,39.503082877715));
#220187=CARTESIAN_POINT('Ctrl Pts',(6.99578455521396,3.69574686964681,39.5085110742401));
#220188=CARTESIAN_POINT('Ctrl Pts',(6.78731004033436,4.07571518047886,39.5274538392275));
#220189=CARTESIAN_POINT('Ctrl Pts',(6.6232802705237,4.33718713788831,39.5411189842109));
#220190=CARTESIAN_POINT('Ctrl Pts',(6.14315761159606,5.01151661952922,39.5773561037032));
#220191=CARTESIAN_POINT('Ctrl Pts',(5.8009572889213,5.40394872300416,39.5994473775974));
#220192=CARTESIAN_POINT('Ctrl Pts',(5.39233664908235,5.78864138728636,39.6222005742356));
#220193=CARTESIAN_POINT('Ctrl Pts',(5.36171576013608,5.81701536834967,39.6238869032296));
#220194=CARTESIAN_POINT('Ctrl Pts',(5.31767323420031,5.85718289459712,39.6262864342426));
#220195=CARTESIAN_POINT('Ctrl Pts',(5.30443416596084,5.8691752630627,39.627004425174));
#220196=CARTESIAN_POINT('Ctrl Pts',(5.28147865477692,5.88982797914241,39.6282437393928));
#220197=CARTESIAN_POINT('Ctrl Pts',(5.27178126336351,5.89850936399747,39.628765556259));
#220198=CARTESIAN_POINT('Ctrl Pts',(5.25314535711491,5.91511009771673,39.6297650880353));
#220199=CARTESIAN_POINT('Ctrl Pts',(5.24421025113421,5.92303321397659,39.630242888993));
#220200=CARTESIAN_POINT('Ctrl Pts',(5.22316430207539,5.94161054399292,39.6313649834139));
#220201=CARTESIAN_POINT('Ctrl Pts',(5.21103873587482,5.95224801888364,39.6320088967503));
#220202=CARTESIAN_POINT('Ctrl Pts',(5.16947504556207,5.98848651671236,39.6342074015884));
#220203=CARTESIAN_POINT('Ctrl Pts',(5.13987995853597,6.0139069702918,39.6357580517973));
#220204=CARTESIAN_POINT('Ctrl Pts',(4.84207088466704,6.26590340091852,39.6512180939256));
#220205=CARTESIAN_POINT('Ctrl Pts',(4.55923559092939,6.47461083434499,39.6647163939174));
#220206=CARTESIAN_POINT('Ctrl Pts',(3.9335669978444,6.8749070762322,39.6926293775717));
#220207=CARTESIAN_POINT('Ctrl Pts',(3.58845862270875,7.0611801730281,39.7069267604959));
#220208=CARTESIAN_POINT('Ctrl Pts',(2.8740147650569,7.38084607139559,39.7357542371441));
#220209=CARTESIAN_POINT('Ctrl Pts',(2.50572392121636,7.51386460852727,39.7502518971484));
#220210=CARTESIAN_POINT('Ctrl Pts',(2.08442051882942,7.63159667229031,39.7675485415777));
#220211=CARTESIAN_POINT('Ctrl Pts',(2.03959589143796,7.6436983954947,39.7693978818927));
#220212=CARTESIAN_POINT('Ctrl Pts',(1.98353662064013,7.6583050208189,39.771724332625));
#220213=CARTESIAN_POINT('Ctrl Pts',(1.97239906432514,7.66118106081746,39.7721872070834));
#220214=CARTESIAN_POINT('Ctrl Pts',(1.95476535337692,7.66569359491175,39.7729211614091));
#220215=CARTESIAN_POINT('Ctrl Pts',(1.94827330074194,7.66734615255485,39.7731916109767));
#220216=CARTESIAN_POINT('Ctrl Pts',(1.93610291201317,7.6704276803579,39.7736990643508));
#220217=CARTESIAN_POINT('Ctrl Pts',(1.93042507035832,7.67185859704151,39.773935990572));
#220218=CARTESIAN_POINT('Ctrl Pts',(1.91773826393014,7.67504092133412,39.774465808676));
#220219=CARTESIAN_POINT('Ctrl Pts',(1.91072848345521,7.67678903286731,39.7747588328634));
#220220=CARTESIAN_POINT('Ctrl Pts',(1.89305550956257,7.68117064495437,39.7754983412253));
#220221=CARTESIAN_POINT('Ctrl Pts',(1.88238922872612,7.68379153993196,39.7759453391509));
#220222=CARTESIAN_POINT('Ctrl Pts',(1.82561207215154,7.69761737991473,39.7783284695209));
#220223=CARTESIAN_POINT('Ctrl Pts',(1.77940722168193,7.70842931880425,39.7802809489069));
#220224=CARTESIAN_POINT('Ctrl Pts',(0.948814859251304,7.89492232092405,
39.8156503759892));
#220225=CARTESIAN_POINT('Ctrl Pts',(0.142344382455355,7.95044911474386,
39.8544822232692));
#220226=CARTESIAN_POINT('Ctrl Pts',(-1.0248819715523,7.85293830026884,39.9069327330826));
#220227=CARTESIAN_POINT('Ctrl Pts',(-1.38861581272634,7.79684655180978,
39.9228169576492));
#220228=CARTESIAN_POINT('Ctrl Pts',(-1.79734250557897,7.7042928213546,39.939975799354));
#220229=CARTESIAN_POINT('Ctrl Pts',(-1.84740927995367,7.69244090304661,
39.94206624299));
#220230=CARTESIAN_POINT('Ctrl Pts',(-1.91025195217123,7.67691571485802,
39.9446759829438));
#220231=CARTESIAN_POINT('Ctrl Pts',(-1.92313837206761,7.67369768872882,
39.9452103822742));
#220232=CARTESIAN_POINT('Ctrl Pts',(-1.94361219817025,7.66853010625162,
39.9460582464532));
#220233=CARTESIAN_POINT('Ctrl Pts',(-1.95120489009336,7.66660171423512,
39.9463724164409));
#220234=CARTESIAN_POINT('Ctrl Pts',(-1.96548643812819,7.66295189631464,
39.9469628715697));
#220235=CARTESIAN_POINT('Ctrl Pts',(-1.97217592523177,7.66123298327091,
39.9472392403276));
#220236=CARTESIAN_POINT('Ctrl Pts',(-1.9871886150494,7.65735439611999,39.9478590238896));
#220237=CARTESIAN_POINT('Ctrl Pts',(-1.99551057103304,7.65518990627137,
39.9482022771631));
#220238=CARTESIAN_POINT('Ctrl Pts',(-2.01662415088057,7.64966162480336,
39.9490723596271));
#220239=CARTESIAN_POINT('Ctrl Pts',(-2.02941092152446,7.64627930785708,
39.9495985671355));
#220240=CARTESIAN_POINT('Ctrl Pts',(-2.09949205655606,7.62755348477661,
39.9524786103381));
#220241=CARTESIAN_POINT('Ctrl Pts',(-2.1566216854424,7.61159787202896,39.9548118121544));
#220242=CARTESIAN_POINT('Ctrl Pts',(-3.18384901983735,7.31221188895279,
39.996514440083));
#220243=CARTESIAN_POINT('Ctrl Pts',(-4.09073894759682,6.84622257074285,
40.0277405781552));
#220244=CARTESIAN_POINT('Ctrl Pts',(-5.11674070738103,6.04064065632391,
40.073635032168));
#220245=CARTESIAN_POINT('Ctrl Pts',(-5.33768091836027,5.84632416592615,
40.0844259993587));
#220246=CARTESIAN_POINT('Ctrl Pts',(-5.55791189271404,5.62972104465172,
40.0967720866748));
#220247=CARTESIAN_POINT('Ctrl Pts',(-5.56852046932466,5.61922800965859,
40.0973709143779));
#220248=CARTESIAN_POINT('Ctrl Pts',(-5.58312226727767,5.60470328812776,
40.0982009465838));
#220249=CARTESIAN_POINT('Ctrl Pts',(-5.58714099214233,5.60069716489918,
40.0984299981913));
#220250=CARTESIAN_POINT('Ctrl Pts',(-5.59390839776516,5.59393644766466,
40.0988167487078));
#220251=CARTESIAN_POINT('Ctrl Pts',(-5.59665936807869,5.59118413761223,
40.0989742529439));
#220252=CARTESIAN_POINT('Ctrl Pts',(-5.60209085489987,5.58574198060863,
40.0992858017266));
#220253=CARTESIAN_POINT('Ctrl Pts',(-5.60477146783886,5.58305223096501,
40.0994398379317));
#220254=CARTESIAN_POINT('Ctrl Pts',(-5.61067328222019,5.5771217665209,40.0997795874119));
#220255=CARTESIAN_POINT('Ctrl Pts',(-5.61389359422322,5.57388020959251,
40.0999653748072));
#220256=CARTESIAN_POINT('Ctrl Pts',(-5.62497167677132,5.5627097037452,40.1006058853756));
#220257=CARTESIAN_POINT('Ctrl Pts',(-5.63281542718606,5.55476695940392,
40.1010618029628));
#220258=CARTESIAN_POINT('Ctrl Pts',(-5.71360813305525,5.4726074939307,40.1057824964462));
#220259=CARTESIAN_POINT('Ctrl Pts',(-5.78509965841184,5.39697792538076,
40.1101673970241));
#220260=CARTESIAN_POINT('Ctrl Pts',(-5.87744926672617,5.29533927831622,
40.116080981103));
#220261=CARTESIAN_POINT('Ctrl Pts',(-5.89966736616873,5.27057424480898,
40.1175234538636));
#220262=CARTESIAN_POINT('Ctrl Pts',(-6.0374092888227,5.11508024181091,40.1265856923867));
#220263=CARTESIAN_POINT('Ctrl Pts',(-6.14873376321625,4.9807051936094,40.1344392800865));
#220264=CARTESIAN_POINT('Ctrl Pts',(-6.60146831300707,4.39589701321909,
40.1682930351166));
#220265=CARTESIAN_POINT('Ctrl Pts',(-6.89854733621004,3.9132363277899,40.1952973119054));
#220266=CARTESIAN_POINT('Ctrl Pts',(-7.22288530682164,3.23256725133725,
40.2293079155267));
#220267=CARTESIAN_POINT('Ctrl Pts',(-7.29797212619905,3.05927643789607,
40.237661179588));
#220268=CARTESIAN_POINT('Ctrl Pts',(-7.42232802915468,2.74156616301702,
40.2523816933558));
#220269=CARTESIAN_POINT('Ctrl Pts',(-7.47375679305211,2.59809573945222,
40.2588185355707));
#220270=CARTESIAN_POINT('Ctrl Pts',(-7.54530838423873,2.37873520591927,
40.2683427038426));
#220271=CARTESIAN_POINT('Ctrl Pts',(-7.56849760516399,2.30388895001688,
40.2715376683309));
#220272=CARTESIAN_POINT('Ctrl Pts',(-7.59472275158966,2.21457093857108,
40.2752869711011));
#220273=CARTESIAN_POINT('Ctrl Pts',(-7.59883439912788,2.20042129906829,
40.2758790536387));
#220274=CARTESIAN_POINT('Ctrl Pts',(-7.60510337470772,2.17862040125772,
40.2767884269391));
#220275=CARTESIAN_POINT('Ctrl Pts',(-7.60728873148677,2.17097727972219,
40.2771066994569));
#220276=CARTESIAN_POINT('Ctrl Pts',(-7.61109214888292,2.15759885350793,
40.2776628543255));
#220277=CARTESIAN_POINT('Ctrl Pts',(-7.6127152544861,2.15186499710866,40.2779009130775));
#220278=CARTESIAN_POINT('Ctrl Pts',(-7.6163668019076,2.13890953636076,40.2784381154137));
#220279=CARTESIAN_POINT('Ctrl Pts',(-7.61839145592972,2.1316868650393,40.2787371264134));
#220280=CARTESIAN_POINT('Ctrl Pts',(-7.62381538778137,2.11223131565829,
40.2795412797663));
#220281=CARTESIAN_POINT('Ctrl Pts',(-7.62719550144084,2.09999309110522,
40.2800457527841));
#220282=CARTESIAN_POINT('Ctrl Pts',(-7.64192742605976,2.0461490934733,40.2822592882439));
#220283=CARTESIAN_POINT('Ctrl Pts',(-7.65296847740238,2.00445864551502,
40.2839575193772));
#220284=CARTESIAN_POINT('Ctrl Pts',(-7.82779901257981,1.32179844281649,
40.3115158432425));
#220285=CARTESIAN_POINT('Ctrl Pts',(-7.91089925752325,0.662823887569133,
40.3342043247919));
#220286=CARTESIAN_POINT('Ctrl Pts',(-7.91108201108098,-0.538491210849919,
40.37501585252));
#220287=CARTESIAN_POINT('Ctrl Pts',(-7.85593626646437,-1.07671278173625,
40.3932271424114));
#220288=CARTESIAN_POINT('Ctrl Pts',(-7.73952615419851,-1.63854383578707,
40.4158612029801));
#220289=CARTESIAN_POINT('Ctrl Pts',(-7.73236927171654,-1.67199173718399,
40.4172229274171));
#220290=CARTESIAN_POINT('Ctrl Pts',(-7.72340608793648,-1.7125927078554,
40.4188943852793));
#220291=CARTESIAN_POINT('Ctrl Pts',(-7.72180630492352,-1.71979149043264,
40.4191914537871));
#220292=CARTESIAN_POINT('Ctrl Pts',(-7.7191413648481,-1.73170463689244,
40.41968423049));
#220293=CARTESIAN_POINT('Ctrl Pts',(-7.7180819449022,-1.73642029804808,
40.4198795914765));
#220294=CARTESIAN_POINT('Ctrl Pts',(-7.71615850065117,-1.74494534322553,
40.4202333103217));
#220295=CARTESIAN_POINT('Ctrl Pts',(-7.71529597389651,-1.7487550694953,
40.420391578355));
#220296=CARTESIAN_POINT('Ctrl Pts',(-7.71344347478094,-1.75690939350378,
40.4207307518267));
#220297=CARTESIAN_POINT('Ctrl Pts',(-7.71245265305085,-1.76125379486147,
40.4209117078258));
#220298=CARTESIAN_POINT('Ctrl Pts',(-7.70975832953071,-1.77302157596164,
40.4214025504843));
#220299=CARTESIAN_POINT('Ctrl Pts',(-7.70804778081875,-1.78044332019545,
40.4217128533897));
#220300=CARTESIAN_POINT('Ctrl Pts',(-7.69950107351774,-1.8172826828606,
40.4232567250017));
#220301=CARTESIAN_POINT('Ctrl Pts',(-7.69250729438803,-1.84666310110749,
40.4244994697214));
#220302=CARTESIAN_POINT('Ctrl Pts',(-7.63154129672951,-2.09642011987007,
40.4351572841536));
#220303=CARTESIAN_POINT('Ctrl Pts',(-7.56828327969176,-2.31440545813413,
40.4450785239092));
#220304=CARTESIAN_POINT('Ctrl Pts',(-7.36903943095525,-2.90486563161531,
40.4731184376421));
#220305=CARTESIAN_POINT('Ctrl Pts',(-7.21429198763766,-3.27031549342397,
40.4917630167172));
#220306=CARTESIAN_POINT('Ctrl Pts',(-6.87031834605332,-3.93809295397977,
40.5267444415144));
#220307=CARTESIAN_POINT('Ctrl Pts',(-6.68676627239349,-4.24229146828261,
40.5430806355035));
#220308=CARTESIAN_POINT('Ctrl Pts',(-6.47723856000872,-4.5419618196085,
40.5592768463925));
#220309=CARTESIAN_POINT('Ctrl Pts',(-6.47106140393932,-4.55075827105341,
40.5597523856308));
#220310=CARTESIAN_POINT('Ctrl Pts',(-6.41199761958388,-4.63450340596798,
40.5642807770836));
#220311=CARTESIAN_POINT('Ctrl Pts',(-6.35782810761078,-4.70854093618355,
40.5682925432195));
#220312=CARTESIAN_POINT('Ctrl Pts',(-6.16060544065873,-4.96848887811672,
40.5824011250004));
#220313=CARTESIAN_POINT('Ctrl Pts',(-6.01058144986155,-5.14896730418382,
40.5922352962012));
#220314=CARTESIAN_POINT('Ctrl Pts',(-5.83751511302868,-5.33927438751271,
40.6026612032246));
#220315=CARTESIAN_POINT('Ctrl Pts',(-5.82220934662197,-5.35596041949393,
40.6035758852737));
#220316=CARTESIAN_POINT('Ctrl Pts',(-5.80057857059859,-5.37933955388652,
40.6048582889587));
#220317=CARTESIAN_POINT('Ctrl Pts',(-5.79431326239355,-5.38608759747377,
40.6052285332949));
#220318=CARTESIAN_POINT('Ctrl Pts',(-5.78340820776284,-5.39779182562199,
40.605870882739));
#220319=CARTESIAN_POINT('Ctrl Pts',(-5.77877384275295,-5.40275299870337,
40.6061432156969));
#220320=CARTESIAN_POINT('Ctrl Pts',(-5.76910639553429,-5.41307550959544,
40.6067099644696));
#220321=CARTESIAN_POINT('Ctrl Pts',(-5.76407221127928,-5.4184358092643,
40.6070043330004));
#220322=CARTESIAN_POINT('Ctrl Pts',(-5.75218089085048,-5.43106212575577,
40.6076978844572));
#220323=CARTESIAN_POINT('Ctrl Pts',(-5.74531744274403,-5.43832219511873,
40.6080967978567));
#220324=CARTESIAN_POINT('Ctrl Pts',(-5.72275241163505,-5.46210080786379,
40.6094037668562));
#220325=CARTESIAN_POINT('Ctrl Pts',(-5.70699313414145,-5.47856457276963,
40.6103093554362));
#220326=CARTESIAN_POINT('Ctrl Pts',(-5.448101584998,-5.74670008974927,40.6250700818318));
#220327=CARTESIAN_POINT('Ctrl Pts',(-5.1885959736697,-5.98204608301881,
40.6381746923237));
#220328=CARTESIAN_POINT('Ctrl Pts',(-4.72124973395091,-6.35251392425787,
40.6596742533094));
#220329=CARTESIAN_POINT('Ctrl Pts',(-4.52111215866887,-6.49647458446487,
40.6683096877142));
#220330=CARTESIAN_POINT('Ctrl Pts',(-4.1214291799933,-6.75654085336454,
40.6848810477597));
#220331=CARTESIAN_POINT('Ctrl Pts',(-3.92288210991624,-6.87371933955018,
40.6928191560776));
#220332=CARTESIAN_POINT('Ctrl Pts',(-3.66502063653614,-7.01108805613906,
40.7030323030737));
#220333=CARTESIAN_POINT('Ctrl Pts',(-3.61019872986792,-7.03947420186448,
40.7051985147615));
#220334=CARTESIAN_POINT('Ctrl Pts',(-3.22853913631383,-7.23146199755547,
40.72027477787));
#220335=CARTESIAN_POINT('Ctrl Pts',(-2.89103775692214,-7.37288417780481,
40.7336328639309));
#220336=CARTESIAN_POINT('Ctrl Pts',(-2.52002064136027,-7.49894062262285,
40.7492130867442));
#220337=CARTESIAN_POINT('Ctrl Pts',(-2.49504425864787,-7.50728770076862,
40.7502650204757));
#220338=CARTESIAN_POINT('Ctrl Pts',(-2.46106023124157,-7.51845679796498,
40.751700166845));
#220339=CARTESIAN_POINT('Ctrl Pts',(-2.45208837107114,-7.5213876847459,
40.752079411001));
#220340=CARTESIAN_POINT('Ctrl Pts',(-2.43686760089633,-7.5263298087165,
40.7527233926932));
#220341=CARTESIAN_POINT('Ctrl Pts',(-2.43062138174445,-7.52834934047339,
40.7529878357527));
#220342=CARTESIAN_POINT('Ctrl Pts',(-2.4185822937369,-7.53222528155159,
40.7534978468833));
#220343=CARTESIAN_POINT('Ctrl Pts',(-2.41278978197055,-7.53408278899374,
40.7537433764912));
#220344=CARTESIAN_POINT('Ctrl Pts',(-2.39911006385869,-7.5384521235378,
40.7543235515642));
#220345=CARTESIAN_POINT('Ctrl Pts',(-2.39122105327994,-7.54095825417148,
40.7546583915292));
#220346=CARTESIAN_POINT('Ctrl Pts',(-2.36818304438918,-7.54823703515138,
40.75563693857));
#220347=CARTESIAN_POINT('Ctrl Pts',(-2.35302362921683,-7.55297643760833,
40.7562817541365));
#220348=CARTESIAN_POINT('Ctrl Pts',(-2.24236509798363,-7.58720696817183,
40.7609949470691));
#220349=CARTESIAN_POINT('Ctrl Pts',(-2.1463307324269,-7.61493101660534,
40.7651191011544));
#220350=CARTESIAN_POINT('Ctrl Pts',(-1.818167507871,-7.70296711661536,40.7792826212084));
#220351=CARTESIAN_POINT('Ctrl Pts',(-1.58383502304826,-7.75454039850525,
40.7895113506033));
#220352=CARTESIAN_POINT('Ctrl Pts',(-0.814949133076653,-7.88745178877353,
40.8229963049838));
#220353=CARTESIAN_POINT('Ctrl Pts',(-0.274309553465448,-7.92469760869911,
40.8463010789948));
#220354=CARTESIAN_POINT('Ctrl Pts',(0.335384128893991,-7.90419331282219,
40.8719167344252));
#220355=CARTESIAN_POINT('Ctrl Pts',(0.404834304556967,-7.90094068605221,
40.8748272482128));
#220356=CARTESIAN_POINT('Ctrl Pts',(0.908082551452367,-7.87071860796951,
40.8958739064551));
#220357=CARTESIAN_POINT('Ctrl Pts',(1.33906373592302,-7.80895323040188,
40.9137387684529));
#220358=CARTESIAN_POINT('Ctrl Pts',(1.82125838895418,-7.6987360311632,40.9338064528476));
#220359=CARTESIAN_POINT('Ctrl Pts',(1.87957671003879,-7.68470624387322,
40.9362332491362));
#220360=CARTESIAN_POINT('Ctrl Pts',(1.9635703156367,-7.66348634430565,40.9397281815936));
#220361=CARTESIAN_POINT('Ctrl Pts',(1.98937742553456,-7.65682759363849,
40.9408019660878));
#220362=CARTESIAN_POINT('Ctrl Pts',(2.0347587269758,-7.64487338589867,40.9426901642683));
#220363=CARTESIAN_POINT('Ctrl Pts',(2.05434710700069,-7.63963285309747,
40.9435051758945));
#220364=CARTESIAN_POINT('Ctrl Pts',(2.09478505724481,-7.62864760357231,
40.945187676698));
#220365=CARTESIAN_POINT('Ctrl Pts',(2.11563166134352,-7.62289258565481,
40.9460550426494));
#220366=CARTESIAN_POINT('Ctrl Pts',(2.16907465960688,-7.60790272752859,
40.9482786988633));
#220367=CARTESIAN_POINT('Ctrl Pts',(2.20163585725308,-7.59854383126085,
40.9496335519723));
#220368=CARTESIAN_POINT('Ctrl Pts',(2.33813513322191,-7.55835949700753,
40.9553137690073));
#220369=CARTESIAN_POINT('Ctrl Pts',(2.44149476556681,-7.52560814285373,
40.9596161189062));
#220370=CARTESIAN_POINT('Ctrl Pts',(2.70817216971802,-7.43503405254023,
40.9707309891727));
#220371=CARTESIAN_POINT('Ctrl Pts',(2.8703225289261,-7.37395266505057,40.9775027729984));
#220372=CARTESIAN_POINT('Ctrl Pts',(3.47687404875542,-7.12242583750333,
41.0029992525202));
#220373=CARTESIAN_POINT('Ctrl Pts',(3.90548841926288,-6.89672025093036,
41.0213029038865));
#220374=CARTESIAN_POINT('Ctrl Pts',(4.44457424347299,-6.54638300702135,
41.046350561226));
#220375=CARTESIAN_POINT('Ctrl Pts',(4.57567577731252,-6.45542869991477,
41.0526238538909));
#220376=CARTESIAN_POINT('Ctrl Pts',(4.72234670403155,-6.34695887931542,
41.0599239047219));
#220377=CARTESIAN_POINT('Ctrl Pts',(4.7406993924828,-6.33326256174149,41.0608425597413));
#220378=CARTESIAN_POINT('Ctrl Pts',(4.76877484565758,-6.31211988471779,
41.0622561541049));
#220379=CARTESIAN_POINT('Ctrl Pts',(4.7785401904589,-6.30473033638202,41.0627493701661));
#220380=CARTESIAN_POINT('Ctrl Pts',(4.79633378708911,-6.29120062918059,
41.0636508375065));
#220381=CARTESIAN_POINT('Ctrl Pts',(4.80436751289362,-6.28506769686039,
41.0640588814064));
#220382=CARTESIAN_POINT('Ctrl Pts',(4.82173909713339,-6.27175349047567,
41.064943432507));
#220383=CARTESIAN_POINT('Ctrl Pts',(4.83107270920755,-6.26456672431373,
41.0654200922201));
#220384=CARTESIAN_POINT('Ctrl Pts',(4.85686294025399,-6.24461664969128,
41.0667410099732));
#220385=CARTESIAN_POINT('Ctrl Pts',(4.8732852286146,-6.23180919130501,41.0675864576568));
#220386=CARTESIAN_POINT('Ctrl Pts',(4.96433863619142,-6.16021819455948,
41.072297762244));
#220387=CARTESIAN_POINT('Ctrl Pts',(5.03795590015163,-6.10015952217814,
41.0761958344638));
#220388=CARTESIAN_POINT('Ctrl Pts',(5.44846570641175,-5.75275565522514,
41.0984012099495));
#220389=CARTESIAN_POINT('Ctrl Pts',(5.76184621752423,-5.43885116326933,
41.1171385065488));
#220390=CARTESIAN_POINT('Ctrl Pts',(6.22086327210754,-4.8946135113089,41.1469272337747));
#220391=CARTESIAN_POINT('Ctrl Pts',(6.38379933645567,-4.68011672686343,
41.1581022538579));
#220392=CARTESIAN_POINT('Ctrl Pts',(6.54772380283569,-4.43978666836273,
41.1700292862554));
#220393=CARTESIAN_POINT('Ctrl Pts',(6.55988748812866,-4.42179474932165,
41.1709187760289));
#220394=CARTESIAN_POINT('Ctrl Pts',(6.63678071393931,-4.30704251078201,
41.1765704304468));
#220395=CARTESIAN_POINT('Ctrl Pts',(6.69944242153006,-4.20891258887597,
41.181306346304));
#220396=CARTESIAN_POINT('Ctrl Pts',(6.78087228530435,-4.07496251945919,
41.1876480776934));
#220397=CARTESIAN_POINT('Ctrl Pts',(6.80156439396075,-4.04033046915947,
41.1892769066331));
#220398=CARTESIAN_POINT('Ctrl Pts',(6.83383169090829,-3.9853748036672,41.1918450406949));
#220399=CARTESIAN_POINT('Ctrl Pts',(6.84558316382334,-3.96515561566891,
41.192786396983));
#220400=CARTESIAN_POINT('Ctrl Pts',(6.86816602078005,-3.92590068287647,
41.1946073451946));
#220401=CARTESIAN_POINT('Ctrl Pts',(6.87900834942608,-3.90687148399961,
41.1954870556991));
#220402=CARTESIAN_POINT('Ctrl Pts',(6.9046779314019,-3.86138106009618,41.1975830073545));
#220403=CARTESIAN_POINT('Ctrl Pts',(6.91943231099754,-3.8348790762309,41.1987984191924));
#220404=CARTESIAN_POINT('Ctrl Pts',(6.96346256409352,-3.75471001293163,
41.2024584876864));
#220405=CARTESIAN_POINT('Ctrl Pts',(6.99226922471156,-3.70078766129468,
41.2048980064924));
#220406=CARTESIAN_POINT('Ctrl Pts',(7.19015650595692,-3.31980769766959,
41.221987628562));
#220407=CARTESIAN_POINT('Ctrl Pts',(7.33685605418884,-2.9816156434677,41.2364668014338));
#220408=CARTESIAN_POINT('Ctrl Pts',(7.63687285613083,-2.13211085690407,
41.271280868553));
#220409=CARTESIAN_POINT('Ctrl Pts',(7.76308427169009,-1.6131531459468,41.2910642235314));
#220410=CARTESIAN_POINT('Ctrl Pts',(7.89494829331881,-0.661183439387172,
41.3267458755949));
#220411=CARTESIAN_POINT('Ctrl Pts',(7.91915967737508,-0.232877693956832,
41.3426309331704));
#220412=CARTESIAN_POINT('Ctrl Pts',(7.90804139615672,0.21747848682177,41.3605743133562));
#220413=CARTESIAN_POINT('Ctrl Pts',(7.90739875941743,0.239709122353434,
41.3614633513774));
#220414=CARTESIAN_POINT('Ctrl Pts',(7.90636380494532,0.270949640312946,
41.3627176842484));
#220415=CARTESIAN_POINT('Ctrl Pts',(7.90604980584113,0.279962123280698,
41.3630801251431));
#220416=CARTESIAN_POINT('Ctrl Pts',(7.90549211774436,0.295219294359333,
41.3636947106507));
#220417=CARTESIAN_POINT('Ctrl Pts',(7.90525643759748,0.301464278188743,
41.3639465565419));
#220418=CARTESIAN_POINT('Ctrl Pts',(7.90477522771567,0.313826513213213,
41.3644456756055));
#220419=CARTESIAN_POINT('Ctrl Pts',(7.90452999637114,0.319943772097463,
41.3646929373109));
#220420=CARTESIAN_POINT('Ctrl Pts',(7.90392160733752,0.334692177593052,
41.3652897608273));
#220421=CARTESIAN_POINT('Ctrl Pts',(7.90355141283754,0.343323014875956,
41.3656395929061));
#220422=CARTESIAN_POINT('Ctrl Pts',(7.90225653096316,0.372399800166932,
41.3668201171148));
#220423=CARTESIAN_POINT('Ctrl Pts',(7.90126664086971,0.392842654933553,
41.3676533679189));
#220424=CARTESIAN_POINT('Ctrl Pts',(7.8852524735081,0.698966067963113,41.380182642444));
#220425=CARTESIAN_POINT('Ctrl Pts',(7.85482572920474,0.983572604281911,
41.3926097470657));
#220426=CARTESIAN_POINT('Ctrl Pts',(7.65043768365785,2.24443644992404,41.449891458383));
#220427=CARTESIAN_POINT('Ctrl Pts',(7.30918761736838,3.18486130846244,41.4971408822131));
#220428=CARTESIAN_POINT('Ctrl Pts',(6.77571982784173,4.08367421582991,41.540008583662));
#220429=CARTESIAN_POINT('Ctrl Pts',(6.74799159735284,4.12933212863205,41.5421832711266));
#220430=CARTESIAN_POINT('Ctrl Pts',(6.71204451494971,4.18719423577374,41.5449359569383));
#220431=CARTESIAN_POINT('Ctrl Pts',(6.7042514950107,4.1996605854889,41.5455288255349));
#220432=CARTESIAN_POINT('Ctrl Pts',(6.69181667839155,4.21942951282276,41.5464686900694));
#220433=CARTESIAN_POINT('Ctrl Pts',(6.68719759135799,4.22674629539127,41.5468164835685));
#220434=CARTESIAN_POINT('Ctrl Pts',(6.67856158556983,4.24037641502107,41.5474642560565));
#220435=CARTESIAN_POINT('Ctrl Pts',(6.67454769801821,4.24669165593355,41.5477643413729));
#220436=CARTESIAN_POINT('Ctrl Pts',(6.66561609809459,4.26070022456332,41.5484298940697));
#220437=CARTESIAN_POINT('Ctrl Pts',(6.66069401124881,4.2683907576479,41.5487952063302));
#220438=CARTESIAN_POINT('Ctrl Pts',(6.6464136015203,4.29061838687088,41.5498508637549));
#220439=CARTESIAN_POINT('Ctrl Pts',(6.63702089926751,4.30513338835862,41.550539990002));
#220440=CARTESIAN_POINT('Ctrl Pts',(6.57244489428123,4.40421222518066,41.5552424584642));
#220441=CARTESIAN_POINT('Ctrl Pts',(6.51569343417278,4.48774522206117,41.5591995337757));
#220442=CARTESIAN_POINT('Ctrl Pts',(6.35453243946062,4.715455330846,41.5699790903228));
#220443=CARTESIAN_POINT('Ctrl Pts',(6.24683111850503,4.85723241383463,41.5766812082956));
#220444=CARTESIAN_POINT('Ctrl Pts',(6.023050648152,5.1320462388652,41.5897364929209));
#220445=CARTESIAN_POINT('Ctrl Pts',(5.90712016905897,5.2650709439302,41.5960885985373));
#220446=CARTESIAN_POINT('Ctrl Pts',(5.68994763933128,5.49805497148893,41.6073796448948));
#220447=CARTESIAN_POINT('Ctrl Pts',(5.59027474376821,5.5993697722298,41.6123514034159));
#220448=CARTESIAN_POINT('Ctrl Pts',(5.4535979885375,5.73100877098024,41.6189466392761));
#220449=CARTESIAN_POINT('Ctrl Pts',(5.41897183773035,5.76376064689435,41.6205993148689));
#220450=CARTESIAN_POINT('Ctrl Pts',(5.35387141337888,5.82423202378489,41.6236758602257));
#220451=CARTESIAN_POINT('Ctrl Pts',(5.32347252886368,5.85203024770597,41.6251002923482));
#220452=CARTESIAN_POINT('Ctrl Pts',(5.26574915612239,5.90399332994155,41.6277843320518));
#220453=CARTESIAN_POINT('Ctrl Pts',(5.23847196168647,5.92820908232838,41.6290441023104));
#220454=CARTESIAN_POINT('Ctrl Pts',(5.18522572474764,5.97482478721945,41.6314881897212));
#220455=CARTESIAN_POINT('Ctrl Pts',(5.15927657852703,5.9972462213741,41.6326724876556));
#220456=CARTESIAN_POINT('Ctrl Pts',(5.1086062635638,6.04045579855471,41.6349731706584));
#220457=CARTESIAN_POINT('Ctrl Pts',(5.08390195689247,6.06126266549168,41.6360894768823));
#220458=CARTESIAN_POINT('Ctrl Pts',(5.0355485660153,6.1014840642528,41.6382650616517));
#220459=CARTESIAN_POINT('Ctrl Pts',(5.01191290297839,6.12091383664271,41.6393242264894));
#220460=CARTESIAN_POINT('Ctrl Pts',(4.61684476853867,6.44185829776546,41.6569652991833));
#220461=CARTESIAN_POINT('Ctrl Pts',(4.2189603037467,6.70917871269953,41.6737852942337));
#220462=CARTESIAN_POINT('Ctrl Pts',(3.77328353440653,6.95321079794561,41.6939104568213));
#220463=CARTESIAN_POINT('Ctrl Pts',(3.74706508671286,6.96737484493203,41.6950989140428));
#220464=CARTESIAN_POINT('Ctrl Pts',(3.71263693429395,6.98572350423005,41.6966647805266));
#220465=CARTESIAN_POINT('Ctrl Pts',(3.70449880711223,6.99004252279446,41.6970353038563));
#220466=CARTESIAN_POINT('Ctrl Pts',(3.69136555731544,6.99698314606487,41.6976338470275));
#220467=CARTESIAN_POINT('Ctrl Pts',(3.68637512669243,6.99961364998906,41.6978614224354));
#220468=CARTESIAN_POINT('Ctrl Pts',(3.67693480431925,7.00457683859597,41.6982921786328));
#220469=CARTESIAN_POINT('Ctrl Pts',(3.67248549357513,7.00691062753917,41.6984953050114));
#220470=CARTESIAN_POINT('Ctrl Pts',(3.6624019328315,7.01218749670569,41.6989558914722));
#220471=CARTESIAN_POINT('Ctrl Pts',(3.65676635702034,7.01512802565935,41.6992134749696));
#220472=CARTESIAN_POINT('Ctrl Pts',(3.64015674522534,7.02376913034822,41.6999731247799));
#220473=CARTESIAN_POINT('Ctrl Pts',(3.62917291122858,7.02945075409312,41.7004760922341));
#220474=CARTESIAN_POINT('Ctrl Pts',(3.54487551154266,7.07280515276999,41.7043406622659));
#220475=CARTESIAN_POINT('Ctrl Pts',(3.47099211339649,7.10935498005472,41.707753551548));
#220476=CARTESIAN_POINT('Ctrl Pts',(3.21041319145589,7.23323209310508,41.7198463035516));
#220477=CARTESIAN_POINT('Ctrl Pts',(3.02089232249659,7.3144106419306,41.728738253241));
#220478=CARTESIAN_POINT('Ctrl Pts',(2.36015294890875,7.56736526403759,41.7596208291027));
#220479=CARTESIAN_POINT('Ctrl Pts',(1.87586435508062,7.70172146626963,41.7819601915515));
#220480=CARTESIAN_POINT('Ctrl Pts',(1.04187134182631,7.84970308737852,41.8183001021839));
#220481=CARTESIAN_POINT('Ctrl Pts',(0.698020577031019,7.88771995460522,
41.8327226117628));
#220482=CARTESIAN_POINT('Ctrl Pts',(0.319519857606371,7.9046148298508,41.8480649197127));
#220483=CARTESIAN_POINT('Ctrl Pts',(0.286263940302587,7.90588904074924,
41.8494086808059));
#220484=CARTESIAN_POINT('Ctrl Pts',(0.236392962909805,7.90748477521783,
41.851417759828));
#220485=CARTESIAN_POINT('Ctrl Pts',(0.219783438972896,7.90796385586357,
41.852085879521));
#220486=CARTESIAN_POINT('Ctrl Pts',(0.191105754536285,7.90870060710512,
41.8532377603289));
#220487=CARTESIAN_POINT('Ctrl Pts',(0.179038304844068,7.90898299331668,
41.8537219529738));
#220488=CARTESIAN_POINT('Ctrl Pts',(0.154053817537983,7.90951043551615,
41.8547233876408));
#220489=CARTESIAN_POINT('Ctrl Pts',(0.141136728312348,7.90975147101862,
41.8552405586643));
#220490=CARTESIAN_POINT('Ctrl Pts',(0.110917285840395,7.91024132290573,
41.8564491670535));
#220491=CARTESIAN_POINT('Ctrl Pts',(0.0936145758183488,7.91046501444356,
41.85714017413));
#220492=CARTESIAN_POINT('Ctrl Pts',(0.0379336129200809,7.91100215015645,
41.8593607597468));
#220493=CARTESIAN_POINT('Ctrl Pts',(-0.000446417369137525,7.91109308534335,
41.8608866579435));
#220494=CARTESIAN_POINT('Ctrl Pts',(-0.657937600988395,7.90786620402613,
41.8869514640247));
#220495=CARTESIAN_POINT('Ctrl Pts',(-1.27455985327542,7.83216355241303,
41.9100206344112));
#220496=CARTESIAN_POINT('Ctrl Pts',(-2.20124744488796,7.60595003412247,
41.945101943823));
#220497=CARTESIAN_POINT('Ctrl Pts',(-2.52105686132487,7.50601280044812,
41.9573365152083));
#220498=CARTESIAN_POINT('Ctrl Pts',(-3.03620611225692,7.3083842404825,41.9781632766603));
#220499=CARTESIAN_POINT('Ctrl Pts',(-3.23555335730512,7.22234129958856,
41.9865189460275));
#220500=CARTESIAN_POINT('Ctrl Pts',(-3.44777701216067,7.12018940735029,
41.9959388376127));
#220501=CARTESIAN_POINT('Ctrl Pts',(-3.46442478062121,7.11210408068141,
41.9966813697875));
#220502=CARTESIAN_POINT('Ctrl Pts',(-3.48830836144234,7.10040077873328,
41.9977519813274));
#220503=CARTESIAN_POINT('Ctrl Pts',(-3.49556730482277,7.0968299725994,41.9980780843184));
#220504=CARTESIAN_POINT('Ctrl Pts',(-3.50813239344269,7.0906250220969,41.9986438132672));
#220505=CARTESIAN_POINT('Ctrl Pts',(-3.51344108842076,7.08799603638857,
41.9988832188529));
#220506=CARTESIAN_POINT('Ctrl Pts',(-3.52366358699059,7.08291931781152,
41.9993449763496));
#220507=CARTESIAN_POINT('Ctrl Pts',(-3.5285778068292,7.08047242759022,41.9995672917061));
#220508=CARTESIAN_POINT('Ctrl Pts',(-3.54104333922466,7.07424938431496,
42.0001320849182));
#220509=CARTESIAN_POINT('Ctrl Pts',(-3.5485911497255,7.07046625995094,42.0004748683441));
#220510=CARTESIAN_POINT('Ctrl Pts',(-3.5743521539647,7.05750265190446,42.0016475912794));
#220511=CARTESIAN_POINT('Ctrl Pts',(-3.59253579578981,7.04826386760933,
42.0024801362335));
#220512=CARTESIAN_POINT('Ctrl Pts',(-3.88395218019158,6.89877970283401,
42.0159020361551));
#220513=CARTESIAN_POINT('Ctrl Pts',(-4.14876607418192,6.74284158376022,
42.0293556189183));
#220514=CARTESIAN_POINT('Ctrl Pts',(-5.03575823288574,6.14847532580657,
42.0775826492922));
#220515=CARTESIAN_POINT('Ctrl Pts',(-5.60347049897522,5.63596163035518,
42.1135700742141));
#220516=CARTESIAN_POINT('Ctrl Pts',(-6.20226648627755,4.91397583051021,
42.1534922700765));
#220517=CARTESIAN_POINT('Ctrl Pts',(-6.31069038605238,4.77393552077865,
42.1608489967513));
#220518=CARTESIAN_POINT('Ctrl Pts',(-6.42647438413755,4.61354295450916,
42.1688539988249));
#220519=CARTESIAN_POINT('Ctrl Pts',(-6.43855390252691,4.59667001819435,
42.1696910832619));
#220520=CARTESIAN_POINT('Ctrl Pts',(-6.45544927921385,4.57287291865571,
42.1708646628838));
#220521=CARTESIAN_POINT('Ctrl Pts',(-6.46032061342598,4.56598835948938,
42.171203360242));
#220522=CARTESIAN_POINT('Ctrl Pts',(-6.46924188268018,4.55333725062501,
42.1718242479178));
#220523=CARTESIAN_POINT('Ctrl Pts',(-6.47329513734873,4.54757305820301,
42.1721065697476));
#220524=CARTESIAN_POINT('Ctrl Pts',(-6.48149829068946,4.53587404490415,
42.1726784143019));
#220525=CARTESIAN_POINT('Ctrl Pts',(-6.48564775297144,4.52993892543764,
42.172967919629));
#220526=CARTESIAN_POINT('Ctrl Pts',(-6.49585093667497,4.51530220179238,
42.1736803963505));
#220527=CARTESIAN_POINT('Ctrl Pts',(-6.50189533768921,4.50659410019524,
42.1741029990117));
#220528=CARTESIAN_POINT('Ctrl Pts',(-6.52391183469455,4.47473868249381,
42.1756442633853));
#220529=CARTESIAN_POINT('Ctrl Pts',(-6.53977806301494,4.45151825915932,
42.1767587465458));
#220530=CARTESIAN_POINT('Ctrl Pts',(-6.76906668787332,4.11207974731767,
42.1929209174369));
#220531=CARTESIAN_POINT('Ctrl Pts',(-6.95947556188112,3.78090014648215,
42.2070243362292));
#220532=CARTESIAN_POINT('Ctrl Pts',(-7.46143197580483,2.74036550525493,
42.2477766617882));
#220533=CARTESIAN_POINT('Ctrl Pts',(-7.693510719254,1.99805136147197,42.2718825976976));
#220534=CARTESIAN_POINT('Ctrl Pts',(-7.81782820231704,1.21079849749936,
42.3010003059383));
#220535=CARTESIAN_POINT('Ctrl Pts',(-7.82138259187117,1.18762163155551,
42.3018609750709));
#220536=CARTESIAN_POINT('Ctrl Pts',(-7.8362578405834,1.08766164772221,42.3055890127478));
#220537=CARTESIAN_POINT('Ctrl Pts',(-7.84655118492198,1.01073176742203,
42.3084988746579));
#220538=CARTESIAN_POINT('Ctrl Pts',(-7.86649340689596,0.842941019962311,
42.3149567807464));
#220539=CARTESIAN_POINT('Ctrl Pts',(-7.87570326841956,0.752040486649506,
42.3185260399074));
#220540=CARTESIAN_POINT('Ctrl Pts',(-7.88416991522032,0.651064694886736,
42.3225881851356));
#220541=CARTESIAN_POINT('Ctrl Pts',(-7.88498452584095,0.641123634296307,
42.3229891469778));
#220542=CARTESIAN_POINT('Ctrl Pts',(-7.88617309362215,0.62627403825458,
42.3235896813882));
#220543=CARTESIAN_POINT('Ctrl Pts',(-7.88656127600493,0.621366617358638,
42.3237884026503));
#220544=CARTESIAN_POINT('Ctrl Pts',(-7.88722110434174,0.612924805331908,
42.3241306968172));
#220545=CARTESIAN_POINT('Ctrl Pts',(-7.88749495612917,0.609390583054566,
42.3242741366023));
#220546=CARTESIAN_POINT('Ctrl Pts',(-7.88803964793819,0.602299128213421,
42.3245622249174));
#220547=CARTESIAN_POINT('Ctrl Pts',(-7.88831045732677,0.59874189433717,
42.3247068752623));
#220548=CARTESIAN_POINT('Ctrl Pts',(-7.88885279295259,0.591553774577943,
42.3249994533008));
#220549=CARTESIAN_POINT('Ctrl Pts',(-7.88912421887864,0.587922882866159,
42.325147387155));
#220550=CARTESIAN_POINT('Ctrl Pts',(-7.88974226027719,0.57957778614266,
42.3254877288672));
#220551=CARTESIAN_POINT('Ctrl Pts',(-7.89008715612654,0.574863472767717,
42.3256802409768));
#220552=CARTESIAN_POINT('Ctrl Pts',(-7.89096650305754,0.562693978209425,
42.3261778201668));
#220553=CARTESIAN_POINT('Ctrl Pts',(-7.89149461315194,0.555238359001871,
42.3264832712027));
#220554=CARTESIAN_POINT('Ctrl Pts',(-7.89236009415005,0.542769190243475,
42.326995129068));
#220555=CARTESIAN_POINT('Ctrl Pts',(-7.89270325669091,0.537756033157323,
42.3272011903006));
#220556=CARTESIAN_POINT('Ctrl Pts',(-7.90496435960736,0.356097193764284,
42.3346778608755));
#220557=CARTESIAN_POINT('Ctrl Pts',(-7.91095283143479,0.179114742897442,
42.3422953872974));
#220558=CARTESIAN_POINT('Ctrl Pts',(-7.91099972245079,0.00209556283347154,
42.3501361000675));
#220559=CARTESIAN_POINT('',(-7.90023482472552,0.00384550184740459,44.3576663208611));
#220560=CARTESIAN_POINT('Ctrl Pts',(-7.92439853970512,0.00241054887052533,
42.3578451112103));
#220561=CARTESIAN_POINT('Ctrl Pts',(-7.90901013703974,-2.42537430455476,
42.4559139907394));
#220562=CARTESIAN_POINT('Ctrl Pts',(-5.39991474507588,-7.5142952426176,
42.6599524474851));
#220563=CARTESIAN_POINT('Ctrl Pts',(1.73928624701431,-8.54502927126578,
42.9169756928389));
#220564=CARTESIAN_POINT('Ctrl Pts',(6.20214295403129,-5.4183663384529,43.128914847272));
#220565=CARTESIAN_POINT('Ctrl Pts',(8.05603662777276,-1.79352951637783,
43.2878692130968));
#220566=CARTESIAN_POINT('Ctrl Pts',(7.91736572010992,2.26730000951632,43.4468235789215));
#220567=CARTESIAN_POINT('Ctrl Pts',(5.19886495601264,7.00699902943489,43.6587627333544));
#220568=CARTESIAN_POINT('Ctrl Pts',(-0.478760874683204,8.7140644824411,
43.8707018877876));
#220569=CARTESIAN_POINT('Ctrl Pts',(-5.3465309654218,6.25325520421469,44.0826410422206));
#220570=CARTESIAN_POINT('Ctrl Pts',(-7.51352671913395,3.24846515819994,
44.2273006934993));
#220571=CARTESIAN_POINT('Ctrl Pts',(-7.90127645816085,0.967839502849978,
44.3189755561699));
#220572=CARTESIAN_POINT('Ctrl Pts',(-7.89681039064019,0.00386106567456798,
44.3576656302323));
#220573=CARTESIAN_POINT('',(-7.9087893072687,-0.00562351359541763,46.3576688933213));
#220574=CARTESIAN_POINT('Ctrl Pts',(-7.91099908898921,0.0037965789759559,
44.3576684917633));
#220575=CARTESIAN_POINT('Ctrl Pts',(-7.91109982716945,-0.206113357618994,
44.3660783104271));
#220576=CARTESIAN_POINT('Ctrl Pts',(-7.90284075888705,-0.415997733834797,
44.3744881290909));
#220577=CARTESIAN_POINT('Ctrl Pts',(-7.88625968517452,-0.625163321053882,
44.3828979477547));
#220578=CARTESIAN_POINT('Ctrl Pts',(-7.87039289892966,-0.825318372513329,
44.3909454842056));
#220579=CARTESIAN_POINT('Ctrl Pts',(-7.84690610496436,-1.02481493022194,
44.3989930206565));
#220580=CARTESIAN_POINT('Ctrl Pts',(-7.81588547481346,-1.22305161158475,
44.4070405571074));
#220581=CARTESIAN_POINT('Ctrl Pts',(-7.78485066183586,-1.42137892800182,
44.4150917729425));
#220582=CARTESIAN_POINT('Ctrl Pts',(-7.74627519257816,-1.61844489821876,
44.4231429887776));
#220583=CARTESIAN_POINT('Ctrl Pts',(-7.70029643748892,-1.81365811960124,
44.4311942046126));
#220584=CARTESIAN_POINT('Ctrl Pts',(-7.65429036665681,-2.00898731615855,
44.4392502036337));
#220585=CARTESIAN_POINT('Ctrl Pts',(-7.60087231183685,-2.20246125254749,
44.4473062026549));
#220586=CARTESIAN_POINT('Ctrl Pts',(-7.54022973211643,-2.39350299496519,
44.455362201676));
#220587=CARTESIAN_POINT('Ctrl Pts',(-7.47954281728029,-2.58468440587652,
44.4634240903485));
#220588=CARTESIAN_POINT('Ctrl Pts',(-7.41162094061861,-2.77342976716646,
44.4714859790209));
#220589=CARTESIAN_POINT('Ctrl Pts',(-7.33670013772784,-2.95918098281675,
44.4795478676933));
#220590=CARTESIAN_POINT('Ctrl Pts',(-7.26167017368218,-3.14520284181893,
44.4876215027038));
#220591=CARTESIAN_POINT('Ctrl Pts',(-7.17962102796923,-3.32822153676562,
44.4956951377143));
#220592=CARTESIAN_POINT('Ctrl Pts',(-7.09083592370065,-3.50770108520613,
44.5037687727248));
#220593=CARTESIAN_POINT('Ctrl Pts',(-7.00197608919707,-3.68733170120405,
44.5118492032969));
#220594=CARTESIAN_POINT('Ctrl Pts',(-6.90636913929137,-3.86341694329685,
44.5199296338689));
#220595=CARTESIAN_POINT('Ctrl Pts',(-6.80434263566374,-4.03544821506715,
44.528010064441));
#220596=CARTESIAN_POINT('Ctrl Pts',(-6.70216180642607,-4.2077397018798,
44.5361027174977));
#220597=CARTESIAN_POINT('Ctrl Pts',(-6.59354219716093,-4.37596469417913,
44.5441953705544));
#220598=CARTESIAN_POINT('Ctrl Pts',(-6.47885362489306,-4.5396449979277,
44.5522880236112));
#220599=CARTESIAN_POINT('Ctrl Pts',(-6.44476484316526,-4.58829554817254,
44.554693395639));
#220600=CARTESIAN_POINT('Ctrl Pts',(-6.41014015950638,-4.63654483022345,
44.5570987676669));
#220601=CARTESIAN_POINT('Ctrl Pts',(-6.3749899338597,-4.68438089219777,
44.5595041396948));
#220602=CARTESIAN_POINT('Ctrl Pts',(-6.2615872279606,-4.83871102145419,
44.5672644226414));
#220603=CARTESIAN_POINT('Ctrl Pts',(-6.14237699780792,-4.98919264526007,
44.575024705588));
#220604=CARTESIAN_POINT('Ctrl Pts',(-6.01765181233345,-5.13534688852856,
44.5827849885346));
#220605=CARTESIAN_POINT('Ctrl Pts',(-5.89307673985873,-5.28132522785431,
44.5905359315925));
#220606=CARTESIAN_POINT('Ctrl Pts',(-5.76300015346301,-5.4229862837319,
44.5982868746503));
#220607=CARTESIAN_POINT('Ctrl Pts',(-5.62775838536374,-5.55987918537517,
44.6060378177082));
#220608=CARTESIAN_POINT('Ctrl Pts',(-5.4926519374696,-5.69663511472216,
44.6137810053277));
#220609=CARTESIAN_POINT('Ctrl Pts',(-5.35239084601381,-5.82863213414115,
44.6215241929472));
#220610=CARTESIAN_POINT('Ctrl Pts',(-5.20735233406623,-5.95545150839926,
44.6292673805666));
#220611=CARTESIAN_POINT('Ctrl Pts',(-5.06242954934239,-6.08216969260859,
44.6370043898436));
#220612=CARTESIAN_POINT('Ctrl Pts',(-4.91273720216241,-6.20371822188837,
44.6447413991205));
#220613=CARTESIAN_POINT('Ctrl Pts',(-4.75869013840848,-6.31971432634529,
44.6524784083974));
#220614=CARTESIAN_POINT('Ctrl Pts',(-4.6047348010644,-6.43564136161024,
44.6602108107181));
#220615=CARTESIAN_POINT('Ctrl Pts',(-4.44643019630563,-6.54602234023068,
44.6679432130388));
#220616=CARTESIAN_POINT('Ctrl Pts',(-4.28422516124588,-6.65051394763952,
44.6756756153595));
#220617=CARTESIAN_POINT('Ctrl Pts',(-4.12208389292393,-6.75496447686031,
44.683404977885));
#220618=CARTESIAN_POINT('Ctrl Pts',(-3.95604554959901,-6.85353005197379,
44.6911343404106));
#220619=CARTESIAN_POINT('Ctrl Pts',(-3.78658900026213,-6.94590992909452,
44.6988637029362));
#220620=CARTESIAN_POINT('Ctrl Pts',(-3.61713251704006,-7.03828977017251,
44.7065930624461));
#220621=CARTESIAN_POINT('Ctrl Pts',(-3.44425814018197,-7.12448373618032,
44.714322421956));
#220622=CARTESIAN_POINT('Ctrl Pts',(-3.26847081325667,-7.20423622203556,
44.7220517814659));
#220623=CARTESIAN_POINT('Ctrl Pts',(-3.0926746752393,-7.28399270537179,
44.7297815283991));
#220624=CARTESIAN_POINT('Ctrl Pts',(-2.91396562323699,-7.3573069162215,
44.7375112753322));
#220625=CARTESIAN_POINT('Ctrl Pts',(-2.73286996688449,-7.42397082053134,
44.7452410222654));
#220626=CARTESIAN_POINT('Ctrl Pts',(-2.55173205000262,-7.4906502815472,
44.7529725730143));
#220627=CARTESIAN_POINT('Ctrl Pts',(-2.36820675677898,-7.55067622135483,
44.7607041237632));
#220628=CARTESIAN_POINT('Ctrl Pts',(-2.18283703457222,-7.60389002290932,
44.7684356745121));
#220629=CARTESIAN_POINT('Ctrl Pts',(-1.99739007695806,-7.65712599631364,
44.776170446658));
#220630=CARTESIAN_POINT('Ctrl Pts',(-1.81009750496497,-7.70354408058446,
44.783905218804));
#220631=CARTESIAN_POINT('Ctrl Pts',(-1.62151401522891,-7.74303643917657,
44.7916399909499));
#220632=CARTESIAN_POINT('Ctrl Pts',(-1.43270563958536,-7.78257589242641,
44.7993839868156));
#220633=CARTESIAN_POINT('Ctrl Pts',(-1.24260362336187,-7.81517305230361,
44.8071279826812));
#220634=CARTESIAN_POINT('Ctrl Pts',(-1.05177041277071,-7.84077164562393,
44.8148719785469));
#220635=CARTESIAN_POINT('Ctrl Pts',(-0.860813341852577,-7.86638685371549,
44.8226210006543));
#220636=CARTESIAN_POINT('Ctrl Pts',(-0.669124487209044,-7.88499441252165,
44.8303700227618));
#220637=CARTESIAN_POINT('Ctrl Pts',(-0.477267761920374,-7.89659018079522,
44.8381190448693));
#220638=CARTESIAN_POINT('Ctrl Pts',(-0.285117834361302,-7.90820367013424,
44.8458799093079));
#220639=CARTESIAN_POINT('Ctrl Pts',(-0.0927998811833496,-7.91278395903853,
44.8536407737465));
#220640=CARTESIAN_POINT('Ctrl Pts',(0.0991246257200402,-7.9103789611229,
44.8614016381851));
#220641=CARTESIAN_POINT('Ctrl Pts',(0.231109408828784,-7.90872506536257,
44.8667387159048));
#220642=CARTESIAN_POINT('Ctrl Pts',(0.362908228918708,-7.90376878181581,
44.8720757936246));
#220643=CARTESIAN_POINT('Ctrl Pts',(0.494341184836341,-7.89553974044679,
44.8774128713443));
#220644=CARTESIAN_POINT('Ctrl Pts',(0.691692154768313,-7.88318356018403,
44.8854266716674));
#220645=CARTESIAN_POINT('Ctrl Pts',(0.888823270522177,-7.86340857175364,
44.8934404719905));
#220646=CARTESIAN_POINT('Ctrl Pts',(1.08514215758107,-7.8362227825554,44.9014542723135));
#220647=CARTESIAN_POINT('Ctrl Pts',(1.28123726428257,-7.80906798194778,
44.9094589378502));
#220648=CARTESIAN_POINT('Ctrl Pts',(1.476521658544,-7.77451925845426,44.9174636033868));
#220649=CARTESIAN_POINT('Ctrl Pts',(1.67040499389583,-7.73263655918005,
44.9254682689235));
#220650=CARTESIAN_POINT('Ctrl Pts',(1.8641002400297,-7.69079449095924,44.9334651690105));
#220651=CARTESIAN_POINT('Ctrl Pts',(2.05639681089065,-7.64163269568441,
44.9414620690975));
#220652=CARTESIAN_POINT('Ctrl Pts',(2.24671108690782,-7.58526270421569,
44.9494589691845));
#220653=CARTESIAN_POINT('Ctrl Pts',(2.43687302432396,-7.52893783456242,
44.9574494680882));
#220654=CARTESIAN_POINT('Ctrl Pts',(2.62505550996796,-7.46541636294701,
44.9654399669918));
#220655=CARTESIAN_POINT('Ctrl Pts',(2.81068629733434,-7.39486061653477,
44.9734304658955));
#220656=CARTESIAN_POINT('Ctrl Pts',(2.99619997191894,-7.32434938310365,
44.9814159236658));
#220657=CARTESIAN_POINT('Ctrl Pts',(3.17916484529946,-7.24681283943503,
44.9894013814361));
#220658=CARTESIAN_POINT('Ctrl Pts',(3.35902459788108,-7.16246289699499,
44.9973868392064));
#220659=CARTESIAN_POINT('Ctrl Pts',(3.54478152141502,-7.07534732175913,
45.0056341210309));
#220660=CARTESIAN_POINT('Ctrl Pts',(3.72722590038802,-6.98096408133548,
45.0138814028554));
#220661=CARTESIAN_POINT('Ctrl Pts',(3.90576689097264,-6.87960071467683,
45.0221286846798));
#220662=CARTESIAN_POINT('Ctrl Pts',(4.07852271811378,-6.78152176825905,
45.0301087344633));
#220663=CARTESIAN_POINT('Ctrl Pts',(4.24762384174879,-6.67690813471623,
45.0380887842467));
#220664=CARTESIAN_POINT('Ctrl Pts',(4.41255965923379,-6.56606718315482,
45.0460688340302));
#220665=CARTESIAN_POINT('Ctrl Pts',(4.57748237876047,-6.45523503374557,
45.0540482500983));
#220666=CARTESIAN_POINT('Ctrl Pts',(4.7382401736902,-6.33817673848495,45.0620276661664));
#220667=CARTESIAN_POINT('Ctrl Pts',(4.89435118121349,-6.21524315815191,
45.0700070822345));
#220668=CARTESIAN_POINT('Ctrl Pts',(5.05047378340941,-6.09230044729924,
45.0779870909496));
#220669=CARTESIAN_POINT('Ctrl Pts',(5.20194864763116,-5.96348178887062,
45.0859670996647));
#220670=CARTESIAN_POINT('Ctrl Pts',(5.34832648350908,-5.82917874368211,
45.0939471083798));
#220671=CARTESIAN_POINT('Ctrl Pts',(5.49473768746913,-5.69484508296349,
45.1019289362063));
#220672=CARTESIAN_POINT('Ctrl Pts',(5.63604930102413,-5.5550247700403,45.1099107640327));
#220673=CARTESIAN_POINT('Ctrl Pts',(5.77184816184117,-5.41014692930337,
45.1178925918592));
#220674=CARTESIAN_POINT('Ctrl Pts',(5.90774799521772,-5.26516136537711,
45.1258803545336));
#220675=CARTESIAN_POINT('Ctrl Pts',(6.03812665892673,-5.11511100604018,
45.1338681172079));
#220676=CARTESIAN_POINT('Ctrl Pts',(6.16260996772766,-4.96045959419726,
45.1418558798823));
#220677=CARTESIAN_POINT('Ctrl Pts',(6.28714810340438,-4.80574006837321,
45.1498471606514));
#220678=CARTESIAN_POINT('Ctrl Pts',(6.40578550402128,-4.64641571502952,
45.1578384414205));
#220679=CARTESIAN_POINT('Ctrl Pts',(6.51819042492076,-4.48298054696553,
45.1658297221896));
#220680=CARTESIAN_POINT('Ctrl Pts',(6.63070110390533,-4.31939160813888,
45.1738285216914));
#220681=CARTESIAN_POINT('Ctrl Pts',(6.73696740993568,-4.15168441024629,
45.1818273211931));
#220682=CARTESIAN_POINT('Ctrl Pts',(6.83670227117521,-3.9803797626995,45.1898261206949));
#220683=CARTESIAN_POINT('Ctrl Pts',(6.85954283053687,-3.94114880651634,
45.1916579481279));
#220684=CARTESIAN_POINT('Ctrl Pts',(6.88204103031947,-3.90172926989703,
45.1934897755608));
#220685=CARTESIAN_POINT('Ctrl Pts',(6.90419377139895,-3.86212757000282,
45.1953216029938));
#220686=CARTESIAN_POINT('Ctrl Pts',(7.00247139146564,-3.68644001954424,
45.2034482560269));
#220687=CARTESIAN_POINT('Ctrl Pts',(7.09411950613567,-3.50685571861464,
45.21157490906));
#220688=CARTESIAN_POINT('Ctrl Pts',(7.17882944288115,-3.32390265050328,
45.2197015620931));
#220689=CARTESIAN_POINT('Ctrl Pts',(7.26346727072994,-3.14110532024741,
45.2278212973548));
#220690=CARTESIAN_POINT('Ctrl Pts',(7.34117856188255,-2.95494522784442,
45.2359410326164));
#220691=CARTESIAN_POINT('Ctrl Pts',(7.41170034204722,-2.7659752420615,45.244060767878));
#220692=CARTESIAN_POINT('Ctrl Pts',(7.48217097162953,-2.57714231925115,
45.252174613765));
#220693=CARTESIAN_POINT('Ctrl Pts',(7.54546237646609,-2.38550386443243,
45.2602884596519));
#220694=CARTESIAN_POINT('Ctrl Pts',(7.60135930856294,-2.1916335601837,45.2684023055389));
#220695=CARTESIAN_POINT('Ctrl Pts',(7.65721652380877,-1.99790100800299,
45.2765103862363));
#220696=CARTESIAN_POINT('Ctrl Pts',(7.70568966018132,-1.80194007576001,
45.2846184669337));
#220697=CARTESIAN_POINT('Ctrl Pts',(7.7466129059657,-1.60434082573676,45.2927265476311));
#220698=CARTESIAN_POINT('Ctrl Pts',(7.78751857500983,-1.40682644558694,
45.3008311458669));
#220699=CARTESIAN_POINT('Ctrl Pts',(7.8208807545832,-1.20767546234247,45.3089357441028));
#220700=CARTESIAN_POINT('Ctrl Pts',(7.84658425365761,-1.00749022340289,
45.3170403423387));
#220701=CARTESIAN_POINT('Ctrl Pts',(7.87227971856832,-0.807367556526994,
45.3251424073137));
#220702=CARTESIAN_POINT('Ctrl Pts',(7.89032123671649,-0.606211594589851,
45.3332444722887));
#220703=CARTESIAN_POINT('Ctrl Pts',(7.90064513463664,-0.404632495658001,
45.3413465372637));
#220704=CARTESIAN_POINT('Ctrl Pts',(7.90613682644405,-0.297404557653095,
45.345656347782));
#220705=CARTESIAN_POINT('Ctrl Pts',(7.90944561592449,-0.190057001995731,
45.3499661583004));
#220706=CARTESIAN_POINT('Ctrl Pts',(7.91056791006032,-0.0826821644845067,
45.3542759688187));
#220707=CARTESIAN_POINT('Ctrl Pts',(7.9127263280764,0.123823221542817,45.3625646806382));
#220708=CARTESIAN_POINT('Ctrl Pts',(7.90679341923676,0.330340691145279,
45.3708533924576));
#220709=CARTESIAN_POINT('Ctrl Pts',(7.89280547003969,0.536230185751951,
45.3791421042771));
#220710=CARTESIAN_POINT('Ctrl Pts',(7.8788094569267,0.742238373638703,45.3874355944578));
#220711=CARTESIAN_POINT('Ctrl Pts',(7.85674915431576,0.947617572038266,
45.3957290846386));
#220712=CARTESIAN_POINT('Ctrl Pts',(7.8267127113667,1.15173310004138,45.4040225748193));
#220713=CARTESIAN_POINT('Ctrl Pts',(7.79665714179197,1.35597860486316,45.4123213461342));
#220714=CARTESIAN_POINT('Ctrl Pts',(7.75861533609209,1.55895854380817,45.420620117449));
#220715=CARTESIAN_POINT('Ctrl Pts',(7.71272666472887,1.76004783888968,45.4289188887638));
#220716=CARTESIAN_POINT('Ctrl Pts',(7.66678457630412,1.9613712135148,45.4372273203274));
#220717=CARTESIAN_POINT('Ctrl Pts',(7.6129774292099,2.16079925958702,45.4455357518909));
#220718=CARTESIAN_POINT('Ctrl Pts',(7.55149510465868,2.35771980615085,45.4538441834544));
#220719=CARTESIAN_POINT('Ctrl Pts',(7.48997485363959,2.55476182666408,45.4621577402221));
#220720=CARTESIAN_POINT('Ctrl Pts',(7.42077006778067,2.7492929830202,45.4704712969897));
#220721=CARTESIAN_POINT('Ctrl Pts',(7.34411952157781,2.94071920672133,45.4787848537574));
#220722=CARTESIAN_POINT('Ctrl Pts',(7.2673851739534,3.13235471516291,45.4871074996693));
#220723=CARTESIAN_POINT('Ctrl Pts',(7.18318891056288,3.32087823705202,45.4954301455813));
#220724=CARTESIAN_POINT('Ctrl Pts',(7.09181705855585,3.50571701766931,45.5037527914932));
#220725=CARTESIAN_POINT('Ctrl Pts',(7.05713335022302,3.57587970141391,45.5069119725433));
#220726=CARTESIAN_POINT('Ctrl Pts',(7.02141619908188,3.64551171933842,45.5100711535933));
#220727=CARTESIAN_POINT('Ctrl Pts',(6.98468296144834,3.71458273942758,45.5132303346434));
#220728=CARTESIAN_POINT('Ctrl Pts',(6.88354481067239,3.90475697110615,45.5219285532038));
#220729=CARTESIAN_POINT('Ctrl Pts',(6.77461103495292,4.09084538653731,45.5306267717642));
#220730=CARTESIAN_POINT('Ctrl Pts',(6.65822115543557,4.27223735825975,45.5393249903246));
#220731=CARTESIAN_POINT('Ctrl Pts',(6.54193354002888,4.45346995282031,45.548015566334));
#220732=CARTESIAN_POINT('Ctrl Pts',(6.41820302540795,4.63001415083212,45.5567061423434));
#220733=CARTESIAN_POINT('Ctrl Pts',(6.28741352878674,4.80128650655525,45.5653967183529));
#220734=CARTESIAN_POINT('Ctrl Pts',(6.15348736160973,4.97666641654763,45.5742957168625));
#220735=CARTESIAN_POINT('Ctrl Pts',(6.0121595041008,5.14651824650132,45.5831947153721));
#220736=CARTESIAN_POINT('Ctrl Pts',(5.86388959808269,5.31024667802708,45.5920937138817));
#220737=CARTESIAN_POINT('Ctrl Pts',(5.7195189483578,5.46966931929405,45.6007586832692));
#220738=CARTESIAN_POINT('Ctrl Pts',(5.56856689393716,5.62328633793491,45.6094236526567));
#220739=CARTESIAN_POINT('Ctrl Pts',(5.41149969380398,5.77057987241832,45.6180886220442));
#220740=CARTESIAN_POINT('Ctrl Pts',(5.248069234209,5.92384070609705,45.6271046351148));
#220741=CARTESIAN_POINT('Ctrl Pts',(5.07801796646155,6.07025483645696,45.6361206481855));
#220742=CARTESIAN_POINT('Ctrl Pts',(4.90191645063256,6.20927822786336,45.6451366612562));
#220743=CARTESIAN_POINT('Ctrl Pts',(4.72581493480356,6.34830161926976,45.6541526743268));
#220744=CARTESIAN_POINT('Ctrl Pts',(4.54366334874069,6.47993404570182,45.6631686873975));
#220745=CARTESIAN_POINT('Ctrl Pts',(4.35607592972436,6.60367499915585,45.6721847004682));
#220746=CARTESIAN_POINT('Ctrl Pts',(4.1935716725746,6.71086999029916,45.6799951416704));
#220747=CARTESIAN_POINT('Ctrl Pts',(4.02705788775809,6.81209615834343,45.6878055828726));
#220748=CARTESIAN_POINT('Ctrl Pts',(3.85702114597265,6.90704776873013,45.6956160240748));
#220749=CARTESIAN_POINT('Ctrl Pts',(3.68699666349458,7.00199253329653,45.7034259021599));
#220750=CARTESIAN_POINT('Ctrl Pts',(3.51345003746774,7.09066346960936,45.711235780245));
#220751=CARTESIAN_POINT('Ctrl Pts',(3.33689361421739,7.17280015108432,45.7190456583301));
#220752=CARTESIAN_POINT('Ctrl Pts',(3.1603187571691,7.25494540823702,45.7268563518243));
#220753=CARTESIAN_POINT('Ctrl Pts',(2.98073379664296,7.33055490386447,45.7346670453185));
#220754=CARTESIAN_POINT('Ctrl Pts',(2.79867241578842,7.39941576809311,45.7424777388127));
#220755=CARTESIAN_POINT('Ctrl Pts',(2.61648183404873,7.46832549982221,45.7502939752096));
#220756=CARTESIAN_POINT('Ctrl Pts',(2.43181165073282,7.53047690725006,45.7581102116064));
#220757=CARTESIAN_POINT('Ctrl Pts',(2.24521295929854,7.5857062800637,45.7659264480033));
#220758=CARTESIAN_POINT('Ctrl Pts',(2.05854527962687,7.64095607197596,45.7737455741759));
#220759=CARTESIAN_POINT('Ctrl Pts',(1.86994801126352,7.68927863918557,45.7815647003485));
#220760=CARTESIAN_POINT('Ctrl Pts',(1.67998402619482,7.73056108388843,45.7893838265211));
#220761=CARTESIAN_POINT('Ctrl Pts',(1.48980880674577,7.77188943345912,45.7972116473327));
#220762=CARTESIAN_POINT('Ctrl Pts',(1.29826418053113,7.80616195614139,45.8050394681443));
#220763=CARTESIAN_POINT('Ctrl Pts',(1.10592085526108,7.83331730889912,45.8128672889559));
#220764=CARTESIAN_POINT('Ctrl Pts',(0.956264286457905,7.85444607389607,
45.8189578814016));
#220765=CARTESIAN_POINT('Ctrl Pts',(0.806124361235694,7.87126719524561,
45.8250484738473));
#220766=CARTESIAN_POINT('Ctrl Pts',(0.655770330981767,7.88377360614852,
45.8311390662929));
#220767=CARTESIAN_POINT('Ctrl Pts',(0.455392368194894,7.90044099533835,
45.8392560452949));
#220768=CARTESIAN_POINT('Ctrl Pts',(0.254235815865489,7.90947658372479,
45.8473730242969));
#220769=CARTESIAN_POINT('Ctrl Pts',(0.0529080594121575,7.91082307584042,
45.8554900032989));
#220770=CARTESIAN_POINT('Ctrl Pts',(-0.148272432775386,7.9121685830438,
45.8636010450124));
#220771=CARTESIAN_POINT('Ctrl Pts',(-0.349623559861184,7.90583620596543,
45.871712086726));
#220772=CARTESIAN_POINT('Ctrl Pts',(-0.55053476441224,7.89182060573944,
45.8798231284396));
#220773=CARTESIAN_POINT('Ctrl Pts',(-0.751327575407982,7.87781326466825,
45.8879293904543));
#220774=CARTESIAN_POINT('Ctrl Pts',(-0.951680661696556,7.85613175097405,
45.8960356524689));
#220775=CARTESIAN_POINT('Ctrl Pts',(-1.15098483876664,7.82682278456139,
45.9041419144836));
#220776=CARTESIAN_POINT('Ctrl Pts',(-1.35019987652316,7.79752692666049,
45.9122445509514));
#220777=CARTESIAN_POINT('Ctrl Pts',(-1.54836662387694,7.76061046584511,
45.9203471874192));
#220778=CARTESIAN_POINT('Ctrl Pts',(-1.74488180554461,7.71617188019288,
45.928449823887));
#220779=CARTESIAN_POINT('Ctrl Pts',(-1.94133698337312,7.67174686339434,
45.9365499863002));
#220780=CARTESIAN_POINT('Ctrl Pts',(-2.13614128887116,7.61980437345477,
45.9446501487134));
#220781=CARTESIAN_POINT('Ctrl Pts',(-2.32870184792713,7.5604939457327,45.9527503111266));
#220782=CARTESIAN_POINT('Ctrl Pts',(-2.52313804086199,7.50060580548137,
45.9609293730772));
#220783=CARTESIAN_POINT('Ctrl Pts',(-2.71528622065873,7.43320550083424,
45.9691084350279));
#220784=CARTESIAN_POINT('Ctrl Pts',(-2.90455106595427,7.35849876708992,
45.9772874969785));
#220785=CARTESIAN_POINT('Ctrl Pts',(-3.0919891346209,7.28451309971699,45.9853876149542));
#220786=CARTESIAN_POINT('Ctrl Pts',(-3.27659898816238,7.20336156377171,
45.9934877329298));
#220787=CARTESIAN_POINT('Ctrl Pts',(-3.45782158877621,7.11529274592361,
46.0015878509055));
#220788=CARTESIAN_POINT('Ctrl Pts',(-3.6390685787649,7.02721207556151,46.0096890590145));
#220789=CARTESIAN_POINT('Ctrl Pts',(-3.81692711812746,6.9322124068927,46.0177902671236));
#220790=CARTESIAN_POINT('Ctrl Pts',(-3.99086146664235,6.83058897563521,
46.0258914752327));
#220791=CARTESIAN_POINT('Ctrl Pts',(-4.16484168715849,6.72893874305754,
46.0339948198871));
#220792=CARTESIAN_POINT('Ctrl Pts',(-4.33489537597066,6.62066142591515,
46.0420981645416));
#220793=CARTESIAN_POINT('Ctrl Pts',(-4.50051408243206,6.50609667879526,
46.050201509196));
#220794=CARTESIAN_POINT('Ctrl Pts',(-4.66886837705556,6.38963962148463,
46.0584386999249));
#220795=CARTESIAN_POINT('Ctrl Pts',(-4.83263961466782,6.26668580812152,
46.0666758906538));
#220796=CARTESIAN_POINT('Ctrl Pts',(-4.99132723906832,6.13763581458973,
46.0749130813826));
#220797=CARTESIAN_POINT('Ctrl Pts',(-5.14763963626277,6.01051743391519,
46.0830269783159));
#220798=CARTESIAN_POINT('Ctrl Pts',(-5.29901931862242,5.87748432973878,
46.0911408752493));
#220799=CARTESIAN_POINT('Ctrl Pts',(-5.44502358725628,5.73895801816173,
46.0992547721826));
#220800=CARTESIAN_POINT('Ctrl Pts',(-5.59435574271114,5.59727426542921,
46.1075536098092));
#220801=CARTESIAN_POINT('Ctrl Pts',(-5.7380642686248,5.449844163697,46.1158524474359));
#220802=CARTESIAN_POINT('Ctrl Pts',(-5.87571744045468,5.29715636544144,
46.1241512850625));
#220803=CARTESIAN_POINT('Ctrl Pts',(-6.01337061228458,5.14446856718585,
46.1324501226891));
#220804=CARTESIAN_POINT('Ctrl Pts',(-6.14496822909381,4.9865233685294,46.1407489603158));
#220805=CARTESIAN_POINT('Ctrl Pts',(-6.27012419589844,4.82384323625976,
46.1490477979425));
#220806=CARTESIAN_POINT('Ctrl Pts',(-6.38962698099469,4.66851121827937,
46.156971784587));
#220807=CARTESIAN_POINT('Ctrl Pts',(-6.50351342195307,4.50852890841244,
46.1648957712315));
#220808=CARTESIAN_POINT('Ctrl Pts',(-6.61140283708434,4.34433809984825,
46.1728197578761));
#220809=CARTESIAN_POINT('Ctrl Pts',(-6.71917673398114,4.180323091962,46.1807352602319));
#220810=CARTESIAN_POINT('Ctrl Pts',(-6.82096620798325,4.01210884387182,
46.1886507625878));
#220811=CARTESIAN_POINT('Ctrl Pts',(-6.91643073493292,3.84017016405202,
46.1965662649436));
#220812=CARTESIAN_POINT('Ctrl Pts',(-7.01180879751107,3.66838721296585,
46.2044745980508));
#220813=CARTESIAN_POINT('Ctrl Pts',(-7.10087315974315,3.49288684740855,
46.2123829311579));
#220814=CARTESIAN_POINT('Ctrl Pts',(-7.1833263914318,3.31417304227757,46.220291264265));
#220815=CARTESIAN_POINT('Ctrl Pts',(-7.26570691397072,3.13561683107651,
46.2281926236228));
#220816=CARTESIAN_POINT('Ctrl Pts',(-7.3414877853863,2.9538531389966,46.2360939829805));
#220817=CARTESIAN_POINT('Ctrl Pts',(-7.41041732906845,2.76941076928686,
46.2439953423382));
#220818=CARTESIAN_POINT('Ctrl Pts',(-7.47931138270548,2.58506336419856,
46.2518926334897));
#220819=CARTESIAN_POINT('Ctrl Pts',(-7.54136101623707,2.39804034864094,
46.2597899246412));
#220820=CARTESIAN_POINT('Ctrl Pts',(-7.59636229280378,2.20889133197376,
46.2676872157926));
#220821=CARTESIAN_POINT('Ctrl Pts',(-7.65134487076883,2.01980661967077,
46.2755818221282));
#220822=CARTESIAN_POINT('Ctrl Pts',(-7.69928377003174,1.82859767441595,
46.2834764284638));
#220823=CARTESIAN_POINT('Ctrl Pts',(-7.74002453821444,1.63583041536658,
46.2913710347994));
#220824=CARTESIAN_POINT('Ctrl Pts',(-7.76863330987008,1.50046638707689,
46.2969147444554));
#220825=CARTESIAN_POINT('Ctrl Pts',(-7.79369367148229,1.3643343046367,46.3024584541113));
#220826=CARTESIAN_POINT('Ctrl Pts',(-7.81516706782015,1.22763378173597,
46.3080021637673));
#220827=CARTESIAN_POINT('Ctrl Pts',(-7.845367225673,1.03537833666277,46.3157988301198));
#220828=CARTESIAN_POINT('Ctrl Pts',(-7.8684564505306,0.842086412083351,
46.3235954964722));
#220829=CARTESIAN_POINT('Ctrl Pts',(-7.88438896608291,0.648329878619016,
46.3313921628247));
#220830=CARTESIAN_POINT('Ctrl Pts',(-7.90033187838918,0.454446909438875,
46.3391939168874));
#220831=CARTESIAN_POINT('Ctrl Pts',(-7.90910873931268,0.260099077667802,
46.34699567095));
#220832=CARTESIAN_POINT('Ctrl Pts',(-7.91072585228101,0.0658596238445143,
46.3547974250127));
#220833=CARTESIAN_POINT('Ctrl Pts',(-7.91092421960704,0.0420327411094098,
46.3557544472629));
#220834=CARTESIAN_POINT('Ctrl Pts',(-7.91101491610168,0.0182074856072361,
46.3567114695131));
#220835=CARTESIAN_POINT('Ctrl Pts',(-7.91099800725439,-0.00561508833863839,
46.3576684917633));
#220836=CARTESIAN_POINT('',(-7.919264176172,0.00076404157701636,48.3576684917633));
#220837=CARTESIAN_POINT('Ctrl Pts',(-7.9087893072687,-0.00562351359541763,
46.3576688933213));
#220838=CARTESIAN_POINT('Ctrl Pts',(-7.91252992283379,-0.912183692134236,
46.3940981054115));
#220839=CARTESIAN_POINT('Ctrl Pts',(-7.33081702863261,-4.44677843272281,
46.5364968947182));
#220840=CARTESIAN_POINT('Ctrl Pts',(-2.13546797111051,-9.11796621008134,
46.7848652612416));
#220841=CARTESIAN_POINT('Ctrl Pts',(6.52665753302942,-6.70593118787837,
47.1027739928909));
#220842=CARTESIAN_POINT('Ctrl Pts',(8.71102287534456,0.400901934475626,
47.3676979359323));
#220843=CARTESIAN_POINT('Ctrl Pts',(6.30989378669818,5.29249576291848,47.5796370903652));
#220844=CARTESIAN_POINT('Ctrl Pts',(3.0142647445543,7.68314273743952,47.7385914561901));
#220845=CARTESIAN_POINT('Ctrl Pts',(-1.01938237615656,8.17228174075617,
47.8975458220149));
#220846=CARTESIAN_POINT('Ctrl Pts',(-5.98723647190021,6.26859805905107,
48.1039048338725));
#220847=CARTESIAN_POINT('Ctrl Pts',(-7.90588447844806,2.48564124360112,
48.2572790571221));
#220848=CARTESIAN_POINT('Ctrl Pts',(-7.919264176172,0.00076404157701636,
48.3576684917633));
#220849=CARTESIAN_POINT('',(-7.91099885442289,0.00182802643405098,52.3592849490288));
#220850=CARTESIAN_POINT('Ctrl Pts',(-7.91099999257641,0.000342718611354188,
48.3529178502397));
#220851=CARTESIAN_POINT('Ctrl Pts',(-7.91100661574924,-0.152540487811379,
48.3586348317909));
#220852=CARTESIAN_POINT('Ctrl Pts',(-7.90658148115475,-0.305390842585058,
48.3645117988981));
#220853=CARTESIAN_POINT('Ctrl Pts',(-7.89699780615803,-0.470644912774039,
48.3711132231136));
#220854=CARTESIAN_POINT('Ctrl Pts',(-7.89623522578758,-0.483270359723247,
48.3716190656282));
#220855=CARTESIAN_POINT('Ctrl Pts',(-7.89496833725055,-0.503441299715581,
48.3724295463481));
#220856=CARTESIAN_POINT('Ctrl Pts',(-7.89448348037355,-0.51098802917705,
48.3727332989232));
#220857=CARTESIAN_POINT('Ctrl Pts',(-7.89363240401814,-0.523944529531292,
48.3732556724732));
#220858=CARTESIAN_POINT('Ctrl Pts',(-7.89327144179119,-0.529354650288003,
48.3734740584775));
#220859=CARTESIAN_POINT('Ctrl Pts',(-7.89258197691212,-0.539530871591092,
48.3738853241614));
#220860=CARTESIAN_POINT('Ctrl Pts',(-7.89225471827215,-0.544297056250423,
48.374078148934));
#220861=CARTESIAN_POINT('Ctrl Pts',(-7.8915630985206,-0.554238011260211,
48.3744807466072));
#220862=CARTESIAN_POINT('Ctrl Pts',(-7.89119796448472,-0.5594127243683,
48.3746905530849));
#220863=CARTESIAN_POINT('Ctrl Pts',(-7.89034505126172,-0.571333279638533,
48.3751744054809));
#220864=CARTESIAN_POINT('Ctrl Pts',(-7.88985371088079,-0.578078856981754,
48.375448604309));
#220865=CARTESIAN_POINT('Ctrl Pts',(-7.88826100268444,-0.599564710918577,
48.3763232246957));
#220866=CARTESIAN_POINT('Ctrl Pts',(-7.88712697675256,-0.614302480473204,
48.3769250246693));
#220867=CARTESIAN_POINT('Ctrl Pts',(-7.87670620086609,-0.744943040559715,
48.3822756802667));
#220868=CARTESIAN_POINT('Ctrl Pts',(-7.86490678359015,-0.860627858398803,
48.3871259461307));
#220869=CARTESIAN_POINT('Ctrl Pts',(-7.84570162601393,-1.01510558565293,
48.3937177240286));
#220870=CARTESIAN_POINT('Ctrl Pts',(-7.84054873943716,-1.05416733342591,
48.3953944606311));
#220871=CARTESIAN_POINT('Ctrl Pts',(-7.83045833566371,-1.12648730171445,
48.3985154460787));
#220872=CARTESIAN_POINT('Ctrl Pts',(-7.82560015480292,-1.15975582612675,
48.3999576987699));
#220873=CARTESIAN_POINT('Ctrl Pts',(-7.71367378093027,-1.89347697473503,
48.4318978521123));
#220874=CARTESIAN_POINT('Ctrl Pts',(-7.51319161944449,-2.57645980247717,
48.463848760742));
#220875=CARTESIAN_POINT('Ctrl Pts',(-7.14652961386596,-3.3981688616766,
48.5017989064571));
#220876=CARTESIAN_POINT('Ctrl Pts',(-7.06236223474376,-3.56980125007885,
48.5097265543574));
#220877=CARTESIAN_POINT('Ctrl Pts',(-6.95046144749486,-3.77850443661812,
48.5193885177295));
#220878=CARTESIAN_POINT('Ctrl Pts',(-6.92851456981222,-3.81859869865115,
48.5212458626885));
#220879=CARTESIAN_POINT('Ctrl Pts',(-6.8889585147471,-3.88939896178052,
48.5245285959484));
#220880=CARTESIAN_POINT('Ctrl Pts',(-6.87148847872423,-3.92018109442377,
48.5259568473936));
#220881=CARTESIAN_POINT('Ctrl Pts',(-6.84547039708444,-3.96531651357632,
48.528052946124));
#220882=CARTESIAN_POINT('Ctrl Pts',(-6.83708259566889,-3.97976149947496,
48.5287240594627));
#220883=CARTESIAN_POINT('Ctrl Pts',(-6.82217211084606,-4.00525320805384,
48.5299089619354));
#220884=CARTESIAN_POINT('Ctrl Pts',(-6.81566819705766,-4.01631081956556,
48.5304231273273));
#220885=CARTESIAN_POINT('Ctrl Pts',(-6.80289571202452,-4.0379055530394,
48.5314276503735));
#220886=CARTESIAN_POINT('Ctrl Pts',(-6.79662948550272,-4.04844401735975,
48.5319180529909));
#220887=CARTESIAN_POINT('Ctrl Pts',(-6.78144746443217,-4.07384236225726,
48.5331004310319));
#220888=CARTESIAN_POINT('Ctrl Pts',(-6.77250728407431,-4.08868761281229,
48.5337919230438));
#220889=CARTESIAN_POINT('Ctrl Pts',(-6.74485538591721,-4.1342643074334,
48.5359162262893));
#220890=CARTESIAN_POINT('Ctrl Pts',(-6.72598264041988,-4.1648977279389,
48.5373459514208));
#220891=CARTESIAN_POINT('Ctrl Pts',(-6.51753243772125,-4.49813282197162,
48.5529221407399));
#220892=CARTESIAN_POINT('Ctrl Pts',(-6.30787906436848,-4.78770396647052,
48.566641454316));
#220893=CARTESIAN_POINT('Ctrl Pts',(-5.76291319535767,-5.44218113988198,
48.5986218239133));
#220894=CARTESIAN_POINT('Ctrl Pts',(-5.41152229067082,-5.79171153527603,
48.616493264834));
#220895=CARTESIAN_POINT('Ctrl Pts',(-4.87011634372129,-6.23768315747306,
48.6425651874563));
#220896=CARTESIAN_POINT('Ctrl Pts',(-4.70533327230349,-6.36290484720138,
48.65034589399));
#220897=CARTESIAN_POINT('Ctrl Pts',(-4.4720880165956,-6.52613239690935,
48.6613578592977));
#220898=CARTESIAN_POINT('Ctrl Pts',(-4.40768484202316,-6.56980130598483,
48.664398523612));
#220899=CARTESIAN_POINT('Ctrl Pts',(-4.31831240962476,-6.62849505238604,
48.6686299082087));
#220900=CARTESIAN_POINT('Ctrl Pts',(-4.29388776915809,-6.64434319754351,
48.6697875039874));
#220901=CARTESIAN_POINT('Ctrl Pts',(-4.25741760587972,-6.66772210806573,
48.6715184502886));
#220902=CARTESIAN_POINT('Ctrl Pts',(-4.24543824605021,-6.67535593635639,
48.672087406372));
#220903=CARTESIAN_POINT('Ctrl Pts',(-4.22363483013553,-6.6891676985892,
48.6731237611976));
#220904=CARTESIAN_POINT('Ctrl Pts',(-4.21381760120947,-6.69535636841934,
48.6735906877806));
#220905=CARTESIAN_POINT('Ctrl Pts',(-4.19832699576839,-6.7050739053632,
48.6743279637802));
#220906=CARTESIAN_POINT('Ctrl Pts',(-4.19266268389706,-6.70861723893145,
48.6745976646051));
#220907=CARTESIAN_POINT('Ctrl Pts',(-4.18247363878874,-6.71497309334601,
48.6750830097549));
#220908=CARTESIAN_POINT('Ctrl Pts',(-4.17795053635783,-6.71778822969965,
48.6752985352102));
#220909=CARTESIAN_POINT('Ctrl Pts',(-4.16759861972971,-6.72421666634182,
48.6757919740803));
#220910=CARTESIAN_POINT('Ctrl Pts',(-4.16176794872268,-6.72782695761993,
48.676070025062));
#220911=CARTESIAN_POINT('Ctrl Pts',(-4.14581290907523,-6.7376774756889,
48.67683123804));
#220912=CARTESIAN_POINT('Ctrl Pts',(-4.13567917643111,-6.74390244524758,
48.6773151069841));
#220913=CARTESIAN_POINT('Ctrl Pts',(-4.08656069818263,-6.77392269573197,
48.6796624711196));
#220914=CARTESIAN_POINT('Ctrl Pts',(-4.04738496354369,-6.7974025817451,
48.6815408735513));
#220915=CARTESIAN_POINT('Ctrl Pts',(-3.6679549366365,-7.02037004560078,
48.6998107317642));
#220916=CARTESIAN_POINT('Ctrl Pts',(-3.31348985693382,-7.19445401575491,
48.7176023183945));
#220917=CARTESIAN_POINT('Ctrl Pts',(-2.9141862889199,-7.35477635369745,
48.7373327793731));
#220918=CARTESIAN_POINT('Ctrl Pts',(-2.88068818691423,-7.36796121709828,
48.738985779723));
#220919=CARTESIAN_POINT('Ctrl Pts',(-2.80985012154015,-7.39528616231137,
48.7424753433348));
#220920=CARTESIAN_POINT('Ctrl Pts',(-2.77249070714876,-7.40937314467989,
48.7443122092073));
#220921=CARTESIAN_POINT('Ctrl Pts',(-2.69292466414668,-7.4386887908924,
48.7482150643918));
#220922=CARTESIAN_POINT('Ctrl Pts',(-2.65069181886143,-7.45384243552452,
48.7502812025828));
#220923=CARTESIAN_POINT('Ctrl Pts',(-2.56010914456161,-7.48547735812721,
48.7546986866358));
#220924=CARTESIAN_POINT('Ctrl Pts',(-2.51172387818537,-7.50185132387944,
48.7570498189509));
#220925=CARTESIAN_POINT('Ctrl Pts',(-2.40702621195399,-7.53615538552259,
48.7621156655851));
#220926=CARTESIAN_POINT('Ctrl Pts',(-2.35066444220565,-7.55392546382175,
48.7648293831232));
#220927=CARTESIAN_POINT('Ctrl Pts',(-2.22715058391424,-7.59135141477335,
48.7707424381434));
#220928=CARTESIAN_POINT('Ctrl Pts',(-2.15992583994453,-7.61075137773288,
48.7739390257932));
#220929=CARTESIAN_POINT('Ctrl Pts',(-2.00949524559602,-7.65200949873924,
48.7810366857959));
#220930=CARTESIAN_POINT('Ctrl Pts',(-1.92617181449688,-7.67340752345283,
48.7849306016099));
#220931=CARTESIAN_POINT('Ctrl Pts',(-1.54067935108595,-7.7657297325216,
48.8027503669159));
#220932=CARTESIAN_POINT('Ctrl Pts',(-1.23483391434615,-7.82019585537871,
48.8163241561035));
#220933=CARTESIAN_POINT('Ctrl Pts',(-0.802353418988295,-7.87120008959691,
48.8345719702348));
#220934=CARTESIAN_POINT('Ctrl Pts',(-0.677817434831919,-7.8829009458555,
48.839720123879));
#220935=CARTESIAN_POINT('Ctrl Pts',(-0.535937842065803,-7.89284397233831,
48.845465888752));
#220936=CARTESIAN_POINT('Ctrl Pts',(-0.518819484888331,-7.89398769249893,
48.8461571756467));
#220937=CARTESIAN_POINT('Ctrl Pts',(-0.493046164904217,-7.89562547405645,
48.847195035469));
#220938=CARTESIAN_POINT('Ctrl Pts',(-0.484393944219274,-7.89616100739766,
48.8475429514724));
#220939=CARTESIAN_POINT('Ctrl Pts',(-0.469491370421446,-7.89705882279947,
48.8481413462082));
#220940=CARTESIAN_POINT('Ctrl Pts',(-0.463241444858093,-7.89742790797418,
48.848392045345));
#220941=CARTESIAN_POINT('Ctrl Pts',(-0.450350636799203,-7.89817381089004,
48.8489085929236));
#220942=CARTESIAN_POINT('Ctrl Pts',(-0.443709703530657,-7.8985496733487,
48.8491744101444));
#220943=CARTESIAN_POINT('Ctrl Pts',(-0.427691631236518,-7.89943599629352,
48.8498148655461));
#220944=CARTESIAN_POINT('Ctrl Pts',(-0.418314030716937,-7.89993813668887,
48.8501892333271));
#220945=CARTESIAN_POINT('Ctrl Pts',(-0.389442718001976,-7.9014325509617,
48.8513400421727));
#220946=CARTESIAN_POINT('Ctrl Pts',(-0.369946140895122,-7.90236938190622,
48.8521146810402));
#220947=CARTESIAN_POINT('Ctrl Pts',(-0.143619541678384,-7.91240518455315,
48.8610784356172));
#220948=CARTESIAN_POINT('Ctrl Pts',(0.0634951013188367,-7.91345428530354,
48.8690003584402));
#220949=CARTESIAN_POINT('Ctrl Pts',(0.958808634332102,-7.88283171187693,
48.9022430620205));
#220950=CARTESIAN_POINT('Ctrl Pts',(1.64112210893485,-7.76949561552535,
48.9247075830862));
#220951=CARTESIAN_POINT('Ctrl Pts',(2.55939489953236,-7.49044948587877,
48.9572919195504));
#220952=CARTESIAN_POINT('Ctrl Pts',(2.8144105518948,-7.39840622688852,48.9666562515675));
#220953=CARTESIAN_POINT('Ctrl Pts',(3.18828566343891,-7.24133096905835,
48.9814903459293));
#220954=CARTESIAN_POINT('Ctrl Pts',(3.31102771276401,-7.18603729132512,
48.9865472699021));
#220955=CARTESIAN_POINT('Ctrl Pts',(3.48456177873523,-7.10247250317492,
48.9940452198641));
#220956=CARTESIAN_POINT('Ctrl Pts',(3.53655007621673,-7.07672944793297,
48.996337293225));
#220957=CARTESIAN_POINT('Ctrl Pts',(3.59618510664614,-7.04637871312041,
48.9990246692971));
#220958=CARTESIAN_POINT('Ctrl Pts',(3.60411408443478,-7.04232645899623,
48.9993831733879));
#220959=CARTESIAN_POINT('Ctrl Pts',(3.61536070831833,-7.03655469048941,
48.9998934031931));
#220960=CARTESIAN_POINT('Ctrl Pts',(3.61868402995509,-7.03484618557877,
49.0000443871616));
#220961=CARTESIAN_POINT('Ctrl Pts',(3.62537367615581,-7.03140107348601,
49.0003487414055));
#220962=CARTESIAN_POINT('Ctrl Pts',(3.62873996635609,-7.02966440197925,
49.0005021160366));
#220963=CARTESIAN_POINT('Ctrl Pts',(3.63521377196227,-7.02631867181486,
49.0007975023784));
#220964=CARTESIAN_POINT('Ctrl Pts',(3.63832147032344,-7.02470996726983,
49.0009394898793));
#220965=CARTESIAN_POINT('Ctrl Pts',(3.64566064517282,-7.02090465615061,
49.0012752596173));
#220966=CARTESIAN_POINT('Ctrl Pts',(3.64989117851192,-7.01870629925154,
49.0014691627196));
#220967=CARTESIAN_POINT('Ctrl Pts',(3.66257068361196,-7.0121029496636,49.0020513784108));
#220968=CARTESIAN_POINT('Ctrl Pts',(3.67101365357332,-7.00768653285817,
49.0024404738746));
#220969=CARTESIAN_POINT('Ctrl Pts',(3.75204687743676,-6.96511238904207,
49.0061883098611));
#220970=CARTESIAN_POINT('Ctrl Pts',(3.82404517609923,-6.92584463465615,
49.0096217384498));
#220971=CARTESIAN_POINT('Ctrl Pts',(4.10019653383469,-6.76961341188309,
49.023150644087));
#220972=CARTESIAN_POINT('Ctrl Pts',(4.29969268660219,-6.64469000790777,
49.0336938035138));
#220973=CARTESIAN_POINT('Ctrl Pts',(4.81087167482887,-6.29192386670885,
49.0621469682306));
#220974=CARTESIAN_POINT('Ctrl Pts',(5.11197234620048,-6.04983747216701,
49.0803915568301));
#220975=CARTESIAN_POINT('Ctrl Pts',(5.79360790095394,-5.41444004763659,
49.1235575187725));
#220976=CARTESIAN_POINT('Ctrl Pts',(6.15343820265702,-5.00174152867317,
49.1479000756468));
#220977=CARTESIAN_POINT('Ctrl Pts',(6.49767599167211,-4.51295882524471,
49.1723497541839));
#220978=CARTESIAN_POINT('Ctrl Pts',(6.52701293761932,-4.47042424230836,
49.1744457630141));
#220979=CARTESIAN_POINT('Ctrl Pts',(6.56317149771846,-4.41688444873617,
49.1770452393478));
#220980=CARTESIAN_POINT('Ctrl Pts',(6.57038523763264,-4.40614640851522,
49.1775646616262));
#220981=CARTESIAN_POINT('Ctrl Pts',(6.58176998967304,-4.38910946259454,
49.1783857293413));
#220982=CARTESIAN_POINT('Ctrl Pts',(6.58595835720279,-4.38282221738789,
49.1786880780354));
#220983=CARTESIAN_POINT('Ctrl Pts',(6.59379725704169,-4.3710184729439,49.1792544867366));
#220984=CARTESIAN_POINT('Ctrl Pts',(6.59744988676893,-4.36550337872447,
49.179518631434));
#220985=CARTESIAN_POINT('Ctrl Pts',(6.60560174291223,-4.35316131842645,
49.1801086382622));
#220986=CARTESIAN_POINT('Ctrl Pts',(6.61009731478669,-4.34633194082252,
49.180434352858));
#220987=CARTESIAN_POINT('Ctrl Pts',(6.62142130366424,-4.32907107378963,
49.1812556644296));
#220988=CARTESIAN_POINT('Ctrl Pts',(6.6282356752216,-4.31863037064045,49.1817506963699));
#220989=CARTESIAN_POINT('Ctrl Pts',(6.66460157881149,-4.26262318136732,
49.1843968292002));
#220990=CARTESIAN_POINT('Ctrl Pts',(6.69370832717306,-4.21676885540567,
49.1865301064493));
#220991=CARTESIAN_POINT('Ctrl Pts',(7.18236075874533,-3.42914255465011,
49.2226236523381));
#220992=CARTESIAN_POINT('Ctrl Pts',(7.51647601648318,-2.6168184078806,49.2506467358803));
#220993=CARTESIAN_POINT('Ctrl Pts',(7.76012010158495,-1.55315726001384,
49.288681172093));
#220994=CARTESIAN_POINT('Ctrl Pts',(7.80009135965436,-1.33803083913816,
49.2964923040738));
#220995=CARTESIAN_POINT('Ctrl Pts',(7.84739975800822,-1.00770155530242,
49.3090344547507));
#220996=CARTESIAN_POINT('Ctrl Pts',(7.86121808071381,-0.893528611771507,
49.3134685427911));
#220997=CARTESIAN_POINT('Ctrl Pts',(7.8744931619752,-0.759388439814313,
49.3188372586612));
#220998=CARTESIAN_POINT('Ctrl Pts',(7.87636987804081,-0.739669456558147,
49.3196305034297));
#220999=CARTESIAN_POINT('Ctrl Pts',(7.87875954302258,-0.713519916311099,
49.3206879967775));
#221000=CARTESIAN_POINT('Ctrl Pts',(7.87933870628537,-0.707095579741262,
49.3209482394462));
#221001=CARTESIAN_POINT('Ctrl Pts',(7.88023410046405,-0.697025760990089,
49.321356840038));
#221002=CARTESIAN_POINT('Ctrl Pts',(7.88055566156894,-0.693380742756694,
49.3215048833921));
#221003=CARTESIAN_POINT('Ctrl Pts',(7.88121598036788,-0.685835981546097,
49.3218116044132));
#221004=CARTESIAN_POINT('Ctrl Pts',(7.881554372733,-0.681936208406209,49.3219703034383));
#221005=CARTESIAN_POINT('Ctrl Pts',(7.88231206479833,-0.673128352011628,
49.3223290919668));
#221006=CARTESIAN_POINT('Ctrl Pts',(7.88272967468943,-0.668220128954483,
49.3225292796412));
#221007=CARTESIAN_POINT('Ctrl Pts',(7.8837866334746,-0.65565867543255,49.323042249917));
#221008=CARTESIAN_POINT('Ctrl Pts',(7.88441942124602,-0.648004915003598,
49.3233554100142));
#221009=CARTESIAN_POINT('Ctrl Pts',(7.88795309570027,-0.604492529093342,
49.3251391459016));
#221010=CARTESIAN_POINT('Ctrl Pts',(7.89062045419689,-0.568615886238823,
49.3266229476336));
#221011=CARTESIAN_POINT('Ctrl Pts',(7.90138341779411,-0.409147349534968,
49.3332726872491));
#221012=CARTESIAN_POINT('Ctrl Pts',(7.90682024283162,-0.285398510364241,
49.3385778210243));
#221013=CARTESIAN_POINT('Ctrl Pts',(7.91122346572789,-0.0698592169688464,
49.3480116480563));
#221014=CARTESIAN_POINT('Ctrl Pts',(7.91150157955322,0.0218839090433246,
49.3520881194122));
#221015=CARTESIAN_POINT('Ctrl Pts',(7.90001394010572,0.821729758698371,
49.3880471709652));
#221016=CARTESIAN_POINT('Ctrl Pts',(7.79481102396731,1.52529913615493,49.4222083583846));
#221017=CARTESIAN_POINT('Ctrl Pts',(7.49231567967891,2.56730278294983,49.4707495100454));
#221018=CARTESIAN_POINT('Ctrl Pts',(7.36157543239759,2.92114643119724,49.4869112064786));
#221019=CARTESIAN_POINT('Ctrl Pts',(7.19421130595928,3.29060401180695,49.5033888048121));
#221020=CARTESIAN_POINT('Ctrl Pts',(7.1821794788057,3.31678293447481,49.5045543432817));
#221021=CARTESIAN_POINT('Ctrl Pts',(7.16536237469439,3.35285307468195,49.5061575634714));
#221022=CARTESIAN_POINT('Ctrl Pts',(7.16069917739773,3.36280076620141,49.5065994271673));
#221023=CARTESIAN_POINT('Ctrl Pts',(7.15279799122516,3.37956488973098,49.5073435964196));
#221024=CARTESIAN_POINT('Ctrl Pts',(7.14957095061672,3.38638644718539,49.5076462773202));
#221025=CARTESIAN_POINT('Ctrl Pts',(7.14317094308289,3.39986533045488,49.5082440940921));
#221026=CARTESIAN_POINT('Ctrl Pts',(7.1399984185725,3.40652285629643,49.5085392447022));
#221027=CARTESIAN_POINT('Ctrl Pts',(7.13299188686917,3.42117323835114,49.5091884746106));
#221028=CARTESIAN_POINT('Ctrl Pts',(7.12915374228704,3.42916411162583,49.5095424112388));
#221029=CARTESIAN_POINT('Ctrl Pts',(7.11573851096625,3.4569742501357,49.5107735848593));
#221030=CARTESIAN_POINT('Ctrl Pts',(7.10609210361164,3.47676006469464,49.511648435281));
#221031=CARTESIAN_POINT('Ctrl Pts',(7.00945630452051,3.67288809452217,49.5203101663974));
#221032=CARTESIAN_POINT('Ctrl Pts',(6.91600070138897,3.84597520775397,49.5278692045383));
#221033=CARTESIAN_POINT('Ctrl Pts',(6.48971679090423,4.56959566521287,49.5593190800551));
#221034=CARTESIAN_POINT('Ctrl Pts',(6.09689795915771,5.08187614184098,49.5809863835182));
#221035=CARTESIAN_POINT('Ctrl Pts',(5.5038362838196,5.68622301205579,49.6106286371034));
#221036=CARTESIAN_POINT('Ctrl Pts',(5.35573175650464,5.82593153716105,49.6178479706202));
#221037=CARTESIAN_POINT('Ctrl Pts',(5.144136819712,6.01063730125885,49.6281469277709));
#221038=CARTESIAN_POINT('Ctrl Pts',(5.08512139320036,6.06064718944004,49.6310179914204));
#221039=CARTESIAN_POINT('Ctrl Pts',(4.92297921660238,6.19401143922407,49.6389281361451));
#221040=CARTESIAN_POINT('Ctrl Pts',(4.81848699848259,6.27564194572297,49.644060491067));
#221041=CARTESIAN_POINT('Ctrl Pts',(4.69663331035553,6.36599733077107,49.6500871031609));
#221042=CARTESIAN_POINT('Ctrl Pts',(4.68123603394261,6.37732825360064,49.650849158632));
#221043=CARTESIAN_POINT('Ctrl Pts',(4.65692972641367,6.39507991474747,49.6520528362937));
#221044=CARTESIAN_POINT('Ctrl Pts',(4.64804808264866,6.40153814428547,49.6524928099804));
#221045=CARTESIAN_POINT('Ctrl Pts',(4.63303220259765,6.41240911909503,49.6532368684981));
#221046=CARTESIAN_POINT('Ctrl Pts',(4.62690502448526,6.41683161653042,49.6535405380033));
#221047=CARTESIAN_POINT('Ctrl Pts',(4.61486127033237,6.42549838341937,49.6541375430188));
#221048=CARTESIAN_POINT('Ctrl Pts',(4.60894515104571,6.42974327745645,49.6544308521191));
#221049=CARTESIAN_POINT('Ctrl Pts',(4.59763868522363,6.4378321935656,49.6549914865852));
#221050=CARTESIAN_POINT('Ctrl Pts',(4.5922493550361,6.44167763034238,49.6552587540299));
#221051=CARTESIAN_POINT('Ctrl Pts',(4.57980057475314,6.45053661853814,49.6558761868436));
#221052=CARTESIAN_POINT('Ctrl Pts',(4.57273771412904,6.45554535022041,49.6562265439412));
#221053=CARTESIAN_POINT('Ctrl Pts',(4.55165348068188,6.47044558223827,49.6572725739305));
#221054=CARTESIAN_POINT('Ctrl Pts',(4.53760817494482,6.48030303973213,49.6579695664457));
#221055=CARTESIAN_POINT('Ctrl Pts',(4.43694161994981,6.55046640374775,49.6629658732885));
#221056=CARTESIAN_POINT('Ctrl Pts',(4.34915486146927,6.60907800669358,49.6673268371874));
#221057=CARTESIAN_POINT('Ctrl Pts',(3.88349400070891,6.9066845115384,49.690400873529));
#221058=CARTESIAN_POINT('Ctrl Pts',(3.48703597589635,7.11508183160246,49.7097881305069));
#221059=CARTESIAN_POINT('Ctrl Pts',(2.54662273391097,7.51183341385169,49.7536213046553));
#221060=CARTESIAN_POINT('Ctrl Pts',(1.99543921507439,7.67666592210404,49.7777368059601));
#221061=CARTESIAN_POINT('Ctrl Pts',(1.15421249347565,7.83141581900206,49.8130058032926));
#221062=CARTESIAN_POINT('Ctrl Pts',(0.874621814571236,7.86754873002635,
49.8245534133192));
#221063=CARTESIAN_POINT('Ctrl Pts',(0.550173865377027,7.89196647060808,
49.8377225142882));
#221064=CARTESIAN_POINT('Ctrl Pts',(0.506623502239162,7.89488180459686,
49.839485464602));
#221065=CARTESIAN_POINT('Ctrl Pts',(0.439345026522528,7.89882654939033,
49.842201726678));
#221066=CARTESIAN_POINT('Ctrl Pts',(0.415632774466015,7.90010976574574,
49.8431576891077));
#221067=CARTESIAN_POINT('Ctrl Pts',(0.373961018304702,7.90217674425358,
49.8448352900434));
#221068=CARTESIAN_POINT('Ctrl Pts',(0.356003968542585,7.90300609369197,
49.845557413228));
#221069=CARTESIAN_POINT('Ctrl Pts',(0.315107312811892,7.90475524261024,
49.8472002650276));
#221070=CARTESIAN_POINT('Ctrl Pts',(0.292166199282699,7.9056364057672,49.8481205656482));
#221071=CARTESIAN_POINT('Ctrl Pts',(0.23033713514553,7.90774174803181,49.8505975449528));
#221072=CARTESIAN_POINT('Ctrl Pts',(0.191443376698478,7.9087789324712,49.8521521330745));
#221073=CARTESIAN_POINT('Ctrl Pts',(0.00458423463766006,7.9123827036578,
49.8596044685682));
#221074=CARTESIAN_POINT('Ctrl Pts',(-0.14342747607543,7.91108403921816,
49.8654573361658));
#221075=CARTESIAN_POINT('Ctrl Pts',(-0.304709530693521,7.90514090296338,
49.871794149227));
#221076=CARTESIAN_POINT('Ctrl Pts',(-0.318100437902277,7.90461338117633,
49.8723199797568));
#221077=CARTESIAN_POINT('Ctrl Pts',(-1.02673932222282,7.87489360253939,
49.9001313274641));
#221078=CARTESIAN_POINT('Ctrl Pts',(-1.71506856455189,7.75413479406379,
49.9260768847217));
#221079=CARTESIAN_POINT('Ctrl Pts',(-2.42154685907048,7.53140441058269,
49.9553849848351));
#221080=CARTESIAN_POINT('Ctrl Pts',(-2.46430143181564,7.51752352732088,
49.9571706617528));
#221081=CARTESIAN_POINT('Ctrl Pts',(-2.53692159645602,7.49326026388894,
49.9602266022773));
#221082=CARTESIAN_POINT('Ctrl Pts',(-2.56684766294533,7.48306178161918,
49.9614925989072));
#221083=CARTESIAN_POINT('Ctrl Pts',(-2.60945912356887,7.46825456194679,
49.9633054870285));
#221084=CARTESIAN_POINT('Ctrl Pts',(-2.62219519606525,7.463792298262,49.9638486442149));
#221085=CARTESIAN_POINT('Ctrl Pts',(-2.64457279545448,7.45588764250573,
49.9648052420404));
#221086=CARTESIAN_POINT('Ctrl Pts',(-2.65421918854743,7.45245907781669,
49.9652183454056));
#221087=CARTESIAN_POINT('Ctrl Pts',(-2.67298221972546,7.44574918547511,
49.966023285584));
#221088=CARTESIAN_POINT('Ctrl Pts',(-2.6820995410196,7.44246981394094,49.9664150755907));
#221089=CARTESIAN_POINT('Ctrl Pts',(-2.70645963948871,7.43365725455341,
49.9674636055986));
#221090=CARTESIAN_POINT('Ctrl Pts',(-2.7216914419776,7.42809394463044,49.9681210370287));
#221091=CARTESIAN_POINT('Ctrl Pts',(-2.77694172355167,7.40772140767843,
49.9705121724703));
#221092=CARTESIAN_POINT('Ctrl Pts',(-2.81685711203906,7.39263537272083,
49.9722519241893));
#221093=CARTESIAN_POINT('Ctrl Pts',(-3.2356632050271,7.23046310318623,49.9906282851724));
#221094=CARTESIAN_POINT('Ctrl Pts',(-3.60279850662276,7.05471090422539,
50.0077673043186));
#221095=CARTESIAN_POINT('Ctrl Pts',(-4.23543921280448,6.68954246540859,
50.0384355816507));
#221096=CARTESIAN_POINT('Ctrl Pts',(-4.50587094352013,6.51045764238882,
50.0519689907399));
#221097=CARTESIAN_POINT('Ctrl Pts',(-4.9022445261573,6.21141422585282,50.0724063327205));
#221098=CARTESIAN_POINT('Ctrl Pts',(-5.03649660314221,6.10306248354741,
50.0794474542288));
#221099=CARTESIAN_POINT('Ctrl Pts',(-5.20087533890208,5.96127554062813,
50.0882367416149));
#221100=CARTESIAN_POINT('Ctrl Pts',(-5.23440243413324,5.93185818673869,
50.0900386748054));
#221101=CARTESIAN_POINT('Ctrl Pts',(-5.28776368598536,5.88423324802794,
50.0929220874912));
#221102=CARTESIAN_POINT('Ctrl Pts',(-5.30775670867709,5.86620528480842,
50.0940059690077));
#221103=CARTESIAN_POINT('Ctrl Pts',(-5.345615820904,5.83171524187965,50.096065358478));
#221104=CARTESIAN_POINT('Ctrl Pts',(-5.36349885759869,5.81527223575232,
50.097041108542));
#221105=CARTESIAN_POINT('Ctrl Pts',(-5.40419455632999,5.77750614585633,
50.0992685795209));
#221106=CARTESIAN_POINT('Ctrl Pts',(-5.42695729807266,5.75612982496213,
50.100519572694));
#221107=CARTESIAN_POINT('Ctrl Pts',(-5.49731689498937,5.68926729310164,
50.104402742031));
#221108=CARTESIAN_POINT('Ctrl Pts',(-5.54447306914706,5.64332117096459,
50.1070288060158));
#221109=CARTESIAN_POINT('Ctrl Pts',(-5.69019741966563,5.49774630353738,
50.1152234795968));
#221110=CARTESIAN_POINT('Ctrl Pts',(-5.78669559525153,5.39608336162977,
50.1207664804448));
#221111=CARTESIAN_POINT('Ctrl Pts',(-6.04285138454884,5.11143956168988,
50.1358577302533));
#221112=CARTESIAN_POINT('Ctrl Pts',(-6.19686849361963,4.92358531291668,
50.1453447110581));
#221113=CARTESIAN_POINT('Ctrl Pts',(-6.88006779501779,4.00734379429515,
50.1894024851266));
#221114=CARTESIAN_POINT('Ctrl Pts',(-7.29095677095426,3.19932370315164,
50.2209451943107));
#221115=CARTESIAN_POINT('Ctrl Pts',(-7.57364965574357,2.28623773066557,
50.2585424156923));
#221116=CARTESIAN_POINT('Ctrl Pts',(-7.58963090453476,2.23261161578721,
50.2607614420685));
#221117=CARTESIAN_POINT('Ctrl Pts',(-7.60849007438963,2.16678484274719,
50.2635030380398));
#221118=CARTESIAN_POINT('Ctrl Pts',(-7.61190988036006,2.15474029478054,
50.2640054001461));
#221119=CARTESIAN_POINT('Ctrl Pts',(-7.61721833305808,2.13587358588345,
50.2647935008947));
#221120=CARTESIAN_POINT('Ctrl Pts',(-7.61912644935336,2.12905689372577,
50.2650784919022));
#221121=CARTESIAN_POINT('Ctrl Pts',(-7.62248920621045,2.11698112299754,
50.2655837985381));
#221122=CARTESIAN_POINT('Ctrl Pts',(-7.62394756113775,2.11172307813934,
50.2658039689641));
#221123=CARTESIAN_POINT('Ctrl Pts',(-7.62728579590833,2.09963866435772,
50.2663103311243));
#221124=CARTESIAN_POINT('Ctrl Pts',(-7.62916195188494,2.09281127788031,
50.2665966698636));
#221125=CARTESIAN_POINT('Ctrl Pts',(-7.63424475844412,2.07421713126053,
50.2673772232649));
#221126=CARTESIAN_POINT('Ctrl Pts',(-7.63743336093345,2.06244548886669,
50.2678721627985));
#221127=CARTESIAN_POINT('Ctrl Pts',(-7.65252025215243,2.00623312193516,
50.2702395409895));
#221128=CARTESIAN_POINT('Ctrl Pts',(-7.66405778238667,1.96169715531895,
50.2721268620331));
#221129=CARTESIAN_POINT('Ctrl Pts',(-7.83174917306884,1.29032357800861,
50.3007852269654));
#221130=CARTESIAN_POINT('Ctrl Pts',(-7.91091770692492,0.646847282851201,
50.3311032181041));
#221131=CARTESIAN_POINT('Ctrl Pts',(-7.9110781458086,-0.613265661808885,
50.3889607529025));
#221132=CARTESIAN_POINT('Ctrl Pts',(-7.83961221315099,-1.22553469161474,
50.4163053721436));
#221133=CARTESIAN_POINT('Ctrl Pts',(-7.68892047427846,-1.86171179354981,
50.4429917766574));
#221134=CARTESIAN_POINT('Ctrl Pts',(-7.67956668600615,-1.89992748100339,
50.4445889437121));
#221135=CARTESIAN_POINT('Ctrl Pts',(-7.66669637470578,-1.95086178829899,
50.4467099645235));
#221136=CARTESIAN_POINT('Ctrl Pts',(-7.66343263670222,-1.9636433596231,
50.4472415690704));
#221137=CARTESIAN_POINT('Ctrl Pts',(-7.658286695103,-1.98358784621849,50.4480700861503));
#221138=CARTESIAN_POINT('Ctrl Pts',(-7.65642638431928,-1.9907563562427,
50.4483676716273));
#221139=CARTESIAN_POINT('Ctrl Pts',(-7.65285141875138,-2.00445297235825,
50.4489358723899));
#221140=CARTESIAN_POINT('Ctrl Pts',(-7.65113847101483,-2.01098151496095,
50.4492065399394));
#221141=CARTESIAN_POINT('Ctrl Pts',(-7.64711834734946,-2.0262238857487,
50.4498380862094));
#221142=CARTESIAN_POINT('Ctrl Pts',(-7.64480462699974,-2.03493598651649,
50.4501987628552));
#221143=CARTESIAN_POINT('Ctrl Pts',(-7.6381508891065,-2.05981851448924,
50.4512280452428));
#221144=CARTESIAN_POINT('Ctrl Pts',(-7.63377440979884,-2.07597918629055,
50.4518955251838));
#221145=CARTESIAN_POINT('Ctrl Pts',(-7.60556724247679,-2.17884214348994,
50.4561376725646));
#221146=CARTESIAN_POINT('Ctrl Pts',(-7.58031069865209,-2.26514823178452,
50.4596680187682));
#221147=CARTESIAN_POINT('Ctrl Pts',(-7.50124455436533,-2.5191811308906,
50.4699831922148));
#221148=CARTESIAN_POINT('Ctrl Pts',(-7.4432980986143,-2.6855653091354,50.4766391382225));
#221149=CARTESIAN_POINT('Ctrl Pts',(-7.25853460608201,-3.16401509616062,
50.4955984443591));
#221150=CARTESIAN_POINT('Ctrl Pts',(-7.11728867606135,-3.47009130871819,
50.5074852468541));
#221151=CARTESIAN_POINT('Ctrl Pts',(-6.63093218700432,-4.36848345296698,
50.542976746542));
#221152=CARTESIAN_POINT('Ctrl Pts',(-6.22812000437783,-4.92577038368863,
50.5657375972308));
#221153=CARTESIAN_POINT('Ctrl Pts',(-5.73111295294465,-5.45342842424301,
50.59428384968));
#221154=CARTESIAN_POINT('Ctrl Pts',(-5.70332658931703,-5.48248145479456,
50.5958818908981));
#221155=CARTESIAN_POINT('Ctrl Pts',(-5.66809643280397,-5.51875994646949,
50.5979098638502));
#221156=CARTESIAN_POINT('Ctrl Pts',(-5.66085804235525,-5.52618446499029,
50.5983266162829));
#221157=CARTESIAN_POINT('Ctrl Pts',(-5.64941556507517,-5.53787510215853,
50.5989855221022));
#221158=CARTESIAN_POINT('Ctrl Pts',(-5.64522117710273,-5.54215073192017,
50.5992270740518));
#221159=CARTESIAN_POINT('Ctrl Pts',(-5.63779748682326,-5.54970104145597,
50.5996546304427));
#221160=CARTESIAN_POINT('Ctrl Pts',(-5.63457017334984,-5.55297767989755,
50.5998405131253));
#221161=CARTESIAN_POINT('Ctrl Pts',(-5.62716437177296,-5.56048356524843,
50.6002670827712));
#221162=CARTESIAN_POINT('Ctrl Pts',(-5.62298397313339,-5.56471091647651,
50.6005078855522));
#221163=CARTESIAN_POINT('Ctrl Pts',(-5.61144035032726,-5.57635790305297,
50.6011728600856));
#221164=CARTESIAN_POINT('Ctrl Pts',(-5.60406719590833,-5.58376764653519,
50.6015976259967));
#221165=CARTESIAN_POINT('Ctrl Pts',(-5.56444556777176,-5.62342836842772,
50.6038802858695));
#221166=CARTESIAN_POINT('Ctrl Pts',(-5.53193374440984,-5.65541422218535,
50.6057535686657));
#221167=CARTESIAN_POINT('Ctrl Pts',(-5.00264858932352,-6.16720558405938,
50.6362271789454));
#221168=CARTESIAN_POINT('Ctrl Pts',(-4.44541680323696,-6.58021745856812,
50.6676222125593));
#221169=CARTESIAN_POINT('Ctrl Pts',(-3.49029581516804,-7.11078553694575,
50.7148572245285));
#221170=CARTESIAN_POINT('Ctrl Pts',(-3.12459714627059,-7.27889873369191,
50.7317256310915));
#221171=CARTESIAN_POINT('Ctrl Pts',(-2.71265007469027,-7.4314767202868,
50.7495184547133));
#221172=CARTESIAN_POINT('Ctrl Pts',(-2.67752549716521,-7.44420404830618,
50.7510267054452));
#221173=CARTESIAN_POINT('Ctrl Pts',(-2.62759340962983,-7.46189772844314,
50.7531587116978));
#221174=CARTESIAN_POINT('Ctrl Pts',(-2.61285948021649,-7.46706971808667,
50.753786338776));
#221175=CARTESIAN_POINT('Ctrl Pts',(-2.58582625646578,-7.47646926780171,
50.754935212084));
#221176=CARTESIAN_POINT('Ctrl Pts',(-2.57353167521449,-7.48071018412298,
50.75545670412));
#221177=CARTESIAN_POINT('Ctrl Pts',(-2.54860953546499,-7.48923816337282,
50.7565117982853));
#221178=CARTESIAN_POINT('Ctrl Pts',(-2.5359814822688,-7.49352365411644,
50.7570453703211));
#221179=CARTESIAN_POINT('Ctrl Pts',(-2.50485960326084,-7.50399758018336,
50.7583578324285));
#221180=CARTESIAN_POINT('Ctrl Pts',(-2.48635359234213,-7.51014960790015,
50.7591360683082));
#221181=CARTESIAN_POINT('Ctrl Pts',(-2.41952424389723,-7.53209186697771,
50.7619387493956));
#221182=CARTESIAN_POINT('Ctrl Pts',(-2.37107127965403,-7.54748478093516,
50.7639563930259));
#221183=CARTESIAN_POINT('Ctrl Pts',(-2.10741176231317,-7.62845661047556,
50.7748600864445));
#221184=CARTESIAN_POINT('Ctrl Pts',(-1.88962625364266,-7.68530107065886,
50.7835902013705));
#221185=CARTESIAN_POINT('Ctrl Pts',(-1.35922573791527,-7.7998282154574,
50.8042984441705));
#221186=CARTESIAN_POINT('Ctrl Pts',(-1.04498338704565,-7.84811016597931,
50.8161073988341));
#221187=CARTESIAN_POINT('Ctrl Pts',(-0.207903721103711,-7.92554276268818,
50.8470925886929));
#221188=CARTESIAN_POINT('Ctrl Pts',(0.316337605352563,-7.92195174394789,
50.865972636626));
#221189=CARTESIAN_POINT('Ctrl Pts',(0.928553727129594,-7.85686367788499,
50.8899343797249));
#221190=CARTESIAN_POINT('Ctrl Pts',(1.02057731670896,-7.84544071648079,
50.8935900097282));
#221191=CARTESIAN_POINT('Ctrl Pts',(1.12726926054586,-7.83028807118377,
50.8979081171873));
#221192=CARTESIAN_POINT('Ctrl Pts',(1.14215574734217,-7.8281305244904,50.8985124250607));
#221193=CARTESIAN_POINT('Ctrl Pts',(1.16451267898166,-7.8248251318643,50.8994228105157));
#221194=CARTESIAN_POINT('Ctrl Pts',(1.17198782723061,-7.82370900890905,
50.8997276762696));
#221195=CARTESIAN_POINT('Ctrl Pts',(1.1852844575232,-7.821704189895,50.900270822695));
#221196=CARTESIAN_POINT('Ctrl Pts',(1.19110657470778,-7.82081970172647,
50.9005089398191));
#221197=CARTESIAN_POINT('Ctrl Pts',(1.20334533267836,-7.81894642272051,
50.9010101131069));
#221198=CARTESIAN_POINT('Ctrl Pts',(1.20976175251835,-7.81795623247324,
50.9012732241577));
#221199=CARTESIAN_POINT('Ctrl Pts',(1.22662957610809,-7.81533190500662,
50.9019658664896));
#221200=CARTESIAN_POINT('Ctrl Pts',(1.23707891235629,-7.81368470476932,
50.9023959184921));
#221201=CARTESIAN_POINT('Ctrl Pts',(1.28356969169995,-7.80626044965329,
50.9043137141617));
#221202=CARTESIAN_POINT('Ctrl Pts',(1.31957380868606,-7.80025501258658,
50.9058107651023));
#221203=CARTESIAN_POINT('Ctrl Pts',(1.57048580536669,-7.75661633244477,
50.9163328450662));
#221204=CARTESIAN_POINT('Ctrl Pts',(1.78376257117131,-7.71036227864182,
50.9257815686554));
#221205=CARTESIAN_POINT('Ctrl Pts',(2.42664186170662,-7.54284117060676,
50.9553694721891));
#221206=CARTESIAN_POINT('Ctrl Pts',(2.84815251033658,-7.3939885097737,50.9762124233281));
#221207=CARTESIAN_POINT('Ctrl Pts',(3.59400176165992,-7.05730305501481,
51.0136176912277));
#221208=CARTESIAN_POINT('Ctrl Pts',(3.92194185326242,-6.88046428132935,
51.0302762608795));
#221209=CARTESIAN_POINT('Ctrl Pts',(4.39363317978894,-6.58138594154004,
51.0541081547688));
#221210=CARTESIAN_POINT('Ctrl Pts',(4.547458196659,-6.47605464462263,51.0618636365923));
#221211=CARTESIAN_POINT('Ctrl Pts',(4.71266346588171,-6.35413901633539,
51.0701733093627));
#221212=CARTESIAN_POINT('Ctrl Pts',(4.72785968284902,-6.34284024767907,
51.0709374985991));
#221213=CARTESIAN_POINT('Ctrl Pts',(4.75041597862298,-6.32594297608029,
51.072071584344));
#221214=CARTESIAN_POINT('Ctrl Pts',(4.7578069907328,-6.32038599661947,51.0724431531572));
#221215=CARTESIAN_POINT('Ctrl Pts',(4.77046670412028,-6.31083292063964,
51.0730795360119));
#221216=CARTESIAN_POINT('Ctrl Pts',(4.77574016153975,-6.30684315938723,
51.0733446061722));
#221217=CARTESIAN_POINT('Ctrl Pts',(4.78600890076762,-6.29905383300283,
51.0738607306304));
#221218=CARTESIAN_POINT('Ctrl Pts',(4.79100467568514,-6.29525492630163,
51.0741118114144));
#221219=CARTESIAN_POINT('Ctrl Pts',(4.80297275199537,-6.28613161694719,
51.0747132749856));
#221220=CARTESIAN_POINT('Ctrl Pts',(4.80994073462674,-6.28080154853001,
51.0750634265904));
#221221=CARTESIAN_POINT('Ctrl Pts',(4.83091374697876,-6.26470314269561,
51.0761172702566));
#221222=CARTESIAN_POINT('Ctrl Pts',(4.84489163058013,-6.25389943876369,
51.0768195151905));
#221223=CARTESIAN_POINT('Ctrl Pts',(4.97133355543121,-6.15549235669783,
51.0831710719581));
#221224=CARTESIAN_POINT('Ctrl Pts',(5.08144987315789,-6.06490835568331,
51.0886957186609));
#221225=CARTESIAN_POINT('Ctrl Pts',(5.35892877845868,-5.82378290359019,
51.1026344550917));
#221226=CARTESIAN_POINT('Ctrl Pts',(5.52242547354013,-5.66898495797105,
51.1108620717518));
#221227=CARTESIAN_POINT('Ctrl Pts',(5.99339894599743,-5.18332940834571,
51.1348995119455));
#221228=CARTESIAN_POINT('Ctrl Pts',(6.2793790958365,-4.8329230006552,51.1499216900156));
#221229=CARTESIAN_POINT('Ctrl Pts',(6.82363446786695,-4.03559532756613,
51.1824267232602));
#221230=CARTESIAN_POINT('Ctrl Pts',(7.07128122062639,-3.58397456001204,
51.1999062801039));
#221231=CARTESIAN_POINT('Ctrl Pts',(7.28663647422192,-3.08058248197096,
51.2215118530094));
#221232=CARTESIAN_POINT('Ctrl Pts',(7.29970936240751,-3.04947580635208,
51.2228553307206));
#221233=CARTESIAN_POINT('Ctrl Pts',(7.31535572090004,-3.01156844589331,
51.2245037334189));
#221234=CARTESIAN_POINT('Ctrl Pts',(7.31811951398557,-3.00484618673897,
51.2247964778157));
#221235=CARTESIAN_POINT('Ctrl Pts',(7.32264532027286,-2.99379497596358,
51.2252784565775));
#221236=CARTESIAN_POINT('Ctrl Pts',(7.3244127728528,-2.98946824322873,51.2254673391091));
#221237=CARTESIAN_POINT('Ctrl Pts',(7.32758071117033,-2.98169344029259,
51.2258070733931));
#221238=CARTESIAN_POINT('Ctrl Pts',(7.32898260139996,-2.97824593995863,
51.2259578336435));
#221239=CARTESIAN_POINT('Ctrl Pts',(7.3319561285575,-2.97091868812755,51.2262785041984));
#221240=CARTESIAN_POINT('Ctrl Pts',(7.3335271192361,-2.96703867751138,51.226448456726));
#221241=CARTESIAN_POINT('Ctrl Pts',(7.33775565707316,-2.95657121920158,
51.2269073549054));
#221242=CARTESIAN_POINT('Ctrl Pts',(7.34040740631352,-2.94998145176252,
51.2271966822495));
#221243=CARTESIAN_POINT('Ctrl Pts',(7.35355119609214,-2.91719083622515,
51.2286384670204));
#221244=CARTESIAN_POINT('Ctrl Pts',(7.36391172199688,-2.89093785441998,
51.2297994417603));
#221245=CARTESIAN_POINT('Ctrl Pts',(7.45109231496194,-2.66651757213358,
51.2397764882567));
#221246=CARTESIAN_POINT('Ctrl Pts',(7.52003283004686,-2.46539761670041,
51.2490649921619));
#221247=CARTESIAN_POINT('Ctrl Pts',(7.7453106022586,-1.71033048793827,51.2845060583133));
#221248=CARTESIAN_POINT('Ctrl Pts',(7.84917815459769,-1.1425921410738,51.3121148467833));
#221249=CARTESIAN_POINT('Ctrl Pts',(7.92376928653246,-0.107455863215498,
51.3595018041555));
#221250=CARTESIAN_POINT('Ctrl Pts',(7.91651540116999,0.355741900989444,
51.3796904883554));
#221251=CARTESIAN_POINT('Ctrl Pts',(7.86557507855181,0.84714107187943,51.3997467850635));
#221252=CARTESIAN_POINT('Ctrl Pts',(7.86212888889296,0.87854919009609,51.4010231026232));
#221253=CARTESIAN_POINT('Ctrl Pts',(7.85720545556633,0.921069511043594,
51.4027435211936));
#221254=CARTESIAN_POINT('Ctrl Pts',(7.85589265232685,0.932200220829996,
51.4031931886683));
#221255=CARTESIAN_POINT('Ctrl Pts',(7.8537869074029,0.949733559674308,51.4039004297629));
#221256=CARTESIAN_POINT('Ctrl Pts',(7.85300978283221,0.956138050846054,
51.404158539072));
#221257=CARTESIAN_POINT('Ctrl Pts',(7.85149744012159,0.968475444926297,
51.4046553141591));
#221258=CARTESIAN_POINT('Ctrl Pts',(7.85076332967054,0.974408477683425,
51.4048940172912));
#221259=CARTESIAN_POINT('Ctrl Pts',(7.84901469924289,0.988410536810985,
51.4054569018433));
#221260=CARTESIAN_POINT('Ctrl Pts',(7.84799445978118,0.996478849751861,
51.4057808891804));
#221261=CARTESIAN_POINT('Ctrl Pts',(7.84498150058779,1.02001444218521,51.4067249291445));
#221262=CARTESIAN_POINT('Ctrl Pts',(7.84295547827992,1.03547746299875,51.4073438526169));
#221263=CARTESIAN_POINT('Ctrl Pts',(7.83829573786301,1.0702431734016,51.4087324598477));
#221264=CARTESIAN_POINT('Ctrl Pts',(7.83563641174783,1.08954236021146,51.4095012740764));
#221265=CARTESIAN_POINT('Ctrl Pts',(7.81260586231883,1.25223263785313,51.4159654449639));
#221266=CARTESIAN_POINT('Ctrl Pts',(7.78837121374084,1.39505326231059,51.4215288095821));
#221267=CARTESIAN_POINT('Ctrl Pts',(7.70536079225613,1.81413195357768,51.4375805343184));
#221268=CARTESIAN_POINT('Ctrl Pts',(7.63569988046149,2.0880041636256,51.4477088983109));
#221269=CARTESIAN_POINT('Ctrl Pts',(7.46312542582521,2.64077602578509,51.4679071480701));
#221270=CARTESIAN_POINT('Ctrl Pts',(7.35884965397134,2.91877954939865,51.4779319646777));
#221271=CARTESIAN_POINT('Ctrl Pts',(7.03822376863279,3.64632842248934,51.5049712475368));
#221272=CARTESIAN_POINT('Ctrl Pts',(6.79461702771615,4.08232351738125,51.5220151060109));
#221273=CARTESIAN_POINT('Ctrl Pts',(6.49385402679533,4.51827011516617,51.5429450989516));
#221274=CARTESIAN_POINT('Ctrl Pts',(6.4758877379527,4.54398315484607,51.5441951960781));
#221275=CARTESIAN_POINT('Ctrl Pts',(6.4532314067712,4.57600121584495,51.5457723623038));
#221276=CARTESIAN_POINT('Ctrl Pts',(6.44868405341011,4.58240730349968,51.5460889512797));
#221277=CARTESIAN_POINT('Ctrl Pts',(6.44148417213284,4.59251820048186,51.5465902532252));
#221278=CARTESIAN_POINT('Ctrl Pts',(6.438837961864,4.59622752507792,51.546774508435));
#221279=CARTESIAN_POINT('Ctrl Pts',(6.43414840242404,4.60278911599557,51.5471010547285));
#221280=CARTESIAN_POINT('Ctrl Pts',(6.43210635535538,4.60564231612314,51.547243252158));
#221281=CARTESIAN_POINT('Ctrl Pts',(6.42741406828286,4.6121892917171,51.5475700065591));
#221282=CARTESIAN_POINT('Ctrl Pts',(6.42476254324614,4.61588214001647,51.547754655433));
#221283=CARTESIAN_POINT('Ctrl Pts',(6.41742310120222,4.62608539720852,51.5482657767697));
#221284=CARTESIAN_POINT('Ctrl Pts',(6.41272847291706,4.63259094825321,51.5485927256276));
#221285=CARTESIAN_POINT('Ctrl Pts',(6.38729957637856,4.66771615651435,51.5503636961705));
#221286=CARTESIAN_POINT('Ctrl Pts',(6.36638389438506,4.69620336336403,51.5518204239993));
#221287=CARTESIAN_POINT('Ctrl Pts',(6.04847316960574,5.12317153045162,51.573951318478));
#221288=CARTESIAN_POINT('Ctrl Pts',(5.71479022107682,5.49290431171215,51.5969875042569));
#221289=CARTESIAN_POINT('Ctrl Pts',(5.15457249096666,6.00697129978001,51.632450132198));
#221290=CARTESIAN_POINT('Ctrl Pts',(4.95168881088706,6.17528177636811,51.6447655609537));
#221291=CARTESIAN_POINT('Ctrl Pts',(4.31431316721881,6.65239915056125,51.6813685007465));
#221292=CARTESIAN_POINT('Ctrl Pts',(3.85664452218045,6.92778102496164,51.7048305115745));
#221293=CARTESIAN_POINT('Ctrl Pts',(3.34335201789069,7.16987586097758,51.7279440336819));
#221294=CARTESIAN_POINT('Ctrl Pts',(3.31190332904333,7.18445676139648,51.7293486614492));
#221295=CARTESIAN_POINT('Ctrl Pts',(3.26921581274263,7.20390858760205,51.7312399236168));
#221296=CARTESIAN_POINT('Ctrl Pts',(3.25806026271668,7.20896069451518,51.731732758106));
#221297=CARTESIAN_POINT('Ctrl Pts',(3.24047625381636,7.21687495831333,51.7325073845961));
#221298=CARTESIAN_POINT('Ctrl Pts',(3.2340556527941,7.2197544660765,51.7327897683564));
#221299=CARTESIAN_POINT('Ctrl Pts',(3.22168486445983,7.22528269718834,51.7333329596235));
#221300=CARTESIAN_POINT('Ctrl Pts',(3.21573523279332,7.22793264585477,51.733593808706));
#221301=CARTESIAN_POINT('Ctrl Pts',(3.20169452538161,7.23416556826426,51.7342084668592));
#221302=CARTESIAN_POINT('Ctrl Pts',(3.19360068950142,7.23774232337614,51.734562064444));
#221303=CARTESIAN_POINT('Ctrl Pts',(3.17000216809267,7.2481234777252,51.7355909166724));
#221304=CARTESIAN_POINT('Ctrl Pts',(3.1544815743588,7.25489170805623,51.7362649454632));
#221305=CARTESIAN_POINT('Ctrl Pts',(3.04365887101114,7.30279647515724,51.7410591091237));
#221306=CARTESIAN_POINT('Ctrl Pts',(2.94757504752495,7.34210446787291,51.7451173363025));
#221307=CARTESIAN_POINT('Ctrl Pts',(2.64085365278465,7.46059252142293,51.7577832761653));
#221308=CARTESIAN_POINT('Ctrl Pts',(2.42759347594129,7.5326852359243,51.7661614800352));
#221309=CARTESIAN_POINT('Ctrl Pts',(1.81932403050469,7.70978964033411,51.7891548467233));
#221310=CARTESIAN_POINT('Ctrl Pts',(1.41884239132787,7.7934391603952,51.8032253428223));
#221311=CARTESIAN_POINT('Ctrl Pts',(0.504071196503408,7.91162956739007,
51.8352107630675));
#221312=CARTESIAN_POINT('Ctrl Pts',(-0.0107690511506302,7.92766572568367,
51.8531772405592));
#221313=CARTESIAN_POINT('Ctrl Pts',(-0.559038632226526,7.89130301784501,
51.8749293513342));
#221314=CARTESIAN_POINT('Ctrl Pts',(-0.594532066426574,7.88870832799293,
51.876347317049));
#221315=CARTESIAN_POINT('Ctrl Pts',(-0.641855534574459,7.88492763252809,
51.8782500900988));
#221316=CARTESIAN_POINT('Ctrl Pts',(-0.653702457337308,7.88395429927047,
51.8787274496849));
#221317=CARTESIAN_POINT('Ctrl Pts',(-0.672183163184198,7.88239399841931,
51.8794736663263));
#221318=CARTESIAN_POINT('Ctrl Pts',(-0.678818500791426,7.88182534657297,
51.8797419019709));
#221319=CARTESIAN_POINT('Ctrl Pts',(-0.692102931663866,7.88066996433184,
51.8802795477937));
#221320=CARTESIAN_POINT('Ctrl Pts',(-0.698752015983833,7.88008319591775,
51.8805489590296));
#221321=CARTESIAN_POINT('Ctrl Pts',(-0.713738016078834,7.87874159485013,
51.8811568601622));
#221322=CARTESIAN_POINT('Ctrl Pts',(-0.722074487042778,7.87798194391178,
51.8814955074101));
#221323=CARTESIAN_POINT('Ctrl Pts',(-0.746670719876964,7.87570127224605,
51.8824960620968));
#221324=CARTESIAN_POINT('Ctrl Pts',(-0.762926949777184,7.87414313806338,
51.8831591546484));
#221325=CARTESIAN_POINT('Ctrl Pts',(-0.890657268889658,7.86150112621064,
51.8883829814816));
#221326=CARTESIAN_POINT('Ctrl Pts',(-1.00188710518627,7.84810113607214,
51.8930138278287));
#221327=CARTESIAN_POINT('Ctrl Pts',(-1.4173907905058,7.78906782060753,51.9105526401867));
#221328=CARTESIAN_POINT('Ctrl Pts',(-1.71919973981018,7.72806047636063,
51.923764983382));
#221329=CARTESIAN_POINT('Ctrl Pts',(-2.15833879410559,7.61228982175401,
51.9433029058731));
#221330=CARTESIAN_POINT('Ctrl Pts',(-2.29893252332808,7.57101658615155,
51.9496094193611));
#221331=CARTESIAN_POINT('Ctrl Pts',(-3.1397074359222,7.29861450688728,51.9875468585231));
#221332=CARTESIAN_POINT('Ctrl Pts',(-3.80593010888782,6.9744177836307,52.0182039409521));
#221333=CARTESIAN_POINT('Ctrl Pts',(-4.51715674106673,6.49566132404436,
52.0532203229488));
#221334=CARTESIAN_POINT('Ctrl Pts',(-4.61516770633612,6.4263946810876,52.0580986816982));
#221335=CARTESIAN_POINT('Ctrl Pts',(-4.74069260370534,6.33333003531172,
52.0644152510801));
#221336=CARTESIAN_POINT('Ctrl Pts',(-4.76967063906559,6.31153528937594,
52.0658783857615));
#221337=CARTESIAN_POINT('Ctrl Pts',(-4.81610291973277,6.27611057959156,
52.0682308341278));
#221338=CARTESIAN_POINT('Ctrl Pts',(-4.83365150353797,6.26260524754771,
52.0691217861421));
#221339=CARTESIAN_POINT('Ctrl Pts',(-4.86644478718618,6.2371476955178,52.0707902615155));
#221340=CARTESIAN_POINT('Ctrl Pts',(-4.88170273341824,6.22521282105096,
52.0715680141047));
#221341=CARTESIAN_POINT('Ctrl Pts',(-4.91658743398862,6.19771863637366,
52.0733495740153));
#221342=CARTESIAN_POINT('Ctrl Pts',(-4.93618445945907,6.18212190749689,
52.0743528502155));
#221343=CARTESIAN_POINT('Ctrl Pts',(-4.99500979439336,6.13484641409477,
52.0773719565386));
#221344=CARTESIAN_POINT('Ctrl Pts',(-5.03400974699968,6.10288532424101,
52.0793837118689));
#221345=CARTESIAN_POINT('Ctrl Pts',(-5.12244505268295,6.02898663855011,
52.0839696579611));
#221346=CARTESIAN_POINT('Ctrl Pts',(-5.17167592738975,5.98680978468854,
52.0865401855486));
#221347=CARTESIAN_POINT('Ctrl Pts',(-5.33316153641293,5.84498405226461,
52.0950340762327));
#221348=CARTESIAN_POINT('Ctrl Pts',(-5.44309929502286,5.74274512833629,
52.1009175962134));
#221349=CARTESIAN_POINT('Ctrl Pts',(-5.74076968088533,5.44968842352764,
52.1171866084284));
#221350=CARTESIAN_POINT('Ctrl Pts',(-5.92182762584419,5.25238045739707,
52.1274752605463));
#221351=CARTESIAN_POINT('Ctrl Pts',(-6.33807021666432,4.74983664057066,
52.1525459708026));
#221352=CARTESIAN_POINT('Ctrl Pts',(-6.56163101543227,4.43588335381606,
52.167277404458));
#221353=CARTESIAN_POINT('Ctrl Pts',(-6.783098461993,4.07126960118406,52.1842540684907));
#221354=CARTESIAN_POINT('Ctrl Pts',(-6.80447051966529,4.03544815461553,
52.1859208580246));
#221355=CARTESIAN_POINT('Ctrl Pts',(-6.83250411751814,3.98760545342949,
52.188147086145));
#221356=CARTESIAN_POINT('Ctrl Pts',(-6.8394191790698,3.97573327299858,52.1886995413469));
#221357=CARTESIAN_POINT('Ctrl Pts',(-6.8511815742741,3.95541740248493,52.1896449113731));
#221358=CARTESIAN_POINT('Ctrl Pts',(-6.85604432307434,3.94698264892919,
52.1900374091311));
#221359=CARTESIAN_POINT('Ctrl Pts',(-6.86546461324758,3.93057260720118,
52.1908010041881));
#221360=CARTESIAN_POINT('Ctrl Pts',(-6.87002386076315,3.92259831339526,
52.1911720563455));
#221361=CARTESIAN_POINT('Ctrl Pts',(-6.87944923989044,3.90604613579889,
52.191942212168));
#221362=CARTESIAN_POINT('Ctrl Pts',(-6.8843132401745,3.89746705819821,52.1923413688658));
#221363=CARTESIAN_POINT('Ctrl Pts',(-6.89533705725171,3.87793833175498,
52.1932499136883));
#221364=CARTESIAN_POINT('Ctrl Pts',(-6.90148685382313,3.86698306735794,
52.1937595456643));
#221365=CARTESIAN_POINT('Ctrl Pts',(-6.91710291469134,3.8390086647724,52.1950607347738));
#221366=CARTESIAN_POINT('Ctrl Pts',(-6.92653246322216,3.82196916419084,
52.1958531497359));
#221367=CARTESIAN_POINT('Ctrl Pts',(-7.01557173815238,3.6596605055552,52.2033991550164));
#221368=CARTESIAN_POINT('Ctrl Pts',(-7.09066176988678,3.51196177598958,
52.2102493619808));
#221369=CARTESIAN_POINT('Ctrl Pts',(-7.38279973148594,2.88971137013535,
52.2388873792428));
#221370=CARTESIAN_POINT('Ctrl Pts',(-7.55727388721529,2.39662130011934,
52.2609806885891));
#221371=CARTESIAN_POINT('Ctrl Pts',(-7.71816766020533,1.7426469761399,52.2888577329158));
#221372=CARTESIAN_POINT('Ctrl Pts',(-7.75016264639936,1.59433702197289,
52.2950957528323));
#221373=CARTESIAN_POINT('Ctrl Pts',(-7.79607812790603,1.34722554614238,
52.3053578060762));
#221374=CARTESIAN_POINT('Ctrl Pts',(-7.81242954179104,1.2489178596798,52.309406401178));
#221375=CARTESIAN_POINT('Ctrl Pts',(-7.83244073755938,1.11276000862184,
52.3149711377105));
#221376=CARTESIAN_POINT('Ctrl Pts',(-7.83769142509056,1.07515388962323,
52.3165036351529));
#221377=CARTESIAN_POINT('Ctrl Pts',(-7.84567886659451,1.01477587126273,
52.3189573249605));
#221378=CARTESIAN_POINT('Ctrl Pts',(-7.848587679112,0.992027415754827,52.3198802521722));
#221379=CARTESIAN_POINT('Ctrl Pts',(-7.85424943783336,0.946165195015163,
52.3217379273752));
#221380=CARTESIAN_POINT('Ctrl Pts',(-7.85699937265996,0.923051282302919,
52.3226726364649));
#221381=CARTESIAN_POINT('Ctrl Pts',(-7.86238184616331,0.876042566886318,
52.3245706389048));
#221382=CARTESIAN_POINT('Ctrl Pts',(-7.86500756444916,0.852147222655544,
52.3255338561054));
#221383=CARTESIAN_POINT('Ctrl Pts',(-7.87083848874207,0.796758777953407,
52.3277630797707));
#221384=CARTESIAN_POINT('Ctrl Pts',(-7.87396366651727,0.765257638552243,
52.3290283088682));
#221385=CARTESIAN_POINT('Ctrl Pts',(-7.88514882816963,0.6451816253484,52.3338418596193));
#221386=CARTESIAN_POINT('Ctrl Pts',(-7.89190400436654,0.556491449336632,
52.3373780185071));
#221387=CARTESIAN_POINT('Ctrl Pts',(-7.90634940986654,0.312582307885866,
52.3470621327352));
#221388=CARTESIAN_POINT('Ctrl Pts',(-7.9109639325235,0.15722082092995,52.3531904209946));
#221389=CARTESIAN_POINT('Ctrl Pts',(-7.91099978939441,0.00182543188703851,
52.3592866701075));
#221390=CARTESIAN_POINT('',(-7.91934491493686,0.00236459517639777,56.3576684917633));
#221391=CARTESIAN_POINT('Ctrl Pts',(-7.9109997887806,0.00182809008343179,
52.3592865658249));
#221392=CARTESIAN_POINT('Ctrl Pts',(-7.91119646617743,-0.849286884464968,
52.3926762906361));
#221393=CARTESIAN_POINT('Ctrl Pts',(-7.7740466783572,-1.69487562970979,
52.423722529026));
#221394=CARTESIAN_POINT('Ctrl Pts',(-7.44295841195928,-2.6878487431774,
52.4630109752596));
#221395=CARTESIAN_POINT('Ctrl Pts',(-7.37424828576619,-2.87099608398839,
52.4704332882737));
#221396=CARTESIAN_POINT('Ctrl Pts',(-7.26632607255126,-3.12914139336323,
52.4813427238853));
#221397=CARTESIAN_POINT('Ctrl Pts',(-7.23258701250455,-3.20635384665817,
52.4846650845882));
#221398=CARTESIAN_POINT('Ctrl Pts',(-7.19177196686032,-3.29583611258907,
52.4885992268777));
#221399=CARTESIAN_POINT('Ctrl Pts',(-7.18588787205115,-3.30864552220287,
52.4891644266056));
#221400=CARTESIAN_POINT('Ctrl Pts',(-7.17685456187478,-3.32817286885108,
52.4900292331509));
#221401=CARTESIAN_POINT('Ctrl Pts',(-7.1737300632019,-3.33490225150739,
52.4903278359422));
#221402=CARTESIAN_POINT('Ctrl Pts',(-7.16803267913505,-3.34712792403135,
52.4908713944099));
#221403=CARTESIAN_POINT('Ctrl Pts',(-7.1654629249818,-3.35262567242916,
52.4911162202184));
#221404=CARTESIAN_POINT('Ctrl Pts',(-7.15991313359746,-3.3644634037863,
52.4916442369079));
#221405=CARTESIAN_POINT('Ctrl Pts',(-7.15693099750073,-3.37080239300474,
52.49192751608));
#221406=CARTESIAN_POINT('Ctrl Pts',(-7.14887160078172,-3.38787497175459,
52.4926919146789));
#221407=CARTESIAN_POINT('Ctrl Pts',(-7.14377860001328,-3.39860107995461,
52.493173709312));
#221408=CARTESIAN_POINT('Ctrl Pts',(-7.1201924955951,-3.44798730080933,
52.4953993509368));
#221409=CARTESIAN_POINT('Ctrl Pts',(-7.10140982208081,-3.48650771356148,
52.4971560054075));
#221410=CARTESIAN_POINT('Ctrl Pts',(-6.83843456813954,-4.01488806981178,
52.521561416813));
#221411=CARTESIAN_POINT('Ctrl Pts',(-6.54439384039041,-4.4781963339638,
52.5468120377884));
#221412=CARTESIAN_POINT('Ctrl Pts',(-6.11888112045396,-5.01622080723766,
52.5784190523372));
#221413=CARTESIAN_POINT('Ctrl Pts',(-6.029951030074,-5.12277936971555,52.5848094843894));
#221414=CARTESIAN_POINT('Ctrl Pts',(-5.91001079051183,-5.25904192237671,
52.5931219020823));
#221415=CARTESIAN_POINT('Ctrl Pts',(-5.88149804853277,-5.29091015055192,
52.5950764406383));
#221416=CARTESIAN_POINT('Ctrl Pts',(-5.81272016056783,-5.36653905115986,
52.5997386153237));
#221417=CARTESIAN_POINT('Ctrl Pts',(-5.77221707065414,-5.41008015153635,
52.6024420373466));
#221418=CARTESIAN_POINT('Ctrl Pts',(-5.38751487540486,-5.81439895944724,
52.6277144984721));
#221419=CARTESIAN_POINT('Ctrl Pts',(-5.01038963351085,-6.14236584293915,
52.6493971512202));
#221420=CARTESIAN_POINT('Ctrl Pts',(-4.5864839144347,-6.44582007393821,
52.6705380287873));
#221421=CARTESIAN_POINT('Ctrl Pts',(-4.56806232492975,-6.45888827346036,
52.6714510474623));
#221422=CARTESIAN_POINT('Ctrl Pts',(-4.54125490759907,-6.47773328750249,
52.6727714948196));
#221423=CARTESIAN_POINT('Ctrl Pts',(-4.53291357146582,-6.48357302992665,
52.673181218036));
#221424=CARTESIAN_POINT('Ctrl Pts',(-4.51832015166986,-6.49374790764697,
52.6738960503734));
#221425=CARTESIAN_POINT('Ctrl Pts',(-4.51207305480041,-6.49809015246708,
52.6742014178902));
#221426=CARTESIAN_POINT('Ctrl Pts',(-4.49997928226364,-6.50647046780809,
52.6747913551646));
#221427=CARTESIAN_POINT('Ctrl Pts',(-4.49413341296765,-6.51050968481054,
52.6750759663727));
#221428=CARTESIAN_POINT('Ctrl Pts',(-4.48024109875156,-6.52008098461047,
52.6757510197887));
#221429=CARTESIAN_POINT('Ctrl Pts',(-4.47218982891529,-6.52560606256914,
52.6761412081885));
#221430=CARTESIAN_POINT('Ctrl Pts',(-4.44376467379382,-6.54503513653207,
52.6775151324094));
#221431=CARTESIAN_POINT('Ctrl Pts',(-4.42333591904498,-6.55885880128651,
52.6784959674633));
#221432=CARTESIAN_POINT('Ctrl Pts',(-4.15522084767664,-6.73846365612211,
52.6912837185592));
#221433=CARTESIAN_POINT('Ctrl Pts',(-3.89841284420971,-6.89022133476271,
52.7025731614423));
#221434=CARTESIAN_POINT('Ctrl Pts',(-3.30337905130952,-7.19790528298636,
52.7270625360408));
#221435=CARTESIAN_POINT('Ctrl Pts',(-2.96148521637809,-7.34518715173454,
52.7400060225158));
#221436=CARTESIAN_POINT('Ctrl Pts',(-2.42815231856111,-7.53162060067291,
52.7595337157709));
#221437=CARTESIAN_POINT('Ctrl Pts',(-2.2435377630356,-7.58866061725906,
52.7661838452677));
#221438=CARTESIAN_POINT('Ctrl Pts',(-1.86262541601725,-7.69123383801406,
52.7799311814493));
#221439=CARTESIAN_POINT('Ctrl Pts',(-1.66630635933668,-7.73614051193638,
52.7870306085686));
#221440=CARTESIAN_POINT('Ctrl Pts',(-1.2531059643277,-7.81419825148433,
52.8023220801888));
#221441=CARTESIAN_POINT('Ctrl Pts',(-1.03613198034881,-7.84591535733134,
52.8105490664315));
#221442=CARTESIAN_POINT('Ctrl Pts',(-0.785689960523596,-7.8719550539589,
52.8205096169565));
#221443=CARTESIAN_POINT('Ctrl Pts',(-0.75322464998402,-7.87512778504,52.8218098358847));
#221444=CARTESIAN_POINT('Ctrl Pts',(-0.711457395074118,-7.87894893282157,
52.8234933859347));
#221445=CARTESIAN_POINT('Ctrl Pts',(-0.702172093536987,-7.87978186633176,
52.8238683415471));
#221446=CARTESIAN_POINT('Ctrl Pts',(-0.687214092755923,-7.88109701772237,
52.8244734489482));
#221447=CARTESIAN_POINT('Ctrl Pts',(-0.681542288638739,-7.88158953007479,
52.8247031445438));
#221448=CARTESIAN_POINT('Ctrl Pts',(-0.670743673371047,-7.88251548661697,
52.8251409338568));
#221449=CARTESIAN_POINT('Ctrl Pts',(-0.665616959167033,-7.88295005284269,
52.8253489784883));
#221450=CARTESIAN_POINT('Ctrl Pts',(-0.653935908396738,-7.8839287213393,
52.825823454277));
#221451=CARTESIAN_POINT('Ctrl Pts',(-0.647381315194075,-7.88446965165159,
52.8260900218814));
#221452=CARTESIAN_POINT('Ctrl Pts',(-0.627866225437084,-7.88605567250676,
52.8268846293151));
#221453=CARTESIAN_POINT('Ctrl Pts',(-0.614903858146825,-7.88707698132475,
52.827413674992));
#221454=CARTESIAN_POINT('Ctrl Pts',(-0.524487526524967,-7.89397666013232,
52.8311123630761));
#221455=CARTESIAN_POINT('Ctrl Pts',(-0.446954764783016,-7.89874582316162,
52.8343271527586));
#221456=CARTESIAN_POINT('Ctrl Pts',(-0.341818402105852,-7.90366002039431,
52.8387339909716));
#221457=CARTESIAN_POINT('Ctrl Pts',(-0.31426426536002,-7.90480357054582,
52.8398933559037));
#221458=CARTESIAN_POINT('Ctrl Pts',(-0.253604906586833,-7.90700338954029,
52.8424546257411));
#221459=CARTESIAN_POINT('Ctrl Pts',(-0.220497938893828,-7.90799586980192,
52.8438584074659));
#221460=CARTESIAN_POINT('Ctrl Pts',(-0.185011916436274,-7.90883665465911,
52.8453687456014));
#221461=CARTESIAN_POINT('Ctrl Pts',(-0.182637837061959,-7.90889183512866,
52.8454698172215));
#221462=CARTESIAN_POINT('Ctrl Pts',(0.425420965005026,-7.92275094494516,
52.8713636159861));
#221463=CARTESIAN_POINT('Ctrl Pts',(1.03069311791269,-7.8669367083047,52.8986734608375));
#221464=CARTESIAN_POINT('Ctrl Pts',(1.88356150178577,-7.68808326487359,
52.9362743536675));
#221465=CARTESIAN_POINT('Ctrl Pts',(2.14053999471102,-7.62053328988184,
52.9475197554204));
#221466=CARTESIAN_POINT('Ctrl Pts',(2.47924432325361,-7.51301099576739,
52.9622222051086));
#221467=CARTESIAN_POINT('Ctrl Pts',(2.56437567350824,-7.48438136862762,
52.9659081796846));
#221468=CARTESIAN_POINT('Ctrl Pts',(2.70594550314423,-7.43407236636109,
52.9720265941409));
#221469=CARTESIAN_POINT('Ctrl Pts',(2.76265546285147,-7.41318473615827,
52.97447448468));
#221470=CARTESIAN_POINT('Ctrl Pts',(2.83837856524004,-7.38430449791696,
52.9777406354176));
#221471=CARTESIAN_POINT('Ctrl Pts',(2.85760738896977,-7.37688456008501,
52.9785698184246));
#221472=CARTESIAN_POINT('Ctrl Pts',(2.88932765143184,-7.36450184178956,
52.979937400091));
#221473=CARTESIAN_POINT('Ctrl Pts',(2.90183579801819,-7.35958223390965,
52.9804766082397));
#221474=CARTESIAN_POINT('Ctrl Pts',(2.9143346659203,-7.3546294573573,52.9810153669147));
#221475=CARTESIAN_POINT('Ctrl Pts',(2.91433796399321,-7.35462815046692,
52.9810155090768));
#221476=CARTESIAN_POINT('Ctrl Pts',(2.91434456184307,-7.35462553600578,
52.9810157934745));
#221477=CARTESIAN_POINT('Ctrl Pts',(2.91434785918889,-7.35462422939838,
52.9810159356052));
#221478=CARTESIAN_POINT('Ctrl Pts',(2.91435445255371,-7.35462161670421,
52.9810162198095));
#221479=CARTESIAN_POINT('Ctrl Pts',(2.91435775226989,-7.3546203091524,52.9810163620425));
#221480=CARTESIAN_POINT('Ctrl Pts',(2.91436434982926,-7.35461769478583,
52.9810166464276));
#221481=CARTESIAN_POINT('Ctrl Pts',(2.91436764912413,-7.35461638739583,
52.9810167886423));
#221482=CARTESIAN_POINT('Ctrl Pts',(2.91437425057796,-7.35461377147575,
52.9810170731953));
#221483=CARTESIAN_POINT('Ctrl Pts',(2.91437754820863,-7.35461246474007,
52.9810172153383));
#221484=CARTESIAN_POINT('Ctrl Pts',(2.91438414645053,-7.35460985008249,
52.9810174997528));
#221485=CARTESIAN_POINT('Ctrl Pts',(2.91438744534538,-7.35460854284073,
52.9810176419503));
#221486=CARTESIAN_POINT('Ctrl Pts',(2.9143940417932,-7.35460592888381,52.9810179262874));
#221487=CARTESIAN_POINT('Ctrl Pts',(2.9143973427108,-7.35460462083536,52.9810180685721));
#221488=CARTESIAN_POINT('Ctrl Pts',(2.91440394373701,-7.35460200505389,
52.9810183531066));
#221489=CARTESIAN_POINT('Ctrl Pts',(2.91440724386871,-7.35460069731173,
52.9810184953574));
#221490=CARTESIAN_POINT('Ctrl Pts',(2.91441384477225,-7.35459808156859,
52.9810187798866));
#221491=CARTESIAN_POINT('Ctrl Pts',(2.9144171450662,-7.35459677375699,52.9810189221444));
#221492=CARTESIAN_POINT('Ctrl Pts',(2.91442374758804,-7.35459415736229,
52.9810192067433));
#221493=CARTESIAN_POINT('Ctrl Pts',(2.91442704764742,-7.3545928496385,52.981019348991));
#221494=CARTESIAN_POINT('Ctrl Pts',(2.91443364709967,-7.3545902344499,52.9810196334576));
#221495=CARTESIAN_POINT('Ctrl Pts',(2.91443694906994,-7.35458892596374,
52.9810197757876));
#221496=CARTESIAN_POINT('Ctrl Pts',(2.91444355359865,-7.35458630875319,
52.981020060473));
#221497=CARTESIAN_POINT('Ctrl Pts',(2.9144468544801,-7.35458500069335,52.9810202027561));
#221498=CARTESIAN_POINT('Ctrl Pts',(2.91445345652773,-7.35458238445571,
52.9810204873345));
#221499=CARTESIAN_POINT('Ctrl Pts',(2.9144567585994,-7.35458107591907,52.9810206296689));
#221500=CARTESIAN_POINT('Ctrl Pts',(2.9144633624289,-7.35457845896502,52.9810209143241));
#221501=CARTESIAN_POINT('Ctrl Pts',(2.91446666469943,-7.35457715034443,
52.9810210566671));
#221502=CARTESIAN_POINT('Ctrl Pts',(2.91447326748367,-7.3545745337943,52.9810213412773));
#221503=CARTESIAN_POINT('Ctrl Pts',(2.91447657087126,-7.3545732247259,52.9810214836684));
#221504=CARTESIAN_POINT('Ctrl Pts',(2.91448317833929,-7.35457060630938,
52.9810217684804));
#221505=CARTESIAN_POINT('Ctrl Pts',(2.91448648043816,-7.35456929774653,
52.9810219108159));
#221506=CARTESIAN_POINT('Ctrl Pts',(2.91449308627621,-7.35456667996564,
52.9810221955577));
#221507=CARTESIAN_POINT('Ctrl Pts',(2.91449638904102,-7.35456537113373,
52.9810223379219));
#221508=CARTESIAN_POINT('Ctrl Pts',(2.91450299337868,-7.35456275393713,
52.981022622599));
#221509=CARTESIAN_POINT('Ctrl Pts',(2.91450629772253,-7.35456144447433,
52.9810227650313));
#221510=CARTESIAN_POINT('Ctrl Pts',(2.91451290647998,-7.35455882551593,
52.9810230498989));
#221511=CARTESIAN_POINT('Ctrl Pts',(2.91451620989901,-7.35455751641447,
52.9810231922913));
#221512=CARTESIAN_POINT('Ctrl Pts',(2.91452281742994,-7.35455489793182,
52.981023477106));
#221513=CARTESIAN_POINT('Ctrl Pts',(2.91452612149604,-7.35455358856878,
52.9810236195263));
#221514=CARTESIAN_POINT('Ctrl Pts',(2.91453273151748,-7.35455096908886,
52.9810239044484));
#221515=CARTESIAN_POINT('Ctrl Pts',(2.91453603515875,-7.35454965988902,
52.9810240468504));
#221516=CARTESIAN_POINT('Ctrl Pts',(2.91454264288666,-7.3545470413077,52.9810243316735));
#221517=CARTESIAN_POINT('Ctrl Pts',(2.9145459479584,-7.35454573153583,52.9810244741372));
#221518=CARTESIAN_POINT('Ctrl Pts',(2.91455255838938,-7.354543111873,52.9810247590768));
#221519=CARTESIAN_POINT('Ctrl Pts',(2.91455586332221,-7.35454180215102,
52.9810249015345));
#221520=CARTESIAN_POINT('Ctrl Pts',(2.91456247215089,-7.35453918311286,
52.9810251864051));
#221521=CARTESIAN_POINT('Ctrl Pts',(2.91456577831281,-7.35453787289865,
52.9810253289157));
#221522=CARTESIAN_POINT('Ctrl Pts',(2.91457239009006,-7.35453525268167,
52.9810256139134));
#221523=CARTESIAN_POINT('Ctrl Pts',(2.91457569588938,-7.35453394260599,
52.9810257564083));
#221524=CARTESIAN_POINT('Ctrl Pts',(2.91458230879692,-7.35453132193076,
52.9810260414547));
#221525=CARTESIAN_POINT('Ctrl Pts',(2.91458561434799,-7.35453001194831,
52.981026183939));
#221526=CARTESIAN_POINT('Ctrl Pts',(2.91459222526276,-7.3545273920525,52.9810264688994));
#221527=CARTESIAN_POINT('Ctrl Pts',(2.91459553218407,-7.35452608152186,
52.9810266114428));
#221528=CARTESIAN_POINT('Ctrl Pts',(2.91460214775043,-7.35452345977231,
52.9810268966037));
#221529=CARTESIAN_POINT('Ctrl Pts',(2.91460545352993,-7.35452214968901,
52.9810270390978));
#221530=CARTESIAN_POINT('Ctrl Pts',(2.9146120675619,-7.35451952853721,52.9810273241926));
#221531=CARTESIAN_POINT('Ctrl Pts',(2.91461537403595,-7.3545182181735,52.9810274667167));
#221532=CARTESIAN_POINT('Ctrl Pts',(2.91462198598216,-7.35451559783797,
52.9810277517215));
#221533=CARTESIAN_POINT('Ctrl Pts',(2.91462529434583,-7.35451428672024,
52.981027894327));
#221534=CARTESIAN_POINT('Ctrl Pts',(2.91463190910869,-7.35451166525814,
52.9810281794533));
#221535=CARTESIAN_POINT('Ctrl Pts',(2.91463521750736,-7.35451035412137,
52.9810283220603));
#221536=CARTESIAN_POINT('Ctrl Pts',(2.91464183561226,-7.35450773132448,
52.9810286073306));
#221537=CARTESIAN_POINT('Ctrl Pts',(2.91464514285756,-7.35450642063963,
52.9810287498879));
#221538=CARTESIAN_POINT('Ctrl Pts',(2.91465175799495,-7.35450379900844,
52.9810290350303));
#221539=CARTESIAN_POINT('Ctrl Pts',(2.91465506664666,-7.35450248776106,
52.9810291776482));
#221540=CARTESIAN_POINT('Ctrl Pts',(2.9146616827465,-7.35449986573812,52.981029462832));
#221541=CARTESIAN_POINT('Ctrl Pts',(2.91466499212062,-7.35449855419927,
52.981029605481));
#221542=CARTESIAN_POINT('Ctrl Pts',(2.91467161061857,-7.3544959312156,52.9810298907682));
#221543=CARTESIAN_POINT('Ctrl Pts',(2.91467491965505,-7.3544946198054,52.9810300334027));
#221544=CARTESIAN_POINT('Ctrl Pts',(2.91468153956378,-7.35449199625228,
52.9810303187507));
#221545=CARTESIAN_POINT('Ctrl Pts',(2.91468484822723,-7.35449068498474,
52.9810304613691));
#221546=CARTESIAN_POINT('Ctrl Pts',(2.92671562101463,-7.34972271957208,
52.9815490420874));
#221547=CARTESIAN_POINT('Ctrl Pts',(2.9387313940353,-7.34492656026756,52.9820669305185));
#221548=CARTESIAN_POINT('Ctrl Pts',(2.96661305715445,-7.33371807551113,
52.9832685793568));
#221549=CARTESIAN_POINT('Ctrl Pts',(2.98247002806966,-7.32728369698994,
52.9839519324171));
#221550=CARTESIAN_POINT('Ctrl Pts',(3.02538151917038,-7.30970886645019,
52.9858011499504));
#221551=CARTESIAN_POINT('Ctrl Pts',(3.05239537216224,-7.29846967185571,
52.9869652357231));
#221552=CARTESIAN_POINT('Ctrl Pts',(3.23295511706357,-7.22216943614654,
52.9947468429668));
#221553=CARTESIAN_POINT('Ctrl Pts',(3.3844757542567,-7.15241611371773,53.0012794331881));
#221554=CARTESIAN_POINT('Ctrl Pts',(4.20685679633496,-6.74183914528896,
53.0368212952316));
#221555=CARTESIAN_POINT('Ctrl Pts',(4.828608559283,-6.31145959244081,53.0635973285695));
#221556=CARTESIAN_POINT('Ctrl Pts',(5.53379228580312,-5.6572925709027,53.0996258844541));
#221557=CARTESIAN_POINT('Ctrl Pts',(5.68166524440177,-5.50876482387663,
53.1075986853947));
#221558=CARTESIAN_POINT('Ctrl Pts',(5.86524467170673,-5.30910882763804,
53.1182653268251));
#221559=CARTESIAN_POINT('Ctrl Pts',(5.90649263824944,-5.26318117431992,
53.1207158651883));
#221560=CARTESIAN_POINT('Ctrl Pts',(5.95550269338952,-5.20730902310365,
53.1236985004562));
#221561=CARTESIAN_POINT('Ctrl Pts',(5.96378453495471,-5.19782200651623,
53.1242049993396));
#221562=CARTESIAN_POINT('Ctrl Pts',(5.9765948052464,-5.18307666256742,53.1249923708119));
#221563=CARTESIAN_POINT('Ctrl Pts',(5.98113904815341,-5.17783206008257,
53.1252724488482));
#221564=CARTESIAN_POINT('Ctrl Pts',(5.98912011610344,-5.16859642214904,
53.1257657188648));
#221565=CARTESIAN_POINT('Ctrl Pts',(5.99255987098294,-5.16460791664533,
53.1259787616843));
#221566=CARTESIAN_POINT('Ctrl Pts',(5.99981288201078,-5.15618081751876,
53.1264289344631));
#221567=CARTESIAN_POINT('Ctrl Pts',(6.0036252002764,-5.15174142367923,53.1266661122774));
#221568=CARTESIAN_POINT('Ctrl Pts',(6.01434757127685,-5.1392273001011,53.1273347746767));
#221569=CARTESIAN_POINT('Ctrl Pts',(6.02124626716762,-5.13114288817535,
53.1277668469999));
#221570=CARTESIAN_POINT('Ctrl Pts',(6.04956908506887,-5.09781630175962,
53.1295484986411));
#221571=CARTESIAN_POINT('Ctrl Pts',(6.07085072683781,-5.07245389992766,
53.1309055785729));
#221572=CARTESIAN_POINT('Ctrl Pts',(6.38457475645071,-4.6937707908609,53.1511959039074));
#221573=CARTESIAN_POINT('Ctrl Pts',(6.64584835604746,-4.31587833869546,
53.1720573887208));
#221574=CARTESIAN_POINT('Ctrl Pts',(7.12990765384459,-3.46665975050171,
53.2170098457722));
#221575=CARTESIAN_POINT('Ctrl Pts',(7.34195941994329,-2.99149422545371,
53.240965374298));
#221576=CARTESIAN_POINT('Ctrl Pts',(7.55886183626264,-2.33999921054791,
53.2707248202692));
#221577=CARTESIAN_POINT('Ctrl Pts',(7.60672215287401,-2.17939697399912,
53.2778374648674));
#221578=CARTESIAN_POINT('Ctrl Pts',(7.67228031744532,-1.93081637273955,
53.2884950348853));
#221579=CARTESIAN_POINT('Ctrl Pts',(7.69364129372632,-1.84386048548167,
53.2921586057735));
#221580=CARTESIAN_POINT('Ctrl Pts',(7.71702306430708,-1.74118483730677,
53.2964097636407));
#221581=CARTESIAN_POINT('Ctrl Pts',(7.72047811409645,-1.72580048277422,
53.2970447750595));
#221582=CARTESIAN_POINT('Ctrl Pts',(7.7256985196037,-1.70222606429507,53.2980148586746));
#221583=CARTESIAN_POINT('Ctrl Pts',(7.72749688798299,-1.69404339866473,
53.2983510242385));
#221584=CARTESIAN_POINT('Ctrl Pts',(7.73060884397527,-1.67977577468526,
53.2989362204085));
#221585=CARTESIAN_POINT('Ctrl Pts',(7.73192825243453,-1.67369210167542,
53.2991854437687));
#221586=CARTESIAN_POINT('Ctrl Pts',(7.73467029510905,-1.66097634965166,
53.2997057256528));
#221587=CARTESIAN_POINT('Ctrl Pts',(7.73609158374099,-1.65434398370694,
53.2999767394061));
#221588=CARTESIAN_POINT('Ctrl Pts',(7.73999427849783,-1.63601726266065,
53.3007246242328));
#221589=CARTESIAN_POINT('Ctrl Pts',(7.7424577142747,-1.62431907556484,53.3012008991494));
#221590=CARTESIAN_POINT('Ctrl Pts',(7.75198752207222,-1.57855034413763,
53.3030599888307));
#221591=CARTESIAN_POINT('Ctrl Pts',(7.75885564729814,-1.54443867346927,
53.30443622465));
#221592=CARTESIAN_POINT('Ctrl Pts',(7.86647901737055,-0.991065962559473,
53.3266130344015));
#221593=CARTESIAN_POINT('Ctrl Pts',(7.91513755553762,-0.463019939003818,
53.3455218999271));
#221594=CARTESIAN_POINT('Ctrl Pts',(7.90691203355497,0.523064402191629,
53.3792121188147));
#221595=CARTESIAN_POINT('Ctrl Pts',(7.86349305738964,0.978932304835636,
53.3941799175719));
#221596=CARTESIAN_POINT('Ctrl Pts',(7.71791560243968,1.7718921920976,53.4221423440559));
#221597=CARTESIAN_POINT('Ctrl Pts',(7.63221175647553,2.11071493466494,53.4347592732188));
#221598=CARTESIAN_POINT('Ctrl Pts',(7.52055111934445,2.45466684629179,53.4492388750309));
#221599=CARTESIAN_POINT('Ctrl Pts',(7.5166480646286,2.46659285937464,53.4497430674054));
#221600=CARTESIAN_POINT('Ctrl Pts',(7.51105909535235,2.48353382458279,53.4504623746172));
#221601=CARTESIAN_POINT('Ctrl Pts',(7.5093964813866,2.48855650464053,53.4506760236377));
#221602=CARTESIAN_POINT('Ctrl Pts',(7.50652629278005,2.49719814411378,53.4510442852934));
#221603=CARTESIAN_POINT('Ctrl Pts',(7.50532113454581,2.50081791068478,53.4511987444298));
#221604=CARTESIAN_POINT('Ctrl Pts',(7.50301578044834,2.50772550703525,53.4514938896054));
#221605=CARTESIAN_POINT('Ctrl Pts',(7.50191604043297,2.51101348911296,53.4516345464708));
#221606=CARTESIAN_POINT('Ctrl Pts',(7.49934122706226,2.51869482819077,53.4519635447833));
#221607=CARTESIAN_POINT('Ctrl Pts',(7.49786446361801,2.52308758516975,53.4521519950838));
#221608=CARTESIAN_POINT('Ctrl Pts',(7.49350833780352,2.53600764921127,53.4527071635878));
#221609=CARTESIAN_POINT('Ctrl Pts',(7.49061829611375,2.54453130184913,53.4530745665352));
#221610=CARTESIAN_POINT('Ctrl Pts',(7.46595341234014,2.61686971717652,53.456202244861));
#221611=CARTESIAN_POINT('Ctrl Pts',(7.44337868640597,2.68040680986584,53.4590129131883));
#221612=CARTESIAN_POINT('Ctrl Pts',(7.26465512515369,3.16375201773333,53.4808340436628));
#221613=CARTESIAN_POINT('Ctrl Pts',(7.07392806428874,3.56987715633135,53.5016737064763));
#221614=CARTESIAN_POINT('Ctrl Pts',(6.64980333807219,4.30395125281107,53.5412757944525));
#221615=CARTESIAN_POINT('Ctrl Pts',(6.42373344697784,4.63460541644503,53.5599647166545));
#221616=CARTESIAN_POINT('Ctrl Pts',(6.0663315835851,5.08064745274554,53.5855550069576));
#221617=CARTESIAN_POINT('Ctrl Pts',(5.95471733042043,5.21101753800589,53.5930930277341));
#221618=CARTESIAN_POINT('Ctrl Pts',(5.70161638419597,5.48788845325515,53.609193272877));
#221619=CARTESIAN_POINT('Ctrl Pts',(5.55853341985669,5.63276700151686,53.6176777546798));
#221620=CARTESIAN_POINT('Ctrl Pts',(5.39560899731263,5.78547442201284,53.6266944099865));
#221621=CARTESIAN_POINT('Ctrl Pts',(5.38115453462074,5.79892116018955,53.627489064347));
#221622=CARTESIAN_POINT('Ctrl Pts',(5.36007088403791,5.81838820463012,53.6286405361458));
#221623=CARTESIAN_POINT('Ctrl Pts',(5.35348163032309,5.82445152921869,53.6289993282473));
#221624=CARTESIAN_POINT('Ctrl Pts',(5.3419351589508,5.83504025780954,53.6296261704756));
#221625=CARTESIAN_POINT('Ctrl Pts',(5.33698245706216,5.83957055835489,53.6298944444511));
#221626=CARTESIAN_POINT('Ctrl Pts',(5.32738150249499,5.84833025920204,53.6304133401011));
#221627=CARTESIAN_POINT('Ctrl Pts',(5.32273396555444,5.85256043334828,53.630663997002));
#221628=CARTESIAN_POINT('Ctrl Pts',(5.31166995101668,5.86260678626034,53.6312594705137));
#221629=CARTESIAN_POINT('Ctrl Pts',(5.30524894690136,5.86841798195408,53.6316040605701));
#221630=CARTESIAN_POINT('Ctrl Pts',(5.282482700742,5.88895419477228,53.6328223336542));
#221631=CARTESIAN_POINT('Ctrl Pts',(5.26608551752779,5.90362162782722,53.6336934097733));
#221632=CARTESIAN_POINT('Ctrl Pts',(5.04870342348825,6.09644562941048,53.6451582399578));
#221633=CARTESIAN_POINT('Ctrl Pts',(4.83882593018278,6.26433042915619,53.6552816843423));
#221634=CARTESIAN_POINT('Ctrl Pts',(4.53439283331565,6.48340459753419,53.6689044957035));
#221635=CARTESIAN_POINT('Ctrl Pts',(4.44673795587198,6.54383495197679,53.6727132047741));
#221636=CARTESIAN_POINT('Ctrl Pts',(3.90006845053592,6.90465773114763,53.6958627326938));
#221637=CARTESIAN_POINT('Ctrl Pts',(3.41209070958504,7.15838194321465,53.7138267259914));
#221638=CARTESIAN_POINT('Ctrl Pts',(2.59289696593736,7.48138121527582,53.7446043561623));
#221639=CARTESIAN_POINT('Ctrl Pts',(2.27665585312476,7.58359902652599,53.7566589582212));
#221640=CARTESIAN_POINT('Ctrl Pts',(1.94288720592805,7.6687199511353,53.7704535844457));
#221641=CARTESIAN_POINT('Ctrl Pts',(1.93080150053543,7.67177176061324,53.7709545358457));
#221642=CARTESIAN_POINT('Ctrl Pts',(1.91345082602626,7.67610945121032,53.7716758177732));
#221643=CARTESIAN_POINT('Ctrl Pts',(1.90819183961635,7.67741846413984,53.7718947123061));
#221644=CARTESIAN_POINT('Ctrl Pts',(1.89906304779282,7.67968075018061,53.7722751501183));
#221645=CARTESIAN_POINT('Ctrl Pts',(1.89519385345344,7.68063650629995,53.7724365434568));
#221646=CARTESIAN_POINT('Ctrl Pts',(1.88775337878041,7.68246846415364,53.7727471830486));
#221647=CARTESIAN_POINT('Ctrl Pts',(1.88418220556449,7.68334510079831,53.7728964032048));
#221648=CARTESIAN_POINT('Ctrl Pts',(1.8757698053407,7.68540392383284,53.773248201615));
#221649=CARTESIAN_POINT('Ctrl Pts',(1.87092807499982,7.68658402497788,53.7734509036962));
#221650=CARTESIAN_POINT('Ctrl Pts',(1.85420175949626,7.69064408049221,53.7741519327338));
#221651=CARTESIAN_POINT('Ctrl Pts',(1.84231166648745,7.69350104036191,53.7746516116642));
#221652=CARTESIAN_POINT('Ctrl Pts',(1.70993435261513,7.72498428189403,53.7802293270365));
#221653=CARTESIAN_POINT('Ctrl Pts',(1.58880311180231,7.75080378720844,53.7854674400192));
#221654=CARTESIAN_POINT('Ctrl Pts',(1.15229894869493,7.83318401914403,53.8047012158067));
#221655=CARTESIAN_POINT('Ctrl Pts',(0.83417617697899,7.87341656915547,53.8193747289654));
#221656=CARTESIAN_POINT('Ctrl Pts',(-0.03065438921563,7.92978268497122,
53.8596186226031));
#221657=CARTESIAN_POINT('Ctrl Pts',(-0.578093233013222,7.9087479508543,
53.8853695287536));
#221658=CARTESIAN_POINT('Ctrl Pts',(-1.33131877502286,7.80112213093109,
53.9191452088183));
#221659=CARTESIAN_POINT('Ctrl Pts',(-1.54231498046819,7.76216399866891,
53.9284390305732));
#221660=CARTESIAN_POINT('Ctrl Pts',(-1.88812614898245,7.68365379446863,
53.9433656909064));
#221661=CARTESIAN_POINT('Ctrl Pts',(-2.02392937984187,7.64900441396915,
53.9491488711969));
#221662=CARTESIAN_POINT('Ctrl Pts',(-2.17625846638252,7.60579722761481,
53.9555524817733));
#221663=CARTESIAN_POINT('Ctrl Pts',(-2.19375432593834,7.6007693257507,53.9562867300508));
#221664=CARTESIAN_POINT('Ctrl Pts',(-2.21998217786313,7.59313394917978,
53.9573855992714));
#221665=CARTESIAN_POINT('Ctrl Pts',(-2.22872721557096,7.5905717202012,53.9577516838276));
#221666=CARTESIAN_POINT('Ctrl Pts',(-2.24374849884163,7.58614240247529,
53.9583799822557));
#221667=CARTESIAN_POINT('Ctrl Pts',(-2.25002687925856,7.58428262392344,
53.9586424324572));
#221668=CARTESIAN_POINT('Ctrl Pts',(-2.26294114735719,7.58043971885191,
53.9591819566745));
#221669=CARTESIAN_POINT('Ctrl Pts',(-2.26957675467967,7.57845566870044,
53.959459000461));
#221670=CARTESIAN_POINT('Ctrl Pts',(-2.28552684237528,7.57366375646814,
53.96012451749));
#221671=CARTESIAN_POINT('Ctrl Pts',(-2.29483877649414,7.57084741848953,
53.960512715921));
#221672=CARTESIAN_POINT('Ctrl Pts',(-2.32333884389236,7.56217033316017,
53.9616997992994));
#221673=CARTESIAN_POINT('Ctrl Pts',(-2.34250996312598,7.55625374186349,
53.9624968751169));
#221674=CARTESIAN_POINT('Ctrl Pts',(-2.55846270306019,7.48870556111712,
53.9714596967271));
#221675=CARTESIAN_POINT('Ctrl Pts',(-2.75279164653053,7.41947355374272,
53.9793737261645));
#221676=CARTESIAN_POINT('Ctrl Pts',(-3.3955273646696,7.16175663551943,54.0052355033074));
#221677=CARTESIAN_POINT('Ctrl Pts',(-3.82922184575607,6.93955709537523,
54.0220953470999));
#221678=CARTESIAN_POINT('Ctrl Pts',(-4.69015958428299,6.39303645141051,
54.0574284590475));
#221679=CARTESIAN_POINT('Ctrl Pts',(-5.11047850810296,6.06230397285203,
54.0758764021775));
#221680=CARTESIAN_POINT('Ctrl Pts',(-5.53067736776218,5.65668494604445,
54.0988492504295));
#221681=CARTESIAN_POINT('Ctrl Pts',(-5.56671212823633,5.62122697116766,
54.1008569842762));
#221682=CARTESIAN_POINT('Ctrl Pts',(-5.61156564497577,5.57623711776027,
54.1034014557561));
#221683=CARTESIAN_POINT('Ctrl Pts',(-5.62070460393262,5.56702516020896,
54.1039222978428));
#221684=CARTESIAN_POINT('Ctrl Pts',(-5.6351921783673,5.55234982403144,54.104751743595));
#221685=CARTESIAN_POINT('Ctrl Pts',(-5.64055563048404,5.54690108389462,
54.1050596406219));
#221686=CARTESIAN_POINT('Ctrl Pts',(-5.65063097395156,5.53663580139107,
54.1056395780295));
#221687=CARTESIAN_POINT('Ctrl Pts',(-5.65534462960088,5.53182099503976,
54.1059115360356));
#221688=CARTESIAN_POINT('Ctrl Pts',(-5.66591169030453,5.52099955259648,
54.1065226389316));
#221689=CARTESIAN_POINT('Ctrl Pts',(-5.67176170214238,5.51498962244065,
54.1068619375626));
#221690=CARTESIAN_POINT('Ctrl Pts',(-5.68659917213833,5.49969797173558,
54.107724996355));
#221691=CARTESIAN_POINT('Ctrl Pts',(-5.69557345448984,5.49040353228363,
54.1082493384872));
#221692=CARTESIAN_POINT('Ctrl Pts',(-5.74511552548725,5.43884186790284,
54.1111567085762));
#221693=CARTESIAN_POINT('Ctrl Pts',(-5.78523512131532,5.3961474850898,54.1135586569343));
#221694=CARTESIAN_POINT('Ctrl Pts',(-5.84706139113431,5.32887127290308,
54.1173310314572));
#221695=CARTESIAN_POINT('Ctrl Pts',(-5.86909609507175,5.30459300556864,
54.1186898985648));
#221696=CARTESIAN_POINT('Ctrl Pts',(-5.9600096526759,5.2031627499176,54.1243548977835));
#221697=CARTESIAN_POINT('Ctrl Pts',(-6.02752226395053,5.12480168981251,
54.1287024776697));
#221698=CARTESIAN_POINT('Ctrl Pts',(-6.29579401683741,4.80078536201363,
54.1465123012092));
#221699=CARTESIAN_POINT('Ctrl Pts',(-6.48322654416945,4.54448375102178,
54.1602053430769));
#221700=CARTESIAN_POINT('Ctrl Pts',(-6.9690666613559,3.78865538307987,54.1988431745692));
#221701=CARTESIAN_POINT('Ctrl Pts',(-7.2285361651983,3.26651468749628,54.2234085490936));
#221702=CARTESIAN_POINT('Ctrl Pts',(-7.5029764598599,2.51718457331221,54.2563829748878));
#221703=CARTESIAN_POINT('Ctrl Pts',(-7.56910680964462,2.31073542341048,
54.2652904526933));
#221704=CARTESIAN_POINT('Ctrl Pts',(-7.65831524081857,1.98703496228163,
54.2790002288049));
#221705=CARTESIAN_POINT('Ctrl Pts',(-7.68735643862039,1.87153726676206,
54.2838396326363));
#221706=CARTESIAN_POINT('Ctrl Pts',(-7.72150907181092,1.72146217345042,
54.2900595690303));
#221707=CARTESIAN_POINT('Ctrl Pts',(-7.72901408993107,1.68744646487597,
54.2914648921472));
#221708=CARTESIAN_POINT('Ctrl Pts',(-7.74085679063939,1.63203361669875,
54.2937470005079));
#221709=CARTESIAN_POINT('Ctrl Pts',(-7.74533097960332,1.61066619726802,
54.2946252516648));
#221710=CARTESIAN_POINT('Ctrl Pts',(-7.75377484409917,1.56949186855227,
54.2963142929539));
#221711=CARTESIAN_POINT('Ctrl Pts',(-7.75775721264313,1.54968773978843,
54.2971252168167));
#221712=CARTESIAN_POINT('Ctrl Pts',(-7.76672275293462,1.50420179989738,
54.2989843862186));
#221713=CARTESIAN_POINT('Ctrl Pts',(-7.77165448062265,1.47851006610452,
54.3000320485255));
#221714=CARTESIAN_POINT('Ctrl Pts',(-7.78447213923758,1.40990021978572,
54.3028234018497));
#221715=CARTESIAN_POINT('Ctrl Pts',(-7.79213058136303,1.36694043295633,
54.3045644926613));
#221716=CARTESIAN_POINT('Ctrl Pts',(-7.87393163691742,0.885036544939357,
54.3240226939874));
#221717=CARTESIAN_POINT('Ctrl Pts',(-7.91125398658139,0.440643456825135,
54.3412395963992));
#221718=CARTESIAN_POINT('Ctrl Pts',(-7.91086706386801,-0.234087545961717,
54.3671770834644));
#221719=CARTESIAN_POINT('Ctrl Pts',(-7.90074428252544,-0.46352253225071,
54.3759721012671));
#221720=CARTESIAN_POINT('Ctrl Pts',(-7.86129618668486,-0.912643246804813,
54.3934206776831));
#221721=CARTESIAN_POINT('Ctrl Pts',(-7.83269150091399,-1.13218111851608,
54.402060868805));
#221722=CARTESIAN_POINT('Ctrl Pts',(-7.79071161378515,-1.37453345827551,
54.4118989447882));
#221723=CARTESIAN_POINT('Ctrl Pts',(-7.78638710016935,-1.39882293362783,
54.4128883681082));
#221724=CARTESIAN_POINT('Ctrl Pts',(-7.77972307662556,-1.43526407699927,
54.414378221559));
#221725=CARTESIAN_POINT('Ctrl Pts',(-7.77746856669707,-1.44743110799853,
54.4148765561077));
#221726=CARTESIAN_POINT('Ctrl Pts',(-7.77331959517379,-1.46953249404212,
54.4157833824846));
#221727=CARTESIAN_POINT('Ctrl Pts',(-7.77143461063091,-1.47946861127073,
54.4161916536715));
#221728=CARTESIAN_POINT('Ctrl Pts',(-7.7673324638568,-1.5008676524494,54.4170721809818));
#221729=CARTESIAN_POINT('Ctrl Pts',(-7.7651089690174,-1.51232933333855,
54.4175445789451));
#221730=CARTESIAN_POINT('Ctrl Pts',(-7.75894019326233,-1.54375588693335,
54.418841917555));
#221731=CARTESIAN_POINT('Ctrl Pts',(-7.75494324185829,-1.5637104819137,
54.4196679801569));
#221732=CARTESIAN_POINT('Ctrl Pts',(-7.7332242437255,-1.67000997002164,
54.4240803529691));
#221733=CARTESIAN_POINT('Ctrl Pts',(-7.71413721812039,-1.75606865396703,
54.4276943446451));
#221734=CARTESIAN_POINT('Ctrl Pts',(-7.6516523701087,-2.0170835511992,54.4387650364541));
#221735=CARTESIAN_POINT('Ctrl Pts',(-7.6037101729826,-2.19089021926288,
54.4462870303886));
#221736=CARTESIAN_POINT('Ctrl Pts',(-7.41194139651707,-2.8036233699511,
54.4731937489262));
#221737=CARTESIAN_POINT('Ctrl Pts',(-7.23567939862982,-3.23143001827603,
54.4926573018446));
#221738=CARTESIAN_POINT('Ctrl Pts',(-7.00125805147646,-3.68355257673471,
54.5136840094165));
#221739=CARTESIAN_POINT('Ctrl Pts',(-6.97903134270909,-3.72549264374597,
54.5156396413139));
#221740=CARTESIAN_POINT('Ctrl Pts',(-6.88085214365688,-3.90678673052697,
54.5241160556178));
#221741=CARTESIAN_POINT('Ctrl Pts',(-6.80109250648502,-4.04403891838817,
54.5305915993251));
#221742=CARTESIAN_POINT('Ctrl Pts',(-6.69338959760291,-4.21716710002389,
54.538847930818));
#221743=CARTESIAN_POINT('Ctrl Pts',(-6.66919350359408,-4.25532850618024,
54.540673536942));
#221744=CARTESIAN_POINT('Ctrl Pts',(-6.62999295380238,-4.31599884320318,
54.5435857055036));
#221745=CARTESIAN_POINT('Ctrl Pts',(-6.6151977487487,-4.33864164607268,
54.5446747572055));
#221746=CARTESIAN_POINT('Ctrl Pts',(-6.5882515373331,-4.37942225393369,
54.5466403262516));
#221747=CARTESIAN_POINT('Ctrl Pts',(-6.57614103070698,-4.39758646814392,
54.5475173149181));
#221748=CARTESIAN_POINT('Ctrl Pts',(-6.54734012708687,-4.44039912161655,
54.549588023646));
#221749=CARTESIAN_POINT('Ctrl Pts',(-6.53058547562071,-4.46500397002371,
54.5507809712487));
#221750=CARTESIAN_POINT('Ctrl Pts',(-6.48062742095259,-4.53748651870606,
54.5543042049303));
#221751=CARTESIAN_POINT('Ctrl Pts',(-6.44703343617735,-4.58509275844188,
54.5566299084139));
#221752=CARTESIAN_POINT('Ctrl Pts',(-6.21838340084642,-4.90163228966447,
54.572179911753));
#221753=CARTESIAN_POINT('Ctrl Pts',(-6.00707170675512,-5.15842908038931,
54.5852613213391));
#221754=CARTESIAN_POINT('Ctrl Pts',(-5.60904732433313,-5.58438728797675,
54.6078867167073));
#221755=CARTESIAN_POINT('Ctrl Pts',(-5.42923799794173,-5.7593552614092,
54.6174778847388));
#221756=CARTESIAN_POINT('Ctrl Pts',(-4.73596972671233,-6.37258868107269,
54.6524278010461));
#221757=CARTESIAN_POINT('Ctrl Pts',(-4.17544233568427,-6.75313522176013,
54.6765714295174));
#221758=CARTESIAN_POINT('Ctrl Pts',(-3.49568977349531,-7.09730080246153,
54.7062397503744));
#221759=CARTESIAN_POINT('Ctrl Pts',(-3.41724431650202,-7.1354023243537,
54.709674515105));
#221760=CARTESIAN_POINT('Ctrl Pts',(-3.32569721832532,-7.17801147898649,
54.7137110346409));
#221761=CARTESIAN_POINT('Ctrl Pts',(-3.31319255663347,-7.18379188592281,
54.7142629960643));
#221762=CARTESIAN_POINT('Ctrl Pts',(-3.29329178320488,-7.19292820723781,
54.7151424686008));
#221763=CARTESIAN_POINT('Ctrl Pts',(-3.28590546146572,-7.196305459158,54.7154691193393));
#221764=CARTESIAN_POINT('Ctrl Pts',(-3.27289843750078,-7.20222846700842,
54.7160447591127));
#221765=CARTESIAN_POINT('Ctrl Pts',(-3.26727992608159,-7.20477903599653,
54.7162935502082));
#221766=CARTESIAN_POINT('Ctrl Pts',(-3.25569369712998,-7.21002235884941,
54.7168068896717));
#221767=CARTESIAN_POINT('Ctrl Pts',(-3.24972561061869,-7.21271428243209,
54.7170714723439));
#221768=CARTESIAN_POINT('Ctrl Pts',(-3.2345118760153,-7.21955376795084,
54.7177463657334));
#221769=CARTESIAN_POINT('Ctrl Pts',(-3.22526160448074,-7.22369097247584,
54.7181571137681));
#221770=CARTESIAN_POINT('Ctrl Pts',(-3.18803904983219,-7.24025309259574,
54.7198116304288));
#221771=CARTESIAN_POINT('Ctrl Pts',(-3.16000295443897,-7.25253328979102,
54.721061647384));
#221772=CARTESIAN_POINT('Ctrl Pts',(-2.98589340877544,-7.32759445087228,
54.7288520001625));
#221773=CARTESIAN_POINT('Ctrl Pts',(-2.8380462943876,-7.3861141699198,54.7356076042871));
#221774=CARTESIAN_POINT('Ctrl Pts',(-2.58992900809067,-7.47577315816816,
54.74710723741));
#221775=CARTESIAN_POINT('Ctrl Pts',(-2.4906141491953,-7.50944449366486,
54.7517494897539));
#221776=CARTESIAN_POINT('Ctrl Pts',(-1.43726275669575,-7.84337414811336,
54.8012165261127));
#221777=CARTESIAN_POINT('Ctrl Pts',(-0.434792823876008,-7.96216655253596,
54.8489632567107));
#221778=CARTESIAN_POINT('Ctrl Pts',(0.616449503353414,-7.88712575600834,
54.8921867569514));
#221779=CARTESIAN_POINT('Ctrl Pts',(0.669582528429679,-7.88279278289727,
54.8943569718477));
#221780=CARTESIAN_POINT('Ctrl Pts',(0.737297255389228,-7.87658108334241,
54.8971047884567));
#221781=CARTESIAN_POINT('Ctrl Pts',(0.751922427519911,-7.87519837662244,
54.8976971969171));
#221782=CARTESIAN_POINT('Ctrl Pts',(0.775153156405917,-7.87293677157096,
54.8986364956258));
#221783=CARTESIAN_POINT('Ctrl Pts',(0.783761236428558,-7.87208448569377,
54.8989841818111));
#221784=CARTESIAN_POINT('Ctrl Pts',(0.799813335686963,-7.87046857715947,
54.8996318538304));
#221785=CARTESIAN_POINT('Ctrl Pts',(0.807257698493105,-7.86970850823591,
54.8999319457178));
#221786=CARTESIAN_POINT('Ctrl Pts',(0.823786502598141,-7.8679972184551,
54.9005976373648));
#221787=CARTESIAN_POINT('Ctrl Pts',(0.832870403531804,-7.86704082378435,
54.9009630816766));
#221788=CARTESIAN_POINT('Ctrl Pts',(0.85915886929496,-7.86422701117024,
54.9020194943953));
#221789=CARTESIAN_POINT('Ctrl Pts',(0.876359068959876,-7.86232886826909,
54.9027092411659));
#221790=CARTESIAN_POINT('Ctrl Pts',(0.994221373760253,-7.84893049708849,
54.9074258349511));
#221791=CARTESIAN_POINT('Ctrl Pts',(1.09466266891507,-7.83555362637779,
54.9113960245377));
#221792=CARTESIAN_POINT('Ctrl Pts',(1.37897901975434,-7.7921141856775,54.9225084722948));
#221793=CARTESIAN_POINT('Ctrl Pts',(1.56209040980258,-7.75748058331131,
54.9295137451526));
#221794=CARTESIAN_POINT('Ctrl Pts',(2.25792280637528,-7.60023094988118,
54.955736439059));
#221795=CARTESIAN_POINT('Ctrl Pts',(2.75914757479126,-7.43295687460698,
54.9737008228036));
#221796=CARTESIAN_POINT('Ctrl Pts',(3.68135926837173,-7.01894369588516,
55.0087212779305));
#221797=CARTESIAN_POINT('Ctrl Pts',(4.10356977213113,-6.78075220247433,
55.0257052435565));
#221798=CARTESIAN_POINT('Ctrl Pts',(4.52604174807477,-6.48843354093584,
55.0460505242683));
#221799=CARTESIAN_POINT('Ctrl Pts',(4.55065131485444,-6.47119743852568,
55.0472486735376));
#221800=CARTESIAN_POINT('Ctrl Pts',(4.58285692998871,-6.44836664068558,
55.0488331527018));
#221801=CARTESIAN_POINT('Ctrl Pts',(4.59054226993995,-6.44289776732519,
55.0492125058542));
#221802=CARTESIAN_POINT('Ctrl Pts',(4.6024042942724,-6.43442477471288,55.0497999230572));
#221803=CARTESIAN_POINT('Ctrl Pts',(4.60658787749039,-6.43143029163432,
55.0500074638262));
#221804=CARTESIAN_POINT('Ctrl Pts',(4.61484158300029,-6.42551035234188,
55.0504176355482));
#221805=CARTESIAN_POINT('Ctrl Pts',(4.61891185250142,-6.42258510437476,
55.0506202553047));
#221806=CARTESIAN_POINT('Ctrl Pts',(4.62789955109062,-6.4161128035415,55.0510684264516));
#221807=CARTESIAN_POINT('Ctrl Pts',(4.63281568345979,-6.41256396502293,
55.0513140725527));
#221808=CARTESIAN_POINT('Ctrl Pts',(4.64302421396867,-6.40517680402366,
55.0518252045324));
#221809=CARTESIAN_POINT('Ctrl Pts',(4.64831594371214,-6.40133756564769,
55.0520907383148));
#221810=CARTESIAN_POINT('Ctrl Pts',(4.66189686041151,-6.39145866381124,
55.0527736978922));
#221811=CARTESIAN_POINT('Ctrl Pts',(4.67017905681166,-6.38540944374524,
55.0531916161231));
#221812=CARTESIAN_POINT('Ctrl Pts',(4.69421276456808,-6.36778373115723,
55.0544084345532));
#221813=CARTESIAN_POINT('Ctrl Pts',(4.70993309386602,-6.35616498904592,
55.0552094590927));
#221814=CARTESIAN_POINT('Ctrl Pts',(5.29193362977246,-5.92266940393472,
55.0850504672423));
#221815=CARTESIAN_POINT('Ctrl Pts',(5.79923763835632,-5.42692318221993,
55.1172000364732));
#221816=CARTESIAN_POINT('Ctrl Pts',(6.48358919502754,-4.55096972711259,
55.1652773749016));
#221817=CARTESIAN_POINT('Ctrl Pts',(6.70825066077856,-4.21279796056472,
55.1822983748031));
#221818=CARTESIAN_POINT('Ctrl Pts',(6.92425700366949,-3.82622330959298,
55.2002345752718));
#221819=CARTESIAN_POINT('Ctrl Pts',(6.9422692131843,-3.79344409058826,55.2017445629007));
#221820=CARTESIAN_POINT('Ctrl Pts',(6.96747478046474,-3.7467933298125,55.2038786024422));
#221821=CARTESIAN_POINT('Ctrl Pts',(6.97486046265915,-3.73302646671918,
55.2045065359381));
#221822=CARTESIAN_POINT('Ctrl Pts',(6.98832055818766,-3.70775753901179,
55.2056557949338));
#221823=CARTESIAN_POINT('Ctrl Pts',(6.99440747229689,-3.69626220724765,
55.2061773668574));
#221824=CARTESIAN_POINT('Ctrl Pts',(7.00667617124315,-3.67295355242057,
55.2072324440797));
#221825=CARTESIAN_POINT('Ctrl Pts',(7.01285649846355,-3.66113950841705,
55.2077659196643));
#221826=CARTESIAN_POINT('Ctrl Pts',(7.02799754695141,-3.63201752973426,
55.2090778166863));
#221827=CARTESIAN_POINT('Ctrl Pts',(7.0369242413197,-3.61469197607792,55.2098555851904));
#221828=CARTESIAN_POINT('Ctrl Pts',(7.06887103757555,-3.55212054298723,
55.2126549217877));
#221829=CARTESIAN_POINT('Ctrl Pts',(7.09151973038163,-3.50668591169718,
55.2146697092169));
#221830=CARTESIAN_POINT('Ctrl Pts',(7.21192339744033,-3.25921114755375,
55.2255497534726));
#221831=CARTESIAN_POINT('Ctrl Pts',(7.30148584487766,-3.05329431063649,
55.2342598561714));
#221832=CARTESIAN_POINT('Ctrl Pts',(7.4949716180313,-2.55103523509234,55.254802660372));
#221833=CARTESIAN_POINT('Ctrl Pts',(7.59025087707266,-2.25177272638997,
55.2664734339752));
#221834=CARTESIAN_POINT('Ctrl Pts',(7.80112650043722,-1.42159167739227,
55.2980519045625));
#221835=CARTESIAN_POINT('Ctrl Pts',(7.88024951926195,-0.883227583544129,
55.3176140994103));
#221836=CARTESIAN_POINT('Ctrl Pts',(7.90703841821882,-0.262412077518545,
55.3419046805517));
#221837=CARTESIAN_POINT('Ctrl Pts',(7.90925787588008,-0.183728086002174,
55.345016780243));
#221838=CARTESIAN_POINT('Ctrl Pts',(7.91047595157171,-0.0919853300617438,
55.3486948175989));
#221839=CARTESIAN_POINT('Ctrl Pts',(7.91061684255294,-0.0789445954374625,
55.3492187952998));
#221840=CARTESIAN_POINT('Ctrl Pts',(7.91079014638393,-0.058142111105068,
55.3500565647246));
#221841=CARTESIAN_POINT('Ctrl Pts',(7.91084338405457,-0.0503805282363616,
55.3503695708268));
#221842=CARTESIAN_POINT('Ctrl Pts',(7.91091652925125,-0.0368033760274333,
55.3509178676722));
#221843=CARTESIAN_POINT('Ctrl Pts',(7.91094144683786,-0.0309878320969655,
55.3511529661507));
#221844=CARTESIAN_POINT('Ctrl Pts',(7.91097961879299,-0.0189914274697496,
55.351638443931));
#221845=CARTESIAN_POINT('Ctrl Pts',(7.91099204223478,-0.0128105694601785,
55.3518888553203));
#221846=CARTESIAN_POINT('Ctrl Pts',(7.91100512741119,0.0028034951340082,
55.3525221640952));
#221847=CARTESIAN_POINT('Ctrl Pts',(7.91099616028461,0.0122366844166195,
55.3529054397927));
#221848=CARTESIAN_POINT('Ctrl Pts',(7.91094053542195,0.0325435852834091,
55.3537319842501));
#221849=CARTESIAN_POINT('Ctrl Pts',(7.91088833067868,0.0434172528264745,
55.3541754747805));
#221850=CARTESIAN_POINT('Ctrl Pts',(7.91067702513212,0.0742070115765184,
55.3554338852622));
#221851=CARTESIAN_POINT('Ctrl Pts',(7.91046513226251,0.0941225662792637,
55.3562509684261));
#221852=CARTESIAN_POINT('Ctrl Pts',(7.90790191464639,0.27192022472201,55.3635746764319));
#221853=CARTESIAN_POINT('Ctrl Pts',(7.90090009270303,0.429675636351487,
55.370299442748));
#221854=CARTESIAN_POINT('Ctrl Pts',(7.88141634415975,0.691485561427953,
55.381777868643));
#221855=CARTESIAN_POINT('Ctrl Pts',(7.87157821093175,0.795695425339125,
55.3864265097527));
#221856=CARTESIAN_POINT('Ctrl Pts',(7.75383859127071,1.82428202577128,55.4329098480358));
#221857=CARTESIAN_POINT('Ctrl Pts',(7.485607250148,2.72332626818989,55.477213874366));
#221858=CARTESIAN_POINT('Ctrl Pts',(7.04436380502909,3.60047786289725,55.5174219828695));
#221859=CARTESIAN_POINT('Ctrl Pts',(7.02109529922987,3.64564441326285,55.5194868007979));
#221860=CARTESIAN_POINT('Ctrl Pts',(6.99099690496271,3.70271133776944,55.5220887725884));
#221861=CARTESIAN_POINT('Ctrl Pts',(6.98456927220815,3.71482180734349,55.5226405548882));
#221862=CARTESIAN_POINT('Ctrl Pts',(6.97433644049507,3.73398130428023,55.5235128891819));
#221863=CARTESIAN_POINT('Ctrl Pts',(6.97055197703984,3.74104133922951,55.5238341999685));
#221864=CARTESIAN_POINT('Ctrl Pts',(6.96349182650797,3.75416436396925,55.5244311985998));
#221865=CARTESIAN_POINT('Ctrl Pts',(6.96021892973312,3.76022884144655,55.5247069885492));
#221866=CARTESIAN_POINT('Ctrl Pts',(6.95295629677151,3.77364408584432,55.525316848845));
#221867=CARTESIAN_POINT('Ctrl Pts',(6.94896281667145,3.78099282259753,55.5256507808675));
#221868=CARTESIAN_POINT('Ctrl Pts',(6.93743911383342,3.80211862687295,55.5266103448307));
#221869=CARTESIAN_POINT('Ctrl Pts',(6.92987950091776,3.8158796649663,55.5272348902411));
#221870=CARTESIAN_POINT('Ctrl Pts',(6.87961244810827,3.90674056717534,55.5313553786714));
#221871=CARTESIAN_POINT('Ctrl Pts',(6.83565926072647,3.98314604550887,55.5348047653676));
#221872=CARTESIAN_POINT('Ctrl Pts',(6.70753364389809,4.19750211085642,55.5444454890998));
#221873=CARTESIAN_POINT('Ctrl Pts',(6.62039734600867,4.33363290545073,55.5505234029967));
#221874=CARTESIAN_POINT('Ctrl Pts',(6.44756714864027,4.58624831506854,55.5617693887955));
#221875=CARTESIAN_POINT('Ctrl Pts',(6.36273176013428,4.70323743725388,55.5669636651061));
#221876=CARTESIAN_POINT('Ctrl Pts',(6.21989164740532,4.88927186892742,55.57524845031));
#221877=CARTESIAN_POINT('Ctrl Pts',(6.1638292366516,4.95976219725351,55.5783939022713));
#221878=CARTESIAN_POINT('Ctrl Pts',(6.06118459520204,5.08439377004502,55.583982441492));
#221879=CARTESIAN_POINT('Ctrl Pts',(6.01505006641264,5.13889010961267,55.5864357677979));
#221880=CARTESIAN_POINT('Ctrl Pts',(5.65044116183605,5.55794569938099,55.6054155013654));
#221881=CARTESIAN_POINT('Ctrl Pts',(5.29986617697838,5.89318520828578,55.6212173823318));
#221882=CARTESIAN_POINT('Ctrl Pts',(4.84985227492496,6.25068634738431,55.641288792889));
#221883=CARTESIAN_POINT('Ctrl Pts',(4.77787352705255,6.30587589948935,55.6444955047424));
#221884=CARTESIAN_POINT('Ctrl Pts',(4.69398335766373,6.36793748210256,55.6482471553391));
#221885=CARTESIAN_POINT('Ctrl Pts',(4.68298251854409,6.37603185896641,55.6487394023981));
#221886=CARTESIAN_POINT('Ctrl Pts',(4.49712898061499,6.51204175245371,55.6570612951302));
#221887=CARTESIAN_POINT('Ctrl Pts',(4.31712767229245,6.63274089344022,55.6652044103897));
#221888=CARTESIAN_POINT('Ctrl Pts',(4.12078984027477,6.75301399004028,55.6744139692693));
#221889=CARTESIAN_POINT('Ctrl Pts',(4.1091463895922,6.76010523599476,55.6749613153992));
#221890=CARTESIAN_POINT('Ctrl Pts',(4.09314504405239,6.76979396923635,55.6757152303537));
#221891=CARTESIAN_POINT('Ctrl Pts',(4.08880283291325,6.77241745102042,55.6759199889666));
#221892=CARTESIAN_POINT('Ctrl Pts',(4.08138761075529,6.77688785692618,55.6762699553073));
#221893=CARTESIAN_POINT('Ctrl Pts',(4.07831585748665,6.77873687504273,55.6764150161143));
#221894=CARTESIAN_POINT('Ctrl Pts',(4.07235573382361,6.78231900780226,55.6766966490261));
#221895=CARTESIAN_POINT('Ctrl Pts',(4.06946751122572,6.78405236723615,55.6768332037838));
#221896=CARTESIAN_POINT('Ctrl Pts',(4.06350569662145,6.78762515789051,55.6771152401273));
#221897=CARTESIAN_POINT('Ctrl Pts',(4.06043195786432,6.78946434897916,55.6772607389915));
#221898=CARTESIAN_POINT('Ctrl Pts',(4.05081979674586,6.79520698449249,55.6777160227102));
#221899=CARTESIAN_POINT('Ctrl Pts',(4.04427701171192,6.79910306139824,55.6780263298881));
#221900=CARTESIAN_POINT('Ctrl Pts',(4.007496446712,6.82093316076346,55.6797729606704));
#221901=CARTESIAN_POINT('Ctrl Pts',(3.97714546095821,6.83867464189511,55.681222699086));
#221902=CARTESIAN_POINT('Ctrl Pts',(3.88928541947689,6.88924997713737,55.6854410384317));
#221903=CARTESIAN_POINT('Ctrl Pts',(3.83148209662901,6.92156418626674,55.6882428045681));
#221904=CARTESIAN_POINT('Ctrl Pts',(3.61021145596674,7.04164165693944,55.6990455965559));
#221905=CARTESIAN_POINT('Ctrl Pts',(3.44408715668642,7.12436663781493,55.7073142573033));
#221906=CARTESIAN_POINT('Ctrl Pts',(3.0852830946315,7.28755702932442,55.725245810854));
#221907=CARTESIAN_POINT('Ctrl Pts',(2.89200826596929,7.36639281472405,55.734946317405));
#221908=CARTESIAN_POINT('Ctrl Pts',(2.433950147589,7.5324239312153,55.7576900166131));
#221909=CARTESIAN_POINT('Ctrl Pts',(2.167213369983,7.61345630018782,55.770743645551));
#221910=CARTESIAN_POINT('Ctrl Pts',(1.41041541625579,7.80035901900882,55.8065585580959));
#221911=CARTESIAN_POINT('Ctrl Pts',(0.913718627602875,7.87401551902733,
55.8285887029286));
#221912=CARTESIAN_POINT('Ctrl Pts',(0.380234885885243,7.90192636349685,
55.8502898363374));
#221913=CARTESIAN_POINT('Ctrl Pts',(0.347135910286013,7.90344959621687,
55.8516287716143));
#221914=CARTESIAN_POINT('Ctrl Pts',(0.302608450095644,7.90521851304922,
55.8534201137061));
#221915=CARTESIAN_POINT('Ctrl Pts',(0.291187844994659,7.90564742785708,
55.8538786896639));
#221916=CARTESIAN_POINT('Ctrl Pts',(0.273274757894683,7.90628130664492,
55.8545965954802));
#221917=CARTESIAN_POINT('Ctrl Pts',(0.266782907955704,7.90650302430878,
55.854856489271));
#221918=CARTESIAN_POINT('Ctrl Pts',(0.254325869587166,7.90691311263696,
55.8553546549386));
#221919=CARTESIAN_POINT('Ctrl Pts',(0.248360728385151,7.90710272903696,
55.8555929685846));
#221920=CARTESIAN_POINT('Ctrl Pts',(0.234357082804797,7.90753200641666,
55.8561518755499));
#221921=CARTESIAN_POINT('Ctrl Pts',(0.226318408897982,7.90776616074927,
55.8564722833496));
#221922=CARTESIAN_POINT('Ctrl Pts',(0.203117438986491,7.90840656298365,
55.857395804963));
#221923=CARTESIAN_POINT('Ctrl Pts',(0.187954273129431,7.90878146456195,
55.8579978640955));
#221924=CARTESIAN_POINT('Ctrl Pts',(0.0859150395957425,7.91101071154047,
55.8620392710231));
#221925=CARTESIAN_POINT('Ctrl Pts',(-0.000987040249993028,7.91147720328216,
55.8654317933009));
#221926=CARTESIAN_POINT('Ctrl Pts',(-0.219174209855252,7.90905327265437,
55.8738342414234));
#221927=CARTESIAN_POINT('Ctrl Pts',(-0.350413887905194,7.90432622629885,
55.8787832286093));
#221928=CARTESIAN_POINT('Ctrl Pts',(-0.715355012722817,7.88207393163809,
55.8923005511797));
#221929=CARTESIAN_POINT('Ctrl Pts',(-0.948488714424283,7.85742956072827,
55.9006523087725));
#221930=CARTESIAN_POINT('Ctrl Pts',(-1.24601193570906,7.81254157969881,
55.9111367234525));
#221931=CARTESIAN_POINT('Ctrl Pts',(-1.31170287182357,7.80178103866956,
55.9134409910735));
#221932=CARTESIAN_POINT('Ctrl Pts',(-1.43117515333971,7.78065918940041,
55.917620260368));
#221933=CARTESIAN_POINT('Ctrl Pts',(-1.48499944668865,7.77056603047045,
55.919498817032));
#221934=CARTESIAN_POINT('Ctrl Pts',(-1.58405744677661,7.7509238027929,55.9229529984494));
#221935=CARTESIAN_POINT('Ctrl Pts',(-1.62932049762711,7.74153554068138,
55.9245301347176));
#221936=CARTESIAN_POINT('Ctrl Pts',(-1.71325995073063,7.7233564103393,55.9274557488279));
#221937=CARTESIAN_POINT('Ctrl Pts',(-1.75195750340065,7.71467036324937,
55.928804845002));
#221938=CARTESIAN_POINT('Ctrl Pts',(-1.8241025079016,7.69790587777259,55.9313226805811));
#221939=CARTESIAN_POINT('Ctrl Pts',(-1.85756571872462,7.68989950940108,
55.9324916157818));
#221940=CARTESIAN_POINT('Ctrl Pts',(-2.1596775417065,7.61552951954678,55.9430614639445));
#221941=CARTESIAN_POINT('Ctrl Pts',(-2.42471646702756,7.53533268053587,
55.9524452512352));
#221942=CARTESIAN_POINT('Ctrl Pts',(-2.95607903622881,7.34360731760556,
55.9723801599168));
#221943=CARTESIAN_POINT('Ctrl Pts',(-3.22158867360532,7.23106554033772,
55.9829510820967));
#221944=CARTESIAN_POINT('Ctrl Pts',(-3.49606027988588,7.09660410990899,
55.9951418009379));
#221945=CARTESIAN_POINT('Ctrl Pts',(-3.51175327603105,7.08885155030967,
55.995843337483));
#221946=CARTESIAN_POINT('Ctrl Pts',(-3.53313260041945,7.07820144900475,
55.9968054142405));
#221947=CARTESIAN_POINT('Ctrl Pts',(-3.53884123849446,7.07534906651966,
55.9970629196426));
#221948=CARTESIAN_POINT('Ctrl Pts',(-3.54790973421809,7.07080417428842,
55.997472951894));
#221949=CARTESIAN_POINT('Ctrl Pts',(-3.55127185748557,7.06911616451666,
55.9976251826567));
#221950=CARTESIAN_POINT('Ctrl Pts',(-3.55779838601845,7.0658335814399,55.9979211023692));
#221951=CARTESIAN_POINT('Ctrl Pts',(-3.56096292715563,7.06423927875445,
55.9980647736179));
#221952=CARTESIAN_POINT('Ctrl Pts',(-3.56750351977011,7.06093860233166,
55.9983621050999));
#221953=CARTESIAN_POINT('Ctrl Pts',(-3.57087942036125,7.0592319323435,55.998515784577));
#221954=CARTESIAN_POINT('Ctrl Pts',(-3.57853197278513,7.05535632791345,
55.9988646290135));
#221955=CARTESIAN_POINT('Ctrl Pts',(-3.58280787566428,7.0531859269385,55.999059888622));
#221956=CARTESIAN_POINT('Ctrl Pts',(-3.603381548481,7.04271942214215,56.0000010204206));
#221957=CARTESIAN_POINT('Ctrl Pts',(-3.61965237131838,7.0343707709444,56.0007502558238));
#221958=CARTESIAN_POINT('Ctrl Pts',(-3.66031519777789,7.01332800916777,
56.0026347901358));
#221959=CARTESIAN_POINT('Ctrl Pts',(-3.68467008840576,7.00056307849199,
56.0037744742592));
#221960=CARTESIAN_POINT('Ctrl Pts',(-3.78099729385834,6.94943395466464,
56.0083241469871));
#221961=CARTESIAN_POINT('Ctrl Pts',(-3.85243910919269,6.91008573813601,
56.011791970731));
#221962=CARTESIAN_POINT('Ctrl Pts',(-4.13745763107289,6.74731143776999,
56.0259677778496));
#221963=CARTESIAN_POINT('Ctrl Pts',(-4.34580693950223,6.61503701137007,
56.0371090797736));
#221964=CARTESIAN_POINT('Ctrl Pts',(-5.30920869592848,5.93822335211284,
56.0912800273718));
#221965=CARTESIAN_POINT('Ctrl Pts',(-5.97066924491027,5.27277118452364,
56.1355515754416));
#221966=CARTESIAN_POINT('Ctrl Pts',(-6.5341371864934,4.46007924211345,56.176158837364));
#221967=CARTESIAN_POINT('Ctrl Pts',(-6.56651967412693,4.41226417757633,
56.1785102187326));
#221968=CARTESIAN_POINT('Ctrl Pts',(-6.6065287644229,4.35177171854595,56.1814386607794));
#221969=CARTESIAN_POINT('Ctrl Pts',(-6.61464681290655,4.33942242113643,
56.1820340913721));
#221970=CARTESIAN_POINT('Ctrl Pts',(-6.62736485325176,4.31995693252685,
56.1829688848917));
#221971=CARTESIAN_POINT('Ctrl Pts',(-6.63198807868977,4.31285600521238,
56.1833091116291));
#221972=CARTESIAN_POINT('Ctrl Pts',(-6.64012398252134,4.3003158512327,56.183908574154));
#221973=CARTESIAN_POINT('Ctrl Pts',(-6.6436414044089,4.29487972049184,56.1841679856497));
#221974=CARTESIAN_POINT('Ctrl Pts',(-6.65166890616065,4.28243986012553,
56.1847605788891));
#221975=CARTESIAN_POINT('Ctrl Pts',(-6.65617460908818,4.27543330747374,
56.1850935986572));
#221976=CARTESIAN_POINT('Ctrl Pts',(-6.66851293711726,4.2561799235453,56.1860066602377));
#221977=CARTESIAN_POINT('Ctrl Pts',(-6.67632290228966,4.24391857147661,
56.1865858668019));
#221978=CARTESIAN_POINT('Ctrl Pts',(-6.7171592949207,4.17941526557387,56.1896210763298));
#221979=CARTESIAN_POINT('Ctrl Pts',(-6.74960687384587,4.12680847860903,
56.192055848706));
#221980=CARTESIAN_POINT('Ctrl Pts',(-7.08204139587035,3.57342620551511,
56.2172590565886));
#221981=CARTESIAN_POINT('Ctrl Pts',(-7.32635415445363,3.0412647168216,56.2378565042868));
#221982=CARTESIAN_POINT('Ctrl Pts',(-7.66838630813713,2.00846680578221,
56.2755917055936));
#221983=CARTESIAN_POINT('Ctrl Pts',(-7.7807572772411,1.51585918976673,56.2928000614765));
#221984=CARTESIAN_POINT('Ctrl Pts',(-7.84981220511726,0.982599014530777,
56.3131926255566));
#221985=CARTESIAN_POINT('Ctrl Pts',(-7.85391919466974,0.949213209538551,
56.3144767962577));
#221986=CARTESIAN_POINT('Ctrl Pts',(-7.86923715244024,0.817781333682439,
56.3195646681704));
#221987=CARTESIAN_POINT('Ctrl Pts',(-7.8788254213886,0.719560665028929,
56.323440829787));
#221988=CARTESIAN_POINT('Ctrl Pts',(-7.88790269596649,0.604316621768899,
56.3280597818904));
#221989=CARTESIAN_POINT('Ctrl Pts',(-7.88917767045129,0.587437825892734,
56.3287380505002));
#221990=CARTESIAN_POINT('Ctrl Pts',(-7.89101957623093,0.561965493110897,
56.3297642134599));
#221991=CARTESIAN_POINT('Ctrl Pts',(-7.89162666633343,0.553374851673178,
56.330110731003));
#221992=CARTESIAN_POINT('Ctrl Pts',(-7.89266831739549,0.538284558459132,
56.3307201797341));
#221993=CARTESIAN_POINT('Ctrl Pts',(-7.89310888095752,0.531785320748647,
56.3309829097867));
#221994=CARTESIAN_POINT('Ctrl Pts',(-7.89396160508928,0.518971312901581,
56.3315013913042));
#221995=CARTESIAN_POINT('Ctrl Pts',(-7.89437421714418,0.512656576740334,
56.3317571277389));
#221996=CARTESIAN_POINT('Ctrl Pts',(-7.89524826889938,0.499028526229135,
56.3323095279262));
#221997=CARTESIAN_POINT('Ctrl Pts',(-7.89570712487282,0.491715055083747,
56.3326062748875));
#221998=CARTESIAN_POINT('Ctrl Pts',(-7.89679491331828,0.473983160246461,
56.3333264730549));
#221999=CARTESIAN_POINT('Ctrl Pts',(-7.89741338941203,0.463564121619056,
56.3337502545563));
#222000=CARTESIAN_POINT('Ctrl Pts',(-7.89904055939394,0.435203580163036,
56.3349053804877));
#222001=CARTESIAN_POINT('Ctrl Pts',(-7.90000874154438,0.417259863033981,
56.3356379667097));
#222002=CARTESIAN_POINT('Ctrl Pts',(-7.90760136725193,0.267030132472929,
56.3417852675347));
#222003=CARTESIAN_POINT('Ctrl Pts',(-7.91096353872841,0.134603956130085,
56.3472937751941));
#222004=CARTESIAN_POINT('Ctrl Pts',(-7.91099970505067,0.00216025190750625,
56.3528639154922));
#222005=CARTESIAN_POINT('',(-7.90376924347838,0.00391285016959399,58.3576684917633));
#222006=CARTESIAN_POINT('Ctrl Pts',(-7.91934491493686,0.00236459517639777,
56.3576684917633));
#222007=CARTESIAN_POINT('Ctrl Pts',(-7.91655862145948,-1.0192215766598,
56.3988061866928));
#222008=CARTESIAN_POINT('Ctrl Pts',(-7.44280733691386,-3.36276887012757,
56.4929286702307));
#222009=CARTESIAN_POINT('Ctrl Pts',(-5.2119713477239,-6.39936160446072,
56.6400359423766));
#222010=CARTESIAN_POINT('Ctrl Pts',(-1.51916769345754,-8.09428556441302,
56.7989903082015));
#222011=CARTESIAN_POINT('Ctrl Pts',(3.93614139152782,-7.78672095142199,
57.0109294626343));
#222012=CARTESIAN_POINT('Ctrl Pts',(8.00548149351692,-3.47511119767746,
57.2228686170676));
#222013=CARTESIAN_POINT('Ctrl Pts',(7.98567764449062,1.97927930609152,57.4348077715004));
#222014=CARTESIAN_POINT('Ctrl Pts',(5.47176008357,6.78967631460865,57.6467469259335));
#222015=CARTESIAN_POINT('Ctrl Pts',(-1.56877482900821,9.23236030490876,
57.9116708689747));
#222016=CARTESIAN_POINT('Ctrl Pts',(-7.21413900831743,4.76026128847,58.1663063204541));
#222017=CARTESIAN_POINT('Ctrl Pts',(-7.90544983343671,1.06880511690692,
58.3149721947169));
#222018=CARTESIAN_POINT('Ctrl Pts',(-7.8990614508284,0.00646042416755821,
58.3576684917633));
#222019=CARTESIAN_POINT('',(-7.90710165646731,-0.00603558549463476,60.3576684917633));
#222020=CARTESIAN_POINT('Ctrl Pts',(-7.911,-6.63413768364762E-12,58.3576684917633));
#222021=CARTESIAN_POINT('Ctrl Pts',(-7.91099999999815,-2.20167589667336,
58.446255927496));
#222022=CARTESIAN_POINT('Ctrl Pts',(-6.94214576672008,-4.38610418339256,
58.5348433632287));
#222023=CARTESIAN_POINT('Ctrl Pts',(-3.67820201487687,-7.34180684107931,
58.7120182346942));
#222024=CARTESIAN_POINT('Ctrl Pts',(-1.40868175871089,-8.08992666571449,
58.8006056704269));
#222025=CARTESIAN_POINT('Ctrl Pts',(2.97309270521885,-7.65454228025018,
58.9777805418924));
#222026=CARTESIAN_POINT('Ctrl Pts',(5.05102072676115,-6.47444880833824,
59.0663679776251));
#222027=CARTESIAN_POINT('Ctrl Pts',(7.66951518848099,-2.93425195367107,
59.2435428490905));
#222028=CARTESIAN_POINT('Ctrl Pts',(8.18956872247117,-0.601881960092826,
59.3321302848233));
#222029=CARTESIAN_POINT('Ctrl Pts',(7.32306689761058,3.71537198233008,59.5093051562887));
#222030=CARTESIAN_POINT('Ctrl Pts',(5.94329958849772,5.6664351893696,59.5978925920214));
#222031=CARTESIAN_POINT('Ctrl Pts',(2.16154501637257,7.92205913233158,59.7750674634869));
#222032=CARTESIAN_POINT('Ctrl Pts',(-0.21081652930643,8.20894963712986,
59.8636548992196));
#222033=CARTESIAN_POINT('Ctrl Pts',(-4.4212390857694,6.91982244717508,60.040829770685));
#222034=CARTESIAN_POINT('Ctrl Pts',(-6.22631625634573,5.35390358803071,
60.1294172064178));
#222035=CARTESIAN_POINT('Ctrl Pts',(-7.65317280859665,2.31334857513947,
60.2645592586881));
#222036=CARTESIAN_POINT('Ctrl Pts',(-7.91100000000094,1.157028378359,60.3111138752257));
#222037=CARTESIAN_POINT('Ctrl Pts',(-7.911,-6.46316333785535E-12,60.3576684917633));
#222038=CARTESIAN_POINT('',(-7.92241601769487,0.00219170473266906,62.357667929495));
#222039=CARTESIAN_POINT('Ctrl Pts',(-7.90475974663917,-0.00966143243572837,
60.3576684917633));
#222040=CARTESIAN_POINT('Ctrl Pts',(-7.91126008640382,-0.81782965792324,
60.3900925685658));
#222041=CARTESIAN_POINT('Ctrl Pts',(-7.42667005382225,-4.25751452650637,
60.5284862225846));
#222042=CARTESIAN_POINT('Ctrl Pts',(-3.54336063882975,-7.96788788067822,
60.7198646652124));
#222043=CARTESIAN_POINT('Ctrl Pts',(1.90559845092771,-8.01211367516218,
60.931803819645));
#222044=CARTESIAN_POINT('Ctrl Pts',(5.51918048952775,-6.13637686246202,
61.09075818547));
#222045=CARTESIAN_POINT('Ctrl Pts',(7.76323891949608,-2.74908180270005,
61.2497125512946));
#222046=CARTESIAN_POINT('Ctrl Pts',(8.30052305478131,2.68841017079816,61.4616517057278));
#222047=CARTESIAN_POINT('Ctrl Pts',(4.66794071633822,7.37390407097891,61.6735908601605));
#222048=CARTESIAN_POINT('Ctrl Pts',(-0.724272964357983,8.19536592754439,
61.8855300145938));
#222049=CARTESIAN_POINT('Ctrl Pts',(-5.82656564660765,6.46618994551645,
62.095894041246));
#222050=CARTESIAN_POINT('Ctrl Pts',(-7.92243276554659,2.58340903040866,
62.2532732792902));
#222051=CARTESIAN_POINT('Ctrl Pts',(-7.92649243633973,0.002197789429415,
62.3576677287261));
#222052=CARTESIAN_POINT('',(-7.90269638755491,0.00610913357140485,64.3576684865946));
#222053=CARTESIAN_POINT('Ctrl Pts',(-7.91099970110201,0.00217466408241333,
62.3576684917633));
#222054=CARTESIAN_POINT('Ctrl Pts',(-7.91101038434451,-0.0366888684033183,
62.3592433651982));
#222055=CARTESIAN_POINT('Ctrl Pts',(-7.91073468951299,-0.0755529221471149,
62.3608182386331));
#222056=CARTESIAN_POINT('Ctrl Pts',(-7.910172578582,-0.114414933681696,
62.362393112068));
#222057=CARTESIAN_POINT('Ctrl Pts',(-7.90740274338427,-0.305909817463608,
62.3701533950146));
#222058=CARTESIAN_POINT('Ctrl Pts',(-7.8976699909024,-0.49764158740683,
62.3779136779612));
#222059=CARTESIAN_POINT('Ctrl Pts',(-7.8809346174063,-0.689050474324599,
62.3856739609078));
#222060=CARTESIAN_POINT('Ctrl Pts',(-7.86421938576937,-0.880228991072,62.3934249039657));
#222061=CARTESIAN_POINT('Ctrl Pts',(-7.84051833923485,-1.07108504540069,
62.4011758470236));
#222062=CARTESIAN_POINT('Ctrl Pts',(-7.80984366553306,-1.26105627151729,
62.4089267900815));
#222063=CARTESIAN_POINT('Ctrl Pts',(-7.77919968429556,-1.45083741622899,
62.4166699777009));
#222064=CARTESIAN_POINT('Ctrl Pts',(-7.74159602285949,-1.63973514400386,
62.4244131653204));
#222065=CARTESIAN_POINT('Ctrl Pts',(-7.69709681919609,-1.82718952381012,
62.4321563529399));
#222066=CARTESIAN_POINT('Ctrl Pts',(-7.65263312175257,-2.01449433248074,
62.4398933622168));
#222067=CARTESIAN_POINT('Ctrl Pts',(-7.60128491870243,-2.20035773882507,
62.4476303714938));
#222068=CARTESIAN_POINT('Ctrl Pts',(-7.54316785991181,-2.38422726206908,
62.4553673807707));
#222069=CARTESIAN_POINT('Ctrl Pts',(-7.48508540657878,-2.5679873012972,
62.4630997830914));
#222070=CARTESIAN_POINT('Ctrl Pts',(-7.42024223106417,-2.74975548035633,
62.4708321854121));
#222071=CARTESIAN_POINT('Ctrl Pts',(-7.34880456351915,-2.92899171852707,
62.4785645877328));
#222072=CARTESIAN_POINT('Ctrl Pts',(-7.27739497985612,-3.10815749457977,
62.4862939502584));
#222073=CARTESIAN_POINT('Ctrl Pts',(-7.19939620021256,-3.28479297919593,
62.494023312784));
#222074=CARTESIAN_POINT('Ctrl Pts',(-7.11502361905996,-3.45837532668434,
62.5017526753095));
#222075=CARTESIAN_POINT('Ctrl Pts',(-7.03065107082583,-3.63195760644853,
62.5094820348194));
#222076=CARTESIAN_POINT('Ctrl Pts',(-6.93990487267707,-3.80248642357877,
62.5172113943294));
#222077=CARTESIAN_POINT('Ctrl Pts',(-6.84304785148925,-3.96946055557029,
62.5249407538393));
#222078=CARTESIAN_POINT('Ctrl Pts',(-6.7461859754797,-4.13644305690495,
62.5326705007724));
#222079=CARTESIAN_POINT('Ctrl Pts',(-6.64321284592823,-4.299870206946,62.5404002477056));
#222080=CARTESIAN_POINT('Ctrl Pts',(-6.53443629959605,-4.45926711988882,
62.5481299946388));
#222081=CARTESIAN_POINT('Ctrl Pts',(-6.42563436914082,-4.61870122973656,
62.5558615453877));
#222082=CARTESIAN_POINT('Ctrl Pts',(-6.31102652740491,-4.77410293280094,
62.5635930961366));
#222083=CARTESIAN_POINT('Ctrl Pts',(-6.19096284210019,-4.92502792760962,
62.5713246468855));
#222084=CARTESIAN_POINT('Ctrl Pts',(-6.07084913154013,-5.07601580622355,
62.5790594190315));
#222085=CARTESIAN_POINT('Ctrl Pts',(-5.94527527420421,-5.2225229815602,
62.5867941911774));
#222086=CARTESIAN_POINT('Ctrl Pts',(-5.81463037939895,-5.36413968414049,
62.5945289633234));
#222087=CARTESIAN_POINT('Ctrl Pts',(-5.68382969049035,-5.50592526471045,
62.602272959189));
#222088=CARTESIAN_POINT('Ctrl Pts',(-5.54794613065987,-5.64280846153232,
62.6100169550547));
#222089=CARTESIAN_POINT('Ctrl Pts',(-5.40740504816606,-5.77441699611902,
62.6177609509203));
#222090=CARTESIAN_POINT('Ctrl Pts',(-5.26677274745945,-5.90611095124683,
62.6255099730278));
#222091=CARTESIAN_POINT('Ctrl Pts',(-5.12147717238078,-6.03252318998137,
62.6332589951353));
#222092=CARTESIAN_POINT('Ctrl Pts',(-4.9719751240282,-6.15332303442983,
62.6410080172427));
#222093=CARTESIAN_POINT('Ctrl Pts',(-4.82224460132833,-6.2743074894968,
62.6487688816814));
#222094=CARTESIAN_POINT('Ctrl Pts',(-4.6682950524527,-6.38966220575165,
62.65652974612));
#222095=CARTESIAN_POINT('Ctrl Pts',(-4.51061150420258,-6.49910031143968,
62.6642906105586));
#222096=CARTESIAN_POINT('Ctrl Pts',(-4.40217392501625,-6.57435992719061,
62.6696276882783));
#222097=CARTESIAN_POINT('Ctrl Pts',(-4.29197101186985,-6.64682241167096,
62.6749647659979));
#222098=CARTESIAN_POINT('Ctrl Pts',(-4.18016645934941,-6.71640747514102,
62.6803018437175));
#222099=CARTESIAN_POINT('Ctrl Pts',(-4.01228819221994,-6.82089177036964,
62.6883156440406));
#222100=CARTESIAN_POINT('Ctrl Pts',(-3.84028294266886,-6.91920718672284,
62.6963294443637));
#222101=CARTESIAN_POINT('Ctrl Pts',(-3.66463773976345,-7.01101641962857,
62.7043432446867));
#222102=CARTESIAN_POINT('Ctrl Pts',(-3.48919275165567,-7.10272100084623,
62.7123479102234));
#222103=CARTESIAN_POINT('Ctrl Pts',(-3.31011637171477,-7.18793402264737,
62.72035257576));
#222104=CARTESIAN_POINT('Ctrl Pts',(-3.12792412429923,-7.26636165303014,
62.7283572412967));
#222105=CARTESIAN_POINT('Ctrl Pts',(-2.94590862439637,-7.34471319955757,
62.7363541413837));
#222106=CARTESIAN_POINT('Ctrl Pts',(-2.76078358620477,-7.41629234117269,
62.7443510414708));
#222107=CARTESIAN_POINT('Ctrl Pts',(-2.57308899641308,-7.48085115588714,
62.7523479415578));
#222108=CARTESIAN_POINT('Ctrl Pts',(-2.38554464827369,-7.54535829397625,
62.7603384404615));
#222109=CARTESIAN_POINT('Ctrl Pts',(-2.19543516287578,-7.60285619673152,
62.7683289393651));
#222110=CARTESIAN_POINT('Ctrl Pts',(-2.00332074872912,-7.65314490766452,
62.7763194382688));
#222111=CARTESIAN_POINT('Ctrl Pts',(-1.81132753782506,-7.70340189190561,
62.7843048960392));
#222112=CARTESIAN_POINT('Ctrl Pts',(-1.61733224222847,-7.74645866584448,
62.7922903538095));
#222113=CARTESIAN_POINT('Ctrl Pts',(-1.42191088052068,-7.78216489467146,
62.8002758115798));
#222114=CARTESIAN_POINT('Ctrl Pts',(-1.22008211993164,-7.81904184531023,
62.8085230934043));
#222115=CARTESIAN_POINT('Ctrl Pts',(-1.01673253755762,-7.84807794077574,
62.8167703752288));
#222116=CARTESIAN_POINT('Ctrl Pts',(-0.812510161289643,-7.86916439260237,
62.8250176570533));
#222117=CARTESIAN_POINT('Ctrl Pts',(-0.61490508798135,-7.88956759197336,
62.8329977068367));
#222118=CARTESIAN_POINT('Ctrl Pts',(-0.416483253234442,-7.90252821824812,
62.8409777566202));
#222119=CARTESIAN_POINT('Ctrl Pts',(-0.217838852862356,-7.90800020448809,
62.8489578064037));
#222120=CARTESIAN_POINT('Ctrl Pts',(-0.0192102273301515,-7.91347175618418,
62.8569372224718));
#222121=CARTESIAN_POINT('Ctrl Pts',(0.179640594185305,-7.9114558438232,
62.8649166385399));
#222122=CARTESIAN_POINT('Ctrl Pts',(0.378117575871898,-7.90195849766479,
62.872896054608));
#222123=CARTESIAN_POINT('Ctrl Pts',(0.57660929883652,-7.89246044611969,
62.8808760633231));
#222124=CARTESIAN_POINT('Ctrl Pts',(0.774726792436858,-7.87547986956123,
62.8888560720383));
#222125=CARTESIAN_POINT('Ctrl Pts',(0.971876922139844,-7.85107484668259,
62.8968360807534));
#222126=CARTESIAN_POINT('Ctrl Pts',(1.16907199390426,-7.82666426046986,
62.9048179085799));
#222127=CARTESIAN_POINT('Ctrl Pts',(1.36529893034396,-7.79482589607605,
62.9127997364064));
#222128=CARTESIAN_POINT('Ctrl Pts',(1.5599722140535,-7.75566939028354,62.9207815642329));
#222129=CARTESIAN_POINT('Ctrl Pts',(1.7547902461029,-7.71648376986831,62.9287693269073));
#222130=CARTESIAN_POINT('Ctrl Pts',(1.94805198961005,-7.66996920457517,
62.9367570895817));
#222131=CARTESIAN_POINT('Ctrl Pts',(2.13918357370322,-7.61628614470323,
62.9447448522561));
#222132=CARTESIAN_POINT('Ctrl Pts',(2.33039933894324,-7.56257944090258,
62.9527361330252));
#222133=CARTESIAN_POINT('Ctrl Pts',(2.51948275470099,-7.50169804572053,
62.9607274137943));
#222134=CARTESIAN_POINT('Ctrl Pts',(2.70587694104146,-7.43385169208669,
62.9687186945635));
#222135=CARTESIAN_POINT('Ctrl Pts',(2.89244649952837,-7.3659415040549,62.9767174940653));
#222136=CARTESIAN_POINT('Ctrl Pts',(3.07632146455346,-7.29105339244926,
62.9847162935671));
#222137=CARTESIAN_POINT('Ctrl Pts',(3.2569657808282,-7.20944484010483,62.992715093069));
#222138=CARTESIAN_POINT('Ctrl Pts',(3.29833564064755,-7.19075543741466,
62.9945469205017));
#222139=CARTESIAN_POINT('Ctrl Pts',(3.33953616636706,-7.17171375837726,
62.9963787479343));
#222140=CARTESIAN_POINT('Ctrl Pts',(3.38056110967398,-7.1523232298156,62.998210575367));
#222141=CARTESIAN_POINT('Ctrl Pts',(3.56256268580738,-7.06629978954222,
63.0063372284001));
#222142=CARTESIAN_POINT('Ctrl Pts',(3.74142748038145,-6.97325526619819,
63.0144638814331));
#222143=CARTESIAN_POINT('Ctrl Pts',(3.91659768441751,-6.87344044699708,
63.0225905344662));
#222144=CARTESIAN_POINT('Ctrl Pts',(4.09161877572136,-6.77371059464572,
63.0307102697278));
#222145=CARTESIAN_POINT('Ctrl Pts',(4.26295127071939,-6.66722209323163,
63.0388300049894));
#222146=CARTESIAN_POINT('Ctrl Pts',(4.43006012935157,-6.55427251877197,
63.046949740251));
#222147=CARTESIAN_POINT('Ctrl Pts',(4.59704778123877,-6.44140486845674,
63.0550635861379));
#222148=CARTESIAN_POINT('Ctrl Pts',(4.75981764161475,-6.32208566696624,
63.0631774320248));
#222149=CARTESIAN_POINT('Ctrl Pts',(4.91786145409672,-6.19665714061297,
63.0712912779117));
#222150=CARTESIAN_POINT('Ctrl Pts',(5.07579297056634,-6.07131773589707,
63.0793993586091));
#222151=CARTESIAN_POINT('Ctrl Pts',(5.22900488937254,-5.93987786428078,
63.0875074393064));
#222152=CARTESIAN_POINT('Ctrl Pts',(5.37701970391702,-5.80272178410167,
63.0956155200038));
#222153=CARTESIAN_POINT('Ctrl Pts',(5.52497094535221,-5.66562461315069,
63.1037201182396));
#222154=CARTESIAN_POINT('Ctrl Pts',(5.66772929983764,-5.52281634526398,
63.1118247164754));
#222155=CARTESIAN_POINT('Ctrl Pts',(5.80485135161792,-5.37472062395988,
63.1199293147112));
#222156=CARTESIAN_POINT('Ctrl Pts',(5.94193054304696,-5.22667119305581,
63.1280313796861));
#222157=CARTESIAN_POINT('Ctrl Pts',(6.07337672896945,-5.07333783854438,
63.136133444661));
#222158=CARTESIAN_POINT('Ctrl Pts',(6.19878391186954,-4.91518046606098,
63.144235509636));
#222159=CARTESIAN_POINT('Ctrl Pts',(6.26549297895872,-4.83105027090261,
63.1485453201546));
#222160=CARTESIAN_POINT('Ctrl Pts',(6.33049389698373,-4.74555567194487,
63.1528551306732));
#222161=CARTESIAN_POINT('Ctrl Pts',(6.39373014667625,-4.65876977446657,
63.1571649411919));
#222162=CARTESIAN_POINT('Ctrl Pts',(6.51534733796135,-4.49186144031034,
63.1654536530113));
#222163=CARTESIAN_POINT('Ctrl Pts',(6.63038262704873,-4.32024691026366,
63.1737423648308));
#222164=CARTESIAN_POINT('Ctrl Pts',(6.73849406084604,-4.14446845710552,
63.1820310766503));
#222165=CARTESIAN_POINT('Ctrl Pts',(6.84666781982837,-3.968588669387,63.1903245668312));
#222166=CARTESIAN_POINT('Ctrl Pts',(6.94790960294631,-3.7885404163034,63.198618057012));
#222167=CARTESIAN_POINT('Ctrl Pts',(7.04192281111767,-3.60489169355483,
63.2069115471929));
#222168=CARTESIAN_POINT('Ctrl Pts',(7.13599588507806,-3.42112602685865,
63.2152103185075));
#222169=CARTESIAN_POINT('Ctrl Pts',(7.22283106273601,-3.23375557424026,
63.2235090898222));
#222170=CARTESIAN_POINT('Ctrl Pts',(7.30217902916827,-3.04337024135664,
63.2318078611369));
#222171=CARTESIAN_POINT('Ctrl Pts',(7.38161936121375,-2.8527632889557,63.2401162927004));
#222172=CARTESIAN_POINT('Ctrl Pts',(7.4535549480545,-2.65913471156,63.2484247242639));
#222173=CARTESIAN_POINT('Ctrl Pts',(7.51778509807714,-2.46309322177,63.2567331558274));
#222174=CARTESIAN_POINT('Ctrl Pts',(7.58205486961288,-2.26693080029209,
63.2650467125951));
#222175=CARTESIAN_POINT('Ctrl Pts',(7.63860963153772,-2.06835277511666,
63.2733602693627));
#222176=CARTESIAN_POINT('Ctrl Pts',(7.68729901393674,-1.86798149624863,
63.2816738261303));
#222177=CARTESIAN_POINT('Ctrl Pts',(7.73604162804305,-1.66739115308481,
63.2899964720422));
#222178=CARTESIAN_POINT('Ctrl Pts',(7.77690161275452,-1.46500392344011,
63.2983191179541));
#222179=CARTESIAN_POINT('Ctrl Pts',(7.80977969206544,-1.2614524015603,63.306641763866));
#222180=CARTESIAN_POINT('Ctrl Pts',(7.82225983434539,-1.18418657558744,
63.3098009449162));
#222181=CARTESIAN_POINT('Ctrl Pts',(7.8335904169355,-1.10675305116369,63.3129601259664));
#222182=CARTESIAN_POINT('Ctrl Pts',(7.84376796813824,-1.02918660213224,
63.3161193070166));
#222183=CARTESIAN_POINT('Ctrl Pts',(7.8717899660437,-0.815621783936255,
63.3248175255771));
#222184=CARTESIAN_POINT('Ctrl Pts',(7.8910923602589,-0.600859395635776,
63.3335157441376));
#222185=CARTESIAN_POINT('Ctrl Pts',(7.90159720958278,-0.38559374672525,
63.3422139626981));
#222186=CARTESIAN_POINT('Ctrl Pts',(7.91209282898842,-0.170517237542343,
63.3509045387076));
#222187=CARTESIAN_POINT('Ctrl Pts',(7.91380632695787,0.0450614210154638,
63.3595951147171));
#222188=CARTESIAN_POINT('Ctrl Pts',(7.90671169159671,0.260444285727001,
63.3682856907266));
#222189=CARTESIAN_POINT('Ctrl Pts',(7.89944690852185,0.480992588849226,
63.3771846892362));
#222190=CARTESIAN_POINT('Ctrl Pts',(7.88294619330481,0.70133535329489,63.3860836877457));
#222191=CARTESIAN_POINT('Ctrl Pts',(7.85723830688212,0.920721015761098,
63.3949826862553));
#222192=CARTESIAN_POINT('Ctrl Pts',(7.83220649587203,1.1343371937263,63.4036476556428));
#222193=CARTESIAN_POINT('Ctrl Pts',(7.79844563548479,1.34704571601964,63.4123126250303));
#222194=CARTESIAN_POINT('Ctrl Pts',(7.75603483252731,1.5581542531544,63.4209775944178));
#222195=CARTESIAN_POINT('Ctrl Pts',(7.71190584179489,1.77781542505187,63.4299936074884));
#222196=CARTESIAN_POINT('Ctrl Pts',(7.65841145220673,1.99574404068841,63.439009620559));
#222197=CARTESIAN_POINT('Ctrl Pts',(7.5957005129222,2.21116591824166,63.4480256336296));
#222198=CARTESIAN_POINT('Ctrl Pts',(7.53298957363764,2.42658779579498,63.4570416467002));
#222199=CARTESIAN_POINT('Ctrl Pts',(7.46106209829464,2.63950264798602,63.4660576597708));
#222200=CARTESIAN_POINT('Ctrl Pts',(7.3801277674481,2.84914638727839,63.4750736728413));
#222201=CARTESIAN_POINT('Ctrl Pts',(7.31001553187736,3.03075771440566,63.4828841140435));
#222202=CARTESIAN_POINT('Ctrl Pts',(7.23317384894474,3.20983572364905,63.4906945552457));
#222203=CARTESIAN_POINT('Ctrl Pts',(7.14982148808359,3.38584903510747,63.4985049964478));
#222204=CARTESIAN_POINT('Ctrl Pts',(7.06647513675998,3.56184965636021,63.5063148745329));
#222205=CARTESIAN_POINT('Ctrl Pts',(6.97661919325035,3.73478570167088,63.514124752618));
#222206=CARTESIAN_POINT('Ctrl Pts',(6.88051971414148,3.90414772560037,63.5219346307031));
#222207=CARTESIAN_POINT('Ctrl Pts',(6.78441020153603,4.07352743217809,63.5297453241972));
#222208=CARTESIAN_POINT('Ctrl Pts',(6.68205602943363,4.23933206820721,63.5375560176913));
#222209=CARTESIAN_POINT('Ctrl Pts',(6.57376823218394,4.40107853026155,63.5453667111854));
#222210=CARTESIAN_POINT('Ctrl Pts',(6.46540358788814,4.56293977660503,63.5531829475822));
#222211=CARTESIAN_POINT('Ctrl Pts',(6.35109710195647,4.72073680232081,63.560999183979));
#222212=CARTESIAN_POINT('Ctrl Pts',(6.2312025193915,4.87401643024816,63.5688154203759));
#222213=CARTESIAN_POINT('Ctrl Pts',(6.11126361006417,5.02735272787231,63.5766345465484));
#222214=CARTESIAN_POINT('Ctrl Pts',(5.98573271174946,5.1761680285087,63.5844536727209));
#222215=CARTESIAN_POINT('Ctrl Pts',(5.85500265344306,5.32004369607757,63.5922727988935));
#222216=CARTESIAN_POINT('Ctrl Pts',(5.72412722714509,5.46407934917006,63.600100619705));
#222217=CARTESIAN_POINT('Ctrl Pts',(5.58804133517596,5.60316414219001,63.6079284405166));
#222218=CARTESIAN_POINT('Ctrl Pts',(5.44717411064738,5.73691687305062,63.6157562613282));
#222219=CARTESIAN_POINT('Ctrl Pts',(5.33756955093011,5.84098585876409,63.6218468537741));
#222220=CARTESIAN_POINT('Ctrl Pts',(5.22507114904329,5.94182760034021,63.6279374462201));
#222221=CARTESIAN_POINT('Ctrl Pts',(5.10989405962437,6.03928006466132,63.6340280386661));
#222222=CARTESIAN_POINT('Ctrl Pts',(4.95639667417045,6.16915570707249,63.642145017668));
#222223=CARTESIAN_POINT('Ctrl Pts',(4.79783563040531,6.29326854203543,63.65026199667));
#222224=CARTESIAN_POINT('Ctrl Pts',(4.63467227805463,6.4112193750512,63.658378975672));
#222225=CARTESIAN_POINT('Ctrl Pts',(4.47162827403193,6.52908393112732,63.6664900173856));
#222226=CARTESIAN_POINT('Ctrl Pts',(4.30398893260069,6.64079528499523,63.6746010590992));
#222227=CARTESIAN_POINT('Ctrl Pts',(4.13224834309014,6.74599471027281,63.6827121008128));
#222228=CARTESIAN_POINT('Ctrl Pts',(3.96060895738772,6.8511321433185,63.6908183628275));
#222229=CARTESIAN_POINT('Ctrl Pts',(3.78487341560353,6.94976513260468,63.6989246248422));
#222230=CARTESIAN_POINT('Ctrl Pts',(3.60556490494635,7.04157814102913,63.7070308868569));
#222231=CARTESIAN_POINT('Ctrl Pts',(3.42633659048856,7.13335008584593,63.7151335233247));
#222232=CARTESIAN_POINT('Ctrl Pts',(3.24353877899788,7.21830798689402,63.7232361597926));
#222233=CARTESIAN_POINT('Ctrl Pts',(3.05771988709311,7.29618188452531,63.7313387962604));
#222234=CARTESIAN_POINT('Ctrl Pts',(2.87195773302711,7.37403200418331,63.7394389586737));
#222235=CARTESIAN_POINT('Ctrl Pts',(2.68317663386522,7.44480231082203,63.747539121087));
#222236=CARTESIAN_POINT('Ctrl Pts',(2.49194617095313,7.50827045870566,63.7556392835002));
#222237=CARTESIAN_POINT('Ctrl Pts',(2.29885302995061,7.57235681734244,63.7638183454509));
#222238=CARTESIAN_POINT('Ctrl Pts',(2.10326286058131,7.62899787763967,63.7719974074015));
#222239=CARTESIAN_POINT('Ctrl Pts',(1.90577985651915,7.6780156380725,63.7801764693522));
#222240=CARTESIAN_POINT('Ctrl Pts',(1.7102029504211,7.72656028106512,63.7882765873278));
#222241=CARTESIAN_POINT('Ctrl Pts',(1.51276990884496,7.76762807751141,63.7963767053035));
#222242=CARTESIAN_POINT('Ctrl Pts',(1.31408025082597,7.80109698019382,63.8044768232792));
#222243=CARTESIAN_POINT('Ctrl Pts',(1.11536385267232,7.83457038720209,63.8125780313883));
#222244=CARTESIAN_POINT('Ctrl Pts',(0.915390817151028,7.86044280758088,
63.8206792394974));
#222245=CARTESIAN_POINT('Ctrl Pts',(0.714768767622149,7.87864370363528,
63.8287804476065));
#222246=CARTESIAN_POINT('Ctrl Pts',(0.51409380770184,7.8968493998427,63.8368837922609));
#222247=CARTESIAN_POINT('Ctrl Pts',(0.312769811839722,7.9073795079036,63.8449871369153));
#222248=CARTESIAN_POINT('Ctrl Pts',(0.111407962529794,7.91021550059699,
63.8530904815697));
#222249=CARTESIAN_POINT('Ctrl Pts',(-0.0932798582425197,7.91309833647741,
63.8613276722986));
#222250=CARTESIAN_POINT('Ctrl Pts',(-0.298006449285327,7.90803065365533,
63.8695648630274));
#222251=CARTESIAN_POINT('Ctrl Pts',(-0.502131696847686,7.89504811632082,
63.8778020537562));
#222252=CARTESIAN_POINT('Ctrl Pts',(-0.703201609483169,7.88225990085599,
63.8859159506895));
#222253=CARTESIAN_POINT('Ctrl Pts',(-0.903687737140456,7.86179217858119,
63.8940298476228));
#222254=CARTESIAN_POINT('Ctrl Pts',(-1.1029849262459,7.83373124714362,63.9021437445562));
#222255=CARTESIAN_POINT('Ctrl Pts',(-1.30682471191427,7.80503072068078,
63.9104425821827));
#222256=CARTESIAN_POINT('Ctrl Pts',(-1.50942036041786,7.76838677815455,
63.9187414198093));
#222257=CARTESIAN_POINT('Ctrl Pts',(-1.71013668760003,7.72394675730772,
63.9270402574359));
#222258=CARTESIAN_POINT('Ctrl Pts',(-1.91085301478221,7.67950673646089,
63.9353390950625));
#222259=CARTESIAN_POINT('Ctrl Pts',(-2.10968968514138,7.62727076180396,
63.9436379326891));
#222260=CARTESIAN_POINT('Ctrl Pts',(-2.30602904505396,7.56744019093429,
63.9519367703157));
#222261=CARTESIAN_POINT('Ctrl Pts',(-2.49349993383965,7.51031211278181,
63.9598607569602));
#222262=CARTESIAN_POINT('Ctrl Pts',(-2.67909644624304,7.4461373865409,63.9677847436047));
#222263=CARTESIAN_POINT('Ctrl Pts',(-2.86225216123665,7.37505481779601,
63.9757087302493));
#222264=CARTESIAN_POINT('Ctrl Pts',(-3.04521176964433,7.30404835784126,
63.9836242326051));
#222265=CARTESIAN_POINT('Ctrl Pts',(-3.22573546964,7.22614890971879,63.9915397349609));
#222266=CARTESIAN_POINT('Ctrl Pts',(-3.40327037852688,7.14154547213987,
63.9994552373167));
#222267=CARTESIAN_POINT('Ctrl Pts',(-3.58064449004641,7.05701866180073,
64.0073635704236));
#222268=CARTESIAN_POINT('Ctrl Pts',(-3.7550348959095,6.96580010408428,64.0152719035306));
#222269=CARTESIAN_POINT('Ctrl Pts',(-3.92590687688866,6.86812756098766,
64.0231802366376));
#222270=CARTESIAN_POINT('Ctrl Pts',(-4.09662817904104,6.77054114777681,
64.0310815959953));
#222271=CARTESIAN_POINT('Ctrl Pts',(-4.26383694567463,6.66651226432804,
64.0389829553529));
#222272=CARTESIAN_POINT('Ctrl Pts',(-4.42702130471118,6.55632544704984,
64.0468843147106));
#222273=CARTESIAN_POINT('Ctrl Pts',(-4.59012164432531,6.44619536212517,
64.0547816058619));
#222274=CARTESIAN_POINT('Ctrl Pts',(-4.7492014211138,6.32991385033155,64.0626788970133));
#222275=CARTESIAN_POINT('Ctrl Pts',(-4.90377556210006,6.20781009991045,
64.0705761881646));
#222276=CARTESIAN_POINT('Ctrl Pts',(-5.05829715303041,6.08574786069473,
64.0784707945001));
#222277=CARTESIAN_POINT('Ctrl Pts',(-5.20831589148195,5.95786753804494,
64.0863654008357));
#222278=CARTESIAN_POINT('Ctrl Pts',(-5.3533775340894,5.82454032327933,64.0942600071712));
#222279=CARTESIAN_POINT('Ctrl Pts',(-5.45524197098643,5.73091597565009,
64.0998037168276));
#222280=CARTESIAN_POINT('Ctrl Pts',(-5.55466266542029,5.6346066245214,64.105347426484));
#222281=CARTESIAN_POINT('Ctrl Pts',(-5.651492361676,5.53575244080856,64.1108911361403));
#222282=CARTESIAN_POINT('Ctrl Pts',(-5.80030425041226,5.38382923587623,
64.1194109388091));
#222283=CARTESIAN_POINT('Ctrl Pts',(-5.94284646280459,5.22604605658933,
64.1279307414778));
#222284=CARTESIAN_POINT('Ctrl Pts',(-6.07869939272208,5.06293735818647,
64.1364505441465));
#222285=CARTESIAN_POINT('Ctrl Pts',(-6.21479802434825,4.89953366367332,
64.1449857556112));
#222286=CARTESIAN_POINT('Ctrl Pts',(-6.3441830342779,4.73078539157157,64.1535209670759));
#222287=CARTESIAN_POINT('Ctrl Pts',(-6.46647708311045,4.55725741357753,
64.1620561785405));
#222288=CARTESIAN_POINT('Ctrl Pts',(-6.5951791548858,4.37463683234712,64.1710386221592));
#222289=CARTESIAN_POINT('Ctrl Pts',(-6.71602711881429,4.18672256643622,
64.180021065778));
#222290=CARTESIAN_POINT('Ctrl Pts',(-6.82863630027726,3.99420170729217,
64.1890035093967));
#222291=CARTESIAN_POINT('Ctrl Pts',(-6.93608788139017,3.81049847418549,
64.1975745491338));
#222292=CARTESIAN_POINT('Ctrl Pts',(-7.03603839763765,3.6226013867786,64.206145588871));
#222293=CARTESIAN_POINT('Ctrl Pts',(-7.12820297121017,3.43112859001677,
64.2147166286082));
#222294=CARTESIAN_POINT('Ctrl Pts',(-7.22048319470356,3.23941552942108,
64.2232984234547));
#222295=CARTESIAN_POINT('Ctrl Pts',(-7.30495785393249,3.04411802202887,
64.2318802183012));
#222296=CARTESIAN_POINT('Ctrl Pts',(-7.38139040831873,2.84587361630489,
64.2404620131477));
#222297=CARTESIAN_POINT('Ctrl Pts',(-7.45795081046058,2.64729760970042,
64.2490581626526));
#222298=CARTESIAN_POINT('Ctrl Pts',(-7.52644212449434,2.44576508249835,
64.2576543121575));
#222299=CARTESIAN_POINT('Ctrl Pts',(-7.5866771208844,2.24193025392163,64.2662504616625));
#222300=CARTESIAN_POINT('Ctrl Pts',(-7.59507418438069,2.21351464670172,
64.26744880843));
#222301=CARTESIAN_POINT('Ctrl Pts',(-7.60331087730045,2.18505431498424,
64.2686471551975));
#222302=CARTESIAN_POINT('Ctrl Pts',(-7.61138677106328,2.1565510476877,64.2698455019651));
#222303=CARTESIAN_POINT('Ctrl Pts',(-7.67423591751027,1.93472965266338,
64.2791714135853));
#222304=CARTESIAN_POINT('Ctrl Pts',(-7.72742685236606,1.71000847173687,
64.2884973252056));
#222305=CARTESIAN_POINT('Ctrl Pts',(-7.77072390541452,1.48316249474539,
64.2978232368259));
#222306=CARTESIAN_POINT('Ctrl Pts',(-7.81383118656715,1.25731078845093,
64.307108272779));
#222307=CARTESIAN_POINT('Ctrl Pts',(-7.84713105685815,1.02935293352636,
64.3163933087322));
#222308=CARTESIAN_POINT('Ctrl Pts',(-7.87043857397434,0.80007352993134,
64.3256783446853));
#222309=CARTESIAN_POINT('Ctrl Pts',(-7.89357025557444,0.572523845639279,
64.3348933328903));
#222310=CARTESIAN_POINT('Ctrl Pts',(-7.90685971761943,0.34367255329281,
64.3441083210953));
#222311=CARTESIAN_POINT('Ctrl Pts',(-7.91017416660382,0.114305091721668,
64.3533233093003));
#222312=CARTESIAN_POINT('Ctrl Pts',(-7.91069511936109,0.0782539676598749,
64.3547716868545));
#222313=CARTESIAN_POINT('Ctrl Pts',(-7.91096974389411,0.0421901279273608,
64.3562200644088));
#222314=CARTESIAN_POINT('Ctrl Pts',(-7.91099763534554,0.00611666226964039,
64.357668441963));
#222315=CARTESIAN_POINT('',(-7.90615846952848,-0.00382583299217227,66.3576684917633));
#222316=CARTESIAN_POINT('Ctrl Pts',(-7.90173504288081,0.00610826169356984,
64.3576684917633));
#222317=CARTESIAN_POINT('Ctrl Pts',(-7.88678469063768,-1.90184896929262,
64.4343637390471));
#222318=CARTESIAN_POINT('Ctrl Pts',(-6.25273451541879,-6.46756077205388,
64.6170285635472));
#222319=CARTESIAN_POINT('Ctrl Pts',(1.42253012608145,-9.24895559998287,
64.9056629652644));
#222320=CARTESIAN_POINT('Ctrl Pts',(7.32623646320802,-4.72957727296922,
65.1705869083054));
#222321=CARTESIAN_POINT('Ctrl Pts',(8.21012473050356,0.647397026181004,
65.3825260627385));
#222322=CARTESIAN_POINT('Ctrl Pts',(6.91400940569619,4.50698881871914,65.5414804285633));
#222323=CARTESIAN_POINT('Ctrl Pts',(3.91324198025052,7.24650719196005,65.7004347943879));
#222324=CARTESIAN_POINT('Ctrl Pts',(-1.37637619322111,8.61578904130303,
65.9123739488212));
#222325=CARTESIAN_POINT('Ctrl Pts',(-6.56595387401644,5.74912006338756,
66.1243131032538));
#222326=CARTESIAN_POINT('Ctrl Pts',(-7.85360726975729,1.67313532969439,
66.2904062137708));
#222327=CARTESIAN_POINT('Ctrl Pts',(-7.90579410487209,0.174089764566414,
66.3505297470712));
#222328=CARTESIAN_POINT('Ctrl Pts',(-7.90615846952848,-0.00382583299217227,
66.3576684917633));
#222329=CARTESIAN_POINT('',(-7.91099999947648,-9.10112777354474E-5,68.357571168238));
#222330=CARTESIAN_POINT('Ctrl Pts',(-7.9109990733941,-0.00382893689472276,
66.3576685222996));
#222331=CARTESIAN_POINT('Ctrl Pts',(-7.91089361564559,-0.221716087729338,
66.366405760205));
#222332=CARTESIAN_POINT('Ctrl Pts',(-7.90178236265442,-0.439340629505819,
66.3751429981104));
#222333=CARTESIAN_POINT('Ctrl Pts',(-7.8837549931329,-0.655994061140797,
66.3838802360158));
#222334=CARTESIAN_POINT('Ctrl Pts',(-7.8656770179853,-0.873255672606956,
66.392642000705));
#222335=CARTESIAN_POINT('Ctrl Pts',(-7.8386328733282,-1.0895405155915,66.4014037653942));
#222336=CARTESIAN_POINT('Ctrl Pts',(-7.8027635950725,-1.30414772146843,
66.4101655300834));
#222337=CARTESIAN_POINT('Ctrl Pts',(-7.76676534922295,-1.51952654518409,
66.4189587976007));
#222338=CARTESIAN_POINT('Ctrl Pts',(-7.72187846929606,-1.733215449891,66.4277520651181));
#222339=CARTESIAN_POINT('Ctrl Pts',(-7.66829529032727,-1.9445226510238,
66.4365453326355));
#222340=CARTESIAN_POINT('Ctrl Pts',(-7.6146169970211,-2.15620493898057,
66.445354208891));
#222341=CARTESIAN_POINT('Ctrl Pts',(-7.55221159940958,-2.36549687437015,
66.4541630851466));
#222342=CARTESIAN_POINT('Ctrl Pts',(-7.48132101428588,-2.571722551366,66.4629719614022));
#222343=CARTESIAN_POINT('Ctrl Pts',(-7.41027988377687,-2.77838617543128,
66.4717995444532));
#222344=CARTESIAN_POINT('Ctrl Pts',(-7.33071758631889,-2.9819703215386,
66.4806271275041));
#222345=CARTESIAN_POINT('Ctrl Pts',(-7.24292485520071,-3.18181717606712,
66.4894547105551));
#222346=CARTESIAN_POINT('Ctrl Pts',(-7.22385673864273,-3.22522285518611,
66.491372014874));
#222347=CARTESIAN_POINT('Ctrl Pts',(-7.20440053691037,-3.26845232266537,
66.4932893191929));
#222348=CARTESIAN_POINT('Ctrl Pts',(-7.18455951561155,-3.31149899088547,
66.4952066235118));
#222349=CARTESIAN_POINT('Ctrl Pts',(-7.10272625102719,-3.48904274414686,
66.503114445859));
#222350=CARTESIAN_POINT('Ctrl Pts',(-7.01420322113214,-3.66377847849524,
66.5110222682062));
#222351=CARTESIAN_POINT('Ctrl Pts',(-6.91920610262592,-3.83516725963605,
66.5189300905533));
#222352=CARTESIAN_POINT('Ctrl Pts',(-6.82430603591275,-4.00638094506046,
66.5268298340414));
#222353=CARTESIAN_POINT('Ctrl Pts',(-6.72294522106175,-4.17425418907617,
66.5347295775294));
#222354=CARTESIAN_POINT('Ctrl Pts',(-6.61538709815423,-4.33826861104458,
66.5426293210174));
#222355=CARTESIAN_POINT('Ctrl Pts',(-6.50791888759448,-4.50214592647606,
66.5505224607785));
#222356=CARTESIAN_POINT('Ctrl Pts',(-6.39426387747894,-4.66217055919256,
66.5584156005395));
#222357=CARTESIAN_POINT('Ctrl Pts',(-6.2747311881986,-4.81784905490487,
66.5663087403005));
#222358=CARTESIAN_POINT('Ctrl Pts',(-6.15527623179081,-4.97342631189548,
66.5741967471022));
#222359=CARTESIAN_POINT('Ctrl Pts',(-6.02995142100922,-5.12466279041883,
66.5820847539039));
#222360=CARTESIAN_POINT('Ctrl Pts',(-5.89910906780965,-5.27109411850006,
66.5899727607056));
#222361=CARTESIAN_POINT('Ctrl Pts',(-5.76832751807179,-5.41745739880141,
66.5978571018891));
#222362=CARTESIAN_POINT('Ctrl Pts',(-5.63203376460771,-5.55901972164596,
66.6057414430726));
#222363=CARTESIAN_POINT('Ctrl Pts',(-5.49062043914128,-5.69534969894597,
66.613625784256));
#222364=CARTESIAN_POINT('Ctrl Pts',(-5.34924658725096,-5.83164162161629,
66.6215079246346));
#222365=CARTESIAN_POINT('Ctrl Pts',(-5.20275625972483,-5.96270387064153,
66.6293900650131));
#222366=CARTESIAN_POINT('Ctrl Pts',(-5.0515791792801,-6.08814165369563,
66.6372722053917));
#222367=CARTESIAN_POINT('Ctrl Pts',(-4.90038556859353,-6.21359315256489,
66.6451552076316));
#222368=CARTESIAN_POINT('Ctrl Pts',(-4.74450444202807,-6.33341873095843,
66.6530382098716));
#222369=CARTESIAN_POINT('Ctrl Pts',(-4.58439934210815,-6.44726326995248,
66.6609212121115));
#222370=CARTESIAN_POINT('Ctrl Pts',(-4.42427493296259,-6.56112153898944,
66.6688051650686));
#222371=CARTESIAN_POINT('Ctrl Pts',(-4.25992581625462,-6.66899713071645,
66.6766891180257));
#222372=CARTESIAN_POINT('Ctrl Pts',(-4.09184528309732,-6.77057775815286,
66.6845730709828));
#222373=CARTESIAN_POINT('Ctrl Pts',(-3.92371621248503,-6.87218771953437,
66.6924593006283));
#222374=CARTESIAN_POINT('Ctrl Pts',(-3.7518538734144,-6.96749891570094,
66.7003455302739));
#222375=CARTESIAN_POINT('Ctrl Pts',(-3.57677716645369,-7.05624447574881,
66.7082317599195));
#222376=CARTESIAN_POINT('Ctrl Pts',(-3.40162045815588,-7.14503058809851,
66.7161215931793));
#222377=CARTESIAN_POINT('Ctrl Pts',(-3.2232467624788,-7.22724493007648,
66.7240114264391));
#222378=CARTESIAN_POINT('Ctrl Pts',(-3.0421962217268,-7.30266822117171,
66.731901259699));
#222379=CARTESIAN_POINT('Ctrl Pts',(-2.86093688271062,-7.37817849489728,
66.7398001919843));
#222380=CARTESIAN_POINT('Ctrl Pts',(-2.67699485087025,-7.44688194155259,
66.7476991242696));
#222381=CARTESIAN_POINT('Ctrl Pts',(-2.49092784047274,-7.50860835931385,
66.755598056555));
#222382=CARTESIAN_POINT('Ctrl Pts',(-2.30473793558527,-7.57037554645498,
66.7635022059675));
#222383=CARTESIAN_POINT('Ctrl Pts',(-2.11642058433851,-7.62515642201285,
66.77140635538));
#222384=CARTESIAN_POINT('Ctrl Pts',(-1.92654528210323,-7.67283156833289,
66.7793105047925));
#222385=CARTESIAN_POINT('Ctrl Pts',(-1.73640976262606,-7.72057205171856,
66.7872254865562));
#222386=CARTESIAN_POINT('Ctrl Pts',(-1.54471236372734,-7.76118728382085,
66.7951404683199));
#222387=CARTESIAN_POINT('Ctrl Pts',(-1.35203048045524,-7.79460932824218,
66.8030554500836));
#222388=CARTESIAN_POINT('Ctrl Pts',(-1.27039788740664,-7.80876908267662,
66.8064087517762));
#222389=CARTESIAN_POINT('Ctrl Pts',(-1.18858862504131,-7.82163835642003,
66.8097620534687));
#222390=CARTESIAN_POINT('Ctrl Pts',(-1.10664666945898,-7.83321480293853,
66.8131153551613));
#222391=CARTESIAN_POINT('Ctrl Pts',(-0.917014832310649,-7.8600052646178,
66.8208756381074));
#222392=CARTESIAN_POINT('Ctrl Pts',(-0.726075308837745,-7.8799526064951,
66.8286359210535));
#222393=CARTESIAN_POINT('Ctrl Pts',(-0.534375051767953,-7.89293128717386,
66.8363962039996));
#222394=CARTESIAN_POINT('Ctrl Pts',(-0.342905515546799,-7.9058943473612,
66.844147147057));
#222395=CARTESIAN_POINT('Ctrl Pts',(-0.150677421537793,-7.91190541633262,
66.8518980901143));
#222396=CARTESIAN_POINT('Ctrl Pts',(0.0417517106779919,-7.91088982319028,
66.8596490331717));
#222397=CARTESIAN_POINT('Ctrl Pts',(0.233988302157394,-7.90987524623009,
66.8673922207907));
#222398=CARTESIAN_POINT('Ctrl Pts',(0.426425175715994,-7.90184800493826,
66.8751354084096));
#222399=CARTESIAN_POINT('Ctrl Pts',(0.618499207052614,-7.88678513279494,
66.8828785960286));
#222400=CARTESIAN_POINT('Ctrl Pts',(0.810419981201786,-7.87173427942066,
66.890615605305));
#222401=CARTESIAN_POINT('Ctrl Pts',(1.00197813373313,-7.84965899983031,
66.8983526145815));
#222402=CARTESIAN_POINT('Ctrl Pts',(1.19260995872977,-7.82058837213279,
66.9060896238579));
#222403=CARTESIAN_POINT('Ctrl Pts',(1.3831282731383,-7.79153505436789,66.9138220261781));
#222404=CARTESIAN_POINT('Ctrl Pts',(1.57272100461281,-7.75549473670529,
66.9215544284983));
#222405=CARTESIAN_POINT('Ctrl Pts',(1.76082889986946,-7.71254838463815,
66.9292868308185));
#222406=CARTESIAN_POINT('Ctrl Pts',(1.94886284534487,-7.66961891582482,
66.9370161933436));
#222407=CARTESIAN_POINT('Ctrl Pts',(2.1354127677142,-7.61978889965393,66.9447455558687));
#222408=CARTESIAN_POINT('Ctrl Pts',(2.3199288618094,-7.56319053549121,66.9524749183938));
#222409=CARTESIAN_POINT('Ctrl Pts',(2.50444488391394,-7.50659219341086,
66.9602042779032));
#222410=CARTESIAN_POINT('Ctrl Pts',(2.68692673275618,-7.4432256029294,66.9679336374127));
#222411=CARTESIAN_POINT('Ctrl Pts',(2.8668386540124,-7.37327316270463,66.9756629969221));
#222412=CARTESIAN_POINT('Ctrl Pts',(3.04675959310001,-7.30331721621243,
66.9833927438548));
#222413=CARTESIAN_POINT('Ctrl Pts',(3.22411001279397,-7.22677489190614,
66.9911224907874));
#222414=CARTESIAN_POINT('Ctrl Pts',(3.39837324029387,-7.14387712097952,
66.9988522377201));
#222415=CARTESIAN_POINT('Ctrl Pts',(3.57267713390611,-7.06096000500739,
67.0065837884685));
#222416=CARTESIAN_POINT('Ctrl Pts',(3.74389207622142,-6.97168464319702,
67.0143153392169));
#222417=CARTESIAN_POINT('Ctrl Pts',(3.9115251012887,-6.87632840853231,67.0220468899654));
#222418=CARTESIAN_POINT('Ctrl Pts',(4.07922797166176,-6.78093244312024,
67.0297816621108));
#222419=CARTESIAN_POINT('Ctrl Pts',(4.24334564106713,-6.67945073710558,
67.0375164342563));
#222420=CARTESIAN_POINT('Ctrl Pts',(4.40341324262927,-6.5722045627504,67.0452512064017));
#222421=CARTESIAN_POINT('Ctrl Pts',(4.56367172488819,-6.46483049727742,
67.0529952022669));
#222422=CARTESIAN_POINT('Ctrl Pts',(4.71987019539429,-6.35167843493897,
67.0607391981321));
#222423=CARTESIAN_POINT('Ctrl Pts',(4.87157524210685,-6.23311123440707,
67.0684831939973));
#222424=CARTESIAN_POINT('Ctrl Pts',(5.0233787530051,-6.11446707781403,67.0762322161042));
#222425=CARTESIAN_POINT('Ctrl Pts',(5.17068275718742,-5.99040101240313,
67.0839812382112));
#222426=CARTESIAN_POINT('Ctrl Pts',(5.31309009588742,-5.86131338805417,
67.0917302603182));
#222427=CARTESIAN_POINT('Ctrl Pts',(5.45571506654717,-5.73202848740665,
67.0994911247564));
#222428=CARTESIAN_POINT('Ctrl Pts',(5.5934281701958,-5.59770695063796,67.1072519891945));
#222429=CARTESIAN_POINT('Ctrl Pts',(5.72587117811032,-5.4587837703728,67.1150128536327));
#222430=CARTESIAN_POINT('Ctrl Pts',(5.81695106143292,-5.363247529928,67.1203499313587));
#222431=CARTESIAN_POINT('Ctrl Pts',(5.90553946723006,-5.26553576951593,
67.1256870090848));
#222432=CARTESIAN_POINT('Ctrl Pts',(5.99153182540679,-5.16579784594186,
67.1310240868108));
#222433=CARTESIAN_POINT('Ctrl Pts',(6.12065222105285,-5.01603802511763,
67.139037887132));
#222434=CARTESIAN_POINT('Ctrl Pts',(6.24431386483648,-4.86124937952612,
67.1470516874533));
#222435=CARTESIAN_POINT('Ctrl Pts',(6.36210838962077,-4.70186110372446,
67.1550654877745));
#222436=CARTESIAN_POINT('Ctrl Pts',(6.47976864255138,-4.54265451174288,
67.1630701533093));
#222437=CARTESIAN_POINT('Ctrl Pts',(6.59157490549445,-4.37885900360627,
67.1710748188441));
#222438=CARTESIAN_POINT('Ctrl Pts',(6.69715737020913,-4.21093863154684,
67.179079484379));
#222439=CARTESIAN_POINT('Ctrl Pts',(6.80263740774437,-4.0431811616334,67.1870763844641));
#222440=CARTESIAN_POINT('Ctrl Pts',(6.90190550233217,-3.8713070837191,67.1950732845494));
#222441=CARTESIAN_POINT('Ctrl Pts',(6.99463343477549,-3.69581169881811,
67.2030701846345));
#222442=CARTESIAN_POINT('Ctrl Pts',(7.08728714239552,-3.52045679061698,
67.2110606835364));
#222443=CARTESIAN_POINT('Ctrl Pts',(7.1734109661304,-3.34148664722052,67.2190511824382));
#222444=CARTESIAN_POINT('Ctrl Pts',(7.25272096058811,-3.15942394557075,
67.2270416813401));
#222445=CARTESIAN_POINT('Ctrl Pts',(7.33198091908907,-2.9774761056295,67.2350271391086));
#222446=CARTESIAN_POINT('Ctrl Pts',(7.40443548388706,-2.79243990236596,
67.2430125968771));
#222447=CARTESIAN_POINT('Ctrl Pts',(7.46984730002809,-2.60486128503287,
67.2509980546456));
#222448=CARTESIAN_POINT('Ctrl Pts',(7.53740381313978,-2.41113241357003,
67.2592453364712));
#222449=CARTESIAN_POINT('Ctrl Pts',(7.59744774193219,-2.21469190318688,
67.2674926182968));
#222450=CARTESIAN_POINT('Ctrl Pts',(7.6497716776,-2.01616325742459,67.2757399001224));
#222451=CARTESIAN_POINT('Ctrl Pts',(7.7004001901487,-1.82406742394096,67.2837199499041));
#222452=CARTESIAN_POINT('Ctrl Pts',(7.7438010761231,-1.63001700415982,67.2916999996857));
#222453=CARTESIAN_POINT('Ctrl Pts',(7.77983719867239,-1.43459198455637,
67.2996800494674));
#222454=CARTESIAN_POINT('Ctrl Pts',(7.81587045950469,-1.23918248413365,
67.3076594655337));
#222455=CARTESIAN_POINT('Ctrl Pts',(7.84454006182957,-1.04239893043744,
67.3156388816));
#222456=CARTESIAN_POINT('Ctrl Pts',(7.8657600592359,-0.844831160960169,
67.3236182976663));
#222457=CARTESIAN_POINT('Ctrl Pts',(7.88698163269343,-0.647248717733632,
67.3315983063796));
#222458=CARTESIAN_POINT('Ctrl Pts',(7.90075246300295,-0.448882275345031,
67.3395783150929));
#222459=CARTESIAN_POINT('Ctrl Pts',(7.9070384770834,-0.250326830209312,
67.3475583238062));
#222460=CARTESIAN_POINT('Ctrl Pts',(7.91332592411466,-0.0517261226573362,
67.355540151631));
#222461=CARTESIAN_POINT('Ctrl Pts',(7.91212514395374,0.147063339189747,
67.3635219794557));
#222462=CARTESIAN_POINT('Ctrl Pts',(7.90345417952032,0.345446135052728,
67.3715038072804));
#222463=CARTESIAN_POINT('Ctrl Pts',(7.89477676783494,0.543976437444913,
67.3794915699531));
#222464=CARTESIAN_POINT('Ctrl Pts',(7.87861809117559,0.742099135384174,
67.3874793326257));
#222465=CARTESIAN_POINT('Ctrl Pts',(7.85504819410101,0.939222480752311,
67.3954670952983));
#222466=CARTESIAN_POINT('Ctrl Pts',(7.83146791600566,1.13643264625102,67.4034583760657));
#222467=CARTESIAN_POINT('Ctrl Pts',(7.80046995710848,1.33264225080553,67.411449656833));
#222468=CARTESIAN_POINT('Ctrl Pts',(7.76217567509884,1.52726873499851,67.4194409376004));
#222469=CARTESIAN_POINT('Ctrl Pts',(7.72384536326102,1.72207833683767,67.4274397371005));
#222470=CARTESIAN_POINT('Ctrl Pts',(7.67820509114356,1.91530151755185,67.4354385366006));
#222471=CARTESIAN_POINT('Ctrl Pts',(7.62542660630291,2.10636893062153,67.4434373361007));
#222472=CARTESIAN_POINT('Ctrl Pts',(7.61333965782149,2.15012581347302,67.4452691635539));
#222473=CARTESIAN_POINT('Ctrl Pts',(7.60087853581273,2.19376970588041,67.4471009910071));
#222474=CARTESIAN_POINT('Ctrl Pts',(7.58804566267132,2.23729390586374,67.4489328184604));
#222475=CARTESIAN_POINT('Ctrl Pts',(7.53111436847256,2.43038309226115,67.4570594715109));
#222476=CARTESIAN_POINT('Ctrl Pts',(7.46676228830706,2.62145561255573,67.4651861245613));
#222477=CARTESIAN_POINT('Ctrl Pts',(7.39515119991861,2.80992165911123,67.4733127776118));
#222478=CARTESIAN_POINT('Ctrl Pts',(7.32360107010053,2.99822727491472,67.4814325128907));
#222479=CARTESIAN_POINT('Ctrl Pts',(7.24480436383578,3.18393054367065,67.4895522481696));
#222480=CARTESIAN_POINT('Ctrl Pts',(7.15897259892058,3.36645693985596,67.4976719834486));
#222481=CARTESIAN_POINT('Ctrl Pts',(7.0732030891675,3.54885094670502,67.5057858293526));
#222482=CARTESIAN_POINT('Ctrl Pts',(6.98040882999578,3.72807238773233,67.5138996752567));
#222483=CARTESIAN_POINT('Ctrl Pts',(6.88084958536843,3.90356631601604,67.5220135211608));
#222484=CARTESIAN_POINT('Ctrl Pts',(6.781361081294,4.07893554932477,67.530121601875));
#222485=CARTESIAN_POINT('Ctrl Pts',(6.67511733837263,4.25058227714498,67.5382296825893));
#222486=CARTESIAN_POINT('Ctrl Pts',(6.56242439132248,4.41797545355062,67.5463377633035));
#222487=CARTESIAN_POINT('Ctrl Pts',(6.44977984646348,4.58529673373972,67.554442361556));
#222488=CARTESIAN_POINT('Ctrl Pts',(6.33069179825181,4.74836784121332,67.5625469598086));
#222489=CARTESIAN_POINT('Ctrl Pts',(6.20551045213857,4.90668534026781,67.5706515580611));
#222490=CARTESIAN_POINT('Ctrl Pts',(6.08036823406626,5.06495335388555,67.5787536230524));
#222491=CARTESIAN_POINT('Ctrl Pts',(5.94913671409405,5.21847047257917,67.5868556880437));
#222492=CARTESIAN_POINT('Ctrl Pts',(5.81220769575312,5.36676464002552,67.594957753035));
#222493=CARTESIAN_POINT('Ctrl Pts',(5.73936970812569,5.44564820221379,67.5992675634517));
#222494=CARTESIAN_POINT('Ctrl Pts',(5.66492024938762,5.52305442511757,67.6035773738683));
#222495=CARTESIAN_POINT('Ctrl Pts',(5.58892283565255,5.59891619307893,67.607887184285));
#222496=CARTESIAN_POINT('Ctrl Pts',(5.4427631216407,5.74481503048304,67.6161758960581));
#222497=CARTESIAN_POINT('Ctrl Pts',(5.29093861110085,5.88493634288509,67.6244646078311));
#222498=CARTESIAN_POINT('Ctrl Pts',(5.13393236485294,6.01885865202993,67.6327533196042));
#222499=CARTESIAN_POINT('Ctrl Pts',(4.97683560604934,6.15285816606791,67.641046809738));
#222500=CARTESIAN_POINT('Ctrl Pts',(4.81455137147102,6.28065135377505,67.6493402998718));
#222501=CARTESIAN_POINT('Ctrl Pts',(4.64759513050342,6.40185758221166,67.6576337900056));
#222502=CARTESIAN_POINT('Ctrl Pts',(4.48053257504112,6.5231409924227,67.665932561273));
#222503=CARTESIAN_POINT('Ctrl Pts',(4.30879231126388,6.63782889902091,67.6742313325405));
#222504=CARTESIAN_POINT('Ctrl Pts',(4.1329187473739,6.74558400938016,67.6825301038079));
#222505=CARTESIAN_POINT('Ctrl Pts',(3.95684045650926,6.85346455290435,67.6908385353238));
#222506=CARTESIAN_POINT('Ctrl Pts',(3.77661949784773,6.9543960158946,67.6991469668397));
#222507=CARTESIAN_POINT('Ctrl Pts',(3.59282635899221,7.04808624763707,67.7074553983556));
#222508=CARTESIAN_POINT('Ctrl Pts',(3.40891984406263,7.14183427386914,67.7157689550757));
#222509=CARTESIAN_POINT('Ctrl Pts',(3.22143701376419,7.22833202552435,67.7240825117957));
#222510=CARTESIAN_POINT('Ctrl Pts',(3.03096958926497,7.30733496898499,67.7323960685157));
#222511=CARTESIAN_POINT('Ctrl Pts',(2.84029392826499,7.38642428572727,67.7407187143803));
#222512=CARTESIAN_POINT('Ctrl Pts',(2.64662742391201,7.45800231085157,67.7490413602449));
#222513=CARTESIAN_POINT('Ctrl Pts',(2.45057979742485,7.52187341401417,67.7573640061095));
#222514=CARTESIAN_POINT('Ctrl Pts',(2.3761623570886,7.54611815542717,67.760523187443));
#222515=CARTESIAN_POINT('Ctrl Pts',(2.30140196972341,7.56925294275549,67.7636823687765));
#222516=CARTESIAN_POINT('Ctrl Pts',(2.2263324580011,7.59126898393482,67.7668415501099));
#222517=CARTESIAN_POINT('Ctrl Pts',(2.01964250937032,7.65188606157403,67.7755397687682));
#222518=CARTESIAN_POINT('Ctrl Pts',(1.81042481073598,7.70407247221576,67.7842379874265));
#222519=CARTESIAN_POINT('Ctrl Pts',(1.59935335019757,7.74764414910828,67.7929362060847));
#222520=CARTESIAN_POINT('Ctrl Pts',(1.3884673442381,7.79117754244048,67.8016267821916));
#222521=CARTESIAN_POINT('Ctrl Pts',(1.17573105250927,7.8261112696819,67.8103173582985));
#222522=CARTESIAN_POINT('Ctrl Pts',(0.961830060516146,7.85231201205655,
67.8190079344054));
#222523=CARTESIAN_POINT('Ctrl Pts',(0.742799172910187,7.8791411155814,67.8279069328662));
#222524=CARTESIAN_POINT('Ctrl Pts',(0.52254724978505,7.89681304929409,67.836805931327));
#222525=CARTESIAN_POINT('Ctrl Pts',(0.301821301022647,7.90524034436961,
67.8457049297878));
#222526=CARTESIAN_POINT('Ctrl Pts',(0.0869000806119238,7.91344601548598,
67.8543698992684));
#222527=CARTESIAN_POINT('Ctrl Pts',(-0.128470297376114,7.91288707579814,
67.8630348687491));
#222528=CARTESIAN_POINT('Ctrl Pts',(-0.343593585467,7.90353493368796,67.8716998382298));
#222529=CARTESIAN_POINT('Ctrl Pts',(-0.567432152443107,7.89380390871769,
67.8807158511806));
#222530=CARTESIAN_POINT('Ctrl Pts',(-0.791002962238243,7.87455234026838,
67.8897318641314));
#222531=CARTESIAN_POINT('Ctrl Pts',(-1.01351814020634,7.8458079239472,67.8987478770822));
#222532=CARTESIAN_POINT('Ctrl Pts',(-1.23603331817452,7.81706350762602,
67.907763890033));
#222533=CARTESIAN_POINT('Ctrl Pts',(-1.45749257836948,7.77882621261139,
67.9167799029838));
#222534=CARTESIAN_POINT('Ctrl Pts',(-1.67710863993402,7.73118539487048,
67.9257959159346));
#222535=CARTESIAN_POINT('Ctrl Pts',(-1.86735884610759,7.68991484601848,
67.933606357077));
#222536=CARTESIAN_POINT('Ctrl Pts',(-2.05614366473886,7.64160470917383,
67.9414167982193));
#222537=CARTESIAN_POINT('Ctrl Pts',(-2.24290433812382,7.58638920238247,
67.9492272393616));
#222538=CARTESIAN_POINT('Ctrl Pts',(-2.42965154643451,7.53117767651968,
67.9570371173865));
#222539=CARTESIAN_POINT('Ctrl Pts',(-2.61437456247086,7.46906187225572,
67.9648469954115));
#222540=CARTESIAN_POINT('Ctrl Pts',(-2.79652900932253,7.40022611141157,
67.9726568734365));
#222541=CARTESIAN_POINT('Ctrl Pts',(-2.97870247444238,7.33138316360611,
67.9804675668704));
#222542=CARTESIAN_POINT('Ctrl Pts',(-3.15830650705467,7.25581898698974,
67.9882782603043));
#222543=CARTESIAN_POINT('Ctrl Pts',(-3.33481582197461,7.17376640500008,
67.9960889537381));
#222544=CARTESIAN_POINT('Ctrl Pts',(-3.51145039772298,7.09165559393396,
68.0039051900745));
#222545=CARTESIAN_POINT('Ctrl Pts',(-3.68498554836475,7.00304732691777,
68.011721426411));
#222546=CARTESIAN_POINT('Ctrl Pts',(-3.85491897140076,6.90822124167535,
68.0195376627474));
#222547=CARTESIAN_POINT('Ctrl Pts',(-4.02491522128161,6.81336009785741,
68.0273567888594));
#222548=CARTESIAN_POINT('Ctrl Pts',(-4.19130678757497,6.7122767350376,68.0351759149715));
#222549=CARTESIAN_POINT('Ctrl Pts',(-4.35361946929871,6.60529473351063,
68.0429950410835));
#222550=CARTESIAN_POINT('Ctrl Pts',(-4.51611263796829,6.49819377113284,
68.0508228618347));
#222551=CARTESIAN_POINT('Ctrl Pts',(-4.67451757258652,6.38518126845022,
68.0586506825859));
#222552=CARTESIAN_POINT('Ctrl Pts',(-4.82839146064093,6.26662244776321,
68.0664785033371));
#222553=CARTESIAN_POINT('Ctrl Pts',(-4.94811612292252,6.17437538137183,
68.0725690961445));
#222554=CARTESIAN_POINT('Ctrl Pts',(-5.0650983463964,6.07877146212607,68.0786596889519));
#222555=CARTESIAN_POINT('Ctrl Pts',(-5.17914486036435,5.97999828723734,
68.0847502817594));
#222556=CARTESIAN_POINT('Ctrl Pts',(-5.32878187294105,5.85040096506739,
68.0927415660241));
#222557=CARTESIAN_POINT('Ctrl Pts',(-5.47368874160669,5.71506514973898,
68.1007328502889));
#222558=CARTESIAN_POINT('Ctrl Pts',(-5.61340759243505,5.57436778488758,
68.1087241345537));
#222559=CARTESIAN_POINT('Ctrl Pts',(-5.75301402109007,5.43378362955262,
68.1167089887803));
#222560=CARTESIAN_POINT('Ctrl Pts',(-5.88744051612372,5.28784675950667,
68.1246938430069));
#222561=CARTESIAN_POINT('Ctrl Pts',(-6.01626352534858,5.13697325217489,
68.1326786972335));
#222562=CARTESIAN_POINT('Ctrl Pts',(-6.1450049258841,4.9861953224054,68.1406584930975));
#222563=CARTESIAN_POINT('Ctrl Pts',(-6.26814969893185,4.83048724323403,
68.1486382889615));
#222564=CARTESIAN_POINT('Ctrl Pts',(-6.38531203854047,4.67030097215053,
68.1566180848256));
#222565=CARTESIAN_POINT('Ctrl Pts',(-6.50824821074617,4.50222062250324,
68.1649911299677));
#222566=CARTESIAN_POINT('Ctrl Pts',(-6.62459715263853,4.32920982727371,
68.1733641751099));
#222567=CARTESIAN_POINT('Ctrl Pts',(-6.73396102446077,4.15182970761606,
68.1817372202521));
#222568=CARTESIAN_POINT('Ctrl Pts',(-6.83811830582926,3.98289429298126,
68.1897116418253));
#222569=CARTESIAN_POINT('Ctrl Pts',(-6.93593994293605,3.80999622431243,
68.1976860633985));
#222570=CARTESIAN_POINT('Ctrl Pts',(-7.02712676734891,3.63364973485455,
68.2056604849716));
#222571=CARTESIAN_POINT('Ctrl Pts',(-7.11830686206389,3.45731625998077,
68.2136343180229));
#222572=CARTESIAN_POINT('Ctrl Pts',(-7.20285296571857,3.27753516944541,
68.2216081510741));
#222573=CARTESIAN_POINT('Ctrl Pts',(-7.28051203477752,3.09484498989201,
68.2295819841253));
#222574=CARTESIAN_POINT('Ctrl Pts',(-7.35817741734007,2.91213995804744,
68.2375564654308));
#222575=CARTESIAN_POINT('Ctrl Pts',(-7.4289545182984,2.72652567467862,68.2455309467363));
#222576=CARTESIAN_POINT('Ctrl Pts',(-7.49263843978814,2.5385606572641,68.2535054280418));
#222577=CARTESIAN_POINT('Ctrl Pts',(-7.55633741607271,2.35055120516801,
68.2614817945042));
#222578=CARTESIAN_POINT('Ctrl Pts',(-7.61293976347384,2.16019022921051,
68.2694581609665));
#222579=CARTESIAN_POINT('Ctrl Pts',(-7.66229033963456,1.96805176536161,
68.2774345274288));
#222580=CARTESIAN_POINT('Ctrl Pts',(-7.7116793054823,1.77576383749292,68.2854170986862));
#222581=CARTESIAN_POINT('Ctrl Pts',(-7.75380514743358,1.58169598472964,
68.2933996699437));
#222582=CARTESIAN_POINT('Ctrl Pts',(-7.78856355251007,1.38643383849056,
68.3013822412011));
#222583=CARTESIAN_POINT('Ctrl Pts',(-7.82333757724496,1.19108394576213,
68.3093683996494));
#222584=CARTESIAN_POINT('Ctrl Pts',(-7.85073751366954,0.994539020857734,
68.3173545580978));
#222585=CARTESIAN_POINT('Ctrl Pts',(-7.87071083101772,0.797390753959685,
68.3253407165462));
#222586=CARTESIAN_POINT('Ctrl Pts',(-7.89070412513149,0.600045304758576,
68.3333348625317));
#222587=CARTESIAN_POINT('Ctrl Pts',(-7.90325593885016,0.402095642404761,
68.3413290085173));
#222588=CARTESIAN_POINT('Ctrl Pts',(-7.90836580526636,0.204135469954951,
68.3493231545028));
#222589=CARTESIAN_POINT('Ctrl Pts',(-7.91012318491482,0.136053224758531,
68.3520724924145));
#222590=CARTESIAN_POINT('Ctrl Pts',(-7.91100078247404,0.0679697153253449,
68.3548218303263));
#222591=CARTESIAN_POINT('Ctrl Pts',(-7.91099999947649,-9.10112777354474E-5,
68.357571168238));
#222592=CARTESIAN_POINT('',(-7.911,-5.21527265817667E-12,72.3576684917632));
#222593=CARTESIAN_POINT('Ctrl Pts',(-7.91099999855147,-0.000151389195569007,
68.3558388064656));
#222594=CARTESIAN_POINT('Ctrl Pts',(-7.91099267116411,-0.383051642702635,
68.3692832323818));
#222595=CARTESIAN_POINT('Ctrl Pts',(-7.88318610730695,-0.765434127276486,
68.3831365286044));
#222596=CARTESIAN_POINT('Ctrl Pts',(-7.82570790785023,-1.15863156054466,
68.3989553848451));
#222597=CARTESIAN_POINT('Ctrl Pts',(-7.82357060661066,-1.1729766882449,
68.3995346283287));
#222598=CARTESIAN_POINT('Ctrl Pts',(-7.82014362030889,-1.19555181953054,
68.4004494428244));
#222599=CARTESIAN_POINT('Ctrl Pts',(-7.81888035569568,-1.20378585219969,
68.4007837929193));
#222600=CARTESIAN_POINT('Ctrl Pts',(-7.81672501576949,-1.21768795291669,
68.4013494332849));
#222601=CARTESIAN_POINT('Ctrl Pts',(-7.81583977327504,-1.22335708649469,
68.4015804140919));
#222602=CARTESIAN_POINT('Ctrl Pts',(-7.81407557906146,-1.23457499010191,
68.402038095322));
#222603=CARTESIAN_POINT('Ctrl Pts',(-7.81319688273769,-1.24012379737284,
68.4022647842345));
#222604=CARTESIAN_POINT('Ctrl Pts',(-7.81149905296429,-1.25077184924765,
68.4027003696608));
#222605=CARTESIAN_POINT('Ctrl Pts',(-7.81068083490817,-1.25587123876143,
68.402909225789));
#222606=CARTESIAN_POINT('Ctrl Pts',(-7.80880327587672,-1.2674999617876,
68.4033860752584));
#222607=CARTESIAN_POINT('Ctrl Pts',(-7.80774073900184,-1.27402876993698,
68.4036542073709));
#222608=CARTESIAN_POINT('Ctrl Pts',(-7.80491844125137,-1.29123437701826,
68.4043618947425));
#222609=CARTESIAN_POINT('Ctrl Pts',(-7.80314496437676,-1.30190888862316,
68.4048020358127));
#222610=CARTESIAN_POINT('Ctrl Pts',(-7.79165457493977,-1.37020230018491,
68.4076247768268));
#222611=CARTESIAN_POINT('Ctrl Pts',(-7.78132158893045,-1.42771476599643,
68.4100329197169));
#222612=CARTESIAN_POINT('Ctrl Pts',(-7.76735303439255,-1.50080083637552,
68.4131283185282));
#222613=CARTESIAN_POINT('Ctrl Pts',(-7.76430591961106,-1.51648603477537,
68.4137947005674));
#222614=CARTESIAN_POINT('Ctrl Pts',(-7.68561737290302,-1.91508520955995,
68.4307800253249));
#222615=CARTESIAN_POINT('Ctrl Pts',(-7.58179044984547,-2.29187687176655,
68.4479969538861));
#222616=CARTESIAN_POINT('Ctrl Pts',(-7.42143069826756,-2.74113287224135,
68.4690066971408));
#222617=CARTESIAN_POINT('Ctrl Pts',(-7.39093334107457,-2.8223301461755,
68.4728256097494));
#222618=CARTESIAN_POINT('Ctrl Pts',(-7.3312520235115,-2.9736218218695,68.4799717258169));
#222619=CARTESIAN_POINT('Ctrl Pts',(-7.30238205928943,-3.04382971719106,
68.4833004782112));
#222620=CARTESIAN_POINT('Ctrl Pts',(-7.20486734381686,-3.27159619849965,
68.4941311044133));
#222621=CARTESIAN_POINT('Ctrl Pts',(-7.13209748889981,-3.4273375706699,
68.5015854153323));
#222622=CARTESIAN_POINT('Ctrl Pts',(-6.90353947332873,-3.87763214491744,
68.5232233510192));
#222623=CARTESIAN_POINT('Ctrl Pts',(-6.73415091316401,-4.16486754002624,
68.5371195904191));
#222624=CARTESIAN_POINT('Ctrl Pts',(-6.5320027790225,-4.46291257803096,
68.5517117487156));
#222625=CARTESIAN_POINT('Ctrl Pts',(-6.51674357505487,-4.48516467615891,
68.5528024463055));
#222626=CARTESIAN_POINT('Ctrl Pts',(-6.49174591880461,-4.5212212174636,
68.55457198989));
#222627=CARTESIAN_POINT('Ctrl Pts',(-6.4820766006714,-4.53507324276247,
68.5552523404065));
#222628=CARTESIAN_POINT('Ctrl Pts',(-6.4632510976959,-4.56185898063703,
68.5565690373003));
#222629=CARTESIAN_POINT('Ctrl Pts',(-6.45410027725383,-4.57479635878669,
68.557205495623));
#222630=CARTESIAN_POINT('Ctrl Pts',(-6.43822743721823,-4.59709487385287,
68.5583033893215));
#222631=CARTESIAN_POINT('Ctrl Pts',(-6.43152373007514,-4.60646896471027,
68.5587652134299));
#222632=CARTESIAN_POINT('Ctrl Pts',(-6.41760422149165,-4.62584361320477,
68.5597203269337));
#222633=CARTESIAN_POINT('Ctrl Pts',(-6.41038547042436,-4.63584201619037,
68.5602135523368));
#222634=CARTESIAN_POINT('Ctrl Pts',(-6.39281228645006,-4.66006239733254,
68.5614091968327));
#222635=CARTESIAN_POINT('Ctrl Pts',(-6.38243372549041,-4.67426681087956,
68.5621111089101));
#222636=CARTESIAN_POINT('Ctrl Pts',(-6.35006682320306,-4.71825634865552,
68.5642871852062));
#222637=CARTESIAN_POINT('Ctrl Pts',(-6.32791659535625,-4.74792198950683,
68.565758062387));
#222638=CARTESIAN_POINT('Ctrl Pts',(-5.92415346049836,-5.28083437618242,
68.5922461044926));
#222639=CARTESIAN_POINT('Ctrl Pts',(-5.48383614965457,-5.73675913105012,
68.6157207141508));
#222640=CARTESIAN_POINT('Ctrl Pts',(-4.81573601843965,-6.28055924018325,
68.6473916385621));
#222641=CARTESIAN_POINT('Ctrl Pts',(-4.63126144119365,-6.41779970849139,
68.6558191605972));
#222642=CARTESIAN_POINT('Ctrl Pts',(-4.26509920350076,-6.66618844531353,
68.6722879951277));
#222643=CARTESIAN_POINT('Ctrl Pts',(-4.08438534066451,-6.77841649412097,
68.6803051892477));
#222644=CARTESIAN_POINT('Ctrl Pts',(-3.84148541821903,-6.91602037258903,
68.6911535938341));
#222645=CARTESIAN_POINT('Ctrl Pts',(-3.78318320161178,-6.94808409577938,
68.6937629200508));
#222646=CARTESIAN_POINT('Ctrl Pts',(-3.70155245617908,-6.99164544597577,
68.6974312947829));
#222647=CARTESIAN_POINT('Ctrl Pts',(-3.67856048631828,-7.00376965341143,
68.6984661567266));
#222648=CARTESIAN_POINT('Ctrl Pts',(-3.63895051481667,-7.02440807363235,
68.7002523512833));
#222649=CARTESIAN_POINT('Ctrl Pts',(-3.62236127977562,-7.03297720639666,
68.7010014425127));
#222650=CARTESIAN_POINT('Ctrl Pts',(-3.59998266934696,-7.04443664513221,
68.7020134717656));
#222651=CARTESIAN_POINT('Ctrl Pts',(-3.59421978260699,-7.04737873403146,
68.7022742222193));
#222652=CARTESIAN_POINT('Ctrl Pts',(-3.58280999475297,-7.05318606295414,
68.7027907523536));
#222653=CARTESIAN_POINT('Ctrl Pts',(-3.57716324970943,-7.05605159999429,
68.7030465190522));
#222654=CARTESIAN_POINT('Ctrl Pts',(-3.5662129094974,-7.06159201365216,
68.7035427785839));
#222655=CARTESIAN_POINT('Ctrl Pts',(-3.56090972896128,-7.06426770338445,
68.7037832359767));
#222656=CARTESIAN_POINT('Ctrl Pts',(-3.54865717673049,-7.07043235656505,
68.704339083303));
#222657=CARTESIAN_POINT('Ctrl Pts',(-3.54170567128436,-7.07391704815259,
68.7046546598619));
#222658=CARTESIAN_POINT('Ctrl Pts',(-3.52306543037367,-7.08322677394313,
68.7055014696299));
#222659=CARTESIAN_POINT('Ctrl Pts',(-3.51136742059046,-7.08903310703499,
68.7060335324084));
#222660=CARTESIAN_POINT('Ctrl Pts',(-3.42954000370042,-7.12939609386607,
68.7097600120389));
#222661=CARTESIAN_POINT('Ctrl Pts',(-3.35891695323342,-7.16294003450221,
68.7130004460642));
#222662=CARTESIAN_POINT('Ctrl Pts',(-3.22304749508098,-7.22502287513372,
68.7192973931093));
#222663=CARTESIAN_POINT('Ctrl Pts',(-3.15789102889086,-7.25373796443689,
68.72234318374));
#222664=CARTESIAN_POINT('Ctrl Pts',(-2.91452953112833,-7.35708942044556,
68.7337914899018));
#222665=CARTESIAN_POINT('Ctrl Pts',(-2.73400217071512,-7.42606710366668,
68.7424250757653));
#222666=CARTESIAN_POINT('Ctrl Pts',(-2.25624090499895,-7.58883107296132,
68.7653231090039));
#222667=CARTESIAN_POINT('Ctrl Pts',(-1.95566689615631,-7.67178893398544,
68.7797685144795));
#222668=CARTESIAN_POINT('Ctrl Pts',(-1.61085615867597,-7.74536940370806,
68.7959373903439));
#222669=CARTESIAN_POINT('Ctrl Pts',(-1.57065983744819,-7.75362060349462,
68.79781641557));
#222670=CARTESIAN_POINT('Ctrl Pts',(-1.48298861968049,-7.77090735270843,
68.8019004650449));
#222671=CARTESIAN_POINT('Ctrl Pts',(-1.43549132550243,-7.77982140128291,
68.8041040025682));
#222672=CARTESIAN_POINT('Ctrl Pts',(-1.33072105479945,-7.79849200249259,
68.8089424089125));
#222673=CARTESIAN_POINT('Ctrl Pts',(-1.27341604509132,-7.80805402934875,
68.8115742725154));
#222674=CARTESIAN_POINT('Ctrl Pts',(-1.01693628396925,-7.84795203404889,
68.8232817349391));
#222675=CARTESIAN_POINT('Ctrl Pts',(-0.816744777269923,-7.87130516574341,
68.8322239127042));
#222676=CARTESIAN_POINT('Ctrl Pts',(-0.448488523544445,-7.90006120217563,
68.848233701133));
#222677=CARTESIAN_POINT('Ctrl Pts',(-0.280725844923976,-7.90780035781369,
68.8553617724685));
#222678=CARTESIAN_POINT('Ctrl Pts',(-0.023395804265896,-7.91147109826808,
68.8660305133032));
#222679=CARTESIAN_POINT('Ctrl Pts',(0.0660621300034966,-7.91122991747475,
68.8696906404969));
#222680=CARTESIAN_POINT('Ctrl Pts',(0.171259219025422,-7.90916176129038,
68.873938282075));
#222681=CARTESIAN_POINT('Ctrl Pts',(0.18701872281499,-7.90880480777876,
68.8745731311813));
#222682=CARTESIAN_POINT('Ctrl Pts',(0.211151443637993,-7.90818602735886,
68.8755430186653));
#222683=CARTESIAN_POINT('Ctrl Pts',(0.219525441755695,-7.90795800168826,
68.8758791497306));
#222684=CARTESIAN_POINT('Ctrl Pts',(0.234788091929472,-7.90751813464895,
68.8764910315976));
#222685=CARTESIAN_POINT('Ctrl Pts',(0.241676853825557,-7.90731059188653,
68.876766921324));
#222686=CARTESIAN_POINT('Ctrl Pts',(0.25656066684261,-7.90684270822007,
68.8773623998683));
#222687=CARTESIAN_POINT('Ctrl Pts',(0.264555616015933,-7.9065792423045,
68.8776818870771));
#222688=CARTESIAN_POINT('Ctrl Pts',(0.286204496454357,-7.90583295095865,
68.8785459797097));
#222689=CARTESIAN_POINT('Ctrl Pts',(0.299857628101998,-7.90532687923897,
68.8790898302436));
#222690=CARTESIAN_POINT('Ctrl Pts',(0.36379316573564,-7.90279115023373,
68.8816314823334));
#222691=CARTESIAN_POINT('Ctrl Pts',(0.414057314165239,-7.90031708827669,
68.8836148153806));
#222692=CARTESIAN_POINT('Ctrl Pts',(1.18707292050748,-7.8548706140366,68.9138953598185));
#222693=CARTESIAN_POINT('Ctrl Pts',(1.90056243693366,-7.71337058912142,
68.938425648029));
#222694=CARTESIAN_POINT('Ctrl Pts',(2.8807247211722,-7.3745043618532,68.9732787214039));
#222695=CARTESIAN_POINT('Ctrl Pts',(3.17020330597196,-7.25476991758539,
68.9837986703218));
#222696=CARTESIAN_POINT('Ctrl Pts',(3.58942916883665,-7.05147573013782,
69.000281574889));
#222697=CARTESIAN_POINT('Ctrl Pts',(3.72507333268752,-6.98076906052019,
69.0058223942346));
#222698=CARTESIAN_POINT('Ctrl Pts',(3.93614406620698,-6.86284093269931,
69.0149015035908));
#222699=CARTESIAN_POINT('Ctrl Pts',(4.01297284516761,-6.81820091398579,
69.018305525603));
#222700=CARTESIAN_POINT('Ctrl Pts',(4.12686057970146,-6.74943668443656,
69.0235251388711));
#222701=CARTESIAN_POINT('Ctrl Pts',(4.1644974755192,-6.72627938985658,69.0252790628599));
#222702=CARTESIAN_POINT('Ctrl Pts',(4.2089645106925,-6.69840335668968,69.0273881769384));
#222703=CARTESIAN_POINT('Ctrl Pts',(4.21598439557585,-6.69398725397687,
69.0277222368543));
#222704=CARTESIAN_POINT('Ctrl Pts',(4.22677575800657,-6.6871748637095,69.0282374866888));
#222705=CARTESIAN_POINT('Ctrl Pts',(4.23055218990476,-6.68478639409126,
69.0284181218006));
#222706=CARTESIAN_POINT('Ctrl Pts',(4.23742894821586,-6.68042890823025,
69.0287476461064));
#222707=CARTESIAN_POINT('Ctrl Pts',(4.24052993338372,-6.67846092846852,
69.0288964610994));
#222708=CARTESIAN_POINT('Ctrl Pts',(4.24728066833008,-6.67417010876501,
69.0292209084398));
#222709=CARTESIAN_POINT('Ctrl Pts',(4.25092988785623,-6.67184643144703,
69.0293966012091));
#222710=CARTESIAN_POINT('Ctrl Pts',(4.26094571556994,-6.66545719897486,
69.0298796657077));
#222711=CARTESIAN_POINT('Ctrl Pts',(4.26730838626577,-6.66138553141146,
69.0301874806836));
#222712=CARTESIAN_POINT('Ctrl Pts',(4.29898312434527,-6.64105189335956,
69.0317245061905));
#222713=CARTESIAN_POINT('Ctrl Pts',(4.32420779092285,-6.62465494083208,
69.0329633777252));
#222714=CARTESIAN_POINT('Ctrl Pts',(4.7360508373138,-6.35358752296343,69.0534252411683));
#222715=CARTESIAN_POINT('Ctrl Pts',(5.09964201529366,-6.06562659517763,
69.0748468048089));
#222716=CARTESIAN_POINT('Ctrl Pts',(5.78957145143553,-5.41310521750574,
69.1191708386676));
#222717=CARTESIAN_POINT('Ctrl Pts',(6.11161874692291,-5.04668612007073,
69.1419679397868));
#222718=CARTESIAN_POINT('Ctrl Pts',(6.45585263016582,-4.5733552155204,69.1678168702819));
#222719=CARTESIAN_POINT('Ctrl Pts',(6.5122608449502,-4.49266855296762,69.1721131791636));
#222720=CARTESIAN_POINT('Ctrl Pts',(6.67613615065987,-4.24868615481598,
69.1847715256489));
#222721=CARTESIAN_POINT('Ctrl Pts',(6.77907586512952,-4.08243385150327,
69.1929609192879));
#222722=CARTESIAN_POINT('Ctrl Pts',(6.89313802199598,-3.88198458271381,
69.2023346454192));
#222723=CARTESIAN_POINT('Ctrl Pts',(6.91031547873694,-3.85132394377513,
69.203755124983));
#222724=CARTESIAN_POINT('Ctrl Pts',(6.93272861315077,-3.81068522443658,
69.205620516761));
#222725=CARTESIAN_POINT('Ctrl Pts',(6.93814795430447,-3.80080923869968,
69.2060724969384));
#222726=CARTESIAN_POINT('Ctrl Pts',(6.94698731077291,-3.78461885410698,
69.2068112661683));
#222727=CARTESIAN_POINT('Ctrl Pts',(6.9504198467011,-3.77831133204551,69.2070985355975));
#222728=CARTESIAN_POINT('Ctrl Pts',(6.95703735435253,-3.76611167003633,
69.2076531090742));
#222729=CARTESIAN_POINT('Ctrl Pts',(6.96022344000786,-3.76022014335748,
69.2079204556589));
#222730=CARTESIAN_POINT('Ctrl Pts',(6.96753713534063,-3.74665493339144,
69.2085349393069));
#222731=CARTESIAN_POINT('Ctrl Pts',(6.97165956053072,-3.73897845607445,
69.2088818780199));
#222732=CARTESIAN_POINT('Ctrl Pts',(6.98262218688279,-3.71848349414215,
69.2098060389638));
#222733=CARTESIAN_POINT('Ctrl Pts',(6.98943978687597,-3.70565292083379,
69.2103823993173));
#222734=CARTESIAN_POINT('Ctrl Pts',(7.01103092801316,-3.66474730170878,
69.2122129709258));
#222735=CARTESIAN_POINT('Ctrl Pts',(7.02567104195463,-3.63660197175208,
69.2134621200273));
#222736=CARTESIAN_POINT('Ctrl Pts',(7.31090912016085,-3.08008560910539,
69.2379603604112));
#222737=CARTESIAN_POINT('Ctrl Pts',(7.52136943827937,-2.5229752637,69.2587061061502));
#222738=CARTESIAN_POINT('Ctrl Pts',(7.75354823923443,-1.60888252737453,
69.2908190019049));
#222739=CARTESIAN_POINT('Ctrl Pts',(7.81703368902067,-1.26490395938088,
69.3025508367558));
#222740=CARTESIAN_POINT('Ctrl Pts',(7.87488659003489,-0.769644385982223,
69.3201719177187));
#222741=CARTESIAN_POINT('Ctrl Pts',(7.88800296910085,-0.620964750366225,
69.3255572171987));
#222742=CARTESIAN_POINT('Ctrl Pts',(7.90281241697206,-0.373196587133696,
69.3348184871047));
#222743=CARTESIAN_POINT('Ctrl Pts',(7.90686322027276,-0.27428532286279,
69.3385915466291));
#222744=CARTESIAN_POINT('Ctrl Pts',(7.91012528879533,-0.127132962586155,
69.3443524357003));
#222745=CARTESIAN_POINT('Ctrl Pts',(7.91075310362411,-0.0789304516088896,
69.3462630678072));
#222746=CARTESIAN_POINT('Ctrl Pts',(7.91097386826388,-0.0220911882680467,
69.3485470334868));
#222747=CARTESIAN_POINT('Ctrl Pts',(7.91099326849609,-0.0134561739420375,
69.3488948591021));
#222748=CARTESIAN_POINT('Ctrl Pts',(7.91100138283853,-0.000141531331991104,
69.3494324715951));
#222749=CARTESIAN_POINT('Ctrl Pts',(7.91100008244892,0.00453812880742098,
69.3496216699129));
#222750=CARTESIAN_POINT('Ctrl Pts',(7.910990130612,0.0130791191128701,69.3499674255897));
#222751=CARTESIAN_POINT('Ctrl Pts',(7.91098280436475,0.0169404525733413,
69.3501239054311));
#222752=CARTESIAN_POINT('Ctrl Pts',(7.91096222122711,0.024768277940188,
69.3504414603468));
#222753=CARTESIAN_POINT('Ctrl Pts',(7.91094880821848,0.0287347684210849,
69.3506025444539));
#222754=CARTESIAN_POINT('Ctrl Pts',(7.91090184056813,0.040096964525484,
69.3510644716996));
#222755=CARTESIAN_POINT('Ctrl Pts',(7.9108608980438,0.0474926179049623,
69.3513657401058));
#222756=CARTESIAN_POINT('Ctrl Pts',(7.91063898918875,0.0794754370881539,
69.3526711511801));
#222757=CARTESIAN_POINT('Ctrl Pts',(7.91035376829573,0.10406150645942,69.3536812069608));
#222758=CARTESIAN_POINT('Ctrl Pts',(7.903898176097,0.500992636726142,69.3700895447515));
#222759=CARTESIAN_POINT('Ctrl Pts',(7.87155893965766,0.872413598769646,
69.3868710105261));
#222760=CARTESIAN_POINT('Ctrl Pts',(7.73899210649224,1.70762216107917,69.4259117223213));
#222761=CARTESIAN_POINT('Ctrl Pts',(7.62297811994877,2.1675356329989,69.4483032668793));
#222762=CARTESIAN_POINT('Ctrl Pts',(7.31544024044349,3.04587027786733,69.4906324823488));
#222763=CARTESIAN_POINT('Ctrl Pts',(7.12719550235307,3.46354837109602,69.5105457574904));
#222764=CARTESIAN_POINT('Ctrl Pts',(6.8858686679488,3.89488075553801,69.5306867679188));
#222765=CARTESIAN_POINT('Ctrl Pts',(6.86762098931882,3.92696643828317,69.5321828122469));
#222766=CARTESIAN_POINT('Ctrl Pts',(6.84309197543201,3.96940294309177,69.5341587725822));
#222767=CARTESIAN_POINT('Ctrl Pts',(6.83701063533985,3.97986847556331,69.5346458567571));
#222768=CARTESIAN_POINT('Ctrl Pts',(6.82697740350053,3.99704405438516,69.5354448874105));
#222769=CARTESIAN_POINT('Ctrl Pts',(6.82303959127708,4.0037622777726,69.5357573395872));
#222770=CARTESIAN_POINT('Ctrl Pts',(6.8153839180573,4.01677937499464,69.5363625726592));
#222771=CARTESIAN_POINT('Ctrl Pts',(6.81166722943277,4.02307892710757,69.5366553953119));
#222772=CARTESIAN_POINT('Ctrl Pts',(6.80305778786671,4.03762525289804,69.5373313801535));
#222773=CARTESIAN_POINT('Ctrl Pts',(6.79815876243496,4.04586831093772,69.5377143157143));
#222774=CARTESIAN_POINT('Ctrl Pts',(6.78239460038087,4.0722834822811,69.5389410439332));
#222775=CARTESIAN_POINT('Ctrl Pts',(6.77147145341944,4.09042096118371,69.539782741335));
#222776=CARTESIAN_POINT('Ctrl Pts',(6.67205524229193,4.25400828041303,69.5473691017637));
#222777=CARTESIAN_POINT('Ctrl Pts',(6.57895847681344,4.39661428572872,69.5539441114009));
#222778=CARTESIAN_POINT('Ctrl Pts',(6.10735555924581,5.07045444105337,69.5849770522167));
#222779=CARTESIAN_POINT('Ctrl Pts',(5.66876101765411,5.55647903212384,69.6070192854743));
#222780=CARTESIAN_POINT('Ctrl Pts',(4.97868738477628,6.15339729266858,69.6388855746637));
#222781=CARTESIAN_POINT('Ctrl Pts',(4.77362263612577,6.31380566900336,69.648104308806));
#222782=CARTESIAN_POINT('Ctrl Pts',(4.47839859854395,6.52212362037798,69.6615227950873));
#222783=CARTESIAN_POINT('Ctrl Pts',(4.3946512411819,6.57884411079101,69.6653450507036));
#222784=CARTESIAN_POINT('Ctrl Pts',(4.23434513926404,6.68298942724517,69.6727313189785));
#222785=CARTESIAN_POINT('Ctrl Pts',(4.15801849158751,6.7307434800034,69.6762770553784));
#222786=CARTESIAN_POINT('Ctrl Pts',(4.06763452276068,6.78516838491791,69.6804965061603));
#222787=CARTESIAN_POINT('Ctrl Pts',(4.05435000539511,6.79311465031172,69.6811171939526));
#222788=CARTESIAN_POINT('Ctrl Pts',(4.03399922461893,6.80520671059323,69.6820687465038));
#222789=CARTESIAN_POINT('Ctrl Pts',(4.02694966151494,6.80938062830892,69.6823984966464));
#222790=CARTESIAN_POINT('Ctrl Pts',(4.01410185384773,6.81696065179618,69.6829996873944));
#222791=CARTESIAN_POINT('Ctrl Pts',(4.00830572043572,6.82037033249869,69.6832709894562));
#222792=CARTESIAN_POINT('Ctrl Pts',(3.99665737169282,6.82720270803515,69.6838163748187));
#222793=CARTESIAN_POINT('Ctrl Pts',(3.99080509021004,6.83062527847498,69.6840904624925));
#222794=CARTESIAN_POINT('Ctrl Pts',(3.97418339086418,6.84031743883636,69.6848691403089));
#222795=CARTESIAN_POINT('Ctrl Pts',(3.96340357073975,6.84656909859529,69.6853743950252));
#222796=CARTESIAN_POINT('Ctrl Pts',(3.91778800794991,6.87287960113444,69.687513365312));
#222797=CARTESIAN_POINT('Ctrl Pts',(3.88281469160793,6.8926980855669,69.6891556397315));
#222798=CARTESIAN_POINT('Ctrl Pts',(3.81846529933082,6.92851807039484,69.6921800107935));
#222799=CARTESIAN_POINT('Ctrl Pts',(3.78913572325624,6.94460152450603,69.6935594785057));
#222800=CARTESIAN_POINT('Ctrl Pts',(3.75297540581836,6.96413347861145,69.6952608525216));
#222801=CARTESIAN_POINT('Ctrl Pts',(3.74624031964666,6.96775881985767,69.6955777710755));
#222802=CARTESIAN_POINT('Ctrl Pts',(3.41025500094192,7.14798398481803,69.7113885773152));
#222803=CARTESIAN_POINT('Ctrl Pts',(3.06891934335209,7.30104346016771,69.7274724741248));
#222804=CARTESIAN_POINT('Ctrl Pts',(2.1556924354718,7.63514874499331,69.7693158043987));
#222805=CARTESIAN_POINT('Ctrl Pts',(1.57175606567315,7.77638412284417,69.7947861802248));
#222806=CARTESIAN_POINT('Ctrl Pts',(0.622803894818848,7.89454100181482,
69.8344114306702));
#222807=CARTESIAN_POINT('Ctrl Pts',(0.265534713305808,7.9146171906137,69.8490851990332));
#222808=CARTESIAN_POINT('Ctrl Pts',(-0.138667298695609,7.90992307022863,
69.8654544432408));
#222809=CARTESIAN_POINT('Ctrl Pts',(-0.185462374825714,7.90896423916535,
69.8673455919368));
#222810=CARTESIAN_POINT('Ctrl Pts',(-0.256642227807109,7.90687368299679,
69.8702162927225));
#222811=CARTESIAN_POINT('Ctrl Pts',(-0.281034701086563,7.90604428102136,
69.8711989901411));
#222812=CARTESIAN_POINT('Ctrl Pts',(-0.323444047688881,7.90440574560732,
69.8729057215475));
#222813=CARTESIAN_POINT('Ctrl Pts',(-0.341462694661206,7.90364785863238,
69.8736302997199));
#222814=CARTESIAN_POINT('Ctrl Pts',(-0.379073405326805,7.90193704755114,
69.8751415586107));
#222815=CARTESIAN_POINT('Ctrl Pts',(-0.398664840305231,7.90097285767418,
69.8759281115913));
#222816=CARTESIAN_POINT('Ctrl Pts',(-0.452873237435632,7.89810285984614,
69.8781026630388));
#222817=CARTESIAN_POINT('Ctrl Pts',(-0.487481631477381,7.8960423394796,
69.8794889375054));
#222818=CARTESIAN_POINT('Ctrl Pts',(-0.626410018028492,7.88685392315334,
69.8850460762369));
#222819=CARTESIAN_POINT('Ctrl Pts',(-0.730598347615395,7.87788555069864,
69.889195835196));
#222820=CARTESIAN_POINT('Ctrl Pts',(-1.39482507476343,7.80741903953486,
69.9155627540954));
#222821=CARTESIAN_POINT('Ctrl Pts',(-1.94711386526339,7.68830796928129,
69.936954011173));
#222822=CARTESIAN_POINT('Ctrl Pts',(-2.65134425786079,7.45560737536659,
69.965587502651));
#222823=CARTESIAN_POINT('Ctrl Pts',(-2.81868809754911,7.39396395741821,
69.9725099945296));
#222824=CARTESIAN_POINT('Ctrl Pts',(-3.06242320530185,7.2947029671966,69.98288680094));
#222825=CARTESIAN_POINT('Ctrl Pts',(-3.14052183444556,7.2614220024738,69.986257760095));
#222826=CARTESIAN_POINT('Ctrl Pts',(-3.23510100330352,7.21930676186637,
69.9904080302097));
#222827=CARTESIAN_POINT('Ctrl Pts',(-3.25210634313778,7.21166228773418,
69.9911569773442));
#222828=CARTESIAN_POINT('Ctrl Pts',(-3.27931597899883,7.19931482495235,
69.9923597665165));
#222829=CARTESIAN_POINT('Ctrl Pts',(-3.28953748680595,7.19465012080496,
69.9928125999241));
#222830=CARTESIAN_POINT('Ctrl Pts',(-3.30899806132569,7.18571891971241,
69.9936766175625));
#222831=CARTESIAN_POINT('Ctrl Pts',(-3.31823890538068,7.18145633761492,
69.9940877038156));
#222832=CARTESIAN_POINT('Ctrl Pts',(-3.33931474275092,7.17168518969149,
69.9950271021966));
#222833=CARTESIAN_POINT('Ctrl Pts',(-3.35114436866679,7.16616514113917,
69.9955556910536));
#222834=CARTESIAN_POINT('Ctrl Pts',(-3.38733423748395,7.14916868540159,
69.9971767496466));
#222835=CARTESIAN_POINT('Ctrl Pts',(-3.41164951593606,7.13759719352427,
69.9982714285053));
#222836=CARTESIAN_POINT('Ctrl Pts',(-3.73852173339539,6.97998880130868,
70.0130594415364));
#222837=CARTESIAN_POINT('Ctrl Pts',(-4.03153001636447,6.81495005697474,
70.0271386478852));
#222838=CARTESIAN_POINT('Ctrl Pts',(-4.35192622129461,6.60657238437597,
70.0431916716659));
#222839=CARTESIAN_POINT('Ctrl Pts',(-4.39047968199022,6.58101425816762,
70.0451349881296));
#222840=CARTESIAN_POINT('Ctrl Pts',(-4.75731807393134,6.33316883693342,
70.0637333821983));
#222841=CARTESIAN_POINT('Ctrl Pts',(-5.06868790616475,6.08683170055626,
70.0803209690402));
#222842=CARTESIAN_POINT('Ctrl Pts',(-5.43342449658723,5.75080082891796,
70.1006879592206));
#222843=CARTESIAN_POINT('Ctrl Pts',(-5.50529118371559,5.68204023481666,
70.1047530957996));
#222844=CARTESIAN_POINT('Ctrl Pts',(-5.62844860799349,5.55967503615597,
70.1118155983288));
#222845=CARTESIAN_POINT('Ctrl Pts',(-5.68031712735868,5.50667029186173,
70.1148212252642));
#222846=CARTESIAN_POINT('Ctrl Pts',(-5.7540491384615,5.42917268713113,70.1191413959629));
#222847=CARTESIAN_POINT('Ctrl Pts',(-5.77651718671456,5.4052610258065,70.1204644269423));
#222848=CARTESIAN_POINT('Ctrl Pts',(-5.81551236097219,5.36323950898299,
70.1227724530622));
#222849=CARTESIAN_POINT('Ctrl Pts',(-5.83210524297471,5.34519134275688,
70.1237583386237));
#222850=CARTESIAN_POINT('Ctrl Pts',(-5.86412151426685,5.31004051084356,
70.1256681474333));
#222851=CARTESIAN_POINT('Ctrl Pts',(-5.87955464526416,5.29294705602304,
70.126592193162));
#222852=CARTESIAN_POINT('Ctrl Pts',(-5.91630085494447,5.25188858823575,
70.128800754827));
#222853=CARTESIAN_POINT('Ctrl Pts',(-5.93754329663954,5.22786085884446,
70.1300843438165));
#222854=CARTESIAN_POINT('Ctrl Pts',(-6.01507482827396,5.13908133473645,
70.1347952230515));
#222855=CARTESIAN_POINT('Ctrl Pts',(-6.07045584296581,5.07354394643626,
70.1382111182776));
#222856=CARTESIAN_POINT('Ctrl Pts',(-6.49114753581666,4.55894941591987,
70.1645903234642));
#222857=CARTESIAN_POINT('Ctrl Pts',(-6.80726010890783,4.0718907899914,70.1870590371129));
#222858=CARTESIAN_POINT('Ctrl Pts',(-7.27669376322296,3.13856880300413,
70.2263595207206));
#222859=CARTESIAN_POINT('Ctrl Pts',(-7.4488261141157,2.704784773958,70.2433794464231));
#222860=CARTESIAN_POINT('Ctrl Pts',(-7.63315808487446,2.08595100320572,
70.2676810524803));
#222861=CARTESIAN_POINT('Ctrl Pts',(-7.67862295448836,1.91181583995978,
70.2745321638661));
#222862=CARTESIAN_POINT('Ctrl Pts',(-7.7355394031686,1.65881205484539,70.2846578370269));
#222863=CARTESIAN_POINT('Ctrl Pts',(-7.75180071658034,1.58107952410888,
70.2877920762707));
#222864=CARTESIAN_POINT('Ctrl Pts',(-7.76952508051071,1.48949439331139,
70.2915240136778));
#222865=CARTESIAN_POINT('Ctrl Pts',(-7.772125583798,1.4758649772674,70.2920804049426));
#222866=CARTESIAN_POINT('Ctrl Pts',(-7.77605287287183,1.45498352902487,
70.2929344851342));
#222867=CARTESIAN_POINT('Ctrl Pts',(-7.77740540757182,1.44773632863859,
70.2932312079769));
#222868=CARTESIAN_POINT('Ctrl Pts',(-7.77974522226511,1.43510113992445,
70.2937490732413));
#222869=CARTESIAN_POINT('Ctrl Pts',(-7.78073704160769,1.42971399039587,
70.2939700421648));
#222870=CARTESIAN_POINT('Ctrl Pts',(-7.7827980377082,1.4184538552255,70.2944322734439));
#222871=CARTESIAN_POINT('Ctrl Pts',(-7.78386616337178,1.4125806828686,70.2946735762766));
#222872=CARTESIAN_POINT('Ctrl Pts',(-7.7867998884772,1.39634500000254,70.2953412154704));
#222873=CARTESIAN_POINT('Ctrl Pts',(-7.78865144518479,1.38597998767521,
70.295768102483));
#222874=CARTESIAN_POINT('Ctrl Pts',(-7.79581537742497,1.34540858094252,
70.2974417299759));
#222875=CARTESIAN_POINT('Ctrl Pts',(-7.80097272174366,1.31517535194466,
70.2986946986105));
#222876=CARTESIAN_POINT('Ctrl Pts',(-7.87588585811102,0.860071845863508,
70.3176523236553));
#222877=CARTESIAN_POINT('Ctrl Pts',(-7.91100437914619,0.430312242319449,
70.3370166920242));
#222878=CARTESIAN_POINT('Ctrl Pts',(-7.91099157029255,-0.828455852205915,
70.3947334112468));
#222879=CARTESIAN_POINT('Ctrl Pts',(-7.78086560444916,-1.65189306722651,
70.4331033463336));
#222880=CARTESIAN_POINT('Ctrl Pts',(-7.50795410839227,-2.49353042565992,
70.469423264854));
#222881=CARTESIAN_POINT('Ctrl Pts',(-7.49008065500436,-2.54671569306175,
70.471708634733));
#222882=CARTESIAN_POINT('Ctrl Pts',(-7.46672124334167,-2.61385140325897,
70.4745815199327));
#222883=CARTESIAN_POINT('Ctrl Pts',(-7.46175963141329,-2.62798182835505,
70.4751855194328));
#222884=CARTESIAN_POINT('Ctrl Pts',(-7.4538467285934,-2.65031430724814,
70.4761390629174));
#222885=CARTESIAN_POINT('Ctrl Pts',(-7.45092196702358,-2.65852568588199,
70.4764894442036));
#222886=CARTESIAN_POINT('Ctrl Pts',(-7.4454866211128,-2.6737062004203,70.4771367874842));
#222887=CARTESIAN_POINT('Ctrl Pts',(-7.44297981006352,-2.6806766717922,
70.4774338684247));
#222888=CARTESIAN_POINT('Ctrl Pts',(-7.43739822157482,-2.6961287218434,
70.4780920789659));
#222889=CARTESIAN_POINT('Ctrl Pts',(-7.43431871643164,-2.70460858798668,
70.4784530583023));
#222890=CARTESIAN_POINT('Ctrl Pts',(-7.42547048555206,-2.72884418543444,
70.4794840714559));
#222891=CARTESIAN_POINT('Ctrl Pts',(-7.41966611666459,-2.74458689817808,
70.4801529734319));
#222892=CARTESIAN_POINT('Ctrl Pts',(-7.38219876330018,-2.84521899854418,
70.4844236960742));
#222893=CARTESIAN_POINT('Ctrl Pts',(-7.34912896718946,-2.9295791169623,
70.4879804969658));
#222894=CARTESIAN_POINT('Ctrl Pts',(-7.24699587358815,-3.17749700386068,
70.4983740594362));
#222895=CARTESIAN_POINT('Ctrl Pts',(-7.17386722885993,-3.33932173581964,
70.5050798721963));
#222896=CARTESIAN_POINT('Ctrl Pts',(-6.94302632394983,-3.80748581263191,
70.5243649622279));
#222897=CARTESIAN_POINT('Ctrl Pts',(-6.77068147873238,-4.10614798780795,
70.5365040480709));
#222898=CARTESIAN_POINT('Ctrl Pts',(-6.20413711655041,-4.95473431817849,
70.5719205789795));
#222899=CARTESIAN_POINT('Ctrl Pts',(-5.7584184554071,-5.4663623039457,70.59443801509));
#222900=CARTESIAN_POINT('Ctrl Pts',(-5.22371792587205,-5.94123270220873,
70.622612218416));
#222901=CARTESIAN_POINT('Ctrl Pts',(-5.19404908804392,-5.96718768738708,
70.6241795543267));
#222902=CARTESIAN_POINT('Ctrl Pts',(-5.15638480129399,-5.99964356275094,
70.6261735230437));
#222903=CARTESIAN_POINT('Ctrl Pts',(-5.14856868111659,-6.00635227350239,
70.6265875319608));
#222904=CARTESIAN_POINT('Ctrl Pts',(-5.13619904930809,-6.01692745592559,
70.6272430482233));
#222905=CARTESIAN_POINT('Ctrl Pts',(-5.13165420381323,-6.02080408385659,
70.6274839645454));
#222906=CARTESIAN_POINT('Ctrl Pts',(-5.12360203253522,-6.02765662340119,
70.6279109109085));
#222907=CARTESIAN_POINT('Ctrl Pts',(-5.12009649012831,-6.03063463402343,
70.6280968208214));
#222908=CARTESIAN_POINT('Ctrl Pts',(-5.11204177255391,-6.03746515124704,
70.6285240691954));
#222909=CARTESIAN_POINT('Ctrl Pts',(-5.10749083980277,-6.04131557344143,
70.62876552497));
#222910=CARTESIAN_POINT('Ctrl Pts',(-5.09489270867644,-6.05195010461731,
70.6294340895036));
#222911=CARTESIAN_POINT('Ctrl Pts',(-5.08683633483922,-6.05872328818189,
70.6298618029537));
#222912=CARTESIAN_POINT('Ctrl Pts',(-5.0430409582497,-6.09539416640215,
70.6321877293022));
#222913=CARTESIAN_POINT('Ctrl Pts',(-5.00705231907065,-6.12499135530667,
70.6341020235493));
#222914=CARTESIAN_POINT('Ctrl Pts',(-4.43402532228738,-6.58782546603999,
70.6646011078195));
#222915=CARTESIAN_POINT('Ctrl Pts',(-3.84282802481101,-6.94930014431599,
70.6959645917874));
#222916=CARTESIAN_POINT('Ctrl Pts',(-2.84537196036472,-7.39249097282537,
70.7431489256086));
#222917=CARTESIAN_POINT('Ctrl Pts',(-2.46663670591237,-7.52733723690445,
70.7599971427778));
#222918=CARTESIAN_POINT('Ctrl Pts',(-2.04323877770246,-7.64267567665813,
70.7777709488822));
#222919=CARTESIAN_POINT('Ctrl Pts',(-2.00713039340839,-7.65223783046748,
70.7792789435391));
#222920=CARTESIAN_POINT('Ctrl Pts',(-1.95583392937872,-7.66543400165097,
70.7814106391181));
#222921=CARTESIAN_POINT('Ctrl Pts',(-1.94070089253754,-7.66927929082834,
70.7820382102926));
#222922=CARTESIAN_POINT('Ctrl Pts',(-1.9129428567909,-7.67624515967114,
70.7831870023427));
#222923=CARTESIAN_POINT('Ctrl Pts',(-1.9003213672853,-7.67937945584948,
70.7837084689452));
#222924=CARTESIAN_POINT('Ctrl Pts',(-1.87474213025496,-7.68566462800248,
70.7847635330229));
#222925=CARTESIAN_POINT('Ctrl Pts',(-1.86178402872431,-7.68881389166745,
70.7852971003599));
#222926=CARTESIAN_POINT('Ctrl Pts',(-1.82985556900204,-7.6964881565451,
70.7866095898017));
#222927=CARTESIAN_POINT('Ctrl Pts',(-1.81087629924963,-7.7009758069879,
70.7873878575732));
#222928=CARTESIAN_POINT('Ctrl Pts',(-1.74235803554529,-7.71690965259505,
70.7901908235108));
#222929=CARTESIAN_POINT('Ctrl Pts',(-1.69272511652909,-7.72794848989756,
70.7922087178548));
#222930=CARTESIAN_POINT('Ctrl Pts',(-1.42286918634173,-7.78524252255262,
70.803114679966));
#222931=CARTESIAN_POINT('Ctrl Pts',(-1.20085078209283,-7.82256483455634,
70.8118467231437));
#222932=CARTESIAN_POINT('Ctrl Pts',(-0.662017941131162,-7.88966090973433,
70.8325687972571));
#222933=CARTESIAN_POINT('Ctrl Pts',(-0.344412789612312,-7.90989289001028,
70.8443890479029));
#222934=CARTESIAN_POINT('Ctrl Pts',(0.494584770115002,-7.91269750895233,
70.875312482633));
#222935=CARTESIAN_POINT('Ctrl Pts',(1.01448141026288,-7.86296135942484,
70.8941239740843));
#222936=CARTESIAN_POINT('Ctrl Pts',(1.57414399919336,-7.75296277109719,
70.9163127209722));
#222937=CARTESIAN_POINT('Ctrl Pts',(1.62252282230501,-7.7429826708429,70.9182476458554));
#222938=CARTESIAN_POINT('Ctrl Pts',(1.71934670691455,-7.72206152957189,
70.9221584352453));
#222939=CARTESIAN_POINT('Ctrl Pts',(1.76778850440719,-7.71111606966892,
70.9241343755342));
#222940=CARTESIAN_POINT('Ctrl Pts',(1.82697858869865,-7.69715496970321,
70.9265752540666));
#222941=CARTESIAN_POINT('Ctrl Pts',(1.83782833432807,-7.6945716192099,70.9270237701683));
#222942=CARTESIAN_POINT('Ctrl Pts',(1.855741721388,-7.69026634930908,70.9277661413006));
#222943=CARTESIAN_POINT('Ctrl Pts',(1.8628085362989,-7.68855761612406,70.9280594827564));
#222944=CARTESIAN_POINT('Ctrl Pts',(1.87556537495691,-7.68545443322404,
70.9285898896411));
#222945=CARTESIAN_POINT('Ctrl Pts',(1.88125622955397,-7.68406339897233,
70.9288268197784));
#222946=CARTESIAN_POINT('Ctrl Pts',(1.89341841672263,-7.68107623481638,
70.9293338545063));
#222947=CARTESIAN_POINT('Ctrl Pts',(1.89988928485461,-7.67947824599973,
70.9296040334775));
#222948=CARTESIAN_POINT('Ctrl Pts',(1.91737625297983,-7.67513636283403,
70.9303352985852));
#222949=CARTESIAN_POINT('Ctrl Pts',(1.92838845318024,-7.67237693647971,
70.9307970162469));
#222950=CARTESIAN_POINT('Ctrl Pts',(1.98266504523857,-7.65865212471821,
70.9330788353388));
#222951=CARTESIAN_POINT('Ctrl Pts',(2.02584144979125,-7.64734459482731,
70.9349131849894));
#222952=CARTESIAN_POINT('Ctrl Pts',(2.57118063346461,-7.49958253244396,
70.9583467681856));
#222953=CARTESIAN_POINT('Ctrl Pts',(3.05870345832054,-7.31429129332358,
70.9823703445208));
#222954=CARTESIAN_POINT('Ctrl Pts',(3.97906444526342,-6.85630008518049,
71.0296999326365));
#222955=CARTESIAN_POINT('Ctrl Pts',(4.41091153929234,-6.58678714778771,
71.0528574581757));
#222956=CARTESIAN_POINT('Ctrl Pts',(4.96120297657999,-6.16480424524337,
71.0824408895058));
#222957=CARTESIAN_POINT('Ctrl Pts',(5.10442545407705,-6.04675065114256,
71.0901609842244));
#222958=CARTESIAN_POINT('Ctrl Pts',(5.25753396170436,-5.91122790774098,
71.0984362422111));
#222959=CARTESIAN_POINT('Ctrl Pts',(5.27165177157368,-5.89864105889531,
71.0991995240868));
#222960=CARTESIAN_POINT('Ctrl Pts',(5.29260030553449,-5.87982894404224,
71.100332485919));
#222961=CARTESIAN_POINT('Ctrl Pts',(5.29946542880635,-5.87364218990048,
71.1007038336044));
#222962=CARTESIAN_POINT('Ctrl Pts',(5.31122315147431,-5.86300889849365,
71.1013399384213));
#222963=CARTESIAN_POINT('Ctrl Pts',(5.31612103953301,-5.8585682382226,71.1016049511629));
#222964=CARTESIAN_POINT('Ctrl Pts',(5.32617418602407,-5.84943058581738,
71.102148969611));
#222965=CARTESIAN_POINT('Ctrl Pts',(5.33132881260921,-5.84473290496227,
71.1024279448225));
#222966=CARTESIAN_POINT('Ctrl Pts',(5.34323760036355,-5.83385094168014,
71.1030725507106));
#222967=CARTESIAN_POINT('Ctrl Pts',(5.34998725492793,-5.82766172976289,
71.1034379645731));
#222968=CARTESIAN_POINT('Ctrl Pts',(5.37116407182459,-5.80817548514979,
71.1045846484303));
#222969=CARTESIAN_POINT('Ctrl Pts',(5.38555257530667,-5.79483644451969,
71.1053640652281));
#222970=CARTESIAN_POINT('Ctrl Pts',(5.58839771817655,-5.60537828368679,
71.1163567572089));
#222971=CARTESIAN_POINT('Ctrl Pts',(5.7681882766061,-5.42019129965922,71.1261499494144));
#222972=CARTESIAN_POINT('Ctrl Pts',(6.27578539534948,-4.84343731462605,
71.1542603424725));
#222973=CARTESIAN_POINT('Ctrl Pts',(6.5750997769323,-4.42859570005681,71.1714013390723));
#222974=CARTESIAN_POINT('Ctrl Pts',(7.11471399516983,-3.50406826544196,
71.2073795007907));
#222975=CARTESIAN_POINT('Ctrl Pts',(7.34485239707152,-2.99176142641056,
71.2261554397885));
#222976=CARTESIAN_POINT('Ctrl Pts',(7.52990797772028,-2.42603571719051,
71.2496216496714));
#222977=CARTESIAN_POINT('Ctrl Pts',(7.54064256190323,-2.39246173051011,
71.2510243341122));
#222978=CARTESIAN_POINT('Ctrl Pts',(7.55335365062155,-2.35177042630304,
71.2527376812737));
#222979=CARTESIAN_POINT('Ctrl Pts',(7.55554517551398,-2.34472015589461,
71.2530350215957));
#222980=CARTESIAN_POINT('Ctrl Pts',(7.5591184472608,-2.33316769207849,71.253523042413));
#222981=CARTESIAN_POINT('Ctrl Pts',(7.56050605285211,-2.32866730205098,
71.2537133558606));
#222982=CARTESIAN_POINT('Ctrl Pts',(7.56298413646254,-2.32060462610301,
71.2540546735051));
#222983=CARTESIAN_POINT('Ctrl Pts',(7.56407611943898,-2.31704280027612,
71.2542055827151));
#222984=CARTESIAN_POINT('Ctrl Pts',(7.56638345373586,-2.30949773205644,
71.2545255257389));
#222985=CARTESIAN_POINT('Ctrl Pts',(7.56759817607682,-2.30551430024735,
71.2546945993788));
#222986=CARTESIAN_POINT('Ctrl Pts',(7.57084708041395,-2.29482995561991,
71.2551485190671));
#222987=CARTESIAN_POINT('Ctrl Pts',(7.57287550586153,-2.28812731555784,
71.2554337324246));
#222988=CARTESIAN_POINT('Ctrl Pts',(7.58269993320535,-2.25550774529017,
71.2568239491827));
#222989=CARTESIAN_POINT('Ctrl Pts',(7.59037171603507,-2.22955391105535,
71.257936756496));
#222990=CARTESIAN_POINT('Ctrl Pts',(7.65214872964639,-2.01654593088892,
71.2671210529241));
#222991=CARTESIAN_POINT('Ctrl Pts',(7.69946044412186,-1.8276038611942,71.2755900200433));
#222992=CARTESIAN_POINT('Ctrl Pts',(7.80535664015676,-1.32696352028802,
71.2984853038982));
#222993=CARTESIAN_POINT('Ctrl Pts',(7.85225665101399,-1.0131511786666,71.3132818361687));
#222994=CARTESIAN_POINT('Ctrl Pts',(7.91309322995383,-0.32572013567189,
71.345525892849));
#222995=CARTESIAN_POINT('Ctrl Pts',(7.91965158157489,0.0478278269703545,
71.3629266662739));
#222996=CARTESIAN_POINT('Ctrl Pts',(7.89154285788762,0.575949664985327,
71.3866453844034));
#222997=CARTESIAN_POINT('Ctrl Pts',(7.878677905796,0.73116667710807,71.3935125826961));
#222998=CARTESIAN_POINT('Ctrl Pts',(7.83605033322369,1.10942854801582,71.4099570442083));
#222999=CARTESIAN_POINT('Ctrl Pts',(7.80133853702477,1.33178280281065,71.4193721069612));
#223000=CARTESIAN_POINT('Ctrl Pts',(7.75306265166879,1.57301745356591,71.429314063165));
#223001=CARTESIAN_POINT('Ctrl Pts',(7.74884824351197,1.59364842376209,71.4301621640269));
#223002=CARTESIAN_POINT('Ctrl Pts',(7.74281716663155,1.62258299129979,71.4313486176197));
#223003=CARTESIAN_POINT('Ctrl Pts',(7.74106943101313,1.63090076472523,71.4316893379124));
#223004=CARTESIAN_POINT('Ctrl Pts',(7.73801466791903,1.64532336511804,71.4322795302557));
#223005=CARTESIAN_POINT('Ctrl Pts',(7.73671381390792,1.651429483412,71.4325292143487));
#223006=CARTESIAN_POINT('Ctrl Pts',(7.73399357829743,1.6641243212275,71.4330479302875));
#223007=CARTESIAN_POINT('Ctrl Pts',(7.7325730017871,1.67071278141943,71.4333169208035));
#223008=CARTESIAN_POINT('Ctrl Pts',(7.72921101956874,1.68620910140554,71.4339490903886));
#223009=CARTESIAN_POINT('Ctrl Pts',(7.72726262951738,1.69511544560198,71.4343120288363));
#223010=CARTESIAN_POINT('Ctrl Pts',(7.72313891453043,1.71381062530068,71.4350730457539));
#223011=CARTESIAN_POINT('Ctrl Pts',(7.72096036435933,1.72359873680813,71.4354710126182));
#223012=CARTESIAN_POINT('Ctrl Pts',(7.71503546507564,1.74998234756904,71.4365424556139));
#223013=CARTESIAN_POINT('Ctrl Pts',(7.71125417248284,1.76656999195839,71.4372147298258));
#223014=CARTESIAN_POINT('Ctrl Pts',(7.61095239261569,2.20011169342071,71.4547507322307));
#223015=CARTESIAN_POINT('Ctrl Pts',(7.48080403500993,2.60858433050395,71.4703688143833));
#223016=CARTESIAN_POINT('Ctrl Pts',(7.2114079641856,3.26475630405798,71.4951327822622));
#223017=CARTESIAN_POINT('Ctrl Pts',(7.09077726743393,3.51907938583672,71.504659573355));
#223018=CARTESIAN_POINT('Ctrl Pts',(6.75570443059019,4.13798078226517,71.5285775372291));
#223019=CARTESIAN_POINT('Ctrl Pts',(6.52512572917753,4.49278362904718,71.5429571990857));
#223020=CARTESIAN_POINT('Ctrl Pts',(6.19368462287517,4.92308485777645,71.5634174895336));
#223021=CARTESIAN_POINT('Ctrl Pts',(6.1178443584561,5.01701818022746,71.5680896686679));
#223022=CARTESIAN_POINT('Ctrl Pts',(6.03294769566524,5.11738005206377,71.5733563490854));
#223023=CARTESIAN_POINT('Ctrl Pts',(6.02599041812151,5.12557079506963,71.5737882182886));
#223024=CARTESIAN_POINT('Ctrl Pts',(6.0156242090462,5.13772456443133,71.5744321028692));
#223025=CARTESIAN_POINT('Ctrl Pts',(6.01222809808811,5.14169832066524,71.5746431112));
#223026=CARTESIAN_POINT('Ctrl Pts',(6.00639507990508,5.148509797536,71.5750056337904));
#223027=CARTESIAN_POINT('Ctrl Pts',(6.00396009025109,5.15134916558816,71.5751569994675));
#223028=CARTESIAN_POINT('Ctrl Pts',(5.99920946646611,5.15688078084582,71.5754523696088));
#223029=CARTESIAN_POINT('Ctrl Pts',(5.99689403089543,5.15957319867772,71.5755963587804));
#223030=CARTESIAN_POINT('Ctrl Pts',(5.99133684732384,5.16602636792826,71.5759420039353));
#223031=CARTESIAN_POINT('Ctrl Pts',(5.98809337312693,5.16978562483354,71.5761437921706));
#223032=CARTESIAN_POINT('Ctrl Pts',(5.9783078788401,5.18110566089641,71.5767527297861));
#223033=CARTESIAN_POINT('Ctrl Pts',(5.97175508422018,5.18865706863606,71.577160698198));
#223034=CARTESIAN_POINT('Ctrl Pts',(5.91266598286916,5.25649084540286,71.5808411160431));
#223035=CARTESIAN_POINT('Ctrl Pts',(5.85923448934556,5.31598395347245,71.5841805354665));
#223036=CARTESIAN_POINT('Ctrl Pts',(5.65045994989739,5.54147152182264,71.5972366174554));
#223037=CARTESIAN_POINT('Ctrl Pts',(5.48889821859864,5.70154252001349,71.6073546406233));
#223038=CARTESIAN_POINT('Ctrl Pts',(4.98105913775226,6.16308233597734,71.6386049207332));
#223039=CARTESIAN_POINT('Ctrl Pts',(4.61522563577888,6.4416017270678,71.6603496219915));
#223040=CARTESIAN_POINT('Ctrl Pts',(3.95188749017471,6.86095327751132,71.6965434586497));
#223041=CARTESIAN_POINT('Ctrl Pts',(3.66595629059359,7.01789761495503,71.7112583315734));
#223042=CARTESIAN_POINT('Ctrl Pts',(3.14614603478404,7.2627502210597,71.7361935944456));
#223043=CARTESIAN_POINT('Ctrl Pts',(2.91626804767273,7.35806844619734,71.746643509954));
#223044=CARTESIAN_POINT('Ctrl Pts',(2.66064294656456,7.45019653283647,71.7576581973014));
#223045=CARTESIAN_POINT('Ctrl Pts',(2.63898633870715,7.45789517107288,71.7585867680611));
#223046=CARTESIAN_POINT('Ctrl Pts',(2.60855142823489,7.46856521158115,71.7598853465347));
#223047=CARTESIAN_POINT('Ctrl Pts',(2.59980109090375,7.47161569955595,71.7602579628025));
#223048=CARTESIAN_POINT('Ctrl Pts',(2.58461730231572,7.47687907392358,71.7609032616196));
#223049=CARTESIAN_POINT('Ctrl Pts',(2.57818632750207,7.47909904644293,71.7611761772865));
#223050=CARTESIAN_POINT('Ctrl Pts',(2.56480975184804,7.48369733716626,71.761743028615));
#223051=CARTESIAN_POINT('Ctrl Pts',(2.55786368607432,7.48607428906018,71.7620369191849));
#223052=CARTESIAN_POINT('Ctrl Pts',(2.54151905395885,7.49164203710807,71.7627273917477));
#223053=CARTESIAN_POINT('Ctrl Pts',(2.53211776190156,7.49482482480951,71.7631237107888));
#223054=CARTESIAN_POINT('Ctrl Pts',(2.50144890816817,7.50514340880997,71.7644138746114));
#223055=CARTESIAN_POINT('Ctrl Pts',(2.48015689393075,7.51220646807339,71.7653053394764));
#223056=CARTESIAN_POINT('Ctrl Pts',(2.07088663585798,7.64604129939103,71.7823606298767));
#223057=CARTESIAN_POINT('Ctrl Pts',(1.67368805803971,7.74269540356035,71.7974868025735));
#223058=CARTESIAN_POINT('Ctrl Pts',(0.973651664704941,7.85662401868755,
71.8227571713165));
#223059=CARTESIAN_POINT('Ctrl Pts',(0.674011368291598,7.88798147197124,
71.8331581214453));
#223060=CARTESIAN_POINT('Ctrl Pts',(-0.157416664472316,7.9272594460788,
71.8620047659941));
#223061=CARTESIAN_POINT('Ctrl Pts',(-0.689337248274834,7.89880153920904,
71.8804813650044));
#223062=CARTESIAN_POINT('Ctrl Pts',(-1.25111560064042,7.81153072482053,
71.9029706469464));
#223063=CARTESIAN_POINT('Ctrl Pts',(-1.28780271249366,7.80556638738845,
71.9044509848803));
#223064=CARTESIAN_POINT('Ctrl Pts',(-1.33636181684843,7.79732032012387,
71.9064248480477));
#223065=CARTESIAN_POINT('Ctrl Pts',(-1.348272901174,7.79526954391305,71.9069101753331));
#223066=CARTESIAN_POINT('Ctrl Pts',(-1.36677328278422,7.79204059280609,
71.9076657492807));
#223067=CARTESIAN_POINT('Ctrl Pts',(-1.37336588997148,7.79088133258608,
71.907935345499));
#223068=CARTESIAN_POINT('Ctrl Pts',(-1.38657690877119,7.78854098496303,
71.9084762815399));
#223069=CARTESIAN_POINT('Ctrl Pts',(-1.39319530180666,7.78735982532539,
71.9087476236088));
#223070=CARTESIAN_POINT('Ctrl Pts',(-1.40798684636991,7.78470057392633,
71.909354815265));
#223071=CARTESIAN_POINT('Ctrl Pts',(-1.41615918704046,7.78321804536101,
71.9096908117686));
#223072=CARTESIAN_POINT('Ctrl Pts',(-1.44011781342516,7.77883277339254,
71.9106773530511));
#223073=CARTESIAN_POINT('Ctrl Pts',(-1.45589757405786,7.77589486058238,
71.9113290372067));
#223074=CARTESIAN_POINT('Ctrl Pts',(-1.57454820754044,7.75343037941236,
71.9162432057093));
#223075=CARTESIAN_POINT('Ctrl Pts',(-1.67702929151945,7.73191157069865,
71.920567030218));
#223076=CARTESIAN_POINT('Ctrl Pts',(-1.93194104340771,7.67307926361051,
71.9314843229525));
#223077=CARTESIAN_POINT('Ctrl Pts',(-2.08374502194059,7.63325267321287,
71.938131662078));
#223078=CARTESIAN_POINT('Ctrl Pts',(-2.42685656466533,7.53223714827264,
71.9533973911316));
#223079=CARTESIAN_POINT('Ctrl Pts',(-2.61722276979147,7.46822423516205,
71.9620407646658));
#223080=CARTESIAN_POINT('Ctrl Pts',(-2.94437925591308,7.34416700173195,
71.9770980241227));
#223081=CARTESIAN_POINT('Ctrl Pts',(-3.08229022865552,7.28736204004305,
71.9835111389092));
#223082=CARTESIAN_POINT('Ctrl Pts',(-3.9015094674697,6.9225107432412,72.0219308591963));
#223083=CARTESIAN_POINT('Ctrl Pts',(-4.53796070296965,6.52302937767378,
72.0528960236787));
#223084=CARTESIAN_POINT('Ctrl Pts',(-5.16558010832075,5.99218018713211,
72.086310519397));
#223085=CARTESIAN_POINT('Ctrl Pts',(-5.22162953362689,5.94340192047556,
72.0893208720212));
#223086=CARTESIAN_POINT('Ctrl Pts',(-5.29720552792464,5.87573581033753,
72.0934162959694));
#223087=CARTESIAN_POINT('Ctrl Pts',(-5.31733395891755,5.85752655083411,
72.0945106448856));
#223088=CARTESIAN_POINT('Ctrl Pts',(-5.35154991008816,5.82625125707545,
72.0963771141525));
#223089=CARTESIAN_POINT('Ctrl Pts',(-5.36568424990266,5.8132368507921,72.0971499672951));
#223090=CARTESIAN_POINT('Ctrl Pts',(-5.39425491760438,5.78673700283436,
72.0987159267158));
#223091=CARTESIAN_POINT('Ctrl Pts',(-5.40868842780447,5.77324871710554,
72.0995089843347));
#223092=CARTESIAN_POINT('Ctrl Pts',(-5.43382503352709,5.74958126025726,
72.10089358198));
#223093=CARTESIAN_POINT('Ctrl Pts',(-5.44455041556772,5.73942592396704,
72.1014854755283));
#223094=CARTESIAN_POINT('Ctrl Pts',(-5.47222447673021,5.71307533787036,
72.1030155931375));
#223095=CARTESIAN_POINT('Ctrl Pts',(-5.48912974322961,5.6968346655181,72.1039531179759));
#223096=CARTESIAN_POINT('Ctrl Pts',(-5.53122212288266,5.65603574099872,
72.1062946137568));
#223097=CARTESIAN_POINT('Ctrl Pts',(-5.55631812750907,5.63138414216991,
72.1076971126576));
#223098=CARTESIAN_POINT('Ctrl Pts',(-5.62655310562677,5.56146631645238,
72.1116408926125));
#223099=CARTESIAN_POINT('Ctrl Pts',(-5.67130918682736,5.51581903562978,
72.1141760187627));
#223100=CARTESIAN_POINT('Ctrl Pts',(-5.81726065000472,5.36330670187768,
72.1225198004269));
#223101=CARTESIAN_POINT('Ctrl Pts',(-5.91602808554049,5.25415957983556,
72.1282901708205));
#223102=CARTESIAN_POINT('Ctrl Pts',(-6.44153883999227,4.63980453477771,
72.1597869003572));
#223103=CARTESIAN_POINT('Ctrl Pts',(-6.80665855149192,4.08540427680142,
72.1844683217585));
#223104=CARTESIAN_POINT('Ctrl Pts',(-7.11640740702316,3.45576416596647,
72.2124003032842));
#223105=CARTESIAN_POINT('Ctrl Pts',(-7.13400084120414,3.41929704852806,
72.2140185152756));
#223106=CARTESIAN_POINT('Ctrl Pts',(-7.15707583306152,3.37051452030001,
72.2161852263665));
#223107=CARTESIAN_POINT('Ctrl Pts',(-7.16280706343204,3.358317671269,72.2167271340219));
#223108=CARTESIAN_POINT('Ctrl Pts',(-7.17255477876143,3.3374347221852,72.2176552548076));
#223109=CARTESIAN_POINT('Ctrl Pts',(-7.17658671916797,3.32875586981402,
72.2180410598546));
#223110=CARTESIAN_POINT('Ctrl Pts',(-7.18440603692826,3.31184435283327,
72.218792979462));
#223111=CARTESIAN_POINT('Ctrl Pts',(-7.18819503677124,3.30361245209955,
72.2191590524219));
#223112=CARTESIAN_POINT('Ctrl Pts',(-7.19602549777607,3.286522908259,72.2199191478036));
#223113=CARTESIAN_POINT('Ctrl Pts',(-7.20006476785826,3.27766427951054,
72.2203132231805));
#223114=CARTESIAN_POINT('Ctrl Pts',(-7.20922715744471,3.25747133606334,
72.2212116398839));
#223115=CARTESIAN_POINT('Ctrl Pts',(-7.21433991602449,3.24613235831654,
72.2217162261814));
#223116=CARTESIAN_POINT('Ctrl Pts',(-7.22732903215772,3.21714308514874,
72.2230064543193));
#223117=CARTESIAN_POINT('Ctrl Pts',(-7.23516747304474,3.19947592612922,
72.2237929578117));
#223118=CARTESIAN_POINT('Ctrl Pts',(-7.32395778147548,2.99735544136753,
72.2327923230002));
#223119=CARTESIAN_POINT('Ctrl Pts',(-7.39789943580156,2.80990708683299,
72.2411502310389));
#223120=CARTESIAN_POINT('Ctrl Pts',(-7.67523641657879,2.01970372487532,
72.2761574661352));
#223121=CARTESIAN_POINT('Ctrl Pts',(-7.81273495777942,1.39631261206159,
72.3030619631906));
#223122=CARTESIAN_POINT('Ctrl Pts',(-7.88418812074589,0.659116211714981,
72.3333280215586));
#223123=CARTESIAN_POINT('Ctrl Pts',(-7.89221192187817,0.55484038951926,
72.3375789131369));
#223124=CARTESIAN_POINT('Ctrl Pts',(-7.90033749776537,0.412362324693237,
72.3433504849001));
#223125=CARTESIAN_POINT('Ctrl Pts',(-7.90223349597277,0.37427404171455,
72.3448898318507));
#223126=CARTESIAN_POINT('Ctrl Pts',(-7.90481343563123,0.31361646145783,
72.347336013787));
#223127=CARTESIAN_POINT('Ctrl Pts',(-7.90567628115004,0.291055455714753,
72.3482446799303));
#223128=CARTESIAN_POINT('Ctrl Pts',(-7.90721753802288,0.245668989415847,
72.3500704149669));
#223129=CARTESIAN_POINT('Ctrl Pts',(-7.90789372403584,0.222843664899516,
72.3509874527183));
#223130=CARTESIAN_POINT('Ctrl Pts',(-7.90905917344906,0.176762665795935,
72.3528366219436));
#223131=CARTESIAN_POINT('Ctrl Pts',(-7.90954471620337,0.153507118007278,
72.3537687074326));
#223132=CARTESIAN_POINT('Ctrl Pts',(-7.91064206092113,0.0868665379281315,
72.3564366156031));
#223133=CARTESIAN_POINT('Ctrl Pts',(-7.91099951148764,0.0434781555137821,
72.3581699259418));
#223134=CARTESIAN_POINT('Ctrl Pts',(-7.91099999949962,8.89775508417708E-5,
72.3598999971));
#223135=CARTESIAN_POINT('',(-7.911,-5.26911847487099E-12,74.3576684917632));
#223136=CARTESIAN_POINT('Ctrl Pts',(-7.911,-5.21527265817667E-12,72.3576684917632));
#223137=CARTESIAN_POINT('Ctrl Pts',(-7.91099999999855,-2.20167589667201,
72.446255927496));
#223138=CARTESIAN_POINT('Ctrl Pts',(-6.94214576672079,-4.38610418339146,
72.5348433632287));
#223139=CARTESIAN_POINT('Ctrl Pts',(-3.67820201487792,-7.34180684107881,
72.7120182346941));
#223140=CARTESIAN_POINT('Ctrl Pts',(-1.40868175871195,-8.08992666571433,
72.8006056704269));
#223141=CARTESIAN_POINT('Ctrl Pts',(2.97309270521799,-7.65454228025054,
72.9777805418923));
#223142=CARTESIAN_POINT('Ctrl Pts',(5.05102072676049,-6.47444880833878,
73.066367977625));
#223143=CARTESIAN_POINT('Ctrl Pts',(7.66951518848077,-2.93425195367174,
73.2435428490905));
#223144=CARTESIAN_POINT('Ctrl Pts',(8.18956872247114,-0.601881960093438,
73.3321302848232));
#223145=CARTESIAN_POINT('Ctrl Pts',(7.32306689761081,3.71537198232967,73.5093051562887));
#223146=CARTESIAN_POINT('Ctrl Pts',(5.943299588498,5.66643518936933,73.5978925920214));
#223147=CARTESIAN_POINT('Ctrl Pts',(2.1615450163728,7.92205913233153,73.7750674634868));
#223148=CARTESIAN_POINT('Ctrl Pts',(-0.210816529306286,8.20894963712988,
73.8636548992196));
#223149=CARTESIAN_POINT('Ctrl Pts',(-4.42123908576941,6.9198224471751,74.040829770685));
#223150=CARTESIAN_POINT('Ctrl Pts',(-6.2263162563458,5.35390358803066,74.1294172064178));
#223151=CARTESIAN_POINT('Ctrl Pts',(-7.65317280859651,2.31334857513973,
74.2645592586881));
#223152=CARTESIAN_POINT('Ctrl Pts',(-7.91100000000077,1.15702837835974,
74.3111138752257));
#223153=CARTESIAN_POINT('Ctrl Pts',(-7.911,-5.26911847487099E-12,74.3576684917632));
#223154=CARTESIAN_POINT('',(-7.911,-4.92828000631107E-12,78.3576684917632));
#223155=CARTESIAN_POINT('Ctrl Pts',(-7.91099999987772,4.39868550092259E-5,
74.3589457483061));
#223156=CARTESIAN_POINT('Ctrl Pts',(-7.91100255781545,-0.459999029859075,
74.37478896162));
#223157=CARTESIAN_POINT('Ctrl Pts',(-7.87087669527066,-0.919148178927294,
74.3902122431434));
#223158=CARTESIAN_POINT('Ctrl Pts',(-7.75556910623801,-1.57384771154762,
74.4143390289438));
#223159=CARTESIAN_POINT('Ctrl Pts',(-7.71223846080161,-1.77403948953629,
74.422021749972));
#223160=CARTESIAN_POINT('Ctrl Pts',(-7.65405480674869,-2.00004655857829,
74.4312663779502));
#223161=CARTESIAN_POINT('Ctrl Pts',(-7.64676414644965,-2.02774240737943,
74.4324091659388));
#223162=CARTESIAN_POINT('Ctrl Pts',(-7.63738158098275,-2.06261470997046,
74.4338612661042));
#223163=CARTESIAN_POINT('Ctrl Pts',(-7.63542959584612,-2.06982891599108,
74.4341623830335));
#223164=CARTESIAN_POINT('Ctrl Pts',(-7.63230658350073,-2.08130650391784,
74.434642602861));
#223165=CARTESIAN_POINT('Ctrl Pts',(-7.63114219597235,-2.08557170399325,
74.4348213112727));
#223166=CARTESIAN_POINT('Ctrl Pts',(-7.62893900387383,-2.09361554074054,
74.435158823249));
#223167=CARTESIAN_POINT('Ctrl Pts',(-7.62790096985216,-2.09739437188012,
74.4353175805888));
#223168=CARTESIAN_POINT('Ctrl Pts',(-7.62554061076717,-2.10596203074823,
74.4356779824742));
#223169=CARTESIAN_POINT('Ctrl Pts',(-7.62421658422282,-2.1107503779696,
74.4358797283332));
#223170=CARTESIAN_POINT('Ctrl Pts',(-7.62079555479545,-2.12307732786204,
74.4363999193981));
#223171=CARTESIAN_POINT('Ctrl Pts',(-7.61869188086996,-2.13061405504613,
74.4367187592679));
#223172=CARTESIAN_POINT('Ctrl Pts',(-7.60630760249972,-2.17472972287422,
74.4385896606587));
#223173=CARTESIAN_POINT('Ctrl Pts',(-7.59577491134693,-2.21123678406558,
74.440156402358));
#223174=CARTESIAN_POINT('Ctrl Pts',(-7.40284776344447,-2.86228927489958,
74.4684098051805));
#223175=CARTESIAN_POINT('Ctrl Pts',(-7.14669633365192,-3.45246665168654,
74.4988232229369));
#223176=CARTESIAN_POINT('Ctrl Pts',(-6.77221950229717,-4.0903175426112,
74.5328593659256));
#223177=CARTESIAN_POINT('Ctrl Pts',(-6.72068200122676,-4.17445666937669,
74.5373797254462));
#223178=CARTESIAN_POINT('Ctrl Pts',(-6.61604537604343,-4.3383216824764,
74.5462276282956));
#223179=CARTESIAN_POINT('Ctrl Pts',(-6.56304510840782,-4.41809132188313,
74.5505562222393));
#223180=CARTESIAN_POINT('Ctrl Pts',(-6.3492767697925,-4.72749125692134,
74.5674067966865));
#223181=CARTESIAN_POINT('Ctrl Pts',(-6.17779273714898,-4.94948342987304,
74.5796228457744));
#223182=CARTESIAN_POINT('Ctrl Pts',(-5.911662629768,-5.25855769531768,74.5967279283866));
#223183=CARTESIAN_POINT('Ctrl Pts',(-5.82612465619924,-5.35317266712475,
74.6019804187158));
#223184=CARTESIAN_POINT('Ctrl Pts',(-5.72900440892965,-5.45551218153069,
74.607683425037));
#223185=CARTESIAN_POINT('Ctrl Pts',(-5.71964976374926,-5.46531895343892,
74.6082301523073));
#223186=CARTESIAN_POINT('Ctrl Pts',(-5.70213029593801,-5.48359092285748,
74.6092492619851));
#223187=CARTESIAN_POINT('Ctrl Pts',(-5.69397171556912,-5.49206203761088,
74.6097219150718));
#223188=CARTESIAN_POINT('Ctrl Pts',(-5.6805051471627,-5.50598221379641,
74.6104989106774));
#223189=CARTESIAN_POINT('Ctrl Pts',(-5.6752081502598,-5.51144185465401,
74.6108037348877));
#223190=CARTESIAN_POINT('Ctrl Pts',(-5.66490037473644,-5.52203551328437,
74.611395358321));
#223191=CARTESIAN_POINT('Ctrl Pts',(-5.65989047218949,-5.52717037088918,
74.6116821955945));
#223192=CARTESIAN_POINT('Ctrl Pts',(-5.64826694583571,-5.5390514313789,
74.6123460494215));
#223193=CARTESIAN_POINT('Ctrl Pts',(-5.64164820239469,-5.54579262252948,
74.6127228393201));
#223194=CARTESIAN_POINT('Ctrl Pts',(-5.62025410432703,-5.56750457891165,
74.6139368180659));
#223195=CARTESIAN_POINT('Ctrl Pts',(-5.60543105633025,-5.58242833495877,
74.6147718916182));
#223196=CARTESIAN_POINT('Ctrl Pts',(-5.46659889325157,-5.72109321662509,
74.622537401475));
#223197=CARTESIAN_POINT('Ctrl Pts',(-5.33856726614387,-5.84074612380135,
74.6292841902116));
#223198=CARTESIAN_POINT('Ctrl Pts',(-4.91547034767126,-6.2106089416447,
74.6503990477461));
#223199=CARTESIAN_POINT('Ctrl Pts',(-4.60599155065285,-6.44347577305572,
74.664073811501));
#223200=CARTESIAN_POINT('Ctrl Pts',(-4.08188854207762,-6.78070807296753,
74.6856549478911));
#223201=CARTESIAN_POINT('Ctrl Pts',(-3.87743546093855,-6.89966012133398,
74.6937350477193));
#223202=CARTESIAN_POINT('Ctrl Pts',(-3.43081695122265,-7.13337612355974,
74.7111755778941));
#223203=CARTESIAN_POINT('Ctrl Pts',(-3.18753496248547,-7.24535496022746,
74.720552883012));
#223204=CARTESIAN_POINT('Ctrl Pts',(-2.78789572095369,-7.40527295776753,
74.7364073513357));
#223205=CARTESIAN_POINT('Ctrl Pts',(-2.63490896036442,-7.46107763215647,
74.7425794297122));
#223206=CARTESIAN_POINT('Ctrl Pts',(-2.44992900290924,-7.5221534847238,
74.7502804100549));
#223207=CARTESIAN_POINT('Ctrl Pts',(-2.41947978599846,-7.53200256763053,
74.7515556753191));
#223208=CARTESIAN_POINT('Ctrl Pts',(-2.38150194279796,-7.54403280071772,
74.7531566545599));
#223209=CARTESIAN_POINT('Ctrl Pts',(-2.37402833663229,-7.54638800080179,
74.7534722093428));
#223210=CARTESIAN_POINT('Ctrl Pts',(-2.36216191967191,-7.55010815981622,
74.7539740495719));
#223211=CARTESIAN_POINT('Ctrl Pts',(-2.35777141050801,-7.55148039362454,
74.7541599027669));
#223212=CARTESIAN_POINT('Ctrl Pts',(-2.3494894962841,-7.55406094163649,
74.7545108083172));
#223213=CARTESIAN_POINT('Ctrl Pts',(-2.34559834772306,-7.55527008082113,
74.7546758125245));
#223214=CARTESIAN_POINT('Ctrl Pts',(-2.3368372213771,-7.55798510088525,
74.7550476310431));
#223215=CARTESIAN_POINT('Ctrl Pts',(-2.33196672249307,-7.55948928099117,
74.7552545434696));
#223216=CARTESIAN_POINT('Ctrl Pts',(-2.31955290473075,-7.56330996258342,
74.7557824470207));
#223217=CARTESIAN_POINT('Ctrl Pts',(-2.31200758376753,-7.56561988205167,
74.7561038135544));
#223218=CARTESIAN_POINT('Ctrl Pts',(-2.26993121056785,-7.57843229148842,
74.7578986330891));
#223219=CARTESIAN_POINT('Ctrl Pts',(-2.23533252576648,-7.58870951617319,
74.7593847002442));
#223220=CARTESIAN_POINT('Ctrl Pts',(-1.62050637068699,-7.76676862332133,
74.7859576510475));
#223221=CARTESIAN_POINT('Ctrl Pts',(-1.02304451363722,-7.86778569835948,
74.814236618596));
#223222=CARTESIAN_POINT('Ctrl Pts',(-0.0659459552973449,-7.91866435171381,
74.8580827739364));
#223223=CARTESIAN_POINT('Ctrl Pts',(0.288942814869212,-7.91366777144239,
74.8740599113042));
#223224=CARTESIAN_POINT('Ctrl Pts',(0.894844434015389,-7.86430962641148,
74.9003569623192));
#223225=CARTESIAN_POINT('Ctrl Pts',(1.1462463730478,-7.83161841484737,74.9109813593004));
#223226=CARTESIAN_POINT('Ctrl Pts',(1.4156646610637,-7.78333010412937,74.9220525573507));
#223227=CARTESIAN_POINT('Ctrl Pts',(1.43565311544551,-7.77966799307198,
74.9228721011929));
#223228=CARTESIAN_POINT('Ctrl Pts',(1.46515615226902,-7.77414512532751,
74.924079063536));
#223229=CARTESIAN_POINT('Ctrl Pts',(1.47468170510054,-7.77234384530687,
74.924468337338));
#223230=CARTESIAN_POINT('Ctrl Pts',(1.49143149282617,-7.76914456329789,
74.9251521144648));
#223231=CARTESIAN_POINT('Ctrl Pts',(1.49865712356671,-7.76775398487626,
74.925446849356));
#223232=CARTESIAN_POINT('Ctrl Pts',(1.51271076223718,-7.76502901165071,
74.9260196408041));
#223233=CARTESIAN_POINT('Ctrl Pts',(1.51953896971166,-7.76369568709483,
74.9262977305323));
#223234=CARTESIAN_POINT('Ctrl Pts',(1.53777219721394,-7.76011036100972,
74.9270397471734));
#223235=CARTESIAN_POINT('Ctrl Pts',(1.54917404631814,-7.75784222069808,
74.9275031686034));
#223236=CARTESIAN_POINT('Ctrl Pts',(1.59017377593742,-7.74959225866892,
74.9291674878776));
#223237=CARTESIAN_POINT('Ctrl Pts',(1.61974251569416,-7.74346608574651,
74.9303638605007));
#223238=CARTESIAN_POINT('Ctrl Pts',(2.09173180150072,-7.64285560803748,
74.9493998775935));
#223239=CARTESIAN_POINT('Ctrl Pts',(2.52529576691775,-7.51076034656274,
74.9659577279597));
#223240=CARTESIAN_POINT('Ctrl Pts',(3.22649636901077,-7.22948705169856,
74.9925398244361));
#223241=CARTESIAN_POINT('Ctrl Pts',(3.50105071584739,-7.10059206025086,
75.0029127712537));
#223242=CARTESIAN_POINT('Ctrl Pts',(4.03248942627739,-6.81276339169449,
75.0238089169988));
#223243=CARTESIAN_POINT('Ctrl Pts',(4.28902032581565,-6.65424709862905,
75.0343167711192));
#223244=CARTESIAN_POINT('Ctrl Pts',(4.67717872089305,-6.3826065876698,75.0517723991173));
#223245=CARTESIAN_POINT('Ctrl Pts',(4.81520633394387,-6.27912805811054,
75.0583185506745));
#223246=CARTESIAN_POINT('Ctrl Pts',(4.97021192529077,-6.15480328849698,
75.0662010274249));
#223247=CARTESIAN_POINT('Ctrl Pts',(4.9906075725137,-6.13827713045954,75.0672491692675));
#223248=CARTESIAN_POINT('Ctrl Pts',(5.01663804408551,-6.11696970166405,
75.0686015168016));
#223249=CARTESIAN_POINT('Ctrl Pts',(5.02234913894389,-6.1122814662213,75.0688991305419));
#223250=CARTESIAN_POINT('Ctrl Pts',(5.03151651934753,-6.10473444419738,
75.069378332311));
#223251=CARTESIAN_POINT('Ctrl Pts',(5.03497696746959,-6.10188069823834,
75.0695595573356));
#223252=CARTESIAN_POINT('Ctrl Pts',(5.04154624502855,-6.09645378439796,
75.0699042409071));
#223253=CARTESIAN_POINT('Ctrl Pts',(5.04465553739504,-6.09388117663758,
75.0700676587275));
#223254=CARTESIAN_POINT('Ctrl Pts',(5.05171530255322,-6.08803086815133,
75.070439336512));
#223255=CARTESIAN_POINT('Ctrl Pts',(5.05566455297499,-6.08475170217899,
75.0706477039822));
#223256=CARTESIAN_POINT('Ctrl Pts',(5.06773675797528,-6.07470796778211,
75.0712860359159));
#223257=CARTESIAN_POINT('Ctrl Pts',(5.07584927910152,-6.06793101757252,
75.0717169236208));
#223258=CARTESIAN_POINT('Ctrl Pts',(5.13758427735328,-6.01614906913351,
75.075010472847));
#223259=CARTESIAN_POINT('Ctrl Pts',(5.19061938504279,-5.97045154659893,
75.0779237779166));
#223260=CARTESIAN_POINT('Ctrl Pts',(5.59905548075049,-5.60896846508895,
75.1009689887324));
#223261=CARTESIAN_POINT('Ctrl Pts',(5.92592111326226,-5.26244732300141,
75.1230039316853));
#223262=CARTESIAN_POINT('Ctrl Pts',(6.39763600440487,-4.66230657695339,
75.1582869219465));
#223263=CARTESIAN_POINT('Ctrl Pts',(6.56310353028825,-4.42634526081582,
75.1715615034023));
#223264=CARTESIAN_POINT('Ctrl Pts',(6.87847552078114,-3.91991507693336,
75.1983872471724));
#223265=CARTESIAN_POINT('Ctrl Pts',(7.0261515530736,-3.6486136016874,75.2118644934768));
#223266=CARTESIAN_POINT('Ctrl Pts',(7.20953427929696,-3.25904899450842,
75.2298744374987));
#223267=CARTESIAN_POINT('Ctrl Pts',(7.25890441416499,-3.14755355400882,
75.2348852948041));
#223268=CARTESIAN_POINT('Ctrl Pts',(7.31224406567963,-3.01915559934486,
75.2404964122261));
#223269=CARTESIAN_POINT('Ctrl Pts',(7.31875748479892,-3.00333193182822,
75.2411852039126));
#223270=CARTESIAN_POINT('Ctrl Pts',(7.32851703815783,-2.97940183055967,
75.242222783988));
#223271=CARTESIAN_POINT('Ctrl Pts',(7.33180115527293,-2.97131100134406,
75.242572890325));
#223272=CARTESIAN_POINT('Ctrl Pts',(7.33743021191441,-2.95737696727229,
75.2431746397299));
#223273=CARTESIAN_POINT('Ctrl Pts',(7.33978158023324,-2.95153637889914,
75.2434265054638));
#223274=CARTESIAN_POINT('Ctrl Pts',(7.34461312728542,-2.93949377046904,
75.2439450760217));
#223275=CARTESIAN_POINT('Ctrl Pts',(7.3470924292694,-2.93329140253549,75.2442117503577));
#223276=CARTESIAN_POINT('Ctrl Pts',(7.35375179750237,-2.91657052244639,
75.2449295786337));
#223277=CARTESIAN_POINT('Ctrl Pts',(7.35791715731509,-2.90604614883611,
75.2453802237446));
#223278=CARTESIAN_POINT('Ctrl Pts',(7.3731352263746,-2.86735305974536,75.2470327671426));
#223279=CARTESIAN_POINT('Ctrl Pts',(7.38404894492617,-2.83912976822201,
75.2482298670331));
#223280=CARTESIAN_POINT('Ctrl Pts',(7.55501982078598,-2.38933768778958,
75.2671782273451));
#223281=CARTESIAN_POINT('Ctrl Pts',(7.67891604551075,-1.95488237722311,
75.2836011282009));
#223282=CARTESIAN_POINT('Ctrl Pts',(7.8691786430854,-0.977889573176178,
75.3183638326138));
#223283=CARTESIAN_POINT('Ctrl Pts',(7.91780052232114,-0.434299729356681,
75.3362857174874));
#223284=CARTESIAN_POINT('Ctrl Pts',(7.90695354038161,0.346105018583208,
75.3642587005676));
#223285=CARTESIAN_POINT('Ctrl Pts',(7.89309717197793,0.58198291796844,75.3730263858001));
#223286=CARTESIAN_POINT('Ctrl Pts',(7.86558100841814,0.84703983716694,75.3835743083525));
#223287=CARTESIAN_POINT('Ctrl Pts',(7.8622754531318,0.877191961548501,75.3847844476465));
#223288=CARTESIAN_POINT('Ctrl Pts',(7.85793372159408,0.914797918671408,
75.3863073499697));
#223289=CARTESIAN_POINT('Ctrl Pts',(7.85706016727825,0.922270639228235,
75.3866106388035));
#223290=CARTESIAN_POINT('Ctrl Pts',(7.85566133366451,0.934090565715141,
75.3870914419696));
#223291=CARTESIAN_POINT('Ctrl Pts',(7.85514310086212,0.938438617607111,
75.3872685400263));
#223292=CARTESIAN_POINT('Ctrl Pts',(7.85416544655165,0.946583734814029,
75.3876007305111));
#223293=CARTESIAN_POINT('Ctrl Pts',(7.85370688063013,0.950380903565148,
75.3877557719475));
#223294=CARTESIAN_POINT('Ctrl Pts',(7.85267688791865,0.958858135240187,
75.3881023038262));
#223295=CARTESIAN_POINT('Ctrl Pts',(7.85210403098808,0.963538019969806,
75.3882938800158));
#223296=CARTESIAN_POINT('Ctrl Pts',(7.85064008321831,0.975409553846123,
75.3887805508474));
#223297=CARTESIAN_POINT('Ctrl Pts',(7.84974329562271,0.982600481423201,
75.3890759899834));
#223298=CARTESIAN_POINT('Ctrl Pts',(7.84467859607688,1.02276252953264,75.3907296305616));
#223299=CARTESIAN_POINT('Ctrl Pts',(7.84031289116645,1.05570790017319,75.3920996244686));
#223300=CARTESIAN_POINT('Ctrl Pts',(7.76585879186209,1.5916163440472,75.4145931992722));
#223301=CARTESIAN_POINT('Ctrl Pts',(7.64771406160099,2.08666720844628,75.4383037912463));
#223302=CARTESIAN_POINT('Ctrl Pts',(7.33381503755783,3.00172930986357,75.4836730363999));
#223303=CARTESIAN_POINT('Ctrl Pts',(7.14703653488529,3.42274068644863,75.505218539365));
#223304=CARTESIAN_POINT('Ctrl Pts',(6.80754038572666,4.03733386179259,75.5364445360822));
#223305=CARTESIAN_POINT('Ctrl Pts',(6.68064724138917,4.24401195603253,75.5469167386318));
#223306=CARTESIAN_POINT('Ctrl Pts',(6.48440906132903,4.53296624502326,75.5614847608781));
#223307=CARTESIAN_POINT('Ctrl Pts',(6.42257605008965,4.62015822003535,75.5658714605769));
#223308=CARTESIAN_POINT('Ctrl Pts',(6.34925266620873,4.71923507611359,75.5708484396384));
#223309=CARTESIAN_POINT('Ctrl Pts',(6.33947099281746,4.73236691927049,75.5715079454101));
#223310=CARTESIAN_POINT('Ctrl Pts',(6.32458222021835,4.75222601247567,75.572505097304));
#223311=CARTESIAN_POINT('Ctrl Pts',(6.31950503337093,4.75897556914844,75.5728439649213));
#223312=CARTESIAN_POINT('Ctrl Pts',(6.31069985741217,4.77064213540199,75.5734296357372));
#223313=CARTESIAN_POINT('Ctrl Pts',(6.30697691176529,4.77556293112161,75.5736766451168));
#223314=CARTESIAN_POINT('Ctrl Pts',(6.29924643047442,4.7857558717302,75.574188264207));
#223315=CARTESIAN_POINT('Ctrl Pts',(6.29523802341134,4.79102735167879,75.5744528378765));
#223316=CARTESIAN_POINT('Ctrl Pts',(6.28430418546764,4.80536909460649,75.5751725928584));
#223317=CARTESIAN_POINT('Ctrl Pts',(6.27736572742716,4.81442943207951,75.575627238457));
#223318=CARTESIAN_POINT('Ctrl Pts',(6.25113068697281,4.84853438906449,75.5773384269291));
#223319=CARTESIAN_POINT('Ctrl Pts',(6.23170350806327,4.87347842981928,75.5785895844747));
#223320=CARTESIAN_POINT('Ctrl Pts',(5.91404250680955,5.27634234293237,75.5987927249157));
#223321=CARTESIAN_POINT('Ctrl Pts',(5.58205684864035,5.62640150080307,75.6162025471674));
#223322=CARTESIAN_POINT('Ctrl Pts',(4.81354129420974,6.30133103701195,75.6517718893306));
#223323=CARTESIAN_POINT('Ctrl Pts',(4.37124324603791,6.61582356277707,75.6696674322865));
#223324=CARTESIAN_POINT('Ctrl Pts',(3.83207786166765,6.92136225548355,75.692128373699));
#223325=CARTESIAN_POINT('Ctrl Pts',(3.76325045477522,6.9590244822036,75.6950086347324));
#223326=CARTESIAN_POINT('Ctrl Pts',(3.56871966367596,7.06174144766385,75.7032150282966));
#223327=CARTESIAN_POINT('Ctrl Pts',(3.44182090656361,7.12445230916788,75.7086516062201));
#223328=CARTESIAN_POINT('Ctrl Pts',(3.28839927274547,7.19521391395797,75.7153664478632));
#223329=CARTESIAN_POINT('Ctrl Pts',(3.26343759394008,7.20656978650558,75.7164627628123));
#223330=CARTESIAN_POINT('Ctrl Pts',(3.23007575052749,7.22153828769013,75.7179326562098));
#223331=CARTESIAN_POINT('Ctrl Pts',(3.22172743809201,7.22526656313712,75.7183008617681));
#223332=CARTESIAN_POINT('Ctrl Pts',(3.20796120529136,7.2313858267981,75.7189086434657));
#223333=CARTESIAN_POINT('Ctrl Pts',(3.20254701560521,7.23378522512571,75.719147837824));
#223334=CARTESIAN_POINT('Ctrl Pts',(3.1920159849293,7.23843810585262,75.719613388622));
#223335=CARTESIAN_POINT('Ctrl Pts',(3.18689943780378,7.2406922482185,75.7198397153873));
#223336=CARTESIAN_POINT('Ctrl Pts',(3.17503066156771,7.24590613041933,75.7203650331848));
#223337=CARTESIAN_POINT('Ctrl Pts',(3.16827668247244,7.24886185656421,75.7206642007303));
#223338=CARTESIAN_POINT('Ctrl Pts',(3.15003583670891,7.2568141868062,75.7214727916144));
#223339=CARTESIAN_POINT('Ctrl Pts',(3.13854124572396,7.26179294395677,75.7219829853023));
#223340=CARTESIAN_POINT('Ctrl Pts',(3.05436751965186,7.29801469167306,75.725723649837));
#223341=CARTESIAN_POINT('Ctrl Pts',(2.98123666457522,7.32819260095663,75.7289984183885));
#223342=CARTESIAN_POINT('Ctrl Pts',(2.5603640999454,7.49452572160723,75.7479446882151));
#223343=CARTESIAN_POINT('Ctrl Pts',(2.20379043847942,7.60701429817823,75.7643609285011));
#223344=CARTESIAN_POINT('Ctrl Pts',(1.45210967108439,7.78684024587518,75.7984382403976));
#223345=CARTESIAN_POINT('Ctrl Pts',(1.05709777199716,7.85022740945161,75.8160481073981));
#223346=CARTESIAN_POINT('Ctrl Pts',(0.311821299954308,7.91252487273128,
75.8480919422494));
#223347=CARTESIAN_POINT('Ctrl Pts',(-0.036888965241275,7.91858232233994,
75.8626157436356));
#223348=CARTESIAN_POINT('Ctrl Pts',(-0.418191306487795,7.90000944545624,
75.8780611293533));
#223349=CARTESIAN_POINT('Ctrl Pts',(-0.451491186756857,7.89817630458115,
75.8794065728138));
#223350=CARTESIAN_POINT('Ctrl Pts',(-0.500338698918058,7.89517733904263,
75.8813751336046));
#223351=CARTESIAN_POINT('Ctrl Pts',(-0.515895951624096,7.89417604299847,
75.8820013382166));
#223352=CARTESIAN_POINT('Ctrl Pts',(-0.543326737103672,7.89232910799169,
75.8831041402679));
#223353=CARTESIAN_POINT('Ctrl Pts',(-0.55520149641962,7.89150264470963,
75.8835811019236));
#223354=CARTESIAN_POINT('Ctrl Pts',(-0.578360075786323,7.88983831569531,
75.8845104315158));
#223355=CARTESIAN_POINT('Ctrl Pts',(-0.589644051186677,7.88900303706528,
75.8849628481302));
#223356=CARTESIAN_POINT('Ctrl Pts',(-0.616761448128302,7.8869372081937,
75.8860491317093));
#223357=CARTESIAN_POINT('Ctrl Pts',(-0.632593049729356,7.88568318192396,
75.8866825406924));
#223358=CARTESIAN_POINT('Ctrl Pts',(-0.681072129444093,7.88169620540049,
75.8886197617215));
#223359=CARTESIAN_POINT('Ctrl Pts',(-0.713706611554314,7.87880810866663,
75.8899205161509));
#223360=CARTESIAN_POINT('Ctrl Pts',(-1.29653564927582,7.82357779374865,
75.9130926152636));
#223361=CARTESIAN_POINT('Ctrl Pts',(-1.83977467643434,7.71392621406561,
75.9335912899948));
#223362=CARTESIAN_POINT('Ctrl Pts',(-2.82901299981564,7.40370678258994,
75.9712776094163));
#223363=CARTESIAN_POINT('Ctrl Pts',(-3.27655092009862,7.21680961232943,
75.9885280548554));
#223364=CARTESIAN_POINT('Ctrl Pts',(-3.79013207565515,6.94465867842439,
76.010989865121));
#223365=CARTESIAN_POINT('Ctrl Pts',(-3.87524358373726,6.89752647135095,
76.0148089468064));
#223366=CARTESIAN_POINT('Ctrl Pts',(-3.97045560350569,6.84248233912221,
76.0192143673533));
#223367=CARTESIAN_POINT('Ctrl Pts',(-3.98143408405275,6.83610012303953,
76.0197243660112));
#223368=CARTESIAN_POINT('Ctrl Pts',(-3.99789160910994,6.82647963357907,
76.0204920091297));
#223369=CARTESIAN_POINT('Ctrl Pts',(-4.00338222494194,6.82326111668929,
76.0207486354436));
#223370=CARTESIAN_POINT('Ctrl Pts',(-4.01281331276942,6.81771745165045,
76.0211903446315));
#223371=CARTESIAN_POINT('Ctrl Pts',(-4.01675566873945,6.81539550071784,
76.0213752600788));
#223372=CARTESIAN_POINT('Ctrl Pts',(-4.02486561051468,6.81060946302465,
76.0217562228724));
#223373=CARTESIAN_POINT('Ctrl Pts',(-4.02903295301425,6.80814496789887,
76.0219522918301));
#223374=CARTESIAN_POINT('Ctrl Pts',(-4.03904981571421,6.80220874834244,
76.022424323896));
#223375=CARTESIAN_POINT('Ctrl Pts',(-4.04489711795348,6.79873330662017,
76.022700486178));
#223376=CARTESIAN_POINT('Ctrl Pts',(-4.06277954751779,6.78807335037843,
76.023546962586));
#223377=CARTESIAN_POINT('Ctrl Pts',(-4.0748000218748,6.78086441683733,76.0241186072022));
#223378=CARTESIAN_POINT('Ctrl Pts',(-4.24886322457027,6.67584504340291,
76.0324357076554));
#223379=CARTESIAN_POINT('Ctrl Pts',(-4.40734466036384,6.57229355039865,
76.040523721009));
#223380=CARTESIAN_POINT('Ctrl Pts',(-5.08269097375305,6.09560933702818,
76.0768429640418));
#223381=CARTESIAN_POINT('Ctrl Pts',(-5.55710617108765,5.66646282998117,
76.1070903356604));
#223382=CARTESIAN_POINT('Ctrl Pts',(-6.29080110260823,4.82100271446624,
76.1577224931605));
#223383=CARTESIAN_POINT('Ctrl Pts',(-6.57281247981719,4.42882411785305,
76.1786422200377));
#223384=CARTESIAN_POINT('Ctrl Pts',(-6.82876344676009,3.99404722670944,
76.1990994496335));
#223385=CARTESIAN_POINT('Ctrl Pts',(-6.84005312966079,3.97468195643466,
76.2000054819511));
#223386=CARTESIAN_POINT('Ctrl Pts',(-6.85631832285003,3.94650762036242,
76.2013162531928));
#223387=CARTESIAN_POINT('Ctrl Pts',(-6.86135943564066,3.93773666434462,
76.2017232728102));
#223388=CARTESIAN_POINT('Ctrl Pts',(-6.8701398821569,3.92239164282142,76.2024335602847));
#223389=CARTESIAN_POINT('Ctrl Pts',(-6.87388663310417,3.91582184933087,
76.202737085282));
#223390=CARTESIAN_POINT('Ctrl Pts',(-6.88111604814793,3.90310297989199,
76.2033235868195));
#223391=CARTESIAN_POINT('Ctrl Pts',(-6.88459990434437,3.89695459264327,
76.2036066044646));
#223392=CARTESIAN_POINT('Ctrl Pts',(-6.89285420439953,3.88234160309588,
76.2042780714797));
#223393=CARTESIAN_POINT('Ctrl Pts',(-6.89761730684863,3.87387285482698,
76.2046662668753));
#223394=CARTESIAN_POINT('Ctrl Pts',(-6.91436963448022,3.84395853386793,
76.2060341819681));
#223395=CARTESIAN_POINT('Ctrl Pts',(-6.9262745983675,3.82246580805148,76.2070109952575));
#223396=CARTESIAN_POINT('Ctrl Pts',(-7.08132887761979,3.53943446423079,
76.2197964999699));
#223397=CARTESIAN_POINT('Ctrl Pts',(-7.20968786287085,3.27005139364672,
76.2310826461926));
#223398=CARTESIAN_POINT('Ctrl Pts',(-7.60372995609988,2.30634264731731,
76.26910644646));
#223399=CARTESIAN_POINT('Ctrl Pts',(-7.78661998319807,1.58251926277892,
76.2933044448404));
#223400=CARTESIAN_POINT('Ctrl Pts',(-7.87693674838221,0.740650574163553,
76.3237888080469));
#223401=CARTESIAN_POINT('Ctrl Pts',(-7.88597654076273,0.637235325388901,
76.3275787382517));
#223402=CARTESIAN_POINT('Ctrl Pts',(-7.89901085438058,0.44445949053502,
76.3347678943308));
#223403=CARTESIAN_POINT('Ctrl Pts',(-7.90352983378602,0.355150785214006,
76.3381480019443));
#223404=CARTESIAN_POINT('Ctrl Pts',(-7.9095138143717,0.17714151986588,76.3450117027852));
#223405=CARTESIAN_POINT('Ctrl Pts',(-7.91100253418007,0.0884597651576268,
76.3484973308441));
#223406=CARTESIAN_POINT('Ctrl Pts',(-7.91099963220847,-0.0129679707314106,
76.3525525794503));
#223407=CARTESIAN_POINT('Ctrl Pts',(-7.91096848474549,-0.0257095316003968,
76.35306321325));
#223408=CARTESIAN_POINT('Ctrl Pts',(-7.91086865393941,-0.0462487621033094,
76.3538882358912));
#223409=CARTESIAN_POINT('Ctrl Pts',(-7.91081922303907,-0.0540465330244665,
76.354201896431));
#223410=CARTESIAN_POINT('Ctrl Pts',(-7.91071069604874,-0.067928688127151,
76.3547610646232));
#223411=CARTESIAN_POINT('Ctrl Pts',(-7.91065610950113,-0.0740131083675887,
76.3550064052051));
#223412=CARTESIAN_POINT('Ctrl Pts',(-7.91052752954996,-0.0867119379314251,
76.3555189968786));
#223413=CARTESIAN_POINT('Ctrl Pts',(-7.91045225964427,-0.0933263281004106,
76.3557862942395));
#223414=CARTESIAN_POINT('Ctrl Pts',(-7.91023509872252,-0.110514766928626,
76.3564816870029));
#223415=CARTESIAN_POINT('Ctrl Pts',(-7.91008030144159,-0.121088621421877,
76.3569102429269));
#223416=CARTESIAN_POINT('Ctrl Pts',(-7.9093267462546,-0.16636018607024,
76.3587483026548));
#223417=CARTESIAN_POINT('Ctrl Pts',(-7.90852088699473,-0.201053793574192,
76.3601649702217));
#223418=CARTESIAN_POINT('Ctrl Pts',(-7.90072335247937,-0.462607747035005,
76.3709011970511));
#223419=CARTESIAN_POINT('Ctrl Pts',(-7.88419992786868,-0.689071620868773,
76.3805108104684));
#223420=CARTESIAN_POINT('Ctrl Pts',(-7.80478393924574,-1.37146263479148,
76.4099505587532));
#223421=CARTESIAN_POINT('Ctrl Pts',(-7.71184492116253,-1.82291744877112,
76.4300212318081));
#223422=CARTESIAN_POINT('Ctrl Pts',(-7.41133833433478,-2.82917047643946,
76.4748148886292));
#223423=CARTESIAN_POINT('Ctrl Pts',(-7.17974367895566,-3.37393875914322,
76.4990761601005));
#223424=CARTESIAN_POINT('Ctrl Pts',(-6.8485465187623,-3.96085219546914,
76.5264408298348));
#223425=CARTESIAN_POINT('Ctrl Pts',(-6.80621757084358,-4.03315534669668,
76.529833181467));
#223426=CARTESIAN_POINT('Ctrl Pts',(-6.74648707499715,-4.13156329880377,
76.5344796399074));
#223427=CARTESIAN_POINT('Ctrl Pts',(-6.73006705451193,-4.15825691785126,
76.5357430339251));
#223428=CARTESIAN_POINT('Ctrl Pts',(-6.70159787450962,-4.20392818823517,
76.5379098688576));
#223429=CARTESIAN_POINT('Ctrl Pts',(-6.68962566393961,-4.22295332236366,
76.5388140760126));
#223430=CARTESIAN_POINT('Ctrl Pts',(-6.66476013538056,-4.26209623127658,
76.5406777035256));
#223431=CARTESIAN_POINT('Ctrl Pts',(-6.65185642691635,-4.28220714424607,
76.541637004512));
#223432=CARTESIAN_POINT('Ctrl Pts',(-6.6215138713567,-4.32902906210366,
76.5438747000131));
#223433=CARTESIAN_POINT('Ctrl Pts',(-6.6040041678896,-4.35569369086335,
76.545152310807));
#223434=CARTESIAN_POINT('Ctrl Pts',(-6.54664141738235,-4.44190740810062,
76.5492939862479));
#223435=CARTESIAN_POINT('Ctrl Pts',(-6.50614035091938,-4.501021340535,76.5521506659481));
#223436=CARTESIAN_POINT('Ctrl Pts',(-6.24385835757158,-4.87290045838385,
76.5702356921297));
#223437=CARTESIAN_POINT('Ctrl Pts',(-6.00038657459935,-5.16974834149366,
76.5851655206213));
#223438=CARTESIAN_POINT('Ctrl Pts',(-5.56470955310888,-5.62850340715576,
76.6096376376599));
#223439=CARTESIAN_POINT('Ctrl Pts',(-5.38462826504667,-5.80101893090419,
76.6192298097057));
#223440=CARTESIAN_POINT('Ctrl Pts',(-5.11156478423377,-6.03892189137479,
76.6332779150652));
#223441=CARTESIAN_POINT('Ctrl Pts',(-5.02484666258029,-6.11126728103273,
76.6376726542771));
#223442=CARTESIAN_POINT('Ctrl Pts',(-4.82428005240047,-6.27143588530811,
76.6477284519601));
#223443=CARTESIAN_POINT('Ctrl Pts',(-4.70952728040981,-6.35806082496251,
76.6534056223974));
#223444=CARTESIAN_POINT('Ctrl Pts',(-4.57446218967838,-6.45435561097018,
76.6600476664002));
#223445=CARTESIAN_POINT('Ctrl Pts',(-4.55639023085987,-6.46712600271583,
76.6609355847764));
#223446=CARTESIAN_POINT('Ctrl Pts',(-4.52747385972399,-6.48737813126574,
76.6623552867094));
#223447=CARTESIAN_POINT('Ctrl Pts',(-4.51666388741157,-6.49490892123612,
76.6628857942449));
#223448=CARTESIAN_POINT('Ctrl Pts',(-4.49752977992603,-6.50816786666971,
76.6638244705906));
#223449=CARTESIAN_POINT('Ctrl Pts',(-4.48921337778987,-6.51390714932612,
76.6642323401517));
#223450=CARTESIAN_POINT('Ctrl Pts',(-4.47196583027777,-6.52576124056592,
76.6650780224806));
#223451=CARTESIAN_POINT('Ctrl Pts',(-4.46303308764215,-6.53187368323698,
76.6655158989007));
#223452=CARTESIAN_POINT('Ctrl Pts',(-4.43985636860782,-6.54766316802918,
76.6666517563069));
#223453=CARTESIAN_POINT('Ctrl Pts',(-4.42559338797976,-6.55731200233249,
76.6673505396136));
#223454=CARTESIAN_POINT('Ctrl Pts',(-4.35580663761875,-6.60419097971223,
76.6707684977405));
#223455=CARTESIAN_POINT('Ctrl Pts',(-4.29984457614301,-6.64076248568217,
76.6735057609012));
#223456=CARTESIAN_POINT('Ctrl Pts',(-3.66030169212112,-7.04723359945113,
76.704711173181));
#223457=CARTESIAN_POINT('Ctrl Pts',(-3.031125569441,-7.33986746085772,76.7344053909393));
#223458=CARTESIAN_POINT('Ctrl Pts',(-2.21346180294125,-7.59684814624296,
76.7697558642873));
#223459=CARTESIAN_POINT('Ctrl Pts',(-2.05345843746716,-7.64165067482622,
76.7765459870432));
#223460=CARTESIAN_POINT('Ctrl Pts',(-1.85284797860512,-7.6910671982888,
76.7849136872439));
#223461=CARTESIAN_POINT('Ctrl Pts',(-1.81346121059945,-7.70044925587654,
76.786549713573));
#223462=CARTESIAN_POINT('Ctrl Pts',(-1.75128868264871,-7.71475548911146,
76.7891218282532));
#223463=CARTESIAN_POINT('Ctrl Pts',(-1.72855031927075,-7.71988200072024,
76.790060350592));
#223464=CARTESIAN_POINT('Ctrl Pts',(-1.68827165425998,-7.72877620730823,
76.7917190915845));
#223465=CARTESIAN_POINT('Ctrl Pts',(-1.67074059005184,-7.7325848669138,
76.7924397939047));
#223466=CARTESIAN_POINT('Ctrl Pts',(-1.63038909534158,-7.74120767958216,
76.7940958197187));
#223467=CARTESIAN_POINT('Ctrl Pts',(-1.60756000967662,-7.74598061967059,
76.7950306513656));
#223468=CARTESIAN_POINT('Ctrl Pts',(-1.54384023063618,-7.75900886176455,
76.7976343165433));
#223469=CARTESIAN_POINT('Ctrl Pts',(-1.50290476220918,-7.76704180976044,
76.799300560192));
#223470=CARTESIAN_POINT('Ctrl Pts',(-1.23695142590228,-7.81704973977265,
76.8100868897481));
#223471=CARTESIAN_POINT('Ctrl Pts',(-1.01026306651008,-7.84956602602521,
76.8190963092071));
#223472=CARTESIAN_POINT('Ctrl Pts',(-0.217984704384075,-7.9283168522101,
76.8502609313704));
#223473=CARTESIAN_POINT('Ctrl Pts',(0.350925627523741,-7.92354827175539,
76.8719460904962));
#223474=CARTESIAN_POINT('Ctrl Pts',(1.32316897105209,-7.81040775349422,
76.908659661111));
#223475=CARTESIAN_POINT('Ctrl Pts',(1.72755639665303,-7.73102700946478,
76.9238734703231));
#223476=CARTESIAN_POINT('Ctrl Pts',(2.31262192602222,-7.56796371712911,
76.9470680183079));
#223477=CARTESIAN_POINT('Ctrl Pts',(2.4992981248048,-7.50838188305888,76.9546619254942));
#223478=CARTESIAN_POINT('Ctrl Pts',(2.70071059881239,-7.43575251977539,
76.9632107171017));
#223479=CARTESIAN_POINT('Ctrl Pts',(2.71783667040661,-7.42950988295323,
76.9639404862569));
#223480=CARTESIAN_POINT('Ctrl Pts',(2.74333440375094,-7.42011572433422,
76.965031432397));
#223481=CARTESIAN_POINT('Ctrl Pts',(2.75172260100697,-7.41700908316175,
76.9653910491678));
#223482=CARTESIAN_POINT('Ctrl Pts',(2.76612681189296,-7.41164656077807,
76.9660098429142));
#223483=CARTESIAN_POINT('Ctrl Pts',(2.77214538907784,-7.40939756140302,
76.9662687748677));
#223484=CARTESIAN_POINT('Ctrl Pts',(2.7845311029556,-7.40475211064766,76.9668024245606));
#223485=CARTESIAN_POINT('Ctrl Pts',(2.79089789977172,-7.4023547737306,76.967077174175));
#223486=CARTESIAN_POINT('Ctrl Pts',(2.80566359717387,-7.39677317893505,
76.967715378823));
#223487=CARTESIAN_POINT('Ctrl Pts',(2.81406017409229,-7.3935828268122,76.968079058053));
#223488=CARTESIAN_POINT('Ctrl Pts',(2.84061845668676,-7.3834399820539,76.9692318267219));
#223489=CARTESIAN_POINT('Ctrl Pts',(2.85875989176211,-7.37643484741358,
76.9700228984838));
#223490=CARTESIAN_POINT('Ctrl Pts',(3.37363761505448,-7.17543525300957,
76.992582118535));
#223491=CARTESIAN_POINT('Ctrl Pts',(3.84939343422768,-6.93182428975471,
77.016835596477));
#223492=CARTESIAN_POINT('Ctrl Pts',(4.52373506539515,-6.49559190686231,
77.0536595166864));
#223493=CARTESIAN_POINT('Ctrl Pts',(4.74288873478383,-6.33734220443818,
77.0660526505566));
#223494=CARTESIAN_POINT('Ctrl Pts',(5.30683188770887,-5.88445331552284,
77.0986151183145));
#223495=CARTESIAN_POINT('Ctrl Pts',(5.63514153606628,-5.57086347889153,
77.1182589329069));
#223496=CARTESIAN_POINT('Ctrl Pts',(5.95345962559196,-5.20970573402456,
77.1378135105385));
#223497=CARTESIAN_POINT('Ctrl Pts',(5.97198235264814,-5.18846240706497,
77.138953677477));
#223498=CARTESIAN_POINT('Ctrl Pts',(5.9969939914618,-5.1594656948837,77.1404964730489));
#223499=CARTESIAN_POINT('Ctrl Pts',(6.00358203583363,-5.15179832003059,
77.1409031494016));
#223500=CARTESIAN_POINT('Ctrl Pts',(6.01472623034433,-5.13877794677304,
77.1415915973854));
#223501=CARTESIAN_POINT('Ctrl Pts',(6.01928996749723,-5.13343147414771,
77.1418736780397));
#223502=CARTESIAN_POINT('Ctrl Pts',(6.02806906903521,-5.12311884799037,
77.1424165969397));
#223503=CARTESIAN_POINT('Ctrl Pts',(6.03228543660801,-5.11815355799759,
77.1426774759119));
#223504=CARTESIAN_POINT('Ctrl Pts',(6.04210756670188,-5.10655779756107,
77.1432855042037));
#223505=CARTESIAN_POINT('Ctrl Pts',(6.04770856069563,-5.09992328892645,
77.1436324598246));
#223506=CARTESIAN_POINT('Ctrl Pts',(6.06309286162972,-5.08163924095278,
77.1445860913525));
#223507=CARTESIAN_POINT('Ctrl Pts',(6.07285352891187,-5.06997065510325,
77.1451918501512));
#223508=CARTESIAN_POINT('Ctrl Pts',(6.09501950047367,-5.04331604759972,
77.1465691713219));
#223509=CARTESIAN_POINT('Ctrl Pts',(6.10740332598903,-5.02831225041406,
77.1473398673863));
#223510=CARTESIAN_POINT('Ctrl Pts',(6.36084238851596,-4.7189370752753,77.1631378338541));
#223511=CARTESIAN_POINT('Ctrl Pts',(6.58041656511223,-4.40758901291123,
77.1772655475297));
#223512=CARTESIAN_POINT('Ctrl Pts',(6.96091227020838,-3.77584873618555,
77.2034777585124));
#223513=CARTESIAN_POINT('Ctrl Pts',(7.12417490566864,-3.45795816443406,
77.2156104395252));
#223514=CARTESIAN_POINT('Ctrl Pts',(7.4881183575066,-2.61320015636736,77.2468958250767));
#223515=CARTESIAN_POINT('Ctrl Pts',(7.65499465531323,-2.07403935846896,
77.2659453806929));
#223516=CARTESIAN_POINT('Ctrl Pts',(7.77013436597465,-1.48667933675384,
77.2895670635791));
#223517=CARTESIAN_POINT('Ctrl Pts',(7.77678467420677,-1.45149012100044,
77.2909931643193));
#223518=CARTESIAN_POINT('Ctrl Pts',(7.78456823384693,-1.40871472963587,
77.2927411385468));
#223519=CARTESIAN_POINT('Ctrl Pts',(7.78592977005468,-1.40117000822365,
77.2930499902626));
#223520=CARTESIAN_POINT('Ctrl Pts',(7.78814731183403,-1.38877884130431,
77.2935581458677));
#223521=CARTESIAN_POINT('Ctrl Pts',(7.78900976833996,-1.38393354224265,
77.2937570772932));
#223522=CARTESIAN_POINT('Ctrl Pts',(7.79054991706618,-1.37523390916273,
77.2941146685741));
#223523=CARTESIAN_POINT('Ctrl Pts',(7.7912292723661,-1.37137986733455,77.2942732316256));
#223524=CARTESIAN_POINT('Ctrl Pts',(7.79266569668858,-1.36319538788206,
77.2946102699534));
#223525=CARTESIAN_POINT('Ctrl Pts',(7.79342201613189,-1.35886482190437,
77.2947887890336));
#223526=CARTESIAN_POINT('Ctrl Pts',(7.79543329961403,-1.34729161732688,
77.2952663724309));
#223527=CARTESIAN_POINT('Ctrl Pts',(7.79668177696388,-1.34004787186593,
77.2955658189194));
#223528=CARTESIAN_POINT('Ctrl Pts',(7.80273772619129,-1.30461590702181,
77.2970331308405));
#223529=CARTESIAN_POINT('Ctrl Pts',(7.80740234816075,-1.27640401212969,
77.2982095401699));
#223530=CARTESIAN_POINT('Ctrl Pts',(7.8458088210817,-1.03602926515093,77.3082977145133));
#223531=CARTESIAN_POINT('Ctrl Pts',(7.87104619629272,-0.822612316093222,
77.3176817122153));
#223532=CARTESIAN_POINT('Ctrl Pts',(7.91681991744016,-0.22923071993547,
77.344410605188));
#223533=CARTESIAN_POINT('Ctrl Pts',(7.91868628182647,0.151596047997172,
77.3622605995352));
#223534=CARTESIAN_POINT('Ctrl Pts',(7.85157213574104,1.14909495846763,77.4086400764158));
#223535=CARTESIAN_POINT('Ctrl Pts',(7.7375437605627,1.76018885134718,77.4364886989475));
#223536=CARTESIAN_POINT('Ctrl Pts',(7.54213941461043,2.3877760018051,77.4632386514524));
#223537=CARTESIAN_POINT('Ctrl Pts',(7.53067919231729,2.42367740055003,77.4647632341558));
#223538=CARTESIAN_POINT('Ctrl Pts',(7.51521943076385,2.47093967551408,77.4667629491241));
#223539=CARTESIAN_POINT('Ctrl Pts',(7.51144997249829,2.48237492837154,77.4672462193244));
#223540=CARTESIAN_POINT('Ctrl Pts',(7.50556779411171,2.50008337923575,77.4679937324917));
#223541=CARTESIAN_POINT('Ctrl Pts',(7.50347329091114,2.5063625811159,77.4682586215396));
#223542=CARTESIAN_POINT('Ctrl Pts',(7.49927100900739,2.51890830425175,77.4687875264812));
#223543=CARTESIAN_POINT('Ctrl Pts',(7.49716325066102,2.52517482662088,77.4690515428222));
#223544=CARTESIAN_POINT('Ctrl Pts',(7.49250290862249,2.53897310087461,77.4696325111202));
#223545=CARTESIAN_POINT('Ctrl Pts',(7.48994681721243,2.54650366552312,77.4699493379941));
#223546=CARTESIAN_POINT('Ctrl Pts',(7.48255654950627,2.56816892777995,77.4708601463924));
#223547=CARTESIAN_POINT('Ctrl Pts',(7.47769367388293,2.58229384097178,77.4714531054398));
#223548=CARTESIAN_POINT('Ctrl Pts',(7.46666087460653,2.61404767080262,77.4727842274293));
#223549=CARTESIAN_POINT('Ctrl Pts',(7.46046846049478,2.63166870979522,77.4735215858361));
#223550=CARTESIAN_POINT('Ctrl Pts',(7.32781121035121,3.00492486421935,77.4891132311119));
#223551=CARTESIAN_POINT('Ctrl Pts',(7.17611332320944,3.35109367064447,77.5030086465629));
#223552=CARTESIAN_POINT('Ctrl Pts',(6.80702504483415,4.0522108850848,77.5308860611456));
#223553=CARTESIAN_POINT('Ctrl Pts',(6.58521176629109,4.40352053079047,77.5446939448114));
#223554=CARTESIAN_POINT('Ctrl Pts',(6.06102167519495,5.10492715990078,77.5743821133893));
#223555=CARTESIAN_POINT('Ctrl Pts',(5.75347103359281,5.44919604848762,77.5902789473847));
#223556=CARTESIAN_POINT('Ctrl Pts',(5.3959102833323,5.78523745015897,77.6096762217839));
#223557=CARTESIAN_POINT('Ctrl Pts',(5.37394360351371,5.80564813251346,77.6108713604107));
#223558=CARTESIAN_POINT('Ctrl Pts',(5.34630499731195,5.83103771289881,77.6123802364051));
#223559=CARTESIAN_POINT('Ctrl Pts',(5.34074100112988,5.83613429348374,77.6126842509345));
#223560=CARTESIAN_POINT('Ctrl Pts',(5.33197677989886,5.84413922820667,77.6131635478668));
#223561=CARTESIAN_POINT('Ctrl Pts',(5.32878144157685,5.84705293696424,77.6133383828464));
#223562=CARTESIAN_POINT('Ctrl Pts',(5.32286762132675,5.85243665296755,77.6136621224598));
#223563=CARTESIAN_POINT('Ctrl Pts',(5.32014979922594,5.85490739507209,77.6138109666877));
#223564=CARTESIAN_POINT('Ctrl Pts',(5.31411984324568,5.86038149629061,77.6141413402678));
#223565=CARTESIAN_POINT('Ctrl Pts',(5.31080688418205,5.86338394011517,77.614322944589));
#223566=CARTESIAN_POINT('Ctrl Pts',(5.30133256211888,5.87195564058169,77.6148425488391));
#223567=CARTESIAN_POINT('Ctrl Pts',(5.29516498843464,5.87751799004787,77.6151811091879));
#223568=CARTESIAN_POINT('Ctrl Pts',(5.25596525936006,5.912759267607,77.6173348161676));
#223569=CARTESIAN_POINT('Ctrl Pts',(5.22269308500364,5.94216877479076,77.6191713637252));
#223570=CARTESIAN_POINT('Ctrl Pts',(5.12168865239798,6.02994364819143,77.6247670525515));
#223571=CARTESIAN_POINT('Ctrl Pts',(5.05321450940839,6.08744092695492,77.6285878689974));
#223572=CARTESIAN_POINT('Ctrl Pts',(4.86721434929003,6.23832311867019,77.6390032106648));
#223573=CARTESIAN_POINT('Ctrl Pts',(4.7479829477844,6.32954222217595,77.6457174580962));
#223574=CARTESIAN_POINT('Ctrl Pts',(4.3472056316177,6.61846233565767,77.6682123913164));
#223575=CARTESIAN_POINT('Ctrl Pts',(4.05536120710385,6.80119657325046,77.6844623802304));
#223576=CARTESIAN_POINT('Ctrl Pts',(3.40855002260958,7.14971394998826,77.7189691097025));
#223577=CARTESIAN_POINT('Ctrl Pts',(3.05125595790959,7.30934343525296,77.7371381856648));
#223578=CARTESIAN_POINT('Ctrl Pts',(2.55815853211328,7.4871576261782,77.7604470378504));
#223579=CARTESIAN_POINT('Ctrl Pts',(2.43158393973321,7.52921683996112,77.7662852437559));
#223580=CARTESIAN_POINT('Ctrl Pts',(2.10535539986208,7.62853311717715,77.7809507864971));
#223581=CARTESIAN_POINT('Ctrl Pts',(1.90439583992086,7.68116686815188,77.7896239977303));
#223582=CARTESIAN_POINT('Ctrl Pts',(1.68250868153269,7.73003668454191,77.7988224927611));
#223583=CARTESIAN_POINT('Ctrl Pts',(1.66341554021376,7.73416778689073,77.7996110128789));
#223584=CARTESIAN_POINT('Ctrl Pts',(1.63511744170344,7.74018089043761,77.8007752859817));
#223585=CARTESIAN_POINT('Ctrl Pts',(1.62592419234598,7.74211726767259,77.801152838846));
#223586=CARTESIAN_POINT('Ctrl Pts',(1.61021523413533,7.74539683668304,77.8017968155789));
#223587=CARTESIAN_POINT('Ctrl Pts',(1.60370125063025,7.74674819243386,77.8020635090713));
#223588=CARTESIAN_POINT('Ctrl Pts',(1.59105397123338,7.74935529283511,77.8025806482088));
#223589=CARTESIAN_POINT('Ctrl Pts',(1.58492087482318,7.75061197679073,77.8028311247043));
#223590=CARTESIAN_POINT('Ctrl Pts',(1.57224824469199,7.75319295362273,77.8033480553484));
#223591=CARTESIAN_POINT('Ctrl Pts',(1.56570851334359,7.75451625638698,77.8036144767077));
#223592=CARTESIAN_POINT('Ctrl Pts',(1.54544374066389,7.75859011588527,77.8044389871983));
#223593=CARTESIAN_POINT('Ctrl Pts',(1.53171303218555,7.76131252634275,77.8049961502282));
#223594=CARTESIAN_POINT('Ctrl Pts',(1.45853933869499,7.77561905236369,77.8079574829352));
#223595=CARTESIAN_POINT('Ctrl Pts',(1.39897127190299,7.78655689251933,77.8103404258614));
#223596=CARTESIAN_POINT('Ctrl Pts',(1.23199578992739,7.81523879740535,77.8169458940189));
#223597=CARTESIAN_POINT('Ctrl Pts',(1.12433774749176,7.83145177101568,77.8211191443115));
#223598=CARTESIAN_POINT('Ctrl Pts',(0.696440555039915,7.8868858611171,77.8374042917127));
#223599=CARTESIAN_POINT('Ctrl Pts',(0.374257070161404,7.90872607166841,
77.8489839292691));
#223600=CARTESIAN_POINT('Ctrl Pts',(-0.682728726760493,7.91562390989119,
77.8860047764095));
#223601=CARTESIAN_POINT('Ctrl Pts',(-1.41414352335224,7.81814241127103,
77.9099116164651));
#223602=CARTESIAN_POINT('Ctrl Pts',(-2.16279527107709,7.60973514527557,
77.9405670438782));
#223603=CARTESIAN_POINT('Ctrl Pts',(-2.20392776828705,7.59792436512276,
77.9422705187981));
#223604=CARTESIAN_POINT('Ctrl Pts',(-2.25609009328976,7.58248726837354,
77.9444537725741));
#223605=CARTESIAN_POINT('Ctrl Pts',(-2.26721104809879,7.57916946278228,
77.9449205732845));
#223606=CARTESIAN_POINT('Ctrl Pts',(-2.28482754738544,7.57387154573944,
77.94566210214));
#223607=CARTESIAN_POINT('Ctrl Pts',(-2.2913279383155,7.57190751339285,77.945936171431));
#223608=CARTESIAN_POINT('Ctrl Pts',(-2.30336772200221,7.5682528816291,77.9464446167069));
#223609=CARTESIAN_POINT('Ctrl Pts',(-2.30890780638163,7.56656456289447,
77.9466789005935));
#223610=CARTESIAN_POINT('Ctrl Pts',(-2.32121642131671,7.56279878446657,
77.9472001314188));
#223611=CARTESIAN_POINT('Ctrl Pts',(-2.32798402266772,7.56071832028621,
77.9474871977965));
#223612=CARTESIAN_POINT('Ctrl Pts',(-2.34740579030132,7.55471922307376,
77.9483123890394));
#223613=CARTESIAN_POINT('Ctrl Pts',(-2.36005288541576,7.55077789762234,
77.9488514017277));
#223614=CARTESIAN_POINT('Ctrl Pts',(-2.44287481713292,7.52473896178988,
77.9523919217114));
#223615=CARTESIAN_POINT('Ctrl Pts',(-2.51274714208484,7.50169548879922,
77.9554292015039));
#223616=CARTESIAN_POINT('Ctrl Pts',(-2.73317966984023,7.42557296862749,
77.965153872295));
#223617=CARTESIAN_POINT('Ctrl Pts',(-2.88245692108499,7.3689106512389,77.9719518520097));
#223618=CARTESIAN_POINT('Ctrl Pts',(-3.50435477055147,7.11106242071615,
78.0009621446071));
#223619=CARTESIAN_POINT('Ctrl Pts',(-3.95851597577381,6.86861581018722,
78.0237736388431));
#223620=CARTESIAN_POINT('Ctrl Pts',(-4.74260182460372,6.34628021883938,
78.0644147080596));
#223621=CARTESIAN_POINT('Ctrl Pts',(-5.07935214457477,6.08011252520854,
78.0823942268664));
#223622=CARTESIAN_POINT('Ctrl Pts',(-5.42239712183903,5.76048223196537,
78.1013904397017));
#223623=CARTESIAN_POINT('Ctrl Pts',(-5.45168082966606,5.73277613880576,
78.1030184423208));
#223624=CARTESIAN_POINT('Ctrl Pts',(-5.4935892406331,5.69251395897022,78.105357772358));
#223625=CARTESIAN_POINT('Ctrl Pts',(-5.50638526724705,5.68013725270134,
78.1060733281485));
#223626=CARTESIAN_POINT('Ctrl Pts',(-5.52835001356206,5.65874830747929,
78.1073038057979));
#223627=CARTESIAN_POINT('Ctrl Pts',(-5.53753872758249,5.64975673118095,
78.1078192329772));
#223628=CARTESIAN_POINT('Ctrl Pts',(-5.55621206840689,5.63139469514049,
78.1088680527892));
#223629=CARTESIAN_POINT('Ctrl Pts',(-5.56569500815437,5.62202257546752,
78.1094014014431));
#223630=CARTESIAN_POINT('Ctrl Pts',(-5.58898003424249,5.59889301012379,
78.1107128046191));
#223631=CARTESIAN_POINT('Ctrl Pts',(-5.60275508531585,5.58510843404367,
78.1114901620989));
#223632=CARTESIAN_POINT('Ctrl Pts',(-5.65302017104975,5.53443549084582,
78.1143324484749));
#223633=CARTESIAN_POINT('Ctrl Pts',(-5.68919819416887,5.4972390563282,78.1163892565158));
#223634=CARTESIAN_POINT('Ctrl Pts',(-5.89483760099557,5.28160640599078,
78.1281455254455));
#223635=CARTESIAN_POINT('Ctrl Pts',(-6.05626983074201,5.09569231729241,
78.1376258254963));
#223636=CARTESIAN_POINT('Ctrl Pts',(-6.43217919107187,4.61962604532561,
78.1605158125718));
#223637=CARTESIAN_POINT('Ctrl Pts',(-6.63598390843638,4.32175900319384,
78.173661290718));
#223638=CARTESIAN_POINT('Ctrl Pts',(-6.97677875995999,3.74240636299991,
78.1981058565199));
#223639=CARTESIAN_POINT('Ctrl Pts',(-7.11877559423572,3.46468899349478,
78.2093999677342));
#223640=CARTESIAN_POINT('Ctrl Pts',(-7.2670819533056,3.12677705606071,78.2232824043481));
#223641=CARTESIAN_POINT('Ctrl Pts',(-7.28957436711832,3.07397467105855,
78.225456029218));
#223642=CARTESIAN_POINT('Ctrl Pts',(-7.32579239824619,2.98631705419967,
78.2290779919308));
#223643=CARTESIAN_POINT('Ctrl Pts',(-7.33984868002205,2.95160043331317,
78.2305159326895));
#223644=CARTESIAN_POINT('Ctrl Pts',(-7.36063596688101,2.89919253829818,
78.2326935039014));
#223645=CARTESIAN_POINT('Ctrl Pts',(-7.367550964607,2.88157456754953,78.2334267007099));
#223646=CARTESIAN_POINT('Ctrl Pts',(-7.40364044764668,2.78864695062231,
78.2373008909252));
#223647=CARTESIAN_POINT('Ctrl Pts',(-7.43172300949163,2.71292023447926,
78.2404816706145));
#223648=CARTESIAN_POINT('Ctrl Pts',(-7.46302583095415,2.62437412547728,
78.2442417199794));
#223649=CARTESIAN_POINT('Ctrl Pts',(-7.46738012459949,2.61195868568348,
78.2447698603604));
#223650=CARTESIAN_POINT('Ctrl Pts',(-7.4738753886561,2.5932896801331,78.2455654896149));
#223651=CARTESIAN_POINT('Ctrl Pts',(-7.47603954031818,2.58704415916208,
78.245831905564));
#223652=CARTESIAN_POINT('Ctrl Pts',(-7.47987568709139,2.5759284190981,78.246306520887));
#223653=CARTESIAN_POINT('Ctrl Pts',(-7.48155076122501,2.57105926063264,
78.2465145756145));
#223654=CARTESIAN_POINT('Ctrl Pts',(-7.48506217617925,2.56081967978592,
78.2469524324354));
#223655=CARTESIAN_POINT('Ctrl Pts',(-7.48689749321258,2.55544891154598,
78.2471822829267));
#223656=CARTESIAN_POINT('Ctrl Pts',(-7.49170691897792,2.5413252249918,78.2477872383819));
#223657=CARTESIAN_POINT('Ctrl Pts',(-7.49467146180025,2.53256907854438,
78.2481628021888));
#223658=CARTESIAN_POINT('Ctrl Pts',(-7.50778462225264,2.49361306015807,
78.2498360480472));
#223659=CARTESIAN_POINT('Ctrl Pts',(-7.51776604064202,2.46335741637706,
78.2511419129291));
#223660=CARTESIAN_POINT('Ctrl Pts',(-7.59191090184999,2.23396141522681,
78.261096088382));
#223661=CARTESIAN_POINT('Ctrl Pts',(-7.64833039736845,2.03241860934034,
78.2701407907994));
#223662=CARTESIAN_POINT('Ctrl Pts',(-7.83905738313568,1.22976457236923,
78.306758924624));
#223663=CARTESIAN_POINT('Ctrl Pts',(-7.91097894886285,0.616079605845327,
78.3358990774571));
#223664=CARTESIAN_POINT('Ctrl Pts',(-7.91099999537971,0.000270374307908966,
78.3636650122822));
#223665=CARTESIAN_POINT('',(-7.911,-4.5324854980322E-12,80.3576684917632));
#223666=CARTESIAN_POINT('Ctrl Pts',(-7.911,-4.92828000631107E-12,78.3576684917632));
#223667=CARTESIAN_POINT('Ctrl Pts',(-7.91099999999863,-2.2016758966715,
78.4462559274959));
#223668=CARTESIAN_POINT('Ctrl Pts',(-6.94214576672116,-4.38610418339077,
78.5348433632287));
#223669=CARTESIAN_POINT('Ctrl Pts',(-3.67820201487898,-7.34180684107821,
78.7120182346941));
#223670=CARTESIAN_POINT('Ctrl Pts',(-1.4086817587134,-8.08992666571401,
78.8006056704268));
#223671=CARTESIAN_POINT('Ctrl Pts',(2.97309270521618,-7.65454228025118,
78.9777805418922));
#223672=CARTESIAN_POINT('Ctrl Pts',(5.05102072675873,-6.47444880834007,
79.066367977625));
#223673=CARTESIAN_POINT('Ctrl Pts',(7.66951518847977,-2.93425195367416,
79.2435428490904));
#223674=CARTESIAN_POINT('Ctrl Pts',(8.18956872247087,-0.601881960096307,
79.3321302848231));
#223675=CARTESIAN_POINT('Ctrl Pts',(7.32306689761226,3.71537198232669,79.5093051562885));
#223676=CARTESIAN_POINT('Ctrl Pts',(5.94329958850042,5.6664351893667,79.5978925920213));
#223677=CARTESIAN_POINT('Ctrl Pts',(2.16154501637666,7.92205913233042,79.7750674634867));
#223678=CARTESIAN_POINT('Ctrl Pts',(-0.210816529302004,8.20894963712993,
79.8636548992194));
#223679=CARTESIAN_POINT('Ctrl Pts',(-4.42123908576541,6.91982244717759,
80.0408297706849));
#223680=CARTESIAN_POINT('Ctrl Pts',(-6.22631625634251,5.3539035880344,80.1294172064176));
#223681=CARTESIAN_POINT('Ctrl Pts',(-7.65317280859565,2.31334857514328,
80.2645592586879));
#223682=CARTESIAN_POINT('Ctrl Pts',(-7.91100000000066,1.1570283783619,80.3111138752256));
#223683=CARTESIAN_POINT('Ctrl Pts',(-7.911,-4.5324854980322E-12,80.3576684917632));
#223684=CARTESIAN_POINT('',(-7.91099794240846,0.00570571723741386,84.3576684917632));
#223685=CARTESIAN_POINT('Ctrl Pts',(-7.91099987852728,-0.00138634102841706,
80.3603921088743));
#223686=CARTESIAN_POINT('Ctrl Pts',(-7.91095793537386,-0.24073025048579,
80.3695915106551));
#223687=CARTESIAN_POINT('Ctrl Pts',(-7.9000542515115,-0.479956577419262,
80.3785790578079));
#223688=CARTESIAN_POINT('Ctrl Pts',(-7.81569063911966,-1.40521807938145,
80.4129340180817));
#223689=CARTESIAN_POINT('Ctrl Pts',(-7.6635114518347,-2.08087428066251,
80.4368573329913));
#223690=CARTESIAN_POINT('Ctrl Pts',(-7.40946242548989,-2.772364669455,80.4658737675769));
#223691=CARTESIAN_POINT('Ctrl Pts',(-7.39282587712584,-2.8164276518804,
80.4677448525175));
#223692=CARTESIAN_POINT('Ctrl Pts',(-7.37197854201269,-2.87018551934564,
80.4700576007669));
#223693=CARTESIAN_POINT('Ctrl Pts',(-7.36814027622444,-2.88002454983967,
80.4704821272609));
#223694=CARTESIAN_POINT('Ctrl Pts',(-7.36210183251155,-2.89541244701035,
80.4711480489127));
#223695=CARTESIAN_POINT('Ctrl Pts',(-7.35991504801162,-2.90096658311365,
80.4713888117564));
#223696=CARTESIAN_POINT('Ctrl Pts',(-7.35603196292923,-2.91079644077777,
80.471815644071));
#223697=CARTESIAN_POINT('Ctrl Pts',(-7.35433821370686,-2.91507317190321,
80.4720015912719));
#223698=CARTESIAN_POINT('Ctrl Pts',(-7.35072802056362,-2.924165767027,80.4723974479248));
#223699=CARTESIAN_POINT('Ctrl Pts',(-7.34881057253635,-2.92898122802785,
80.4726074059676));
#223700=CARTESIAN_POINT('Ctrl Pts',(-7.34331976918453,-2.94273144652949,
80.4732078255246));
#223701=CARTESIAN_POINT('Ctrl Pts',(-7.33973485098251,-2.95166155155004,
80.4735988540301));
#223702=CARTESIAN_POINT('Ctrl Pts',(-7.32429967848262,-2.98990888649565,
80.475278355521));
#223703=CARTESIAN_POINT('Ctrl Pts',(-7.31229005405701,-3.01916131986956,
80.4765748322347));
#223704=CARTESIAN_POINT('Ctrl Pts',(-7.12013556792224,-3.47932902306754,
80.4971696743844));
#223705=CARTESIAN_POINT('Ctrl Pts',(-6.90236700072341,-3.89349611162777,
80.5184320397395));
#223706=CARTESIAN_POINT('Ctrl Pts',(-6.56805011579318,-4.41216161926071,
80.5468415634856));
#223707=CARTESIAN_POINT('Ctrl Pts',(-6.48315239239182,-4.53598805123894,
80.553774624271));
#223708=CARTESIAN_POINT('Ctrl Pts',(-6.31777510742065,-4.76306090839403,
80.5667063731205));
#223709=CARTESIAN_POINT('Ctrl Pts',(-6.23815543313102,-4.86687262062322,
80.57270874959));
#223710=CARTESIAN_POINT('Ctrl Pts',(-6.13038887501367,-5.00039155576887,
80.5805240127588));
#223711=CARTESIAN_POINT('Ctrl Pts',(-6.10453527998605,-5.03192135473416,
80.5823767754192));
#223712=CARTESIAN_POINT('Ctrl Pts',(-5.93869806269754,-5.23100917251759,
80.594118759109));
#223713=CARTESIAN_POINT('Ctrl Pts',(-5.79206716241005,-5.39291732373115,
80.6038604241587));
#223714=CARTESIAN_POINT('Ctrl Pts',(-5.44063571003916,-5.75007203217559,
80.6256919331491));
#223715=CARTESIAN_POINT('Ctrl Pts',(-5.23168180123048,-5.94082246340584,
80.6376075846975));
#223716=CARTESIAN_POINT('Ctrl Pts',(-4.9964776490394,-6.13348069283378,
80.6499306919887));
#223717=CARTESIAN_POINT('Ctrl Pts',(-4.97995234760287,-6.14690563870763,
80.6507910754564));
#223718=CARTESIAN_POINT('Ctrl Pts',(-4.95563367044605,-6.16649938814303,
80.6520493183198));
#223719=CARTESIAN_POINT('Ctrl Pts',(-4.94788261014304,-6.17272042593602,
80.6524491867495));
#223720=CARTESIAN_POINT('Ctrl Pts',(-4.9342073266964,-6.18365396512743,
80.6531526270698));
#223721=CARTESIAN_POINT('Ctrl Pts',(-4.92828803243892,-6.18837259487222,
80.6534564338072));
#223722=CARTESIAN_POINT('Ctrl Pts',(-4.91674365329109,-6.19754825347419,
80.6540476369052));
#223723=CARTESIAN_POINT('Ctrl Pts',(-4.91111925984339,-6.20200613690654,
80.654335065817));
#223724=CARTESIAN_POINT('Ctrl Pts',(-4.89761714119421,-6.2126780063063,
80.6550236345171));
#223725=CARTESIAN_POINT('Ctrl Pts',(-4.88973363603806,-6.21888467824472,
80.6554244951526));
#223726=CARTESIAN_POINT('Ctrl Pts',(-4.86567588721527,-6.23775128062091,
80.6566442196407));
#223727=CARTESIAN_POINT('Ctrl Pts',(-4.84946407340832,-6.25036327638874,
80.6574612613718));
#223728=CARTESIAN_POINT('Ctrl Pts',(-4.67293970306116,-6.38659034673561,
80.6663051093463));
#223729=CARTESIAN_POINT('Ctrl Pts',(-4.50798252653677,-6.50407580453327,
80.6740974921286));
#223730=CARTESIAN_POINT('Ctrl Pts',(-3.99548681892427,-6.84020952683684,
80.6970687377426));
#223731=CARTESIAN_POINT('Ctrl Pts',(-3.63527099537886,-7.03826782921289,
80.7115469612408));
#223732=CARTESIAN_POINT('Ctrl Pts',(-3.08120565376169,-7.28897576366361,
80.7326249854692));
#223733=CARTESIAN_POINT('Ctrl Pts',(-2.89811986318283,-7.3636877419717,
80.7394176322963));
#223734=CARTESIAN_POINT('Ctrl Pts',(-2.528347432509,-7.49865189982054,80.7530436453756));
#223735=CARTESIAN_POINT('Ctrl Pts',(-2.34183706319534,-7.55897593552349,
80.7598717422723));
#223736=CARTESIAN_POINT('Ctrl Pts',(-1.85368237466897,-7.697059561135,80.7779800655483));
#223737=CARTESIAN_POINT('Ctrl Pts',(-1.54934176187841,-7.76404596926381,
80.789526415985));
#223738=CARTESIAN_POINT('Ctrl Pts',(-1.22322088076005,-7.8158817133152,
80.8026935060415));
#223739=CARTESIAN_POINT('Ctrl Pts',(-1.20459528325662,-7.81877397520732,
80.8034477538113));
#223740=CARTESIAN_POINT('Ctrl Pts',(-1.17770093522285,-7.8228518636963,
80.8045399195286));
#223741=CARTESIAN_POINT('Ctrl Pts',(-1.16944027996602,-7.82409101462229,
80.8048757985141));
#223742=CARTESIAN_POINT('Ctrl Pts',(-1.15505942069356,-7.82622495154673,
80.8054612363056));
#223743=CARTESIAN_POINT('Ctrl Pts',(-1.14894009189633,-7.82712564882711,
80.8057105750701));
#223744=CARTESIAN_POINT('Ctrl Pts',(-1.13714052641633,-7.828848278252,80.8061917854172));
#223745=CARTESIAN_POINT('Ctrl Pts',(-1.1314604379527,-7.82967120751795,
80.8064236203898));
#223746=CARTESIAN_POINT('Ctrl Pts',(-1.11802851524996,-7.83160229826112,
80.8069722899079));
#223747=CARTESIAN_POINT('Ctrl Pts',(-1.11027592802888,-7.83270513182781,
80.8072893156823));
#223748=CARTESIAN_POINT('Ctrl Pts',(-1.08321920133923,-7.83651307212582,
80.8083969264799));
#223749=CARTESIAN_POINT('Ctrl Pts',(-1.06390679203152,-7.83915832841082,
80.8091896110198));
#223750=CARTESIAN_POINT('Ctrl Pts',(-0.715263154346291,-7.88560060326201,
80.8235355695218));
#223751=CARTESIAN_POINT('Ctrl Pts',(-0.383516257476511,-7.90867854893081,
80.8377420696769));
#223752=CARTESIAN_POINT('Ctrl Pts',(0.453292814945432,-7.91410700853291,
80.8738137113066));
#223753=CARTESIAN_POINT('Ctrl Pts',(0.957086507945457,-7.86909071114896,
80.895670344785));
#223754=CARTESIAN_POINT('Ctrl Pts',(1.74797015052176,-7.7212997216921,80.9295163748176));
#223755=CARTESIAN_POINT('Ctrl Pts',(2.03941333682996,-7.64948822650898,
80.9419125583887));
#223756=CARTESIAN_POINT('Ctrl Pts',(2.53512223128145,-7.49699336929173,
80.9631413083895));
#223757=CARTESIAN_POINT('Ctrl Pts',(2.74141063437854,-7.4240436779781,80.9720455145676));
#223758=CARTESIAN_POINT('Ctrl Pts',(2.98873004121259,-7.32486817192277,
80.9828200691888));
#223759=CARTESIAN_POINT('Ctrl Pts',(3.03288714042946,-7.3066953279378,80.9847474855872));
#223760=CARTESIAN_POINT('Ctrl Pts',(3.09826238214475,-7.27909541437862,
80.9876066245835));
#223761=CARTESIAN_POINT('Ctrl Pts',(3.11960782437201,-7.26997296181839,
80.9885410423733));
#223762=CARTESIAN_POINT('Ctrl Pts',(3.16262980782737,-7.25136218802389,
80.9904261946402));
#223763=CARTESIAN_POINT('Ctrl Pts',(3.18430455384401,-7.24187029676157,
80.9913768857457));
#223764=CARTESIAN_POINT('Ctrl Pts',(3.23081898312706,-7.22125131127351,
80.993419145273));
#223765=CARTESIAN_POINT('Ctrl Pts',(3.25564450102866,-7.21009297378671,
80.9945104014346));
#223766=CARTESIAN_POINT('Ctrl Pts',(3.32272462936286,-7.17952534425862,
80.9974625730817));
#223767=CARTESIAN_POINT('Ctrl Pts',(3.3648665870068,-7.15987122863654,80.9993210321844));
#223768=CARTESIAN_POINT('Ctrl Pts',(3.57145093136669,-7.06129791398134,
81.0084512408306));
#223769=CARTESIAN_POINT('Ctrl Pts',(3.73330489017435,-6.97707862897671,
81.0156655775695));
#223770=CARTESIAN_POINT('Ctrl Pts',(4.12353642253008,-6.75655485303899,
81.033267744533));
#223771=CARTESIAN_POINT('Ctrl Pts',(4.34823076894736,-6.61418764680973,
81.0435835300217));
#223772=CARTESIAN_POINT('Ctrl Pts',(4.85180298629871,-6.25835201303758,
81.0674370532624));
#223773=CARTESIAN_POINT('Ctrl Pts',(5.12448782893615,-6.03710023523412,
81.0809193590969));
#223774=CARTESIAN_POINT('Ctrl Pts',(5.47602470542838,-5.71083847505918,
81.0997582262461));
#223775=CARTESIAN_POINT('Ctrl Pts',(5.56830852423742,-5.62089510610995,
81.1048580446437));
#223776=CARTESIAN_POINT('Ctrl Pts',(5.67382646128203,-5.5129034549772,81.1109078950903));
#223777=CARTESIAN_POINT('Ctrl Pts',(5.68923336570411,-5.49700235768921,
81.1117969001049));
#223778=CARTESIAN_POINT('Ctrl Pts',(5.71156847651353,-5.47375634066113,
81.1130941623482));
#223779=CARTESIAN_POINT('Ctrl Pts',(5.71854973736505,-5.46646246117536,
81.1135008637168));
#223780=CARTESIAN_POINT('Ctrl Pts',(5.73258908392174,-5.45173811028733,
81.1143212295277));
#223781=CARTESIAN_POINT('Ctrl Pts',(5.73964673187823,-5.44430724893198,
81.1147349058878));
#223782=CARTESIAN_POINT('Ctrl Pts',(5.75332612615036,-5.42984831530666,
81.115539218677));
#223783=CARTESIAN_POINT('Ctrl Pts',(5.75994948478011,-5.4228217906585,81.1159298045814));
#223784=CARTESIAN_POINT('Ctrl Pts',(5.77575378420161,-5.40599385695902,
81.1168645840447));
#223785=CARTESIAN_POINT('Ctrl Pts',(5.78492265960937,-5.39618116623948,
81.1174091558369));
#223786=CARTESIAN_POINT('Ctrl Pts',(5.82068340246384,-5.35771350116169,
81.1195420863586));
#223787=CARTESIAN_POINT('Ctrl Pts',(5.84708753669568,-5.32888511135394,
81.121136379339));
#223788=CARTESIAN_POINT('Ctrl Pts',(6.2209255082974,-4.91460004225055,81.1439792650136));
#223789=CARTESIAN_POINT('Ctrl Pts',(6.52982118227819,-4.4960693730446,81.1661315478555));
#223790=CARTESIAN_POINT('Ctrl Pts',(6.96113102891696,-3.77243007450554,
81.2014735723344));
#223791=CARTESIAN_POINT('Ctrl Pts',(7.10956169887988,-3.4846402505623,81.214884497823));
#223792=CARTESIAN_POINT('Ctrl Pts',(7.26826772330108,-3.12428214550926,
81.2309134748122));
#223793=CARTESIAN_POINT('Ctrl Pts',(7.29572097510323,-3.05962582736397,
81.2337613819408));
#223794=CARTESIAN_POINT('Ctrl Pts',(7.33318442751359,-2.96802164113235,
81.2377585138106));
#223795=CARTESIAN_POINT('Ctrl Pts',(7.34391424519294,-2.94137210804497,
81.2389169096192));
#223796=CARTESIAN_POINT('Ctrl Pts',(7.36194061613685,-2.89588662776988,
81.2408866585347));
#223797=CARTESIAN_POINT('Ctrl Pts',(7.36931061064185,-2.87708013847965,
81.241698929542));
#223798=CARTESIAN_POINT('Ctrl Pts',(7.3840187892947,-2.83912102258128,81.2433341799274));
#223799=CARTESIAN_POINT('Ctrl Pts',(7.39135467976364,-2.8199676704655,81.244157125335));
#223800=CARTESIAN_POINT('Ctrl Pts',(7.4091091386683,-2.77306711280438,81.2461670707101));
#223801=CARTESIAN_POINT('Ctrl Pts',(7.41944643263451,-2.74528943518467,
81.2473530695204));
#223802=CARTESIAN_POINT('Ctrl Pts',(7.45515230772397,-2.64766816042951,
81.251506095322));
#223803=CARTESIAN_POINT('Ctrl Pts',(7.47969283879862,-2.57752551596964,
81.2544632161534));
#223804=CARTESIAN_POINT('Ctrl Pts',(7.73162887285294,-1.82351618160533,
81.285991052157));
#223805=CARTESIAN_POINT('Ctrl Pts',(7.86556005425078,-1.1119223363754,81.3137087882593));
#223806=CARTESIAN_POINT('Ctrl Pts',(7.91457622043815,-0.12407446912366,
81.3508654404041));
#223807=CARTESIAN_POINT('Ctrl Pts',(7.91423131011837,0.144407793103972,
81.3608545458554));
#223808=CARTESIAN_POINT('Ctrl Pts',(7.88798191323639,0.647319257892521,
81.3797418201335));
#223809=CARTESIAN_POINT('Ctrl Pts',(7.86524170847977,0.881616976885259,
81.3886154158048));
#223810=CARTESIAN_POINT('Ctrl Pts',(7.81289836057658,1.24944215341381,81.4029721490455));
#223811=CARTESIAN_POINT('Ctrl Pts',(7.79022055809496,1.38381651902715,81.4083089711112));
#223812=CARTESIAN_POINT('Ctrl Pts',(7.76081282121446,1.53427385930797,81.4144389491362));
#223813=CARTESIAN_POINT('Ctrl Pts',(7.75748684524419,1.55100282472295,81.415122692386));
#223814=CARTESIAN_POINT('Ctrl Pts',(7.75241838394963,1.5760719501794,81.4161507033002));
#223815=CARTESIAN_POINT('Ctrl Pts',(7.75071647337759,1.5844203169084,81.4164936097246));
#223816=CARTESIAN_POINT('Ctrl Pts',(7.74776985141665,1.59875599346317,81.4170834329636));
#223817=CARTESIAN_POINT('Ctrl Pts',(7.74653167617132,1.60474464853645,81.4173301256056));
#223818=CARTESIAN_POINT('Ctrl Pts',(7.74397055468193,1.61705993231343,81.4178380531386));
#223819=CARTESIAN_POINT('Ctrl Pts',(7.74264679672763,1.62338638570648,81.418099316106));
#223820=CARTESIAN_POINT('Ctrl Pts',(7.73944697959424,1.63858588443645,81.4187278303027));
#223821=CARTESIAN_POINT('Ctrl Pts',(7.73756341483344,1.64745732911463,81.4190953467729));
#223822=CARTESIAN_POINT('Ctrl Pts',(7.73064700683451,1.67975956243382,81.4204360341884));
#223823=CARTESIAN_POINT('Ctrl Pts',(7.72552298428528,1.70317055389527,81.4214125007712));
#223824=CARTESIAN_POINT('Ctrl Pts',(7.64656598108964,2.05622632553145,81.4362149782184));
#223825=CARTESIAN_POINT('Ctrl Pts',(7.55181638850403,2.38076000285328,81.4510147315965));
#223826=CARTESIAN_POINT('Ctrl Pts',(7.30787984703686,3.05308762090558,81.4833146319153));
#223827=CARTESIAN_POINT('Ctrl Pts',(7.15387658658543,3.39830899248751,81.5008054031428));
#223828=CARTESIAN_POINT('Ctrl Pts',(6.818780190892,4.02479919207307,81.5331039380034));
#223829=CARTESIAN_POINT('Ctrl Pts',(6.64336259496362,4.30819370359075,81.5479546116735));
#223830=CARTESIAN_POINT('Ctrl Pts',(6.32950281334622,4.75027057655303,81.5711917709364));
#223831=CARTESIAN_POINT('Ctrl Pts',(6.20168673598109,4.91597056960559,81.5799241509856));
#223832=CARTESIAN_POINT('Ctrl Pts',(6.05283955405643,5.09387597567603,81.5893233840186));
#223833=CARTESIAN_POINT('Ctrl Pts',(6.03815782714681,5.11127079974586,81.5902426988214));
#223834=CARTESIAN_POINT('Ctrl Pts',(6.01692753983949,5.13620518424576,81.5915609456116));
#223835=CARTESIAN_POINT('Ctrl Pts',(6.0104395261145,5.14379601249999,81.5919623250743));
#223836=CARTESIAN_POINT('Ctrl Pts',(5.99914929265777,5.15695480172843,81.592658234461));
#223837=CARTESIAN_POINT('Ctrl Pts',(5.99435365794574,5.16252838118148,81.5929530315727));
#223838=CARTESIAN_POINT('Ctrl Pts',(5.98511436853565,5.17323623102756,81.5935194602497));
#223839=CARTESIAN_POINT('Ctrl Pts',(5.98067186198861,5.17837148010471,81.5937911381978));
#223840=CARTESIAN_POINT('Ctrl Pts',(5.97018627942039,5.19046064086167,81.5944307853124));
#223841=CARTESIAN_POINT('Ctrl Pts',(5.96413765049933,5.19740973581731,81.5947985266634));
#223842=CARTESIAN_POINT('Ctrl Pts',(5.94316376480033,5.22142120030768,81.5960694101149));
#223843=CARTESIAN_POINT('Ctrl Pts',(5.92817725401173,5.23843004555065,81.5969700307434));
#223844=CARTESIAN_POINT('Ctrl Pts',(5.75659028637497,5.43149221051784,81.6071974000554));
#223845=CARTESIAN_POINT('Ctrl Pts',(5.59226673986383,5.6005359629502,81.6161920728563));
#223846=CARTESIAN_POINT('Ctrl Pts',(5.28906469099099,5.88577485801962,81.6315777226181));
#223847=CARTESIAN_POINT('Ctrl Pts',(5.15329268966539,6.00500867541816,81.6380830008919));
#223848=CARTESIAN_POINT('Ctrl Pts',(4.56284328516325,6.48874966564526,81.6650464799613));
#223849=CARTESIAN_POINT('Ctrl Pts',(4.07274610511969,6.80706311478944,81.6841219929992));
#223850=CARTESIAN_POINT('Ctrl Pts',(3.38322563201565,7.15356210590033,81.7112001400796));
#223851=CARTESIAN_POINT('Ctrl Pts',(3.2113093555447,7.23236840931404,81.7179830039537));
#223852=CARTESIAN_POINT('Ctrl Pts',(2.94502523962398,7.34306566051393,81.7287516512723));
#223853=CARTESIAN_POINT('Ctrl Pts',(2.85260022555226,7.37946187871021,81.7325363168097));
#223854=CARTESIAN_POINT('Ctrl Pts',(2.70744972211006,7.43348664039645,81.738585643333));
#223855=CARTESIAN_POINT('Ctrl Pts',(2.65518030475908,7.45231674756735,81.740785086895));
#223856=CARTESIAN_POINT('Ctrl Pts',(2.59406797067548,7.47360798207317,81.7433853837973));
#223857=CARTESIAN_POINT('Ctrl Pts',(2.58541268416741,7.47660659373052,81.7437543301238));
#223858=CARTESIAN_POINT('Ctrl Pts',(2.57222145259777,7.48115103197362,81.7443176718346));
#223859=CARTESIAN_POINT('Ctrl Pts',(2.567689253967,7.48270778924813,81.7445114101748));
#223860=CARTESIAN_POINT('Ctrl Pts',(2.55981769004762,7.48540358581523,81.7448482259304));
#223861=CARTESIAN_POINT('Ctrl Pts',(2.55647896775854,7.48654451240003,81.7449911890297));
#223862=CARTESIAN_POINT('Ctrl Pts',(2.54953076460418,7.48891370075458,81.7452889247662));
#223863=CARTESIAN_POINT('Ctrl Pts',(2.54592115754027,7.49014158721355,81.7454437202009));
#223864=CARTESIAN_POINT('Ctrl Pts',(2.53711168708902,7.49313121662858,81.7458218062986));
#223865=CARTESIAN_POINT('Ctrl Pts',(2.53191088156307,7.49489015462524,81.7460452685698));
#223866=CARTESIAN_POINT('Ctrl Pts',(2.5118890539416,7.50163841684503,81.7469065320414));
#223867=CARTESIAN_POINT('Ctrl Pts',(2.4970553860401,7.50658910167934,81.7475467264879));
#223868=CARTESIAN_POINT('Ctrl Pts',(2.23647118891562,7.59270031099475,81.7588290508521));
#223869=CARTESIAN_POINT('Ctrl Pts',(1.98691753267487,7.66179073754788,81.7701887889786));
#223870=CARTESIAN_POINT('Ctrl Pts',(1.69341242801769,7.72774511815841,81.7837912253489));
#223871=CARTESIAN_POINT('Ctrl Pts',(1.65230067566767,7.73663962438062,81.7857020905813));
#223872=CARTESIAN_POINT('Ctrl Pts',(1.61095367510114,7.74524042787896,81.7876281357673));
#223873=CARTESIAN_POINT('Ctrl Pts',(1.61078702816548,7.74527508735915,81.7876358986615));
#223874=CARTESIAN_POINT('Ctrl Pts',(1.61027838362078,7.74538085889022,81.7876595930001));
#223875=CARTESIAN_POINT('Ctrl Pts',(1.60993638246581,7.74545195365849,81.7876755248316));
#223876=CARTESIAN_POINT('Ctrl Pts',(1.60891396167713,7.74566442255782,81.7877231542983));
#223877=CARTESIAN_POINT('Ctrl Pts',(1.60823352819894,7.74580572966649,81.7877548534371));
#223878=CARTESIAN_POINT('Ctrl Pts',(1.60627654705985,7.74621187123596,81.7878460259853));
#223879=CARTESIAN_POINT('Ctrl Pts',(1.60499995277116,7.74647647974964,81.7879055044472));
#223880=CARTESIAN_POINT('Ctrl Pts',(1.60154968021547,7.74719075206476,81.7880662686424));
#223881=CARTESIAN_POINT('Ctrl Pts',(1.59937587860581,7.74763981648615,81.7881675676888));
#223882=CARTESIAN_POINT('Ctrl Pts',(1.59394343081634,7.74875966901115,81.788420747875));
#223883=CARTESIAN_POINT('Ctrl Pts',(1.59068455102749,7.74942931626785,81.7885726540629));
#223884=CARTESIAN_POINT('Ctrl Pts',(1.58311676995922,7.75097939840382,81.7889254688787));
#223885=CARTESIAN_POINT('Ctrl Pts',(1.57880755640599,7.7518582960204,81.789126410662));
#223886=CARTESIAN_POINT('Ctrl Pts',(1.56931133234322,7.7537868779784,81.7895693191143));
#223887=CARTESIAN_POINT('Ctrl Pts',(1.56412399828654,7.75483495148737,81.7898113196925));
#223888=CARTESIAN_POINT('Ctrl Pts',(1.5530331485394,7.7570642182638,81.7903288568955));
#223889=CARTESIAN_POINT('Ctrl Pts',(1.54712932940918,7.75824387891118,81.7906044248241));
#223890=CARTESIAN_POINT('Ctrl Pts',(1.53461513075224,7.7607295277699,81.7911886921897));
#223891=CARTESIAN_POINT('Ctrl Pts',(1.52800441885909,7.76203381196496,81.791497425244));
#223892=CARTESIAN_POINT('Ctrl Pts',(1.09765160112955,7.8463707388102,81.811601242663));
#223893=CARTESIAN_POINT('Ctrl Pts',(0.667820828851879,7.89458090532381,
81.8319728907238));
#223894=CARTESIAN_POINT('Ctrl Pts',(-0.0271539508753081,7.91533926038405,
81.8637145230358));
#223895=CARTESIAN_POINT('Ctrl Pts',(-0.290739402635426,7.91004548402641,
81.8754903903777));
#223896=CARTESIAN_POINT('Ctrl Pts',(-0.778609303229863,7.87582208437207,
81.8966102169183));
#223897=CARTESIAN_POINT('Ctrl Pts',(-1.0028658017784,7.85041897234444,81.9060521923009));
#223898=CARTESIAN_POINT('Ctrl Pts',(-1.24674586899656,7.81216984187532,
81.9160272586093));
#223899=CARTESIAN_POINT('Ctrl Pts',(-1.26773384431033,7.8087914436263,81.9168833484167));
#223900=CARTESIAN_POINT('Ctrl Pts',(-1.29781473948881,7.80382490156138,
81.9181069985101));
#223901=CARTESIAN_POINT('Ctrl Pts',(-1.30691879835144,7.80230539312487,
81.9184769006093));
#223902=CARTESIAN_POINT('Ctrl Pts',(-1.32268504658034,7.7996455657929,81.9191167345214));
#223903=CARTESIAN_POINT('Ctrl Pts',(-1.32934846189865,7.79851263713773,
81.9193869185405));
#223904=CARTESIAN_POINT('Ctrl Pts',(-1.34213685063274,7.79632146009281,
81.9199050066194));
#223905=CARTESIAN_POINT('Ctrl Pts',(-1.34826204245178,7.79526453047266,
81.9201529555133));
#223906=CARTESIAN_POINT('Ctrl Pts',(-1.36265548076988,7.79276340524096,
81.9207351428442));
#223907=CARTESIAN_POINT('Ctrl Pts',(-1.37092269549307,7.79131326625609,
81.9210691777513));
#223908=CARTESIAN_POINT('Ctrl Pts',(-1.39932843396219,7.78628404970597,
81.9222156805535));
#223909=CARTESIAN_POINT('Ctrl Pts',(-1.41945546002415,7.78264001316065,
81.9230259241));
#223910=CARTESIAN_POINT('Ctrl Pts',(-1.63773325234848,7.74224547781596,
81.9317903944476));
#223911=CARTESIAN_POINT('Ctrl Pts',(-1.8344318129604,7.69801290440657,81.9394828332048));
#223912=CARTESIAN_POINT('Ctrl Pts',(-2.68966166940109,7.47104552090079,
81.9722470607308));
#223913=CARTESIAN_POINT('Ctrl Pts',(-3.32453706002264,7.21097903172215,
81.9944509037068));
#223914=CARTESIAN_POINT('Ctrl Pts',(-4.09183705892401,6.77353533795482,
82.0247386285417));
#223915=CARTESIAN_POINT('Ctrl Pts',(-4.26173987697471,6.66794411905766,
82.0317167529024));
#223916=CARTESIAN_POINT('Ctrl Pts',(-4.54824429813732,6.47446057082404,
82.044274005449));
#223917=CARTESIAN_POINT('Ctrl Pts',(-4.66675292640679,6.38956798004194,
82.0497176262539));
#223918=CARTESIAN_POINT('Ctrl Pts',(-4.83103586247086,6.26487621872617,
82.0577285895207));
#223919=CARTESIAN_POINT('Ctrl Pts',(-4.87880620038059,6.22774688153805,
82.0601158307149));
#223920=CARTESIAN_POINT('Ctrl Pts',(-4.93309294665807,6.1845447555156,82.0629017841679));
#223921=CARTESIAN_POINT('Ctrl Pts',(-4.94003183833697,6.17900358377093,
82.0632592678746));
#223922=CARTESIAN_POINT('Ctrl Pts',(-4.95051747999784,6.17060114142821,
82.0638016008171));
#223923=CARTESIAN_POINT('Ctrl Pts',(-4.95407111546102,6.16774846673863,
82.0639857710088));
#223924=CARTESIAN_POINT('Ctrl Pts',(-4.96051487157396,6.16256659086966,
82.0643203957692));
#223925=CARTESIAN_POINT('Ctrl Pts',(-4.96340582233012,6.16023842239672,
82.0644707686589));
#223926=CARTESIAN_POINT('Ctrl Pts',(-4.96961807384124,6.15522829991797,
82.0647944253526));
#223927=CARTESIAN_POINT('Ctrl Pts',(-4.9729388428885,6.15254569172029,82.0649677604811));
#223928=CARTESIAN_POINT('Ctrl Pts',(-4.98185196334507,6.14533349843203,
82.0654338677595));
#223929=CARTESIAN_POINT('Ctrl Pts',(-4.98744029594451,6.14079897776614,
82.0657270244584));
#223930=CARTESIAN_POINT('Ctrl Pts',(-5.01285540452236,6.120118910123,82.0670644182324));
#223931=CARTESIAN_POINT('Ctrl Pts',(-5.03260980985598,6.10388509493277,
82.068115453591));
#223932=CARTESIAN_POINT('Ctrl Pts',(-5.36505351018126,5.82797793232107,
82.0859932118389));
#223933=CARTESIAN_POINT('Ctrl Pts',(-5.6573215476664,5.54470645178441,82.1045432310019));
#223934=CARTESIAN_POINT('Ctrl Pts',(-6.29108301346846,4.82795255213831,
82.149180758206));
#223935=CARTESIAN_POINT('Ctrl Pts',(-6.61167625526668,4.37866205571579,
82.1754013955193));
#223936=CARTESIAN_POINT('Ctrl Pts',(-7.052285985175,3.60098211660418,82.2154878805488));
#223937=CARTESIAN_POINT('Ctrl Pts',(-7.20192362117619,3.29152650347996,
82.2302808829215));
#223938=CARTESIAN_POINT('Ctrl Pts',(-7.34983305079788,2.92683930140138,
82.2463896059893));
#223939=CARTESIAN_POINT('Ctrl Pts',(-7.36823286280451,2.88020464142071,
82.2484260781635));
#223940=CARTESIAN_POINT('Ctrl Pts',(-7.39090328854906,2.82110667597188,
82.2509778313498));
#223941=CARTESIAN_POINT('Ctrl Pts',(-7.39558752059712,2.80880393145235,
82.251507467849));
#223942=CARTESIAN_POINT('Ctrl Pts',(-7.40300090621415,2.78918617846562,
82.2523495235542));
#223943=CARTESIAN_POINT('Ctrl Pts',(-7.40574996725616,2.78187874978493,
82.2526626312999));
#223944=CARTESIAN_POINT('Ctrl Pts',(-7.410911812419,2.76809589083751,82.2532521647126));
#223945=CARTESIAN_POINT('Ctrl Pts',(-7.41332693729977,2.76162134865589,
82.2535286709953));
#223946=CARTESIAN_POINT('Ctrl Pts',(-7.41874206089802,2.74704602367712,
82.2541501734305));
#223947=CARTESIAN_POINT('Ctrl Pts',(-7.42173728296416,2.73894346886283,
82.254495004814));
#223948=CARTESIAN_POINT('Ctrl Pts',(-7.42932948898273,2.71830143913055,
82.2553718045485));
#223949=CARTESIAN_POINT('Ctrl Pts',(-7.43390800975065,2.70575517641983,
82.2559031383485));
#223950=CARTESIAN_POINT('Ctrl Pts',(-7.45920301797278,2.63589183168084,
82.2588530913417));
#223951=CARTESIAN_POINT('Ctrl Pts',(-7.47928865541226,2.57834769465273,
82.261250098861));
#223952=CARTESIAN_POINT('Ctrl Pts',(-7.77234805148472,1.70649680452938,
82.2970931324115));
#223953=CARTESIAN_POINT('Ctrl Pts',(-7.91157906642316,0.853414248781925,
82.3251486570467));
#223954=CARTESIAN_POINT('Ctrl Pts',(-7.91077331315912,-0.3378085693112,
82.3672811834467));
#223955=CARTESIAN_POINT('Ctrl Pts',(-7.88959213361958,-0.669922515704042,
82.3794870143087));
#223956=CARTESIAN_POINT('Ctrl Pts',(-7.84479873300275,-1.02153659819372,
82.3936223337489));
#223957=CARTESIAN_POINT('Ctrl Pts',(-7.84193003947626,-1.04332996965621,
82.3945027533589));
#223958=CARTESIAN_POINT('Ctrl Pts',(-7.83788396125921,-1.07310817072276,
82.3957114153547));
#223959=CARTESIAN_POINT('Ctrl Pts',(-7.83678511378554,-1.08110370269847,
82.3960365037062));
#223960=CARTESIAN_POINT('Ctrl Pts',(-7.83489317745713,-1.09471551989898,
82.3965908824659));
#223961=CARTESIAN_POINT('Ctrl Pts',(-7.83410627899595,-1.10033266825351,
82.3968199288134));
#223962=CARTESIAN_POINT('Ctrl Pts',(-7.83257208771091,-1.11119917435111,
82.3972635465748));
#223963=CARTESIAN_POINT('Ctrl Pts',(-7.83182555668265,-1.11644863911374,
82.3974780883156));
#223964=CARTESIAN_POINT('Ctrl Pts',(-7.83004073379113,-1.1289092906493,
82.3979879008959));
#223965=CARTESIAN_POINT('Ctrl Pts',(-7.82899775775516,-1.13611979472033,
82.3982833514167));
#223966=CARTESIAN_POINT('Ctrl Pts',(-7.82588979960558,-1.15739882156305,
82.3991565465952));
#223967=CARTESIAN_POINT('Ctrl Pts',(-7.82379685209385,-1.17146318834051,
82.3997353455173));
#223968=CARTESIAN_POINT('Ctrl Pts',(-7.80717755231707,-1.28111162705549,
82.4042604073615));
#223969=CARTESIAN_POINT('Ctrl Pts',(-7.79093831936637,-1.37642564016029,
82.4082687695339));
#223970=CARTESIAN_POINT('Ctrl Pts',(-7.72630650776583,-1.71785212681102,
82.4228522917019));
#223971=CARTESIAN_POINT('Ctrl Pts',(-7.66796435740848,-1.96192317875596,
82.4336964550047));
#223972=CARTESIAN_POINT('Ctrl Pts',(-7.4223711763198,-2.80904870025764,
82.4721764003748));
#223973=CARTESIAN_POINT('Ctrl Pts',(-7.17466700541084,-3.39213933116439,
82.4999977809956));
#223974=CARTESIAN_POINT('Ctrl Pts',(-6.75825811163003,-4.11726198080747,
82.5349523138276));
#223975=CARTESIAN_POINT('Ctrl Pts',(-6.64936149261017,-4.29090844788996,
82.5433753329582));
#223976=CARTESIAN_POINT('Ctrl Pts',(-6.51427612181203,-4.48880074467213,
82.5530676090506));
#223977=CARTESIAN_POINT('Ctrl Pts',(-6.49452061189002,-4.51733633497682,
82.5544676689171));
#223978=CARTESIAN_POINT('Ctrl Pts',(-6.46504753216663,-4.55931535381337,
82.5565309620976));
#223979=CARTESIAN_POINT('Ctrl Pts',(-6.45547447802529,-4.57285964738681,
82.557197235464));
#223980=CARTESIAN_POINT('Ctrl Pts',(-6.43843094884148,-4.59681325202846,
82.558376561052));
#223981=CARTESIAN_POINT('Ctrl Pts',(-6.4309776560482,-4.60723469616784,
82.5588899836728));
#223982=CARTESIAN_POINT('Ctrl Pts',(-6.4153071872829,-4.62903355553002,
82.5599646293773));
#223983=CARTESIAN_POINT('Ctrl Pts',(-6.40708498356156,-4.64040730759268,
82.5605257390872));
#223984=CARTESIAN_POINT('Ctrl Pts',(-6.38547731826575,-4.67013022050076,
82.5619931399957));
#223985=CARTESIAN_POINT('Ctrl Pts',(-6.37204300111364,-4.68844375640407,
82.562898327873));
#223986=CARTESIAN_POINT('Ctrl Pts',(-6.31221779763707,-4.76926480087159,
82.5668978200427));
#223987=CARTESIAN_POINT('Ctrl Pts',(-6.2649842569111,-4.83114404586901,
82.5699724868492));
#223988=CARTESIAN_POINT('Ctrl Pts',(-5.7541423162739,-5.4802894499713,82.6023693136571));
#223989=CARTESIAN_POINT('Ctrl Pts',(-5.21040549354036,-5.99961446857308,
82.6289908979123));
#223990=CARTESIAN_POINT('Ctrl Pts',(-4.33742871092313,-6.62391840200282,
82.6683845693374));
#223991=CARTESIAN_POINT('Ctrl Pts',(-4.06163996236525,-6.79651639335913,
82.6805235458911));
#223992=CARTESIAN_POINT('Ctrl Pts',(-3.7599676482456,-6.96038065463423,
82.6942251026017));
#223993=CARTESIAN_POINT('Ctrl Pts',(-3.74386431908072,-6.96905556913394,
82.6949577583295));
#223994=CARTESIAN_POINT('Ctrl Pts',(-3.72163497689141,-6.98093130382919,
82.6959710565294));
#223995=CARTESIAN_POINT('Ctrl Pts',(-3.71553455623929,-6.98418010442027,
82.6962493362241));
#223996=CARTESIAN_POINT('Ctrl Pts',(-3.70508418523015,-6.98972791945096,
82.6967263988581));
#223997=CARTESIAN_POINT('Ctrl Pts',(-3.70073632720209,-6.9920308812205,
82.6969249844896));
#223998=CARTESIAN_POINT('Ctrl Pts',(-3.69227288228109,-6.99650367033614,
82.6973117555037));
#223999=CARTESIAN_POINT('Ctrl Pts',(-3.68815752419057,-6.99867392602734,
82.6974999190925));
#224000=CARTESIAN_POINT('Ctrl Pts',(-3.67830953709404,-7.00385621531218,
82.6979504261005));
#224001=CARTESIAN_POINT('Ctrl Pts',(-3.67257512548434,-7.00686483976604,
82.6982129429197));
#224002=CARTESIAN_POINT('Ctrl Pts',(-3.65536729800244,-7.01586619520672,
82.6990012909677));
#224003=CARTESIAN_POINT('Ctrl Pts',(-3.6438829015453,-7.02183778999953,
82.6995282115491));
#224004=CARTESIAN_POINT('Ctrl Pts',(-3.53080063714065,-7.0802855695115,
82.7047247516858));
#224005=CARTESIAN_POINT('Ctrl Pts',(-3.42810174862639,-7.1305757784351,
82.7095163738962));
#224006=CARTESIAN_POINT('Ctrl Pts',(-3.21542307986974,-7.22906539100864,
82.7195496061427));
#224007=CARTESIAN_POINT('Ctrl Pts',(-3.10536024016603,-7.27702328033204,
82.7247983650968));
#224008=CARTESIAN_POINT('Ctrl Pts',(-2.50267359694306,-7.5234701060025,
82.7536976899882));
#224009=CARTESIAN_POINT('Ctrl Pts',(-1.99210882143967,-7.67446935100861,
82.778659208289));
#224010=CARTESIAN_POINT('Ctrl Pts',(-0.946833949408674,-7.87217987137696,
82.8271596900419));
#224011=CARTESIAN_POINT('Ctrl Pts',(-0.414682023245925,-7.91807321898009,
82.8505449018719));
#224012=CARTESIAN_POINT('Ctrl Pts',(0.151558302360977,-7.90961886281755,
82.8736131146609));
#224013=CARTESIAN_POINT('Ctrl Pts',(0.185009860855236,-7.90890712171439,
82.8749696798301));
#224014=CARTESIAN_POINT('Ctrl Pts',(0.230794097781978,-7.90764234303347,
82.8768179816804));
#224015=CARTESIAN_POINT('Ctrl Pts',(0.243131256760908,-7.90727263565717,
82.8773151965656));
#224016=CARTESIAN_POINT('Ctrl Pts',(0.262700212086144,-7.90664037153556,
82.8781025546574));
#224017=CARTESIAN_POINT('Ctrl Pts',(0.269932576694688,-7.9063967627866,
82.8783932644828));
#224018=CARTESIAN_POINT('Ctrl Pts',(0.283950964554022,-7.90590532203296,
82.8789561934256));
#224019=CARTESIAN_POINT('Ctrl Pts',(0.290737021961011,-7.90565867563084,
82.8792284477929));
#224020=CARTESIAN_POINT('Ctrl Pts',(0.306885877416345,-7.90505090750927,
82.8798757426573));
#224021=CARTESIAN_POINT('Ctrl Pts',(0.316248377168858,-7.90468188839704,
82.8802505463851));
#224022=CARTESIAN_POINT('Ctrl Pts',(0.344024687195734,-7.90353766883258,
82.8813611034298));
#224023=CARTESIAN_POINT('Ctrl Pts',(0.362436523467322,-7.90271475128366,
82.882095427242));
#224024=CARTESIAN_POINT('Ctrl Pts',(0.510761194825826,-7.89556592808002,
82.8879966098208));
#224025=CARTESIAN_POINT('Ctrl Pts',(0.640506041467702,-7.88610120546517,
82.8930685798915));
#224026=CARTESIAN_POINT('Ctrl Pts',(1.08603635849855,-7.84253174683352,
82.9102141535868));
#224027=CARTESIAN_POINT('Ctrl Pts',(1.39997485186861,-7.79261632392008,
82.9218126748684));
#224028=CARTESIAN_POINT('Ctrl Pts',(1.97567957711024,-7.66515578786913,
82.9427285896526));
#224029=CARTESIAN_POINT('Ctrl Pts',(2.23807488375363,-7.59269042865542,
82.9521242474289));
#224030=CARTESIAN_POINT('Ctrl Pts',(2.7822979240428,-7.41172251067891,82.9719142542052));
#224031=CARTESIAN_POINT('Ctrl Pts',(3.06269904234073,-7.30032038348587,
82.9822910784481));
#224032=CARTESIAN_POINT('Ctrl Pts',(3.60758530853732,-7.04690912909354,
83.0037826169518));
#224033=CARTESIAN_POINT('Ctrl Pts',(3.8717289957021,-6.90531092995292,83.0149021430282));
#224034=CARTESIAN_POINT('Ctrl Pts',(4.1453031290591,-6.73801398379112,83.0276694023004));
#224035=CARTESIAN_POINT('Ctrl Pts',(4.1633454950578,-6.72688075969151,83.028516896351));
#224036=CARTESIAN_POINT('Ctrl Pts',(4.18823199666722,-6.71138581832311,
83.0296932621845));
#224037=CARTESIAN_POINT('Ctrl Pts',(4.19511459772902,-6.70708583302821,
83.0300193821187));
#224038=CARTESIAN_POINT('Ctrl Pts',(4.20691627733504,-6.69968732357613,
83.03057991696));
#224039=CARTESIAN_POINT('Ctrl Pts',(4.21183858729832,-6.69659394860776,
83.0308141068948));
#224040=CARTESIAN_POINT('Ctrl Pts',(4.22143209266467,-6.6905502472934,83.0312713118254));
#224041=CARTESIAN_POINT('Ctrl Pts',(4.22610361662003,-6.68760044753913,
83.0314943040955));
#224042=CARTESIAN_POINT('Ctrl Pts',(4.23730904450276,-6.68050843209629,
83.0320300413071));
#224043=CARTESIAN_POINT('Ctrl Pts',(4.24383996404174,-6.67636152474065,
83.0323429852616));
#224044=CARTESIAN_POINT('Ctrl Pts',(4.26354620584603,-6.66380814615335,
83.0332893405968));
#224045=CARTESIAN_POINT('Ctrl Pts',(4.27670266951694,-6.65537223081037,
83.0339239760548));
#224046=CARTESIAN_POINT('Ctrl Pts',(4.40033962514064,-6.57557830868276,
83.0399139586767));
#224047=CARTESIAN_POINT('Ctrl Pts',(4.50904673191947,-6.50151632875985,
83.0453764135102));
#224048=CARTESIAN_POINT('Ctrl Pts',(4.81775263480765,-6.27972803232172,
83.061368059381));
#224049=CARTESIAN_POINT('Ctrl Pts',(5.01269815945171,-6.12524096805037,
83.0720649522018));
#224050=CARTESIAN_POINT('Ctrl Pts',(5.49539747835406,-5.7042202377735,83.0997192224108));
#224051=CARTESIAN_POINT('Ctrl Pts',(5.77121007323627,-5.42500431346597,
83.1166648191338));
#224052=CARTESIAN_POINT('Ctrl Pts',(6.2832098679501,-4.82324834506387,83.1501402722954));
#224053=CARTESIAN_POINT('Ctrl Pts',(6.51796769969943,-4.50095162963353,
83.1666099030009));
#224054=CARTESIAN_POINT('Ctrl Pts',(6.82855019362817,-3.99896638413514,
83.1907340465467));
#224055=CARTESIAN_POINT('Ctrl Pts',(6.92364858310609,-3.83196057614499,
83.1985522584594));
#224056=CARTESIAN_POINT('Ctrl Pts',(7.03452778330465,-3.61961182303977,
83.2082383304687));
#224057=CARTESIAN_POINT('Ctrl Pts',(7.05610389450611,-3.57736896889967,
83.2101529161304));
#224058=CARTESIAN_POINT('Ctrl Pts',(7.08959355692613,-3.51031925443538,
83.2131725775974));
#224059=CARTESIAN_POINT('Ctrl Pts',(7.10175978056362,-3.48563998356122,
83.2142799568727));
#224060=CARTESIAN_POINT('Ctrl Pts',(7.12332588765428,-3.44131133771696,
83.2162617613255));
#224061=CARTESIAN_POINT('Ctrl Pts',(7.13277383303186,-3.42168567731919,
83.2171366351646));
#224062=CARTESIAN_POINT('Ctrl Pts',(7.15465770366415,-3.37574308283499,
83.2191787923347));
#224063=CARTESIAN_POINT('Ctrl Pts',(7.16702968930932,-3.34939601377875,
83.2203454429381));
#224064=CARTESIAN_POINT('Ctrl Pts',(7.20091579904378,-3.27618553159718,
83.2235749298959));
#224065=CARTESIAN_POINT('Ctrl Pts',(7.22211761118548,-3.2291790334804,83.2256346217858));
#224066=CARTESIAN_POINT('Ctrl Pts',(7.36620075273548,-2.90121418707225,
83.2399112293772));
#224067=CARTESIAN_POINT('Ctrl Pts',(7.47311635429268,-2.61352176066586,
83.2519484734084));
#224068=CARTESIAN_POINT('Ctrl Pts',(7.67367808667517,-1.95979955702333,
83.2785494734345));
#224069=CARTESIAN_POINT('Ctrl Pts',(7.75836933962422,-1.5918080378604,83.2930178503985));
#224070=CARTESIAN_POINT('Ctrl Pts',(7.85153372898945,-0.994508137693976,
83.3165228182334));
#224071=CARTESIAN_POINT('Ctrl Pts',(7.87687360764529,-0.76843067980944,
83.3254296696135));
#224072=CARTESIAN_POINT('Ctrl Pts',(7.89425818301156,-0.515086468564058,
83.3355914905457));
#224073=CARTESIAN_POINT('Ctrl Pts',(7.8959428886597,-0.488581843384374,
83.3366568372539));
#224074=CARTESIAN_POINT('Ctrl Pts',(7.89825431245943,-0.449075964246679,
83.3382484730032));
#224075=CARTESIAN_POINT('Ctrl Pts',(7.89898246499564,-0.436080751931087,
83.3387726290335));
#224076=CARTESIAN_POINT('Ctrl Pts',(7.90019066843466,-0.413521584896281,
83.3396836335847));
#224077=CARTESIAN_POINT('Ctrl Pts',(7.90068543116149,-0.403958433553598,
83.3400701614623));
#224078=CARTESIAN_POINT('Ctrl Pts',(7.90163211961558,-0.384992801212348,
83.3408374222254));
#224079=CARTESIAN_POINT('Ctrl Pts',(7.90208462927214,-0.375590364586619,
83.3412181414479));
#224080=CARTESIAN_POINT('Ctrl Pts',(7.90324148151608,-0.350624856639488,
83.3422299693235));
#224081=CARTESIAN_POINT('Ctrl Pts',(7.90391663223043,-0.335060554196697,
83.3428617450956));
#224082=CARTESIAN_POINT('Ctrl Pts',(7.9064881195928,-0.271439889146017,
83.3454483171678));
#224083=CARTESIAN_POINT('Ctrl Pts',(7.90799216933934,-0.223369143930525,
83.3474121728015));
#224084=CARTESIAN_POINT('Ctrl Pts',(7.91658069307538,0.164147980571805,
83.3633103526081));
#224085=CARTESIAN_POINT('Ctrl Pts',(7.90224410556563,0.503710038774721,
83.3776387815922));
#224086=CARTESIAN_POINT('Ctrl Pts',(7.81439987833045,1.32506035679555,83.4124861127088));
#224087=CARTESIAN_POINT('Ctrl Pts',(7.7181407126294,1.80304461020453,83.4328809339111));
#224088=CARTESIAN_POINT('Ctrl Pts',(7.55765683534286,2.33903039394703,83.4556716194591));
#224089=CARTESIAN_POINT('Ctrl Pts',(7.53577208895681,2.40860523768575,83.4586301650926));
#224090=CARTESIAN_POINT('Ctrl Pts',(7.50445571268423,2.50355690193685,83.4626696701596));
#224091=CARTESIAN_POINT('Ctrl Pts',(7.49585142908382,2.5292022586484,83.4637608858997));
#224092=CARTESIAN_POINT('Ctrl Pts',(7.48091545657614,2.57297367792859,83.4656238310926));
#224093=CARTESIAN_POINT('Ctrl Pts',(7.47464901457149,2.59112171216366,83.4663963617202));
#224094=CARTESIAN_POINT('Ctrl Pts',(7.46166049499911,2.62829810204554,83.4679792393806));
#224095=CARTESIAN_POINT('Ctrl Pts',(7.45493154605436,2.64732391338453,83.4687894955948));
#224096=CARTESIAN_POINT('Ctrl Pts',(7.43920460010276,2.69125568777074,83.4706609431245));
#224097=CARTESIAN_POINT('Ctrl Pts',(7.43015419298055,2.71614265716186,83.471721486329));
#224098=CARTESIAN_POINT('Ctrl Pts',(7.40220261246189,2.79181916922449,83.4749478519308));
#224099=CARTESIAN_POINT('Ctrl Pts',(7.38290431375928,2.84246050722346,83.4771088742181));
#224100=CARTESIAN_POINT('Ctrl Pts',(7.1747808307712,3.37218205102407,83.4997442403497));
#224101=CARTESIAN_POINT('Ctrl Pts',(6.9401150812684,3.83196190948123,83.5197918389516));
#224102=CARTESIAN_POINT('Ctrl Pts',(6.25104012678044,4.90820965896344,83.5686855664903));
#224103=CARTESIAN_POINT('Ctrl Pts',(5.74889553623901,5.48781111356882,83.5961851812145));
#224104=CARTESIAN_POINT('Ctrl Pts',(5.14831676399449,6.00663829463994,83.6270070190922));
#224105=CARTESIAN_POINT('Ctrl Pts',(5.1248987834675,6.0266310276842,83.6282068501316));
#224106=CARTESIAN_POINT('Ctrl Pts',(5.06348481828428,6.07844542350151,83.6313495925962));
#224107=CARTESIAN_POINT('Ctrl Pts',(5.02530570382728,6.11004744310652,83.6332995480799));
#224108=CARTESIAN_POINT('Ctrl Pts',(4.95557042497136,6.16667369841242,83.6368583374995));
#224109=CARTESIAN_POINT('Ctrl Pts',(4.92411519212769,6.19181978533826,83.6384625545024));
#224110=CARTESIAN_POINT('Ctrl Pts',(4.88267009232263,6.22443646260455,83.6405764886028));
#224111=CARTESIAN_POINT('Ctrl Pts',(4.8728523575697,6.23212535230677,83.6410772657497));
#224112=CARTESIAN_POINT('Ctrl Pts',(4.85766769709547,6.24395960364342,83.6418518785545));
#224113=CARTESIAN_POINT('Ctrl Pts',(4.85231353058334,6.2481213486893,83.6421250256679));
#224114=CARTESIAN_POINT('Ctrl Pts',(4.84163945601494,6.2563962148506,83.6426696153642));
#224115=CARTESIAN_POINT('Ctrl Pts',(4.83631964183338,6.26050944739533,83.6429410527959));
#224116=CARTESIAN_POINT('Ctrl Pts',(4.8246388371033,6.26951716719819,83.6435371118081));
#224117=CARTESIAN_POINT('Ctrl Pts',(4.81827563348594,6.27440876397808,83.6438618577877));
#224118=CARTESIAN_POINT('Ctrl Pts',(4.80010063547729,6.28833650976067,83.6447895561835));
#224119=CARTESIAN_POINT('Ctrl Pts',(4.78827082394726,6.29734902031241,83.6453935455298));
#224120=CARTESIAN_POINT('Ctrl Pts',(4.76180404865713,6.31739496778729,83.6467453569093));
#224121=CARTESIAN_POINT('Ctrl Pts',(4.74715403669076,6.32841097920356,83.6474939635037));
#224122=CARTESIAN_POINT('Ctrl Pts',(4.70181287381567,6.36225902863544,83.6498123002648));
#224123=CARTESIAN_POINT('Ctrl Pts',(4.67099458592989,6.38491924435384,83.6513900814732));
#224124=CARTESIAN_POINT('Ctrl Pts',(4.55854858534755,6.46634925450629,83.6571581378105));
#224125=CARTESIAN_POINT('Ctrl Pts',(4.4759739579674,6.52377901991802,83.6614207117391));
#224126=CARTESIAN_POINT('Ctrl Pts',(4.14493139596264,6.74477173448362,83.6785862126986));
#224127=CARTESIAN_POINT('Ctrl Pts',(3.88842867827139,6.89583250529151,83.6920230123419));
#224128=CARTESIAN_POINT('Ctrl Pts',(3.04749100116697,7.32921712540238,83.7352395680662));
#224129=CARTESIAN_POINT('Ctrl Pts',(2.43649411675311,7.55435760765001,83.7652022853264));
#224130=CARTESIAN_POINT('Ctrl Pts',(1.63809467658986,7.74144014381819,83.8000002643202));
#224131=CARTESIAN_POINT('Ctrl Pts',(1.47012438352523,7.77508769754772,83.8071066567348));
#224132=CARTESIAN_POINT('Ctrl Pts',(1.28053940133635,7.80670084080667,83.8148896763576));
#224133=CARTESIAN_POINT('Ctrl Pts',(1.25987814557453,7.8100618591148,83.8157347551638));
#224134=CARTESIAN_POINT('Ctrl Pts',(1.2304892191868,7.81472297229582,83.816932396698));
#224135=CARTESIAN_POINT('Ctrl Pts',(1.22177242510334,7.81609051854859,83.8172870675629));
#224136=CARTESIAN_POINT('Ctrl Pts',(1.20577640991618,7.81857266245478,83.8179369091646));
#224137=CARTESIAN_POINT('Ctrl Pts',(1.19849789029871,7.81969168421257,83.8182322180597));
#224138=CARTESIAN_POINT('Ctrl Pts',(1.18374433515528,7.82193885795055,83.8188300360461));
#224139=CARTESIAN_POINT('Ctrl Pts',(1.17626922318441,7.82306646165835,83.8191325277064));
#224140=CARTESIAN_POINT('Ctrl Pts',(1.15786330295216,7.82581597562434,83.8198763648368));
#224141=CARTESIAN_POINT('Ctrl Pts',(1.14693067603073,7.82742570314811,83.8203173285272));
#224142=CARTESIAN_POINT('Ctrl Pts',(1.10706399198377,7.83321038429453,83.8219222331473));
#224143=CARTESIAN_POINT('Ctrl Pts',(1.07811006236087,7.83724787942993,83.8230818668319));
#224144=CARTESIAN_POINT('Ctrl Pts',(0.662326208235594,7.89287931993071,
83.8396501980792));
#224145=CARTESIAN_POINT('Ctrl Pts',(0.272203034349274,7.91594391967045,
83.8541129800971));
#224146=CARTESIAN_POINT('Ctrl Pts',(-0.616048464188318,7.90268624582155,
83.8856154149718));
#224147=CARTESIAN_POINT('Ctrl Pts',(-1.11220543198012,7.84824572459026,
83.9021693582787));
#224148=CARTESIAN_POINT('Ctrl Pts',(-1.73247216290351,7.7201536336102,83.9239588351184));
#224149=CARTESIAN_POINT('Ctrl Pts',(-1.864267496859,7.68939122006654,83.9286588253206));
#224150=CARTESIAN_POINT('Ctrl Pts',(-2.24164075069757,7.59103569760671,
83.9424610574042));
#224151=CARTESIAN_POINT('Ctrl Pts',(-2.48481384750551,7.5149490078564,83.9517803870244));
#224152=CARTESIAN_POINT('Ctrl Pts',(-2.7754075646578,7.40837677864145,83.9638670844904));
#224153=CARTESIAN_POINT('Ctrl Pts',(-2.82673977489904,7.38894279485918,
83.9660391564227));
#224154=CARTESIAN_POINT('Ctrl Pts',(-2.88612109598342,7.36575214005795,
83.9685991231355));
#224155=CARTESIAN_POINT('Ctrl Pts',(-2.89437226758516,7.36251375176632,
83.9689559029708));
#224156=CARTESIAN_POINT('Ctrl Pts',(-2.90748101629529,7.35734343825061,
83.9695244445711));
#224157=CARTESIAN_POINT('Ctrl Pts',(-2.91234216869083,7.35542054682404,
83.9697356550837));
#224158=CARTESIAN_POINT('Ctrl Pts',(-2.92089020079191,7.35202946020039,
83.9701077239152));
#224159=CARTESIAN_POINT('Ctrl Pts',(-2.92457789302919,7.35056330468839,
83.9702684565481));
#224160=CARTESIAN_POINT('Ctrl Pts',(-2.93217207143489,7.34753738588908,
83.9705999123453));
#224161=CARTESIAN_POINT('Ctrl Pts',(-2.93607841908332,7.34597728082528,
83.9707706566976));
#224162=CARTESIAN_POINT('Ctrl Pts',(-2.94394586398515,7.34282792703042,
83.971115041016));
#224163=CARTESIAN_POINT('Ctrl Pts',(-2.9479069227592,7.3412385869593,83.9712886866683));
#224164=CARTESIAN_POINT('Ctrl Pts',(-2.95751917116754,7.33737272262775,
83.971710698124));
#224165=CARTESIAN_POINT('Ctrl Pts',(-2.96316902220273,7.33509287360441,
83.9719592737827));
#224166=CARTESIAN_POINT('Ctrl Pts',(-3.01179712076684,7.31540492893928,
83.9741033386373));
#224167=CARTESIAN_POINT('Ctrl Pts',(-3.054623313679,7.29762614879642,83.9760223703351));
#224168=CARTESIAN_POINT('Ctrl Pts',(-3.18473579924077,7.24226553128536,
83.9819405886828));
#224169=CARTESIAN_POINT('Ctrl Pts',(-3.2715011616058,7.20348741774783,83.9860086356401));
#224170=CARTESIAN_POINT('Ctrl Pts',(-3.52134392085782,7.08638012351287,
83.9980281507908));
#224171=CARTESIAN_POINT('Ctrl Pts',(-3.68245547971792,7.00401041396173,
84.0061625001843));
#224172=CARTESIAN_POINT('Ctrl Pts',(-3.9726999178255,6.84283639324876,84.0213320101033));
#224173=CARTESIAN_POINT('Ctrl Pts',(-4.10267489034448,6.76570852137468,
84.0283248803467));
#224174=CARTESIAN_POINT('Ctrl Pts',(-4.86806100040528,6.2813550632928,84.070392995994));
#224175=CARTESIAN_POINT('Ctrl Pts',(-5.44488931594817,5.78852936302091,
84.1053048693084));
#224176=CARTESIAN_POINT('Ctrl Pts',(-5.97525459222509,5.18484483300554,
84.1381433884286));
#224177=CARTESIAN_POINT('Ctrl Pts',(-6.00699727577083,5.1480352788246,84.140114567468));
#224178=CARTESIAN_POINT('Ctrl Pts',(-6.04688416521127,5.10091025063367,
84.1425992260308));
#224179=CARTESIAN_POINT('Ctrl Pts',(-6.0553442597492,5.09086430684931,84.1431266775751));
#224180=CARTESIAN_POINT('Ctrl Pts',(-6.0687093849896,5.07491343039701,84.1439606630954));
#224181=CARTESIAN_POINT('Ctrl Pts',(-6.07363088646257,5.06902236934853,
84.1442679223739));
#224182=CARTESIAN_POINT('Ctrl Pts',(-6.08277139370409,5.05804871509945,
84.1448388778819));
#224183=CARTESIAN_POINT('Ctrl Pts',(-6.08699262068158,5.05296798608959,
84.1451026716101));
#224184=CARTESIAN_POINT('Ctrl Pts',(-6.09632412366518,5.04170779395371,
84.1456860807374));
#224185=CARTESIAN_POINT('Ctrl Pts',(-6.1014313809285,5.03552583200022,84.1460055637652));
#224186=CARTESIAN_POINT('Ctrl Pts',(-6.11610244324625,5.01771249258475,
84.1469238186304));
#224187=CARTESIAN_POINT('Ctrl Pts',(-6.12564247458783,5.00606152893751,
84.1475215516014));
#224188=CARTESIAN_POINT('Ctrl Pts',(-6.1885796777465,4.92874885477668,84.1514691463573));
#224189=CARTESIAN_POINT('Ctrl Pts',(-6.24095446927867,4.86225992822554,
84.1547744897285));
#224190=CARTESIAN_POINT('Ctrl Pts',(-6.38804443069569,4.66923833814942,
84.1641249129226));
#224191=CARTESIAN_POINT('Ctrl Pts',(-6.48004983869782,4.54068891678361,
84.1700568376414));
#224192=CARTESIAN_POINT('Ctrl Pts',(-6.7520430594211,4.13553968877194,84.1879523586286));
#224193=CARTESIAN_POINT('Ctrl Pts',(-6.91863003999255,3.85037005191991,
84.1994267418065));
#224194=CARTESIAN_POINT('Ctrl Pts',(-7.12439989321341,3.44139470085532,
84.2150183840971));
#224195=CARTESIAN_POINT('Ctrl Pts',(-7.17909309925279,3.32579222176747,
84.2193376615019));
#224196=CARTESIAN_POINT('Ctrl Pts',(-7.25663207896628,3.15106606429279,
84.2257896634228));
#224197=CARTESIAN_POINT('Ctrl Pts',(-7.28160858365655,3.09291171788683,
84.2279247968904));
#224198=CARTESIAN_POINT('Ctrl Pts',(-7.33224290043826,2.97100271693194,
84.2323851086089));
#224199=CARTESIAN_POINT('Ctrl Pts',(-7.35777316287724,2.90720090731082,
84.2347106803973));
#224200=CARTESIAN_POINT('Ctrl Pts',(-7.48318454524311,2.5815515024007,84.2465690620951));
#224201=CARTESIAN_POINT('Ctrl Pts',(-7.56992767889091,2.31487327588627,
84.2562367340625));
#224202=CARTESIAN_POINT('Ctrl Pts',(-7.65001962945739,2.0154416681411,84.2675843648592));
#224203=CARTESIAN_POINT('Ctrl Pts',(-7.65754211608016,1.98666911158072,
84.268679769749));
#224204=CARTESIAN_POINT('Ctrl Pts',(-7.70236406505108,1.81119348197654,
84.2753945642773));
#224205=CARTESIAN_POINT('Ctrl Pts',(-7.73560683611332,1.66349502048231,
84.2811916657058));
#224206=CARTESIAN_POINT('Ctrl Pts',(-7.76693080147547,1.50294918398679,
84.2877395926663));
#224207=CARTESIAN_POINT('Ctrl Pts',(-7.76924307459088,1.490950156478,84.2882304575188));
#224208=CARTESIAN_POINT('Ctrl Pts',(-7.77242525392877,1.47422852080638,
84.2889166405472));
#224209=CARTESIAN_POINT('Ctrl Pts',(-7.77331868524816,1.46951035281488,
84.2891104890733));
#224210=CARTESIAN_POINT('Ctrl Pts',(-7.77485735096298,1.46134406554483,
84.289446415832));
#224211=CARTESIAN_POINT('Ctrl Pts',(-7.77550458508005,1.4578963450964,84.2895883667165));
#224212=CARTESIAN_POINT('Ctrl Pts',(-7.77684481387798,1.45073086507197,
84.2898836470429));
#224213=CARTESIAN_POINT('Ctrl Pts',(-7.77753743613674,1.44701303774437,
84.2900369996036));
#224214=CARTESIAN_POINT('Ctrl Pts',(-7.77915872442144,1.43827556454946,
84.2903977417281));
#224215=CARTESIAN_POINT('Ctrl Pts',(-7.7800851972655,1.43325551886765,84.2906052666353));
#224216=CARTESIAN_POINT('Ctrl Pts',(-7.78202190883545,1.42270433491175,
84.2910419927238));
#224217=CARTESIAN_POINT('Ctrl Pts',(-7.78303111062175,1.41717301164568,
84.2912712571515));
#224218=CARTESIAN_POINT('Ctrl Pts',(-7.78573793332209,1.40224711579425,
84.2918907557057));
#224219=CARTESIAN_POINT('Ctrl Pts',(-7.78742444213325,1.39285056506307,
84.2922816610334));
#224220=CARTESIAN_POINT('Ctrl Pts',(-7.8698932032324,0.928535663717718,
84.3116413221783));
#224221=CARTESIAN_POINT('Ctrl Pts',(-7.91067346782161,0.467472541057296,
84.3329021201673));
#224222=CARTESIAN_POINT('Ctrl Pts',(-7.91099804691657,0.00555892815145176,
84.354531530966));
#224223=CARTESIAN_POINT('',(-7.91099985457727,0.00151686464269769,86.3576684917632));
#224224=CARTESIAN_POINT('Ctrl Pts',(-7.91099794240846,0.00570571723741387,
84.3576684917632));
#224225=CARTESIAN_POINT('Ctrl Pts',(-7.91113604848863,-0.185778871053852,
84.3653996801986));
#224226=CARTESIAN_POINT('Ctrl Pts',(-7.90431775442304,-0.377536863908371,
84.3731308686339));
#224227=CARTESIAN_POINT('Ctrl Pts',(-7.89051010449761,-0.56900904282895,
84.3808620570693));
#224228=CARTESIAN_POINT('Ctrl Pts',(-7.87671499291532,-0.76030735118546,
84.3885862250273));
#224229=CARTESIAN_POINT('Ctrl Pts',(-7.85594318587293,-0.951320004677742,
84.3963103929853));
#224230=CARTESIAN_POINT('Ctrl Pts',(-7.82821373839945,-1.14148616545889,
84.4040345609433));
#224231=CARTESIAN_POINT('Ctrl Pts',(-7.80050379262063,-1.33151858529892,
84.4117532966126));
#224232=CARTESIAN_POINT('Ctrl Pts',(-7.76584600076575,-1.52070534188531,
84.4194720322819));
#224233=CARTESIAN_POINT('Ctrl Pts',(-7.72431137276304,-1.70848904491763,
84.4271907679511));
#224234=CARTESIAN_POINT('Ctrl Pts',(-7.68197768574935,-1.89988540243222,
84.4350579996004));
#224235=CARTESIAN_POINT('Ctrl Pts',(-7.63249989493742,-2.0898237926873,
84.4429252312498));
#224236=CARTESIAN_POINT('Ctrl Pts',(-7.57600833561745,-2.27772226108779,
84.4507924628991));
#224237=CARTESIAN_POINT('Ctrl Pts',(-7.52062078331188,-2.4619486547641,
84.4585059462888));
#224238=CARTESIAN_POINT('Ctrl Pts',(-7.45849118039364,-2.64421376180912,
84.4662194296786));
#224239=CARTESIAN_POINT('Ctrl Pts',(-7.38979331569571,-2.82398225052831,
84.4739329130683));
#224240=CARTESIAN_POINT('Ctrl Pts',(-7.32109843615863,-3.00374292768225,
84.4816460612804));
#224241=CARTESIAN_POINT('Ctrl Pts',(-7.24583599174336,-3.18100686477606,
84.4893592094926));
#224242=CARTESIAN_POINT('Ctrl Pts',(-7.16422858305065,-3.35525704079435,
84.4970723577047));
#224243=CARTESIAN_POINT('Ctrl Pts',(-7.08260961283277,-3.52953190326976,
84.5047865986577));
#224244=CARTESIAN_POINT('Ctrl Pts',(-6.9946440423981,-3.70079182754728,
84.5125008396108));
#224245=CARTESIAN_POINT('Ctrl Pts',(-6.90060125580291,-3.86854278875279,
84.5202150805638));
#224246=CARTESIAN_POINT('Ctrl Pts',(-6.80328894119551,-4.04212584497161,
84.5281975178114));
#224247=CARTESIAN_POINT('Ctrl Pts',(-6.69946944564072,-4.21195119241786,
84.536179955059));
#224248=CARTESIAN_POINT('Ctrl Pts',(-6.58949077703927,-4.37750297536329,
84.5441623923065));
#224249=CARTESIAN_POINT('Ctrl Pts',(-6.48306975367048,-4.53769940604956,
84.5518866096631));
#224250=CARTESIAN_POINT('Ctrl Pts',(-6.37088206819916,-4.69389417900211,
84.5596108270196));
#224251=CARTESIAN_POINT('Ctrl Pts',(-6.25328460762502,-4.84565296075153,
84.5673350443762));
#224252=CARTESIAN_POINT('Ctrl Pts',(-6.12979023826714,-5.00502166612291,
84.5754465915692));
#224253=CARTESIAN_POINT('Ctrl Pts',(-6.00032990717017,-5.15949770095725,
84.5835581387623));
#224254=CARTESIAN_POINT('Ctrl Pts',(-5.8653609453887,-5.3086214764578,84.5916696859554));
#224255=CARTESIAN_POINT('Ctrl Pts',(-5.73039198360722,-5.45774525195836,
84.5997812331484));
#224256=CARTESIAN_POINT('Ctrl Pts',(-5.58991475892938,-5.6015164931973,
84.6078927803415));
#224257=CARTESIAN_POINT('Ctrl Pts',(-5.4444264966568,-5.739524468325,84.6160043275345));
#224258=CARTESIAN_POINT('Ctrl Pts',(-5.29028986392483,-5.88573615746103,
84.6245980556542));
#224259=CARTESIAN_POINT('Ctrl Pts',(-5.13016600954508,-6.02582518548657,
84.633191783774));
#224260=CARTESIAN_POINT('Ctrl Pts',(-4.96454415718908,-6.15931995526453,
84.6417855118937));
#224261=CARTESIAN_POINT('Ctrl Pts',(-4.7991614341823,-6.29262198165163,
84.6503668321543));
#224262=CARTESIAN_POINT('Ctrl Pts',(-4.62829674783593,-6.41934859482711,
84.658948152415));
#224263=CARTESIAN_POINT('Ctrl Pts',(-4.45247390254535,-6.53906699362781,
84.6675294726756));
#224264=CARTESIAN_POINT('Ctrl Pts',(-4.26904727864673,-6.66396283224461,
84.6764819077325));
#224265=CARTESIAN_POINT('Ctrl Pts',(-4.08022430269794,-6.78123065431066,
84.6854343427895));
#224266=CARTESIAN_POINT('Ctrl Pts',(-3.88663929913602,-6.89042494759296,
84.6943867778465));
#224267=CARTESIAN_POINT('Ctrl Pts',(-3.70181026101123,-6.99468031771324,
84.702934288914));
#224268=CARTESIAN_POINT('Ctrl Pts',(-3.5126406794845,-7.09157613834774,
84.7114817999816));
#224269=CARTESIAN_POINT('Ctrl Pts',(-3.31971423384642,-7.18076725744523,
84.7200293110491));
#224270=CARTESIAN_POINT('Ctrl Pts',(-3.12708439685608,-7.26982125248418,
84.7285636810167));
#224271=CARTESIAN_POINT('Ctrl Pts',(-2.930709442653,-7.35119407246323,84.7370980509843));
#224272=CARTESIAN_POINT('Ctrl Pts',(-2.73119816444677,-7.42458602122183,
84.745632420952));
#224273=CARTESIAN_POINT('Ctrl Pts',(-2.53212126793053,-7.49781817891989,
84.754148209644));
#224274=CARTESIAN_POINT('Ctrl Pts',(-2.32992190578842,-7.56310405227874,
84.762663998336));
#224275=CARTESIAN_POINT('Ctrl Pts',(-2.12522945593439,-7.62019164848423,
84.771179787028));
#224276=CARTESIAN_POINT('Ctrl Pts',(-2.09495182995846,-7.62863591150911,
84.7724394224717));
#224277=CARTESIAN_POINT('Ctrl Pts',(-2.06461969657883,-7.63690088298914,
84.7736990579155));
#224278=CARTESIAN_POINT('Ctrl Pts',(-2.03423513389271,-7.64498583517566,
84.7749586933592));
#224279=CARTESIAN_POINT('Ctrl Pts',(-1.8438052755895,-7.69565683923694,
84.782853235122));
#224280=CARTESIAN_POINT('Ctrl Pts',(-1.65149082274922,-7.73920588467801,
84.7907477768848));
#224281=CARTESIAN_POINT('Ctrl Pts',(-1.45786565126126,-7.77550954876094,
84.7986423186475));
#224282=CARTESIAN_POINT('Ctrl Pts',(-1.26419684484369,-7.8118213941553,
84.8065386395063));
#224283=CARTESIAN_POINT('Ctrl Pts',(-1.06921706769643,-7.84088454089397,
84.8144349603651));
#224284=CARTESIAN_POINT('Ctrl Pts',(-0.873508646527078,-7.8626270192883,
84.8223312812239));
#224285=CARTESIAN_POINT('Ctrl Pts',(-0.67772385586492,-7.88437798204952,
84.8302306833912));
#224286=CARTESIAN_POINT('Ctrl Pts',(-0.481210194663697,-7.89880254565144,
84.8381300855585));
#224287=CARTESIAN_POINT('Ctrl Pts',(-0.284553626403908,-7.90588073738153,
84.8460294877258));
#224288=CARTESIAN_POINT('Ctrl Pts',(-0.0876806601074991,-7.91296671785119,
84.8539375822807));
#224289=CARTESIAN_POINT('Ctrl Pts',(0.109335184935045,-7.91269016399037,
84.8618456768356));
#224290=CARTESIAN_POINT('Ctrl Pts',(0.305908196360126,-7.90508324911254,
84.8697537713905));
#224291=CARTESIAN_POINT('Ctrl Pts',(0.502598322842411,-7.89747180215646,
84.8776665774617));
#224292=CARTESIAN_POINT('Ctrl Pts',(0.698844748872493,-7.88252131195011,
84.8855793835329));
#224293=CARTESIAN_POINT('Ctrl Pts',(0.89406802737253,-7.86031572918227,
84.8934921896041));
#224294=CARTESIAN_POINT('Ctrl Pts',(1.08956487888816,-7.83807902897655,
84.9014160841594));
#224295=CARTESIAN_POINT('Ctrl Pts',(1.28403537992718,-7.80856697254367,
84.9093399787147));
#224296=CARTESIAN_POINT('Ctrl Pts',(1.47691003068571,-7.77191467794519,
84.91726387327));
#224297=CARTESIAN_POINT('Ctrl Pts',(1.61199536850572,-7.74624418377584,
84.922813601908));
#224298=CARTESIAN_POINT('Ctrl Pts',(1.74629814737207,-7.71707224984252,
84.928363330546));
#224299=CARTESIAN_POINT('Ctrl Pts',(1.87962762946362,-7.68445970609235,
84.9339130591839));
#224300=CARTESIAN_POINT('Ctrl Pts',(2.07481455226748,-7.63671676162467,
84.9420375522686));
#224301=CARTESIAN_POINT('Ctrl Pts',(2.26834439119837,-7.58149306887894,
84.9501620453533));
#224302=CARTESIAN_POINT('Ctrl Pts',(2.45962225138909,-7.51892142401234,
84.958286538438));
#224303=CARTESIAN_POINT('Ctrl Pts',(2.65073111809408,-7.45640506102918,
84.9664038535545));
#224304=CARTESIAN_POINT('Ctrl Pts',(2.83959166948251,-7.38655378831354,
84.974521168671));
#224305=CARTESIAN_POINT('Ctrl Pts',(3.02562192866049,-7.3095508032169,84.9826384837875));
#224306=CARTESIAN_POINT('Ctrl Pts',(3.21151431841751,-7.23260488602423,
84.9907497830571));
#224307=CARTESIAN_POINT('Ctrl Pts',(3.39458030307072,-7.14851794693131,
84.9988610823268));
#224308=CARTESIAN_POINT('Ctrl Pts',(3.57425518234388,-7.05752229124981,
85.0069723815965));
#224309=CARTESIAN_POINT('Ctrl Pts',(3.75382245118213,-6.96658113446165,
85.0150788228669));
#224310=CARTESIAN_POINT('Ctrl Pts',(3.93000237929859,-6.86873965682307,
85.0231852641373));
#224311=CARTESIAN_POINT('Ctrl Pts',(4.10225177013506,-6.76427759738051,
85.0312917054076));
#224312=CARTESIAN_POINT('Ctrl Pts',(4.27442246418287,-6.65986326425253,
85.0393944430313));
#224313=CARTESIAN_POINT('Ctrl Pts',(4.44266592860689,-6.54883454786702,
85.0474971806549));
#224314=CARTESIAN_POINT('Ctrl Pts',(4.60646453285016,-6.43151657912763,
85.0555999182785));
#224315=CARTESIAN_POINT('Ctrl Pts',(4.77174236002558,-6.31313914208254,
85.063775829635));
#224316=CARTESIAN_POINT('Ctrl Pts',(4.93249436129339,-6.18835846000633,
85.0719517409914));
#224317=CARTESIAN_POINT('Ctrl Pts',(5.08821866783614,-6.05755328398222,
85.0801276523479));
#224318=CARTESIAN_POINT('Ctrl Pts',(5.2424904198382,-5.92796822353672,85.0882273009973));
#224319=CARTESIAN_POINT('Ctrl Pts',(5.39182763156347,-5.79247080162955,
85.0963269496468));
#224320=CARTESIAN_POINT('Ctrl Pts',(5.53577535425382,-5.65146991739635,
85.1044265982962));
#224321=CARTESIAN_POINT('Ctrl Pts',(5.67972209868514,-5.51046999139567,
85.112526191901));
#224322=CARTESIAN_POINT('Ctrl Pts',(5.81827919810207,-5.36396690215908,
85.1206257855058));
#224323=CARTESIAN_POINT('Ctrl Pts',(5.95102817406918,-5.21240680218216,
85.1287253791106));
#224324=CARTESIAN_POINT('Ctrl Pts',(6.08379338683677,-5.06082816457747,
85.1368259633933));
#224325=CARTESIAN_POINT('Ctrl Pts',(6.21074884848166,-4.90419152427333,
85.144926547676));
#224326=CARTESIAN_POINT('Ctrl Pts',(6.33151567088062,-4.74297694590572,
85.1530271319588));
#224327=CARTESIAN_POINT('Ctrl Pts',(6.45425493476013,-4.57912930727102,
85.1612600201983));
#224328=CARTESIAN_POINT('Ctrl Pts',(6.57060144306575,-4.4105531653976,85.1694929084379));
#224329=CARTESIAN_POINT('Ctrl Pts',(6.68020258790092,-4.23778413614967,
85.1777257966775));
#224330=CARTESIAN_POINT('Ctrl Pts',(6.78814540013673,-4.06762920836751,
85.1858341162643));
#224331=CARTESIAN_POINT('Ctrl Pts',(6.88954538753533,-3.89340767100451,
85.193942435851));
#224332=CARTESIAN_POINT('Ctrl Pts',(6.98411140464275,-3.71565726185005,
85.2020507554378));
#224333=CARTESIAN_POINT('Ctrl Pts',(7.08085665776017,-3.53381066566912,
85.2103459280038));
#224334=CARTESIAN_POINT('Ctrl Pts',(7.17044901172711,-3.34827091383366,
85.2186411005697));
#224335=CARTESIAN_POINT('Ctrl Pts',(7.25262812550995,-3.15963704767841,
85.2269362731357));
#224336=CARTESIAN_POINT('Ctrl Pts',(7.3348072392928,-2.97100318152317,85.2352314457016));
#224337=CARTESIAN_POINT('Ctrl Pts',(7.40957300812188,-2.7792755437729,85.2435266182676));
#224338=CARTESIAN_POINT('Ctrl Pts',(7.47671889352995,-2.58507167930259,
85.2518217908336));
#224339=CARTESIAN_POINT('Ctrl Pts',(7.54008315516352,-2.40180528250461,
85.2596497832946));
#224340=CARTESIAN_POINT('Ctrl Pts',(7.59678305044347,-2.21598231132712,
85.2674777757557));
#224341=CARTESIAN_POINT('Ctrl Pts',(7.64660662407232,-2.02813415155245,
85.2753057682167));
#224342=CARTESIAN_POINT('Ctrl Pts',(7.69638811586044,-1.84044465153988,
85.2831271490217));
#224343=CARTESIAN_POINT('Ctrl Pts',(7.73930476051446,-1.65073370680453,
85.2909485298267));
#224344=CARTESIAN_POINT('Ctrl Pts',(7.77519342645454,-1.45955067785194,
85.2987699106317));
#224345=CARTESIAN_POINT('Ctrl Pts',(7.81105811794983,-1.26849536350931,
85.3065860665765));
#224346=CARTESIAN_POINT('Ctrl Pts',(7.83990411592811,-1.07597026803862,
85.3144022225213));
#224347=CARTESIAN_POINT('Ctrl Pts',(7.86161864288046,-0.88253799573413,
85.3222183784661));
#224348=CARTESIAN_POINT('Ctrl Pts',(7.88332273809248,-0.689198649019919,
85.3300307795002));
#224349=CARTESIAN_POINT('Ctrl Pts',(7.89790214722644,-0.494953342733305,
85.3378431805343));
#224350=CARTESIAN_POINT('Ctrl Pts',(7.90529550428984,-0.30037308443819,
85.3456555815685));
#224351=CARTESIAN_POINT('Ctrl Pts',(7.91268670035618,-0.105849699815022,
85.3534656991236));
#224352=CARTESIAN_POINT('Ctrl Pts',(7.91289601589372,0.0890080901747599,
85.3612758166787));
#224353=CARTESIAN_POINT('Ctrl Pts',(7.90591407798284,0.283625794935357,
85.3690859342338));
#224354=CARTESIAN_POINT('Ctrl Pts',(7.89893174226187,0.478254588434868,
85.3768964967862));
#224355=CARTESIAN_POINT('Ctrl Pts',(7.8847573406027,0.672642917142711,85.3847070593387));
#224356=CARTESIAN_POINT('Ctrl Pts',(7.86343361833381,0.866217484271463,
85.3925176218911));
#224357=CARTESIAN_POINT('Ctrl Pts',(7.846817660913,1.01705544420197,85.3986038001468));
#224358=CARTESIAN_POINT('Ctrl Pts',(7.82586175405752,1.16739927011033,85.4046899784025));
#224359=CARTESIAN_POINT('Ctrl Pts',(7.80060791314723,1.31698032838185,85.4107761566583));
#224360=CARTESIAN_POINT('Ctrl Pts',(7.76475578734917,1.52933610179506,85.4194165226615));
#224361=CARTESIAN_POINT('Ctrl Pts',(7.72025736249287,1.74005315430232,85.4280568886648));
#224362=CARTESIAN_POINT('Ctrl Pts',(7.66729613795211,1.94845860437031,85.4366972546681));
#224363=CARTESIAN_POINT('Ctrl Pts',(7.61424681291079,2.15721073495082,85.4453519938392));
#224364=CARTESIAN_POINT('Ctrl Pts',(7.55270660496586,2.36364335393564,85.4540067330103));
#224365=CARTESIAN_POINT('Ctrl Pts',(7.48290875299718,2.56709906203835,85.4626614721814));
#224366=CARTESIAN_POINT('Ctrl Pts',(7.41095212923674,2.77684743432968,85.4715838930399));
#224367=CARTESIAN_POINT('Ctrl Pts',(7.33021903219875,2.98343155973446,85.4805063138983));
#224368=CARTESIAN_POINT('Ctrl Pts',(7.24101746202913,3.18615553835483,85.4894287347568));
#224369=CARTESIAN_POINT('Ctrl Pts',(7.15420168632371,3.3834574403791,85.4981125156199));
#224370=CARTESIAN_POINT('Ctrl Pts',(7.05936472485675,3.57710283796482,85.506796296483));
#224371=CARTESIAN_POINT('Ctrl Pts',(6.95683702361201,3.76647575684501,85.5154800773461));
#224372=CARTESIAN_POINT('Ctrl Pts',(6.8500829587818,3.96365494465266,85.5245218182023));
#224373=CARTESIAN_POINT('Ctrl Pts',(6.734990861555,4.15620173043621,85.5335635590584));
#224374=CARTESIAN_POINT('Ctrl Pts',(6.61198423995321,4.34345316661874,85.5426052999146));
#224375=CARTESIAN_POINT('Ctrl Pts',(6.48897761835143,4.53070460280126,85.5516470407707));
#224376=CARTESIAN_POINT('Ctrl Pts',(6.35805665142987,4.71266047486259,85.5606887816269));
#224377=CARTESIAN_POINT('Ctrl Pts',(6.21969377629556,4.88869413331519,85.569730522483));
#224378=CARTESIAN_POINT('Ctrl Pts',(6.09234496111341,5.05071503534079,85.5780525162555));
#224379=CARTESIAN_POINT('Ctrl Pts',(5.9585836531275,5.20785666569505,85.5863745100281));
#224380=CARTESIAN_POINT('Ctrl Pts',(5.81880209117596,5.35961409279869,85.5946965038006));
#224381=CARTESIAN_POINT('Ctrl Pts',(5.67914485336173,5.51123654422353,85.603011095848));
#224382=CARTESIAN_POINT('Ctrl Pts',(5.53347824063766,5.65748413123612,85.6113256878954));
#224383=CARTESIAN_POINT('Ctrl Pts',(5.38223448981308,5.79788520899358,85.6196402799428));
#224384=CARTESIAN_POINT('Ctrl Pts',(5.23111603421675,5.93816997394481,85.6279479839125));
#224385=CARTESIAN_POINT('Ctrl Pts',(5.07442987155089,6.07261769380693,85.6362556878822));
#224386=CARTESIAN_POINT('Ctrl Pts',(4.91264539316631,6.20079319450358,85.6445633918519));
#224387=CARTESIAN_POINT('Ctrl Pts',(4.75102414802908,6.32883937189666,85.6528627137227));
#224388=CARTESIAN_POINT('Ctrl Pts',(4.5843150835293,6.4506257809609,85.6611620355935));
#224389=CARTESIAN_POINT('Ctrl Pts',(4.41302127921891,6.56575693954331,85.6694613574643));
#224390=CARTESIAN_POINT('Ctrl Pts',(4.24183691465861,6.68081454073539,85.6777553768917));
#224391=CARTESIAN_POINT('Ctrl Pts',(4.06607389509714,6.78922521017799,85.686049396319));
#224392=CARTESIAN_POINT('Ctrl Pts',(3.88626610731897,6.8906354382672,85.6943434157464));
#224393=CARTESIAN_POINT('Ctrl Pts',(3.70659165595874,6.99197046562834,85.7026312847458));
#224394=CARTESIAN_POINT('Ctrl Pts',(3.52287867679531,7.0863152689388,85.7109191537452));
#224395=CARTESIAN_POINT('Ctrl Pts',(3.33568806308976,7.17336086822352,85.7192070227446));
#224396=CARTESIAN_POINT('Ctrl Pts',(3.26433206588753,7.2065421555545,85.7223663112657));
#224397=CARTESIAN_POINT('Ctrl Pts',(3.19247100940407,7.23866326756346,85.7255255997868));
#224398=CARTESIAN_POINT('Ctrl Pts',(3.12013692538982,7.26970883645411,85.7286848883079));
#224399=CARTESIAN_POINT('Ctrl Pts',(2.93462896820803,7.34932828754603,85.7367871981343));
#224400=CARTESIAN_POINT('Ctrl Pts',(2.74608624849957,7.42183683932858,85.7448895079607));
#224401=CARTESIAN_POINT('Ctrl Pts',(2.5550838464558,7.48701993703641,85.7529918177871));
#224402=CARTESIAN_POINT('Ctrl Pts',(2.36403928567685,7.55221742219133,85.7610959159844));
#224403=CARTESIAN_POINT('Ctrl Pts',(2.170534261616,7.61008612551288,85.7692000141818));
#224404=CARTESIAN_POINT('Ctrl Pts',(1.97515980724869,7.66046113075638,85.7773041123791));
#224405=CARTESIAN_POINT('Ctrl Pts',(1.77971772182673,7.7108535738719,85.7854110159007));
#224406=CARTESIAN_POINT('Ctrl Pts',(1.58240522414939,7.7537470657263,85.7935179194223));
#224407=CARTESIAN_POINT('Ctrl Pts',(1.38382490644727,7.78902751492741,85.8016248229439));
#224408=CARTESIAN_POINT('Ctrl Pts',(1.18506549931651,7.8243397817606,85.809739037667));
#224409=CARTESIAN_POINT('Ctrl Pts',(0.985036301616426,7.852025230093,85.8178532523902));
#224410=CARTESIAN_POINT('Ctrl Pts',(0.784347771465897,7.8720213143383,85.8259674671133));
#224411=CARTESIAN_POINT('Ctrl Pts',(0.583561158362665,7.89202717131443,
85.8340856475147));
#224412=CARTESIAN_POINT('Ctrl Pts',(0.382114887803085,7.90433614324904,
85.8422038279161));
#224413=CARTESIAN_POINT('Ctrl Pts',(0.180621766553604,7.90893777807406,
85.8503220083174));
#224414=CARTESIAN_POINT('Ctrl Pts',(-0.0210880415602115,7.9135443615237,
85.8584489190568));
#224415=CARTESIAN_POINT('Ctrl Pts',(-0.222844482137192,7.91042704530252,
85.8665758297962));
#224416=CARTESIAN_POINT('Ctrl Pts',(-0.424036111522702,7.89962748337697,
85.8747027405356));
#224417=CARTESIAN_POINT('Ctrl Pts',(-0.530789191201968,7.89389719281637,
85.8790149117346));
#224418=CARTESIAN_POINT('Ctrl Pts',(-0.637383339135011,7.88600491528602,
85.8833270829335));
#224419=CARTESIAN_POINT('Ctrl Pts',(-0.743728062832032,7.87596277089704,
85.8876392541325));
#224420=CARTESIAN_POINT('Ctrl Pts',(-0.940965729908816,7.85733759549695,
85.895637042436));
#224421=CARTESIAN_POINT('Ctrl Pts',(-1.13768722476516,7.83128161932807,
85.9036348307394));
#224422=CARTESIAN_POINT('Ctrl Pts',(-1.33329998644681,7.79783509354622,
85.9116326190429));
#224423=CARTESIAN_POINT('Ctrl Pts',(-1.52875303054633,7.764415876812,85.9196238771619));
#224424=CARTESIAN_POINT('Ctrl Pts',(-1.72309881744133,7.72361819231812,
85.927615135281));
#224425=CARTESIAN_POINT('Ctrl Pts',(-1.91574988369583,7.67553407803779,
85.9356063934));
#224426=CARTESIAN_POINT('Ctrl Pts',(-2.10827631892025,7.62748107063275,
85.9435924817645));
#224427=CARTESIAN_POINT('Ctrl Pts',(-2.29910989511405,7.57215110917399,
85.9515785701289));
#224428=CARTESIAN_POINT('Ctrl Pts',(-2.48767291357099,7.50968737532297,
85.9595646584934));
#224429=CARTESIAN_POINT('Ctrl Pts',(-2.67614590701011,7.44725346332567,
85.9675469340861));
#224430=CARTESIAN_POINT('Ctrl Pts',(-2.86235018657887,7.37769267290381,
85.9755292096789));
#224431=CARTESIAN_POINT('Ctrl Pts',(-3.04572240669765,7.30119825928182,
85.9835114852716));
#224432=CARTESIAN_POINT('Ctrl Pts',(-3.22903815125117,7.224727404655,85.9914913024575));
#224433=CARTESIAN_POINT('Ctrl Pts',(-3.40952326682269,7.14132731276972,
85.9994711196433));
#224434=CARTESIAN_POINT('Ctrl Pts',(-3.58663323146954,7.05123982452153,
86.0074509368292));
#224435=CARTESIAN_POINT('Ctrl Pts',(-3.76982958233562,6.95805647857785,
86.0157049805356));
#224436=CARTESIAN_POINT('Ctrl Pts',(-3.94941433989758,6.85771808629206,
86.0239590242419));
#224437=CARTESIAN_POINT('Ctrl Pts',(-4.12481074975638,6.75054496160822,
86.0322130679483));
#224438=CARTESIAN_POINT('Ctrl Pts',(-4.29440284545406,6.64691846872714,
86.0401939643148));
#224439=CARTESIAN_POINT('Ctrl Pts',(-4.46007907286651,6.53690255942615,
86.0481748606813));
#224440=CARTESIAN_POINT('Ctrl Pts',(-4.6213459701,6.42083191063592,86.0561557570479));
#224441=CARTESIAN_POINT('Ctrl Pts',(-4.78264867064435,6.30473549267923,
86.0641384252753));
#224442=CARTESIAN_POINT('Ctrl Pts',(-4.93953981750619,6.18258185067508,
86.0721210935028));
#224443=CARTESIAN_POINT('Ctrl Pts',(-5.09155724222624,6.0547473811162,86.0801037617302));
#224444=CARTESIAN_POINT('Ctrl Pts',(-5.24363178438832,5.92686488036671,
86.0880894292822));
#224445=CARTESIAN_POINT('Ctrl Pts',(-5.39082869761023,5.7932975121146,86.0960750968341));
#224446=CARTESIAN_POINT('Ctrl Pts',(-5.53272075889855,5.65446036364683,
86.1040607643861));
#224447=CARTESIAN_POINT('Ctrl Pts',(-5.67468794819326,5.51554970466632,
86.1120506601329));
#224448=CARTESIAN_POINT('Ctrl Pts',(-5.81134444700214,5.37136393659938,
86.1200405558797));
#224449=CARTESIAN_POINT('Ctrl Pts',(-5.94230133112456,5.22235348191936,
86.1280304516265));
#224450=CARTESIAN_POINT('Ctrl Pts',(-6.07341334448758,5.07316651205398,
86.1360298120645));
#224451=CARTESIAN_POINT('Ctrl Pts',(-6.19881203488972,4.91914368996471,
86.1440291725025));
#224452=CARTESIAN_POINT('Ctrl Pts',(-6.31814929029164,4.76076785251993,
86.1520285329404));
#224453=CARTESIAN_POINT('Ctrl Pts',(-6.43756996916001,4.60228130143995,
86.1600334853821));
#224454=CARTESIAN_POINT('Ctrl Pts',(-6.55092057149521,4.43943593975026,
86.1680384378238));
#224455=CARTESIAN_POINT('Ctrl Pts',(-6.65789719176911,4.27274220891374,
86.1760433902654));
#224456=CARTESIAN_POINT('Ctrl Pts',(-6.7650134252622,4.10583092915557,86.1840587898233));
#224457=CARTESIAN_POINT('Ctrl Pts',(-6.86573889120565,3.9350615352411,86.1920741893811));
#224458=CARTESIAN_POINT('Ctrl Pts',(-6.95981580439282,3.76096862110334,
86.200089588939));
#224459=CARTESIAN_POINT('Ctrl Pts',(-6.98117091057466,3.72145018304063,
86.2019090545533));
#224460=CARTESIAN_POINT('Ctrl Pts',(-7.00218363185694,3.68176057224964,
86.2037285201677));
#224461=CARTESIAN_POINT('Ctrl Pts',(-7.02285130238581,3.64190617459841,
86.205547985782));
#224462=CARTESIAN_POINT('Ctrl Pts',(-7.11591107381369,3.46245483630463,
86.2137404453026));
#224463=CARTESIAN_POINT('Ctrl Pts',(-7.20222462229796,3.27917296624159,
86.2219329048231));
#224464=CARTESIAN_POINT('Ctrl Pts',(-7.28147094893788,3.09258820727457,
86.2301253643437));
#224465=CARTESIAN_POINT('Ctrl Pts',(-7.36057633600453,2.90633528925743,
86.2383032535769));
#224466=CARTESIAN_POINT('Ctrl Pts',(-7.43263943396914,2.71679147092681,
86.2464811428101));
#224467=CARTESIAN_POINT('Ctrl Pts',(-7.49738407016285,2.52451046828258,
86.2546590320433));
#224468=CARTESIAN_POINT('Ctrl Pts',(-7.56534486261059,2.32267800646674,
86.2632431536867));
#224469=CARTESIAN_POINT('Ctrl Pts',(-7.62524141955897,2.11782974578302,
86.27182727533));
#224470=CARTESIAN_POINT('Ctrl Pts',(-7.67680871449751,1.91063574786381,
86.2804113969733));
#224471=CARTESIAN_POINT('Ctrl Pts',(-7.72574556083931,1.71401071932198,
86.2885576424248));
#224472=CARTESIAN_POINT('Ctrl Pts',(-7.76718150490366,1.51527364761672,
86.2967038878763));
#224473=CARTESIAN_POINT('Ctrl Pts',(-7.80093890573647,1.31501832267354,
86.3048501333278));
#224474=CARTESIAN_POINT('Ctrl Pts',(-7.83465351447246,1.11501684859099,
86.3129860523052));
#224475=CARTESIAN_POINT('Ctrl Pts',(-7.86070892734315,0.913501258557734,
86.3211219712826));
#224476=CARTESIAN_POINT('Ctrl Pts',(-7.87897754926956,0.711079305075185,
86.3292578902601));
#224477=CARTESIAN_POINT('Ctrl Pts',(-7.89721819453409,0.508967341616738,
86.3373813498492));
#224478=CARTESIAN_POINT('Ctrl Pts',(-7.90769580288915,0.305952088394149,
86.3455048094383));
#224479=CARTESIAN_POINT('Ctrl Pts',(-7.91033399567166,0.102650265081471,
86.3536282690274));
#224480=CARTESIAN_POINT('Ctrl Pts',(-7.91077136624201,0.0689460433861521,
86.3549750099394));
#224481=CARTESIAN_POINT('Ctrl Pts',(-7.91099338961968,0.0352339657993602,
86.3563217508513));
#224482=CARTESIAN_POINT('Ctrl Pts',(-7.91099985457727,0.00151686464269769,
86.3576684917632));
#224483=CARTESIAN_POINT('',(-7.91729508967814,0.000522195832882638,90.3577115106449));
#224484=CARTESIAN_POINT('Ctrl Pts',(-7.91099999344164,0.00032212781326103,
86.3656351409683));
#224485=CARTESIAN_POINT('Ctrl Pts',(-7.91100080997057,-0.0197306589497159,
86.3664459662309));
#224486=CARTESIAN_POINT('Ctrl Pts',(-7.91092538186667,-0.0397834962520868,
86.3672542192267));
#224487=CARTESIAN_POINT('Ctrl Pts',(-7.910713182016,-0.0678379502749371,
86.3683814149145));
#224488=CARTESIAN_POINT('Ctrl Pts',(-7.91064051456589,-0.0758398671859283,
86.3687025162124));
#224489=CARTESIAN_POINT('Ctrl Pts',(-7.91048823017332,-0.0902080694887452,
86.3692783568725));
#224490=CARTESIAN_POINT('Ctrl Pts',(-7.91041306906146,-0.0965743889316467,
86.3695332462364));
#224491=CARTESIAN_POINT('Ctrl Pts',(-7.91024521821163,-0.10947265626111,
86.3700491384557));
#224492=CARTESIAN_POINT('Ctrl Pts',(-7.91015212300533,-0.11600459432782,
86.3703101274322));
#224493=CARTESIAN_POINT('Ctrl Pts',(-7.90994949763443,-0.12908459942319,
86.3708322128475));
#224494=CARTESIAN_POINT('Ctrl Pts',(-7.90983992698668,-0.13563266078522,
86.3710933077157));
#224495=CARTESIAN_POINT('Ctrl Pts',(-7.90951205263652,-0.153872809060541,
86.3718198602508));
#224496=CARTESIAN_POINT('Ctrl Pts',(-7.90927595439742,-0.165564582518292,
86.3722847176708));
#224497=CARTESIAN_POINT('Ctrl Pts',(-7.90822827504168,-0.212311202249965,
86.3741399323737));
#224498=CARTESIAN_POINT('Ctrl Pts',(-7.90720955481084,-0.247361266830406,
86.3755233005311));
#224499=CARTESIAN_POINT('Ctrl Pts',(-7.89911209452814,-0.474051554622186,
86.3844220510694));
#224500=CARTESIAN_POINT('Ctrl Pts',(-7.88529988808621,-0.665393730805927,
86.3917072471893));
#224501=CARTESIAN_POINT('Ctrl Pts',(-7.78440005472862,-1.59235766819493,
86.4261284881292));
#224502=CARTESIAN_POINT('Ctrl Pts',(-7.60127252092226,-2.31366250068811,
86.4497912572859));
#224503=CARTESIAN_POINT('Ctrl Pts',(-7.22302588665172,-3.23696937748152,
86.4845111112983));
#224504=CARTESIAN_POINT('Ctrl Pts',(-7.1139809506084,-3.4700620689676,86.4937436339693));
#224505=CARTESIAN_POINT('Ctrl Pts',(-6.955967207387,-3.76895068721524,86.5067314190248));
#224506=CARTESIAN_POINT('Ctrl Pts',(-6.91705291563581,-3.83990197187149,
86.5099035065655));
#224507=CARTESIAN_POINT('Ctrl Pts',(-6.8723717250825,-3.91848411764104,
86.5135314146414));
#224508=CARTESIAN_POINT('Ctrl Pts',(-6.86767018701722,-3.92671836381037,
86.5139129874863));
#224509=CARTESIAN_POINT('Ctrl Pts',(-6.86062750466591,-3.93900153808379,
86.5144843429472));
#224510=CARTESIAN_POINT('Ctrl Pts',(-6.85829755248642,-3.94305687963214,
86.5146733307154));
#224511=CARTESIAN_POINT('Ctrl Pts',(-6.85428205350724,-3.95003163214844,
86.5149989748387));
#224512=CARTESIAN_POINT('Ctrl Pts',(-6.85259823684805,-3.95295203212586,
86.5151355080476));
#224513=CARTESIAN_POINT('Ctrl Pts',(-6.84912343505769,-3.95896981205482,
86.5154172237893));
#224514=CARTESIAN_POINT('Ctrl Pts',(-6.8473322148897,-3.96206705398455,
86.5155624228958));
#224515=CARTESIAN_POINT('Ctrl Pts',(-6.84300977062074,-3.96952941046667,
86.5159127516772));
#224516=CARTESIAN_POINT('Ctrl Pts',(-6.84047647320407,-3.97389331520969,
86.5161180267254));
#224517=CARTESIAN_POINT('Ctrl Pts',(-6.83116963763305,-3.98989017249295,
86.5168719909511));
#224518=CARTESIAN_POINT('Ctrl Pts',(-6.82437062156164,-4.00150819339113,
86.5174224513293));
#224519=CARTESIAN_POINT('Ctrl Pts',(-6.71307412918163,-4.19058069675694,
86.5264269311842));
#224520=CARTESIAN_POINT('Ctrl Pts',(-6.6017239104728,-4.36389265796386,
86.5353450064085));
#224521=CARTESIAN_POINT('Ctrl Pts',(-6.4662798921334,-4.55763919649667,
86.5459111944932));
#224522=CARTESIAN_POINT('Ctrl Pts',(-6.44866584843267,-4.582527624766,86.5472802400863));
#224523=CARTESIAN_POINT('Ctrl Pts',(-6.38906597817513,-4.66571738887227,
86.551894151413));
#224524=CARTESIAN_POINT('Ctrl Pts',(-6.34643046391109,-4.72354769588965,
86.5551644431527));
#224525=CARTESIAN_POINT('Ctrl Pts',(-5.86818333086136,-5.35407099606345,
86.5914512676185));
#224526=CARTESIAN_POINT('Ctrl Pts',(-5.35707603827227,-5.86546037841427,
86.6262947345837));
#224527=CARTESIAN_POINT('Ctrl Pts',(-4.61599112944313,-6.42813970254441,
86.6675129438308));
#224528=CARTESIAN_POINT('Ctrl Pts',(-4.44307230151566,-6.54885272425989,
86.6766128403462));
#224529=CARTESIAN_POINT('Ctrl Pts',(-4.19836059940411,-6.70552384023978,
86.6887830503198));
#224530=CARTESIAN_POINT('Ctrl Pts',(-4.13054533756924,-6.74750897920067,
86.6920845387099));
#224531=CARTESIAN_POINT('Ctrl Pts',(-4.03496585602683,-6.80470218490236,
86.6966406039261));
#224532=CARTESIAN_POINT('Ctrl Pts',(-4.00772900570744,-6.82077924676423,
86.69792810286));
#224533=CARTESIAN_POINT('Ctrl Pts',(-3.9604061292534,-6.84833113615353,
86.7001465755725));
#224534=CARTESIAN_POINT('Ctrl Pts',(-3.94036494183646,-6.85988193750319,
86.7010804007526));
#224535=CARTESIAN_POINT('Ctrl Pts',(-3.91179639207971,-6.87618100647102,
86.7024035470075));
#224536=CARTESIAN_POINT('Ctrl Pts',(-3.9033105573464,-6.8810015942932,86.7027955659575));
#224537=CARTESIAN_POINT('Ctrl Pts',(-3.8891691281601,-6.88900040489715,
86.7034471977288));
#224538=CARTESIAN_POINT('Ctrl Pts',(-3.88351851744834,-6.89218738942948,
86.7037071361753));
#224539=CARTESIAN_POINT('Ctrl Pts',(-3.87170709452342,-6.8988299783935,
86.7042495680634));
#224540=CARTESIAN_POINT('Ctrl Pts',(-3.86554556041542,-6.90228428980156,
86.7045320134045));
#224541=CARTESIAN_POINT('Ctrl Pts',(-3.85195975473014,-6.90987693763166,
86.7051536485966));
#224542=CARTESIAN_POINT('Ctrl Pts',(-3.84453341844849,-6.91401157363263,
86.7054927014495));
#224543=CARTESIAN_POINT('Ctrl Pts',(-3.81860505733569,-6.92839257894107,
86.7066738746354));
#224544=CARTESIAN_POINT('Ctrl Pts',(-3.80006854091723,-6.93857675646127,
86.707513702498));
#224545=CARTESIAN_POINT('Ctrl Pts',(-3.61453636789031,-7.03954379494797,
86.7158740809038));
#224546=CARTESIAN_POINT('Ctrl Pts',(-3.44435556272662,-7.12435756566815,
86.723173608394));
#224547=CARTESIAN_POINT('Ctrl Pts',(-2.95562501459095,-7.34631803580239,
86.7432488431515));
#224548=CARTESIAN_POINT('Ctrl Pts',(-2.63088044060601,-7.46877469895862,
86.7555445586615));
#224549=CARTESIAN_POINT('Ctrl Pts',(-2.09279555569682,-7.63221021107031,
86.7750967370254));
#224550=CARTESIAN_POINT('Ctrl Pts',(-1.88397665847125,-7.68642037077053,
86.7824985683819));
#224551=CARTESIAN_POINT('Ctrl Pts',(-1.61016904236078,-7.74567209629457,
86.7921876548449));
#224552=CARTESIAN_POINT('Ctrl Pts',(-1.54696916739977,-7.75854154443141,
86.7944231853528));
#224553=CARTESIAN_POINT('Ctrl Pts',(-1.2828972574553,-7.8089598292688,86.8037816813999));
#224554=CARTESIAN_POINT('Ctrl Pts',(-1.08077156150081,-7.83949020440895,
86.8109859434624));
#224555=CARTESIAN_POINT('Ctrl Pts',(-0.721487165227515,-7.87959917684714,
86.8241745858946));
#224556=CARTESIAN_POINT('Ctrl Pts',(-0.564798054676068,-7.89237769646901,
86.8300543409894));
#224557=CARTESIAN_POINT('Ctrl Pts',(-0.332450052560969,-7.90437200046374,
86.8390880587341));
#224558=CARTESIAN_POINT('Ctrl Pts',(-0.257010673168978,-7.90718436597017,
86.8420704654145));
#224559=CARTESIAN_POINT('Ctrl Pts',(-0.168197491439732,-7.90922302448745,
86.8456320271209));
#224560=CARTESIAN_POINT('Ctrl Pts',(-0.154849381716239,-7.9094956168707,
86.846168649934));
#224561=CARTESIAN_POINT('Ctrl Pts',(-0.134398957736245,-7.90986146345503,
86.8469928014412));
#224562=CARTESIAN_POINT('Ctrl Pts',(-0.127297062045217,-7.90997894488089,
86.8472793771911));
#224563=CARTESIAN_POINT('Ctrl Pts',(-0.114347507489207,-7.91017571543004,
86.8478025820219));
#224564=CARTESIAN_POINT('Ctrl Pts',(-0.108499895419027,-7.91025808516443,
86.8480390918719));
#224565=CARTESIAN_POINT('Ctrl Pts',(-0.0967427837715226,-7.91041065691015,
86.8485151053803));
#224566=CARTESIAN_POINT('Ctrl Pts',(-0.0908332862093388,-7.91048072123581,
86.8487546141378));
#224567=CARTESIAN_POINT('Ctrl Pts',(-0.0740218888743161,-7.91066120016003,
86.8494366716147));
#224568=CARTESIAN_POINT('Ctrl Pts',(-0.0631198552882879,-7.91075570006669,
86.8498798175897));
#224569=CARTESIAN_POINT('Ctrl Pts',(-0.0167954266850209,-7.91106147779371,
86.8517662953784));
#224570=CARTESIAN_POINT('Ctrl Pts',(0.0186276770786875,-7.91105737263887,
86.8532174860652));
#224571=CARTESIAN_POINT('Ctrl Pts',(0.696898345013335,-7.90642321145098,
86.8811580069799));
#224572=CARTESIAN_POINT('Ctrl Pts',(1.33680656792559,-7.82369079059429,
86.9099536411519));
#224573=CARTESIAN_POINT('Ctrl Pts',(2.22372433341331,-7.59692541375302,
86.9497204339889));
#224574=CARTESIAN_POINT('Ctrl Pts',(2.48415866729134,-7.51579608691643,
86.9614109236797));
#224575=CARTESIAN_POINT('Ctrl Pts',(2.94325129735218,-7.34630410881085,
86.9819742569405));
#224576=CARTESIAN_POINT('Ctrl Pts',(3.14344288454988,-7.26289781113607,
86.9909270730247));
#224577=CARTESIAN_POINT('Ctrl Pts',(3.38502426818469,-7.1503847983006,87.0017451099702));
#224578=CARTESIAN_POINT('Ctrl Pts',(3.42988799727005,-7.12897330921446,
87.0037549603082));
#224579=CARTESIAN_POINT('Ctrl Pts',(3.49190134627194,-7.09865615014279,
87.0065347915504));
#224580=CARTESIAN_POINT('Ctrl Pts',(3.50922448338432,-7.09010843916444,
87.0073114931489));
#224581=CARTESIAN_POINT('Ctrl Pts',(3.53841919874099,-7.07556975741225,
87.0086207456193));
#224582=CARTESIAN_POINT('Ctrl Pts',(3.55030727074349,-7.06961216069184,
87.0091539501184));
#224583=CARTESIAN_POINT('Ctrl Pts',(3.5736843235827,-7.0578231314884,87.0102026100713));
#224584=CARTESIAN_POINT('Ctrl Pts',(3.58517419047641,-7.05199354970652,
87.0107181005766));
#224585=CARTESIAN_POINT('Ctrl Pts',(3.61073973870512,-7.03894379808993,
87.0118652538032));
#224586=CARTESIAN_POINT('Ctrl Pts',(3.62480811816114,-7.03170941962386,
87.0124966253805));
#224587=CARTESIAN_POINT('Ctrl Pts',(3.67180122785184,-7.00736566081812,
87.0146059844207));
#224588=CARTESIAN_POINT('Ctrl Pts',(3.70462740351025,-6.99006678014924,
87.0160800384539));
#224589=CARTESIAN_POINT('Ctrl Pts',(4.09144692105395,-6.78272870435253,
87.0334577051192));
#224590=CARTESIAN_POINT('Ctrl Pts',(4.43059814643726,-6.56621476713183,
87.048721533589));
#224591=CARTESIAN_POINT('Ctrl Pts',(5.30401681726587,-5.91001761965357,
87.0891137448454));
#224592=CARTESIAN_POINT('Ctrl Pts',(5.79941080327842,-5.42471405632217,
87.1130656522426));
#224593=CARTESIAN_POINT('Ctrl Pts',(6.25371368432081,-4.84531553019176,
87.142081680206));
#224594=CARTESIAN_POINT('Ctrl Pts',(6.28165192373258,-4.80904007306202,
87.1439012558184));
#224595=CARTESIAN_POINT('Ctrl Pts',(6.31558736616769,-4.76417744881517,
87.1461577316284));
#224596=CARTESIAN_POINT('Ctrl Pts',(6.32188485329516,-4.75581774710273,
87.1465784641479));
#224597=CARTESIAN_POINT('Ctrl Pts',(6.33173525827635,-4.74268752924207,
87.1472397389886));
#224598=CARTESIAN_POINT('Ctrl Pts',(6.33529943177351,-4.73792544162726,
87.1474796634325));
#224599=CARTESIAN_POINT('Ctrl Pts',(6.34160993788723,-4.72947413022372,
87.1479056309369));
#224600=CARTESIAN_POINT('Ctrl Pts',(6.3443584331467,-4.72578651912962,87.1480915537724));
#224601=CARTESIAN_POINT('Ctrl Pts',(6.3506770856694,-4.71729343926865,87.1485198980597));
#224602=CARTESIAN_POINT('Ctrl Pts',(6.35424500404566,-4.71248631476798,
87.14876244468));
#224603=CARTESIAN_POINT('Ctrl Pts',(6.36397032094023,-4.69935208391768,
87.149425431448));
#224604=CARTESIAN_POINT('Ctrl Pts',(6.37011681459522,-4.6910169495814,87.149846488723));
#224605=CARTESIAN_POINT('Ctrl Pts',(6.39995661033749,-4.65038502095655,
87.1519007185575));
#224606=CARTESIAN_POINT('Ctrl Pts',(6.42342028146211,-4.61792132121841,
87.1535472717164));
#224607=CARTESIAN_POINT('Ctrl Pts',(6.81921875183373,-4.06145174842563,
87.181876278338));
#224608=CARTESIAN_POINT('Ctrl Pts',(7.12654388958106,-3.49419710615459,
87.2120952085419));
#224609=CARTESIAN_POINT('Ctrl Pts',(7.58501847296354,-2.32874997926644,
87.2696355149641));
#224610=CARTESIAN_POINT('Ctrl Pts',(7.74189920187815,-1.73746297631295,
87.2967842337955));
#224611=CARTESIAN_POINT('Ctrl Pts',(7.83332894162752,-1.10619420938644,
87.3228425372274));
#224612=CARTESIAN_POINT('Ctrl Pts',(7.83720227789363,-1.07841013179822,
87.3239840992476));
#224613=CARTESIAN_POINT('Ctrl Pts',(7.84375594292394,-1.02949853113753,
87.3259844229303));
#224614=CARTESIAN_POINT('Ctrl Pts',(7.84649888591375,-1.00837976972269,
87.3268450656254));
#224615=CARTESIAN_POINT('Ctrl Pts',(7.85039201066779,-0.977427383861025,
87.3281020344587));
#224616=CARTESIAN_POINT('Ctrl Pts',(7.85160905203771,-0.967602349482378,
87.3285003751994));
#224617=CARTESIAN_POINT('Ctrl Pts',(7.85367190939861,-0.950688960129488,
87.3291849864326));
#224618=CARTESIAN_POINT('Ctrl Pts',(7.85452657869798,-0.9436017084756,87.3294715234497));
#224619=CARTESIAN_POINT('Ctrl Pts',(7.85620581465859,-0.929516459933167,
87.3300403217283));
#224620=CARTESIAN_POINT('Ctrl Pts',(7.8570306267173,-0.922518499915964,
87.3303225901182));
#224621=CARTESIAN_POINT('Ctrl Pts',(7.85894950610844,-0.906048878052633,
87.3309861389019));
#224622=CARTESIAN_POINT('Ctrl Pts',(7.86003580313419,-0.896576312002753,
87.3313671850038));
#224623=CARTESIAN_POINT('Ctrl Pts',(7.86318682501633,-0.868653345077344,
87.3324886735253));
#224624=CARTESIAN_POINT('Ctrl Pts',(7.86520373523742,-0.850197558213323,
87.3332276762771));
#224625=CARTESIAN_POINT('Ctrl Pts',(7.88199617357621,-0.691362395781781,
87.3395685891973));
#224626=CARTESIAN_POINT('Ctrl Pts',(7.89307747108192,-0.550614269424851,
87.345058332559));
#224627=CARTESIAN_POINT('Ctrl Pts',(7.94586149357713,0.467386207393339,
87.3839429104912));
#224628=CARTESIAN_POINT('Ctrl Pts',(7.84499507891126,1.34575759054625,87.4123719819369));
#224629=CARTESIAN_POINT('Ctrl Pts',(7.58595076924457,2.24513139283784,87.4458430470043));
#224630=CARTESIAN_POINT('Ctrl Pts',(7.56933939906867,2.30051406641358,87.4479254870153));
#224631=CARTESIAN_POINT('Ctrl Pts',(7.48609315914763,2.56739159145599,87.4580815321679));
#224632=CARTESIAN_POINT('Ctrl Pts',(7.41119382945113,2.77620183849515,87.4664037871057));
#224633=CARTESIAN_POINT('Ctrl Pts',(7.31359220570024,3.0160695519762,87.4766333534637));
#224634=CARTESIAN_POINT('Ctrl Pts',(7.299320449289,3.05044708360466,87.4781147265758));
#224635=CARTESIAN_POINT('Ctrl Pts',(7.28055621858089,3.09476024554365,87.4800429369869));
#224636=CARTESIAN_POINT('Ctrl Pts',(7.27628492544599,3.10478944721812,87.4804805846549));
#224637=CARTESIAN_POINT('Ctrl Pts',(7.26934788545216,3.12098501283162,87.4811892946056));
#224638=CARTESIAN_POINT('Ctrl Pts',(7.26669498077498,3.12715688542911,87.4814598380453));
#224639=CARTESIAN_POINT('Ctrl Pts',(7.2616132901407,3.13893784349771,87.4819771350045));
#224640=CARTESIAN_POINT('Ctrl Pts',(7.25918585768141,3.14454751025898,87.4822238347049));
#224641=CARTESIAN_POINT('Ctrl Pts',(7.25361728092996,3.15737538331515,87.4827888387962));
#224642=CARTESIAN_POINT('Ctrl Pts',(7.2504718615776,3.16459171984505,87.4831073099816));
#224643=CARTESIAN_POINT('Ctrl Pts',(7.24099655912272,3.18624202437329,87.4840646419385));
#224644=CARTESIAN_POINT('Ctrl Pts',(7.23463432629258,3.20066173904904,87.4847047388569));
#224645=CARTESIAN_POINT('Ctrl Pts',(7.18730907245739,3.30706023008099,87.4894457491503));
#224646=CARTESIAN_POINT('Ctrl Pts',(7.14463728426783,3.39826665236209,87.4936088898356));
#224647=CARTESIAN_POINT('Ctrl Pts',(7.0880642319882,3.51340695765493,87.4989725116867));
#224648=CARTESIAN_POINT('Ctrl Pts',(7.07576154331384,3.53811836628076,87.5001300942847));
#224649=CARTESIAN_POINT('Ctrl Pts',(7.05560999291647,3.57806965610495,87.5020115782177));
#224650=CARTESIAN_POINT('Ctrl Pts',(7.04784045032624,3.59334938736389,87.5027335549588));
#224651=CARTESIAN_POINT('Ctrl Pts',(6.85448901178064,3.97055851397311,87.5206143732838));
#224652=CARTESIAN_POINT('Ctrl Pts',(6.64132061157659,4.31766283054549,87.5383296955375));
#224653=CARTESIAN_POINT('Ctrl Pts',(6.13473853989593,5.01563210302715,87.5754876507643));
#224654=CARTESIAN_POINT('Ctrl Pts',(5.83569201552565,5.36062626807766,87.5947917088525));
#224655=CARTESIAN_POINT('Ctrl Pts',(5.26806793090443,5.91131880782493,87.6275119117655));
#224656=CARTESIAN_POINT('Ctrl Pts',(5.01294702321836,6.12915974701263,87.6411730088532));
#224657=CARTESIAN_POINT('Ctrl Pts',(4.69796491102103,6.36525488511783,87.6571107062464));
#224658=CARTESIAN_POINT('Ctrl Pts',(4.65076130454223,6.39982526275107,87.6594746651094));
#224659=CARTESIAN_POINT('Ctrl Pts',(4.57892975210359,6.45121789339013,87.6630353829554));
#224660=CARTESIAN_POINT('Ctrl Pts',(4.55458317547364,6.46842964614736,87.664236006972));
#224661=CARTESIAN_POINT('Ctrl Pts',(4.51223793280284,6.49800790079411,87.6663134752363));
#224662=CARTESIAN_POINT('Ctrl Pts',(4.49428431089011,6.51043826302279,87.6671909725844));
#224663=CARTESIAN_POINT('Ctrl Pts',(4.45681171833629,6.53615389827236,87.6690156268913));
#224664=CARTESIAN_POINT('Ctrl Pts',(4.43728426761626,6.54942644866664,87.6699626419246));
#224665=CARTESIAN_POINT('Ctrl Pts',(4.38327252502149,6.58578507701514,87.6725715362533));
#224666=CARTESIAN_POINT('Ctrl Pts',(4.34866548634216,6.60868758655402,87.6742314177128));
#224667=CARTESIAN_POINT('Ctrl Pts',(4.20982525625314,6.69900751472013,87.680844730775));
#224668=CARTESIAN_POINT('Ctrl Pts',(4.10419112116401,6.76424024817593,87.6857735524406));
#224669=CARTESIAN_POINT('Ctrl Pts',(3.84990988423524,6.91311741879084,87.697412078626));
#224670=CARTESIAN_POINT('Ctrl Pts',(3.70000640861012,6.99449442756818,87.7040955139439));
#224671=CARTESIAN_POINT('Ctrl Pts',(3.13407717418437,7.27842802094015,87.7287771377114));
#224672=CARTESIAN_POINT('Ctrl Pts',(2.70316879030007,7.4492164167693,87.7464552979666));
#224673=CARTESIAN_POINT('Ctrl Pts',(2.08805530787275,7.63256634686153,87.7715214270525));
#224674=CARTESIAN_POINT('Ctrl Pts',(1.91460739493355,7.67791117145885,87.7785780233219));
#224675=CARTESIAN_POINT('Ctrl Pts',(1.71590530383868,7.72270604270233,87.7867352930723));
#224676=CARTESIAN_POINT('Ctrl Pts',(1.69201256055684,7.72797600407672,87.7877173608471));
#224677=CARTESIAN_POINT('Ctrl Pts',(1.65582098115427,7.73578280211078,87.7892070809978));
#224678=CARTESIAN_POINT('Ctrl Pts',(1.64353985416293,7.73840134844053,87.7897129681732));
#224679=CARTESIAN_POINT('Ctrl Pts',(1.62134434564484,7.74307858963739,87.7906279705967));
#224680=CARTESIAN_POINT('Ctrl Pts',(1.61143213845709,7.74514751279154,87.7910368569473));
#224681=CARTESIAN_POINT('Ctrl Pts',(1.59166984882534,7.7492328124804,87.7918526121139));
#224682=CARTESIAN_POINT('Ctrl Pts',(1.58181983998259,7.75124945301157,87.7922594740462));
#224683=CARTESIAN_POINT('Ctrl Pts',(1.55397890853426,7.7568941844088,87.7934102667248));
#224684=CARTESIAN_POINT('Ctrl Pts',(1.53597930340683,7.76047842669492,87.7941552384448));
#224685=CARTESIAN_POINT('Ctrl Pts',(1.45107130388154,7.77707909280664,87.797674012409));
#224686=CARTESIAN_POINT('Ctrl Pts',(1.38400970133299,7.78929291346083,87.8004663097038));
#224687=CARTESIAN_POINT('Ctrl Pts',(0.633794979466337,7.91593412443728,
87.8318123023659));
#224688=CARTESIAN_POINT('Ctrl Pts',(-0.0614089438128411,7.94103310830199,
87.8615694260812));
#224689=CARTESIAN_POINT('Ctrl Pts',(-0.913482989596982,7.85977807747364,
87.8968468073517));
#224690=CARTESIAN_POINT('Ctrl Pts',(-1.07545210965178,7.83925806134967,
87.9035147448832));
#224691=CARTESIAN_POINT('Ctrl Pts',(-1.27503551001025,7.80767020368677,
87.9116951463416));
#224692=CARTESIAN_POINT('Ctrl Pts',(-1.31335310697317,7.80131611967476,
87.9132640815826));
#224693=CARTESIAN_POINT('Ctrl Pts',(-1.37400597830323,7.79079871753301,
87.9157453503438));
#224694=CARTESIAN_POINT('Ctrl Pts',(-1.39637268782135,7.78682094351948,
87.916659883563));
#224695=CARTESIAN_POINT('Ctrl Pts',(-1.4384019705062,7.77915939819513,87.9183775842211));
#224696=CARTESIAN_POINT('Ctrl Pts',(-1.45806829883422,7.77549728377791,
87.9191810006594));
#224697=CARTESIAN_POINT('Ctrl Pts',(-1.50225831000621,7.76709500643872,
87.9209856092262));
#224698=CARTESIAN_POINT('Ctrl Pts',(-1.52677387854837,7.76231321180602,
87.9219863059004));
#224699=CARTESIAN_POINT('Ctrl Pts',(-1.58939574296139,7.74979058770908,
87.924541483828));
#224700=CARTESIAN_POINT('Ctrl Pts',(-1.62746842884367,7.74188475202751,
87.9260940497014));
#224701=CARTESIAN_POINT('Ctrl Pts',(-1.88635747285399,7.68613201134486,
87.9366471649885));
#224702=CARTESIAN_POINT('Ctrl Pts',(-2.10509674706303,7.62912447065724,
87.9455400162122));
#224703=CARTESIAN_POINT('Ctrl Pts',(-2.33231028974806,7.55939066701257,
87.9548432703343));
#224704=CARTESIAN_POINT('Ctrl Pts',(-2.34351439834022,7.55592474877756,
87.9553022018588));
#224705=CARTESIAN_POINT('Ctrl Pts',(-2.35960716713393,7.55090731780756,
87.9559616574063));
#224706=CARTESIAN_POINT('Ctrl Pts',(-2.36450208738591,7.54937594666487,
87.9561622807256));
#224707=CARTESIAN_POINT('Ctrl Pts',(-2.59507035312394,7.47699663971959,
87.9656141087257));
#224708=CARTESIAN_POINT('Ctrl Pts',(-2.81745712368215,7.39606701524068,
87.9748041215321));
#224709=CARTESIAN_POINT('Ctrl Pts',(-3.08829899464355,7.28351233109193,
87.9860806855725));
#224710=CARTESIAN_POINT('Ctrl Pts',(-3.14047627668738,7.26116735524773,
87.9882573733916));
#224711=CARTESIAN_POINT('Ctrl Pts',(-3.71980475264395,7.0056566927738,88.0124784115644));
#224712=CARTESIAN_POINT('Ctrl Pts',(-4.22018742908342,6.71611328896293,
88.0337119031437));
#224713=CARTESIAN_POINT('Ctrl Pts',(-4.86823051933445,6.23988377540042,
88.0640485545537));
#224714=CARTESIAN_POINT('Ctrl Pts',(-5.04588398340681,6.09711950886217,
88.0727313860423));
#224715=CARTESIAN_POINT('Ctrl Pts',(-5.27193993800442,5.89880393378416,
88.0845309448591));
#224716=CARTESIAN_POINT('Ctrl Pts',(-5.32608852104222,5.84995891340575,
88.0874181618653));
#224717=CARTESIAN_POINT('Ctrl Pts',(-5.39023750492656,5.79046396985332,
88.09092091153));
#224718=CARTESIAN_POINT('Ctrl Pts',(-5.40089437221624,5.78052535006996,
88.091505587918));
#224719=CARTESIAN_POINT('Ctrl Pts',(-5.41735723667327,5.7650867754221,88.0924132032141));
#224720=CARTESIAN_POINT('Ctrl Pts',(-5.42318248280896,5.75960734039428,
88.0927352131094));
#224721=CARTESIAN_POINT('Ctrl Pts',(-5.43340428760738,5.74996308882354,
88.0933017839848));
#224722=CARTESIAN_POINT('Ctrl Pts',(-5.43780439620327,5.74580203486148,
88.0935461706383));
#224723=CARTESIAN_POINT('Ctrl Pts',(-5.44779585102022,5.73633165165722,
88.0941022513311));
#224724=CARTESIAN_POINT('Ctrl Pts',(-5.45338421737433,5.73101919639127,
88.0944140926257));
#224725=CARTESIAN_POINT('Ctrl Pts',(-5.46832350686898,5.71677585924211,
88.0952499470565));
#224726=CARTESIAN_POINT('Ctrl Pts',(-5.47766029383313,5.70783022729303,
88.09577467035));
#224727=CARTESIAN_POINT('Ctrl Pts',(-5.51967617407549,5.66737651975696,
88.0981466618111));
#224728=CARTESIAN_POINT('Ctrl Pts',(-5.55210523739451,5.63561079263626,
88.1000067834171));
#224729=CARTESIAN_POINT('Ctrl Pts',(-6.14830562214165,5.04146487184841,
88.1347870544739));
#224730=CARTESIAN_POINT('Ctrl Pts',(-6.62416848020391,4.39751159722814,
88.1728936578792));
#224731=CARTESIAN_POINT('Ctrl Pts',(-7.1465903781655,3.40799045111042,88.2230720140554));
#224732=CARTESIAN_POINT('Ctrl Pts',(-7.27971319486202,3.11351210739892,
88.2371603675924));
#224733=CARTESIAN_POINT('Ctrl Pts',(-7.43710405713788,2.699590703408,88.2556745106913));
#224734=CARTESIAN_POINT('Ctrl Pts',(-7.47717890441449,2.58652353326187,
88.260607488423));
#224735=CARTESIAN_POINT('Ctrl Pts',(-7.5201561265799,2.45590738905284,88.2661664041054));
#224736=CARTESIAN_POINT('Ctrl Pts',(-7.52558826565268,2.43921104718805,
88.2668744028457));
#224737=CARTESIAN_POINT('Ctrl Pts',(-7.53371455678899,2.41394834497199,
88.2679417703779));
#224738=CARTESIAN_POINT('Ctrl Pts',(-7.536449764568,2.40539530684519,88.2683024712615));
#224739=CARTESIAN_POINT('Ctrl Pts',(-7.54114865056292,2.39061512229162,
88.2689246294653));
#224740=CARTESIAN_POINT('Ctrl Pts',(-7.54311919026548,2.38439017665291,
88.2691863092788));
#224741=CARTESIAN_POINT('Ctrl Pts',(-7.54717983482096,2.37150716612742,
88.269727146537));
#224742=CARTESIAN_POINT('Ctrl Pts',(-7.54926884166676,2.36484875936864,
88.2700062681858));
#224743=CARTESIAN_POINT('Ctrl Pts',(-7.55491208255456,2.34677806732403,
88.2707627056684));
#224744=CARTESIAN_POINT('Ctrl Pts',(-7.5584492730617,2.33536045623653,88.2712394682537));
#224745=CARTESIAN_POINT('Ctrl Pts',(-7.57156320299398,2.29268842450722,
88.2730169388504));
#224746=CARTESIAN_POINT('Ctrl Pts',(-7.58097213383292,2.26138256101762,
88.2743122024809));
#224747=CARTESIAN_POINT('Ctrl Pts',(-7.72840851147747,1.75956188909231,
88.2949368270008));
#224748=CARTESIAN_POINT('Ctrl Pts',(-7.82259783315802,1.27725907156672,
88.3127298887389));
#224749=CARTESIAN_POINT('Ctrl Pts',(-7.89781751367036,0.52710037195774,
88.3389136277887));
#224750=CARTESIAN_POINT('Ctrl Pts',(-7.91099178079852,0.263756986168273,
88.3478486968288));
#224751=CARTESIAN_POINT('Ctrl Pts',(-7.91101694035408,-0.543244617673399,
88.3753081746271));
#224752=CARTESIAN_POINT('Ctrl Pts',(-7.85502632930673,-1.08523180736228,
88.3938192804968));
#224753=CARTESIAN_POINT('Ctrl Pts',(-7.737144850556,-1.64973341490619,88.4166116165124));
#224754=CARTESIAN_POINT('Ctrl Pts',(-7.73012929889818,-1.68229953938953,
88.4179393682475));
#224755=CARTESIAN_POINT('Ctrl Pts',(-7.72128933436136,-1.72211143726707,
88.4195792816945));
#224756=CARTESIAN_POINT('Ctrl Pts',(-7.71965998436012,-1.72940062231682,
88.4198802230356));
#224757=CARTESIAN_POINT('Ctrl Pts',(-7.71695331049812,-1.74142936339991,
88.4203779935989));
#224758=CARTESIAN_POINT('Ctrl Pts',(-7.71588193456887,-1.74617026537544,
88.4205744760918));
#224759=CARTESIAN_POINT('Ctrl Pts',(-7.71394117352235,-1.75472158663843,
88.4209294159117));
#224760=CARTESIAN_POINT('Ctrl Pts',(-7.7130733316943,-1.75853235824049,
88.4210877824789));
#224761=CARTESIAN_POINT('Ctrl Pts',(-7.71121423376137,-1.76666797331657,
88.4214262937414));
#224762=CARTESIAN_POINT('Ctrl Pts',(-7.71022216290022,-1.77099262716503,
88.4216064866274));
#224763=CARTESIAN_POINT('Ctrl Pts',(-7.70753633687523,-1.78265569783465,
88.4220931253795));
#224764=CARTESIAN_POINT('Ctrl Pts',(-7.70583574354406,-1.78999251786735,
88.4223999791152));
#224765=CARTESIAN_POINT('Ctrl Pts',(-7.69712481441774,-1.82733134870511,
88.4239653789702));
#224766=CARTESIAN_POINT('Ctrl Pts',(-7.68994985400923,-1.85729411770513,
88.4252339070756));
#224767=CARTESIAN_POINT('Ctrl Pts',(-7.6201803035531,-2.14131683950218,
88.4373703258417));
#224768=CARTESIAN_POINT('Ctrl Pts',(-7.54519667171131,-2.39214768773682,
88.4489348301647));
#224769=CARTESIAN_POINT('Ctrl Pts',(-7.26573593112366,-3.18198222994523,
88.4869884300581));
#224770=CARTESIAN_POINT('Ctrl Pts',(-7.01476776392652,-3.70257268025828,
88.5144423311623));
#224771=CARTESIAN_POINT('Ctrl Pts',(-6.63172581499798,-4.31574525202144,
88.5469255406739));
#224772=CARTESIAN_POINT('Ctrl Pts',(-6.5505499425266,-4.43798858169724,
88.5534206457648));
#224773=CARTESIAN_POINT('Ctrl Pts',(-6.32269495318178,-4.76123218775531,
88.5706071862891));
#224774=CARTESIAN_POINT('Ctrl Pts',(-6.1698536050818,-4.95769360216837,
88.5810609127793));
#224775=CARTESIAN_POINT('Ctrl Pts',(-5.99395479275036,-5.16303135740085,
88.5919900401683));
#224776=CARTESIAN_POINT('Ctrl Pts',(-5.97984605447867,-5.17936560112691,
88.5928595083835));
#224777=CARTESIAN_POINT('Ctrl Pts',(-5.96002931770756,-5.20211930960653,
88.5940708278627));
#224778=CARTESIAN_POINT('Ctrl Pts',(-5.95437751293358,-5.20858744895521,
88.5944151830864));
#224779=CARTESIAN_POINT('Ctrl Pts',(-5.9445845715237,-5.21975809152442,
88.5950099252724));
#224780=CARTESIAN_POINT('Ctrl Pts',(-5.9404483671787,-5.22446489692322,
88.5952605326552));
#224781=CARTESIAN_POINT('Ctrl Pts',(-5.93186242116831,-5.23421191967796,
88.5957795215033));
#224782=CARTESIAN_POINT('Ctrl Pts',(-5.92741183635443,-5.23925138987717,
88.5960478647947));
#224783=CARTESIAN_POINT('Ctrl Pts',(-5.91697335439893,-5.25104072909789,
88.5966756583168));
#224784=CARTESIAN_POINT('Ctrl Pts',(-5.9109803169816,-5.25778604626653,
88.597034876796));
#224785=CARTESIAN_POINT('Ctrl Pts',(-5.89159126730898,-5.27953386824249,
88.5981931318671));
#224786=CARTESIAN_POINT('Ctrl Pts',(-5.87814952568701,-5.2944956028725,
88.5989901023857));
#224787=CARTESIAN_POINT('Ctrl Pts',(-5.55240493376366,-5.65430577486697,
88.6181601508027));
#224788=CARTESIAN_POINT('Ctrl Pts',(-5.21033552532158,-5.97100033731662,
88.6350366501181));
#224789=CARTESIAN_POINT('Ctrl Pts',(-4.74483721245125,-6.33132327105307,
88.6554057210577));
#224790=CARTESIAN_POINT('Ctrl Pts',(-4.64554717602665,-6.40453172455108,
88.6596217873688));
#224791=CARTESIAN_POINT('Ctrl Pts',(-4.43858457962816,-6.54978308298424,
88.6682094156754));
#224792=CARTESIAN_POINT('Ctrl Pts',(-4.33077309649846,-6.62156296491187,
88.6725768947865));
#224793=CARTESIAN_POINT('Ctrl Pts',(-3.8225551286767,-6.94220588656738,
88.6928583743673));
#224794=CARTESIAN_POINT('Ctrl Pts',(-3.40221254233858,-7.15758450384787,
88.7087245874296));
#224795=CARTESIAN_POINT('Ctrl Pts',(-2.9479910767082,-7.34122716143946,
88.7273557736604));
#224796=CARTESIAN_POINT('Ctrl Pts',(-2.93070609902059,-7.34814462133207,
88.7280669810845));
#224797=CARTESIAN_POINT('Ctrl Pts',(-2.83806114565047,-7.38484230895787,
88.7318916224475));
#224798=CARTESIAN_POINT('Ctrl Pts',(-2.76227377166025,-7.41352343515758,
88.7350651184924));
#224799=CARTESIAN_POINT('Ctrl Pts',(-2.67713023843656,-7.44425851611172,
88.7386946002181));
#224800=CARTESIAN_POINT('Ctrl Pts',(-2.66819289052675,-7.44746654007975,
88.739076364801));
#224801=CARTESIAN_POINT('Ctrl Pts',(-2.6547673029491,-7.4522583301866,88.7396510566824));
#224802=CARTESIAN_POINT('Ctrl Pts',(-2.65028335142292,-7.45385415807101,
88.7398431979907));
#224803=CARTESIAN_POINT('Ctrl Pts',(-2.64250196837033,-7.45661562498681,
88.7401769911241));
#224804=CARTESIAN_POINT('Ctrl Pts',(-2.63920521856608,-7.45778311871919,
88.7403185195026));
#224805=CARTESIAN_POINT('Ctrl Pts',(-2.63233486637463,-7.46021102319318,
88.7406136883837));
#224806=CARTESIAN_POINT('Ctrl Pts',(-2.62876113138943,-7.46147105290219,
88.7407673535259));
#224807=CARTESIAN_POINT('Ctrl Pts',(-2.62032959490861,-7.4644370398999,
88.741130195725));
#224808=CARTESIAN_POINT('Ctrl Pts',(-2.61547103579838,-7.46614082168484,
88.7413395126198));
#224809=CARTESIAN_POINT('Ctrl Pts',(-2.59952826134319,-7.47171410397762,
88.7420271194424));
#224810=CARTESIAN_POINT('Ctrl Pts',(-2.58843714338575,-7.47556365666566,
88.7425066781246));
#224811=CARTESIAN_POINT('Ctrl Pts',(-2.18074201189771,-7.61605214399134,
88.7601776328176));
#224812=CARTESIAN_POINT('Ctrl Pts',(-1.77394553591557,-7.72094065130411,
88.7792801012561));
#224813=CARTESIAN_POINT('Ctrl Pts',(-0.9476121671058,-7.86523295458176,
88.8183932288109));
#224814=CARTESIAN_POINT('Ctrl Pts',(-0.52931208548964,-7.90441073791194,
88.8383280646829));
#224815=CARTESIAN_POINT('Ctrl Pts',(0.387914087462226,-7.91715149784917,
88.8805185944954));
#224816=CARTESIAN_POINT('Ctrl Pts',(0.885295356752189,-7.87706426171078,
88.902380205155));
#224817=CARTESIAN_POINT('Ctrl Pts',(1.40954616123498,-7.78448995176033,
88.9240515020288));
#224818=CARTESIAN_POINT('Ctrl Pts',(1.44338053315756,-7.77828752792368,
88.9254444374308));
#224819=CARTESIAN_POINT('Ctrl Pts',(1.48886297999582,-7.76964282338008,
88.9273094256373));
#224820=CARTESIAN_POINT('Ctrl Pts',(1.50054729508004,-7.76739469790199,
88.9277878695766));
#224821=CARTESIAN_POINT('Ctrl Pts',(1.51887333532028,-7.76382577386114,
88.9285372401026));
#224822=CARTESIAN_POINT('Ctrl Pts',(1.52551848842739,-7.76252279850979,
88.9288087533365));
#224823=CARTESIAN_POINT('Ctrl Pts',(1.53827146157543,-7.76000519916228,
88.9293294167995));
#224824=CARTESIAN_POINT('Ctrl Pts',(1.54437953471024,-7.75879189265492,
88.9295786101808));
#224825=CARTESIAN_POINT('Ctrl Pts',(1.55872321325263,-7.75592505788742,
88.9301633744871));
#224826=CARTESIAN_POINT('Ctrl Pts',(1.56695763790714,-7.75426562097835,
88.9304987506442));
#224827=CARTESIAN_POINT('Ctrl Pts',(1.59074247285435,-7.7494329643363,88.9314665389876));
#224828=CARTESIAN_POINT('Ctrl Pts',(1.60628603898638,-7.74622605198929,
88.9320978421508));
#224829=CARTESIAN_POINT('Ctrl Pts',(1.71157474274845,-7.72417259399143,
88.9363664528819));
#224830=CARTESIAN_POINT('Ctrl Pts',(1.80099765769058,-7.70381324515539,
88.9399537732689));
#224831=CARTESIAN_POINT('Ctrl Pts',(1.99299572387748,-7.65657421826673,
88.9475832749825));
#224832=CARTESIAN_POINT('Ctrl Pts',(2.09542555195124,-7.62917777172763,
88.9516082288176));
#224833=CARTESIAN_POINT('Ctrl Pts',(2.51514707477109,-7.50782555350359,
88.9679516055825));
#224834=CARTESIAN_POINT('Ctrl Pts',(2.82694961431663,-7.39606536926273,
88.9797205709783));
#224835=CARTESIAN_POINT('Ctrl Pts',(3.45223152302835,-7.12660417506277,
89.0034388245891));
#224836=CARTESIAN_POINT('Ctrl Pts',(3.76406426169689,-6.96693645160515,
89.0153346777934));
#224837=CARTESIAN_POINT('Ctrl Pts',(4.37591260307645,-6.60054808698712,
89.0403683026975));
#224838=CARTESIAN_POINT('Ctrl Pts',(4.67431209451183,-6.39270406833882,
89.0535483406642));
#224839=CARTESIAN_POINT('Ctrl Pts',(4.97790416914924,-6.1485839516202,89.0690402716622));
#224840=CARTESIAN_POINT('Ctrl Pts',(4.99834441144837,-6.13197909724792,
89.0700931055343));
#224841=CARTESIAN_POINT('Ctrl Pts',(5.02659289353847,-6.10879604404624,
89.0715613961585));
#224842=CARTESIAN_POINT('Ctrl Pts',(5.03447202655267,-6.10230420724019,
89.0719723784135));
#224843=CARTESIAN_POINT('Ctrl Pts',(5.04678262352544,-6.09212109319449,
89.0726167473329));
#224844=CARTESIAN_POINT('Ctrl Pts',(5.05122267136329,-6.08844017687189,
89.0728496081757));
#224845=CARTESIAN_POINT('Ctrl Pts',(5.05971908841751,-6.08138073260774,
89.0732960785586));
#224846=CARTESIAN_POINT('Ctrl Pts',(5.06377611006337,-6.07800299239878,
89.0735096485714));
#224847=CARTESIAN_POINT('Ctrl Pts',(5.07315829300004,-6.07017578734881,
89.0740044244693));
#224848=CARTESIAN_POINT('Ctrl Pts',(5.07848098242425,-6.06572337532063,
89.0742857764904));
#224849=CARTESIAN_POINT('Ctrl Pts',(5.09358928316965,-6.05305150583187,
89.0750862394353));
#224850=CARTESIAN_POINT('Ctrl Pts',(5.10336082103688,-6.04481535249912,
89.0756061662113));
#224851=CARTESIAN_POINT('Ctrl Pts',(5.12531085871779,-6.02622312610047,
89.0767790173081));
#224852=CARTESIAN_POINT('Ctrl Pts',(5.13747799334752,-6.01585375714953,
89.0774325733103));
#224853=CARTESIAN_POINT('Ctrl Pts',(5.40418037700571,-5.78715902915146,
89.0918328070513));
#224854=CARTESIAN_POINT('Ctrl Pts',(5.64459837793763,-5.55291473319003,
89.1062933403793));
#224855=CARTESIAN_POINT('Ctrl Pts',(6.28301977483555,-4.84645509327848,
89.1478396790811));
#224856=CARTESIAN_POINT('Ctrl Pts',(6.64170755335334,-4.34192158305693,
89.1750306117343));
#224857=CARTESIAN_POINT('Ctrl Pts',(7.0422408391639,-3.61077902904357,89.2099485105464));
#224858=CARTESIAN_POINT('Ctrl Pts',(7.13850520234323,-3.41652311684236,
89.2188671420879));
#224859=CARTESIAN_POINT('Ctrl Pts',(7.24103665745436,-3.18630745760502,
89.2290630511905));
#224860=CARTESIAN_POINT('Ctrl Pts',(7.25518240576039,-3.15396502425295,
89.2304872088299));
#224861=CARTESIAN_POINT('Ctrl Pts',(7.27563181797133,-3.10634443278226,
89.2325720701079));
#224862=CARTESIAN_POINT('Ctrl Pts',(7.28210480690269,-3.09113954221639,
89.2332359531901));
#224863=CARTESIAN_POINT('Ctrl Pts',(7.29352356704223,-3.06408223010943,
89.234414147183));
#224864=CARTESIAN_POINT('Ctrl Pts',(7.29848820236185,-3.05223785066061,
89.2349288190136));
#224865=CARTESIAN_POINT('Ctrl Pts',(7.30877781075989,-3.02752076338877,
89.236000586599));
#224866=CARTESIAN_POINT('Ctrl Pts',(7.31409767069249,-3.01464597006946,
89.2365575815631));
#224867=CARTESIAN_POINT('Ctrl Pts',(7.32782419289511,-2.98117568096985,
89.238002282422));
#224868=CARTESIAN_POINT('Ctrl Pts',(7.33617805761328,-2.96055862226515,
89.2388889480326));
#224869=CARTESIAN_POINT('Ctrl Pts',(7.37175341906241,-2.87168461292541,
89.2426971869306));
#224870=CARTESIAN_POINT('Ctrl Pts',(7.39811033756079,-2.80308484427902,
89.2456014074783));
#224871=CARTESIAN_POINT('Ctrl Pts',(7.57479916722589,-2.32335186561229,
89.2656712060856));
#224872=CARTESIAN_POINT('Ctrl Pts',(7.69173832209123,-1.90072096707954,
89.2820686020286));
#224873=CARTESIAN_POINT('Ctrl Pts',(7.8890732413498,-0.857646648316181,
89.3209611424736));
#224874=CARTESIAN_POINT('Ctrl Pts',(7.93211630525977,-0.233237506243383,
89.3428624459517));
#224875=CARTESIAN_POINT('Ctrl Pts',(7.89986951178722,0.420648519860349,
89.368822955207));
#224876=CARTESIAN_POINT('Ctrl Pts',(7.89815916154212,0.451625178697357,
89.3700604266088));
#224877=CARTESIAN_POINT('Ctrl Pts',(7.89568457378939,0.492114989354451,
89.3716887936087));
#224878=CARTESIAN_POINT('Ctrl Pts',(7.89508525268277,0.501638219478262,
89.3720725726294));
#224879=CARTESIAN_POINT('Ctrl Pts',(7.89413469811329,0.516318786670662,
89.3726654304444));
#224880=CARTESIAN_POINT('Ctrl Pts',(7.89379563574389,0.521476924081097,
89.372873972338));
#224881=CARTESIAN_POINT('Ctrl Pts',(7.89311113535584,0.531736541343692,
89.3732892420114));
#224882=CARTESIAN_POINT('Ctrl Pts',(7.8927658066103,0.536838026128945,89.3734959648196));
#224883=CARTESIAN_POINT('Ctrl Pts',(7.89199886739546,0.54800718196608,89.3739490821931));
#224884=CARTESIAN_POINT('Ctrl Pts',(7.89157520495236,0.554074705003744,
89.3741955692982));
#224885=CARTESIAN_POINT('Ctrl Pts',(7.8903751126361,0.570981322721977,89.3748833343878));
#224886=CARTESIAN_POINT('Ctrl Pts',(7.8895833480246,0.581819286158091,89.3753253141265));
#224887=CARTESIAN_POINT('Ctrl Pts',(7.8877555387337,0.606149043888864,89.3763200090322));
#224888=CARTESIAN_POINT('Ctrl Pts',(7.88670720562293,0.619639856172831,
89.3768732997237));
#224889=CARTESIAN_POINT('Ctrl Pts',(7.84827506856253,1.09831315307018,89.3965683888143));
#224890=CARTESIAN_POINT('Ctrl Pts',(7.76984113715447,1.55921713442513,89.4177377404537));
#224891=CARTESIAN_POINT('Ctrl Pts',(7.52972908385702,2.47302449974956,89.4612007333255));
#224892=CARTESIAN_POINT('Ctrl Pts',(7.3664753035758,2.92365598710213,89.4833901677259));
#224893=CARTESIAN_POINT('Ctrl Pts',(7.09483577063776,3.50334412523636,89.5117360187883));
#224894=CARTESIAN_POINT('Ctrl Pts',(7.02167876149942,3.64775898533374,89.518787531536));
#224895=CARTESIAN_POINT('Ctrl Pts',(6.84997276692335,3.96237720463552,89.5341012455857));
#224896=CARTESIAN_POINT('Ctrl Pts',(6.74940332083147,4.13135835279973,89.5422925922031));
#224897=CARTESIAN_POINT('Ctrl Pts',(6.63050175427649,4.31519024927493,89.5511713779665));
#224898=CARTESIAN_POINT('Ctrl Pts',(6.61828553873177,4.33390319907581,89.5520748284619));
#224899=CARTESIAN_POINT('Ctrl Pts',(6.60088703628817,4.36030931954863,89.5533492411625));
#224900=CARTESIAN_POINT('Ctrl Pts',(6.5957703138219,4.36804544344368,89.5537225460679));
#224901=CARTESIAN_POINT('Ctrl Pts',(6.58639175393044,4.38217111174358,89.5544040789044));
#224902=CARTESIAN_POINT('Ctrl Pts',(6.58213419712742,4.38856347798309,89.5547124598697));
#224903=CARTESIAN_POINT('Ctrl Pts',(6.57352140529801,4.40145413807569,89.5553342605217));
#224904=CARTESIAN_POINT('Ctrl Pts',(6.56916582694053,4.40795219280863,89.5556476673492));
#224905=CARTESIAN_POINT('Ctrl Pts',(6.55848210269377,4.42384015578137,89.5564138715508));
#224906=CARTESIAN_POINT('Ctrl Pts',(6.55214341316844,4.43322297091472,89.5568662882951));
#224907=CARTESIAN_POINT('Ctrl Pts',(6.52931285684642,4.46686186864544,89.5584880283742));
#224908=CARTESIAN_POINT('Ctrl Pts',(6.51270617463136,4.49103992875739,89.5596531965669));
#224909=CARTESIAN_POINT('Ctrl Pts',(6.28838421364665,4.81377464802117,89.5752012715354));
#224910=CARTESIAN_POINT('Ctrl Pts',(6.06044690048255,5.09776612378701,89.5888001135856));
#224911=CARTESIAN_POINT('Ctrl Pts',(5.7467590370768,5.43768713906179,89.6054314335121));
#224912=CARTESIAN_POINT('Ctrl Pts',(5.67840542845199,5.50902832692753,89.6089455902053));
#224913=CARTESIAN_POINT('Ctrl Pts',(5.49274258668274,5.69567825184592,89.6182337838134));
#224914=CARTESIAN_POINT('Ctrl Pts',(5.3731429924138,5.80864075880536,89.6239542223849));
#224915=CARTESIAN_POINT('Ctrl Pts',(4.88013385055123,6.24602522249206,89.6467583500699));
#224916=CARTESIAN_POINT('Ctrl Pts',(4.48021536229425,6.53881892026914,89.6635114877978));
#224917=CARTESIAN_POINT('Ctrl Pts',(3.89351107514106,6.88913184997641,89.6888044120073));
#224918=CARTESIAN_POINT('Ctrl Pts',(3.72802304411072,6.98007232576191,89.6960305867875));
#224919=CARTESIAN_POINT('Ctrl Pts',(3.54346877045847,7.07305230436783,89.704275316243));
#224920=CARTESIAN_POINT('Ctrl Pts',(3.52749540246873,7.08103212861304,89.7049900767568));
#224921=CARTESIAN_POINT('Ctrl Pts',(3.50425389099129,7.09254474579114,89.7060316254028));
#224922=CARTESIAN_POINT('Ctrl Pts',(3.4970070664154,7.0961206218905,89.7063566053943));
#224923=CARTESIAN_POINT('Ctrl Pts',(3.4842231848722,7.10240436680213,89.7069302635156));
#224924=CARTESIAN_POINT('Ctrl Pts',(3.4786884111821,7.10511688357183,89.7071787510516));
#224925=CARTESIAN_POINT('Ctrl Pts',(3.46802550696183,7.11032718092058,89.7076576982074));
#224926=CARTESIAN_POINT('Ctrl Pts',(3.46289783233325,7.11282588984812,89.707888120312));
#224927=CARTESIAN_POINT('Ctrl Pts',(3.4494311584266,7.11937016799325,89.70849353045));
#224928=CARTESIAN_POINT('Ctrl Pts',(3.44108775672879,7.12340662571423,89.7088688780094));
#224929=CARTESIAN_POINT('Ctrl Pts',(3.41120294246717,7.13779985576776,89.7102142012905));
#224930=CARTESIAN_POINT('Ctrl Pts',(3.38962182093009,7.148073600117,89.7111873596248));
#224931=CARTESIAN_POINT('Ctrl Pts',(3.33628080932876,7.17317083149837,89.7135961791555));
#224932=CARTESIAN_POINT('Ctrl Pts',(3.30446845674579,7.18788130076766,89.7150358424057));
#224933=CARTESIAN_POINT('Ctrl Pts',(3.18125506181018,7.24386601711875,89.7206210698701));
#224934=CARTESIAN_POINT('Ctrl Pts',(3.08917144639956,7.28361158012059,89.7248145538047));
#224935=CARTESIAN_POINT('Ctrl Pts',(2.61149700329055,7.47909960635989,89.7465940071312));
#224936=CARTESIAN_POINT('Ctrl Pts',(2.21481825961996,7.60601248213001,89.7647165187889));
#224937=CARTESIAN_POINT('Ctrl Pts',(1.10847252472751,7.86603747543558,89.8136564115216));
#224938=CARTESIAN_POINT('Ctrl Pts',(0.38767293313818,7.93429597415291,89.8435105576992));
#224939=CARTESIAN_POINT('Ctrl Pts',(-0.424582505072139,7.90013692017579,
89.8765519541056));
#224940=CARTESIAN_POINT('Ctrl Pts',(-0.516690679117052,7.89464784364581,
89.8802914154652));
#224941=CARTESIAN_POINT('Ctrl Pts',(-0.649111671634326,7.88442891495911,
89.8856564092761));
#224942=CARTESIAN_POINT('Ctrl Pts',(-0.689516670322647,7.88099816363337,
89.8872919249779));
#224943=CARTESIAN_POINT('Ctrl Pts',(-0.753229285302769,7.87509465803832,
89.8898686025099));
#224944=CARTESIAN_POINT('Ctrl Pts',(-0.776555277528733,7.87282872502474,
89.8908114733203));
#224945=CARTESIAN_POINT('Ctrl Pts',(-0.824081979906426,7.86799860965712,
89.8927316113695));
#224946=CARTESIAN_POINT('Ctrl Pts',(-0.848281624364969,7.86542634068607,
89.8937087985975));
#224947=CARTESIAN_POINT('Ctrl Pts',(-0.903830946221119,7.85926245263223,
89.8959507669192));
#224948=CARTESIAN_POINT('Ctrl Pts',(-0.935171803801835,7.85559484600503,
89.8972148573639));
#224949=CARTESIAN_POINT('Ctrl Pts',(-1.00033311460267,7.84757398016518,
89.8998414412593));
#224950=CARTESIAN_POINT('Ctrl Pts',(-1.03414907418209,7.84318936515009,
89.9012036235906));
#224951=CARTESIAN_POINT('Ctrl Pts',(-1.27281181811938,7.81067374841976,
89.9108117095876));
#224952=CARTESIAN_POINT('Ctrl Pts',(-1.47651727089769,7.77473944208692,
89.9189802029492));
#224953=CARTESIAN_POINT('Ctrl Pts',(-1.84497300572026,7.69473757420097,
89.9337589236691));
#224954=CARTESIAN_POINT('Ctrl Pts',(-2.01015406069892,7.65324723826584,
89.9403862599132));
#224955=CARTESIAN_POINT('Ctrl Pts',(-2.29237348608272,7.57259105006406,
89.9517691599466));
#224956=CARTESIAN_POINT('Ctrl Pts',(-2.41007086980918,7.53595846292259,
89.9565349050008));
#224957=CARTESIAN_POINT('Ctrl Pts',(-2.68788025409696,7.44231767676551,
89.9678669340323));
#224958=CARTESIAN_POINT('Ctrl Pts',(-2.84710504134614,7.38287106254389,
89.9744283754043));
#224959=CARTESIAN_POINT('Ctrl Pts',(-3.23603907112414,7.22320774276778,
89.9907501450847));
#224960=CARTESIAN_POINT('Ctrl Pts',(-3.46313186657929,7.11711953451216,
90.0005407255389));
#224961=CARTESIAN_POINT('Ctrl Pts',(-3.70853159368869,6.98794916479542,
90.0116372971271));
#224962=CARTESIAN_POINT('Ctrl Pts',(-3.73219751766202,6.97533811284435,
90.0127129446798));
#224963=CARTESIAN_POINT('Ctrl Pts',(-3.76729752894372,6.95640431714803,
90.0143169086905));
#224964=CARTESIAN_POINT('Ctrl Pts',(-3.77878088581273,6.95017314250423,
90.0148430432491));
#224965=CARTESIAN_POINT('Ctrl Pts',(-3.79899377745614,6.93914018735975,
90.0157716311196));
#224966=CARTESIAN_POINT('Ctrl Pts',(-3.80772978591342,6.93435030394225,
90.0161737896032));
#224967=CARTESIAN_POINT('Ctrl Pts',(-3.82605657570935,6.92425679699983,
90.0170192151313));
#224968=CARTESIAN_POINT('Ctrl Pts',(-3.8356454280898,6.91894972234862,90.0174625693701));
#224969=CARTESIAN_POINT('Ctrl Pts',(-3.86032232133006,6.90522491179611,
90.018606206727));
#224970=CARTESIAN_POINT('Ctrl Pts',(-3.8753937685858,6.89677769995755,90.0193072731166));
#224971=CARTESIAN_POINT('Ctrl Pts',(-3.94789256821951,6.85583104864192,
90.0226922477453));
#224972=CARTESIAN_POINT('Ctrl Pts',(-4.00493883193406,6.82266369295523,
90.0253936829161));
#224973=CARTESIAN_POINT('Ctrl Pts',(-4.16630066885229,6.72612490785261,
90.0331352077428));
#224974=CARTESIAN_POINT('Ctrl Pts',(-4.26957299051384,6.66104820734109,
90.0382108514524));
#224975=CARTESIAN_POINT('Ctrl Pts',(-4.69408723622533,6.37961239821007,
90.0595156877767));
#224976=CARTESIAN_POINT('Ctrl Pts',(-5.00072802467814,6.14220089914491,
90.0759578256208));
#224977=CARTESIAN_POINT('Ctrl Pts',(-5.43208037849606,5.75443914104567,
90.1002563264523));
#224978=CARTESIAN_POINT('Ctrl Pts',(-5.57065846399161,5.62039443164324,
90.1082739126623));
#224979=CARTESIAN_POINT('Ctrl Pts',(-5.81171831454006,5.36953707134801,
90.1226040288587));
#224980=CARTESIAN_POINT('Ctrl Pts',(-5.91591842822285,5.25451316954187,
90.1289416196723));
#224981=CARTESIAN_POINT('Ctrl Pts',(-6.04233342450657,5.10643614507045,
90.1368255868165));
#224982=CARTESIAN_POINT('Ctrl Pts',(-6.06777161433447,5.07618271690519,
90.1384225499012));
#224983=CARTESIAN_POINT('Ctrl Pts',(-6.10771568750982,5.0279482593246,90.1409472982731));
#224984=CARTESIAN_POINT('Ctrl Pts',(-6.12237131244892,5.01009222817514,
90.1418773649009));
#224985=CARTESIAN_POINT('Ctrl Pts',(-6.14954853077716,4.97668288589911,
90.1436091525843));
#224986=CARTESIAN_POINT('Ctrl Pts',(-6.16208984896194,4.96114587321428,
90.1444111647053));
#224987=CARTESIAN_POINT('Ctrl Pts',(-6.18985843475167,4.92647657669666,
90.1461934136246));
#224988=CARTESIAN_POINT('Ctrl Pts',(-6.20505610196316,4.90732082500633,
90.1471732082018));
#224989=CARTESIAN_POINT('Ctrl Pts',(-6.24922105904906,4.85112033877046,
90.1500335996376));
#224990=CARTESIAN_POINT('Ctrl Pts',(-6.27794722334512,4.81388731497672,
90.1519107153334));
#224991=CARTESIAN_POINT('Ctrl Pts',(-6.44874626807695,4.58837924130525,
90.1631762681679));
#224992=CARTESIAN_POINT('Ctrl Pts',(-6.58267429353875,4.3940817554646,90.1724490387872));
#224993=CARTESIAN_POINT('Ctrl Pts',(-6.94704595983688,3.81133201517904,
90.1993306021307));
#224994=CARTESIAN_POINT('Ctrl Pts',(-7.15317481661213,3.40878451382984,
90.2166965377758));
#224995=CARTESIAN_POINT('Ctrl Pts',(-7.46758790260554,2.63886435708357,
90.2480930516166));
#224996=CARTESIAN_POINT('Ctrl Pts',(-7.5857651023487,2.27698040406869,90.2621934591091));
#224997=CARTESIAN_POINT('Ctrl Pts',(-7.6902188556557,1.85667773415046,90.2784756864801));
#224998=CARTESIAN_POINT('Ctrl Pts',(-7.70245975924784,1.80522349713467,
90.2804680417822));
#224999=CARTESIAN_POINT('Ctrl Pts',(-7.7752604537458,1.48497843806964,90.2928753407252));
#225000=CARTESIAN_POINT('Ctrl Pts',(-7.82225683670705,1.21330974372384,
90.3034248837244));
#225001=CARTESIAN_POINT('Ctrl Pts',(-7.85726750318379,0.920672503587411,
90.3151868848032));
#225002=CARTESIAN_POINT('Ctrl Pts',(-7.85948130156511,0.901578692610415,
90.3159561564195));
#225003=CARTESIAN_POINT('Ctrl Pts',(-7.86265110519296,0.873340215743733,
90.3170967605841));
#225004=CARTESIAN_POINT('Ctrl Pts',(-7.86366079920464,0.864201578742495,
90.3174663360601));
#225005=CARTESIAN_POINT('Ctrl Pts',(-7.86535687073511,0.848601506695357,
90.3180980095393));
#225006=CARTESIAN_POINT('Ctrl Pts',(-7.86605122427481,0.842140937139422,
90.3183598405009));
#225007=CARTESIAN_POINT('Ctrl Pts',(-7.86742411739459,0.829217095454429,
90.3188840852809));
#225008=CARTESIAN_POINT('Ctrl Pts',(-7.86810265383972,0.822753828731993,
90.3191464989553));
#225009=CARTESIAN_POINT('Ctrl Pts',(-7.86944749626716,0.809789975935379,
90.3196733265499));
#225010=CARTESIAN_POINT('Ctrl Pts',(-7.87011371352183,0.803289385943585,
90.3199377433063));
#225011=CARTESIAN_POINT('Ctrl Pts',(-7.87161333374309,0.788475948970979,
90.3205408609559));
#225012=CARTESIAN_POINT('Ctrl Pts',(-7.87244162350826,0.780162599648683,
90.3208797407798));
#225013=CARTESIAN_POINT('Ctrl Pts',(-7.87451196677343,0.759044005517582,
90.3217416700244));
#225014=CARTESIAN_POINT('Ctrl Pts',(-7.87573595249364,0.746237041021348,
90.322265364541));
#225015=CARTESIAN_POINT('Ctrl Pts',(-7.89962297498831,0.489693004688716,
90.3327765289753));
#225016=CARTESIAN_POINT('Ctrl Pts',(-7.91098842582327,0.245089548895191,
90.343250676027));
#225017=CARTESIAN_POINT('Ctrl Pts',(-7.91099999116524,0.000373876422793476,
90.3540864678166));
#225018=CARTESIAN_POINT('',(-7.90697312323461,0.00395131442269322,92.3576684917631));
#225019=CARTESIAN_POINT('Ctrl Pts',(-7.91729508967814,0.000522195832882638,
90.3577115106449));
#225020=CARTESIAN_POINT('Ctrl Pts',(-7.90068245752772,-2.46740656103677,
90.4572310833883));
#225021=CARTESIAN_POINT('Ctrl Pts',(-5.36653499073731,-7.5605983309967,
90.6627202333486));
#225022=CARTESIAN_POINT('Ctrl Pts',(3.36342892092229,-8.73984422960058,
90.9741789605246));
#225023=CARTESIAN_POINT('Ctrl Pts',(8.17091791536676,-3.04564661273073,
91.2391029035664));
#225024=CARTESIAN_POINT('Ctrl Pts',(7.877328711738,2.37408643071016,91.4510420579989));
#225025=CARTESIAN_POINT('Ctrl Pts',(5.11028731654382,7.0745385235803,91.6629812124325));
#225026=CARTESIAN_POINT('Ctrl Pts',(-0.58978711048923,8.70507802341428,
91.8749203668651));
#225027=CARTESIAN_POINT('Ctrl Pts',(-5.43791012976105,6.18501921579393,
92.0868595212981));
#225028=CARTESIAN_POINT('Ctrl Pts',(-7.52009634502631,3.17273990218627,
92.230113966728));
#225029=CARTESIAN_POINT('Ctrl Pts',(-7.90704442232692,0.931371954907319,
92.3203836235497));
#225030=CARTESIAN_POINT('Ctrl Pts',(-7.90697312323461,0.00395131442269322,
92.3576684917631));
#225031=CARTESIAN_POINT('',(-7.91099999858106,-0.000149834679674665,96.3535680629415));
#225032=CARTESIAN_POINT('Ctrl Pts',(-7.9109989942205,0.00398916560548777,
92.3599925715499));
#225033=CARTESIAN_POINT('Ctrl Pts',(-7.91100938498044,-0.0166169709954872,
92.3608274381967));
#225034=CARTESIAN_POINT('Ctrl Pts',(-7.91093926512935,-0.0372231259525087,
92.3616613362639));
#225035=CARTESIAN_POINT('Ctrl Pts',(-7.91063655989461,-0.0786321807808416,
92.363335207322));
#225036=CARTESIAN_POINT('Ctrl Pts',(-7.91040242391774,-0.0994348909806759,
92.3641751545412));
#225037=CARTESIAN_POINT('Ctrl Pts',(-7.90978919970167,-0.139777527739423,
92.3658022719579));
#225038=CARTESIAN_POINT('Ctrl Pts',(-7.90941975715157,-0.159317446761974,
92.366589550345));
#225039=CARTESIAN_POINT('Ctrl Pts',(-7.90854413621853,-0.198037272686675,
92.3681480490989));
#225040=CARTESIAN_POINT('Ctrl Pts',(-7.90804058205259,-0.217217105688372,
92.36891929487));
#225041=CARTESIAN_POINT('Ctrl Pts',(-7.90689568000985,-0.255514351188711,
92.3704578308992));
#225042=CARTESIAN_POINT('Ctrl Pts',(-7.90625476052629,-0.27463164842514,
92.3712251209344));
#225043=CARTESIAN_POINT('Ctrl Pts',(-7.90435117265783,-0.325862558156829,
92.3732794806724));
#225044=CARTESIAN_POINT('Ctrl Pts',(-7.90296213596042,-0.357971166897346,
92.3745650976691));
#225045=CARTESIAN_POINT('Ctrl Pts',(-7.89707498725394,-0.477222900635277,
92.3793333297991));
#225046=CARTESIAN_POINT('Ctrl Pts',(-7.8913308281871,-0.564298694092066,
92.382801926403));
#225047=CARTESIAN_POINT('Ctrl Pts',(-7.83017837327691,-1.30460721407445,
92.4122146422615));
#225048=CARTESIAN_POINT('Ctrl Pts',(-7.69520025481478,-1.94876153228048,
92.4375076951123));
#225049=CARTESIAN_POINT('Ctrl Pts',(-7.36253101271792,-2.91772214554893,
92.4761089506171));
#225050=CARTESIAN_POINT('Ctrl Pts',(-7.21851089450144,-3.25776959262321,
92.4897858538874));
#225051=CARTESIAN_POINT('Ctrl Pts',(-6.94877001984275,-3.78809420973568,
92.5121839715152));
#225052=CARTESIAN_POINT('Ctrl Pts',(-6.83765174551799,-3.98516943178604,
92.5207723245413));
#225053=CARTESIAN_POINT('Ctrl Pts',(-6.66814912926701,-4.25778233649769,
92.5332958043001));
#225054=CARTESIAN_POINT('Ctrl Pts',(-6.61660548561992,-4.3374479095469,
92.5370378978809));
#225055=CARTESIAN_POINT('Ctrl Pts',(-6.5548931927439,-4.4291694353639,92.5414612985536));
#225056=CARTESIAN_POINT('Ctrl Pts',(-6.54610522256729,-4.44214734860757,
92.5420899051164));
#225057=CARTESIAN_POINT('Ctrl Pts',(-6.53264214494182,-4.46190266525581,
92.5430510659916));
#225058=CARTESIAN_POINT('Ctrl Pts',(-6.52799490369737,-4.46869906402541,
92.5433825088896));
#225059=CARTESIAN_POINT('Ctrl Pts',(-6.51953146434152,-4.48103511887802,
92.5439855368851));
#225060=CARTESIAN_POINT('Ctrl Pts',(-6.51571879082492,-4.48657719088195,
92.5442569781028));
#225061=CARTESIAN_POINT('Ctrl Pts',(-6.50806621359993,-4.49767058837432,
92.5448013800863));
#225062=CARTESIAN_POINT('Ctrl Pts',(-6.50422626476366,-4.50322187534129,
92.5450743426261));
#225063=CARTESIAN_POINT('Ctrl Pts',(-6.49334867548826,-4.51890430825782,
92.5458469986067));
#225064=CARTESIAN_POINT('Ctrl Pts',(-6.48629445341719,-4.52902389375338,
92.5463473934074));
#225065=CARTESIAN_POINT('Ctrl Pts',(-6.4568179292362,-4.57109911862609,
92.54843565204));
#225066=CARTESIAN_POINT('Ctrl Pts',(-6.43418314635648,-4.60290474521572,
92.5500327995815));
#225067=CARTESIAN_POINT('Ctrl Pts',(-6.07306714245963,-5.10246404580114,
92.575431774828));
#225068=CARTESIAN_POINT('Ctrl Pts',(-5.68468124080384,-5.53185391562479,
92.6020957239176));
#225069=CARTESIAN_POINT('Ctrl Pts',(-5.11885266772687,-6.03436248066652,
92.6367696783688));
#225070=CARTESIAN_POINT('Ctrl Pts',(-4.98052718605918,-6.14902709888229,
92.6449725018298));
#225071=CARTESIAN_POINT('Ctrl Pts',(-4.63168936426824,-6.41869534487419,
92.6648755179029));
#225072=CARTESIAN_POINT('Ctrl Pts',(-4.41716260374373,-6.56817208396009,
92.6764538430598));
#225073=CARTESIAN_POINT('Ctrl Pts',(-4.06681200061117,-6.78734453143579,
92.6942107741201));
#225074=CARTESIAN_POINT('Ctrl Pts',(-3.93570524263836,-6.86419937992903,
92.7006189097873));
#225075=CARTESIAN_POINT('Ctrl Pts',(-3.75716715237918,-6.96206032262379,
92.7090288612561));
#225076=CARTESIAN_POINT('Ctrl Pts',(-3.71163026549438,-6.98644329038017,
92.7111470889938));
#225077=CARTESIAN_POINT('Ctrl Pts',(-3.64541325462485,-7.02106939495927,
92.7141889823475));
#225078=CARTESIAN_POINT('Ctrl Pts',(-3.62492246132342,-7.03167052746739,
92.7151250402943));
#225079=CARTESIAN_POINT('Ctrl Pts',(-3.5882089842486,-7.05046151082425,
92.7167928508726));
#225080=CARTESIAN_POINT('Ctrl Pts',(-3.57200394584062,-7.05868536250372,
92.7175257785663));
#225081=CARTESIAN_POINT('Ctrl Pts',(-3.54763615075159,-7.07094630613488,
92.7186230734468));
#225082=CARTESIAN_POINT('Ctrl Pts',(-3.53949457859831,-7.07502523325229,
92.7189888877827));
#225083=CARTESIAN_POINT('Ctrl Pts',(-3.52548750805267,-7.08201254536804,
92.7196168693265));
#225084=CARTESIAN_POINT('Ctrl Pts',(-3.51962541797617,-7.08492771872567,
92.7198792710638));
#225085=CARTESIAN_POINT('Ctrl Pts',(-3.50755256984423,-7.09091277391166,
92.7204188308959));
#225086=CARTESIAN_POINT('Ctrl Pts',(-3.50134138404111,-7.09398178106876,
92.7206959586091));
#225087=CARTESIAN_POINT('Ctrl Pts',(-3.48639139773006,-7.10134429684321,
92.7213618800303));
#225088=CARTESIAN_POINT('Ctrl Pts',(-3.47764867637372,-7.10562984436176,
92.7217503987316));
#225089=CARTESIAN_POINT('Ctrl Pts',(-3.45083963354855,-7.11870989416034,
92.7229389891278));
#225090=CARTESIAN_POINT('Ctrl Pts',(-3.43274763695967,-7.12745174674585,
92.7237372452002));
#225091=CARTESIAN_POINT('Ctrl Pts',(-3.22890593023575,-7.22498962682392,
92.7326881233595));
#225092=CARTESIAN_POINT('Ctrl Pts',(-3.03978456449599,-7.30657415660692,
92.740588629205));
#225093=CARTESIAN_POINT('Ctrl Pts',(-2.49757698115558,-7.51577367860479,
92.7622555933756));
#225094=CARTESIAN_POINT('Ctrl Pts',(-2.13828685354568,-7.62577860371302,
92.7754524668928));
#225095=CARTESIAN_POINT('Ctrl Pts',(-1.49926631792096,-7.772692036761,92.7979739588008));
#225096=CARTESIAN_POINT('Ctrl Pts',(-1.22285744503376,-7.82094367356461,
92.8074265627922));
#225097=CARTESIAN_POINT('Ctrl Pts',(-0.832815915349954,-7.86784506087785,
92.820879457616));
#225098=CARTESIAN_POINT('Ctrl Pts',(-0.720887854965985,-7.87888877844551,
92.824754039082));
#225099=CARTESIAN_POINT('Ctrl Pts',(-0.452133448357972,-7.89963135618467,
92.8341568930095));
#225100=CARTESIAN_POINT('Ctrl Pts',(-0.295182120274044,-7.90705158855909,
92.8397288157136));
#225101=CARTESIAN_POINT('Ctrl Pts',(0.0501372317934248,-7.91308148057443,
92.8523405174425));
#225102=CARTESIAN_POINT('Ctrl Pts',(0.238439895594762,-7.9096466523416,
92.8594480916385));
#225103=CARTESIAN_POINT('Ctrl Pts',(0.453820756865387,-7.89802001993127,
92.8680060939527));
#225104=CARTESIAN_POINT('Ctrl Pts',(0.481204685471592,-7.89639889639212,
92.8691021304385));
#225105=CARTESIAN_POINT('Ctrl Pts',(0.515931635378348,-7.89416175591615,
92.8705027322171));
#225106=CARTESIAN_POINT('Ctrl Pts',(0.523283267102684,-7.89367784385905,
92.8707998435465));
#225107=CARTESIAN_POINT('Ctrl Pts',(0.535024615419098,-7.89288850952927,
92.8712753449931));
#225108=CARTESIAN_POINT('Ctrl Pts',(0.53941478669654,-7.89258969228144,
92.8714533577446));
#225109=CARTESIAN_POINT('Ctrl Pts',(0.547708930880645,-7.89201819830882,
92.8717900870345));
#225110=CARTESIAN_POINT('Ctrl Pts',(0.551612956943343,-7.89174628716801,
92.8719487594642));
#225111=CARTESIAN_POINT('Ctrl Pts',(0.560421157791934,-7.89112623762177,
92.8723071516092));
#225112=CARTESIAN_POINT('Ctrl Pts',(0.565325209022588,-7.89077642440936,
92.8725069683021));
#225113=CARTESIAN_POINT('Ctrl Pts',(0.577851127287873,-7.88987119515674,
92.8730180574294));
#225114=CARTESIAN_POINT('Ctrl Pts',(0.585472520853694,-7.88930930617988,
92.8733297085931));
#225115=CARTESIAN_POINT('Ctrl Pts',(0.630884317619753,-7.88589514434616,
92.8751907725022));
#225116=CARTESIAN_POINT('Ctrl Pts',(0.668654019531223,-7.88278243742453,
92.8767555422772));
#225117=CARTESIAN_POINT('Ctrl Pts',(1.31915090443823,-7.82446446900298,
92.90397700445));
#225118=CARTESIAN_POINT('Ctrl Pts',(1.92337088229537,-7.69824570717951,
92.9332463235326));
#225119=CARTESIAN_POINT('Ctrl Pts',(2.79779135388342,-7.40610513746522,
92.9759252735163));
#225120=CARTESIAN_POINT('Ctrl Pts',(3.08286788282679,-7.29204886941688,
92.9899285621019));
#225121=CARTESIAN_POINT('Ctrl Pts',(3.55501379689497,-7.07049573562311,
93.0128962197114));
#225122=CARTESIAN_POINT('Ctrl Pts',(3.74562634417476,-6.97139342888992,
93.0221060445501));
#225123=CARTESIAN_POINT('Ctrl Pts',(3.98772276131054,-6.83272380931817,
93.0336953026738));
#225124=CARTESIAN_POINT('Ctrl Pts',(4.04307394327187,-6.80011770785419,
93.0363376968675));
#225125=CARTESIAN_POINT('Ctrl Pts',(4.12076090437963,-6.75307020624562,
93.0400364374367));
#225126=CARTESIAN_POINT('Ctrl Pts',(4.14342960387535,-6.73918532010579,
93.0411145054489));
#225127=CARTESIAN_POINT('Ctrl Pts',(4.17777028518914,-6.71791241639486,
93.0427458869343));
#225128=CARTESIAN_POINT('Ctrl Pts',(4.18949349500327,-6.71060772569821,
93.0433024907732));
#225129=CARTESIAN_POINT('Ctrl Pts',(4.20856312930315,-6.69865605539308,
93.0442073887338));
#225130=CARTESIAN_POINT('Ctrl Pts',(4.21592110589361,-6.69402762104716,
93.0445564186348));
#225131=CARTESIAN_POINT('Ctrl Pts',(4.23016462653967,-6.68503512985991,
93.0452318334574));
#225132=CARTESIAN_POINT('Ctrl Pts',(4.23705108102411,-6.68067254042836,
93.0455582761753));
#225133=CARTESIAN_POINT('Ctrl Pts',(4.24897797505282,-6.67309095809721,
93.0461234716154));
#225134=CARTESIAN_POINT('Ctrl Pts',(4.25402152347942,-6.66987688383469,
93.0463624202564));
#225135=CARTESIAN_POINT('Ctrl Pts',(4.26449053864898,-6.66318864741752,
93.0468582954444));
#225136=CARTESIAN_POINT('Ctrl Pts',(4.26991541733665,-6.6597135699945,93.0471151851519));
#225137=CARTESIAN_POINT('Ctrl Pts',(4.28472824441541,-6.65019920586704,
93.0478164564955));
#225138=CARTESIAN_POINT('Ctrl Pts',(4.29410768227187,-6.64414665857638,
93.0482603066853));
#225139=CARTESIAN_POINT('Ctrl Pts',(4.32972733759817,-6.62105437828654,
93.0499451716143));
#225140=CARTESIAN_POINT('Ctrl Pts',(4.35587936853312,-6.60387877352104,
93.0511807229141));
#225141=CARTESIAN_POINT('Ctrl Pts',(4.76406439674376,-6.33231956949401,
93.0704440758127));
#225142=CARTESIAN_POINT('Ctrl Pts',(5.12337140268718,-6.04530470249025,
93.0870273555765));
#225143=CARTESIAN_POINT('Ctrl Pts',(5.81347914967821,-5.38807634900018,
93.1199413898806));
#225144=CARTESIAN_POINT('Ctrl Pts',(6.13846185931715,-5.01469429243429,
93.1360883442968));
#225145=CARTESIAN_POINT('Ctrl Pts',(6.47235547374767,-4.54958447763153,
93.1560966421463));
#225146=CARTESIAN_POINT('Ctrl Pts',(6.51725684192208,-4.48502699800584,
93.1588736174151));
#225147=CARTESIAN_POINT('Ctrl Pts',(6.62741212455137,-4.32150205945998,
93.1659349775229));
#225148=CARTESIAN_POINT('Ctrl Pts',(6.69141659073724,-4.22171927942477,
93.1702682016949));
#225149=CARTESIAN_POINT('Ctrl Pts',(6.81100185861919,-4.02573097601757,
93.1789020253756));
#225150=CARTESIAN_POINT('Ctrl Pts',(6.86684546382416,-3.92971849728949,
93.1831865549045));
#225151=CARTESIAN_POINT('Ctrl Pts',(6.9300234931657,-3.81563493860856,93.1883802159809));
#225152=CARTESIAN_POINT('Ctrl Pts',(6.93933778128576,-3.79866907542071,
93.1891552148171));
#225153=CARTESIAN_POINT('Ctrl Pts',(6.95155493025224,-3.77622080013829,
93.190184345447));
#225154=CARTESIAN_POINT('Ctrl Pts',(6.95451381331411,-3.77076876778859,
93.1904345784268));
#225155=CARTESIAN_POINT('Ctrl Pts',(6.95936724639826,-3.76180069667185,
93.1908466680273));
#225156=CARTESIAN_POINT('Ctrl Pts',(6.96126554484257,-3.75828670617201,
93.1910082591212));
#225157=CARTESIAN_POINT('Ctrl Pts',(6.96495386352822,-3.75144678024166,
93.1913230257674));
#225158=CARTESIAN_POINT('Ctrl Pts',(6.96674416496649,-3.7481209966951,93.1914761817259));
#225159=CARTESIAN_POINT('Ctrl Pts',(6.97089350013284,-3.74039967058265,
93.1918320023187));
#225160=CARTESIAN_POINT('Ctrl Pts',(6.97325075703691,-3.73600318055833,
93.1920347892064));
#225161=CARTESIAN_POINT('Ctrl Pts',(6.98086898587666,-3.72176218937561,
93.1926922393008));
#225162=CARTESIAN_POINT('Ctrl Pts',(6.98611325987225,-3.7119088229527,93.1931480394696));
#225163=CARTESIAN_POINT('Ctrl Pts',(7.03523950192268,-3.61913357369488,
93.1974479609954));
#225164=CARTESIAN_POINT('Ctrl Pts',(7.07766230447068,-3.53545153765817,
93.2013886367707));
#225165=CARTESIAN_POINT('Ctrl Pts',(7.34323923851818,-2.98763611351291,
93.2274853362286));
#225166=CARTESIAN_POINT('Ctrl Pts',(7.52209281168821,-2.50343451769239,
93.251858772893));
#225167=CARTESIAN_POINT('Ctrl Pts',(7.73667318431216,-1.68456651734583,
93.2916331421163));
#225168=CARTESIAN_POINT('Ctrl Pts',(7.80048132052756,-1.35881894988339,
93.3071163607108));
#225169=CARTESIAN_POINT('Ctrl Pts',(7.88312283668575,-0.729495809077691,
93.3357927506921));
#225170=CARTESIAN_POINT('Ctrl Pts',(7.90528555523668,-0.426939614350551,
93.3490467108417));
#225171=CARTESIAN_POINT('Ctrl Pts',(7.91189723898176,-0.00460770748252659,
93.3667292619499));
#225172=CARTESIAN_POINT('Ctrl Pts',(7.91106799101316,0.114647751889499,
93.3716335736553));
#225173=CARTESIAN_POINT('Ctrl Pts',(7.90704156296035,0.250804025094959,
93.3771360921947));
#225174=CARTESIAN_POINT('Ctrl Pts',(7.9064854089161,0.267763740682974,93.3778197792648));
#225175=CARTESIAN_POINT('Ctrl Pts',(7.90556408676369,0.293346124639158,
93.3788485144518));
#225176=CARTESIAN_POINT('Ctrl Pts',(7.90523937084471,0.301970145961379,
93.3791948714548));
#225177=CARTESIAN_POINT('Ctrl Pts',(7.90465493970392,0.316844468840303,
93.3797915019353));
#225178=CARTESIAN_POINT('Ctrl Pts',(7.90440192196381,0.323095016218909,
93.3800419917666));
#225179=CARTESIAN_POINT('Ctrl Pts',(7.90386391937633,0.336006841605739,
93.3805589612405));
#225180=CARTESIAN_POINT('Ctrl Pts',(7.90357792679258,0.342668074144689,
93.3808254081194));
#225181=CARTESIAN_POINT('Ctrl Pts',(7.90278128627859,0.360691418258543,
93.3815456391873));
#225182=CARTESIAN_POINT('Ctrl Pts',(7.9022545552573,0.372052823275241,93.3819989037226));
#225183=CARTESIAN_POINT('Ctrl Pts',(7.90020875533877,0.414214410003667,
93.3836781907799));
#225184=CARTESIAN_POINT('Ctrl Pts',(7.8985340914399,0.445006954890051,93.3848991939718));
#225185=CARTESIAN_POINT('Ctrl Pts',(7.86824129531418,0.947776927959096,
93.4047485300279));
#225186=CARTESIAN_POINT('Ctrl Pts',(7.79754359296911,1.41628977528384,93.421913978139));
#225187=CARTESIAN_POINT('Ctrl Pts',(7.56526084763376,2.36802920960121,93.456195367089));
#225188=CARTESIAN_POINT('Ctrl Pts',(7.3980855505712,2.84763391166258,93.4731518462819));
#225189=CARTESIAN_POINT('Ctrl Pts',(7.09080731427141,3.51517012172091,93.4997264244385));
#225190=CARTESIAN_POINT('Ctrl Pts',(6.98649305502315,3.71818323144582,93.5082665550157));
#225191=CARTESIAN_POINT('Ctrl Pts',(6.85505131169054,3.9488717828786,93.5187732418155));
#225192=CARTESIAN_POINT('Ctrl Pts',(6.83632591529052,3.98120142137484,93.5202632020728));
#225193=CARTESIAN_POINT('Ctrl Pts',(6.81196052771146,4.0225897837538,93.5221922560521));
#225194=CARTESIAN_POINT('Ctrl Pts',(6.80653004293423,4.03177176593947,93.5226215917408));
#225195=CARTESIAN_POINT('Ctrl Pts',(6.79775449156869,4.04654139772446,93.523314388061));
#225196=CARTESIAN_POINT('Ctrl Pts',(6.79442105717944,4.05213596866749,93.5235773190727));
#225197=CARTESIAN_POINT('Ctrl Pts',(6.78806251204761,4.06277773919609,93.5240784151784));
#225198=CARTESIAN_POINT('Ctrl Pts',(6.78503866942263,4.06782569436965,93.5243165232858));
#225199=CARTESIAN_POINT('Ctrl Pts',(6.77813728577621,4.07931765075101,93.5248595216778));
#225200=CARTESIAN_POINT('Ctrl Pts',(6.77425618525469,4.08575950058308,93.5251645695953));
#225201=CARTESIAN_POINT('Ctrl Pts',(6.76267561736756,4.10491906333621,93.5260738268494));
#225202=CARTESIAN_POINT('Ctrl Pts',(6.75494950345145,4.11762057800221,93.5266791969676));
#225203=CARTESIAN_POINT('Ctrl Pts',(6.70063243420383,4.20635201233481,93.5309260961685));
#225204=CARTESIAN_POINT('Ctrl Pts',(6.65279568702758,4.28160964000401,93.5346199660138));
#225205=CARTESIAN_POINT('Ctrl Pts',(6.49060547752171,4.52748777581894,93.5469626826401));
#225206=CARTESIAN_POINT('Ctrl Pts',(6.37088220214842,4.69446053740996,93.5557882744055));
#225207=CARTESIAN_POINT('Ctrl Pts',(5.73738355623192,5.50904076248536,93.6006092768132));
#225208=CARTESIAN_POINT('Ctrl Pts',(5.13074565646177,6.07806307536993,93.6371338650679));
#225209=CARTESIAN_POINT('Ctrl Pts',(4.40287684945072,6.57278043374012,93.6730914924105));
#225210=CARTESIAN_POINT('Ctrl Pts',(4.35845152702862,6.602322890394,93.675261735693));
#225211=CARTESIAN_POINT('Ctrl Pts',(4.27987143886916,6.6534391867632,93.6790589930235));
#225212=CARTESIAN_POINT('Ctrl Pts',(4.24584397623971,6.67520497888694,93.6806899270685));
#225213=CARTESIAN_POINT('Ctrl Pts',(4.19668176798468,6.70612375777788,93.6830272510761));
#225214=CARTESIAN_POINT('Ctrl Pts',(4.18168077487292,6.71548804007421,93.6837379134559));
#225215=CARTESIAN_POINT('Ctrl Pts',(4.15561175855939,6.73164025207384,93.6849685285133));
#225216=CARTESIAN_POINT('Ctrl Pts',(4.14455820671209,6.73845136834701,93.6854889619464));
#225217=CARTESIAN_POINT('Ctrl Pts',(4.12327685056646,6.75149260785739,93.6864883362116));
#225218=CARTESIAN_POINT('Ctrl Pts',(4.11305157122084,6.75772677708905,93.6869673610576));
#225219=CARTESIAN_POINT('Ctrl Pts',(4.08892038560573,6.7723640676628,93.6880951185734));
#225220=CARTESIAN_POINT('Ctrl Pts',(4.07500265616423,6.78074762392845,93.6887434352382));
#225221=CARTESIAN_POINT('Ctrl Pts',(4.03374708655778,6.80542565176369,93.6906589449656));
#225222=CARTESIAN_POINT('Ctrl Pts',(4.00633655104851,6.8215981498265,93.691923520908));
#225223=CARTESIAN_POINT('Ctrl Pts',(3.73788080786514,6.97781359786196,93.7042300672765));
#225224=CARTESIAN_POINT('Ctrl Pts',(3.48968357178826,7.10519215339375,93.7149812447937));
#225225=CARTESIAN_POINT('Ctrl Pts',(2.8198451895752,7.40537853194782,93.7426375706072));
#225226=CARTESIAN_POINT('Ctrl Pts',(2.38913294412111,7.5553429467244,93.7590342458436));
#225227=CARTESIAN_POINT('Ctrl Pts',(1.74852787663755,7.71808851307111,93.7831396311856));
#225228=CARTESIAN_POINT('Ctrl Pts',(1.54724990728456,7.76094413759684,93.7906870954495));
#225229=CARTESIAN_POINT('Ctrl Pts',(1.17116705281317,7.82580600339481,93.8050369900584));
#225230=CARTESIAN_POINT('Ctrl Pts',(0.996855508088804,7.84991374547872,
93.8117857421288));
#225231=CARTESIAN_POINT('Ctrl Pts',(0.793540975126717,7.87115152685873,
93.8199037060692));
#225232=CARTESIAN_POINT('Ctrl Pts',(0.765172884231253,7.87395987200559,
93.8210419599621));
#225233=CARTESIAN_POINT('Ctrl Pts',(0.727955951045604,7.87744120037873,
93.8225432434986));
#225234=CARTESIAN_POINT('Ctrl Pts',(0.719120049607398,7.87825273048601,
93.8229002614678));
#225235=CARTESIAN_POINT('Ctrl Pts',(0.704712803339993,7.87955151909762,
93.8234833773497));
#225236=CARTESIAN_POINT('Ctrl Pts',(0.699142258559244,7.88004773966276,
93.8237090785524));
#225237=CARTESIAN_POINT('Ctrl Pts',(0.688418471399684,7.88099154704123,
93.8241440429175));
#225238=CARTESIAN_POINT('Ctrl Pts',(0.683265305541657,7.88143998761343,
93.8243532677057));
#225239=CARTESIAN_POINT('Ctrl Pts',(0.671468575278274,7.88245491013709,
93.8248327141972));
#225240=CARTESIAN_POINT('Ctrl Pts',(0.664824733326373,7.88301804713609,
93.8251030873265));
#225241=CARTESIAN_POINT('Ctrl Pts',(0.643952603914165,7.88476061015299,
93.8259536113917));
#225242=CARTESIAN_POINT('Ctrl Pts',(0.629721888180468,7.88590991419918,
93.8265351467812));
#225243=CARTESIAN_POINT('Ctrl Pts',(0.494167361238814,7.89648833371844,
93.8320908375226));
#225244=CARTESIAN_POINT('Ctrl Pts',(0.372657028259306,7.90315449398576,
93.8372034640449));
#225245=CARTESIAN_POINT('Ctrl Pts',(0.044010437756169,7.91358911027385,
93.851326418367));
#225246=CARTESIAN_POINT('Ctrl Pts',(-0.163197428941168,7.91202803036976,
93.8605406246455));
#225247=CARTESIAN_POINT('Ctrl Pts',(-0.942609019082659,7.87552550398702,
93.8958621692219));
#225248=CARTESIAN_POINT('Ctrl Pts',(-1.51052601414932,7.78657729178238,
93.922822854702));
#225249=CARTESIAN_POINT('Ctrl Pts',(-2.45583749880284,7.53111150939652,
93.9665911341828));
#225250=CARTESIAN_POINT('Ctrl Pts',(-2.8390950056219,7.39515911864513,93.98403220925));
#225251=CARTESIAN_POINT('Ctrl Pts',(-3.23336712280999,7.22010370088025,
94.0015458693013));
#225252=CARTESIAN_POINT('Ctrl Pts',(-3.2564287748672,7.20973176001715,94.0025688248642));
#225253=CARTESIAN_POINT('Ctrl Pts',(-3.289144640983,7.19482885433623,94.0040180158385));
#225254=CARTESIAN_POINT('Ctrl Pts',(-3.29883992084115,7.19038871621482,
94.0044472299036));
#225255=CARTESIAN_POINT('Ctrl Pts',(-3.31551391633487,7.18271171976697,
94.0051849690741));
#225256=CARTESIAN_POINT('Ctrl Pts',(-3.32249693096221,7.17948426579795,
94.0054938030563));
#225257=CARTESIAN_POINT('Ctrl Pts',(-3.33582056485977,7.17330266259076,
94.006082816973));
#225258=CARTESIAN_POINT('Ctrl Pts',(-3.34216199265932,7.17035028050864,
94.0063630547244));
#225259=CARTESIAN_POINT('Ctrl Pts',(-3.35695089770015,7.16344112044127,
94.0070163565512));
#225260=CARTESIAN_POINT('Ctrl Pts',(-3.36539531719436,7.15947780046607,
94.0073892043283));
#225261=CARTESIAN_POINT('Ctrl Pts',(-3.39516599821417,7.14544086325066,
94.008703028755));
#225262=CARTESIAN_POINT('Ctrl Pts',(-3.41645429269883,7.13528677512961,
94.0096413426246));
#225263=CARTESIAN_POINT('Ctrl Pts',(-3.64427234825545,7.02536883700728,
94.0196707365327));
#225264=CARTESIAN_POINT('Ctrl Pts',(-3.84642311307951,6.91675987626382,
94.0284595773323));
#225265=CARTESIAN_POINT('Ctrl Pts',(-4.20178737822674,6.70542956646218,
94.0438416196255));
#225266=CARTESIAN_POINT('Ctrl Pts',(-4.35666790088356,6.60584978440244,
94.0505218341207));
#225267=CARTESIAN_POINT('Ctrl Pts',(-5.05429608060325,6.12209553391066,
94.0807859764034));
#225268=CARTESIAN_POINT('Ctrl Pts',(-5.55067548035882,5.67590264991658,
94.1026395842793));
#225269=CARTESIAN_POINT('Ctrl Pts',(-6.06629520315752,5.07930088074213,
94.1313435886781));
#225270=CARTESIAN_POINT('Ctrl Pts',(-6.14500339632481,4.98379035997132,
94.1359314726989));
#225271=CARTESIAN_POINT('Ctrl Pts',(-6.29614708634102,4.79135498140239,
94.1452336258219));
#225272=CARTESIAN_POINT('Ctrl Pts',(-6.3686573440028,4.69454493083037,94.1499490730039));
#225273=CARTESIAN_POINT('Ctrl Pts',(-6.44774678490864,4.58374443732366,
94.1553886517839));
#225274=CARTESIAN_POINT('Ctrl Pts',(-6.4565348812596,4.57135745616198,94.1559972312646));
#225275=CARTESIAN_POINT('Ctrl Pts',(-6.46969394550482,4.5526958745461,94.1569146884381));
#225276=CARTESIAN_POINT('Ctrl Pts',(-6.47409160484178,4.54644007617127,
94.1572223430037));
#225277=CARTESIAN_POINT('Ctrl Pts',(-6.48164502223485,4.53566193803275,
94.1577525641087));
#225278=CARTESIAN_POINT('Ctrl Pts',(-6.48480513953105,4.53114264976563,
94.1579749354299));
#225279=CARTESIAN_POINT('Ctrl Pts',(-6.49130864574305,4.52182123755353,
94.1584336900456));
#225280=CARTESIAN_POINT('Ctrl Pts',(-6.49465143644311,4.51701870237035,
94.1586700993812));
#225281=CARTESIAN_POINT('Ctrl Pts',(-6.50364540311766,4.50406658721538,
94.1593078105225));
#225282=CARTESIAN_POINT('Ctrl Pts',(-6.5092865786265,4.49591009561214,94.1597095435943));
#225283=CARTESIAN_POINT('Ctrl Pts',(-6.52999850518052,4.46584233423246,
94.1611909318397));
#225284=CARTESIAN_POINT('Ctrl Pts',(-6.54497399374246,4.44386584336544,
94.1622745649921));
#225285=CARTESIAN_POINT('Ctrl Pts',(-6.64584547236964,4.29422125743691,
94.1696573567015));
#225286=CARTESIAN_POINT('Ctrl Pts',(-6.72810940619944,4.16414928980825,
94.1760933792891));
#225287=CARTESIAN_POINT('Ctrl Pts',(-6.81040714676181,4.02521223178472,
94.1829337085062));
#225288=CARTESIAN_POINT('Ctrl Pts',(-6.81427950313355,4.01865324064847,
94.18325655262));
#225289=CARTESIAN_POINT('Ctrl Pts',(-6.83221206120797,3.98817865642534,
94.1847561796137));
#225290=CARTESIAN_POINT('Ctrl Pts',(-6.84615582458517,3.96419488157962,
94.1859353105009));
#225291=CARTESIAN_POINT('Ctrl Pts',(-6.8728184469609,3.91777395524983,94.1882149379885));
#225292=CARTESIAN_POINT('Ctrl Pts',(-6.88555432364497,3.89534694443504,
94.1893151187998));
#225293=CARTESIAN_POINT('Ctrl Pts',(-7.2239141726075,3.29267389086386,94.2188435588778));
#225294=CARTESIAN_POINT('Ctrl Pts',(-7.4751656363043,2.67369422110814,94.2479024486583));
#225295=CARTESIAN_POINT('Ctrl Pts',(-7.72152983219981,1.74601342728185,
94.2880591896939));
#225296=CARTESIAN_POINT('Ctrl Pts',(-7.78115169498604,1.45748777314945,
94.300164573372));
#225297=CARTESIAN_POINT('Ctrl Pts',(-7.84209318887623,1.04864093691202,
94.317040744289));
#225298=CARTESIAN_POINT('Ctrl Pts',(-7.85697562913057,0.930595354712951,
94.321885558924));
#225299=CARTESIAN_POINT('Ctrl Pts',(-7.87752105116231,0.73155060892787,
94.3300053577431));
#225300=CARTESIAN_POINT('Ctrl Pts',(-7.88460965892463,0.650718720851011,
94.3332890979757));
#225301=CARTESIAN_POINT('Ctrl Pts',(-7.89289316547287,0.536009048793502,
94.3379295905942));
#225302=CARTESIAN_POINT('Ctrl Pts',(-7.89511572941062,0.502210962620324,
94.339294478028));
#225303=CARTESIAN_POINT('Ctrl Pts',(-7.89858305094691,0.443752629603006,
94.341651150523));
#225304=CARTESIAN_POINT('Ctrl Pts',(-7.89992953729559,0.419098936628841,
94.342643778216));
#225305=CARTESIAN_POINT('Ctrl Pts',(-7.90229472965168,0.371720887862366,
94.3445489748828));
#225306=CARTESIAN_POINT('Ctrl Pts',(-7.90333088359629,0.348997650837556,
94.3454616860851));
#225307=CARTESIAN_POINT('Ctrl Pts',(-7.90554565331897,0.295342323872047,
94.3476143889633));
#225308=CARTESIAN_POINT('Ctrl Pts',(-7.90664075587045,0.264407130490534,
94.3488536244774));
#225309=CARTESIAN_POINT('Ctrl Pts',(-7.90985060311432,0.155688880748797,
94.3532022416483));
#225310=CARTESIAN_POINT('Ctrl Pts',(-7.91099931732731,0.0778814711349728,
94.3563026675399));
#225311=CARTESIAN_POINT('Ctrl Pts',(-7.91100311735682,-0.355436634977919,
94.3735104335096));
#225312=CARTESIAN_POINT('Ctrl Pts',(-7.88704271218661,-0.710543157949429,
94.3873734868895));
#225313=CARTESIAN_POINT('Ctrl Pts',(-7.80633970902302,-1.30579201857021,
94.4106411291279));
#225314=CARTESIAN_POINT('Ctrl Pts',(-7.76212394814162,-1.54708234257868,
94.4200865099885));
#225315=CARTESIAN_POINT('Ctrl Pts',(-7.64608724613857,-2.04781279598876,
94.4400198483939));
#225316=CARTESIAN_POINT('Ctrl Pts',(-7.57209172869083,-2.30642729521904,
94.4505075308377));
#225317=CARTESIAN_POINT('Ctrl Pts',(-7.47618419940208,-2.58676358543974,
94.4623626944828));
#225318=CARTESIAN_POINT('Ctrl Pts',(-7.46715436354632,-2.6127153937246,
94.4634649042376));
#225319=CARTESIAN_POINT('Ctrl Pts',(-7.45359948224675,-2.65102791368683,
94.4650995299478));
#225320=CARTESIAN_POINT('Ctrl Pts',(-7.44917846992508,-2.66342530637054,
94.4656296281301));
#225321=CARTESIAN_POINT('Ctrl Pts',(-7.44127971493652,-2.68540146918219,
94.4665714138426));
#225322=CARTESIAN_POINT('Ctrl Pts',(-7.43781436076781,-2.69498467169194,
94.4669828144461));
#225323=CARTESIAN_POINT('Ctrl Pts',(-7.43050825356696,-2.71506778792675,
94.4678464985998));
#225324=CARTESIAN_POINT('Ctrl Pts',(-7.42666374026287,-2.72556630582662,
94.4682988707544));
#225325=CARTESIAN_POINT('Ctrl Pts',(-7.41644416267689,-2.75329155437023,
94.4694959036888));
#225326=CARTESIAN_POINT('Ctrl Pts',(-7.41003138084584,-2.77050416561249,
94.4702415036757));
#225327=CARTESIAN_POINT('Ctrl Pts',(-7.3751378736,-2.86317434392187,94.4742689563162));
#225328=CARTESIAN_POINT('Ctrl Pts',(-7.34556475986508,-2.93821442608593,
94.477577251185));
#225329=CARTESIAN_POINT('Ctrl Pts',(-7.25214224166292,-3.16503810086119,
94.4877044270859));
#225330=CARTESIAN_POINT('Ctrl Pts',(-7.18469743902851,-3.31529099579833,
94.4945876254037));
#225331=CARTESIAN_POINT('Ctrl Pts',(-6.87751762639847,-3.94614434673074,
94.5240726357052));
#225332=CARTESIAN_POINT('Ctrl Pts',(-6.59385787640216,-4.40379155007968,
94.546841043515));
#225333=CARTESIAN_POINT('Ctrl Pts',(-6.17976896788432,-4.94108714641089,
94.5747346564772));
#225334=CARTESIAN_POINT('Ctrl Pts',(-6.09053017596727,-5.0506761822404,
94.5804999236285));
#225335=CARTESIAN_POINT('Ctrl Pts',(-5.97312099419522,-5.18721989677197,
94.587790126787));
#225336=CARTESIAN_POINT('Ctrl Pts',(-5.94762311156027,-5.21643594927226,
94.5893565008894));
#225337=CARTESIAN_POINT('Ctrl Pts',(-5.90685747058384,-5.2624586724597,
94.5918346563528));
#225338=CARTESIAN_POINT('Ctrl Pts',(-5.89173045790178,-5.27938904351281,
94.5927486278947));
#225339=CARTESIAN_POINT('Ctrl Pts',(-5.86326501852637,-5.31097325880319,
94.5944581533772));
#225340=CARTESIAN_POINT('Ctrl Pts',(-5.84994401770068,-5.32564255519518,
94.5952539716704));
#225341=CARTESIAN_POINT('Ctrl Pts',(-5.8197567849657,-5.35863529000138,
94.5970480695286));
#225342=CARTESIAN_POINT('Ctrl Pts',(-5.80285884728956,-5.37692945938086,
94.5980458452744));
#225343=CARTESIAN_POINT('Ctrl Pts',(-5.75228805457715,-5.43116272858518,
94.6010128568565));
#225344=CARTESIAN_POINT('Ctrl Pts',(-5.71836559191151,-5.46686760802811,
94.6029782021669));
#225345=CARTESIAN_POINT('Ctrl Pts',(-5.39471560465398,-5.80121474382613,
94.6215026173401));
#225346=CARTESIAN_POINT('Ctrl Pts',(-5.08217254270664,-6.07688957964575,
94.6377550941958));
#225347=CARTESIAN_POINT('Ctrl Pts',(-4.23646627352083,-6.71175391712623,
94.6786001540875));
#225348=CARTESIAN_POINT('Ctrl Pts',(-3.67861936862207,-7.03299680558552,
94.7023284389113));
#225349=CARTESIAN_POINT('Ctrl Pts',(-2.77958218484106,-7.41418633553808,
94.7390221070907));
#225350=CARTESIAN_POINT('Ctrl Pts',(-2.46304921729124,-7.52526423277672,
94.7517388038982));
#225351=CARTESIAN_POINT('Ctrl Pts',(-2.12178906712441,-7.62117496172933,
94.7658845745831));
#225352=CARTESIAN_POINT('Ctrl Pts',(-2.10311134444142,-7.62635032689576,
94.7666601978689));
#225353=CARTESIAN_POINT('Ctrl Pts',(-2.07550831575809,-7.63388966884469,
94.7678087275509));
#225354=CARTESIAN_POINT('Ctrl Pts',(-2.06659751991481,-7.63630676012746,
94.7681798436649));
#225355=CARTESIAN_POINT('Ctrl Pts',(-2.05139826970505,-7.64040106909934,
94.7688134796344));
#225356=CARTESIAN_POINT('Ctrl Pts',(-2.04511192876923,-7.64208613901881,
94.7690757288671));
#225357=CARTESIAN_POINT('Ctrl Pts',(-2.03292525048982,-7.64533669570523,
94.7695844836222));
#225358=CARTESIAN_POINT('Ctrl Pts',(-2.02702516587332,-7.64690311442734,
94.7698309563094));
#225359=CARTESIAN_POINT('Ctrl Pts',(-2.01298312185734,-7.65061375579703,
94.7704179528391));
#225360=CARTESIAN_POINT('Ctrl Pts',(-2.0048395495188,-7.65275181025254,
94.7707586950401));
#225361=CARTESIAN_POINT('Ctrl Pts',(-1.98066483169606,-7.65905752633964,
94.7717711876686));
#225362=CARTESIAN_POINT('Ctrl Pts',(-1.96462404742732,-7.66318782978493,
94.7724442869267));
#225363=CARTESIAN_POINT('Ctrl Pts',(-1.8322429071636,-7.69683136388682,
94.7780104482887));
#225364=CARTESIAN_POINT('Ctrl Pts',(-1.71526177069653,-7.72374287066485,
94.783003628501));
#225365=CARTESIAN_POINT('Ctrl Pts',(-1.50449684846218,-7.76720467731892,
94.7921740754335));
#225366=CARTESIAN_POINT('Ctrl Pts',(-1.41094638844822,-7.78474203441101,
94.7962995881021));
#225367=CARTESIAN_POINT('Ctrl Pts',(-1.12152431016233,-7.83361006070977,
94.8091888406299));
#225368=CARTESIAN_POINT('Ctrl Pts',(-0.924777211435029,-7.85926491513839,
94.8181265007611));
#225369=CARTESIAN_POINT('Ctrl Pts',(-0.216809522595592,-7.92462729157328,
94.8504963226563));
#225370=CARTESIAN_POINT('Ctrl Pts',(0.297075373271897,-7.92202815092615,
94.8742940643039));
#225371=CARTESIAN_POINT('Ctrl Pts',(0.958710551606543,-7.85417227414245,
94.9036474528743));
#225372=CARTESIAN_POINT('Ctrl Pts',(1.10984289361545,-7.83424532252421,
94.9102722219331));
#225373=CARTESIAN_POINT('Ctrl Pts',(1.44977810268847,-7.7793892637523,94.9249635234814));
#225374=CARTESIAN_POINT('Ctrl Pts',(1.63807784143411,-7.74192879736747,
94.9329529040568));
#225375=CARTESIAN_POINT('Ctrl Pts',(1.84399165277139,-7.69311401633058,
94.9415246932727));
#225376=CARTESIAN_POINT('Ctrl Pts',(1.86312847499661,-7.68850185514843,
94.9423197590846));
#225377=CARTESIAN_POINT('Ctrl Pts',(1.89160629556575,-7.68152585467548,
94.943500604155));
#225378=CARTESIAN_POINT('Ctrl Pts',(1.90096044233482,-7.67921631619811,
94.9438881067535));
#225379=CARTESIAN_POINT('Ctrl Pts',(1.91700688133529,-7.67522333466126,
94.9445522091324));
#225380=CARTESIAN_POINT('Ctrl Pts',(1.92370122323677,-7.67354821605128,
94.9448290736016));
#225381=CARTESIAN_POINT('Ctrl Pts',(1.9374599780665,-7.67008624018572,94.9453977201063));
#225382=CARTESIAN_POINT('Ctrl Pts',(1.94452413267082,-7.66829837684532,
94.9456894697582));
#225383=CARTESIAN_POINT('Ctrl Pts',(1.9608706308643,-7.66413720930678,94.9463640955198));
#225384=CARTESIAN_POINT('Ctrl Pts',(1.97015116195069,-7.66175679553687,
94.9467467441555));
#225385=CARTESIAN_POINT('Ctrl Pts',(1.99934901109399,-7.65421112262899,
94.9479494778538));
#225386=CARTESIAN_POINT('Ctrl Pts',(2.01925058736795,-7.64898499485241,
94.9487676140312));
#225387=CARTESIAN_POINT('Ctrl Pts',(2.30869676470766,-7.57176842344998,
94.9606426991289));
#225388=CARTESIAN_POINT('Ctrl Pts',(2.57428032063671,-7.4856433525196,94.9712280419606));
#225389=CARTESIAN_POINT('Ctrl Pts',(3.21352206506899,-7.2402885659004,94.9962627482606));
#225390=CARTESIAN_POINT('Ctrl Pts',(3.58053712545472,-7.06599450743142,
95.0102271887046));
#225391=CARTESIAN_POINT('Ctrl Pts',(4.41893686528471,-6.58567451776689,
95.0431336541905));
#225392=CARTESIAN_POINT('Ctrl Pts',(4.87426402384145,-6.25616014019791,
95.0618305689935));
#225393=CARTESIAN_POINT('Ctrl Pts',(5.35104459947213,-5.82724526231747,
95.08633975079));
#225394=CARTESIAN_POINT('Ctrl Pts',(5.41035288108064,-5.77222197901689,
95.0894881776148));
#225395=CARTESIAN_POINT('Ctrl Pts',(5.48611496764926,-5.69974012036319,
95.0936558851752));
#225396=CARTESIAN_POINT('Ctrl Pts',(5.50334933894179,-5.68310134596841,
95.0946139666527));
#225397=CARTESIAN_POINT('Ctrl Pts',(5.52575107594743,-5.66127632564756,
95.095872823852));
#225398=CARTESIAN_POINT('Ctrl Pts',(5.53098734425356,-5.6561606753786,95.096168044941));
#225399=CARTESIAN_POINT('Ctrl Pts',(5.53903902473622,-5.64827259393717,
95.0966235092425));
#225400=CARTESIAN_POINT('Ctrl Pts',(5.54185948439862,-5.64550529784895,
95.096783342029));
#225401=CARTESIAN_POINT('Ctrl Pts',(5.5474592636113,-5.64000283017586,95.0971012478024));
#225402=CARTESIAN_POINT('Ctrl Pts',(5.55023863677766,-5.63726771410929,
95.0972593163278));
#225403=CARTESIAN_POINT('Ctrl Pts',(5.55627699482406,-5.63131671278909,
95.0976033426708));
#225404=CARTESIAN_POINT('Ctrl Pts',(5.55953521057789,-5.6281000528706,95.0977893634665));
#225405=CARTESIAN_POINT('Ctrl Pts',(5.56880115835381,-5.61893638677033,
95.0983194964332));
#225406=CARTESIAN_POINT('Ctrl Pts',(5.57480214986017,-5.61298258054092,
95.0986641664747));
#225407=CARTESIAN_POINT('Ctrl Pts',(5.58820827309988,-5.59963916146452,
95.0994371741608));
#225408=CARTESIAN_POINT('Ctrl Pts',(5.59560828128917,-5.5922444870057,95.0998659320829));
#225409=CARTESIAN_POINT('Ctrl Pts',(5.85206507970058,-5.33495385228391,
95.1147962010079));
#225410=CARTESIAN_POINT('Ctrl Pts',(6.08411935213516,-5.06871205931401,
95.1306248953303));
#225411=CARTESIAN_POINT('Ctrl Pts',(6.50607578164984,-4.51370618108745,
95.1626837849411));
#225412=CARTESIAN_POINT('Ctrl Pts',(6.69641278960825,-4.22618337785823,
95.1788572399632));
#225413=CARTESIAN_POINT('Ctrl Pts',(7.04744980020009,-3.61232779564468,
95.2114213267389));
#225414=CARTESIAN_POINT('Ctrl Pts',(7.20564149441936,-3.28545788860019,
95.2277342273834));
#225415=CARTESIAN_POINT('Ctrl Pts',(7.4130606911038,-2.76911087488665,95.2515525030292));
#225416=CARTESIAN_POINT('Ctrl Pts',(7.47864302004084,-2.58676438374428,
95.2596181596478));
#225417=CARTESIAN_POINT('Ctrl Pts',(7.54310995074024,-2.38448284201722,
95.2681944841267));
#225418=CARTESIAN_POINT('Ctrl Pts',(7.54868892372849,-2.36676185794345,
95.2689427651741));
#225419=CARTESIAN_POINT('Ctrl Pts',(7.55686865789422,-2.34045669315049,
95.2700490237938));
#225420=CARTESIAN_POINT('Ctrl Pts',(7.55951730761193,-2.33188754484616,
95.2704086918688));
#225421=CARTESIAN_POINT('Ctrl Pts',(7.56402122153669,-2.31722776122552,
95.2710227962964));
#225422=CARTESIAN_POINT('Ctrl Pts',(7.56588371364676,-2.31113936600717,
95.2712774875131));
#225423=CARTESIAN_POINT('Ctrl Pts',(7.56948837565898,-2.29930484791211,
95.2717718655606));
#225424=CARTESIAN_POINT('Ctrl Pts',(7.57123135756137,-2.29355897752457,
95.2720115809091));
#225425=CARTESIAN_POINT('Ctrl Pts',(7.57537731951149,-2.27983527626451,
95.2725833802332));
#225426=CARTESIAN_POINT('Ctrl Pts',(7.57777424349534,-2.27185561492547,
95.2729152506915));
#225427=CARTESIAN_POINT('Ctrl Pts',(7.58489601311404,-2.24800968237248,
95.2739051981634));
#225428=CARTESIAN_POINT('Ctrl Pts',(7.5895836808108,-2.23213230305818,95.2745619665853));
#225429=CARTESIAN_POINT('Ctrl Pts',(7.62874939616838,-2.09792613284254,
95.280093557864));
#225430=CARTESIAN_POINT('Ctrl Pts',(7.66050858339328,-1.97881819764149,
95.2848722477829));
#225431=CARTESIAN_POINT('Ctrl Pts',(7.73246221433118,-1.6811949463027,95.2965155270619));
#225432=CARTESIAN_POINT('Ctrl Pts',(7.76927205767993,-1.50193374837558,
95.3032649610828));
#225433=CARTESIAN_POINT('Ctrl Pts',(7.90916911912388,-0.676256499060295,
95.3333998599116));
#225434=CARTESIAN_POINT('Ctrl Pts',(7.93799782165575,-0.0199530447597436,
95.35445016023));
#225435=CARTESIAN_POINT('Ctrl Pts',(7.86609003060477,0.876713959469128,
95.3857692659853));
#225436=CARTESIAN_POINT('Ctrl Pts',(7.83515312778967,1.11998208707394,95.3945629168146));
#225437=CARTESIAN_POINT('Ctrl Pts',(7.77770596322982,1.44882231462876,95.4073232137154));
#225438=CARTESIAN_POINT('Ctrl Pts',(7.76096504677763,1.53597413628007,95.4107900543444));
#225439=CARTESIAN_POINT('Ctrl Pts',(7.74076314876747,1.63236082039198,95.4147377530691));
#225440=CARTESIAN_POINT('Ctrl Pts',(7.73874640772947,1.64189524891376,95.4151294915976));
#225441=CARTESIAN_POINT('Ctrl Pts',(7.73570555030763,1.65614126415098,95.4157166988722));
#225442=CARTESIAN_POINT('Ctrl Pts',(7.73469472965689,1.66085570923426,95.4159113329517));
#225443=CARTESIAN_POINT('Ctrl Pts',(7.732940005443,1.66900335900794,95.4162482430516));
#225444=CARTESIAN_POINT('Ctrl Pts',(7.73219812821894,1.67243697819914,95.4163903899198));
#225445=CARTESIAN_POINT('Ctrl Pts',(7.73065352581933,1.6795628421741,95.416685730574));
#225446=CARTESIAN_POINT('Ctrl Pts',(7.729850442098,1.68325500735021,95.416838946791));
#225447=CARTESIAN_POINT('Ctrl Pts',(7.72796030958165,1.69191498439407,95.4171987581437));
#225448=CARTESIAN_POINT('Ctrl Pts',(7.72687111636236,1.69688232113088,95.4174054866333));
#225449=CARTESIAN_POINT('Ctrl Pts',(7.72337576336947,1.71274995962605,95.4180669434725));
#225450=CARTESIAN_POINT('Ctrl Pts',(7.72095133152585,1.72364617600235,95.418522797581));
#225451=CARTESIAN_POINT('Ctrl Pts',(7.69187126317123,1.85304935276744,95.4239556366843));
#225452=CARTESIAN_POINT('Ctrl Pts',(7.66251399609224,1.97092661600016,95.4290951999472));
#225453=CARTESIAN_POINT('Ctrl Pts',(7.56786631338446,2.31679779787797,95.4446424938688));
#225454=CARTESIAN_POINT('Ctrl Pts',(7.49502762631491,2.54257733094657,95.4553958813207));
#225455=CARTESIAN_POINT('Ctrl Pts',(7.32665523349672,2.99397923415774,95.4776744496272));
#225456=CARTESIAN_POINT('Ctrl Pts',(7.23055683625024,3.21913545343965,95.4892004382441));
#225457=CARTESIAN_POINT('Ctrl Pts',(6.81303711039458,4.08394425872501,95.5343272624876));
#225458=CARTESIAN_POINT('Ctrl Pts',(6.41582353996539,4.68333817199578,95.5671125421243));
#225459=CARTESIAN_POINT('Ctrl Pts',(5.91053559431507,5.25851300232902,95.5984569785344));
#225460=CARTESIAN_POINT('Ctrl Pts',(5.87738989983026,5.2955337875968,95.6004760232698));
#225461=CARTESIAN_POINT('Ctrl Pts',(5.83473235205424,5.34228455448099,95.6030282523511));
#225462=CARTESIAN_POINT('Ctrl Pts',(5.82554160637273,5.35230519272411,95.6035754521454));
#225463=CARTESIAN_POINT('Ctrl Pts',(5.81091323789715,5.36817213642894,95.6044421579996));
#225464=CARTESIAN_POINT('Ctrl Pts',(5.80549254166501,5.37403396843314,95.6047624065745));
#225465=CARTESIAN_POINT('Ctrl Pts',(5.79537552501334,5.38494113565621,95.6053584037892));
#225466=CARTESIAN_POINT('Ctrl Pts',(5.7906814694577,5.38998855564706,95.6056342516189));
#225467=CARTESIAN_POINT('Ctrl Pts',(5.78025521409997,5.40117034985979,95.6062454495056));
#225468=CARTESIAN_POINT('Ctrl Pts',(5.77451982980509,5.40730175079031,95.6065806586117));
#225469=CARTESIAN_POINT('Ctrl Pts',(5.75792796806482,5.42498274373831,95.6075474930593));
#225470=CARTESIAN_POINT('Ctrl Pts',(5.7470464959024,5.43650888282897,95.6081780127852));
#225471=CARTESIAN_POINT('Ctrl Pts',(5.6732680102981,5.51418928621705,95.6124291917285));
#225472=CARTESIAN_POINT('Ctrl Pts',(5.60926353845871,5.57928460152488,95.616000333285));
#225473=CARTESIAN_POINT('Ctrl Pts',(5.44522127844096,5.74044575411594,95.6248750262381));
#225474=CARTESIAN_POINT('Ctrl Pts',(5.34375640511205,5.83501687186271,95.6301135421232));
#225475=CARTESIAN_POINT('Ctrl Pts',(4.90281728975392,6.22484406412965,95.6519330883453));
#225476=CARTESIAN_POINT('Ctrl Pts',(4.54096662598676,6.49353117907175,95.6674937695733));
#225477=CARTESIAN_POINT('Ctrl Pts',(3.70167429740342,7.01210047603634,95.7015242947141));
#225478=CARTESIAN_POINT('Ctrl Pts',(3.21760062047393,7.24699701786401,95.719916291599));
#225479=CARTESIAN_POINT('Ctrl Pts',(2.66829779604019,7.447578384699,95.7429223354167));
#225480=CARTESIAN_POINT('Ctrl Pts',(2.62294424126368,7.46367203787041,95.7448352532185));
#225481=CARTESIAN_POINT('Ctrl Pts',(2.56700911476872,7.48294775483598,95.7472088739514));
#225482=CARTESIAN_POINT('Ctrl Pts',(2.55656335280786,7.48652300593243,95.7476527569251));
#225483=CARTESIAN_POINT('Ctrl Pts',(2.53925312566767,7.49240729112723,95.7483893232753));
#225484=CARTESIAN_POINT('Ctrl Pts',(2.53239289249868,7.49472879362012,95.7486814882004));
#225485=CARTESIAN_POINT('Ctrl Pts',(2.51997925428017,7.49891057814395,95.7492106146666));
#225486=CARTESIAN_POINT('Ctrl Pts',(2.51442694755972,7.50077412179241,95.7494474429402));
#225487=CARTESIAN_POINT('Ctrl Pts',(2.50265970287279,7.50470907683185,95.7499497032018));
#225488=CARTESIAN_POINT('Ctrl Pts',(2.49644425315105,7.50677893685754,95.7502151973066));
#225489=CARTESIAN_POINT('Ctrl Pts',(2.47975030991459,7.51231530329536,95.7509288097155));
#225490=CARTESIAN_POINT('Ctrl Pts',(2.46926714210567,7.51576759852443,95.7513774888817));
#225491=CARTESIAN_POINT('Ctrl Pts',(2.44608346967278,7.52334865661364,95.752370937552));
#225492=CARTESIAN_POINT('Ctrl Pts',(2.43337967885803,7.52746721583356,95.7529160972669));
#225493=CARTESIAN_POINT('Ctrl Pts',(2.39519647830983,7.53973941943001,95.7545569176983));
#225494=CARTESIAN_POINT('Ctrl Pts',(2.36968620922721,7.54779596518536,95.755656168534));
#225495=CARTESIAN_POINT('Ctrl Pts',(2.27801783385412,7.57623574767693,95.7596160423244));
#225496=CARTESIAN_POINT('Ctrl Pts',(2.2116345583565,7.59587951614912,95.7625019661246));
#225497=CARTESIAN_POINT('Ctrl Pts',(2.0031047593703,7.65462116887048,95.7716105123528));
#225498=CARTESIAN_POINT('Ctrl Pts',(1.86012000677474,7.69061800946029,95.7779177269329));
#225499=CARTESIAN_POINT('Ctrl Pts',(0.98918698741493,7.88416816158806,95.8164681990765));
#225500=CARTESIAN_POINT('Ctrl Pts',(0.242874917137029,7.94227882690981,
95.849633988647));
#225501=CARTESIAN_POINT('Ctrl Pts',(-0.689331782249625,7.88318051767555,
95.8885771653028));
#225502=CARTESIAN_POINT('Ctrl Pts',(-0.877655499756,7.86444135706684,95.8963434571706));
#225503=CARTESIAN_POINT('Ctrl Pts',(-1.09866423585044,7.83441147262645,
95.9053637810009));
#225504=CARTESIAN_POINT('Ctrl Pts',(-1.13216793682291,7.82963996693112,
95.9067287465753));
#225505=CARTESIAN_POINT('Ctrl Pts',(-1.18187290458387,7.82223540871206,
95.9087500877257));
#225506=CARTESIAN_POINT('Ctrl Pts',(-1.1980981871931,7.81976669013278,95.9094093326295));
#225507=CARTESIAN_POINT('Ctrl Pts',(-1.22695426435346,7.81528424439515,
95.9105807288982));
#225508=CARTESIAN_POINT('Ctrl Pts',(-1.23958806478099,7.81329034519343,
95.9110932334639));
#225509=CARTESIAN_POINT('Ctrl Pts',(-1.26616243628537,7.80903023160124,
95.9121704992509));
#225510=CARTESIAN_POINT('Ctrl Pts',(-1.28010189121267,7.80675730523104,
95.912735136582));
#225511=CARTESIAN_POINT('Ctrl Pts',(-1.316836423216,7.8006664473461,95.914221967605));
#225512=CARTESIAN_POINT('Ctrl Pts',(-1.33962102861553,7.79678592080007,
95.9151430028793));
#225513=CARTESIAN_POINT('Ctrl Pts',(-1.4429283725739,7.77872506674225,95.9193137546079));
#225514=CARTESIAN_POINT('Ctrl Pts',(-1.52324609814851,7.76339665254577,
95.9225416556768));
#225515=CARTESIAN_POINT('Ctrl Pts',(-2.33714390950144,7.5949492440655,95.9551103551461));
#225516=CARTESIAN_POINT('Ctrl Pts',(-3.04562407628151,7.33959384271519,
95.9817422378083));
#225517=CARTESIAN_POINT('Ctrl Pts',(-3.91841477401823,6.87654728846172,
96.0180338644231));
#225518=CARTESIAN_POINT('Ctrl Pts',(-4.12405948538945,6.75522027622282,
96.0269218884242));
#225519=CARTESIAN_POINT('Ctrl Pts',(-4.39741303990627,6.57680672757507,
96.0395758928123));
#225520=CARTESIAN_POINT('Ctrl Pts',(-4.47012455291757,6.52760399294634,
96.0430277776526));
#225521=CARTESIAN_POINT('Ctrl Pts',(-4.55318250199247,6.46936137748287,
96.04708833144));
#225522=CARTESIAN_POINT('Ctrl Pts',(-4.56434437741481,6.46149115374658,
96.0476365060947));
#225523=CARTESIAN_POINT('Ctrl Pts',(-4.58088542161116,6.44976383799779,
96.0484526478827));
#225524=CARTESIAN_POINT('Ctrl Pts',(-4.58628025824946,6.4459288085019,96.0487194318479));
#225525=CARTESIAN_POINT('Ctrl Pts',(-4.59586426734274,6.43909769780573,
96.0491944579694));
#225526=CARTESIAN_POINT('Ctrl Pts',(-4.60005534367424,6.43610428447769,
96.0494025545518));
#225527=CARTESIAN_POINT('Ctrl Pts',(-4.60813230933346,6.43032351357419,
96.049804310977));
#225528=CARTESIAN_POINT('Ctrl Pts',(-4.61201860126713,6.42753672031224,
96.0499979396032));
#225529=CARTESIAN_POINT('Ctrl Pts',(-4.62256652427517,6.41995849393949,
96.0505243517563));
#225530=CARTESIAN_POINT('Ctrl Pts',(-4.62922321833875,6.41516022631306,
96.0508575177392));
#225531=CARTESIAN_POINT('Ctrl Pts',(-4.65427118332568,6.39704590486054,
96.0521148008158));
#225532=CARTESIAN_POINT('Ctrl Pts',(-4.67261242905173,6.3836611460421,96.0530428430758));
#225533=CARTESIAN_POINT('Ctrl Pts',(-4.71759747003296,6.35053499488541,
96.0553379511365));
#225534=CARTESIAN_POINT('Ctrl Pts',(-4.74417440436931,6.33070531036108,
96.0567105544983));
#225535=CARTESIAN_POINT('Ctrl Pts',(-4.85037850963349,6.25041956142837,
96.0622615662839));
#225536=CARTESIAN_POINT('Ctrl Pts',(-4.92897869434102,6.18862537689729,
96.0665190586318));
#225537=CARTESIAN_POINT('Ctrl Pts',(-5.11825236490796,6.03392808609395,
96.0771026902919));
#225538=CARTESIAN_POINT('Ctrl Pts',(-5.22759112484819,5.93945144247613,
96.0835038000803));
#225539=CARTESIAN_POINT('Ctrl Pts',(-6.0600908488128,5.17930836899359,96.1341780073597));
#225540=CARTESIAN_POINT('Ctrl Pts',(-6.65631139006487,4.38683471995058,
96.1809947286347));
#225541=CARTESIAN_POINT('Ctrl Pts',(-7.11576627382732,3.45726284832877,
96.2235291415259));
#225542=CARTESIAN_POINT('Ctrl Pts',(-7.13903588058207,3.40895334438121,
96.2257123214576));
#225543=CARTESIAN_POINT('Ctrl Pts',(-7.16806676225463,3.34708181172404,
96.228474194963));
#225544=CARTESIAN_POINT('Ctrl Pts',(-7.17428349305476,3.3337357613821,96.2290679352078));
#225545=CARTESIAN_POINT('Ctrl Pts',(-7.18409674531395,3.31251413740988,
96.2300088686513));
#225546=CARTESIAN_POINT('Ctrl Pts',(-7.18771764363688,3.30464991073399,
96.2303568654387));
#225547=CARTESIAN_POINT('Ctrl Pts',(-7.19444385795732,3.28997789705409,
96.2310048281613));
#225548=CARTESIAN_POINT('Ctrl Pts',(-7.19755243751562,3.28317162177041,
96.2313049013309));
#225549=CARTESIAN_POINT('Ctrl Pts',(-7.20443032676624,3.26805567954645,
96.2319701927862));
#225550=CARTESIAN_POINT('Ctrl Pts',(-7.20819492832488,3.25974387549168,
96.2323352560016));
#225551=CARTESIAN_POINT('Ctrl Pts',(-7.21903890337987,3.23569099411405,
96.2333894939135));
#225552=CARTESIAN_POINT('Ctrl Pts',(-7.22608117307899,3.21993319536517,
96.2340774503846));
#225553=CARTESIAN_POINT('Ctrl Pts',(-7.2737145924873,3.11240524405664,96.2387536291785));
#225554=CARTESIAN_POINT('Ctrl Pts',(-7.31260884192761,3.01989125318424,
96.2426861106858));
#225555=CARTESIAN_POINT('Ctrl Pts',(-7.40471796364719,2.78857725201936,
96.2523073539752));
#225556=CARTESIAN_POINT('Ctrl Pts',(-7.45580166083015,2.64896873229796,
96.2579285248489));
#225557=CARTESIAN_POINT('Ctrl Pts',(-7.77324781735989,1.69929785443723,
96.2950870966343));
#225558=CARTESIAN_POINT('Ctrl Pts',(-7.91101614490582,0.852346899750275,
96.3224167912368));
#225559=CARTESIAN_POINT('Ctrl Pts',(-7.91099999858106,-0.000149834679674665,
96.3535680629415));
#225560=CARTESIAN_POINT('',(-7.91099998983997,0.000400938813840742,100.360997295013));
#225561=CARTESIAN_POINT('Ctrl Pts',(-7.91099999844005,-0.00015710359732031,
96.3535683285568));
#225562=CARTESIAN_POINT('Ctrl Pts',(-7.91099547183649,-0.228095618794251,
96.3618974865411));
#225563=CARTESIAN_POINT('Ctrl Pts',(-7.90114013362385,-0.455922551071472,
96.3705375672487));
#225564=CARTESIAN_POINT('Ctrl Pts',(-7.88039505359977,-0.695303428629795,
96.3801233621209));
#225565=CARTESIAN_POINT('Ctrl Pts',(-7.87930168561817,-0.707586039626178,
96.3806164462078));
#225566=CARTESIAN_POINT('Ctrl Pts',(-7.87746571638615,-0.727678800481275,
96.3814250427537));
#225567=CARTESIAN_POINT('Ctrl Pts',(-7.87674020433675,-0.735490518183862,
96.3817398997601));
#225568=CARTESIAN_POINT('Ctrl Pts',(-7.87543924029822,-0.749275505734465,
96.3822963623341));
#225569=CARTESIAN_POINT('Ctrl Pts',(-7.87486860897096,-0.755249231924752,
96.3825377868069));
#225570=CARTESIAN_POINT('Ctrl Pts',(-7.87373569209671,-0.766968433314642,
96.3830119562606));
#225571=CARTESIAN_POINT('Ctrl Pts',(-7.87317391339796,-0.772713954763641,
96.383244682401));
#225572=CARTESIAN_POINT('Ctrl Pts',(-7.87204253423117,-0.784155667159567,
96.3837086425232));
#225573=CARTESIAN_POINT('Ctrl Pts',(-7.87147303891542,-0.78985186490412,
96.3839398725461));
#225574=CARTESIAN_POINT('Ctrl Pts',(-7.87011571281016,-0.803280824711324,
96.3844855864139));
#225575=CARTESIAN_POINT('Ctrl Pts',(-7.86932266800957,-0.811013047129047,
96.3848002565994));
#225576=CARTESIAN_POINT('Ctrl Pts',(-7.86653541309912,-0.837799886668064,
96.3858919238506));
#225577=CARTESIAN_POINT('Ctrl Pts',(-7.86448338847706,-0.856848341698109,
96.386670942257));
#225578=CARTESIAN_POINT('Ctrl Pts',(-7.83475236111732,-1.12372701046691,
96.3976219756003));
#225579=CARTESIAN_POINT('Ctrl Pts',(-7.79544028618084,-1.37011243253586,
96.4081684378632));
#225580=CARTESIAN_POINT('Ctrl Pts',(-7.73511039132125,-1.65955815149987,
96.4208333911937));
#225581=CARTESIAN_POINT('Ctrl Pts',(-7.72526211798902,-1.70481412506614,
96.4228218998646));
#225582=CARTESIAN_POINT('Ctrl Pts',(-7.60948566179,-2.21522962116972,96.4453313650302));
#225583=CARTESIAN_POINT('Ctrl Pts',(-7.4620800375311,-2.67000066021761,
96.466063583998));
#225584=CARTESIAN_POINT('Ctrl Pts',(-7.18922794257249,-3.30849225958182,
96.4954635245194));
#225585=CARTESIAN_POINT('Ctrl Pts',(-7.09566192538619,-3.50466901269359,
96.5045560704901));
#225586=CARTESIAN_POINT('Ctrl Pts',(-6.86170768879972,-3.94730332843422,
96.5252939947216));
#225587=CARTESIAN_POINT('Ctrl Pts',(-6.71590782422891,-4.1905634285916,
96.5368689893605));
#225588=CARTESIAN_POINT('Ctrl Pts',(-6.51808292967413,-4.48368684803633,
96.5512449244125));
#225589=CARTESIAN_POINT('Ctrl Pts',(-6.47802388354467,-4.54137198063387,
96.5540939215078));
#225590=CARTESIAN_POINT('Ctrl Pts',(-6.41445166012157,-4.63036312796215,
96.5585199920225));
#225591=CARTESIAN_POINT('Ctrl Pts',(-6.39146529786671,-4.66204077172549,
96.5601017423418));
#225592=CARTESIAN_POINT('Ctrl Pts',(-6.34766617888135,-4.72146779638247,
96.5630809182373));
#225593=CARTESIAN_POINT('Ctrl Pts',(-6.32690415212631,-4.74925340775851,
96.5644788079145));
#225594=CARTESIAN_POINT('Ctrl Pts',(-6.29096333772848,-4.79669866743941,
96.5668743535523));
#225595=CARTESIAN_POINT('Ctrl Pts',(-6.27587348959498,-4.81642499884057,
96.567872927643));
#225596=CARTESIAN_POINT('Ctrl Pts',(-6.24688921792902,-4.85394744862527,
96.5697773344805));
#225597=CARTESIAN_POINT('Ctrl Pts',(-6.23301101594554,-4.87175578341792,
96.5706833338061));
#225598=CARTESIAN_POINT('Ctrl Pts',(-6.20034979039231,-4.91329823738387,
96.5728019138365));
#225599=CARTESIAN_POINT('Ctrl Pts',(-6.18150639828315,-4.9369844792358,
96.5740137976861));
#225600=CARTESIAN_POINT('Ctrl Pts',(-6.11628491889484,-5.01800940274258,
96.5781731102492));
#225601=CARTESIAN_POINT('Ctrl Pts',(-6.06924108375768,-5.07480761734321,
96.5811126083227));
#225602=CARTESIAN_POINT('Ctrl Pts',(-5.65920630471633,-5.55600353761578,
96.6062314527234));
#225603=CARTESIAN_POINT('Ctrl Pts',(-5.2530112736366,-5.94152149207426,
96.6277014713144));
#225604=CARTESIAN_POINT('Ctrl Pts',(-4.56065890113762,-6.47167888016717,
96.6614498985478));
#225605=CARTESIAN_POINT('Ctrl Pts',(-4.30060140213634,-6.64733434620611,
96.6736265400546));
#225606=CARTESIAN_POINT('Ctrl Pts',(-4.00499732372843,-6.82237625595014,
96.687362812733));
#225607=CARTESIAN_POINT('Ctrl Pts',(-3.97909202315596,-6.83751767790462,
96.6885658181687));
#225608=CARTESIAN_POINT('Ctrl Pts',(-3.9412842054516,-6.85932838761716,
96.6903209848783));
#225609=CARTESIAN_POINT('Ctrl Pts',(-3.92944949403805,-6.86611489777649,
96.6908703108593));
#225610=CARTESIAN_POINT('Ctrl Pts',(-3.90915122132476,-6.87768509334585,
96.6918124080321));
#225611=CARTESIAN_POINT('Ctrl Pts',(-3.90069627544968,-6.88248385980615,
96.692204801681));
#225612=CARTESIAN_POINT('Ctrl Pts',(-3.8830351214881,-6.89246478802746,
96.6930244342126));
#225613=CARTESIAN_POINT('Ctrl Pts',(-3.87382733794453,-6.89764411693488,
96.6934517444074));
#225614=CARTESIAN_POINT('Ctrl Pts',(-3.85081599766598,-6.91052726200476,
96.6945196557035));
#225615=CARTESIAN_POINT('Ctrl Pts',(-3.83699974948331,-6.91820813563104,
96.6951608588306));
#225616=CARTESIAN_POINT('Ctrl Pts',(-3.78089754683806,-6.94917730202297,
96.697764732388));
#225617=CARTESIAN_POINT('Ctrl Pts',(-3.73842224834018,-6.97211950939762,
96.6997364715091));
#225618=CARTESIAN_POINT('Ctrl Pts',(-3.51234379191757,-7.09157146814619,
96.7102265755632));
#225619=CARTESIAN_POINT('Ctrl Pts',(-3.32521091544579,-7.18121951894139,
96.7188915217075));
#225620=CARTESIAN_POINT('Ctrl Pts',(-2.64361144581839,-7.47538744184029,
96.7500979745021));
#225621=CARTESIAN_POINT('Ctrl Pts',(-2.13218791315477,-7.63700932828069,
96.7727691426322));
#225622=CARTESIAN_POINT('Ctrl Pts',(-1.47092733809158,-7.7743166077336,
96.8005288181542));
#225623=CARTESIAN_POINT('Ctrl Pts',(-1.33274788861426,-7.79919290916647,
96.8062541329836));
#225624=CARTESIAN_POINT('Ctrl Pts',(-1.15717629169226,-7.82599833650151,
96.8134417973244));
#225625=CARTESIAN_POINT('Ctrl Pts',(-1.12033529402086,-7.83135721192357,
96.8149452405692));
#225626=CARTESIAN_POINT('Ctrl Pts',(-1.06130560157301,-7.83951857683851,
96.8173468536801));
#225627=CARTESIAN_POINT('Ctrl Pts',(-1.03914055450353,-7.84248736106824,
96.8182469852547));
#225628=CARTESIAN_POINT('Ctrl Pts',(-0.997068678588804,-7.84794097146024,
96.819952503946));
#225629=CARTESIAN_POINT('Ctrl Pts',(-0.97716441225162,-7.85044413747507,
96.8207580997162));
#225630=CARTESIAN_POINT('Ctrl Pts',(-0.931889584993449,-7.85596305682155,
96.8225876899034));
#225631=CARTESIAN_POINT('Ctrl Pts',(-0.906513483038265,-7.85893167418894,
96.8236111310436));
#225632=CARTESIAN_POINT('Ctrl Pts',(-0.840598223579007,-7.86631925011927,
96.8262645106965));
#225633=CARTESIAN_POINT('Ctrl Pts',(-0.800038411933684,-7.87054778780272,
96.8278922743001));
#225634=CARTESIAN_POINT('Ctrl Pts',(-0.482186699644027,-7.90120279613035,
96.8406126490297));
#225635=CARTESIAN_POINT('Ctrl Pts',(-0.203703911787188,-7.91328111759463,
96.8515425985047));
#225636=CARTESIAN_POINT('Ctrl Pts',(0.0802563238618417,-7.91059474928651,
96.8626264199348));
#225637=CARTESIAN_POINT('Ctrl Pts',(0.0856749730396105,-7.91053791875003,
96.8628378950546));
#225638=CARTESIAN_POINT('Ctrl Pts',(0.565725856991825,-7.9050098636676,
96.8815701937917));
#225639=CARTESIAN_POINT('Ctrl Pts',(1.03891298264263,-7.85683847286887,
96.8997059611012));
#225640=CARTESIAN_POINT('Ctrl Pts',(1.75788659866591,-7.71752182985089,
96.9272290993342));
#225641=CARTESIAN_POINT('Ctrl Pts',(2.00829301566487,-7.65617839568246,
96.9368273188885));
#225642=CARTESIAN_POINT('Ctrl Pts',(2.52484080425947,-7.50254643520879,
96.9570210189468));
#225643=CARTESIAN_POINT('Ctrl Pts',(2.78994749304644,-7.40805017928735,
96.9676124107701));
#225644=CARTESIAN_POINT('Ctrl Pts',(3.11674604150809,-7.27152902189387,
96.9813816425818));
#225645=CARTESIAN_POINT('Ctrl Pts',(3.18364980349044,-7.24248671621858,
96.9842399746396));
#225646=CARTESIAN_POINT('Ctrl Pts',(3.27627426072687,-7.20074784790378,
96.9882619893091));
#225647=CARTESIAN_POINT('Ctrl Pts',(3.30234271919194,-7.18882988701723,
96.9894011909934));
#225648=CARTESIAN_POINT('Ctrl Pts',(3.34155051976329,-7.17064662322809,
96.9911261755855));
#225649=CARTESIAN_POINT('Ctrl Pts',(3.35473840699098,-7.16448624041209,
96.9917083763873));
#225650=CARTESIAN_POINT('Ctrl Pts',(3.37889544993873,-7.15312057459422,
96.9927785829963));
#225651=CARTESIAN_POINT('Ctrl Pts',(3.38986978188682,-7.14792636198583,
96.9932661946));
#225652=CARTESIAN_POINT('Ctrl Pts',(3.40751194197308,-7.13952646197214,
96.9940524228808));
#225653=CARTESIAN_POINT('Ctrl Pts',(3.41418732725791,-7.13633663933164,
96.9943504566522));
#225654=CARTESIAN_POINT('Ctrl Pts',(3.42694654637268,-7.13021766577263,
96.994921167605));
#225655=CARTESIAN_POINT('Ctrl Pts',(3.43303112599411,-7.12729007973062,
96.9951937860206));
#225656=CARTESIAN_POINT('Ctrl Pts',(3.44679812100053,-7.1206443919729,96.995811667542));
#225657=CARTESIAN_POINT('Ctrl Pts',(3.45447827593597,-7.11692164382133,
96.9961571076197));
#225658=CARTESIAN_POINT('Ctrl Pts',(3.47705071774455,-7.10593511434129,
96.9971746025724));
#225659=CARTESIAN_POINT('Ctrl Pts',(3.49192617570184,-7.09863699039693,
96.9978479955809));
#225660=CARTESIAN_POINT('Ctrl Pts',(3.5889593463041,-7.05065224678577,97.0022598064176));
#225661=CARTESIAN_POINT('Ctrl Pts',(3.67042600644359,-7.00858749078639,
97.006054171164));
#225662=CARTESIAN_POINT('Ctrl Pts',(4.27538044189192,-6.68278252195722,
97.035025511134));
#225663=CARTESIAN_POINT('Ctrl Pts',(4.7660444399419,-6.34217841030185,97.0628742895321));
#225664=CARTESIAN_POINT('Ctrl Pts',(5.36669744536995,-5.81582268587094,
97.0993099841394));
#225665=CARTESIAN_POINT('Ctrl Pts',(5.51435047035643,-5.67601784211672,
97.1085039253896));
#225666=CARTESIAN_POINT('Ctrl Pts',(5.741198866624,-5.44401034281534,97.122919997594));
#225667=CARTESIAN_POINT('Ctrl Pts',(5.82393759965858,-5.35540523930648,
97.1282458997021));
#225668=CARTESIAN_POINT('Ctrl Pts',(6.02259908069153,-5.13260681267485,
97.1411854386722));
#225669=CARTESIAN_POINT('Ctrl Pts',(6.13611117103182,-4.99634838432643,
97.1487131239244));
#225670=CARTESIAN_POINT('Ctrl Pts',(6.30040453350522,-4.78507920594545,
97.1598064022359));
#225671=CARTESIAN_POINT('Ctrl Pts',(6.35463112082665,-4.71282763422311,
97.1635036637587));
#225672=CARTESIAN_POINT('Ctrl Pts',(6.41717453817223,-4.62645198051672,
97.1678122652857));
#225673=CARTESIAN_POINT('Ctrl Pts',(6.42669860568185,-4.61321276522296,
97.1684696311704));
#225674=CARTESIAN_POINT('Ctrl Pts',(6.44125004171768,-4.59285258617101,
97.1694759431189));
#225675=CARTESIAN_POINT('Ctrl Pts',(6.44630666805044,-4.58575264490919,
97.1698260011463));
#225676=CARTESIAN_POINT('Ctrl Pts',(6.45511288616091,-4.57334460343449,
97.1704362749591));
#225677=CARTESIAN_POINT('Ctrl Pts',(6.45886768614249,-4.56804021961416,
97.1706966883102));
#225678=CARTESIAN_POINT('Ctrl Pts',(6.46730760163202,-4.55608599088633,
97.1712824997253));
#225679=CARTESIAN_POINT('Ctrl Pts',(6.47198900859316,-4.54943352997186,
97.1716077570809));
#225680=CARTESIAN_POINT('Ctrl Pts',(6.48450365325546,-4.53159132537088,
97.1724781267602));
#225681=CARTESIAN_POINT('Ctrl Pts',(6.4923182012014,-4.52038847290719,97.1730225315924));
#225682=CARTESIAN_POINT('Ctrl Pts',(6.52602968935439,-4.47179230265024,
97.1753750842385));
#225683=CARTESIAN_POINT('Ctrl Pts',(6.55163311604825,-4.43419592531209,
97.1771721514604));
#225684=CARTESIAN_POINT('Ctrl Pts',(6.95452331100971,-3.83147897144885,
97.205622702174));
#225685=CARTESIAN_POINT('Ctrl Pts',(7.2577820270356,-3.22029861498986,97.2291479340883));
#225686=CARTESIAN_POINT('Ctrl Pts',(7.56509326849239,-2.32867683549825,
97.2612349974756));
#225687=CARTESIAN_POINT('Ctrl Pts',(7.63846228352745,-2.07539416867657,
97.2701629216353));
#225688=CARTESIAN_POINT('Ctrl Pts',(7.75084400605901,-1.59971138835418,
97.2872114056735));
#225689=CARTESIAN_POINT('Ctrl Pts',(7.79324602661001,-1.37839251122473,
97.2952548950128));
#225690=CARTESIAN_POINT('Ctrl Pts',(7.84038694720149,-1.05913097588485,
97.3073568110061));
#225691=CARTESIAN_POINT('Ctrl Pts',(7.85284342424922,-0.962431717163583,
97.3110873262495));
#225692=CARTESIAN_POINT('Ctrl Pts',(7.86874486523778,-0.817964057433518,
97.3167872120169));
#225693=CARTESIAN_POINT('Ctrl Pts',(7.8735486387958,-0.770352263021179,
97.3186861183502));
#225694=CARTESIAN_POINT('Ctrl Pts',(7.878721260414,-0.713967237865432,97.3209618640779));
#225695=CARTESIAN_POINT('Ctrl Pts',(7.87950792393595,-0.705232437932734,
97.3213151717509));
#225696=CARTESIAN_POINT('Ctrl Pts',(7.88069803326697,-0.691767335910473,
97.3218610119056));
#225697=CARTESIAN_POINT('Ctrl Pts',(7.88111175073392,-0.68703792532019,
97.3220529579735));
#225698=CARTESIAN_POINT('Ctrl Pts',(7.88182509144429,-0.678797938889844,
97.3223877842976));
#225699=CARTESIAN_POINT('Ctrl Pts',(7.88212662747459,-0.675287525680402,
97.3225305544656));
#225700=CARTESIAN_POINT('Ctrl Pts',(7.88275144822702,-0.667956069208977,
97.3228289952043));
#225701=CARTESIAN_POINT('Ctrl Pts',(7.88307429995726,-0.664134990926276,
97.3229846907889));
#225702=CARTESIAN_POINT('Ctrl Pts',(7.88385920386712,-0.654764130988174,
97.323366894811));
#225703=CARTESIAN_POINT('Ctrl Pts',(7.88431817373639,-0.649214100745314,
97.3235935826308));
#225704=CARTESIAN_POINT('Ctrl Pts',(7.88608837269084,-0.627529460222969,
97.3244805512199));
#225705=CARTESIAN_POINT('Ctrl Pts',(7.88735591136494,-0.611391656063683,
97.3251434120767));
#225706=CARTESIAN_POINT('Ctrl Pts',(7.90875491336743,-0.327800647260582,
97.3368395425324));
#225707=CARTESIAN_POINT('Ctrl Pts',(7.91531996182526,-0.059519098985165,
97.3486416614873));
#225708=CARTESIAN_POINT('Ctrl Pts',(7.89123618552217,0.853736761718965,
97.3900427745075));
#225709=CARTESIAN_POINT('Ctrl Pts',(7.79533734154688,1.49443656619456,97.420925222916));
#225710=CARTESIAN_POINT('Ctrl Pts',(7.53143407129858,2.44492242450904,97.4647105745562));
#225711=CARTESIAN_POINT('Ctrl Pts',(7.41908471514528,2.76719491001734,97.4792315600571));
#225712=CARTESIAN_POINT('Ctrl Pts',(7.27865842188863,3.09926367564651,97.4937885888836));
#225713=CARTESIAN_POINT('Ctrl Pts',(7.27097157630804,3.11725457701841,97.4945760512397));
#225714=CARTESIAN_POINT('Ctrl Pts',(7.25968243504384,3.14340763047326,97.4957190339759));
#225715=CARTESIAN_POINT('Ctrl Pts',(7.25613297764106,3.15159242296956,97.4960764904644));
#225716=CARTESIAN_POINT('Ctrl Pts',(7.24989087415495,3.16591981802518,97.4967017826272));
#225717=CARTESIAN_POINT('Ctrl Pts',(7.24720425137891,3.17206502461992,97.4969698392007));
#225718=CARTESIAN_POINT('Ctrl Pts',(7.24198137326416,3.18397022586088,97.4974888807895));
#225719=CARTESIAN_POINT('Ctrl Pts',(7.23944605351197,3.18973062317209,97.4977398999078));
#225720=CARTESIAN_POINT('Ctrl Pts',(7.23339156716608,3.20344237412281,97.4983371240578));
#225721=CARTESIAN_POINT('Ctrl Pts',(7.22986615602592,3.21139097198033,97.4986830988146));
#225722=CARTESIAN_POINT('Ctrl Pts',(7.21729004904704,3.23962012629002,97.4999110002761));
#225723=CARTESIAN_POINT('Ctrl Pts',(7.20816702504041,3.25986845822123,97.5007902570765));
#225724=CARTESIAN_POINT('Ctrl Pts',(7.08379332390719,3.53283790920206,97.5126239006332));
#225725=CARTESIAN_POINT('Ctrl Pts',(6.95539151596179,3.77936751685317,97.5230720243156));
#225726=CARTESIAN_POINT('Ctrl Pts',(6.64366230950462,4.30795538938865,97.5452735363578));
#225727=CARTESIAN_POINT('Ctrl Pts',(6.45479141596844,4.58611066683757,97.5568142626404));
#225728=CARTESIAN_POINT('Ctrl Pts',(6.02319011598133,5.14202819215417,97.5806538326943));
#225729=CARTESIAN_POINT('Ctrl Pts',(5.7775851715395,5.41652704018834,97.5928913284044));
#225730=CARTESIAN_POINT('Ctrl Pts',(5.37064471927252,5.81205121208812,97.6128144815226));
#225731=CARTESIAN_POINT('Ctrl Pts',(5.22230064376214,5.94569857918039,97.6200198514225));
#225732=CARTESIAN_POINT('Ctrl Pts',(4.99686823289023,6.13384654129154,97.6311621041247));
#225733=CARTESIAN_POINT('Ctrl Pts',(4.92359975116294,6.19281274532406,97.6348118178087));
#225734=CARTESIAN_POINT('Ctrl Pts',(4.83989476177235,6.25775370309663,97.6390356430057));
#225735=CARTESIAN_POINT('Ctrl Pts',(4.83047276018806,6.26502957883436,97.6395118463631));
#225736=CARTESIAN_POINT('Ctrl Pts',(4.81371671477996,6.27790869434471,97.6403601463575));
#225737=CARTESIAN_POINT('Ctrl Pts',(4.80638920055243,6.2835204333263,97.6407315934619));
#225738=CARTESIAN_POINT('Ctrl Pts',(4.79533995735754,6.29195180329596,97.6412924546718));
#225739=CARTESIAN_POINT('Ctrl Pts',(4.79162552229719,6.29478098549499,97.6414811282059));
#225740=CARTESIAN_POINT('Ctrl Pts',(4.78522589452983,6.29964645794024,97.6418064146796));
#225741=CARTESIAN_POINT('Ctrl Pts',(4.7825419048714,6.30168432125908,97.6419429052726));
#225742=CARTESIAN_POINT('Ctrl Pts',(4.77700322941131,6.30588407514947,97.6422247018895));
#225743=CARTESIAN_POINT('Ctrl Pts',(4.77414837718096,6.30804574298635,97.6423700248229));
#225744=CARTESIAN_POINT('Ctrl Pts',(4.76725831530157,6.31325547787101,97.642720931286));
#225745=CARTESIAN_POINT('Ctrl Pts',(4.76322165367694,6.31630161181189,97.642926661226));
#225746=CARTESIAN_POINT('Ctrl Pts',(4.74837343154869,6.3274840057802,97.6436839311086));
#225747=CARTESIAN_POINT('Ctrl Pts',(4.73754397975144,6.33559635111259,97.6442372622774));
#225748=CARTESIAN_POINT('Ctrl Pts',(4.55811567422073,6.46928886961355,97.6534212393237));
#225749=CARTESIAN_POINT('Ctrl Pts',(4.38461020285829,6.58811782416493,97.6625353368626));
#225750=CARTESIAN_POINT('Ctrl Pts',(3.76137989566182,6.97941948458593,97.695470354475));
#225751=CARTESIAN_POINT('Ctrl Pts',(3.28942223245733,7.21387325520067,97.7206667935144));
#225752=CARTESIAN_POINT('Ctrl Pts',(2.47187406201008,7.52297169109212,97.7613890603567));
#225753=CARTESIAN_POINT('Ctrl Pts',(2.13823938070407,7.62451518065699,97.7772875098587));
#225754=CARTESIAN_POINT('Ctrl Pts',(1.56321109901522,7.75879544377492,97.8030833485542));
#225755=CARTESIAN_POINT('Ctrl Pts',(1.32503454735889,7.80300157161696,97.8133242429023));
#225756=CARTESIAN_POINT('Ctrl Pts',(1.0445859698114,7.84183915792317,97.8248751974729));
#225757=CARTESIAN_POINT('Ctrl Pts',(1.00393939693293,7.8471464229465,97.826537140895));
#225758=CARTESIAN_POINT('Ctrl Pts',(0.951092865194161,7.85362931742629,
97.8286824030371));
#225759=CARTESIAN_POINT('Ctrl Pts',(0.938929260661309,7.85509280270145,
97.8291751095672));
#225760=CARTESIAN_POINT('Ctrl Pts',(0.919211683745207,7.85741870368982,
97.8299720879975));
#225761=CARTESIAN_POINT('Ctrl Pts',(0.911659804927863,7.85829849300339,
97.8302769254328));
#225762=CARTESIAN_POINT('Ctrl Pts',(0.897200543415067,7.85996186444046,
97.830859808803));
#225763=CARTESIAN_POINT('Ctrl Pts',(0.890293375590038,7.86074723110165,
97.831137912534));
#225764=CARTESIAN_POINT('Ctrl Pts',(0.874589487059018,7.86251184864004,
97.8317694324102));
#225765=CARTESIAN_POINT('Ctrl Pts',(0.865792133049322,7.86348544373966,
97.8321226645511));
#225766=CARTESIAN_POINT('Ctrl Pts',(0.842720663683838,7.86599955540351,
97.833047607024));
#225767=CARTESIAN_POINT('Ctrl Pts',(0.828443926474746,7.86751598575828,
97.833618536016));
#225768=CARTESIAN_POINT('Ctrl Pts',(0.77586990251867,7.87295554159818,97.8357157680262));
#225769=CARTESIAN_POINT('Ctrl Pts',(0.737547965979794,7.87663799585846,
97.8372342906579));
#225770=CARTESIAN_POINT('Ctrl Pts',(0.0385986760178754,7.93865614902397,
97.8647504927799));
#225771=CARTESIAN_POINT('Ctrl Pts',(-0.62672874199101,7.91397707627933,
97.8877110379457));
#225772=CARTESIAN_POINT('Ctrl Pts',(-1.79444034881421,7.72233070518094,
97.9285340081368));
#225773=CARTESIAN_POINT('Ctrl Pts',(-2.29809799756727,7.58769673231528,
97.9464646536779));
#225774=CARTESIAN_POINT('Ctrl Pts',(-2.82687578773917,7.38882313738592,
97.9687370056147));
#225775=CARTESIAN_POINT('Ctrl Pts',(-2.86873541897305,7.37267190750078,
97.9705227743298));
#225776=CARTESIAN_POINT('Ctrl Pts',(-2.92103077785455,7.35198133536311,
97.9727805090986));
#225777=CARTESIAN_POINT('Ctrl Pts',(-2.93159770198906,7.34777417131288,
97.9732380894682));
#225778=CARTESIAN_POINT('Ctrl Pts',(-2.9483473620747,7.34106350102359,97.9739655538734));
#225779=CARTESIAN_POINT('Ctrl Pts',(-2.95453609196583,7.33857492803828,
97.9742348073474));
#225780=CARTESIAN_POINT('Ctrl Pts',(-2.96615434398524,7.33388599100251,
97.9747411530418));
#225781=CARTESIAN_POINT('Ctrl Pts',(-2.97158458674744,7.33168741593191,
97.9749781707658));
#225782=CARTESIAN_POINT('Ctrl Pts',(-2.98374313835775,7.32674898309896,
97.9755096581231));
#225783=CARTESIAN_POINT('Ctrl Pts',(-2.99047012069428,7.32400588706953,
97.975804260529));
#225784=CARTESIAN_POINT('Ctrl Pts',(-3.00749696443932,7.31703539468532,
97.9765513047736));
#225785=CARTESIAN_POINT('Ctrl Pts',(-3.01779167950126,7.31279552125958,
97.9770042499056));
#225786=CARTESIAN_POINT('Ctrl Pts',(-3.06455451726518,7.29342070652667,
97.9790674006498));
#225787=CARTESIAN_POINT('Ctrl Pts',(-3.10091761961902,7.27803475135415,
97.9806874658829));
#225788=CARTESIAN_POINT('Ctrl Pts',(-3.64818762825039,7.04162792893815,
98.0052950396016));
#225789=CARTESIAN_POINT('Ctrl Pts',(-4.13447150310487,6.76756346515747,
98.0300237236067));
#225790=CARTESIAN_POINT('Ctrl Pts',(-4.86211254384341,6.24956373282065,
98.0690354277152));
#225791=CARTESIAN_POINT('Ctrl Pts',(-5.12355794879224,6.0370817331948,98.083569190072));
#225792=CARTESIAN_POINT('Ctrl Pts',(-5.5392910443434,5.6526903314339,98.107415175593));
#225793=CARTESIAN_POINT('Ctrl Pts',(-5.70103531946369,5.489522393476,98.1169127748497));
#225794=CARTESIAN_POINT('Ctrl Pts',(-5.89006814094829,5.28144560593661,
98.1283289027479));
#225795=CARTESIAN_POINT('Ctrl Pts',(-5.92430691229725,5.24301040100238,
98.1304105134284));
#225796=CARTESIAN_POINT('Ctrl Pts',(-5.97106499191914,5.18947860511051,
98.1332731969114));
#225797=CARTESIAN_POINT('Ctrl Pts',(-5.98390680020672,5.17466566466596,
98.1340615149998));
#225798=CARTESIAN_POINT('Ctrl Pts',(-6.0054051119838,5.14968046022803,98.1353847646924));
#225799=CARTESIAN_POINT('Ctrl Pts',(-6.01409113713178,5.1395337528861,98.1359203816579));
#225800=CARTESIAN_POINT('Ctrl Pts',(-6.03117305403424,5.11947666237961,
98.1369756625038));
#225801=CARTESIAN_POINT('Ctrl Pts',(-6.03957031802873,5.10956750411814,
98.1374953575957));
#225802=CARTESIAN_POINT('Ctrl Pts',(-6.05796716193314,5.08774966668146,
98.1386359654884));
#225803=CARTESIAN_POINT('Ctrl Pts',(-6.0679561171447,5.07583208630414,98.1392566254849));
#225804=CARTESIAN_POINT('Ctrl Pts',(-6.10254338786483,5.03431883898408,
98.1414103775079));
#225805=CARTESIAN_POINT('Ctrl Pts',(-6.12696094512677,5.0045730669092,98.1429391438879));
#225806=CARTESIAN_POINT('Ctrl Pts',(-6.45537265462178,4.5984916112999,98.1636147973657));
#225807=CARTESIAN_POINT('Ctrl Pts',(-6.72444605504976,4.19521519982848,
98.1817939801042));
#225808=CARTESIAN_POINT('Ctrl Pts',(-7.15527352312746,3.40038275201998,
98.2149174703692));
#225809=CARTESIAN_POINT('Ctrl Pts',(-7.32577578648008,3.01554823521631,
98.2299455050489));
#225810=CARTESIAN_POINT('Ctrl Pts',(-7.51690779666314,2.47076858777956,
98.2515044409374));
#225811=CARTESIAN_POINT('Ctrl Pts',(-7.56448724807535,2.32101911524334,
98.2574645104757));
#225812=CARTESIAN_POINT('Ctrl Pts',(-7.62755998726831,2.09989473099575,
98.2664312742758));
#225813=CARTESIAN_POINT('Ctrl Pts',(-7.64657532172659,2.02956020802687,
98.2693076857157));
#225814=CARTESIAN_POINT('Ctrl Pts',(-7.66758403521467,1.94736224667472,
98.2727073325733));
#225815=CARTESIAN_POINT('Ctrl Pts',(-7.67052560689406,1.93574315666371,
98.2731887717426));
#225816=CARTESIAN_POINT('Ctrl Pts',(-7.67496740081584,1.91802914337357,
98.2739241573202));
#225817=CARTESIAN_POINT('Ctrl Pts',(-7.67648680141312,1.91193901205368,
98.2741772373399));
#225818=CARTESIAN_POINT('Ctrl Pts',(-7.67923167384485,1.90088087011957,
98.2746372346061));
#225819=CARTESIAN_POINT('Ctrl Pts',(-7.68045957781583,1.89591346224504,
98.2748440403623));
#225820=CARTESIAN_POINT('Ctrl Pts',(-7.68308976052964,1.88522873567911,
98.2752892471517));
#225821=CARTESIAN_POINT('Ctrl Pts',(-7.68449047812275,1.87951103895206,
98.2755277202829));
#225822=CARTESIAN_POINT('Ctrl Pts',(-7.6882364845701,1.86414573843466,98.2761692061615));
#225823=CARTESIAN_POINT('Ctrl Pts',(-7.69056999001595,1.85449529632038,
98.2765727708293));
#225824=CARTESIAN_POINT('Ctrl Pts',(-7.70116444731239,1.81031698171258,
98.278423389243));
#225825=CARTESIAN_POINT('Ctrl Pts',(-7.70921102447997,1.77573838083047,
98.2798807524509));
#225826=CARTESIAN_POINT('Ctrl Pts',(-7.84593585391419,1.16973934828971,
98.3055912540705));
#225827=CARTESIAN_POINT('Ctrl Pts',(-7.91098363973838,0.585864373381105,
98.3328497194227));
#225828=CARTESIAN_POINT('Ctrl Pts',(-7.91101873720173,-0.670743544786332,
98.3907569465403));
#225829=CARTESIAN_POINT('Ctrl Pts',(-7.82567762832376,-1.33908526720668,
98.4209363875106));
#225830=CARTESIAN_POINT('Ctrl Pts',(-7.64628732108988,-2.02978156441373,
98.4500986923818));
#225831=CARTESIAN_POINT('Ctrl Pts',(-7.63528548029237,-2.07078214711567,
98.451823212657));
#225832=CARTESIAN_POINT('Ctrl Pts',(-7.62032294958488,-2.12480215298481,
98.4540868686438));
#225833=CARTESIAN_POINT('Ctrl Pts',(-7.61665803010437,-2.13790235980257,
98.4546351602644));
#225834=CARTESIAN_POINT('Ctrl Pts',(-7.61092312184153,-2.15819978593878,
98.4554836696857));
#225835=CARTESIAN_POINT('Ctrl Pts',(-7.6088766801701,-2.16540359955203,
98.4557846184494));
#225836=CARTESIAN_POINT('Ctrl Pts',(-7.60476382065264,-2.17980372711546,
98.456385809281));
#225837=CARTESIAN_POINT('Ctrl Pts',(-7.60269740971548,-2.18700003505791,
98.4566860511905));
#225838=CARTESIAN_POINT('Ctrl Pts',(-7.59806864169619,-2.20303394994832,
98.4573545772178));
#225839=CARTESIAN_POINT('Ctrl Pts',(-7.59550107370888,-2.21187004784318,
98.4577226986473));
#225840=CARTESIAN_POINT('Ctrl Pts',(-7.58797095520063,-2.23761667286436,
98.4587944777998));
#225841=CARTESIAN_POINT('Ctrl Pts',(-7.58296729188018,-2.25451516891353,
98.4594968532769));
#225842=CARTESIAN_POINT('Ctrl Pts',(-7.54673402656659,-2.37539775219195,
98.4645137099034));
#225843=CARTESIAN_POINT('Ctrl Pts',(-7.51342251781657,-2.47874809691327,
98.4687626613628));
#225844=CARTESIAN_POINT('Ctrl Pts',(-7.40074878849384,-2.80515202141151,
98.4820730093524));
#225845=CARTESIAN_POINT('Ctrl Pts',(-7.31349672209356,-3.02534883182184,
98.4908848770619));
#225846=CARTESIAN_POINT('Ctrl Pts',(-6.94099281301107,-3.85469623306248,
98.5238340332307));
#225847=CARTESIAN_POINT('Ctrl Pts',(-6.58843178329839,-4.43041419571599,
98.545995230871));
#225848=CARTESIAN_POINT('Ctrl Pts',(-5.9747327248717,-5.19432968054969,
98.5809925291853));
#225849=CARTESIAN_POINT('Ctrl Pts',(-5.76831998543478,-5.42263603990238,
98.5924005709364));
#225850=CARTESIAN_POINT('Ctrl Pts',(-5.5352728381868,-5.65199556551644,
98.6054315508172));
#225851=CARTESIAN_POINT('Ctrl Pts',(-5.52136086053785,-5.66558677498388,
98.6062094868047));
#225852=CARTESIAN_POINT('Ctrl Pts',(-5.50178434511155,-5.68457132865936,
98.6073040581866));
#225853=CARTESIAN_POINT('Ctrl Pts',(-5.49616164511361,-5.69000785069846,
98.607618423863));
#225854=CARTESIAN_POINT('Ctrl Pts',(-5.48640119716941,-5.69941714630616,
98.6081640946727));
#225855=CARTESIAN_POINT('Ctrl Pts',(-5.48226716823733,-5.7033937791229,
98.60839520167));
#225856=CARTESIAN_POINT('Ctrl Pts',(-5.47366677684582,-5.71164873469736,
98.6088759642936));
#225857=CARTESIAN_POINT('Ctrl Pts',(-5.46919971486687,-5.71592632310298,
98.6091256566775));
#225858=CARTESIAN_POINT('Ctrl Pts',(-5.45868946179345,-5.72596717552358,
98.6097130929393));
#225859=CARTESIAN_POINT('Ctrl Pts',(-5.45264215796011,-5.73172611279303,
98.6100510497705));
#225860=CARTESIAN_POINT('Ctrl Pts',(-5.43292311905883,-5.75044539750492,
98.6111529066858));
#225861=CARTESIAN_POINT('Ctrl Pts',(-5.4192142594299,-5.7633664373078,98.6119186902154));
#225862=CARTESIAN_POINT('Ctrl Pts',(-5.13288345468371,-6.03131756173488,
98.6279061365615));
#225863=CARTESIAN_POINT('Ctrl Pts',(-4.84260276689632,-6.26677445135892,
98.6439484209776));
#225864=CARTESIAN_POINT('Ctrl Pts',(-4.27390255252831,-6.66488274681919,
98.673918804139));
#225865=CARTESIAN_POINT('Ctrl Pts',(-4.00004598469345,-6.83275521322612,
98.6878049456468));
#225866=CARTESIAN_POINT('Ctrl Pts',(-3.44212601675245,-7.12968928874179,
98.7147638393729));
#225867=CARTESIAN_POINT('Ctrl Pts',(-3.15911564739508,-7.25952475633295,
98.7278259953252));
#225868=CARTESIAN_POINT('Ctrl Pts',(-2.64198312911293,-7.4607832332036,
98.7507802882766));
#225869=CARTESIAN_POINT('Ctrl Pts',(-2.41081092964281,-7.53865732956205,
98.7607449958936));
#225870=CARTESIAN_POINT('Ctrl Pts',(-2.05940076095497,-7.63921473906827,
98.775624463039));
#225871=CARTESIAN_POINT('Ctrl Pts',(-1.94163343364575,-7.66999304525702,
98.7805623636893));
#225872=CARTESIAN_POINT('Ctrl Pts',(-1.78380533569913,-7.70737300924631,
98.7871140685367));
#225873=CARTESIAN_POINT('Ctrl Pts',(-1.74433728215809,-7.71640121053048,
98.7887470345179));
#225874=CARTESIAN_POINT('Ctrl Pts',(-1.68192841604885,-7.73017376671745,
98.7913206761723));
#225875=CARTESIAN_POINT('Ctrl Pts',(-1.65903292598478,-7.73511987070554,
98.7922630539052));
#225876=CARTESIAN_POINT('Ctrl Pts',(-1.6123019019529,-7.74499812895948,
98.7941828683496));
#225877=CARTESIAN_POINT('Ctrl Pts',(-1.58846488851236,-7.74992211202235,
98.7951602237806));
#225878=CARTESIAN_POINT('Ctrl Pts',(-1.53364193106535,-7.76098326228714,
98.7974036824061));
#225879=CARTESIAN_POINT('Ctrl Pts',(-1.50264116615804,-7.76704501754189,
98.7986690917331));
#225880=CARTESIAN_POINT('Ctrl Pts',(-1.40539072386973,-7.78545691502914,
98.802628873742));
#225881=CARTESIAN_POINT('Ctrl Pts',(-1.33901881075219,-7.79714634795118,
98.8053170528809));
#225882=CARTESIAN_POINT('Ctrl Pts',(-0.937927380250833,-7.86251416057637,
98.8214803021833));
#225883=CARTESIAN_POINT('Ctrl Pts',(-0.600185919568113,-7.89548110125634,
98.8347334863076));
#225884=CARTESIAN_POINT('Ctrl Pts',(-0.0246677904935639,-7.91450567373134,
98.8570695051716));
#225885=CARTESIAN_POINT('Ctrl Pts',(0.212262926423433,-7.91169723486317,
98.8661982021483));
#225886=CARTESIAN_POINT('Ctrl Pts',(0.759972172086068,-7.88058120306497,
98.8874337134158));
#225887=CARTESIAN_POINT('Ctrl Pts',(1.06990866691048,-7.84451415959061,
98.8995478124556));
#225888=CARTESIAN_POINT('Ctrl Pts',(1.40376157272442,-7.78550696426278,
98.9131138329763));
#225889=CARTESIAN_POINT('Ctrl Pts',(1.43060116509962,-7.78061986846865,
98.9142081852918));
#225890=CARTESIAN_POINT('Ctrl Pts',(1.47031382070948,-7.77317634548602,
98.915833375055));
#225891=CARTESIAN_POINT('Ctrl Pts',(1.48320675079332,-7.77072654018406,
98.9163619330019));
#225892=CARTESIAN_POINT('Ctrl Pts',(1.50609523145509,-7.76631842631278,
98.9173019794369));
#225893=CARTESIAN_POINT('Ctrl Pts',(1.51609321894849,-7.76437287202534,
98.9177131846985));
#225894=CARTESIAN_POINT('Ctrl Pts',(1.53707686316422,-7.76024749301256,
98.9185774679981));
#225895=CARTESIAN_POINT('Ctrl Pts',(1.54806170063479,-7.75806363766974,
98.9190306369322));
#225896=CARTESIAN_POINT('Ctrl Pts',(1.57714518747676,-7.7522174267336,98.9202324111841));
#225897=CARTESIAN_POINT('Ctrl Pts',(1.59523558129246,-7.74851504541726,
98.9209819700916));
#225898=CARTESIAN_POINT('Ctrl Pts',(1.69370014617598,-7.72800383934418,
98.9250728845901));
#225899=CARTESIAN_POINT('Ctrl Pts',(1.77382085339344,-7.71000796148252,
98.9284416655938));
#225900=CARTESIAN_POINT('Ctrl Pts',(2.01821425200847,-7.65110373003592,
98.9388226137978));
#225901=CARTESIAN_POINT('Ctrl Pts',(2.18146487550481,-7.60616765252071,
98.9459026261555));
#225902=CARTESIAN_POINT('Ctrl Pts',(2.68719672269585,-7.44933883790576,
98.9681609105973));
#225903=CARTESIAN_POINT('Ctrl Pts',(3.02356479363775,-7.31927160074027,
98.9834224472502));
#225904=CARTESIAN_POINT('Ctrl Pts',(3.48770527884947,-7.10232167752844,
99.0048263390568));
#225905=CARTESIAN_POINT('Ctrl Pts',(3.62362831538655,-7.03394485904147,
99.0111423730151));
#225906=CARTESIAN_POINT('Ctrl Pts',(3.76166445949593,-6.95944135133719,
99.0176046637327));
#225907=CARTESIAN_POINT('Ctrl Pts',(3.76583001924336,-6.95718820319961,
99.0177997249003));
#225908=CARTESIAN_POINT('Ctrl Pts',(3.84118415175708,-6.91634170435553,
99.021329187333));
#225909=CARTESIAN_POINT('Ctrl Pts',(3.91177854312674,-6.87666104163887,
99.0246493140159));
#225910=CARTESIAN_POINT('Ctrl Pts',(4.05664281298024,-6.79228103450938,
99.031492475074));
#225911=CARTESIAN_POINT('Ctrl Pts',(4.13081247487797,-6.74743070373213,
99.0350128964895));
#225912=CARTESIAN_POINT('Ctrl Pts',(4.23154456760542,-6.68423452995794,
99.0398199092137));
#225913=CARTESIAN_POINT('Ctrl Pts',(4.25875341140569,-6.66693183346884,
99.0411209768227));
#225914=CARTESIAN_POINT('Ctrl Pts',(4.30194473364927,-6.63909322871091,
99.0431907244313));
#225915=CARTESIAN_POINT('Ctrl Pts',(4.31799601499919,-6.62866485861541,
99.0439608934649));
#225916=CARTESIAN_POINT('Ctrl Pts',(4.3509141434526,-6.60710794845414,99.0455424544446));
#225917=CARTESIAN_POINT('Ctrl Pts',(4.36777652176863,-6.59597283082689,
99.0463537483332));
#225918=CARTESIAN_POINT('Ctrl Pts',(4.40678942579361,-6.56999534903854,
99.0482334934496));
#225919=CARTESIAN_POINT('Ctrl Pts',(4.42890796742315,-6.5551053502039,99.0493012779171));
#225920=CARTESIAN_POINT('Ctrl Pts',(4.49926030241381,-6.50722617329936,
99.052704457633));
#225921=CARTESIAN_POINT('Ctrl Pts',(4.54720419930508,-6.47381415965826,
99.0550340474065));
#225922=CARTESIAN_POINT('Ctrl Pts',(5.24646893870848,-5.97489704992239,
99.0891817507046));
#225923=CARTESIAN_POINT('Ctrl Pts',(5.82386893201732,-5.4136424181868,99.1198409935087));
#225924=CARTESIAN_POINT('Ctrl Pts',(6.64221580538611,-4.33277928054284,
99.1706381247242));
#225925=CARTESIAN_POINT('Ctrl Pts',(6.92973663164825,-3.85625118077057,
99.1910123616771));
#225926=CARTESIAN_POINT('Ctrl Pts',(7.17019824564363,-3.34250331177446,
99.2134958864722));
#225927=CARTESIAN_POINT('Ctrl Pts',(7.17536900682167,-3.33138873225042,
99.2139825987286));
#225928=CARTESIAN_POINT('Ctrl Pts',(7.19278697138116,-3.29372003962416,
99.2156332448697));
#225929=CARTESIAN_POINT('Ctrl Pts',(7.20491269926392,-3.26711020436851,
99.2168011669056));
#225930=CARTESIAN_POINT('Ctrl Pts',(7.22137695041343,-3.23044206040998,
99.2184137642866));
#225931=CARTESIAN_POINT('Ctrl Pts',(7.22584260538315,-3.2204409025077,99.218853923675));
#225932=CARTESIAN_POINT('Ctrl Pts',(7.23291627397618,-3.20451012410709,
99.2195556096784));
#225933=CARTESIAN_POINT('Ctrl Pts',(7.23553780732859,-3.19858650036404,
99.2198166439741));
#225934=CARTESIAN_POINT('Ctrl Pts',(7.24062001124114,-3.18706451917233,
99.2203246276588));
#225935=CARTESIAN_POINT('Ctrl Pts',(7.24308147196374,-3.18146651511298,
99.2205715475689));
#225936=CARTESIAN_POINT('Ctrl Pts',(7.24894743708985,-3.16808368710794,
99.2211621271317));
#225937=CARTESIAN_POINT('Ctrl Pts',(7.25234589179522,-3.16029622967963,
99.2215060128619));
#225938=CARTESIAN_POINT('Ctrl Pts',(7.26248234121273,-3.13696640238405,
99.2225369497129));
#225939=CARTESIAN_POINT('Ctrl Pts',(7.26918294289581,-3.12140790405018,
99.223225425313));
#225940=CARTESIAN_POINT('Ctrl Pts',(7.32870920387433,-2.98195937300613,
99.2294054645787));
#225941=CARTESIAN_POINT('Ctrl Pts',(7.37840681388255,-2.85677652079024,
99.2350260527524));
#225942=CARTESIAN_POINT('Ctrl Pts',(7.44935769551707,-2.66383503064301,
99.2438340069574));
#225943=CARTESIAN_POINT('Ctrl Pts',(7.47293020285764,-2.59697148874598,
99.246908825913));
#225944=CARTESIAN_POINT('Ctrl Pts',(7.55238080543388,-2.3615656903002,99.2577922049086));
#225945=CARTESIAN_POINT('Ctrl Pts',(7.60347931466858,-2.19147127737009,
99.2657584727625));
#225946=CARTESIAN_POINT('Ctrl Pts',(7.7706368263004,-1.55846266697287,99.2954662118341));
#225947=CARTESIAN_POINT('Ctrl Pts',(7.85048012432108,-1.08701359333058,
99.3176475870243));
#225948=CARTESIAN_POINT('Ctrl Pts',(7.90410469806455,-0.395055029340094,
99.3486391877209));
#225949=CARTESIAN_POINT('Ctrl Pts',(7.91196380928407,-0.17825985578506,
99.3581406332996));
#225950=CARTESIAN_POINT('Ctrl Pts',(7.90996582736476,0.231277259141387,
99.375617604322));
#225951=CARTESIAN_POINT('Ctrl Pts',(7.90198648914165,0.423868870817894,
99.3836398312914));
#225952=CARTESIAN_POINT('Ctrl Pts',(7.88544742337866,0.6356321597011,99.3922435974754));
#225953=CARTESIAN_POINT('Ctrl Pts',(7.8838396532414,0.655272186597666,99.3930395153676));
#225954=CARTESIAN_POINT('Ctrl Pts',(7.88133608038385,0.6845111552324,99.3942214184362));
#225955=CARTESIAN_POINT('Ctrl Pts',(7.88049609358636,0.694114726383551,
99.394609131192));
#225956=CARTESIAN_POINT('Ctrl Pts',(7.8790245802502,0.710591516297084,99.3952734997001));
#225957=CARTESIAN_POINT('Ctrl Pts',(7.87840160993954,0.717465477952482,
99.3955504206153));
#225958=CARTESIAN_POINT('Ctrl Pts',(7.87710251092903,0.731594232613963,
99.3961190976005));
#225959=CARTESIAN_POINT('Ctrl Pts',(7.87642535378712,0.738848926012412,
99.3964108214559));
#225960=CARTESIAN_POINT('Ctrl Pts',(7.87483499467366,0.755636497234123,
99.3970852453478));
#225961=CARTESIAN_POINT('Ctrl Pts',(7.87391450286643,0.765168681835595,
99.3974677183516));
#225962=CARTESIAN_POINT('Ctrl Pts',(7.87109962839674,0.793775193009246,
99.3986141246069));
#225963=CARTESIAN_POINT('Ctrl Pts',(7.86915322119475,0.812844391697003,
99.3993764374307));
#225964=CARTESIAN_POINT('Ctrl Pts',(7.85344592962012,0.961384444731322,
99.4052999713715));
#225965=CARTESIAN_POINT('Ctrl Pts',(7.83655965069292,1.09050806284452,99.4103627189021));
#225966=CARTESIAN_POINT('Ctrl Pts',(7.76572813182077,1.54463554969295,99.4278988366886));
#225967=CARTESIAN_POINT('Ctrl Pts',(7.69468161645525,1.86663601457365,99.4398264764234));
#225968=CARTESIAN_POINT('Ctrl Pts',(7.52496664335182,2.45770457073493,99.4613792201013));
#225969=CARTESIAN_POINT('Ctrl Pts',(7.43137347190531,2.72765971308225,99.4710877813163));
#225970=CARTESIAN_POINT('Ctrl Pts',(7.14201751954367,3.43591193272017,99.4971100332526));
#225971=CARTESIAN_POINT('Ctrl Pts',(6.92066575446557,3.86241050028523,99.5133517542529));
#225972=CARTESIAN_POINT('Ctrl Pts',(6.59827504956847,4.36585508380428,99.5359785540405));
#225973=CARTESIAN_POINT('Ctrl Pts',(6.53223462772573,4.46406010133416,99.5405728360392));
#225974=CARTESIAN_POINT('Ctrl Pts',(6.4569133424467,4.57081426256553,99.5458089232293));
#225975=CARTESIAN_POINT('Ctrl Pts',(6.44978372757322,4.58086921872577,99.5463045140328));
#225976=CARTESIAN_POINT('Ctrl Pts',(6.43980445550087,4.59487358835497,99.5469981948218));
#225977=CARTESIAN_POINT('Ctrl Pts',(6.43697457505507,4.59883713975062,99.5471949065805));
#225978=CARTESIAN_POINT('Ctrl Pts',(6.43201802876971,4.60576577694451,99.54753945347));
#225979=CARTESIAN_POINT('Ctrl Pts',(6.42989296565739,4.60873201266815,99.5476871758118));
#225980=CARTESIAN_POINT('Ctrl Pts',(6.42542860009387,4.61495442883033,99.5479975191016));
#225981=CARTESIAN_POINT('Ctrl Pts',(6.42308887373719,4.6182103021671,99.5481601701002));
#225982=CARTESIAN_POINT('Ctrl Pts',(6.41750368342175,4.6259699837609,99.5485484477531));
#225983=CARTESIAN_POINT('Ctrl Pts',(6.41425595588301,4.63047215189779,99.5487742361499));
#225984=CARTESIAN_POINT('Ctrl Pts',(6.40324302910806,4.64570502257368,99.5495399199206));
#225985=CARTESIAN_POINT('Ctrl Pts',(6.39545577811958,4.65641942163472,99.5500814228644));
#225986=CARTESIAN_POINT('Ctrl Pts',(6.19722667876004,4.92772549688855,99.5638675442345));
#225987=CARTESIAN_POINT('Ctrl Pts',(5.99105739798228,5.17641658403769,99.5782333546393));
#225988=CARTESIAN_POINT('Ctrl Pts',(5.41993088809848,5.78537753992614,99.6164302182257));
#225989=CARTESIAN_POINT('Ctrl Pts',(5.03407603840127,6.12408151391154,99.6407002800454));
#225990=CARTESIAN_POINT('Ctrl Pts',(4.28250626289484,6.66445773220789,99.682484282267));
#225991=CARTESIAN_POINT('Ctrl Pts',(3.92839257188176,6.87914681779897,99.7003562911821));
#225992=CARTESIAN_POINT('Ctrl Pts',(3.53554684585869,7.07704200256692,99.7181746442548));
#225993=CARTESIAN_POINT('Ctrl Pts',(3.51196023590244,7.0887763630854,99.7192373389474));
#225994=CARTESIAN_POINT('Ctrl Pts',(3.47992325037195,7.10451564823155,99.7206711980472));
#225995=CARTESIAN_POINT('Ctrl Pts',(3.47152389039472,7.1086236574798,99.7210462357114));
#225996=CARTESIAN_POINT('Ctrl Pts',(3.4572986767142,7.1155497849202,99.7216799062755));
#225997=CARTESIAN_POINT('Ctrl Pts',(3.45147662225779,7.11837565797071,99.721938830037));
#225998=CARTESIAN_POINT('Ctrl Pts',(3.44027402499826,7.12379613091841,99.7224362307485));
#225999=CARTESIAN_POINT('Ctrl Pts',(3.43489399963865,7.12639178641137,99.7226747471569));
#226000=CARTESIAN_POINT('Ctrl Pts',(3.42222039983532,7.13248862524414,99.7232357708466));
#226001=CARTESIAN_POINT('Ctrl Pts',(3.41492437745777,7.13598472189183,99.7235580876067));
#226002=CARTESIAN_POINT('Ctrl Pts',(3.39495045267268,7.14551814788077,99.7244386854815));
#226003=CARTESIAN_POINT('Ctrl Pts',(3.38226178948552,7.15153293832773,99.7249961242341));
#226004=CARTESIAN_POINT('Ctrl Pts',(3.30224808529317,7.18920114969296,99.7284989553831));
#226005=CARTESIAN_POINT('Ctrl Pts',(3.23449426377056,7.21993787035328,99.7314101218146));
#226006=CARTESIAN_POINT('Ctrl Pts',(3.03478114565198,7.30716264832339,99.7398369059276));
#226007=CARTESIAN_POINT('Ctrl Pts',(2.90170398506538,7.36102161355111,99.7452566758439));
#226008=CARTESIAN_POINT('Ctrl Pts',(2.45031442786735,7.52956294805092,99.7630626215027));
#226009=CARTESIAN_POINT('Ctrl Pts',(2.12612378533902,7.62744887504805,99.7748868692137));
#226010=CARTESIAN_POINT('Ctrl Pts',(1.11075455528472,7.86423420933607,99.8104736048209));
#226011=CARTESIAN_POINT('Ctrl Pts',(0.406690666053647,7.93185002458857,
99.8329572724607));
#226012=CARTESIAN_POINT('Ctrl Pts',(-0.338035826160578,7.90388185081331,
99.8622130333718));
#226013=CARTESIAN_POINT('Ctrl Pts',(-0.379170216534957,7.9020153350695,
99.8638474514539));
#226014=CARTESIAN_POINT('Ctrl Pts',(-0.427966331734888,7.89941927939347,
99.8658102803397));
#226015=CARTESIAN_POINT('Ctrl Pts',(-0.435644628270546,7.89899954993055,
99.8661198457778));
#226016=CARTESIAN_POINT('Ctrl Pts',(-0.448083273495483,7.89830140717396,
99.8666224944332));
#226017=CARTESIAN_POINT('Ctrl Pts',(-0.452843992029466,7.89802988453942,
99.8668151523714));
#226018=CARTESIAN_POINT('Ctrl Pts',(-0.461329434976493,7.8975382287393,
99.8671590348939));
#226019=CARTESIAN_POINT('Ctrl Pts',(-0.465054244069399,7.89731976508169,
99.8673101557158));
#226020=CARTESIAN_POINT('Ctrl Pts',(-0.472905817002281,7.89685368863958,
99.86762905851));
#226021=CARTESIAN_POINT('Ctrl Pts',(-0.477032542688414,7.89660547606497,
99.8677968770894));
#226022=CARTESIAN_POINT('Ctrl Pts',(-0.487927225552354,7.89594161583414,
99.8682404630001));
#226023=CARTESIAN_POINT('Ctrl Pts',(-0.494694832863919,7.89552050214902,
99.8685165615946));
#226024=CARTESIAN_POINT('Ctrl Pts',(-0.525201471588934,7.89358285295974,
99.869763595958));
#226025=CARTESIAN_POINT('Ctrl Pts',(-0.548933896884607,7.89196796716087,
99.8707404137593));
#226026=CARTESIAN_POINT('Ctrl Pts',(-0.724856136695996,7.87919987974183,
99.8780290851628));
#226027=CARTESIAN_POINT('Ctrl Pts',(-0.876693656528433,7.86375291250337,
99.8845848860862));
#226028=CARTESIAN_POINT('Ctrl Pts',(-1.22110303201062,7.81861659708257,
99.8999104414949));
#226029=CARTESIAN_POINT('Ctrl Pts',(-1.41321695100678,7.78618448157754,
99.9087853264157));
#226030=CARTESIAN_POINT('Ctrl Pts',(-2.02289269791113,7.65995314096664,
99.9375995350762));
#226031=CARTESIAN_POINT('Ctrl Pts',(-2.43413094089788,7.53936313303955,
99.9579828949913));
#226032=CARTESIAN_POINT('Ctrl Pts',(-2.94204080598174,7.34450850181288,
99.9831749588147));
#226033=CARTESIAN_POINT('Ctrl Pts',(-3.04954667650439,7.30052569107931,
99.9885115869853));
#226034=CARTESIAN_POINT('Ctrl Pts',(-3.52844454229034,7.09217380966174,
100.012254229967));
#226035=CARTESIAN_POINT('Ctrl Pts',(-3.88784257573235,6.90170974331125,
100.029946247056));
#226036=CARTESIAN_POINT('Ctrl Pts',(-4.27621615772971,6.65588101810236,
100.048789482886));
#226037=CARTESIAN_POINT('Ctrl Pts',(-4.32107990253558,6.62684279153073,
100.050962600504));
#226038=CARTESIAN_POINT('Ctrl Pts',(-4.37729986957994,6.58964051483371,
100.053681834073));
#226039=CARTESIAN_POINT('Ctrl Pts',(-4.38893273794415,6.58189833463449,
100.054244274717));
#226040=CARTESIAN_POINT('Ctrl Pts',(-4.40725271524248,6.56963542792334,
100.055129708881));
#226041=CARTESIAN_POINT('Ctrl Pts',(-4.41395349574257,6.5651352377371,100.055453499973));
#226042=CARTESIAN_POINT('Ctrl Pts',(-4.42578884400816,6.5571604025512,100.056025283168));
#226043=CARTESIAN_POINT('Ctrl Pts',(-4.43092623089538,6.55368996620407,
100.056273438725));
#226044=CARTESIAN_POINT('Ctrl Pts',(-4.44269484299823,6.54571980399677,
100.056841820331));
#226045=CARTESIAN_POINT('Ctrl Pts',(-4.44932332641263,6.54121603052424,
100.057161888295));
#226046=CARTESIAN_POINT('Ctrl Pts',(-4.46758875441763,6.52876483729024,
100.058043696273));
#226047=CARTESIAN_POINT('Ctrl Pts',(-4.47921135129115,6.52079636642775,
100.058604614279));
#226048=CARTESIAN_POINT('Ctrl Pts',(-4.53868904410173,6.47978431273023,
100.061474151067));
#226049=CARTESIAN_POINT('Ctrl Pts',(-4.58620060277757,6.44624442569634,
100.063763309444));
#226050=CARTESIAN_POINT('Ctrl Pts',(-4.71402705842803,6.35387912016852,
100.069916615734));
#226051=CARTESIAN_POINT('Ctrl Pts',(-4.79360933159158,6.29405603926756,
100.073741433449));
#226052=CARTESIAN_POINT('Ctrl Pts',(-5.07942099013546,6.07064137567329,
100.087480445971));
#226053=CARTESIAN_POINT('Ctrl Pts',(-5.27858640632783,5.89828291865341,
100.097052707928));
#226054=CARTESIAN_POINT('Ctrl Pts',(-5.60729108466952,5.58381087315769,
100.11318185826));
#226055=CARTESIAN_POINT('Ctrl Pts',(-5.74092604192876,5.44632237629273,
100.119847616671));
#226056=CARTESIAN_POINT('Ctrl Pts',(-6.28239925648062,4.84713788875576,
100.147769130589));
#226057=CARTESIAN_POINT('Ctrl Pts',(-6.64057738476161,4.34350109300738,
100.168481894583));
#226058=CARTESIAN_POINT('Ctrl Pts',(-6.95620979018949,3.76785268141195,
100.194408357079));
#226059=CARTESIAN_POINT('Ctrl Pts',(-6.97544972951901,3.73211326997488,
100.196025014702));
#226060=CARTESIAN_POINT('Ctrl Pts',(-6.99972811589647,3.68617100640897,
100.198110850572));
#226061=CARTESIAN_POINT('Ctrl Pts',(-7.00502098498729,3.67610274381265,
100.198568430119));
#226062=CARTESIAN_POINT('Ctrl Pts',(-7.01341415730664,3.66005303887433,
100.199298562521));
#226063=CARTESIAN_POINT('Ctrl Pts',(-7.0165285778904,3.65407896802547,100.199570490907));
#226064=CARTESIAN_POINT('Ctrl Pts',(-7.02233395673365,3.64290832245376,
100.200079240985));
#226065=CARTESIAN_POINT('Ctrl Pts',(-7.02502678930221,3.63771272299616,
100.200315981043));
#226066=CARTESIAN_POINT('Ctrl Pts',(-7.03100777589281,3.62614149145517,
100.200843477906));
#226067=CARTESIAN_POINT('Ctrl Pts',(-7.03429302564407,3.61976436935683,
100.201134358607));
#226068=CARTESIAN_POINT('Ctrl Pts',(-7.04382014383441,3.6012089710082,100.201981199657));
#226069=CARTESIAN_POINT('Ctrl Pts',(-7.05003907495541,3.58901898995439,
100.202538121082));
#226070=CARTESIAN_POINT('Ctrl Pts',(-7.09374963978311,3.50278813594496,
100.206481627742));
#226071=CARTESIAN_POINT('Ctrl Pts',(-7.13010501193297,3.42817890692869,
100.209913859396));
#226072=CARTESIAN_POINT('Ctrl Pts',(-7.24354722690091,3.18575661924743,
100.221105052021));
#226073=CARTESIAN_POINT('Ctrl Pts',(-7.31593287202391,3.015815599745,100.22900877245));
#226074=CARTESIAN_POINT('Ctrl Pts',(-7.69508737201932,2.03145472543838,
100.274677109224));
#226075=CARTESIAN_POINT('Ctrl Pts',(-7.8717964715237,1.1731838255701,100.313261996288));
#226076=CARTESIAN_POINT('Ctrl Pts',(-7.90778348611013,0.235565568481009,
100.351510221745));
#226077=CARTESIAN_POINT('Ctrl Pts',(-7.90951398097792,0.167688775737525,
100.354262554791));
#226078=CARTESIAN_POINT('Ctrl Pts',(-7.91063518710626,0.0788173711341605,
100.357846248243));
#226079=CARTESIAN_POINT('Ctrl Pts',(-7.91081640755467,0.0578360815328407,
100.358690834597));
#226080=CARTESIAN_POINT('Ctrl Pts',(-7.91095939646905,0.0271429402881354,
100.359924196337));
#226081=CARTESIAN_POINT('Ctrl Pts',(-7.91098675602236,0.0174315323452157,
100.360314118503));
#226082=CARTESIAN_POINT('Ctrl Pts',(-7.9109986139482,0.00528037141865606,
100.36080160118));
#226083=CARTESIAN_POINT('Ctrl Pts',(-7.91099986619226,0.0028406554486198,
100.36089945812));
#226084=CARTESIAN_POINT('Ctrl Pts',(-7.91099998983997,0.000400938813840742,
100.360997295013));
#226085=CARTESIAN_POINT('',(-7.91099966760513,0.0022932840043321,104.357668491763));
#226086=CARTESIAN_POINT('Ctrl Pts',(-7.91099998985159,0.000400709535323949,
100.360997304208));
#226087=CARTESIAN_POINT('Ctrl Pts',(-7.91100005916832,-0.00096777466909486,
100.361052182811));
#226088=CARTESIAN_POINT('Ctrl Pts',(-7.91099977339425,-0.0023362592533744,
100.361107055113));
#226089=CARTESIAN_POINT('Ctrl Pts',(-7.91099481889614,-0.0129159455629224,
100.361531221317));
#226090=CARTESIAN_POINT('Ctrl Pts',(-7.91097441761624,-0.0221271438946392,
100.361900235188));
#226091=CARTESIAN_POINT('Ctrl Pts',(-7.9108839673096,-0.0449601254811435,
100.362814247241));
#226092=CARTESIAN_POINT('Ctrl Pts',(-7.91079482285094,-0.0585818167777481,
100.363358901693));
#226093=CARTESIAN_POINT('Ctrl Pts',(-7.91047650445436,-0.0934571507487213,
100.364751764797));
#226094=CARTESIAN_POINT('Ctrl Pts',(-7.91019685774666,-0.114710259158208,
100.365599052871));
#226095=CARTESIAN_POINT('Ctrl Pts',(-7.90875991398719,-0.198306994295018,
100.368925776633));
#226096=CARTESIAN_POINT('Ctrl Pts',(-7.90695119593621,-0.260637607527513,
100.371393086984));
#226097=CARTESIAN_POINT('Ctrl Pts',(-7.90249133677941,-0.36979856628818,
100.375691679267));
#226098=CARTESIAN_POINT('Ctrl Pts',(-7.90016029240393,-0.416638596432845,
100.377528920584));
#226099=CARTESIAN_POINT('Ctrl Pts',(-7.84862792702768,-1.29476478794368,
100.411841212678));
#226100=CARTESIAN_POINT('Ctrl Pts',(-7.66891076730538,-2.11305738826948,
100.44078653494));
#226101=CARTESIAN_POINT('Ctrl Pts',(-7.30927976399866,-3.03011227916851,
100.477635387858));
#226102=CARTESIAN_POINT('Ctrl Pts',(-7.24954767217067,-3.17036380904551,
100.48342851042));
#226103=CARTESIAN_POINT('Ctrl Pts',(-7.15675422184594,-3.37188582833366,
100.492090936159));
#226104=CARTESIAN_POINT('Ctrl Pts',(-7.12687537517983,-3.43458760615161,
100.494835201216));
#226105=CARTESIAN_POINT('Ctrl Pts',(-7.09094407331893,-3.50750241825568,
100.498092809226));
#226106=CARTESIAN_POINT('Ctrl Pts',(-7.08568891353161,-3.5181065480568,
100.498568226209));
#226107=CARTESIAN_POINT('Ctrl Pts',(-7.07762446072729,-3.53428804595264,
100.499296285653));
#226108=CARTESIAN_POINT('Ctrl Pts',(-7.07483231129418,-3.53987397594719,
100.499548088056));
#226109=CARTESIAN_POINT('Ctrl Pts',(-7.06974115123421,-3.55002918556588,
100.500006734873));
#226110=CARTESIAN_POINT('Ctrl Pts',(-7.06744431572416,-3.55459955659971,
100.500213470987));
#226111=CARTESIAN_POINT('Ctrl Pts',(-7.06248339828401,-3.56444724978386,
100.500659620807));
#226112=CARTESIAN_POINT('Ctrl Pts',(-7.05981783171737,-3.56972381707702,
100.500899109287));
#226113=CARTESIAN_POINT('Ctrl Pts',(-7.05261156336944,-3.58394919545232,
100.501545941749));
#226114=CARTESIAN_POINT('Ctrl Pts',(-7.04805975554051,-3.59289234186743,
100.501953853564));
#226115=CARTESIAN_POINT('Ctrl Pts',(-7.02683902294677,-3.63439018384741,
100.503852622512));
#226116=CARTESIAN_POINT('Ctrl Pts',(-7.00996164324436,-3.66683738680443,
100.50535447422));
#226117=CARTESIAN_POINT('Ctrl Pts',(-6.70604959406883,-4.24134902490025,
100.532268565335));
#226118=CARTESIAN_POINT('Ctrl Pts',(-6.35717693381678,-4.74829909701657,
100.560950994744));
#226119=CARTESIAN_POINT('Ctrl Pts',(-5.89970098056773,-5.27105985696377,
100.592927251231));
#226120=CARTESIAN_POINT('Ctrl Pts',(-5.84516589666356,-5.33147066726718,
100.596665848537));
#226121=CARTESIAN_POINT('Ctrl Pts',(-5.67328505447062,-5.51606247539534,
100.608210721887));
#226122=CARTESIAN_POINT('Ctrl Pts',(-5.55283970542294,-5.63729390171303,
100.615966660102));
#226123=CARTESIAN_POINT('Ctrl Pts',(-5.22584614081406,-5.94576451901958,
100.636082923621));
#226124=CARTESIAN_POINT('Ctrl Pts',(-5.01315853501962,-6.12616058863582,
100.64823983385));
#226125=CARTESIAN_POINT('Ctrl Pts',(-4.67712960497867,-6.38192721901521,
100.666017629867));
#226126=CARTESIAN_POINT('Ctrl Pts',(-4.56052961069703,-6.4657643614975,
100.671948211451));
#226127=CARTESIAN_POINT('Ctrl Pts',(-4.42602670540259,-6.55702430384257,
100.678529492214));
#226128=CARTESIAN_POINT('Ctrl Pts',(-4.41030691548808,-6.56760786249891,
100.679294755282));
#226129=CARTESIAN_POINT('Ctrl Pts',(-4.38666934192807,-6.58339903756214,
100.680439642338));
#226130=CARTESIAN_POINT('Ctrl Pts',(-4.3787800348527,-6.58864904288807,
100.680820792555));
#226131=CARTESIAN_POINT('Ctrl Pts',(-4.36520877535687,-6.59764500891665,
100.681474792782));
#226132=CARTESIAN_POINT('Ctrl Pts',(-4.35953139658114,-6.60139783065872,
100.68174788911));
#226133=CARTESIAN_POINT('Ctrl Pts',(-4.34784198503017,-6.6091030283048,
100.682309159904));
#226134=CARTESIAN_POINT('Ctrl Pts',(-4.34182938763695,-6.61305453890542,
100.682597303221));
#226135=CARTESIAN_POINT('Ctrl Pts',(-4.32566470163404,-6.62364650695907,
100.683370485952));
#226136=CARTESIAN_POINT('Ctrl Pts',(-4.31550269821128,-6.63027183631714,
100.683854983857));
#226137=CARTESIAN_POINT('Ctrl Pts',(-4.27839620460869,-6.6543427373366,
100.685618443905));
#226138=CARTESIAN_POINT('Ctrl Pts',(-4.2513606816658,-6.67164775250914,
100.686892393602));
#226139=CARTESIAN_POINT('Ctrl Pts',(-3.81382648893587,-6.9479670039561,
100.707336783204));
#226140=CARTESIAN_POINT('Ctrl Pts',(-3.38043850933824,-7.16883667239189,
100.725063383063));
#226141=CARTESIAN_POINT('Ctrl Pts',(-2.84720211064242,-7.38140976604101,
100.745227892795));
#226142=CARTESIAN_POINT('Ctrl Pts',(-2.76435998044787,-7.41283239400004,
100.748318652713));
#226143=CARTESIAN_POINT('Ctrl Pts',(-2.43402420655599,-7.53182332837274,
100.760515467844));
#226144=CARTESIAN_POINT('Ctrl Pts',(-2.18276736766272,-7.60844020606949,
100.769506912133));
#226145=CARTESIAN_POINT('Ctrl Pts',(-1.84167196983505,-7.69416138619284,
100.781724609971));
#226146=CARTESIAN_POINT('Ctrl Pts',(-1.75481518895129,-7.71443442395475,
100.784837201403));
#226147=CARTESIAN_POINT('Ctrl Pts',(-1.53823893740258,-7.76113805571743,
100.792633668757));
#226148=CARTESIAN_POINT('Ctrl Pts',(-1.40816548850933,-7.78578907201624,
100.797347232527));
#226149=CARTESIAN_POINT('Ctrl Pts',(-1.05840165874163,-7.84302323090708,
100.810221403693));
#226150=CARTESIAN_POINT('Ctrl Pts',(-0.837855640838945,-7.86963948626871,
100.818554502827));
#226151=CARTESIAN_POINT('Ctrl Pts',(-0.579343375109531,-7.88984599264882,
100.828797216712));
#226152=CARTESIAN_POINT('Ctrl Pts',(-0.54218740047322,-7.89248638226708,
100.830279669501));
#226153=CARTESIAN_POINT('Ctrl Pts',(-0.494133034163816,-7.89556029914677,
100.832209090516));
#226154=CARTESIAN_POINT('Ctrl Pts',(-0.483250077759971,-7.89623386519002,
100.832646854621));
#226155=CARTESIAN_POINT('Ctrl Pts',(-0.465659242591914,-7.89728609134848,
100.83335570745));
#226156=CARTESIAN_POINT('Ctrl Pts',(-0.458952191503839,-7.8976787111398,
100.83362627694));
#226157=CARTESIAN_POINT('Ctrl Pts',(-0.446142465048931,-7.89841219864895,
100.834143593219));
#226158=CARTESIAN_POINT('Ctrl Pts',(-0.440039876332967,-7.89875453890491,
100.834390286114));
#226159=CARTESIAN_POINT('Ctrl Pts',(-0.426077969227882,-7.89952153699445,
100.83495523163));
#226160=CARTESIAN_POINT('Ctrl Pts',(-0.41821840786343,-7.89994153852388,
100.835273650924));
#226161=CARTESIAN_POINT('Ctrl Pts',(-0.397732550399217,-7.90100561047211,
100.836104616503));
#226162=CARTESIAN_POINT('Ctrl Pts',(-0.385105338999635,-7.90163114262455,
100.836617811781));
#226163=CARTESIAN_POINT('Ctrl Pts',(-0.305865402588814,-7.9053661700103,
100.839844348893));
#226164=CARTESIAN_POINT('Ctrl Pts',(-0.239218046762037,-7.90766352166946,
100.842585003055));
#226165=CARTESIAN_POINT('Ctrl Pts',(0.459836101678615,-7.92291456581624,
100.871565607677));
#226166=CARTESIAN_POINT('Ctrl Pts',(1.09160157046669,-7.86081892124048,
100.899484006929));
#226167=CARTESIAN_POINT('Ctrl Pts',(2.25074628292139,-7.60431839871772,
100.950136841868));
#226168=CARTESIAN_POINT('Ctrl Pts',(2.77816658765272,-7.42787622751898,
100.973003691385));
#226169=CARTESIAN_POINT('Ctrl Pts',(3.39813805748106,-7.14511353541758,
101.000747912315));
#226170=CARTESIAN_POINT('Ctrl Pts',(3.51219080823494,-7.08974652916456,
101.005891423149));
#226171=CARTESIAN_POINT('Ctrl Pts',(3.66024580239727,-7.01342328465121,
101.012619174058));
#226172=CARTESIAN_POINT('Ctrl Pts',(3.69548897919018,-6.9949172063736,101.014224541886));
#226173=CARTESIAN_POINT('Ctrl Pts',(3.75065085023848,-6.96541862836639,
101.016743410991));
#226174=CARTESIAN_POINT('Ctrl Pts',(3.77066430089724,-6.95460489185226,
101.017658580189));
#226175=CARTESIAN_POINT('Ctrl Pts',(3.80911675744417,-6.93361335072045,
101.019419435291));
#226176=CARTESIAN_POINT('Ctrl Pts',(3.82756230668795,-6.92344793870984,
101.020265234119));
#226177=CARTESIAN_POINT('Ctrl Pts',(3.87134428700345,-6.899091079969,101.022275505455));
#226178=CARTESIAN_POINT('Ctrl Pts',(3.89664362678815,-6.88483353252962,
101.023439299797));
#226179=CARTESIAN_POINT('Ctrl Pts',(3.96917665107978,-6.84342937539568,
101.026782242814));
#226180=CARTESIAN_POINT('Ctrl Pts',(4.01620929610038,-6.8159336732329,101.028957700803));
#226181=CARTESIAN_POINT('Ctrl Pts',(4.41605306701844,-6.57660575090095,
101.047522276427));
#226182=CARTESIAN_POINT('Ctrl Pts',(4.75212759784963,-6.33802527947089,
101.063562877318));
#226183=CARTESIAN_POINT('Ctrl Pts',(5.27529237619319,-5.90152608548048,
101.089937214565));
#226184=CARTESIAN_POINT('Ctrl Pts',(5.47348532135607,-5.71818824218199,
101.100325569543));
#226185=CARTESIAN_POINT('Ctrl Pts',(5.77156886456959,-5.41272220065917,
101.116923132515));
#226186=CARTESIAN_POINT('Ctrl Pts',(5.87784527551233,-5.29712208291849,
101.123061142573));
#226187=CARTESIAN_POINT('Ctrl Pts',(6.0331678807113,-5.11773905591105,101.132449264833));
#226188=CARTESIAN_POINT('Ctrl Pts',(6.08479795655919,-5.05624379065121,
101.135644736944));
#226189=CARTESIAN_POINT('Ctrl Pts',(6.14795112896188,-4.97865524500463,
101.139657082936));
#226190=CARTESIAN_POINT('Ctrl Pts',(6.16036237328176,-4.96328989257336,
101.140450745238));
#226191=CARTESIAN_POINT('Ctrl Pts',(6.17999134344313,-4.93880180905347,
101.141714323082));
#226192=CARTESIAN_POINT('Ctrl Pts',(6.18724674062582,-4.92970933055073,
101.142183209729));
#226193=CARTESIAN_POINT('Ctrl Pts',(6.20077459498975,-4.91267928632703,
101.143060940007));
#226194=CARTESIAN_POINT('Ctrl Pts',(6.20705193494342,-4.90474562280118,
101.143469645702));
#226195=CARTESIAN_POINT('Ctrl Pts',(6.2210079192751,-4.88703754527129,101.144381480321));
#226196=CARTESIAN_POINT('Ctrl Pts',(6.22867877464739,-4.87725703869315,
101.144884830793));
#226197=CARTESIAN_POINT('Ctrl Pts',(6.25170195895001,-4.84775907900361,
101.146402195357));
#226198=CARTESIAN_POINT('Ctrl Pts',(6.26698382969566,-4.82798706833381,
101.147418318326));
#226199=CARTESIAN_POINT('Ctrl Pts',(6.43621251127311,-4.60687808560089,
101.158769536299));
#226200=CARTESIAN_POINT('Ctrl Pts',(6.58048878899962,-4.3983312933797,101.169359868471));
#226201=CARTESIAN_POINT('Ctrl Pts',(6.90398041715958,-3.8790944094191,101.195095066997));
#226202=CARTESIAN_POINT('Ctrl Pts',(7.07257935107417,-3.56243545856963,
101.21026932914));
#226203=CARTESIAN_POINT('Ctrl Pts',(7.32623582837749,-2.99645991642265,
101.236157494663));
#226204=CARTESIAN_POINT('Ctrl Pts',(7.42140998372079,-2.75230513497619,
101.246962134732));
#226205=CARTESIAN_POINT('Ctrl Pts',(7.5241502452779,-2.44438481050283,101.260160327724));
#226206=CARTESIAN_POINT('Ctrl Pts',(7.54329149933407,-2.38466086942852,
101.26270112367));
#226207=CARTESIAN_POINT('Ctrl Pts',(7.56978994556906,-2.298468014344,101.266341761741));
#226208=CARTESIAN_POINT('Ctrl Pts',(7.57772250846246,-2.27217882773768,
101.267448693727));
#226209=CARTESIAN_POINT('Ctrl Pts',(7.59064366273581,-2.22853668732433,
101.269280671657));
#226210=CARTESIAN_POINT('Ctrl Pts',(7.59570999937156,-2.21120704343135,
101.270006660184));
#226211=CARTESIAN_POINT('Ctrl Pts',(7.60635096546553,-2.1743409877202,101.271548034982));
#226212=CARTESIAN_POINT('Ctrl Pts',(7.61190975628225,-2.15480013130315,
101.272363225454));
#226213=CARTESIAN_POINT('Ctrl Pts',(7.62530685042445,-2.10700642774324,
101.274352712888));
#226214=CARTESIAN_POINT('Ctrl Pts',(7.63306348906893,-2.07873096626329,
101.275526032187));
#226215=CARTESIAN_POINT('Ctrl Pts',(7.65942393061049,-1.9805013668055,101.279589835149));
#226216=CARTESIAN_POINT('Ctrl Pts',(7.67722477270231,-1.9103351857398,101.282470970352));
#226217=CARTESIAN_POINT('Ctrl Pts',(7.89729692987313,-0.990058558941479,
101.320006150638));
#226218=CARTESIAN_POINT('Ctrl Pts',(7.95833190498834,-0.112304059540934,
101.353170914501));
#226219=CARTESIAN_POINT('Ctrl Pts',(7.83927230885938,1.12522379101394,101.39965769443));
#226220=CARTESIAN_POINT('Ctrl Pts',(7.77820526873281,1.48990706853756,101.413416232623));
#226221=CARTESIAN_POINT('Ctrl Pts',(7.6634649773623,1.967236535514,101.432447323821));
#226222=CARTESIAN_POINT('Ctrl Pts',(7.6323142229527,2.08482450204241,101.43722284046));
#226223=CARTESIAN_POINT('Ctrl Pts',(7.59383411895244,2.21762967049555,101.442752665435));
#226224=CARTESIAN_POINT('Ctrl Pts',(7.58915199659253,2.23360022155599,101.44341992122));
#226225=CARTESIAN_POINT('Ctrl Pts',(7.58202083237059,2.25764307521548,101.444427985319));
#226226=CARTESIAN_POINT('Ctrl Pts',(7.57960920373895,2.26572647854178,101.444767509556));
#226227=CARTESIAN_POINT('Ctrl Pts',(7.57543042168483,2.27965176652856,101.445353470827));
#226228=CARTESIAN_POINT('Ctrl Pts',(7.57366942558344,2.28549550036317,101.445599691788));
#226229=CARTESIAN_POINT('Ctrl Pts',(7.57002011958822,2.29755491544697,101.446108481042));
#226230=CARTESIAN_POINT('Ctrl Pts',(7.56813091320335,2.30377031858125,101.446371081109));
#226231=CARTESIAN_POINT('Ctrl Pts',(7.56300261091426,2.32056781410366,101.44708179057));
#226232=CARTESIAN_POINT('Ctrl Pts',(7.55974896854687,2.33114542739003,101.447530426397));
#226233=CARTESIAN_POINT('Ctrl Pts',(7.54761972911092,2.37028521479327,101.449194632818));
#226234=CARTESIAN_POINT('Ctrl Pts',(7.53860443425562,2.3988036034688,101.450415399509));
#226235=CARTESIAN_POINT('Ctrl Pts',(7.42609301827079,2.74781570205716,101.465462074449));
#226236=CARTESIAN_POINT('Ctrl Pts',(7.30241715924047,3.06136647774508,101.480258866279));
#226237=CARTESIAN_POINT('Ctrl Pts',(6.99575079669148,3.71361144334974,101.512842903827));
#226238=CARTESIAN_POINT('Ctrl Pts',(6.80723407151014,4.04882794291579,101.530643011971));
#226239=CARTESIAN_POINT('Ctrl Pts',(6.4126718746228,4.64442568530208,101.56307557485));
#226240=CARTESIAN_POINT('Ctrl Pts',(6.21314911762186,4.90814182622734,101.577774236613));
#226241=CARTESIAN_POINT('Ctrl Pts',(5.90838107768859,5.26248225490896,101.597752204288));
#226242=CARTESIAN_POINT('Ctrl Pts',(5.81636918978122,5.36400394144666,101.603507992191));
#226243=CARTESIAN_POINT('Ctrl Pts',(5.67151050549033,5.5157216461343,101.612156834108));
#226244=CARTESIAN_POINT('Ctrl Pts',(5.6205321273874,5.56765980119811,101.615126656836));
#226245=CARTESIAN_POINT('Ctrl Pts',(5.56100348343034,5.62665825315384,101.618511347816));
#226246=CARTESIAN_POINT('Ctrl Pts',(5.55314723047137,5.63441200823218,101.618956401246));
#226247=CARTESIAN_POINT('Ctrl Pts',(5.53813369423426,5.64916776509272,101.619803798435));
#226248=CARTESIAN_POINT('Ctrl Pts',(5.53097929930793,5.65617266753311,101.62020626783));
#226249=CARTESIAN_POINT('Ctrl Pts',(5.51854470624005,5.6683012849824,101.620903457087));
#226250=CARTESIAN_POINT('Ctrl Pts',(5.51327063162163,5.67343124352167,101.621198446886));
#226251=CARTESIAN_POINT('Ctrl Pts',(5.50311989623314,5.68327708533786,101.621764818774));
#226252=CARTESIAN_POINT('Ctrl Pts',(5.49824431282853,5.68799406625638,101.622036248155));
#226253=CARTESIAN_POINT('Ctrl Pts',(5.48675101410622,5.69908490277653,101.622674662552));
#226254=CARTESIAN_POINT('Ctrl Pts',(5.48012824332055,5.70545351899075,101.623041421925));
#226255=CARTESIAN_POINT('Ctrl Pts',(5.4572292853893,5.7273970542991,101.624305703633));
#226256=CARTESIAN_POINT('Ctrl Pts',(5.44089760660451,5.74291404567405,101.625200739425));
#226257=CARTESIAN_POINT('Ctrl Pts',(5.25713706375049,5.91602042080533,101.635197600733));
#226258=CARTESIAN_POINT('Ctrl Pts',(5.08297426266895,6.06631441966097,101.643983652174));
#226259=CARTESIAN_POINT('Ctrl Pts',(4.78185207503718,6.3040815045025,101.658187464135));
#226260=CARTESIAN_POINT('Ctrl Pts',(4.65844841703589,6.39581219610273,101.663754411411));
#226261=CARTESIAN_POINT('Ctrl Pts',(4.02438910800785,6.83903988745184,101.691282926015));
#226262=CARTESIAN_POINT('Ctrl Pts',(3.47638624463482,7.1332223252011,101.711495174422));
#226263=CARTESIAN_POINT('Ctrl Pts',(2.7248463785409,7.4292964907886,101.739868734176));
#226264=CARTESIAN_POINT('Ctrl Pts',(2.54761520587758,7.49192131832584,101.746619168375));
#226265=CARTESIAN_POINT('Ctrl Pts',(2.27076744670681,7.57878564650835,101.75746834213));
#226266=CARTESIAN_POINT('Ctrl Pts',(2.1726230989006,7.60750183158416,101.761372343206));
#226267=CARTESIAN_POINT('Ctrl Pts',(2.02577142320548,7.64739589355367,101.76733383238));
#226268=CARTESIAN_POINT('Ctrl Pts',(1.97746776458933,7.66002838451151,101.769313861859));
#226269=CARTESIAN_POINT('Ctrl Pts',(1.92041884334143,7.67437239450965,101.771678025428));
#226270=CARTESIAN_POINT('Ctrl Pts',(1.9117853178829,7.67652767080179,101.772036497268));
#226271=CARTESIAN_POINT('Ctrl Pts',(1.89855072150598,7.67980784871366,101.772587089985));
#226272=CARTESIAN_POINT('Ctrl Pts',(1.89395222256896,7.68094319818439,101.772778598846));
#226273=CARTESIAN_POINT('Ctrl Pts',(1.88556538001958,7.68300588371648,101.77312824505));
#226274=CARTESIAN_POINT('Ctrl Pts',(1.88177736226349,7.68393455010604,101.773286303813));
#226275=CARTESIAN_POINT('Ctrl Pts',(1.87416220147529,7.68579550591782,101.773604331513));
#226276=CARTESIAN_POINT('Ctrl Pts',(1.87033504567331,7.68672773896978,101.773764303751));
#226277=CARTESIAN_POINT('Ctrl Pts',(1.85944752238259,7.68937115039387,101.774219798406));
#226278=CARTESIAN_POINT('Ctrl Pts',(1.85238550832352,7.69107545827402,101.774515731048));
#226279=CARTESIAN_POINT('Ctrl Pts',(1.8215613895581,7.69846946576185,101.775809556101));
#226280=CARTESIAN_POINT('Ctrl Pts',(1.79777575019328,7.70405869149959,101.776813538316));
#226281=CARTESIAN_POINT('Ctrl Pts',(1.38538859640253,7.79894899712448,101.794311873737));
#226282=CARTESIAN_POINT('Ctrl Pts',(0.990641383771469,7.85884708564601,
101.812442911936));
#226283=CARTESIAN_POINT('Ctrl Pts',(0.131139386026713,7.92346792267918,
101.852333732414));
#226284=CARTESIAN_POINT('Ctrl Pts',(-0.333022073000432,7.91755571718185,
101.874095304605));
#226285=CARTESIAN_POINT('Ctrl Pts',(-0.97823645412795,7.85246838059121,
101.903130740182));
#226286=CARTESIAN_POINT('Ctrl Pts',(-1.16176184292804,7.82742113503187,
101.911260611669));
#226287=CARTESIAN_POINT('Ctrl Pts',(-1.51976401526566,7.76569122562137,
101.926815803433));
#226288=CARTESIAN_POINT('Ctrl Pts',(-1.69421504182749,7.72950736660577,
101.934251806786));
#226289=CARTESIAN_POINT('Ctrl Pts',(-1.89945574223054,7.67965386974466,
101.942829218535));
#226290=CARTESIAN_POINT('Ctrl Pts',(-1.93155769537997,7.67164262610024,
101.944165870249));
#226291=CARTESIAN_POINT('Ctrl Pts',(-1.97427337694746,7.6606975423293,101.945937963322));
#226292=CARTESIAN_POINT('Ctrl Pts',(-1.98493234237679,7.65794266102388,
101.946379618963));
#226293=CARTESIAN_POINT('Ctrl Pts',(-2.00247953939511,7.65336837288868,
101.947105806372));
#226294=CARTESIAN_POINT('Ctrl Pts',(-2.00937110773991,7.65156189993774,
101.947390787998));
#226295=CARTESIAN_POINT('Ctrl Pts',(-2.02275958873118,7.64803306885342,
101.947943996919));
#226296=CARTESIAN_POINT('Ctrl Pts',(-2.02925676373576,7.64631173594315,
101.948212259644));
#226297=CARTESIAN_POINT('Ctrl Pts',(-2.04430800678826,7.64230359084514,
101.94883325338));
#226298=CARTESIAN_POINT('Ctrl Pts',(-2.05286045293176,7.64001069127248,
101.949185771736));
#226299=CARTESIAN_POINT('Ctrl Pts',(-2.0804534559024,7.63256336544137,101.950322009204));
#226300=CARTESIAN_POINT('Ctrl Pts',(-2.0994786624646,7.62735206105405,101.951103741579));
#226301=CARTESIAN_POINT('Ctrl Pts',(-2.27618076738009,7.57823933329035,
101.958348792452));
#226302=CARTESIAN_POINT('Ctrl Pts',(-2.43248409934646,7.52952425532047,
101.964641152945));
#226303=CARTESIAN_POINT('Ctrl Pts',(-3.2912235966148,7.23234563404386,101.998703255845));
#226304=CARTESIAN_POINT('Ctrl Pts',(-3.95724804379451,6.89050746818473,
102.022733455498));
#226305=CARTESIAN_POINT('Ctrl Pts',(-4.72921261343966,6.34496573219549,
102.055286368333));
#226306=CARTESIAN_POINT('Ctrl Pts',(-4.88833526020827,6.223199657322,102.062321926151));
#226307=CARTESIAN_POINT('Ctrl Pts',(-5.1415302443183,6.01373873494089,102.074364761423));
#226308=CARTESIAN_POINT('Ctrl Pts',(-5.23839306547455,5.92955496332986,
102.079191043471));
#226309=CARTESIAN_POINT('Ctrl Pts',(-5.37451684279496,5.80531005160545,
102.086367726004));
#226310=CARTESIAN_POINT('Ctrl Pts',(-5.41546947915409,5.76712633004835,
102.088580255351));
#226311=CARTESIAN_POINT('Ctrl Pts',(-5.46231953483101,5.72250488563383,
102.091178700688));
#226312=CARTESIAN_POINT('Ctrl Pts',(-5.46861677578066,5.71648733271724,
102.091529388404));
#226313=CARTESIAN_POINT('Ctrl Pts',(-5.4781685914276,5.7073295276684,102.092063511409));
#226314=CARTESIAN_POINT('Ctrl Pts',(-5.48143043629186,5.70419686066637,
102.0922462988));
#226315=CARTESIAN_POINT('Ctrl Pts',(-5.48736314812334,5.69848931245899,
102.092579464802));
#226316=CARTESIAN_POINT('Ctrl Pts',(-5.49003489558143,5.69591534424395,
102.09272976533));
#226317=CARTESIAN_POINT('Ctrl Pts',(-5.49579626490353,5.69035700698463,
102.093054437749));
#226318=CARTESIAN_POINT('Ctrl Pts',(-5.49888526710921,5.68737200043111,
102.093228863761));
#226319=CARTESIAN_POINT('Ctrl Pts',(-5.50722485609883,5.67930002996268,
102.093700716961));
#226320=CARTESIAN_POINT('Ctrl Pts',(-5.5124708136108,5.67420831256058,102.093998544958));
#226321=CARTESIAN_POINT('Ctrl Pts',(-5.53680386870649,5.65052509786252,
102.095384675183));
#226322=CARTESIAN_POINT('Ctrl Pts',(-5.55580380764055,5.63184472254529,
102.09648038816));
#226323=CARTESIAN_POINT('Ctrl Pts',(-5.86027209043677,5.32945720042755,
102.114249690311));
#226324=CARTESIAN_POINT('Ctrl Pts',(-6.12374840860168,5.0244940981396,102.132608310082));
#226325=CARTESIAN_POINT('Ctrl Pts',(-6.68695182748333,4.2621685154702,102.176815405996));
#226326=CARTESIAN_POINT('Ctrl Pts',(-6.96484615878175,3.79109631327008,
102.202805037158));
#226327=CARTESIAN_POINT('Ctrl Pts',(-7.35332848749448,2.94319135485258,
102.244701423262));
#226328=CARTESIAN_POINT('Ctrl Pts',(-7.48854966190747,2.5798251595956,102.261321006705));
#226329=CARTESIAN_POINT('Ctrl Pts',(-7.60270692669792,2.18706257386873,
102.277880734497));
#226330=CARTESIAN_POINT('Ctrl Pts',(-7.60869907336325,2.16612412768465,
102.278759559651));
#226331=CARTESIAN_POINT('Ctrl Pts',(-7.61719646555212,2.13596122620519,
102.280019879222));
#226332=CARTESIAN_POINT('Ctrl Pts',(-7.61977155152352,2.12675665230545,
102.280403722566));
#226333=CARTESIAN_POINT('Ctrl Pts',(-7.62421407805264,2.11076532061459,
102.281069272828));
#226334=CARTESIAN_POINT('Ctrl Pts',(-7.62608915083823,2.1039807058259,102.28135123569));
#226335=CARTESIAN_POINT('Ctrl Pts',(-7.62967866455126,2.09092485353419,
102.281893042218));
#226336=CARTESIAN_POINT('Ctrl Pts',(-7.63139443420316,2.08465398982704,
102.282152930205));
#226337=CARTESIAN_POINT('Ctrl Pts',(-7.63542025553442,2.06986868018247,
102.282764872836));
#226338=CARTESIAN_POINT('Ctrl Pts',(-7.63772380090847,2.06135246223299,
102.283116709702));
#226339=CARTESIAN_POINT('Ctrl Pts',(-7.64564752684936,2.031862782375,102.284332845349));
#226340=CARTESIAN_POINT('Ctrl Pts',(-7.6511956249906,2.01086995830706,102.2851947386));
#226341=CARTESIAN_POINT('Ctrl Pts',(-7.71375122810141,1.77016551230626,
102.295033894612));
#226342=CARTESIAN_POINT('Ctrl Pts',(-7.76136584925352,1.54811303075789,
102.303693074474));
#226343=CARTESIAN_POINT('Ctrl Pts',(-7.8121259399081,1.24916702187163,102.314913841405));
#226344=CARTESIAN_POINT('Ctrl Pts',(-7.82379824227897,1.17384467408581,
102.317704887032));
#226345=CARTESIAN_POINT('Ctrl Pts',(-7.83830899652329,1.07034280412142,
102.32149699441));
#226346=CARTESIAN_POINT('Ctrl Pts',(-7.84208721696192,1.04230021540008,
102.322520101876));
#226347=CARTESIAN_POINT('Ctrl Pts',(-7.88949208347646,0.675596217674615,
102.335845939355));
#226348=CARTESIAN_POINT('Ctrl Pts',(-7.91129923408663,0.33446853751554,
102.34763225072));
#226349=CARTESIAN_POINT('Ctrl Pts',(-7.9105135010674,-0.552979556538924,
102.378243440295));
#226350=CARTESIAN_POINT('Ctrl Pts',(-7.85351089883097,-1.0974420703393,
102.39697895592));
#226351=CARTESIAN_POINT('Ctrl Pts',(-7.73311163939765,-1.668631607545,102.420065163984));
#226352=CARTESIAN_POINT('Ctrl Pts',(-7.72505838799676,-1.7055262832714,
102.421570447011));
#226353=CARTESIAN_POINT('Ctrl Pts',(-7.71427584963855,-1.75328104778071,
102.423536066676));
#226354=CARTESIAN_POINT('Ctrl Pts',(-7.7117871457801,-1.76419537843943,
102.423986479541));
#226355=CARTESIAN_POINT('Ctrl Pts',(-7.70778755054815,-1.78156561397224,
102.424705148206));
#226356=CARTESIAN_POINT('Ctrl Pts',(-7.7062916890954,-1.78802498962012,
102.424972799758));
#226357=CARTESIAN_POINT('Ctrl Pts',(-7.70347037188664,-1.80013859373368,
102.425475491031));
#226358=CARTESIAN_POINT('Ctrl Pts',(-7.70214680622793,-1.80579326122002,
102.425710455827));
#226359=CARTESIAN_POINT('Ctrl Pts',(-7.69914628586926,-1.81854906648088,
102.426241176095));
#226360=CARTESIAN_POINT('Ctrl Pts',(-7.69746573235635,-1.82564934671549,
102.426537071923));
#226361=CARTESIAN_POINT('Ctrl Pts',(-7.69246899130551,-1.84663085199819,
102.427412855211));
#226362=CARTESIAN_POINT('Ctrl Pts',(-7.68912507009595,-1.86050539877712,
102.427993806308));
#226363=CARTESIAN_POINT('Ctrl Pts',(-7.66248115917167,-1.96975713953592,
102.43258236548));
#226364=CARTESIAN_POINT('Ctrl Pts',(-7.63744550460029,-2.06469996177659,
102.43665402664));
#226365=CARTESIAN_POINT('Ctrl Pts',(-7.54015105154648,-2.40764700267757,
102.451620788147));
#226366=CARTESIAN_POINT('Ctrl Pts',(-7.45752590461562,-2.65253475415538,
102.462800669732));
#226367=CARTESIAN_POINT('Ctrl Pts',(-7.15964538621602,-3.41069841602233,
102.498360784226));
#226368=CARTESIAN_POINT('Ctrl Pts',(-6.90215527302022,-3.90559883129204,
102.52287856345));
#226369=CARTESIAN_POINT('Ctrl Pts',(-6.4477167670995,-4.59149807003878,
102.557615149195));
#226370=CARTESIAN_POINT('Ctrl Pts',(-6.28943189325535,-4.80603398931511,
102.568630219762));
#226371=CARTESIAN_POINT('Ctrl Pts',(-6.09693839310463,-5.04109710498091,
102.580928359718));
#226372=CARTESIAN_POINT('Ctrl Pts',(-6.07305472440847,-5.06984458690464,
102.582436691265));
#226373=CARTESIAN_POINT('Ctrl Pts',(-6.03805953313594,-5.11136425810804,
102.584621508952));
#226374=CARTESIAN_POINT('Ctrl Pts',(-6.02710936711312,-5.1242716735365,
102.58530160994));
#226375=CARTESIAN_POINT('Ctrl Pts',(-6.00773710391849,-5.14695856355616,
102.586498576701));
#226376=CARTESIAN_POINT('Ctrl Pts',(-5.9993323533238,-5.15675274570047,
102.587015842585));
#226377=CARTESIAN_POINT('Ctrl Pts',(-5.98191918240937,-5.17694438367749,
102.58808331457));
#226378=CARTESIAN_POINT('Ctrl Pts',(-5.97290753010803,-5.1873389994071,
102.588633441824));
#226379=CARTESIAN_POINT('Ctrl Pts',(-5.94976870746713,-5.21388855685571,
102.590040082865));
#226380=CARTESIAN_POINT('Ctrl Pts',(-5.93560280761871,-5.2300096435207,
102.590895658928));
#226381=CARTESIAN_POINT('Ctrl Pts',(-5.87715900307138,-5.29597660193595,
102.594402651206));
#226382=CARTESIAN_POINT('Ctrl Pts',(-5.83231708253384,-5.34531979689645,
102.597040002323));
#226383=CARTESIAN_POINT('Ctrl Pts',(-5.53355388377572,-5.66583715557513,
102.614267865631));
#226384=CARTESIAN_POINT('Ctrl Pts',(-5.2614189859492,-5.91941065421507,
102.628324531081));
#226385=CARTESIAN_POINT('Ctrl Pts',(-4.42862584826985,-6.59242769396648,
102.667871738866));
#226386=CARTESIAN_POINT('Ctrl Pts',(-3.82900579519542,-6.95782357448853,
102.692098243892));
#226387=CARTESIAN_POINT('Ctrl Pts',(-3.16128979765534,-7.25197236569389,
102.721036984712));
#226388=CARTESIAN_POINT('Ctrl Pts',(-3.13323032448645,-7.26413959635661,
102.722257067898));
#226389=CARTESIAN_POINT('Ctrl Pts',(-3.09637381157708,-7.27986814847662,
102.723865709839));
#226390=CARTESIAN_POINT('Ctrl Pts',(-3.08763967894946,-7.28357688584858,
102.724247363525));
#226391=CARTESIAN_POINT('Ctrl Pts',(-3.07414708221909,-7.2892775586892,
102.724837659927));
#226392=CARTESIAN_POINT('Ctrl Pts',(-3.06939328761387,-7.29128057727119,
102.725045773201));
#226393=CARTESIAN_POINT('Ctrl Pts',(-3.0603934733858,-7.29506230135016,
102.725440034084));
#226394=CARTESIAN_POINT('Ctrl Pts',(-3.05614785268475,-7.29684195353759,
102.725626135838));
#226395=CARTESIAN_POINT('Ctrl Pts',(-3.04635696004198,-7.30093599331547,
102.726055568892));
#226396=CARTESIAN_POINT('Ctrl Pts',(-3.04081060417867,-7.30324776902099,
102.726299027341));
#226397=CARTESIAN_POINT('Ctrl Pts',(-3.02534208974715,-7.30967452233391,
102.72697857166));
#226398=CARTESIAN_POINT('Ctrl Pts',(-3.01541420219895,-7.3137756029198,
102.727415342708));
#226399=CARTESIAN_POINT('Ctrl Pts',(-2.95853363056975,-7.33713672102073,
102.729921536307));
#226400=CARTESIAN_POINT('Ctrl Pts',(-2.91140783761361,-7.3559636180685,
102.732013196208));
#226401=CARTESIAN_POINT('Ctrl Pts',(-2.77177352063081,-7.41019588857052,
102.738257830478));
#226402=CARTESIAN_POINT('Ctrl Pts',(-2.67878220428987,-7.44431703637101,
102.742474355842));
#226403=CARTESIAN_POINT('Ctrl Pts',(-2.48824741424025,-7.51019737599392,
102.751199157523));
#226404=CARTESIAN_POINT('Ctrl Pts',(-2.39067677561764,-7.54182360045362,
102.755711664976));
#226405=CARTESIAN_POINT('Ctrl Pts',(-1.91492511453467,-7.68587230974907,
102.777849352505));
#226406=CARTESIAN_POINT('Ctrl Pts',(-1.52931476610035,-7.77179216328433,
102.796177584676));
#226407=CARTESIAN_POINT('Ctrl Pts',(-0.72251106458374,-7.88916742361963,
102.833709107039));
#226408=CARTESIAN_POINT('Ctrl Pts',(-0.301906919710609,-7.91643153467123,
102.852816447499));
#226409=CARTESIAN_POINT('Ctrl Pts',(0.125923726172375,-7.91000086071323,
102.871329541374));
#226410=CARTESIAN_POINT('Ctrl Pts',(0.132951404656118,-7.90988586046578,
102.871633403476));
#226411=CARTESIAN_POINT('Ctrl Pts',(0.16882141587529,-7.90925106941212,
102.873183120322));
#226412=CARTESIAN_POINT('Ctrl Pts',(0.197661070810024,-7.90858288642949,
102.874425048364));
#226413=CARTESIAN_POINT('Ctrl Pts',(0.439437232381221,-7.90165785306008,
102.884802367676));
#226414=CARTESIAN_POINT('Ctrl Pts',(0.652053434278941,-7.88695994251887,
102.893701513969));
#226415=CARTESIAN_POINT('Ctrl Pts',(0.884524536447429,-7.86142295289256,
102.903187969697));
#226416=CARTESIAN_POINT('Ctrl Pts',(0.905211740432468,-7.85906776997854,
102.904030055333));
#226417=CARTESIAN_POINT('Ctrl Pts',(0.935922963434576,-7.85544850883296,
102.905277094851));
#226418=CARTESIAN_POINT('Ctrl Pts',(0.945954169452295,-7.85424686259701,
102.905683926892));
#226419=CARTESIAN_POINT('Ctrl Pts',(0.963125790518057,-7.85215648635099,
102.906379519066));
#226420=CARTESIAN_POINT('Ctrl Pts',(0.970267334577204,-7.85127722566981,
102.906668564181));
#226421=CARTESIAN_POINT('Ctrl Pts',(0.984160883865129,-7.84954741799592,
102.907230411359));
#226422=CARTESIAN_POINT('Ctrl Pts',(0.990913010292175,-7.84869789959059,
102.907503244188));
#226423=CARTESIAN_POINT('Ctrl Pts',(1.00706316344464,-7.84664479609154,
102.90815530043));
#226424=CARTESIAN_POINT('Ctrl Pts',(1.01646014983422,-7.84543303685376,
102.908534276978));
#226425=CARTESIAN_POINT('Ctrl Pts',(1.04463714455635,-7.84174808574261,
102.9096693829));
#226426=CARTESIAN_POINT('Ctrl Pts',(1.06341052847631,-7.83922431482134,
102.910423985417));
#226427=CARTESIAN_POINT('Ctrl Pts',(1.22748154563073,-7.81656745330419,
102.917004399839));
#226428=CARTESIAN_POINT('Ctrl Pts',(1.37220611662675,-7.79246371547353,
102.922708845393));
#226429=CARTESIAN_POINT('Ctrl Pts',(1.8317545964935,-7.70272548245994,102.940555523329));
#226430=CARTESIAN_POINT('Ctrl Pts',(2.1432894220011,-7.62191804575855,102.95223809563));
#226431=CARTESIAN_POINT('Ctrl Pts',(2.74573158978619,-7.42578107943707,
102.974626528167));
#226432=CARTESIAN_POINT('Ctrl Pts',(3.03643651033686,-7.31172507076696,
102.98533413929));
#226433=CARTESIAN_POINT('Ctrl Pts',(3.79388794695346,-6.96155922536145,
103.014160078732));
#226434=CARTESIAN_POINT('Ctrl Pts',(4.24524168261052,-6.69587950753181,
103.032342864703));
#226435=CARTESIAN_POINT('Ctrl Pts',(4.69483116159098,-6.36739048500372,
103.054361119655));
#226436=CARTESIAN_POINT('Ctrl Pts',(4.72243767803881,-6.34694285089252,
103.055728952403));
#226437=CARTESIAN_POINT('Ctrl Pts',(4.75854707536771,-6.31983127848204,
103.057538089855));
#226438=CARTESIAN_POINT('Ctrl Pts',(4.76717099645756,-6.31332862649009,
103.057971674058));
#226439=CARTESIAN_POINT('Ctrl Pts',(4.78109212463166,-6.30278696051444,
103.058674000708));
#226440=CARTESIAN_POINT('Ctrl Pts',(4.7863976112701,-6.29875886824868,103.058942233816));
#226441=CARTESIAN_POINT('Ctrl Pts',(4.7964444304158,-6.29111098369043,103.059451248374));
#226442=CARTESIAN_POINT('Ctrl Pts',(4.80118677099405,-6.28749251872111,
103.059691968893));
#226443=CARTESIAN_POINT('Ctrl Pts',(4.81195562227484,-6.27925646317358,
103.060239617743));
#226444=CARTESIAN_POINT('Ctrl Pts',(4.81797958298133,-6.27463555742869,
103.060546695806));
#226445=CARTESIAN_POINT('Ctrl Pts',(4.83582418240097,-6.26090633742654,
103.061458490809));
#226446=CARTESIAN_POINT('Ctrl Pts',(4.84762567761959,-6.25177326646535,
103.062064304693));
#226447=CARTESIAN_POINT('Ctrl Pts',(4.94317798467285,-6.17739296274878,
103.06699169395));
#226448=CARTESIAN_POINT('Ctrl Pts',(5.02563166480635,-6.11050061117071,
103.071383094474));
#226449=CARTESIAN_POINT('Ctrl Pts',(5.33688247869962,-5.84742945330845,
103.088435848353));
#226450=CARTESIAN_POINT('Ctrl Pts',(5.55574343514753,-5.639898290658,103.101430035675));
#226451=CARTESIAN_POINT('Ctrl Pts',(5.94368682903356,-5.22748967347134,
103.125889304387));
#226452=CARTESIAN_POINT('Ctrl Pts',(6.11534900139186,-5.02559165327295,
103.137335662844));
#226453=CARTESIAN_POINT('Ctrl Pts',(6.65909162905771,-4.31686756192522,
103.175527248456));
#226454=CARTESIAN_POINT('Ctrl Pts',(6.9808563308753,-3.77445905809207,103.20138271375));
#226455=CARTESIAN_POINT('Ctrl Pts',(7.27020421796336,-3.12019341722742,
103.230430669976));
#226456=CARTESIAN_POINT('Ctrl Pts',(7.30404812498197,-3.04012458097429,
103.233950380115));
#226457=CARTESIAN_POINT('Ctrl Pts',(7.34861079439945,-2.92965476510445,
103.238758389564));
#226458=CARTESIAN_POINT('Ctrl Pts',(7.3604733735777,-2.89972229282019,103.240056375177));
#226459=CARTESIAN_POINT('Ctrl Pts',(7.38051901876886,-2.84822609964404,
103.242281305089));
#226460=CARTESIAN_POINT('Ctrl Pts',(7.38879111212421,-2.82669750869779,
103.243209035795));
#226461=CARTESIAN_POINT('Ctrl Pts',(7.40565626201868,-2.78222511138245,
103.245120509821));
#226462=CARTESIAN_POINT('Ctrl Pts',(7.41423711864489,-2.75927693318314,
103.246104131693));
#226463=CARTESIAN_POINT('Ctrl Pts',(7.43402135517971,-2.70560838323863,
103.24839822615));
#226464=CARTESIAN_POINT('Ctrl Pts',(7.44514115552639,-2.67485764415331,
103.24970789585));
#226465=CARTESIAN_POINT('Ctrl Pts',(7.48064082204575,-2.57475018702315,
103.253956132854));
#226466=CARTESIAN_POINT('Ctrl Pts',(7.50424472473221,-2.50512212377008,
103.256887098778));
#226467=CARTESIAN_POINT('Ctrl Pts',(7.7042404958447,-1.88695577744984,103.282707785775));
#226468=CARTESIAN_POINT('Ctrl Pts',(7.82118269288217,-1.32099886795408,
103.304831832444));
#226469=CARTESIAN_POINT('Ctrl Pts',(7.904203045034,-0.446146461133101,103.338859961155));
#226470=CARTESIAN_POINT('Ctrl Pts',(7.91548219648333,-0.143540911452603,
103.350627064907));
#226471=CARTESIAN_POINT('Ctrl Pts',(7.908864396144,0.185750328063237,103.363805937198));
#226472=CARTESIAN_POINT('Ctrl Pts',(7.9081897613279,0.212541544195681,103.36488092154));
#226473=CARTESIAN_POINT('Ctrl Pts',(7.90698389329729,0.25238321569165,103.366484036457));
#226474=CARTESIAN_POINT('Ctrl Pts',(7.90655645220347,0.265436702617317,
103.367009988176));
#226475=CARTESIAN_POINT('Ctrl Pts',(7.90573637282956,0.288718145752481,
103.367949379758));
#226476=CARTESIAN_POINT('Ctrl Pts',(7.90535620580901,0.298946521843469,
103.368362547875));
#226477=CARTESIAN_POINT('Ctrl Pts',(7.90452502957055,0.320198015622069,
103.369221973725));
#226478=CARTESIAN_POINT('Ctrl Pts',(7.90407081016079,0.331220982650436,
103.369668302186));
#226479=CARTESIAN_POINT('Ctrl Pts',(7.90283056328759,0.35986264610135,103.370829508655));
#226480=CARTESIAN_POINT('Ctrl Pts',(7.90200868009032,0.377479605379283,
103.37154522002));
#226481=CARTESIAN_POINT('Ctrl Pts',(7.89760783332676,0.465488226258899,
103.375128140699));
#226482=CARTESIAN_POINT('Ctrl Pts',(7.89314720800499,0.535831792455592,
103.3780154227));
#226483=CARTESIAN_POINT('Ctrl Pts',(7.83444006368487,1.29983590891204,103.409589995928));
#226484=CARTESIAN_POINT('Ctrl Pts',(7.68984714882252,1.98351866001974,103.4394810665));
#226485=CARTESIAN_POINT('Ctrl Pts',(7.40537194881248,2.78728781814451,103.474607160953));
#226486=CARTESIAN_POINT('Ctrl Pts',(7.34867270343761,2.93351631877009,103.481012144068));
#226487=CARTESIAN_POINT('Ctrl Pts',(7.27223360981663,3.11450032075621,103.48896782148));
#226488=CARTESIAN_POINT('Ctrl Pts',(7.25652831350302,3.15091903765182,103.490570228675));
#226489=CARTESIAN_POINT('Ctrl Pts',(7.2312306852643,3.20838881916228,103.493101647804));
#226490=CARTESIAN_POINT('Ctrl Pts',(7.22181878324293,3.22951846331162,103.494032961595));
#226491=CARTESIAN_POINT('Ctrl Pts',(7.20411082473884,3.26880816513423,103.495765916297));
#226492=CARTESIAN_POINT('Ctrl Pts',(7.19583843590211,3.28697867391424,103.496567851599));
#226493=CARTESIAN_POINT('Ctrl Pts',(7.17729775115692,3.32729830369259,103.498348478842));
#226494=CARTESIAN_POINT('Ctrl Pts',(7.16699552563286,3.34943161612485,103.499326732497));
#226495=CARTESIAN_POINT('Ctrl Pts',(7.13662992162976,3.41388753089522,103.502178076006));
#226496=CARTESIAN_POINT('Ctrl Pts',(7.11629289081814,3.45608018395123,103.504047718402));
#226497=CARTESIAN_POINT('Ctrl Pts',(6.93719760317999,3.81935996949329,103.520177726733));
#226498=CARTESIAN_POINT('Ctrl Pts',(6.75717207857305,4.129510274642,103.534193049738));
#226499=CARTESIAN_POINT('Ctrl Pts',(6.35956145314151,4.7184849148636,103.561776832244));
#226500=CARTESIAN_POINT('Ctrl Pts',(6.14307256667544,4.99707831118731,103.575232829187));
#226501=CARTESIAN_POINT('Ctrl Pts',(5.59679641021371,5.61069116482583,103.606197225456));
#226502=CARTESIAN_POINT('Ctrl Pts',(5.25432973085988,5.93262048307298,103.623481171852));
#226503=CARTESIAN_POINT('Ctrl Pts',(4.71425526879374,6.35665394662141,103.649616406839));
#226504=CARTESIAN_POINT('Ctrl Pts',(4.53767483433895,6.4838840279869,103.65802161916));
#226505=CARTESIAN_POINT('Ctrl Pts',(4.33918359116201,6.61481796087853,103.667514113218));
#226506=CARTESIAN_POINT('Ctrl Pts',(4.32224083443446,6.62590107491069,103.668324733923));
#226507=CARTESIAN_POINT('Ctrl Pts',(4.29754825961059,6.6419187257959,103.669506893814));
#226508=CARTESIAN_POINT('Ctrl Pts',(4.28983202950851,6.64690503629937,103.669876415455));
#226509=CARTESIAN_POINT('Ctrl Pts',(4.27642493363103,6.65553577518509,103.670518675778));
#226510=CARTESIAN_POINT('Ctrl Pts',(4.27073804346122,6.65918637909803,103.670791168682));
#226511=CARTESIAN_POINT('Ctrl Pts',(4.25974931508833,6.6662205432022,103.671317841451));
#226512=CARTESIAN_POINT('Ctrl Pts',(4.25444810441001,6.6696050771112,103.671571981747));
#226513=CARTESIAN_POINT('Ctrl Pts',(4.24075718700752,6.67832301654717,103.672228495657));
#226514=CARTESIAN_POINT('Ctrl Pts',(4.2323614664137,6.68364692731906,103.672631256667));
#226515=CARTESIAN_POINT('Ctrl Pts',(4.20290690172965,6.70224695950866,103.67404489975));
#226516=CARTESIAN_POINT('Ctrl Pts',(4.181795570517,6.71543941375966,103.675059267274));
#226517=CARTESIAN_POINT('Ctrl Pts',(3.89647060903419,6.89187157801256,103.688788146536));
#226518=CARTESIAN_POINT('Ctrl Pts',(3.62298749997597,7.03947928388921,103.702319116291));
#226519=CARTESIAN_POINT('Ctrl Pts',(2.65082037431713,7.49251929629156,103.750547533893));
#226520=CARTESIAN_POINT('Ctrl Pts',(1.91701530476906,7.71297932275493,103.786442346441));
#226521=CARTESIAN_POINT('Ctrl Pts',(0.978372810038053,7.85248706292999,
103.826875259803));
#226522=CARTESIAN_POINT('Ctrl Pts',(0.792811334313815,7.87338699311333,
103.834639802152));
#226523=CARTESIAN_POINT('Ctrl Pts',(0.585031038117041,7.88936822143292,
103.843080299582));
#226524=CARTESIAN_POINT('Ctrl Pts',(0.563379827306682,7.89094388706255,
103.843956782869));
#226525=CARTESIAN_POINT('Ctrl Pts',(0.532928486811197,7.89303401255125,
103.845185274643));
#226526=CARTESIAN_POINT('Ctrl Pts',(0.524133660699422,7.89362290723916,
103.845539585659));
#226527=CARTESIAN_POINT('Ctrl Pts',(0.5079917610494,7.89467665998413,103.846188974694));
#226528=CARTESIAN_POINT('Ctrl Pts',(0.500644992513982,7.89514596361971,
103.84648419015));
#226529=CARTESIAN_POINT('Ctrl Pts',(0.485749697261641,7.896076584249,103.847082030624));
#226530=CARTESIAN_POINT('Ctrl Pts',(0.478201142059657,7.89653733359465,
103.847384637752));
#226531=CARTESIAN_POINT('Ctrl Pts',(0.459607071743803,7.89764552013317,
103.848129147004));
#226532=CARTESIAN_POINT('Ctrl Pts',(0.448560822010508,7.89828061113949,
103.84857066579));
#226533=CARTESIAN_POINT('Ctrl Pts',(0.408231545195871,7.90051441705673,
103.850179814796));
#226534=CARTESIAN_POINT('Ctrl Pts',(0.378940856210546,7.90197348132454,
103.85134310757));
#226535=CARTESIAN_POINT('Ctrl Pts',(-0.0401653747111206,7.92051484063087,
103.867911896506));
#226536=CARTESIAN_POINT('Ctrl Pts',(-0.430730966989419,7.90889891653234,
103.88237186308));
#226537=CARTESIAN_POINT('Ctrl Pts',(-0.923458946856395,7.85762051124463,
103.899938980386));
#226538=CARTESIAN_POINT('Ctrl Pts',(-1.02781323110723,7.84465276764938,
103.903623191188));
#226539=CARTESIAN_POINT('Ctrl Pts',(-1.2132892001396,7.81783962422734,103.910131911088));
#226540=CARTESIAN_POINT('Ctrl Pts',(-1.29451108939239,7.8048016182882,103.912968601785));
#226541=CARTESIAN_POINT('Ctrl Pts',(-1.44239887394455,7.77869007864867,
103.91812294844));
#226542=CARTESIAN_POINT('Ctrl Pts',(-1.50912769967523,7.76602005559466,
103.92044467713));
#226543=CARTESIAN_POINT('Ctrl Pts',(-1.63230384283162,7.74098464326481,
103.924731817012));
#226544=CARTESIAN_POINT('Ctrl Pts',(-1.68879467670604,7.72885707215091,
103.926698537813));
#226545=CARTESIAN_POINT('Ctrl Pts',(-1.79400936284059,7.70506073934629,
103.930368439178));
#226546=CARTESIAN_POINT('Ctrl Pts',(-1.84276499066233,7.69354585219021,
103.932071816118));
#226547=CARTESIAN_POINT('Ctrl Pts',(-1.93416419386295,7.67104092030055,
103.935274266467));
#226548=CARTESIAN_POINT('Ctrl Pts',(-1.97683175220599,7.66015640472539,
103.936773061735));
#226549=CARTESIAN_POINT('Ctrl Pts',(-2.14751771150057,7.61509325243354,
103.942790127807));
#226550=CARTESIAN_POINT('Ctrl Pts',(-2.27475806731773,7.57805731037085,
103.947323645382));
#226551=CARTESIAN_POINT('Ctrl Pts',(-2.68330630466245,7.44792366549738,
103.962177800813));
#226552=CARTESIAN_POINT('Ctrl Pts',(-2.96031438222329,7.34222143500387,
103.972709714878));
#226553=CARTESIAN_POINT('Ctrl Pts',(-3.25409758198842,7.21078537508867,
103.984975951814));
#226554=CARTESIAN_POINT('Ctrl Pts',(-3.27742222932424,7.2002139070118,103.985957574412));
#226555=CARTESIAN_POINT('Ctrl Pts',(-3.34711747620623,7.16821699409926,
103.988915077347));
#226556=CARTESIAN_POINT('Ctrl Pts',(-3.39333162759222,7.14645580274434,
103.990908608273));
#226557=CARTESIAN_POINT('Ctrl Pts',(-3.46864176616134,7.11009877944754,
103.99421532469));
#226558=CARTESIAN_POINT('Ctrl Pts',(-3.49786462754324,7.0957679884593,103.995512912344));
#226559=CARTESIAN_POINT('Ctrl Pts',(-3.53362680915434,7.07795573724664,
103.997119598829));
#226560=CARTESIAN_POINT('Ctrl Pts',(-3.54025112943678,7.07464471084221,
103.997418001981));
#226561=CARTESIAN_POINT('Ctrl Pts',(-3.55119766647502,7.06915409125499,
103.997912432289));
#226562=CARTESIAN_POINT('Ctrl Pts',(-3.55552256001436,7.06697981865559,
103.998108120774));
#226563=CARTESIAN_POINT('Ctrl Pts',(-3.56312740649478,7.06314785284663,
103.998452825005));
#226564=CARTESIAN_POINT('Ctrl Pts',(-3.56640820895334,7.06149183905997,
103.99860173286));
#226565=CARTESIAN_POINT('Ctrl Pts',(-3.57350893888364,7.05790147262813,
103.998924451936));
#226566=CARTESIAN_POINT('Ctrl Pts',(-3.57732845022648,7.05596630467197,
103.99909831588));
#226567=CARTESIAN_POINT('Ctrl Pts',(-3.58739002597015,7.0508583046246,103.99955703995));
#226568=CARTESIAN_POINT('Ctrl Pts',(-3.59362943974904,7.04768029066821,
103.99984223795));
#226569=CARTESIAN_POINT('Ctrl Pts',(-3.62208534656855,7.03313880455226,
104.001146311763));
#226570=CARTESIAN_POINT('Ctrl Pts',(-3.64425179495893,7.02167875301273,
104.002171608329));
#226571=CARTESIAN_POINT('Ctrl Pts',(-3.70334879541277,6.99077040190886,
104.004929604827));
#226572=CARTESIAN_POINT('Ctrl Pts',(-3.74018001223325,6.97113451782528,
104.006674177917));
#226573=CARTESIAN_POINT('Ctrl Pts',(-3.84072335425268,6.9165055318967,104.011503236261));
#226574=CARTESIAN_POINT('Ctrl Pts',(-3.90411022455767,6.88092489660138,
104.014621724334));
#226575=CARTESIAN_POINT('Ctrl Pts',(-4.09343632235216,6.77119322754072,
104.024137582085));
#226576=CARTESIAN_POINT('Ctrl Pts',(-4.21781684708899,6.6944227706998,104.030661433935));
#226577=CARTESIAN_POINT('Ctrl Pts',(-5.12587168843778,6.09859560842986,
104.07991183628));
#226578=CARTESIAN_POINT('Ctrl Pts',(-5.81390203939381,5.44673491787291,
104.125124322255));
#226579=CARTESIAN_POINT('Ctrl Pts',(-6.40335301967687,4.64584796381104,
104.165842123544));
#226580=CARTESIAN_POINT('Ctrl Pts',(-6.43489595765177,4.60205903639653,
104.168033205165));
#226581=CARTESIAN_POINT('Ctrl Pts',(-6.47315525012999,4.54778372633621,
104.170706433047));
#226582=CARTESIAN_POINT('Ctrl Pts',(-6.48029771376349,4.53760038531198,
104.171206170787));
#226583=CARTESIAN_POINT('Ctrl Pts',(-6.49209008166837,4.5207028294275,104.172032395572));
#226584=CARTESIAN_POINT('Ctrl Pts',(-6.49675364533883,4.51399820257221,
104.172359444604));
#226585=CARTESIAN_POINT('Ctrl Pts',(-6.50517531338007,4.50185060736039,
104.172950590257));
#226586=CARTESIAN_POINT('Ctrl Pts',(-6.50893698651854,4.4964101297176,104.173214833315));
#226587=CARTESIAN_POINT('Ctrl Pts',(-6.51698421277751,4.48474023124861,
104.17378054792));
#226588=CARTESIAN_POINT('Ctrl Pts',(-6.52126766888685,4.47850936836607,
104.17408193342));
#226589=CARTESIAN_POINT('Ctrl Pts',(-6.53287199665189,4.46157736505054,
104.174899133248));
#226590=CARTESIAN_POINT('Ctrl Pts',(-6.54017551962917,4.45086432995026,
104.17541423807));
#226591=CARTESIAN_POINT('Ctrl Pts',(-6.57664940707072,4.397079672211,104.177990622748));
#226592=CARTESIAN_POINT('Ctrl Pts',(-6.60542110872749,4.35373852958503,
104.180035654169));
#226593=CARTESIAN_POINT('Ctrl Pts',(-6.9312629576137,3.85223051579598,104.203351103466));
#226594=CARTESIAN_POINT('Ctrl Pts',(-7.1805725468827,3.3647499328151,104.222545757408));
#226595=CARTESIAN_POINT('Ctrl Pts',(-7.54437659947113,2.42478078451246,
104.256786922232));
#226596=CARTESIAN_POINT('Ctrl Pts',(-7.67302194342936,1.98037085670152,
104.27199968181));
#226597=CARTESIAN_POINT('Ctrl Pts',(-7.7669124643957,1.50319515790408,104.28941954837));
#226598=CARTESIAN_POINT('Ctrl Pts',(-7.77154446621564,1.47906102237896,
104.29030360783));
#226599=CARTESIAN_POINT('Ctrl Pts',(-7.81508163153357,1.24636707679826,
104.298859770764));
#226600=CARTESIAN_POINT('Ctrl Pts',(-7.84569187805009,1.03635781168871,
104.306830807747));
#226601=CARTESIAN_POINT('Ctrl Pts',(-7.86921209141696,0.812157052864072,
104.315847017301));
#226602=CARTESIAN_POINT('Ctrl Pts',(-7.8705668494434,0.798921449377772,
104.316381155163));
#226603=CARTESIAN_POINT('Ctrl Pts',(-7.87238258706678,0.780729263276773,
104.317117968936));
#226604=CARTESIAN_POINT('Ctrl Pts',(-7.87287229392831,0.775775497938781,
104.317318874509));
#226605=CARTESIAN_POINT('Ctrl Pts',(-7.87370349478392,0.767285408646501,
104.317663666046));
#226606=CARTESIAN_POINT('Ctrl Pts',(-7.87404728115733,0.763749328058591,
104.317807408258));
#226607=CARTESIAN_POINT('Ctrl Pts',(-7.87473315746019,0.756644929113058,
104.318096479118));
#226608=CARTESIAN_POINT('Ctrl Pts',(-7.87507520427521,0.753076607575596,
104.318241810375));
#226609=CARTESIAN_POINT('Ctrl Pts',(-7.87576040850192,0.745876861759802,
104.318535323293));
#226610=CARTESIAN_POINT('Ctrl Pts',(-7.87610347990846,0.742245430244154,
104.31868351017));
#226611=CARTESIAN_POINT('Ctrl Pts',(-7.87688444354181,0.733917374887801,
104.319023678722));
#226612=CARTESIAN_POINT('Ctrl Pts',(-7.87732064658357,0.72922059816389,
104.319215762732));
#226613=CARTESIAN_POINT('Ctrl Pts',(-7.8784277896093,0.71718261793078,104.319708687229));
#226614=CARTESIAN_POINT('Ctrl Pts',(-7.87909266814807,0.709840876216685,
104.320009891584));
#226615=CARTESIAN_POINT('Ctrl Pts',(-7.88442274332827,0.650054754388907,
104.32246734418));
#226616=CARTESIAN_POINT('Ctrl Pts',(-7.88857442631856,0.59756710309949,
104.324653929315));
#226617=CARTESIAN_POINT('Ctrl Pts',(-7.90468572739658,0.364276148668387,
104.334489649893));
#226618=CARTESIAN_POINT('Ctrl Pts',(-7.91095452025883,0.183146265022534,
104.34243748295));
#226619=CARTESIAN_POINT('Ctrl Pts',(-7.91099975343153,0.00197514715529489,
104.350590048145));
#226620=CARTESIAN_POINT('',(-7.91212843677151,0.00142906907571687,106.355715790758));
#226621=CARTESIAN_POINT('Ctrl Pts',(-7.91099966760513,0.0022932840043321,
104.357668491763));
#226622=CARTESIAN_POINT('Ctrl Pts',(-7.91105540365936,-0.189975927168933,
104.365452204501));
#226623=CARTESIAN_POINT('Ctrl Pts',(-7.90409755832876,-0.382548785251838,
104.373235917239));
#226624=CARTESIAN_POINT('Ctrl Pts',(-7.89008583166137,-0.574862217419591,
104.381019629977));
#226625=CARTESIAN_POINT('Ctrl Pts',(-7.87608942923311,-0.766965321688851,
104.388794829884));
#226626=CARTESIAN_POINT('Ctrl Pts',(-7.85505452960641,-0.958809212370408,
104.39657002979));
#226627=CARTESIAN_POINT('Ctrl Pts',(-7.82699276817718,-1.1498283380149,
104.404345229696));
#226628=CARTESIAN_POINT('Ctrl Pts',(-7.79895606160157,-1.34067691284624,
104.41211348754));
#226629=CARTESIAN_POINT('Ctrl Pts',(-7.76390503675182,-1.53070183793467,
104.419881745383));
#226630=CARTESIAN_POINT('Ctrl Pts',(-7.72190330477566,-1.71934009192329,
104.427650003227));
#226631=CARTESIAN_POINT('Ctrl Pts',(-7.6799306472337,-1.90784776676084,
104.435412883729));
#226632=CARTESIAN_POINT('Ctrl Pts',(-7.63101694138477,-2.09497033484641,
104.44317576423));
#226633=CARTESIAN_POINT('Ctrl Pts',(-7.57527732234824,-2.28015229524619,
104.450938644731));
#226634=CARTESIAN_POINT('Ctrl Pts',(-7.5174414684052,-2.47229851008754,
104.458993468761));
#226635=CARTESIAN_POINT('Ctrl Pts',(-7.45225636839487,-2.66235493024437,
104.467048292791));
#226636=CARTESIAN_POINT('Ctrl Pts',(-7.37990848984268,-2.84971431577762,
104.475103116821));
#226637=CARTESIAN_POINT('Ctrl Pts',(-7.31022957258088,-3.03016188914186,
104.482860793043));
#226638=CARTESIAN_POINT('Ctrl Pts',(-7.23390704747383,-3.2081074994048,
104.490618469265));
#226639=CARTESIAN_POINT('Ctrl Pts',(-7.15115772006215,-3.38302590335864,
104.498376145487));
#226640=CARTESIAN_POINT('Ctrl Pts',(-7.06841177366112,-3.55793716041467,
104.506133504743));
#226641=CARTESIAN_POINT('Ctrl Pts',(-6.97923970021827,-3.72982113424552,
104.513890863998));
#226642=CARTESIAN_POINT('Ctrl Pts',(-6.88390556306171,-3.89817459830215,
104.521648223253));
#226643=CARTESIAN_POINT('Ctrl Pts',(-6.78855801588808,-4.06655174351742,
104.529406673684));
#226644=CARTESIAN_POINT('Ctrl Pts',(-6.68704685527186,-4.23139707923972,
104.537165124115));
#226645=CARTESIAN_POINT('Ctrl Pts',(-6.57968104908572,-4.39223386129453,
104.544923574547));
#226646=CARTESIAN_POINT('Ctrl Pts',(-6.47228064805728,-4.55312246732672,
104.552684524865));
#226647=CARTESIAN_POINT('Ctrl Pts',(-6.35902204361093,-4.70999965104927,
104.560445475183));
#226648=CARTESIAN_POINT('Ctrl Pts',(-6.24025632262631,-4.862419359529,104.568206425501));
#226649=CARTESIAN_POINT('Ctrl Pts',(-6.12137695518243,-5.01498491783851,
104.575974802242));
#226650=CARTESIAN_POINT('Ctrl Pts',(-5.99698016904949,-5.16308420280908,
104.583743178984));
#226651=CARTESIAN_POINT('Ctrl Pts',(-5.86745651897299,-5.3063052115348,
104.591511555725));
#226652=CARTESIAN_POINT('Ctrl Pts',(-5.73785926939866,-5.44960760303745,
104.599284346708));
#226653=CARTESIAN_POINT('Ctrl Pts',(-5.60312960014719,-5.58802594057014,
104.60705713769));
#226654=CARTESIAN_POINT('Ctrl Pts',(-5.46369334513455,-5.721186592861,104.614829928673));
#226655=CARTESIAN_POINT('Ctrl Pts',(-5.32409135039537,-5.85450552543623,
104.622611958718));
#226656=CARTESIAN_POINT('Ctrl Pts',(-5.17977186798612,-5.98255406145579,
104.630393988763));
#226657=CARTESIAN_POINT('Ctrl Pts',(-5.03119268895238,-6.10499968277085,
104.638176018807));
#226658=CARTESIAN_POINT('Ctrl Pts',(-4.99250852085789,-6.13687970141269,
104.640202153023));
#226659=CARTESIAN_POINT('Ctrl Pts',(-4.9535357447777,-6.16838014373279,
104.642228287239));
#226660=CARTESIAN_POINT('Ctrl Pts',(-4.91428273928625,-6.19949563741706,
104.644254421454));
#226661=CARTESIAN_POINT('Ctrl Pts',(-4.74779344431759,-6.33147015863494,
104.652848149574));
#226662=CARTESIAN_POINT('Ctrl Pts',(-4.57588316661556,-6.4568154454824,
104.661441877694));
#226663=CARTESIAN_POINT('Ctrl Pts',(-4.39908100386116,-6.57510511866296,
104.670035605814));
#226664=CARTESIAN_POINT('Ctrl Pts',(-4.2225341128925,-6.69322400198644,
104.678616926074));
#226665=CARTESIAN_POINT('Ctrl Pts',(-4.0411096380926,-6.80430746372126,
104.687198246335));
#226666=CARTESIAN_POINT('Ctrl Pts',(-3.8553676831306,-6.90797083287648,
104.695779566596));
#226667=CARTESIAN_POINT('Ctrl Pts',(-3.6615929796295,-7.01611731290082,
104.704732001653));
#226668=CARTESIAN_POINT('Ctrl Pts',(-3.46311926290425,-7.11618749880798,
104.713684436709));
#226669=CARTESIAN_POINT('Ctrl Pts',(-3.26061784832021,-7.20779385437844,
104.722636871766));
#226670=CARTESIAN_POINT('Ctrl Pts',(-3.06727569377342,-7.29525679972406,
104.731184382834));
#226671=CARTESIAN_POINT('Ctrl Pts',(-2.87026238401813,-7.3750044417643,
104.739731893902));
#226672=CARTESIAN_POINT('Ctrl Pts',(-2.67018989329174,-7.44674472059857,
104.748279404969));
#226673=CARTESIAN_POINT('Ctrl Pts',(-2.47042499767427,-7.51837470461518,
104.756813774937));
#226674=CARTESIAN_POINT('Ctrl Pts',(-2.26761053651013,-7.58202180048187,
104.765348144904));
#226675=CARTESIAN_POINT('Ctrl Pts',(-2.06237947018481,-7.63744145122961,
104.773882514872));
#226676=CARTESIAN_POINT('Ctrl Pts',(-1.85759523883733,-7.69274044072047,
104.782398303564));
#226677=CARTESIAN_POINT('Ctrl Pts',(-1.65040514059566,-7.73984766417033,
104.790914092256));
#226678=CARTESIAN_POINT('Ctrl Pts',(-1.44145841140395,-7.77856790471053,
104.799429880948));
#226679=CARTESIAN_POINT('Ctrl Pts',(-1.41055150242955,-7.7842953116648,
104.800689516392));
#226680=CARTESIAN_POINT('Ctrl Pts',(-1.37960619187283,-7.78983930151628,
104.801949151836));
#226681=CARTESIAN_POINT('Ctrl Pts',(-1.34862461415533,-7.79519933357027,
104.803208787279));
#226682=CARTESIAN_POINT('Ctrl Pts',(-1.1544530700158,-7.82879238393236,
104.811103329042));
#226683=CARTESIAN_POINT('Ctrl Pts',(-0.959035595012537,-7.85512446690431,
104.818997870805));
#226684=CARTESIAN_POINT('Ctrl Pts',(-0.762954745848102,-7.87412351032087,
104.826892412568));
#226685=CARTESIAN_POINT('Ctrl Pts',(-0.5668297083475,-7.89312683531883,
104.834788733427));
#226686=CARTESIAN_POINT('Ctrl Pts',(-0.370041339620588,-7.90479379417677,
104.842685054285));
#226687=CARTESIAN_POINT('Ctrl Pts',(-0.173176053447485,-7.90910431430212,
104.850581375144));
#226688=CARTESIAN_POINT('Ctrl Pts',(0.0237660536522444,-7.91341651648201,
104.858480777312));
#226689=CARTESIAN_POINT('Ctrl Pts',(0.220784795879588,-7.91036655159211,
104.866380179479));
#226690=CARTESIAN_POINT('Ctrl Pts',(0.417294745685731,-7.89998646171138,
104.874279581647));
#226691=CARTESIAN_POINT('Ctrl Pts',(0.614020932190244,-7.88959494973032,
104.882187676201));
#226692=CARTESIAN_POINT('Ctrl Pts',(0.810236865532022,-7.87185721642027,
104.890095770756));
#226693=CARTESIAN_POINT('Ctrl Pts',(1.00536199019258,-7.84685722239649,
104.898003865311));
#226694=CARTESIAN_POINT('Ctrl Pts',(1.200603367283,-7.82184233377595,104.905916671383));
#226695=CARTESIAN_POINT('Ctrl Pts',(1.39475230272953,-7.78955661321012,
104.913829477454));
#226696=CARTESIAN_POINT('Ctrl Pts',(1.5872390708678,-7.75013503959194,104.921742283525));
#226697=CARTESIAN_POINT('Ctrl Pts',(1.77999557725638,-7.71065822318281,
104.92966617808));
#226698=CARTESIAN_POINT('Ctrl Pts',(1.97108492994987,-7.66402565369724,
104.937590072636));
#226699=CARTESIAN_POINT('Ctrl Pts',(2.15995184656808,-7.61042239435546,
104.945513967191));
#226700=CARTESIAN_POINT('Ctrl Pts',(2.29223025190917,-7.57287980196408,
104.951063695829));
#226701=CARTESIAN_POINT('Ctrl Pts',(2.423418832233,-7.53191891169716,104.956613424467));
#226702=CARTESIAN_POINT('Ctrl Pts',(2.55333299200044,-7.48761721991463,
104.962163153104));
#226703=CARTESIAN_POINT('Ctrl Pts',(2.74352007348458,-7.4227620149084,104.970287646189));
#226704=CARTESIAN_POINT('Ctrl Pts',(2.93139354558582,-7.35060237745438,
104.978412139274));
#226705=CARTESIAN_POINT('Ctrl Pts',(3.11637262500933,-7.27132330886837,
104.986536632358));
#226706=CARTESIAN_POINT('Ctrl Pts',(3.3011882759034,-7.19211428313064,104.994653947475));
#226707=CARTESIAN_POINT('Ctrl Pts',(3.48311433912189,-7.10579849261481,
105.002771262591));
#226708=CARTESIAN_POINT('Ctrl Pts',(3.66158736575237,-7.0126099964965,105.010888577708));
#226709=CARTESIAN_POINT('Ctrl Pts',(3.83992812372441,-6.91949056357275,
105.018999876977));
#226710=CARTESIAN_POINT('Ctrl Pts',(4.01482066445471,-6.81950872892337,
105.027111176247));
#226711=CARTESIAN_POINT('Ctrl Pts',(4.18572310027882,-6.71294593511614,
105.035222475517));
#226712=CARTESIAN_POINT('Ctrl Pts',(4.35652317963895,-6.60644696363369,
105.043328916787));
#226713=CARTESIAN_POINT('Ctrl Pts',(4.52333764808086,-6.49337506201214,
105.051435358057));
#226714=CARTESIAN_POINT('Ctrl Pts',(4.68565024125884,-6.37405701391123,
105.059541799328));
#226715=CARTESIAN_POINT('Ctrl Pts',(4.84788867754221,-6.25479347948512,
105.067644536951));
#226716=CARTESIAN_POINT('Ctrl Pts',(5.00562908260075,-6.12928967956017,
105.075747274575));
#226717=CARTESIAN_POINT('Ctrl Pts',(5.1583846807232,-5.99791534499115,105.083850012199));
#226718=CARTESIAN_POINT('Ctrl Pts',(5.31251977523874,-5.86535460270345,
105.092025923555));
#226719=CARTESIAN_POINT('Ctrl Pts',(5.46157931214299,-5.72681695804001,
105.100201834912));
#226720=CARTESIAN_POINT('Ctrl Pts',(5.605096967992,-5.58272415397778,105.108377746268));
#226721=CARTESIAN_POINT('Ctrl Pts',(5.74727592966195,-5.4399754089228,105.116477394917));
#226722=CARTESIAN_POINT('Ctrl Pts',(5.88401573682601,-5.29177493899788,
105.124577043567));
#226723=CARTESIAN_POINT('Ctrl Pts',(6.01489947357244,-5.13857035787368,
105.132676692216));
#226724=CARTESIAN_POINT('Ctrl Pts',(6.14578232084147,-4.98536681791789,
105.140776285821));
#226725=CARTESIAN_POINT('Ctrl Pts',(6.2708089688368,-4.82715947850089,105.148875879426));
#226726=CARTESIAN_POINT('Ctrl Pts',(6.38960213034008,-4.66442982753021,
105.15697547303));
#226727=CARTESIAN_POINT('Ctrl Pts',(6.50840982167866,-4.50168027276208,
105.165076057313));
#226728=CARTESIAN_POINT('Ctrl Pts',(6.62098231733734,-4.33440756265213,
105.173176641596));
#226729=CARTESIAN_POINT('Ctrl Pts',(6.72698477035619,-4.16312345473875,
105.181277225878));
#226730=CARTESIAN_POINT('Ctrl Pts',(6.83471852367279,-3.9890418245173,105.189510114118));
#226731=CARTESIAN_POINT('Ctrl Pts',(6.93566557619923,-3.81081691551062,
105.197743002358));
#226732=CARTESIAN_POINT('Ctrl Pts',(7.02952218148843,-3.62901348853406,
105.205975890597));
#226733=CARTESIAN_POINT('Ctrl Pts',(7.12195867872563,-3.44996085900788,
105.214084210184));
#226734=CARTESIAN_POINT('Ctrl Pts',(7.20751766270693,-3.26743754053747,
105.222192529771));
#226735=CARTESIAN_POINT('Ctrl Pts',(7.28595679560303,-3.08200495986072,
105.230300849357));
#226736=CARTESIAN_POINT('Ctrl Pts',(7.36620352691879,-2.89229915958795,
105.238596021923));
#226737=CARTESIAN_POINT('Ctrl Pts',(7.43899817239824,-2.69954872770601,
105.246891194489));
#226738=CARTESIAN_POINT('Ctrl Pts',(7.50413451096247,-2.50437342291082,
105.255186367055));
#226739=CARTESIAN_POINT('Ctrl Pts',(7.5692708495267,-2.30919811811563,105.263481539621));
#226740=CARTESIAN_POINT('Ctrl Pts',(7.6267488071954,-2.11159829106925,105.271776712187));
#226741=CARTESIAN_POINT('Ctrl Pts',(7.67641739374365,-1.91220736245574,
105.280071884753));
#226742=CARTESIAN_POINT('Ctrl Pts',(7.72328866953158,-1.72404603445868,
105.287899877215));
#226743=CARTESIAN_POINT('Ctrl Pts',(7.76329520909628,-1.53392888232882,
105.295727869676));
#226744=CARTESIAN_POINT('Ctrl Pts',(7.79627299009179,-1.34240398687027,
105.303555862137));
#226745=CARTESIAN_POINT('Ctrl Pts',(7.82922291749054,-1.15104085660777,
105.311377242942));
#226746=CARTESIAN_POINT('Ctrl Pts',(7.85515584751052,-0.958272695125778,
105.319198623747));
#226747=CARTESIAN_POINT('Ctrl Pts',(7.87395798253529,-0.76466115977527,
105.327020004552));
#226748=CARTESIAN_POINT('Ctrl Pts',(7.89274755730638,-0.571178961332209,
105.334836160496));
#226749=CARTESIAN_POINT('Ctrl Pts',(7.90441578986685,-0.376854860062968,
105.342652316441));
#226750=CARTESIAN_POINT('Ctrl Pts',(7.90890021233917,-0.182259241909436,
105.350468472386));
#226751=CARTESIAN_POINT('Ctrl Pts',(7.9133824804781,0.0122428917785477,
105.35828087342));
#226752=CARTESIAN_POINT('Ctrl Pts',(7.91068780466358,0.207015931256116,
105.366093274454));
#226753=CARTESIAN_POINT('Ctrl Pts',(7.90080567100698,0.401485677183981,
105.373905675488));
#226754=CARTESIAN_POINT('Ctrl Pts',(7.89092642578947,0.595898581742127,
105.381715793043));
#226755=CARTESIAN_POINT('Ctrl Pts',(7.87386392630452,0.790008017999797,
105.389525910599));
#226756=CARTESIAN_POINT('Ctrl Pts',(7.84965975582054,0.983240925639028,
105.397336028154));
#226757=CARTESIAN_POINT('Ctrl Pts',(7.82545420625492,1.17648484311458,105.405146590706));
#226758=CARTESIAN_POINT('Ctrl Pts',(7.79410621004036,1.36885178188897,105.412957153259));
#226759=CARTESIAN_POINT('Ctrl Pts',(7.75570915775862,1.55977449019374,105.420767715811));
#226760=CARTESIAN_POINT('Ctrl Pts',(7.72578925082309,1.70854605792873,105.426853894067));
#226761=CARTESIAN_POINT('Ctrl Pts',(7.69159027227738,1.85644077009817,105.432940072323));
#226762=CARTESIAN_POINT('Ctrl Pts',(7.65317788216522,2.00319477433851,105.439026250578));
#226763=CARTESIAN_POINT('Ctrl Pts',(7.59864495597029,2.21153706334161,105.447666616582));
#226764=CARTESIAN_POINT('Ctrl Pts',(7.53564500625163,2.41748072643363,105.456306982585));
#226765=CARTESIAN_POINT('Ctrl Pts',(7.46442045024432,2.62037179460747,105.464947348588));
#226766=CARTESIAN_POINT('Ctrl Pts',(7.39307741285503,2.82360037017338,105.473602087759));
#226767=CARTESIAN_POINT('Ctrl Pts',(7.31348249750433,3.02376598366972,105.482256826931));
#226768=CARTESIAN_POINT('Ctrl Pts',(7.22592629292175,3.22023449600524,105.490911566102));
#226769=CARTESIAN_POINT('Ctrl Pts',(7.13566206998034,3.42277956614581,105.49983398696));
#226770=CARTESIAN_POINT('Ctrl Pts',(7.03693637482808,3.62139495060253,105.508756407819));
#226771=CARTESIAN_POINT('Ctrl Pts',(6.93011767567737,3.81541478757737,105.517678828677));
#226772=CARTESIAN_POINT('Ctrl Pts',(6.82615596055228,4.00424534983444,105.52636260954));
#226773=CARTESIAN_POINT('Ctrl Pts',(6.71452871879979,4.18872285026605,105.535046390404));
#226774=CARTESIAN_POINT('Ctrl Pts',(6.59561969201529,4.36826302760034,105.543730171267));
#226775=CARTESIAN_POINT('Ctrl Pts',(6.47180903596822,4.55520415178306,105.552771912123));
#226776=CARTESIAN_POINT('Ctrl Pts',(6.34010375121489,4.73679207408774,105.561813652979));
#226777=CARTESIAN_POINT('Ctrl Pts',(6.20098443854627,4.91240399325086,105.570855393835));
#226778=CARTESIAN_POINT('Ctrl Pts',(6.06186512587764,5.08801591241399,105.579897134691));
#226779=CARTESIAN_POINT('Ctrl Pts',(5.91533198265794,5.25765163063006,105.588938875547));
#226780=CARTESIAN_POINT('Ctrl Pts',(5.76191112895378,5.42072883863772,105.597980616403));
#226781=CARTESIAN_POINT('Ctrl Pts',(5.62070299111643,5.57082465879838,105.606302610176));
#226782=CARTESIAN_POINT('Ctrl Pts',(5.4735400667773,5.71549204698301,105.614624603948));
#226783=CARTESIAN_POINT('Ctrl Pts',(5.32085780504846,5.85426282451129,105.62294659772));
#226784=CARTESIAN_POINT('Ctrl Pts',(5.16831134156209,5.99291017691159,105.631261189768));
#226785=CARTESIAN_POINT('Ctrl Pts',(5.01025554918787,6.12567118499115,105.639575781815));
#226786=CARTESIAN_POINT('Ctrl Pts',(4.84716276725742,6.25211437097191,105.647890373862));
#226787=CARTESIAN_POINT('Ctrl Pts',(4.6842050966759,6.37845280731739,105.656198077832));
#226788=CARTESIAN_POINT('Ctrl Pts',(4.51621899160593,6.49848368439002,105.664505781802));
#226789=CARTESIAN_POINT('Ctrl Pts',(4.34371056714706,6.61181514478853,105.672813485772));
#226790=CARTESIAN_POINT('Ctrl Pts',(4.17137619591483,6.72503225885048,105.681112807642));
#226791=CARTESIAN_POINT('Ctrl Pts',(3.99452885677393,6.83156328840419,105.689412129513));
#226792=CARTESIAN_POINT('Ctrl Pts',(3.81370470239067,6.93105889766948,105.697711451384));
#226793=CARTESIAN_POINT('Ctrl Pts',(3.63299607670489,7.0304909391101,105.706005470811));
#226794=CARTESIAN_POINT('Ctrl Pts',(3.44831595931696,7.12289638557427,105.714299490238));
#226795=CARTESIAN_POINT('Ctrl Pts',(3.26022746868949,7.20797043920149,105.722593509666));
#226796=CARTESIAN_POINT('Ctrl Pts',(3.07227845503456,7.29298140618581,105.730881378665));
#226797=CARTESIAN_POINT('Ctrl Pts',(2.88092637839446,7.37067171053527,105.739169247664));
#226798=CARTESIAN_POINT('Ctrl Pts',(2.68675731058709,7.4407833024492,105.747457116664));
#226799=CARTESIAN_POINT('Ctrl Pts',(2.61274116637358,7.4675094424917,105.750616405185));
#226800=CARTESIAN_POINT('Ctrl Pts',(2.53831591804569,7.49313481443207,105.753775693706));
#226801=CARTESIAN_POINT('Ctrl Pts',(2.46351483339233,7.51764695005398,105.756934982227));
#226802=CARTESIAN_POINT('Ctrl Pts',(2.271680007557,7.58051076131652,105.765037292054));
#226803=CARTESIAN_POINT('Ctrl Pts',(2.07745262938128,7.63602267718541,105.77313960188));
#226804=CARTESIAN_POINT('Ctrl Pts',(1.88142453251002,7.68401995888021,105.781241911706));
#226805=CARTESIAN_POINT('Ctrl Pts',(1.68535316761434,7.73202783470713,105.789346009904));
#226806=CARTESIAN_POINT('Ctrl Pts',(1.48748060110207,7.77251769248018,105.797450108101));
#226807=CARTESIAN_POINT('Ctrl Pts',(1.28841015696449,7.8053776505324,105.805554206298));
#226808=CARTESIAN_POINT('Ctrl Pts',(1.08927080236307,7.83824898342715,105.81366110982));
#226809=CARTESIAN_POINT('Ctrl Pts',(0.88893305766179,7.86348509705911,105.821768013342));
#226810=CARTESIAN_POINT('Ctrl Pts',(0.688007255811946,7.88102575912236,
105.829874916863));
#226811=CARTESIAN_POINT('Ctrl Pts',(0.486900249261919,7.89858224021124,
105.837989131586));
#226812=CARTESIAN_POINT('Ctrl Pts',(0.285204443780371,7.90842937344495,
105.84610334631));
#226813=CARTESIAN_POINT('Ctrl Pts',(0.0835334385470369,7.91055896663722,
105.854217561033));
#226814=CARTESIAN_POINT('Ctrl Pts',(-0.118236129806538,7.91268960063032,
105.862335741434));
#226815=CARTESIAN_POINT('Ctrl Pts',(-0.319980555027692,7.90709517442139,
105.870453921836));
#226816=CARTESIAN_POINT('Ctrl Pts',(-0.521088515780572,7.89381959248637,
105.878572102237));
#226817=CARTESIAN_POINT('Ctrl Pts',(-0.722412749193519,7.88052973391401,
105.886699012976));
#226818=CARTESIAN_POINT('Ctrl Pts',(-0.923098832767194,7.85954224158228,
105.894825923716));
#226819=CARTESIAN_POINT('Ctrl Pts',(-1.12254142126977,7.83095280010892,
105.902952834455));
#226820=CARTESIAN_POINT('Ctrl Pts',(-1.22836645289374,7.81578312862227,
105.907265005654));
#226821=CARTESIAN_POINT('Ctrl Pts',(-1.33384155310845,7.79847406587492,
105.911577176853));
#226822=CARTESIAN_POINT('Ctrl Pts',(-1.43887765982924,7.77904570497207,
105.915889348052));
#226823=CARTESIAN_POINT('Ctrl Pts',(-1.63368823366864,7.74301190426861,
105.923887136356));
#226824=CARTESIAN_POINT('Ctrl Pts',(-1.82732604650489,7.69962229868353,
105.931884924659));
#226825=CARTESIAN_POINT('Ctrl Pts',(-2.01920443715297,7.64896950189905,
105.939882712963));
#226826=CARTESIAN_POINT('Ctrl Pts',(-2.21092615932943,7.59835806306128,
105.947873971082));
#226827=CARTESIAN_POINT('Ctrl Pts',(-2.40089100033975,7.54049533650564,
105.955865229201));
#226828=CARTESIAN_POINT('Ctrl Pts',(-2.58852196651859,7.47552506710069,
105.96385648732));
#226829=CARTESIAN_POINT('Ctrl Pts',(-2.77603154930131,7.41059682866806,
105.971842575685));
#226830=CARTESIAN_POINT('Ctrl Pts',(-2.96120995140607,7.33857032082342,
105.979828664049));
#226831=CARTESIAN_POINT('Ctrl Pts',(-3.14349443852666,7.25963936535087,
105.987814752414));
#226832=CARTESIAN_POINT('Ctrl Pts',(-3.32569189816689,7.18074609362358,
105.995797028006));
#226833=CARTESIAN_POINT('Ctrl Pts',(-3.50499789047128,7.09495507767446,
106.003779303599));
#226834=CARTESIAN_POINT('Ctrl Pts',(-3.6808684159817,7.00250874360242,106.011761579192));
#226835=CARTESIAN_POINT('Ctrl Pts',(-3.85668477632484,6.91009088144821,
106.019741396378));
#226836=CARTESIAN_POINT('Ctrl Pts',(-4.0290674834548,6.81102194306289,106.027721213564));
#226837=CARTESIAN_POINT('Ctrl Pts',(-4.19749559379963,6.70559108058587,
106.03570103075));
#226838=CARTESIAN_POINT('Ctrl Pts',(-4.37171173832614,6.59653708516166,
106.043955074456));
#226839=CARTESIAN_POINT('Ctrl Pts',(-4.54169632465342,6.48067631299969,
106.052209118162));
#226840=CARTESIAN_POINT('Ctrl Pts',(-4.70690325897771,6.35837893732554,
106.060463161869));
#226841=CARTESIAN_POINT('Ctrl Pts',(-4.86664307485283,6.24012869345955,
106.068444058235));
#226842=CARTESIAN_POINT('Ctrl Pts',(-5.02191611579783,6.1158612585264,106.076424954602));
#226843=CARTESIAN_POINT('Ctrl Pts',(-5.17226052574444,5.98595372967632,
106.084405850968));
#226844=CARTESIAN_POINT('Ctrl Pts',(-5.32263831407062,5.85601735969534,
106.092388519196));
#226845=CARTESIAN_POINT('Ctrl Pts',(-5.46808503643004,5.72043861809531,
106.100371187423));
#226846=CARTESIAN_POINT('Ctrl Pts',(-5.60817370479094,5.57963338373513,
106.108353855651));
#226847=CARTESIAN_POINT('Ctrl Pts',(-5.74831500860744,5.4387752446843,106.116339523203));
#226848=CARTESIAN_POINT('Ctrl Pts',(-5.88309400892707,5.2926869351,106.124325190755));
#226849=CARTESIAN_POINT('Ctrl Pts',(-6.01212195496138,5.14181977500879,
106.132310858307));
#226850=CARTESIAN_POINT('Ctrl Pts',(-6.1412182178009,4.99087273483959,106.140300754053));
#226851=CARTESIAN_POINT('Ctrl Pts',(-6.26455713846359,4.83514205375893,
106.1482906498));
#226852=CARTESIAN_POINT('Ctrl Pts',(-6.38179124611312,4.67511085334176,
106.156280545547));
#226853=CARTESIAN_POINT('Ctrl Pts',(-6.49916422724139,4.51489008275636,
106.164279905985));
#226854=CARTESIAN_POINT('Ctrl Pts',(-6.61041775138325,4.35035888618521,
106.172279266423));
#226855=CARTESIAN_POINT('Ctrl Pts',(-6.7152478722501,4.18202905468631,106.180278626861));
#226856=CARTESIAN_POINT('Ctrl Pts',(-6.82015127527881,4.01358155114949,
106.188283579303));
#226857=CARTESIAN_POINT('Ctrl Pts',(-6.9186221538547,3.84133040617136,106.196288531744));
#226858=CARTESIAN_POINT('Ctrl Pts',(-7.0104030409166,3.6658109885682,106.204293484186));
#226859=CARTESIAN_POINT('Ctrl Pts',(-7.10230370952609,3.49006250380142,
106.212308883744));
#226860=CARTESIAN_POINT('Ctrl Pts',(-7.18749680345879,3.31103752751581,
106.220324283302));
#226861=CARTESIAN_POINT('Ctrl Pts',(-7.26577293518402,3.12929139811993,
106.22833968286));
#226862=CARTESIAN_POINT('Ctrl Pts',(-7.28354132327757,3.08803570892796,
106.230159148474));
#226863=CARTESIAN_POINT('Ctrl Pts',(-7.30095350231,3.04663986757932,106.231978614088));
#226864=CARTESIAN_POINT('Ctrl Pts',(-7.31800738292345,3.00511047109384,
106.233798079702));
#226865=CARTESIAN_POINT('Ctrl Pts',(-7.39877472521689,2.8084268506786,106.242415086315));
#226866=CARTESIAN_POINT('Ctrl Pts',(-7.47170868025304,2.60824228953016,
106.251032092929));
#226867=CARTESIAN_POINT('Ctrl Pts',(-7.53651565036496,2.40517210440419,
106.259649099543));
#226868=CARTESIAN_POINT('Ctrl Pts',(-7.6010415810271,2.20298254574469,106.268228737972));
#226869=CARTESIAN_POINT('Ctrl Pts',(-7.6575107334181,1.99793254499741,106.276808376402));
#226870=CARTESIAN_POINT('Ctrl Pts',(-7.70567814829004,1.79065498490509,
106.285388014831));
#226871=CARTESIAN_POINT('Ctrl Pts',(-7.75372047593898,1.58391570934492,
106.293945372573));
#226872=CARTESIAN_POINT('Ctrl Pts',(-7.79350400063278,1.37496063973674,
106.302502730314));
#226873=CARTESIAN_POINT('Ctrl Pts',(-7.82483228615782,1.1644400772484,106.311060088056));
#226874=CARTESIAN_POINT('Ctrl Pts',(-7.85602840229548,0.954807669771018,
106.319581343575));
#226875=CARTESIAN_POINT('Ctrl Pts',(-7.87884037064651,0.743623174706886,
106.328102599094));
#226876=CARTESIAN_POINT('Ctrl Pts',(-7.8931222040916,0.531547619010923,
106.336623854613));
#226877=CARTESIAN_POINT('Ctrl Pts',(-7.90487931359323,0.356962504255063,
106.343638733663));
#226878=CARTESIAN_POINT('Ctrl Pts',(-7.91085644909219,0.181773925383775,
106.350653612713));
#226879=CARTESIAN_POINT('Ctrl Pts',(-7.91099744449602,0.00635870878843768,
106.357668491763));
#226880=CARTESIAN_POINT('',(-7.90668697097569,-0.00507742928152955,108.357668491763));
#226881=CARTESIAN_POINT('Ctrl Pts',(-7.911,-2.54019028034236E-12,106.357668491763));
#226882=CARTESIAN_POINT('Ctrl Pts',(-7.91099999999929,-2.20167589666934,
106.446255927496));
#226883=CARTESIAN_POINT('Ctrl Pts',(-6.94214576672228,-4.38610418338912,
106.534843363229));
#226884=CARTESIAN_POINT('Ctrl Pts',(-3.6782020148804,-7.34180684107756,
106.712018234694));
#226885=CARTESIAN_POINT('Ctrl Pts',(-1.40868175871469,-8.08992666571385,
106.800605670427));
#226886=CARTESIAN_POINT('Ctrl Pts',(2.9730927052154,-7.65454228025154,106.977780541892));
#226887=CARTESIAN_POINT('Ctrl Pts',(5.0510207267583,-6.47444880834049,107.066367977625));
#226888=CARTESIAN_POINT('Ctrl Pts',(7.66951518847977,-2.93425195367433,
107.24354284909));
#226889=CARTESIAN_POINT('Ctrl Pts',(8.18956872247094,-0.601881960096207,
107.332130284823));
#226890=CARTESIAN_POINT('Ctrl Pts',(7.32306689761207,3.7153719823272,107.509305156289));
#226891=CARTESIAN_POINT('Ctrl Pts',(5.94329958849991,5.66643518936733,107.597892592021));
#226892=CARTESIAN_POINT('Ctrl Pts',(2.16154501637548,7.9220591323308,107.775067463487));
#226893=CARTESIAN_POINT('Ctrl Pts',(-0.210816529303511,8.20894963712995,
107.863654899219));
#226894=CARTESIAN_POINT('Ctrl Pts',(-4.42123908576707,6.9198224471766,108.040829770685));
#226895=CARTESIAN_POINT('Ctrl Pts',(-6.22631625634399,5.35390358803276,
108.129417206418));
#226896=CARTESIAN_POINT('Ctrl Pts',(-7.65317280859563,2.31334857514252,
108.264559258688));
#226897=CARTESIAN_POINT('Ctrl Pts',(-7.91100000000028,1.15702837836286,
108.311113875226));
#226898=CARTESIAN_POINT('Ctrl Pts',(-7.911,-1.9195756095769E-12,108.357668491763));
#226899=CARTESIAN_POINT('',(-7.92015086488778,-0.000676322392208838,110.357668491763));
#226900=CARTESIAN_POINT('Ctrl Pts',(-7.90464730954992,-0.00747858090497255,
108.357668491763));
#226901=CARTESIAN_POINT('Ctrl Pts',(-7.91210078102921,-0.847847773565596,
108.391498728258));
#226902=CARTESIAN_POINT('Ctrl Pts',(-7.40339374633633,-4.31311009557957,
108.531298541969));
#226903=CARTESIAN_POINT('Ctrl Pts',(-2.33386570890254,-9.06921176931051,
108.777067932898));
#226904=CARTESIAN_POINT('Ctrl Pts',(4.88597846667002,-7.2226779862135,109.041991875939));
#226905=CARTESIAN_POINT('Ctrl Pts',(7.79261686719547,-2.6388854416884,109.253931030372));
#226906=CARTESIAN_POINT('Ctrl Pts',(8.26759383351024,2.79482092152063,109.465870184806));
#226907=CARTESIAN_POINT('Ctrl Pts',(4.57231411070881,7.4310279169445,109.677809339238));
#226908=CARTESIAN_POINT('Ctrl Pts',(-0.838290124238692,8.19283827172977,
109.889748493671));
#226909=CARTESIAN_POINT('Ctrl Pts',(-4.65967318531691,6.81204228408581,
110.048702859496));
#226910=CARTESIAN_POINT('Ctrl Pts',(-7.28542678060952,3.80108478578778,
110.204676192194));
#226911=CARTESIAN_POINT('Ctrl Pts',(-7.92152424932248,1.2396389119941,110.307664736282));
#226912=CARTESIAN_POINT('Ctrl Pts',(-7.92015086488778,-0.000676322392208838,
110.357668491763));
#226913=CARTESIAN_POINT('',(-7.90798625669136,0.00451216966572269,112.357668491763));
#226914=CARTESIAN_POINT('Ctrl Pts',(-7.92015086488778,-0.000676322392208838,
110.357668491763));
#226915=CARTESIAN_POINT('Ctrl Pts',(-7.92006898894752,-0.0746191846174104,
110.360649524891));
#226916=CARTESIAN_POINT('Ctrl Pts',(-7.9188845772038,-0.148550187530037,
110.363630558018));
#226917=CARTESIAN_POINT('Ctrl Pts',(-7.83490291760856,-2.8490699327844,
110.472581168362));
#226918=CARTESIAN_POINT('Ctrl Pts',(-4.85753102683806,-7.99819754528262,
110.684520322796));
#226919=CARTESIAN_POINT('Ctrl Pts',(4.12483722040859,-8.40733305923675,
111.002429054444));
#226920=CARTESIAN_POINT('Ctrl Pts',(8.40870675888375,-2.30944008633724,
111.267352997486));
#226921=CARTESIAN_POINT('Ctrl Pts',(7.63590137194488,3.06294045831641,111.479292151919));
#226922=CARTESIAN_POINT('Ctrl Pts',(4.46313123637914,7.49963941440561,111.691231306351));
#226923=CARTESIAN_POINT('Ctrl Pts',(-1.35903023235194,8.61854216541067,
111.903170460786));
#226924=CARTESIAN_POINT('Ctrl Pts',(-5.96470993446413,5.67869392350227,
112.115109615218));
#226925=CARTESIAN_POINT('Ctrl Pts',(-7.65292984181716,2.70307941383637,
112.248947362674));
#226926=CARTESIAN_POINT('Ctrl Pts',(-7.90915144490032,0.696989207157879,
112.329800321523));
#226927=CARTESIAN_POINT('Ctrl Pts',(-7.90798625669136,0.00451216966572269,
112.357668491763));
#226928=CARTESIAN_POINT('',(-7.911,-1.68698388591793E-12,116.357668491763));
#226929=CARTESIAN_POINT('Ctrl Pts',(-7.91099909341042,0.00378735521236961,
112.359438569417));
#226930=CARTESIAN_POINT('Ctrl Pts',(-7.91110391793188,-0.215169317115718,
112.368531704429));
#226931=CARTESIAN_POINT('Ctrl Pts',(-7.90211847162492,-0.434041754412859,
112.377526913421));
#226932=CARTESIAN_POINT('Ctrl Pts',(-7.88108246637407,-0.688308156281573,
112.387881319802));
#226933=CARTESIAN_POINT('Ctrl Pts',(-7.87785345400522,-0.724329990006576,
112.389346070283));
#226934=CARTESIAN_POINT('Ctrl Pts',(-7.8720841184119,-0.784080380183848,
112.391772375696));
#226935=CARTESIAN_POINT('Ctrl Pts',(-7.86968324575642,-0.80782177882518,
112.392735581477));
#226936=CARTESIAN_POINT('Ctrl Pts',(-7.86516700529536,-0.85054917756705,
112.394467590496));
#226937=CARTESIAN_POINT('Ctrl Pts',(-7.86309021752687,-0.86953904925642,
112.395236844623));
#226938=CARTESIAN_POINT('Ctrl Pts',(-7.85871900643568,-0.908212123988966,
112.396802429831));
#226939=CARTESIAN_POINT('Ctrl Pts',(-7.85641936817883,-0.927894605184168,
112.39759869399));
#226940=CARTESIAN_POINT('Ctrl Pts',(-7.85129336098033,-0.970382198386325,
112.399316473813));
#226941=CARTESIAN_POINT('Ctrl Pts',(-7.84844153078315,-0.99318406813759,
112.400237686468));
#226942=CARTESIAN_POINT('Ctrl Pts',(-7.84047545541975,-1.05469923960324,
112.402721294243));
#226943=CARTESIAN_POINT('Ctrl Pts',(-7.83517384599178,-1.09338770616955,
112.404281529201));
#226944=CARTESIAN_POINT('Ctrl Pts',(-7.80724111346652,-1.28658106376407,
112.412065404366));
#226945=CARTESIAN_POINT('Ctrl Pts',(-7.78032515087,-1.44043265128534,112.418240217163));
#226946=CARTESIAN_POINT('Ctrl Pts',(-7.71946914944251,-1.73638400145209,
112.430122324764));
#226947=CARTESIAN_POINT('Ctrl Pts',(-7.68611230144968,-1.87853972945209,
112.435835263813));
#226948=CARTESIAN_POINT('Ctrl Pts',(-7.4358977017971,-2.82613602366019,
112.47405799312));
#226949=CARTESIAN_POINT('Ctrl Pts',(-7.0967628488701,-3.59381851737072,
112.504736754193));
#226950=CARTESIAN_POINT('Ctrl Pts',(-6.53707512693398,-4.45975115321796,
112.543696044146));
#226951=CARTESIAN_POINT('Ctrl Pts',(-6.42399579831044,-4.62114763320364,
112.551215180201));
#226952=CARTESIAN_POINT('Ctrl Pts',(-6.25284548959735,-4.84698923599435,
112.562294026589));
#226953=CARTESIAN_POINT('Ctrl Pts',(-6.19955397931614,-4.91496808548651,
112.565705655712));
#226954=CARTESIAN_POINT('Ctrl Pts',(-6.13553354891786,-4.99393459921745,
112.56977406205));
#226955=CARTESIAN_POINT('Ctrl Pts',(-6.12587160035205,-5.00578184139577,
112.570387282534));
#226956=CARTESIAN_POINT('Ctrl Pts',(-6.11100531676054,-5.02390301103125,
112.571329716701));
#226957=CARTESIAN_POINT('Ctrl Pts',(-6.10582549833209,-5.03019705668593,
112.571657884525));
#226958=CARTESIAN_POINT('Ctrl Pts',(-6.09639627480391,-5.04161857035328,
112.572254926099));
#226959=CARTESIAN_POINT('Ctrl Pts',(-6.09215010180067,-5.04674870438436,
112.572523658712));
#226960=CARTESIAN_POINT('Ctrl Pts',(-6.08356689682495,-5.05709212889711,
112.573066628641));
#226961=CARTESIAN_POINT('Ctrl Pts',(-6.07922962955142,-5.06230521592135,
112.573340876347));
#226962=CARTESIAN_POINT('Ctrl Pts',(-6.06688367817154,-5.07710542411794,
112.574121176705));
#226963=CARTESIAN_POINT('Ctrl Pts',(-6.05885900073047,-5.08667913861518,
112.574627953717));
#226964=CARTESIAN_POINT('Ctrl Pts',(-6.02485094157122,-5.12705726326551,
112.576774087429));
#226965=CARTESIAN_POINT('Ctrl Pts',(-5.99865532668357,-5.15768157646999,
112.578423385601));
#226966=CARTESIAN_POINT('Ctrl Pts',(-5.62110291550108,-5.59229675746159,
112.602158449571));
#226967=CARTESIAN_POINT('Ctrl Pts',(-5.22992590767809,-5.95971630803955,
112.626709873887));
#226968=CARTESIAN_POINT('Ctrl Pts',(-4.66511587914959,-6.39151873578675,
112.659310489173));
#226969=CARTESIAN_POINT('Ctrl Pts',(-4.52195329497706,-6.49359359529973,
112.667362624421));
#226970=CARTESIAN_POINT('Ctrl Pts',(-4.21533781734595,-6.6971493484238,
112.684063874268));
#226971=CARTESIAN_POINT('Ctrl Pts',(-4.0513402853464,-6.79761199024794,
112.692692307174));
#226972=CARTESIAN_POINT('Ctrl Pts',(-3.67881505754575,-7.00754058808218,
112.711526260314));
#226973=CARTESIAN_POINT('Ctrl Pts',(-3.46872724239839,-7.11387716125557,
112.721640843663));
#226974=CARTESIAN_POINT('Ctrl Pts',(-3.1572777764017,-7.25443484992384,
112.73587097101));
#226975=CARTESIAN_POINT('Ctrl Pts',(-3.05948239035484,-7.296217964917,112.740234815822));
#226976=CARTESIAN_POINT('Ctrl Pts',(-2.94507203749039,-7.3423948403118,
112.745221366311));
#226977=CARTESIAN_POINT('Ctrl Pts',(-2.92925166161774,-7.34872070530823,
112.745908294875));
#226978=CARTESIAN_POINT('Ctrl Pts',(-2.90516317970548,-7.35826247138739,
112.746950298369));
#226979=CARTESIAN_POINT('Ctrl Pts',(-2.89690994425414,-7.36151563701957,
112.747306611587));
#226980=CARTESIAN_POINT('Ctrl Pts',(-2.88194300212572,-7.36738606670268,
112.747951508545));
#226981=CARTESIAN_POINT('Ctrl Pts',(-2.87523116439721,-7.37000805121509,
112.748240248919));
#226982=CARTESIAN_POINT('Ctrl Pts',(-2.86180870316945,-7.37523041949227,
112.748816760699));
#226983=CARTESIAN_POINT('Ctrl Pts',(-2.85509809496872,-7.37783082366342,
112.749104532592));
#226984=CARTESIAN_POINT('Ctrl Pts',(-2.83621561657294,-7.38511828603602,
112.749912990048));
#226985=CARTESIAN_POINT('Ctrl Pts',(-2.82403566463424,-7.38978441426982,
112.750432980452));
#226986=CARTESIAN_POINT('Ctrl Pts',(-2.77400499419833,-7.40880936040276,
112.752562796256));
#226987=CARTESIAN_POINT('Ctrl Pts',(-2.7360555648631,-7.4229077762043,112.754163978913));
#226988=CARTESIAN_POINT('Ctrl Pts',(-2.14551303640637,-7.63715336867258,
112.778862374931));
#226989=CARTESIAN_POINT('Ctrl Pts',(-1.57240802252616,-7.77540770426758,
112.799688643695));
#226990=CARTESIAN_POINT('Ctrl Pts',(-0.687423736733492,-7.88694473036076,
112.830220914817));
#226991=CARTESIAN_POINT('Ctrl Pts',(-0.383689152701452,-7.90754244968169,
112.840456887215));
#226992=CARTESIAN_POINT('Ctrl Pts',(-0.037365374191139,-7.91102411903661,
112.852406943225));
#226993=CARTESIAN_POINT('Ctrl Pts',(0.00479878470609816,-7.91111090314451,
112.853866719993));
#226994=CARTESIAN_POINT('Ctrl Pts',(0.185755773332728,-7.91003668417216,
112.860158922853));
#226995=CARTESIAN_POINT('Ctrl Pts',(0.324501274579026,-7.90556023642795,
112.865051896828));
#226996=CARTESIAN_POINT('Ctrl Pts',(0.68185420656507,-7.88460741903093,
112.877971698729));
#226997=CARTESIAN_POINT('Ctrl Pts',(0.900013055256525,-7.86269184129545,
112.886166329226));
#226998=CARTESIAN_POINT('Ctrl Pts',(1.14638554205417,-7.82755417543703,
112.896026935467));
#226999=CARTESIAN_POINT('Ctrl Pts',(1.17578194491904,-7.82319250401897,
112.89721335305));
#227000=CARTESIAN_POINT('Ctrl Pts',(1.21263889942198,-7.81751145020797,
112.898713994789));
#227001=CARTESIAN_POINT('Ctrl Pts',(1.22012340279418,-7.81634679730411,
112.899019408456));
#227002=CARTESIAN_POINT('Ctrl Pts',(1.23199898070919,-7.81448138293267,
112.899505099109));
#227003=CARTESIAN_POINT('Ctrl Pts',(1.23639117288685,-7.81378766285104,
112.899684969854));
#227004=CARTESIAN_POINT('Ctrl Pts',(1.24464160440901,-7.81247742670176,
112.900023294816));
#227005=CARTESIAN_POINT('Ctrl Pts',(1.24849997833709,-7.81186175441789,
112.90018169994));
#227006=CARTESIAN_POINT('Ctrl Pts',(1.2571432261738,-7.8104760032265,112.900536964976));
#227007=CARTESIAN_POINT('Ctrl Pts',(1.26192784804837,-7.80970438583998,
112.900733914889));
#227008=CARTESIAN_POINT('Ctrl Pts',(1.27403280069354,-7.80774080198006,
112.901232924162));
#227009=CARTESIAN_POINT('Ctrl Pts',(1.28135216304042,-7.80654293794121,
112.90153533178));
#227010=CARTESIAN_POINT('Ctrl Pts',(1.32297696445081,-7.79967063501432,
112.903259010896));
#227011=CARTESIAN_POINT('Ctrl Pts',(1.35724587437818,-7.79378044501303,
112.904693159579));
#227012=CARTESIAN_POINT('Ctrl Pts',(1.94123807873922,-7.68943463857647,
112.929375784607));
#227013=CARTESIAN_POINT('Ctrl Pts',(2.47901890126596,-7.53327277421705,
112.955663656277));
#227014=CARTESIAN_POINT('Ctrl Pts',(3.209169117443,-7.23452048933398,112.992314636444));
#227015=CARTESIAN_POINT('Ctrl Pts',(3.41859487278246,-7.13794567891392,
113.002964997158));
#227016=CARTESIAN_POINT('Ctrl Pts',(3.87118663982711,-6.9047422230209,113.026025639755));
#227017=CARTESIAN_POINT('Ctrl Pts',(4.1119618519506,-6.76412161807801,113.038319595422));
#227018=CARTESIAN_POINT('Ctrl Pts',(4.43843949654639,-6.54955898637998,
113.054896555846));
#227019=CARTESIAN_POINT('Ctrl Pts',(4.53073263492991,-6.48605668569394,
113.05957319829));
#227020=CARTESIAN_POINT('Ctrl Pts',(4.65434640757037,-6.39707773841129,
113.065823899636));
#227021=CARTESIAN_POINT('Ctrl Pts',(4.68686394305266,-6.37329196884744,
113.067466970943));
#227022=CARTESIAN_POINT('Ctrl Pts',(4.7342659135548,-6.33805961609715,113.069860505458));
#227023=CARTESIAN_POINT('Ctrl Pts',(4.7492932772553,-6.32680699965637,113.070619061501));
#227024=CARTESIAN_POINT('Ctrl Pts',(4.77636171659958,-6.30638714074617,
113.071985022468));
#227025=CARTESIAN_POINT('Ctrl Pts',(4.78841678632789,-6.2972386568037,113.072593213018));
#227026=CARTESIAN_POINT('Ctrl Pts',(4.80683198267604,-6.2831800743934,113.073522067685));
#227027=CARTESIAN_POINT('Ctrl Pts',(4.81321096880611,-6.27829481047383,
113.073843782161));
#227028=CARTESIAN_POINT('Ctrl Pts',(4.82431462711144,-6.26976434869976,
113.074403713303));
#227029=CARTESIAN_POINT('Ctrl Pts',(4.82904263196144,-6.26612351206904,
113.074642114774));
#227030=CARTESIAN_POINT('Ctrl Pts',(4.83891153452042,-6.25850608396308,
113.075139695514));
#227031=CARTESIAN_POINT('Ctrl Pts',(4.84405166175257,-6.25452849865389,
113.075398832223));
#227032=CARTESIAN_POINT('Ctrl Pts',(4.8582315274726,-6.24352772614433,113.076113639642));
#227033=CARTESIAN_POINT('Ctrl Pts',(4.8672609501161,-6.2364912319877,113.076568742474));
#227034=CARTESIAN_POINT('Ctrl Pts',(4.90247055816215,-6.20892986713702,
113.078343129357));
#227035=CARTESIAN_POINT('Ctrl Pts',(4.92853663255235,-6.18825939721531,
113.079656173752));
#227036=CARTESIAN_POINT('Ctrl Pts',(5.33765698439499,-5.85960112397001,
113.100258677564));
#227037=CARTESIAN_POINT('Ctrl Pts',(5.6913420690343,-5.51672041297941,113.117876688909));
#227038=CARTESIAN_POINT('Ctrl Pts',(6.36690502540627,-4.72717974376021,
113.15354471197));
#227039=CARTESIAN_POINT('Ctrl Pts',(6.67869135551183,-4.27536109999382,
113.171322632807));
#227040=CARTESIAN_POINT('Ctrl Pts',(7.04175631420485,-3.61129191145059,
113.198523797016));
#227041=CARTESIAN_POINT('Ctrl Pts',(7.13485900466652,-3.42367289360687,
113.206330502067));
#227042=CARTESIAN_POINT('Ctrl Pts',(7.23185916858235,-3.20701103946101,
113.215729808808));
#227043=CARTESIAN_POINT('Ctrl Pts',(7.24317775071759,-3.18136493872878,
113.216848376715));
#227044=CARTESIAN_POINT('Ctrl Pts',(7.25718659932713,-3.14916082276682,
113.218261123051));
#227045=CARTESIAN_POINT('Ctrl Pts',(7.26000481357919,-3.14265832239199,
113.218546792701));
#227046=CARTESIAN_POINT('Ctrl Pts',(7.26447234677335,-3.13231224758086,
113.219001992224));
#227047=CARTESIAN_POINT('Ctrl Pts',(7.26612736706759,-3.12847112481371,
113.219171138576));
#227048=CARTESIAN_POINT('Ctrl Pts',(7.26924950071512,-3.12120914888068,
113.219491200025));
#227049=CARTESIAN_POINT('Ctrl Pts',(7.27071724812643,-3.11778856762346,
113.219642072818));
#227050=CARTESIAN_POINT('Ctrl Pts',(7.27402473882655,-3.11006543268988,
113.219982978173));
#227051=CARTESIAN_POINT('Ctrl Pts',(7.27586307839314,-3.10576228339939,
113.220173103432));
#227052=CARTESIAN_POINT('Ctrl Pts',(7.28055411377078,-3.09475457597844,
113.220659912145));
#227053=CARTESIAN_POINT('Ctrl Pts',(7.2834013607103,-3.08804771775673,113.220956951919));
#227054=CARTESIAN_POINT('Ctrl Pts',(7.29947243618667,-3.05004547920541,
113.222642442401));
#227055=CARTESIAN_POINT('Ctrl Pts',(7.3125036295819,-3.01866955275799,113.224043290719));
#227056=CARTESIAN_POINT('Ctrl Pts',(7.52739699507563,-2.49170135578868,
113.247713083894));
#227057=CARTESIAN_POINT('Ctrl Pts',(7.67864615754396,-1.97701063565568,
113.272856248665));
#227058=CARTESIAN_POINT('Ctrl Pts',(7.83376938138709,-1.14564515426838,
113.312610247343));
#227059=CARTESIAN_POINT('Ctrl Pts',(7.87271707739679,-0.837129145396408,
113.327199153451));
#227060=CARTESIAN_POINT('Ctrl Pts',(7.91679991703811,-0.176997222439834,
113.357455722306));
#227061=CARTESIAN_POINT('Ctrl Pts',(7.91686215876792,0.174310392148266,
113.372978577639));
#227062=CARTESIAN_POINT('Ctrl Pts',(7.88456468887725,0.660385353834943,
113.393477711963));
#227063=CARTESIAN_POINT('Ctrl Pts',(7.87202737273524,0.796025595825848,
113.399094915723));
#227064=CARTESIAN_POINT('Ctrl Pts',(7.85393469127237,0.948650008243326,
113.405305041202));
#227065=CARTESIAN_POINT('Ctrl Pts',(7.85181791582858,0.966013661854685,
113.406009940833));
#227066=CARTESIAN_POINT('Ctrl Pts',(7.84855745976568,0.992039890028385,
113.407064125316));
#227067=CARTESIAN_POINT('Ctrl Pts',(7.84745699644182,1.00070776569241,113.407414818286));
#227068=CARTESIAN_POINT('Ctrl Pts',(7.84554206918107,1.015593404926,113.40801639839));
#227069=CARTESIAN_POINT('Ctrl Pts',(7.84473456953753,1.02181204589919,113.408267512124));
#227070=CARTESIAN_POINT('Ctrl Pts',(7.843058684269,1.03459913663296,113.408783449678));
#227071=CARTESIAN_POINT('Ctrl Pts',(7.84218943904832,1.04116747009265,113.4090482453));
#227072=CARTESIAN_POINT('Ctrl Pts',(7.83983375724926,1.05879753958153,113.409758381213));
#227073=CARTESIAN_POINT('Ctrl Pts',(7.83833215862413,1.06985725382443,113.410203227722));
#227074=CARTESIAN_POINT('Ctrl Pts',(7.83277985626358,1.11011238197129,113.411820083304));
#227075=CARTESIAN_POINT('Ctrl Pts',(7.82858937730947,1.13928844608132,113.412987545689));
#227076=CARTESIAN_POINT('Ctrl Pts',(7.75843857498311,1.60903968331242,113.431715436527));
#227077=CARTESIAN_POINT('Ctrl Pts',(7.65553970168657,2.04331686113108,113.44798649548));
#227078=CARTESIAN_POINT('Ctrl Pts',(7.38892898988996,2.85575890663298,113.478043427477));
#227079=CARTESIAN_POINT('Ctrl Pts',(7.23122169912992,3.2343554663412,113.491894666743));
#227080=CARTESIAN_POINT('Ctrl Pts',(6.87209045805419,3.93733525900934,113.519588844311));
#227081=CARTESIAN_POINT('Ctrl Pts',(6.67511837697347,4.2627513887646,113.53339371771));
#227082=CARTESIAN_POINT('Ctrl Pts',(6.44521138912371,4.58731829371914,113.549296253781));
#227083=CARTESIAN_POINT('Ctrl Pts',(6.4348549380833,4.6018345143263,113.55001168697));
#227084=CARTESIAN_POINT('Ctrl Pts',(6.41978588157494,4.62280586973609,113.551051229688));
#227085=CARTESIAN_POINT('Ctrl Pts',(6.41511238820293,4.62928913772402,113.551373432809));
#227086=CARTESIAN_POINT('Ctrl Pts',(6.40694071231118,4.6405890947951,113.551936450492));
#227087=CARTESIAN_POINT('Ctrl Pts',(6.40344689751289,4.64540894521621,113.552177055654));
#227088=CARTESIAN_POINT('Ctrl Pts',(6.39668631094385,4.65471331256008,113.552642404484));
#227089=CARTESIAN_POINT('Ctrl Pts',(6.39342025454864,4.65919834642077,113.552867114248));
#227090=CARTESIAN_POINT('Ctrl Pts',(6.38566505020503,4.66982448624168,113.553400438384));
#227091=CARTESIAN_POINT('Ctrl Pts',(6.38117176254886,4.6759625535309,113.553709246292));
#227092=CARTESIAN_POINT('Ctrl Pts',(6.36771636976929,4.694287814086,113.554633388443));
#227093=CARTESIAN_POINT('Ctrl Pts',(6.35872818070992,4.70645575430839,113.555249922279));
#227094=CARTESIAN_POINT('Ctrl Pts',(6.27141623491458,4.82394936998101,113.561230863727));
#227095=CARTESIAN_POINT('Ctrl Pts',(6.19051976092825,4.92733316274009,113.566709192393));
#227096=CARTESIAN_POINT('Ctrl Pts',(5.70678285797201,5.51481165091869,113.59893609962));
#227097=CARTESIAN_POINT('Ctrl Pts',(5.24985412705107,5.9514358048604,113.627129031921));
#227098=CARTESIAN_POINT('Ctrl Pts',(4.44878940704382,6.55211280762734,113.670227265589));
#227099=CARTESIAN_POINT('Ctrl Pts',(4.13625447685716,6.75376454892645,113.685833570334));
#227100=CARTESIAN_POINT('Ctrl Pts',(3.75026236030472,6.96593195919709,113.703786433901));
#227101=CARTESIAN_POINT('Ctrl Pts',(3.68940199107702,6.99835615881094,113.706581249646));
#227102=CARTESIAN_POINT('Ctrl Pts',(3.60845490327048,7.0401323980446,113.710253229917));
#227103=CARTESIAN_POINT('Ctrl Pts',(3.58874216557697,7.05020146135516,113.711143924879));
#227104=CARTESIAN_POINT('Ctrl Pts',(3.55657778430463,7.06646084079189,113.712591482818));
#227105=CARTESIAN_POINT('Ctrl Pts',(3.54415165922709,7.07270127801969,113.713149330364));
#227106=CARTESIAN_POINT('Ctrl Pts',(3.52020978345086,7.08464602005354,113.714221481858));
#227107=CARTESIAN_POINT('Ctrl Pts',(3.50869646249076,7.09035508872612,113.714735879444));
#227108=CARTESIAN_POINT('Ctrl Pts',(3.48230004910934,7.10336414397074,113.715912518658));
#227109=CARTESIAN_POINT('Ctrl Pts',(3.46740780731474,7.11064546255504,113.716574382687));
#227110=CARTESIAN_POINT('Ctrl Pts',(3.42039172861212,7.13345038095268,113.718657750478));
#227111=CARTESIAN_POINT('Ctrl Pts',(3.38818558328636,7.14880356375863,113.720075773544));
#227112=CARTESIAN_POINT('Ctrl Pts',(3.09338535191011,7.28689983344149,113.732973337495));
#227113=CARTESIAN_POINT('Ctrl Pts',(2.82432757882454,7.39534506147803,113.744137725305));
#227114=CARTESIAN_POINT('Ctrl Pts',(2.15641584556803,7.62276746168111,113.77067123349));
#227115=CARTESIAN_POINT('Ctrl Pts',(1.75297346276947,7.72552936251439,113.785695606884));
#227116=CARTESIAN_POINT('Ctrl Pts',(1.00720051997519,7.85403069464445,113.813253009672));
#227117=CARTESIAN_POINT('Ctrl Pts',(0.667704405565595,7.89014560768651,
113.825735307388));
#227118=CARTESIAN_POINT('Ctrl Pts',(0.236678896904833,7.90797499995271,
113.842453276867));
#227119=CARTESIAN_POINT('Ctrl Pts',(0.146343353599015,7.91016234248309,
113.846006323216));
#227120=CARTESIAN_POINT('Ctrl Pts',(0.043352051265991,7.91089131463553,
113.850131613114));
#227121=CARTESIAN_POINT('Ctrl Pts',(0.0307113248932789,7.91095048677443,
113.850639213784));
#227122=CARTESIAN_POINT('Ctrl Pts',(0.0116570841825131,7.9109940112052,
113.851406352323));
#227123=CARTESIAN_POINT('Ctrl Pts',(0.00524360287973972,7.91100086191436,
113.851664905096));
#227124=CARTESIAN_POINT('Ctrl Pts',(-0.00581179448030742,7.91099922706025,
113.852111189915));
#227125=CARTESIAN_POINT('Ctrl Pts',(-0.0104537146909189,7.91099445501144,
113.85229875693));
#227126=CARTESIAN_POINT('Ctrl Pts',(-0.0200369077773404,7.91097616851029,
113.852686366837));
#227127=CARTESIAN_POINT('Ctrl Pts',(-0.0249781774822837,7.91096211006675,
113.852886434102));
#227128=CARTESIAN_POINT('Ctrl Pts',(-0.0369099305279455,7.9109169838234,
113.853370049368));
#227129=CARTESIAN_POINT('Ctrl Pts',(-0.0439003826038125,7.91088127984601,
113.853653807631));
#227130=CARTESIAN_POINT('Ctrl Pts',(-0.0696841907078328,7.91071541146477,
113.85470201851));
#227131=CARTESIAN_POINT('Ctrl Pts',(-0.0884770020701102,7.91052754359945,
113.855469129858));
#227132=CARTESIAN_POINT('Ctrl Pts',(-0.40090984731379,7.90629073550376,
113.86827668661));
#227133=CARTESIAN_POINT('Ctrl Pts',(-0.694063027933667,7.88596175562164,
113.881130812795));
#227134=CARTESIAN_POINT('Ctrl Pts',(-1.58438845386493,7.77419549238371,
113.921550005572));
#227135=CARTESIAN_POINT('Ctrl Pts',(-2.17284410502626,7.63067624980089,
113.950032454192));
#227136=CARTESIAN_POINT('Ctrl Pts',(-3.12075156759568,7.2808091132448,113.995176417622));
#227137=CARTESIAN_POINT('Ctrl Pts',(-3.49083400230011,7.1107953456663,114.012631633916));
#227138=CARTESIAN_POINT('Ctrl Pts',(-3.86654691882151,6.9017589119921,114.030072457503));
#227139=CARTESIAN_POINT('Ctrl Pts',(-3.88680657111852,6.89036979014518,
114.031012164163));
#227140=CARTESIAN_POINT('Ctrl Pts',(-3.91597410871349,6.8738034535794,114.032363999145));
#227141=CARTESIAN_POINT('Ctrl Pts',(-3.92492244188336,6.86869790897473,
114.032778586829));
#227142=CARTESIAN_POINT('Ctrl Pts',(-3.94047888764842,6.85978172562282,
114.033499093715));
#227143=CARTESIAN_POINT('Ctrl Pts',(-3.94709149943844,6.85597898790885,
114.033805284475));
#227144=CARTESIAN_POINT('Ctrl Pts',(-3.95982634105648,6.84863098720405,
114.034394814258));
#227145=CARTESIAN_POINT('Ctrl Pts',(-3.96594933339578,6.84508706558619,
114.034678199114));
#227146=CARTESIAN_POINT('Ctrl Pts',(-3.98040888461964,6.83669211984154,
114.035347266919));
#227147=CARTESIAN_POINT('Ctrl Pts',(-3.98874135087479,6.83183404854993,
114.035732705804));
#227148=CARTESIAN_POINT('Ctrl Pts',(-4.01774923103656,6.81485044707601,
114.037074135406));
#227149=CARTESIAN_POINT('Ctrl Pts',(-4.0383784969098,6.80264614893191,114.038027394298));
#227150=CARTESIAN_POINT('Ctrl Pts',(-4.2863791308345,6.65440298682244,114.049479294935));
#227151=CARTESIAN_POINT('Ctrl Pts',(-4.50684187677284,6.50711272365055,
114.059570954346));
#227152=CARTESIAN_POINT('Ctrl Pts',(-5.23717595321437,5.96422343360179,
114.093108797631));
#227153=CARTESIAN_POINT('Ctrl Pts',(-5.70581632969501,5.51757399025604,
114.114649427063));
#227154=CARTESIAN_POINT('Ctrl Pts',(-6.24129167229568,4.86516230569001,
114.144210619873));
#227155=CARTESIAN_POINT('Ctrl Pts',(-6.36169656723498,4.70662700340428,
114.151287719837));
#227156=CARTESIAN_POINT('Ctrl Pts',(-6.55790251242576,4.42698251285291,
114.16384876517));
#227157=CARTESIAN_POINT('Ctrl Pts',(-6.63663822890178,4.308049372721,114.169213909542));
#227158=CARTESIAN_POINT('Ctrl Pts',(-6.75063307453688,4.12530857840029,
114.177576742986));
#227159=CARTESIAN_POINT('Ctrl Pts',(-6.78829692042551,4.06303356582502,
114.180448362466));
#227160=CARTESIAN_POINT('Ctrl Pts',(-6.83194371453909,3.98856484667433,
114.183900906737));
#227161=CARTESIAN_POINT('Ctrl Pts',(-6.83876255775517,3.97686197026392,
114.18444401212));
#227162=CARTESIAN_POINT('Ctrl Pts',(-6.84921110549794,3.95882325308944,
114.185281905799));
#227163=CARTESIAN_POINT('Ctrl Pts',(-6.85286216801887,3.9524997688279,114.185575772447));
#227164=CARTESIAN_POINT('Ctrl Pts',(-6.85923494263708,3.94142702139087,
114.186090586076));
#227165=CARTESIAN_POINT('Ctrl Pts',(-6.86196049324754,3.93667996567686,
114.186311370902));
#227166=CARTESIAN_POINT('Ctrl Pts',(-6.86810481870518,3.92595270605843,
114.18681046046));
#227167=CARTESIAN_POINT('Ctrl Pts',(-6.87152071200877,3.9199708614996,114.187088884494));
#227168=CARTESIAN_POINT('Ctrl Pts',(-6.88069932929613,3.90384858534741,
114.187839592956));
#227169=CARTESIAN_POINT('Ctrl Pts',(-6.88644743629607,3.89369987838445,
114.188312470227));
#227170=CARTESIAN_POINT('Ctrl Pts',(-6.91172589162478,3.84883783117163,
114.190404103119));
#227171=CARTESIAN_POINT('Ctrl Pts',(-6.93101618851922,3.81399029666978,
114.192032231833));
#227172=CARTESIAN_POINT('Ctrl Pts',(-6.95945928513589,3.76167995516114,
114.194479858436));
#227173=CARTESIAN_POINT('Ctrl Pts',(-6.96881145293289,3.74432591436242,
114.195292452261));
#227174=CARTESIAN_POINT('Ctrl Pts',(-6.98080365893185,3.72187241110995,
114.19634443735));
#227175=CARTESIAN_POINT('Ctrl Pts',(-6.98350318553716,3.71680470654052,
114.19658190811));
#227176=CARTESIAN_POINT('Ctrl Pts',(-7.25257773447291,3.21035466999441,
114.220317695055));
#227177=CARTESIAN_POINT('Ctrl Pts',(-7.46421101672682,2.68175804945603,
114.245273218623));
#227178=CARTESIAN_POINT('Ctrl Pts',(-7.72799653396587,1.74063006208821,
114.28720414022));
#227179=CARTESIAN_POINT('Ctrl Pts',(-7.80775184094904,1.33819215334711,
114.304447118835));
#227180=CARTESIAN_POINT('Ctrl Pts',(-7.8926253055992,0.622299896547812,
114.334199202781));
#227181=CARTESIAN_POINT('Ctrl Pts',(-7.91099712768033,0.31132281523364,
114.346883831773));
#227182=CARTESIAN_POINT('Ctrl Pts',(-7.91100046921692,-0.0508125362661093,
114.361542464529));
#227183=CARTESIAN_POINT('Ctrl Pts',(-7.91050997602132,-0.101697042451125,
114.363598538078));
#227184=CARTESIAN_POINT('Ctrl Pts',(-7.90892569116772,-0.183827639839791,
114.366911308835));
#227185=CARTESIAN_POINT('Ctrl Pts',(-7.90813755703808,-0.215078070272413,
114.368170440797));
#227186=CARTESIAN_POINT('Ctrl Pts',(-7.90640767271903,-0.27060871720694,
114.370405473599));
#227187=CARTESIAN_POINT('Ctrl Pts',(-7.90553924734589,-0.29489078910114,
114.37138198172));
#227188=CARTESIAN_POINT('Ctrl Pts',(-7.90347359279863,-0.346048993979574,
114.373437641103));
#227189=CARTESIAN_POINT('Ctrl Pts',(-7.90225110803007,-0.372923811469791,
114.374516559514));
#227190=CARTESIAN_POINT('Ctrl Pts',(-7.89864173147062,-0.444254149842892,
114.377377677623));
#227191=CARTESIAN_POINT('Ctrl Pts',(-7.89601662118153,-0.488696730055696,
114.379157707979));
#227192=CARTESIAN_POINT('Ctrl Pts',(-7.88146242786094,-0.70417839197012,
114.38777651036));
#227193=CARTESIAN_POINT('Ctrl Pts',(-7.86435017178404,-0.874822803298755,
114.394565005318));
#227194=CARTESIAN_POINT('Ctrl Pts',(-7.79933150743108,-1.36282810323231,
114.413924157409));
#227195=CARTESIAN_POINT('Ctrl Pts',(-7.73764604538597,-1.67800794404747,
114.426351899085));
#227196=CARTESIAN_POINT('Ctrl Pts',(-7.55364373798267,-2.38650791108691,
114.45465010542));
#227197=CARTESIAN_POINT('Ctrl Pts',(-7.41943633296866,-2.77576993859876,
114.470455242708));
#227198=CARTESIAN_POINT('Ctrl Pts',(-7.23868404502707,-3.19173533043536,
114.488530549082));
#227199=CARTESIAN_POINT('Ctrl Pts',(-7.22146232733047,-3.23051124955968,
114.490227592927));
#227200=CARTESIAN_POINT('Ctrl Pts',(-7.19724409067357,-3.28387884023547,
114.49258145412));
#227201=CARTESIAN_POINT('Ctrl Pts',(-7.1905133918184,-3.29859059257909,
114.493232262768));
#227202=CARTESIAN_POINT('Ctrl Pts',(-7.1796826728208,-3.32207336707161,
114.494274252522));
#227203=CARTESIAN_POINT('Ctrl Pts',(-7.17561158635427,-3.33085771232942,
114.494664748293));
#227204=CARTESIAN_POINT('Ctrl Pts',(-7.16720107313771,-3.34891843119276,
114.495469105643));
#227205=CARTESIAN_POINT('Ctrl Pts',(-7.16285973944643,-3.3581938946182,
114.495883013033));
#227206=CARTESIAN_POINT('Ctrl Pts',(-7.15274585166959,-3.3796938532829,
114.496844347737));
#227207=CARTESIAN_POINT('Ctrl Pts',(-7.14695995511448,-3.39191202107821,
114.497392108035));
#227208=CARTESIAN_POINT('Ctrl Pts',(-7.1274692568734,-3.43279954928797,
114.499230129098));
#227209=CARTESIAN_POINT('Ctrl Pts',(-7.11362312090812,-3.46140099088234,
114.500524080103));
#227210=CARTESIAN_POINT('Ctrl Pts',(-7.07964453918537,-3.53052425123799,
114.503670429529));
#227211=CARTESIAN_POINT('Ctrl Pts',(-7.0593360745306,-3.570958193539,114.505526970269));
#227212=CARTESIAN_POINT('Ctrl Pts',(-6.98030617585935,-3.724996727436,114.512657758108));
#227213=CARTESIAN_POINT('Ctrl Pts',(-6.91918074534351,-3.83734437446094,
114.517980038605));
#227214=CARTESIAN_POINT('Ctrl Pts',(-6.64325322131385,-4.31644928591205,
114.54112408142));
#227215=CARTESIAN_POINT('Ctrl Pts',(-6.40181229919149,-4.66704992478172,
114.55917947104));
#227216=CARTESIAN_POINT('Ctrl Pts',(-6.03798316807709,-5.11365739297227,
114.583231000718));
#227217=CARTESIAN_POINT('Ctrl Pts',(-5.9392548849071,-5.22800011441727,
114.589497903788));
#227218=CARTESIAN_POINT('Ctrl Pts',(-5.73509946839674,-5.45119154951351,
114.601951298568));
#227219=CARTESIAN_POINT('Ctrl Pts',(-5.6296974057503,-5.55997874241855,
114.608134961385));
#227220=CARTESIAN_POINT('Ctrl Pts',(-5.4931507360499,-5.69304434150861,
114.615854916244));
#227221=CARTESIAN_POINT('Ctrl Pts',(-5.46486202839355,-5.72020470927214,
114.617439268702));
#227222=CARTESIAN_POINT('Ctrl Pts',(-5.41964247483699,-5.76297898451397,
114.61994856147));
#227223=CARTESIAN_POINT('Ctrl Pts',(-5.40284345820501,-5.77873116709164,
114.620875735899));
#227224=CARTESIAN_POINT('Ctrl Pts',(-5.37134716496034,-5.80800736276362,
114.622604836508));
#227225=CARTESIAN_POINT('Ctrl Pts',(-5.35666699918144,-5.82154949778256,
114.623407046012));
#227226=CARTESIAN_POINT('Ctrl Pts',(-5.32383260523814,-5.85160916203313,
114.625193148465));
#227227=CARTESIAN_POINT('Ctrl Pts',(-5.30565246171449,-5.86809810367799,
114.626176589886));
#227228=CARTESIAN_POINT('Ctrl Pts',(-5.25208407361887,-5.91623085345773,
114.629058449194));
#227229=CARTESIAN_POINT('Ctrl Pts',(-5.21648729321816,-5.94764112760066,
114.6309533053));
#227230=CARTESIAN_POINT('Ctrl Pts',(-4.89860821440357,-6.22308552634251,
114.647702296468));
#227231=CARTESIAN_POINT('Ctrl Pts',(-4.59966312507277,-6.44719047553382,
114.662295929651));
#227232=CARTESIAN_POINT('Ctrl Pts',(-3.98780530654852,-6.84157948303174,
114.690517662134));
#227233=CARTESIAN_POINT('Ctrl Pts',(-3.67699450072474,-7.01352428025668,
114.704039301233));
#227234=CARTESIAN_POINT('Ctrl Pts',(-2.90838226381092,-7.37354820581,114.735989960386));
#227235=CARTESIAN_POINT('Ctrl Pts',(-2.44245500137967,-7.54070850188199,
114.75415341825));
#227236=CARTESIAN_POINT('Ctrl Pts',(-1.79381878329526,-7.70694497782435,
114.779815810314));
#227237=CARTESIAN_POINT('Ctrl Pts',(-1.62223196417972,-7.74487870719792,
114.786648708209));
#227238=CARTESIAN_POINT('Ctrl Pts',(-1.43006646431055,-7.78069553055407,
114.794455046235));
#227239=CARTESIAN_POINT('Ctrl Pts',(-1.41058842887558,-7.78425033694811,
114.795248061723));
#227240=CARTESIAN_POINT('Ctrl Pts',(-1.38227864882495,-7.78930722130641,
114.796403410766));
#227241=CARTESIAN_POINT('Ctrl Pts',(-1.37345729974141,-7.79086749315856,
114.79676380772));
#227242=CARTESIAN_POINT('Ctrl Pts',(-1.35790419708779,-7.79359120441833,
114.797399940862));
#227243=CARTESIAN_POINT('Ctrl Pts',(-1.35117354281084,-7.79476091531577,
114.797675463623));
#227244=CARTESIAN_POINT('Ctrl Pts',(-1.33727320503375,-7.79715809036756,
114.798244976801));
#227245=CARTESIAN_POINT('Ctrl Pts',(-1.33010332842332,-7.79838438693538,
114.798539007233));
#227246=CARTESIAN_POINT('Ctrl Pts',(-1.31177986011599,-7.80149232787706,
114.799291150671));
#227247=CARTESIAN_POINT('Ctrl Pts',(-1.30062392565899,-7.80335993952415,
114.799749755957));
#227248=CARTESIAN_POINT('Ctrl Pts',(-1.25534861128635,-7.81083967913317,
114.801613813791));
#227249=CARTESIAN_POINT('Ctrl Pts',(-1.22119691350172,-7.81625195857195,
114.803026458787));
#227250=CARTESIAN_POINT('Ctrl Pts',(-1.01052729553345,-7.84822397240568,
114.811785888706));
#227251=CARTESIAN_POINT('Ctrl Pts',(-0.833216060158749,-7.86902304349495,
114.81938451316));
#227252=CARTESIAN_POINT('Ctrl Pts',(-0.3765139858485,-7.9069874257473,114.839444543487));
#227253=CARTESIAN_POINT('Ctrl Pts',(-0.0966461626634426,-7.91535594265123,
114.852157377885));
#227254=CARTESIAN_POINT('Ctrl Pts',(0.937484913179871,-7.89141940733783,
114.899502089259));
#227255=CARTESIAN_POINT('Ctrl Pts',(1.68568462350727,-7.76609480531195,
114.934036512435));
#227256=CARTESIAN_POINT('Ctrl Pts',(2.44924172806315,-7.52245361173462,
114.966812755988));
#227257=CARTESIAN_POINT('Ctrl Pts',(2.49351924675345,-7.50789286319354,
114.968706149439));
#227258=CARTESIAN_POINT('Ctrl Pts',(2.55072611703099,-7.48851837192134,
114.971143230204));
#227259=CARTESIAN_POINT('Ctrl Pts',(2.56377469014718,-7.48406109484297,
114.971698492594));
#227260=CARTESIAN_POINT('Ctrl Pts',(2.5845299208604,-7.47691064086798,114.972580718251));
#227261=CARTESIAN_POINT('Ctrl Pts',(2.5922441501592,-7.47423962084607,114.972908404333));
#227262=CARTESIAN_POINT('Ctrl Pts',(2.60608871014328,-7.46942198723165,
114.973496109205));
#227263=CARTESIAN_POINT('Ctrl Pts',(2.61222055198045,-7.46727975748451,
114.973756271118));
#227264=CARTESIAN_POINT('Ctrl Pts',(2.62653787897491,-7.46225804054248,
114.974363410327));
#227265=CARTESIAN_POINT('Ctrl Pts',(2.63472128604847,-7.45937263037536,
114.974710193086));
#227266=CARTESIAN_POINT('Ctrl Pts',(2.65809872577036,-7.45108664477432,
114.975700156336));
#227267=CARTESIAN_POINT('Ctrl Pts',(2.67328105538915,-7.44565305575614,
114.976342251259));
#227268=CARTESIAN_POINT('Ctrl Pts',(2.77002942598582,-7.4106938098248,114.980428737664));
#227269=CARTESIAN_POINT('Ctrl Pts',(2.851123231997,-7.37987416389321,114.983830204505));
#227270=CARTESIAN_POINT('Ctrl Pts',(3.08821746960157,-7.28527509247047,
114.993712601705));
#227271=CARTESIAN_POINT('Ctrl Pts',(3.24270856101847,-7.21783661557888,
115.000070366208));
#227272=CARTESIAN_POINT('Ctrl Pts',(3.57225493447896,-7.06126449634528,
115.013522514855));
#227273=CARTESIAN_POINT('Ctrl Pts',(3.7463834905061,-6.97044309740656,115.020560176763));
#227274=CARTESIAN_POINT('Ctrl Pts',(4.36351771523466,-6.61874711751563,
115.045523529907));
#227275=CARTESIAN_POINT('Ctrl Pts',(4.78419632755308,-6.32135644391238,
115.062505885464));
#227276=CARTESIAN_POINT('Ctrl Pts',(5.45076177937666,-5.74524609382843,
115.093120893189));
#227277=CARTESIAN_POINT('Ctrl Pts',(5.711406248275,-5.4862048937083,115.106318667656));
#227278=CARTESIAN_POINT('Ctrl Pts',(5.96910558537377,-5.19175211594869,
115.121868938784));
#227279=CARTESIAN_POINT('Ctrl Pts',(5.98502505642458,-5.17339217272492,
115.122840685189));
#227280=CARTESIAN_POINT('Ctrl Pts',(6.00565662369404,-5.14937508001318,
115.124115037774));
#227281=CARTESIAN_POINT('Ctrl Pts',(6.01044591369807,-5.14378412398889,
115.124411918834));
#227282=CARTESIAN_POINT('Ctrl Pts',(6.01779918117103,-5.13517572183373,
115.124869383742));
#227283=CARTESIAN_POINT('Ctrl Pts',(6.02036871951092,-5.13216300988515,
115.125029551333));
#227284=CARTESIAN_POINT('Ctrl Pts',(6.02546392776124,-5.12617992830821,
115.125347771049));
#227285=CARTESIAN_POINT('Ctrl Pts',(6.02798966610444,-5.12320961774751,
115.125505817956));
#227286=CARTESIAN_POINT('Ctrl Pts',(6.03355916207464,-5.116649976845,115.125854997987));
#227287=CARTESIAN_POINT('Ctrl Pts',(6.03660191276698,-5.11305979765488,
115.126046207096));
#227288=CARTESIAN_POINT('Ctrl Pts',(6.04529845321364,-5.10278005867984,
115.126593982228));
#227289=CARTESIAN_POINT('Ctrl Pts',(6.05094433659836,-5.09608382495479,
115.12695115145));
#227290=CARTESIAN_POINT('Ctrl Pts',(6.09004190623342,-5.04955603463053,
115.129435390882));
#227291=CARTESIAN_POINT('Ctrl Pts',(6.12311041011407,-5.00940567598472,
115.131591718052));
#227292=CARTESIAN_POINT('Ctrl Pts',(6.16041664094631,-4.96318872376782,
115.134084807249));
#227293=CARTESIAN_POINT('Ctrl Pts',(6.1650454140451,-4.95743790076046,115.134395216588));
#227294=CARTESIAN_POINT('Ctrl Pts',(6.25646955912382,-4.84352577820048,
115.140547420832));
#227295=CARTESIAN_POINT('Ctrl Pts',(6.34041004262891,-4.73311209194905,
115.146574958172));
#227296=CARTESIAN_POINT('Ctrl Pts',(6.70929675339811,-4.2204530329368,115.174608850229));
#227297=CARTESIAN_POINT('Ctrl Pts',(6.9591632550898,-3.79432834520779,115.197960311305));
#227298=CARTESIAN_POINT('Ctrl Pts',(7.32433485857248,-3.01246723627982,
115.237768744965));
#227299=CARTESIAN_POINT('Ctrl Pts',(7.45721630304886,-2.66661001770044,
115.254462095115));
#227300=CARTESIAN_POINT('Ctrl Pts',(7.6245880294134,-2.11909436696631,115.279029475194));
#227301=CARTESIAN_POINT('Ctrl Pts',(7.67631916182465,-1.92328788684706,
115.287471164522));
#227302=CARTESIAN_POINT('Ctrl Pts',(7.72494900949725,-1.7057264475141,115.296477684661));
#227303=CARTESIAN_POINT('Ctrl Pts',(7.7293362380623,-1.68573462943908,115.297301898305));
#227304=CARTESIAN_POINT('Ctrl Pts',(7.73541365628183,-1.65751834239886,
115.298460429486));
#227305=CARTESIAN_POINT('Ctrl Pts',(7.73716839406809,-1.64930795535596,
115.298796972283));
#227306=CARTESIAN_POINT('Ctrl Pts',(7.74019960232129,-1.63501368762621,
115.29938190912));
#227307=CARTESIAN_POINT('Ctrl Pts',(7.74148197679239,-1.6289310745878,115.299630506517));
#227308=CARTESIAN_POINT('Ctrl Pts',(7.74414362495616,-1.61623209796531,
115.300148871166));
#227309=CARTESIAN_POINT('Ctrl Pts',(7.74552159236152,-1.60961546371343,
115.30041859325));
#227310=CARTESIAN_POINT('Ctrl Pts',(7.74876083397874,-1.59396100456534,
115.301055874813));
#227311=CARTESIAN_POINT('Ctrl Pts',(7.75061477999538,-1.58492166342505,
115.30142318172));
#227312=CARTESIAN_POINT('Ctrl Pts',(7.75668470957422,-1.55506096923214,
115.302634319699));
#227313=CARTESIAN_POINT('Ctrl Pts',(7.76083265746889,-1.5342257898421,115.303475809457));
#227314=CARTESIAN_POINT('Ctrl Pts',(7.80436195135305,-1.31088347060548,
115.312458259013));
#227315=CARTESIAN_POINT('Ctrl Pts',(7.8358929832383,-1.10691920188111,115.320324773723));
#227316=CARTESIAN_POINT('Ctrl Pts',(7.87146680556487,-0.796933974362133,
115.331859772975));
#227317=CARTESIAN_POINT('Ctrl Pts',(7.88141221054073,-0.691690605637102,
115.335704055763));
#227318=CARTESIAN_POINT('Ctrl Pts',(7.92519909013768,-0.102472081404216,
115.356889971864));
#227319=CARTESIAN_POINT('Ctrl Pts',(7.91657251543921,0.383626567769483,
115.373017014852));
#227320=CARTESIAN_POINT('Ctrl Pts',(7.81257706791243,1.32808098499041,115.405217440915));
#227321=CARTESIAN_POINT('Ctrl Pts',(7.72103087389865,1.78486438183143,115.421237306732));
#227322=CARTESIAN_POINT('Ctrl Pts',(7.5814368592811,2.25978818781267,115.440804056808));
#227323=CARTESIAN_POINT('Ctrl Pts',(7.5727816181309,2.2886253560514,115.44200402192));
#227324=CARTESIAN_POINT('Ctrl Pts',(7.56174866143145,2.32463658987252,115.443518233396));
#227325=CARTESIAN_POINT('Ctrl Pts',(7.55952489017749,2.3318579561401,115.443822672566));
#227326=CARTESIAN_POINT('Ctrl Pts',(7.55601148934728,2.34320935754085,115.444302490332));
#227327=CARTESIAN_POINT('Ctrl Pts',(7.5547288092541,2.34734154710282,115.444477419813));
#227328=CARTESIAN_POINT('Ctrl Pts',(7.55235105870395,2.35497940012985,115.444801241424));
#227329=CARTESIAN_POINT('Ctrl Pts',(7.55125693327885,2.35848536490217,115.444950072884));
#227330=CARTESIAN_POINT('Ctrl Pts',(7.54882640371201,2.36625461187455,115.445280302166));
#227331=CARTESIAN_POINT('Ctrl Pts',(7.54748882951831,2.3705175236068,115.445461774653));
#227332=CARTESIAN_POINT('Ctrl Pts',(7.5436587975669,2.38268791211798,115.445980660677));
#227333=CARTESIAN_POINT('Ctrl Pts',(7.54115752588845,2.39059258539437,115.446318632273));
#227334=CARTESIAN_POINT('Ctrl Pts',(7.52525967482702,2.44056072077617,115.448461039643));
#227335=CARTESIAN_POINT('Ctrl Pts',(7.51152388379876,2.48251457098658,115.450286620838));
#227336=CARTESIAN_POINT('Ctrl Pts',(7.46912290988269,2.60844743199752,115.455842432686));
#227337=CARTESIAN_POINT('Ctrl Pts',(7.43939589865643,2.69205917474495,115.459633388966));
#227338=CARTESIAN_POINT('Ctrl Pts',(7.34878770878699,2.93393795262027,115.470861755087));
#227339=CARTESIAN_POINT('Ctrl Pts',(7.28421851391765,3.09076490238342,115.478471561948));
#227340=CARTESIAN_POINT('Ctrl Pts',(7.06360205280373,3.58120665738194,115.503058170901));
#227341=CARTESIAN_POINT('Ctrl Pts',(6.88928045816948,3.90606218817292,115.520512853899));
#227342=CARTESIAN_POINT('Ctrl Pts',(6.44984367420417,4.60341273534195,115.559146806795));
#227343=CARTESIAN_POINT('Ctrl Pts',(6.17378840619966,4.96752538413764,115.580117856845));
#227344=CARTESIAN_POINT('Ctrl Pts',(5.71213461696114,5.47807950511128,115.609922011658));
#227345=CARTESIAN_POINT('Ctrl Pts',(5.54888647996662,5.64337740120692,115.619659140253));
#227346=CARTESIAN_POINT('Ctrl Pts',(5.36252565471285,5.81616021112204,115.629950841878));
#227347=CARTESIAN_POINT('Ctrl Pts',(5.34639762526163,5.83098906206626,115.630835126201));
#227348=CARTESIAN_POINT('Ctrl Pts',(5.32366395247655,5.85171782919558,115.632072721508));
#227349=CARTESIAN_POINT('Ctrl Pts',(5.3171097627054,5.85767387308551,115.632428496));
#227350=CARTESIAN_POINT('Ctrl Pts',(5.30572040596201,5.86798895305928,115.633044956603));
#227351=CARTESIAN_POINT('Ctrl Pts',(5.30088984063395,5.87235304432713,115.633305863545));
#227352=CARTESIAN_POINT('Ctrl Pts',(5.29082975811026,5.88141912526233,115.633848080099));
#227353=CARTESIAN_POINT('Ctrl Pts',(5.28559934546498,5.88612011565128,115.634129346137));
#227354=CARTESIAN_POINT('Ctrl Pts',(5.27327303863231,5.89716907575898,115.634790689271));
#227355=CARTESIAN_POINT('Ctrl Pts',(5.26617193218292,5.90351122888612,115.635170513975));
#227356=CARTESIAN_POINT('Ctrl Pts',(5.24294311845491,5.92418212675156,115.636409174016));
#227357=CARTESIAN_POINT('Ctrl Pts',(5.2267681802668,5.93845778074769,115.637265718514));
#227358=CARTESIAN_POINT('Ctrl Pts',(4.90890585901931,6.21669150221918,115.653982543674));
#227359=CARTESIAN_POINT('Ctrl Pts',(4.58763028114866,6.45742226445213,115.668805236461));
#227360=CARTESIAN_POINT('Ctrl Pts',(3.84874103221612,6.92797366636466,115.699914436927));
#227361=CARTESIAN_POINT('Ctrl Pts',(3.42585608702336,7.14654630848013,115.715891152156));
#227362=CARTESIAN_POINT('Ctrl Pts',(2.65945964723125,7.45891946632256,115.744974653488));
#227363=CARTESIAN_POINT('Ctrl Pts',(2.32446287689067,7.57001238927081,115.757778891481));
#227364=CARTESIAN_POINT('Ctrl Pts',(1.95338339815199,7.6661046700647,115.772993485803));
#227365=CARTESIAN_POINT('Ctrl Pts',(1.92355587959227,7.67364321910505,115.774222301238));
#227366=CARTESIAN_POINT('Ctrl Pts',(1.88366756217731,7.68347733601705,115.775872834761));
#227367=CARTESIAN_POINT('Ctrl Pts',(1.87364489326573,7.68592754783054,115.776288170449));
#227368=CARTESIAN_POINT('Ctrl Pts',(1.85799114219552,7.68972193458691,115.776937781258));
#227369=CARTESIAN_POINT('Ctrl Pts',(1.85236330768408,7.6910795530839,115.777171515743));
#227370=CARTESIAN_POINT('Ctrl Pts',(1.84108768430507,7.6937865097095,115.777640181255));
#227371=CARTESIAN_POINT('Ctrl Pts',(1.83543989002038,7.69513580959907,115.777875113618));
#227372=CARTESIAN_POINT('Ctrl Pts',(1.82270017870578,7.69816459778535,115.77840545977));
#227373=CARTESIAN_POINT('Ctrl Pts',(1.81560742108134,7.69984050536865,115.778701013114));
#227374=CARTESIAN_POINT('Ctrl Pts',(1.79601233838172,7.70444193614334,115.779518310111));
#227375=CARTESIAN_POINT('Ctrl Pts',(1.78350522149186,7.70734681907788,115.780040843859));
#227376=CARTESIAN_POINT('Ctrl Pts',(1.69848191329918,7.72687615818212,115.783598731874));
#227377=CARTESIAN_POINT('Ctrl Pts',(1.62574269991136,7.74250710207346,115.786670737522));
#227378=CARTESIAN_POINT('Ctrl Pts',(1.39330975624231,7.78903484342039,115.796558288458));
#227379=CARTESIAN_POINT('Ctrl Pts',(1.23288190322035,7.81603320176458,115.803488669266));
#227380=CARTESIAN_POINT('Ctrl Pts',(0.644976039080087,7.89642074702735,
115.829072779577));
#227381=CARTESIAN_POINT('Ctrl Pts',(0.214158742873291,7.91982289611658,
115.848137723667));
#227382=CARTESIAN_POINT('Ctrl Pts',(-0.4142838620456,7.90262418194324,115.875459685748));
#227383=CARTESIAN_POINT('Ctrl Pts',(-0.611877672184438,7.88978511101164,
115.883987302897));
#227384=CARTESIAN_POINT('Ctrl Pts',(-1.11963246733086,7.83760105803829,
115.90568466056));
#227385=CARTESIAN_POINT('Ctrl Pts',(-1.42832365770927,7.78726365027231,
115.918657643377));
#227386=CARTESIAN_POINT('Ctrl Pts',(-1.76737409262188,7.71113050203308,
115.932728466672));
#227387=CARTESIAN_POINT('Ctrl Pts',(-1.80145605158341,7.70323963795825,
115.934141072386));
#227388=CARTESIAN_POINT('Ctrl Pts',(-1.85209442092933,7.69116108510853,
115.936237282013));
#227389=CARTESIAN_POINT('Ctrl Pts',(-1.86869136720885,7.68714544924807,
115.936923897418));
#227390=CARTESIAN_POINT('Ctrl Pts',(-1.89711651343863,7.68017047944249,
115.938099106876));
#227391=CARTESIAN_POINT('Ctrl Pts',(-1.9089510932208,7.67723748385643,115.938588176066));
#227392=CARTESIAN_POINT('Ctrl Pts',(-1.93325217684861,7.67115521617233,
115.939591975422));
#227393=CARTESIAN_POINT('Ctrl Pts',(-1.94571788080572,7.66800288597811,
115.940106647775));
#227394=CARTESIAN_POINT('Ctrl Pts',(-1.97030940848329,7.66172034641187,
115.941121473797));
#227395=CARTESIAN_POINT('Ctrl Pts',(-1.98243559403818,7.65859170790232,
115.941621655067));
#227396=CARTESIAN_POINT('Ctrl Pts',(-2.01033869523115,7.65132180668212,
115.942772065033));
#227397=CARTESIAN_POINT('Ctrl Pts',(-2.0261103484449,7.64716051337231,115.943421913879));
#227398=CARTESIAN_POINT('Ctrl Pts',(-2.11003254448707,7.62474009655097,
115.946877705694));
#227399=CARTESIAN_POINT('Ctrl Pts',(-2.17795000157489,7.60561850654065,
115.949667001964));
#227400=CARTESIAN_POINT('Ctrl Pts',(-2.35064869761054,7.55449358164935,
115.956741737866));
#227401=CARTESIAN_POINT('Ctrl Pts',(-2.45503826509474,7.52121734984968,
115.961001091233));
#227402=CARTESIAN_POINT('Ctrl Pts',(-2.82084914964607,7.39618006234371,
115.975882508051));
#227403=CARTESIAN_POINT('Ctrl Pts',(-3.07811094143381,7.29286715493864,
115.986257694316));
#227404=CARTESIAN_POINT('Ctrl Pts',(-3.53236907042016,7.08211398175384,
116.004707874759));
#227405=CARTESIAN_POINT('Ctrl Pts',(-3.73122345337743,6.97939414065008,
116.012835405181));
#227406=CARTESIAN_POINT('Ctrl Pts',(-4.2607608151437,6.676749982985,116.035016948536));
#227407=CARTESIAN_POINT('Ctrl Pts',(-4.58156305601182,6.46082964463733,
116.049039398213));
#227408=CARTESIAN_POINT('Ctrl Pts',(-4.95707818367383,6.16600567789951,
116.067524435051));
#227409=CARTESIAN_POINT('Ctrl Pts',(-5.02787918340899,6.10841061142607,
116.071110021645));
#227410=CARTESIAN_POINT('Ctrl Pts',(-5.10822900128518,6.04070428617413,
116.075315419447));
#227411=CARTESIAN_POINT('Ctrl Pts',(-5.11876863511714,6.03177581308082,
116.075869800701));
#227412=CARTESIAN_POINT('Ctrl Pts',(-5.13434742505062,6.01850826523902,
116.076693412202));
#227413=CARTESIAN_POINT('Ctrl Pts',(-5.13940461769222,6.01419033579106,
116.07696142748));
#227414=CARTESIAN_POINT('Ctrl Pts',(-5.14837196697733,6.00651426836845,
116.077437842975));
#227415=CARTESIAN_POINT('Ctrl Pts',(-5.15228430176099,6.00315867190863,
116.077646094546));
#227416=CARTESIAN_POINT('Ctrl Pts',(-5.16048215338354,5.99611348486725,
116.078083303486));
#227417=CARTESIAN_POINT('Ctrl Pts',(-5.16476699766767,5.99242311910205,
116.078312306806));
#227418=CARTESIAN_POINT('Ctrl Pts',(-5.17343162351136,5.98494442504219,
116.07877637497));
#227419=CARTESIAN_POINT('Ctrl Pts',(-5.17781120930317,5.98115587612727,
116.079011453085));
#227420=CARTESIAN_POINT('Ctrl Pts',(-5.18857665790152,5.97182256842947,
116.079590570088));
#227421=CARTESIAN_POINT('Ctrl Pts',(-5.19495778629881,5.96627238076075,
116.079934940573));
#227422=CARTESIAN_POINT('Ctrl Pts',(-5.25904919593762,5.91034608013402,
116.083405018026));
#227423=CARTESIAN_POINT('Ctrl Pts',(-5.31602874442575,5.85914895132501,
116.086584565166));
#227424=CARTESIAN_POINT('Ctrl Pts',(-5.54270233925726,5.64945023392989,
116.099607814317));
#227425=CARTESIAN_POINT('Ctrl Pts',(-5.70611451665905,5.48434872308587,
116.109848377242));
#227426=CARTESIAN_POINT('Ctrl Pts',(-5.9717239372144,5.19125459972362,116.127680049546));
#227427=CARTESIAN_POINT('Ctrl Pts',(-6.07765080057738,5.06683034454545,
116.135153206328));
#227428=CARTESIAN_POINT('Ctrl Pts',(-6.55156443883811,4.47389869719932,
116.170057294602));
#227429=CARTESIAN_POINT('Ctrl Pts',(-6.86977708828372,3.9680049032834,116.197694417281));
#227430=CARTESIAN_POINT('Ctrl Pts',(-7.14033791464335,3.40591840761649,
116.22467221222));
#227431=CARTESIAN_POINT('Ctrl Pts',(-7.15235368251749,3.38061274829772,
116.225879766427));
#227432=CARTESIAN_POINT('Ctrl Pts',(-7.25694358293501,3.15728869501609,
116.236474574776));
#227433=CARTESIAN_POINT('Ctrl Pts',(-7.34141195291808,2.95556800409414,
116.245613599181));
#227434=CARTESIAN_POINT('Ctrl Pts',(-7.42471026007466,2.73094086926193,
116.255332104383));
#227435=CARTESIAN_POINT('Ctrl Pts',(-7.43192106652402,2.71125611974983,
116.25618001467));
#227436=CARTESIAN_POINT('Ctrl Pts',(-7.442502820251,2.68200961042053,116.2574342728));
#227437=CARTESIAN_POINT('Ctrl Pts',(-7.44593374286168,2.67246973372288,
116.257842528636));
#227438=CARTESIAN_POINT('Ctrl Pts',(-7.45177158504158,2.65613876814522,
116.258539927045));
#227439=CARTESIAN_POINT('Ctrl Pts',(-7.45418757906757,2.64935094838669,
116.258829357858));
#227440=CARTESIAN_POINT('Ctrl Pts',(-7.45886631476097,2.63614881250399,
116.259391447375));
#227441=CARTESIAN_POINT('Ctrl Pts',(-7.46113006359658,2.62973486069258,
116.2596641379));
#227442=CARTESIAN_POINT('Ctrl Pts',(-7.46651907194479,2.61440303771855,
116.260315050352));
#227443=CARTESIAN_POINT('Ctrl Pts',(-7.46963663348633,2.60548246199862,
116.260693027836));
#227444=CARTESIAN_POINT('Ctrl Pts',(-7.47891497420166,2.57877993637777,
116.261822231897));
#227445=CARTESIAN_POINT('Ctrl Pts',(-7.48502831331312,2.56098151233283,
116.262571955318));
#227446=CARTESIAN_POINT('Ctrl Pts',(-7.53686705025708,2.40828651131292,
116.268978972365));
#227447=CARTESIAN_POINT('Ctrl Pts',(-7.57900629934637,2.27219603766529,
116.274521986621));
#227448=CARTESIAN_POINT('Ctrl Pts',(-7.71591282562359,1.78373693304042,
116.293881111327));
#227449=CARTESIAN_POINT('Ctrl Pts',(-7.78996080841559,1.42603134276949,
116.307056744525));
#227450=CARTESIAN_POINT('Ctrl Pts',(-7.88696644315222,0.711657536121887,
116.332372618769));
#227451=CARTESIAN_POINT('Ctrl Pts',(-7.91100122708638,0.356016607322614,
116.344506208184));
#227452=CARTESIAN_POINT('Ctrl Pts',(-7.91099999995301,-2.72658871074832E-5,
116.356884209101));
#227453=CARTESIAN_POINT('',(-7.91099986567554,0.00144650702262969,118.357610289563));
#227454=CARTESIAN_POINT('Ctrl Pts',(-7.911,-1.68698388591793E-12,116.357668491763));
#227455=CARTESIAN_POINT('Ctrl Pts',(-7.91099999999953,-2.20167589666848,
116.446255927496));
#227456=CARTESIAN_POINT('Ctrl Pts',(-6.94214576672275,-4.38610418338837,
116.534843363229));
#227457=CARTESIAN_POINT('Ctrl Pts',(-3.67820201488119,-7.34180684107717,
116.712018234694));
#227458=CARTESIAN_POINT('Ctrl Pts',(-1.40868175871556,-8.0899266657137,
116.800605670427));
#227459=CARTESIAN_POINT('Ctrl Pts',(2.97309270521457,-7.65454228025186,
116.977780541892));
#227460=CARTESIAN_POINT('Ctrl Pts',(5.0510207267576,-6.47444880834103,117.066367977625));
#227461=CARTESIAN_POINT('Ctrl Pts',(7.66951518847946,-2.93425195367516,
117.24354284909));
#227462=CARTESIAN_POINT('Ctrl Pts',(8.18956872247087,-0.60188196009709,
117.332130284823));
#227463=CARTESIAN_POINT('Ctrl Pts',(7.32306689761247,3.71537198232641,117.509305156289));
#227464=CARTESIAN_POINT('Ctrl Pts',(5.94329958850052,5.66643518936668,117.597892592021));
#227465=CARTESIAN_POINT('Ctrl Pts',(2.16154501637633,7.92205913233057,117.775067463487));
#227466=CARTESIAN_POINT('Ctrl Pts',(-0.210816529302626,8.20894963712997,
117.863654899219));
#227467=CARTESIAN_POINT('Ctrl Pts',(-4.42123908576632,6.91982244717707,
118.040829770685));
#227468=CARTESIAN_POINT('Ctrl Pts',(-6.22631625634341,5.35390358803343,
118.129417206418));
#227469=CARTESIAN_POINT('Ctrl Pts',(-7.6529679718098,2.31378507137994,118.264539857955));
#227470=CARTESIAN_POINT('Ctrl Pts',(-7.91078507045206,1.15799210747852,
118.311075073758));
#227471=CARTESIAN_POINT('Ctrl Pts',(-7.91099986567554,0.00144650702262969,
118.357610289563));
#227472=CARTESIAN_POINT('',(-7.90626572818492,0.00396378192042368,120.357668491763));
#227473=CARTESIAN_POINT('Ctrl Pts',(-7.91099986706751,0.00145026131998307,
118.357704282581));
#227474=CARTESIAN_POINT('Ctrl Pts',(-7.91103615013821,-0.196469495286411,
118.36570021141));
#227475=CARTESIAN_POINT('Ctrl Pts',(-7.90364072243202,-0.394584910582694,
118.37369614024));
#227476=CARTESIAN_POINT('Ctrl Pts',(-7.888795715768,-0.592303262594768,
118.381692069069));
#227477=CARTESIAN_POINT('Ctrl Pts',(-7.87396372149712,-0.789848304551604,
118.389680989066));
#227478=CARTESIAN_POINT('Ctrl Pts',(-7.85169518682542,-0.986996644197289,
118.397669909062));
#227479=CARTESIAN_POINT('Ctrl Pts',(-7.82202428542851,-1.18315555958067,
118.405658829059));
#227480=CARTESIAN_POINT('Ctrl Pts',(-7.79237432198154,-1.37917605094059,
118.413642111492));
#227481=CARTESIAN_POINT('Ctrl Pts',(-7.75533245337266,-1.57420817929061,
118.421625393924));
#227482=CARTESIAN_POINT('Ctrl Pts',(-7.71098470962028,-1.76766394091248,
118.429608676357));
#227483=CARTESIAN_POINT('Ctrl Pts',(-7.66666068619764,-1.96101622862415,
118.437587688762));
#227484=CARTESIAN_POINT('Ctrl Pts',(-7.61503865223227,-2.15279350427088,
118.445566701167));
#227485=CARTESIAN_POINT('Ctrl Pts',(-7.5562558740262,-2.34241716315532,
118.453545713572));
#227486=CARTESIAN_POINT('Ctrl Pts',(-7.49749132357651,-2.53198202226942,
118.461522251791));
#227487=CARTESIAN_POINT('Ctrl Pts',(-7.43157055276323,-2.71939427544401,
118.469498790011));
#227488=CARTESIAN_POINT('Ctrl Pts',(-7.35868104682497,-2.90408922919027,
118.477475328231));
#227489=CARTESIAN_POINT('Ctrl Pts',(-7.28580243285818,-3.08875658373496,
118.485450674506));
#227490=CARTESIAN_POINT('Ctrl Pts',(-7.20595728206472,-3.27070713624327,
118.493426020781));
#227491=CARTESIAN_POINT('Ctrl Pts',(-7.11938184059797,-3.44939461467716,
118.501401367056));
#227492=CARTESIAN_POINT('Ctrl Pts',(-7.03280593132814,-3.62808305863376,
118.509376756426));
#227493=CARTESIAN_POINT('Ctrl Pts',(-6.93949980539527,-3.80350809174866,
118.517352145795));
#227494=CARTESIAN_POINT('Ctrl Pts',(-6.83974659367512,-3.97514622804113,
118.525327535165));
#227495=CARTESIAN_POINT('Ctrl Pts',(-6.73997739799885,-4.14681186677078,
118.533304202471));
#227496=CARTESIAN_POINT('Ctrl Pts',(-6.63375922651977,-4.31468910969268,
118.541280869777));
#227497=CARTESIAN_POINT('Ctrl Pts',(-6.52141981929608,-4.47828142712049,
118.549257537083));
#227498=CARTESIAN_POINT('Ctrl Pts',(-6.40900368710289,-4.64198547395719,
118.55723965225));
#227499=CARTESIAN_POINT('Ctrl Pts',(-6.29045815669429,-4.80139847184263,
118.565221767418));
#227500=CARTESIAN_POINT('Ctrl Pts',(-6.1661533379606,-4.95605427863309,
118.573203882585));
#227501=CARTESIAN_POINT('Ctrl Pts',(-6.04180093508365,-5.1107692879882,
118.581189053323));
#227502=CARTESIAN_POINT('Ctrl Pts',(-5.91168506425132,-5.26072321916806,
118.589174224061));
#227503=CARTESIAN_POINT('Ctrl Pts',(-5.77621472687111,-5.40548466181131,
118.597159394799));
#227504=CARTESIAN_POINT('Ctrl Pts',(-5.64061596056753,-5.55038334155446,
118.605152135659));
#227505=CARTESIAN_POINT('Ctrl Pts',(-5.49965282233508,-5.69007946015305,
118.613144876518));
#227506=CARTESIAN_POINT('Ctrl Pts',(-5.35377039212665,-5.82417922014665,
118.621137617377));
#227507=CARTESIAN_POINT('Ctrl Pts',(-5.28623242659609,-5.88626226164222,
118.624837949596));
#227508=CARTESIAN_POINT('Ctrl Pts',(-5.21764055852171,-5.94714638170074,
118.628538281814));
#227509=CARTESIAN_POINT('Ctrl Pts',(-5.14804124519898,-6.00679551322751,
118.632238614033));
#227510=CARTESIAN_POINT('Ctrl Pts',(-5.00080503293966,-6.1329822781721,
118.640066606494));
#227511=CARTESIAN_POINT('Ctrl Pts',(-4.84874534686315,-6.2539074889938,
118.647894598955));
#227512=CARTESIAN_POINT('Ctrl Pts',(-4.69227874488835,-6.36917900362904,
118.655722591416));
#227513=CARTESIAN_POINT('Ctrl Pts',(-4.53594429727526,-6.48435315797622,
118.663543972221));
#227514=CARTESIAN_POINT('Ctrl Pts',(-4.37521062660918,-6.59388291674253,
118.671365353027));
#227515=CARTESIAN_POINT('Ctrl Pts',(-4.21052892568385,-6.69741496145935,
118.679186733832));
#227516=CARTESIAN_POINT('Ctrl Pts',(-4.04595723588101,-6.8008778444151,
118.687002889776));
#227517=CARTESIAN_POINT('Ctrl Pts',(-3.87744306508657,-6.89835080592899,
118.694819045721));
#227518=CARTESIAN_POINT('Ctrl Pts',(-3.70546840147755,-6.98952251056189,
118.702635201666));
#227519=CARTESIAN_POINT('Ctrl Pts',(-3.53357635514205,-7.08065041596588,
118.7104476027));
#227520=CARTESIAN_POINT('Ctrl Pts',(-3.35822743780163,-7.16548292961773,
118.718260003734));
#227521=CARTESIAN_POINT('Ctrl Pts',(-3.17993031807008,-7.24375345882359,
118.726072404768));
#227522=CARTESIAN_POINT('Ctrl Pts',(-3.0016853126272,-7.32200111041393,
118.733882522323));
#227523=CARTESIAN_POINT('Ctrl Pts',(-2.82049414387768,-7.39369045760067,
118.741692639879));
#227524=CARTESIAN_POINT('Ctrl Pts',(-2.63688779715974,-7.45860199670086,
118.749502757434));
#227525=CARTESIAN_POINT('Ctrl Pts',(-2.45327098909801,-7.52351723426757,
118.757313319986));
#227526=CARTESIAN_POINT('Ctrl Pts',(-2.26723905805088,-7.58165376865885,
118.765123882539));
#227527=CARTESIAN_POINT('Ctrl Pts',(-2.07934100134186,-7.6328410176119,
118.772934445091));
#227528=CARTESIAN_POINT('Ctrl Pts',(-1.93292631490113,-7.67272735351387,
118.779020623347));
#227529=CARTESIAN_POINT('Ctrl Pts',(-1.78537894391127,-7.70839511676152,
118.785106801602));
#227530=CARTESIAN_POINT('Ctrl Pts',(-1.63696420259712,-7.73978482901273,
118.791192979858));
#227531=CARTESIAN_POINT('Ctrl Pts',(-1.42626421463101,-7.78434786860722,
118.799833345861));
#227532=CARTESIAN_POINT('Ctrl Pts',(-1.21391627437396,-7.82026636386086,
118.808473711865));
#227533=CARTESIAN_POINT('Ctrl Pts',(-1.00061366223356,-7.84746413174036,
118.817114077868));
#227534=CARTESIAN_POINT('Ctrl Pts',(-0.786956223196841,-7.87470714285185,
118.825768817039));
#227535=CARTESIAN_POINT('Ctrl Pts',(-0.572341165909358,-7.89320040003454,
118.83442355621));
#227536=CARTESIAN_POINT('Ctrl Pts',(-0.357465618056908,-7.9029196713561,
118.843078295381));
#227537=CARTESIAN_POINT('Ctrl Pts',(-0.135944202772329,-7.91293954918866,
118.85200071624));
#227538=CARTESIAN_POINT('Ctrl Pts',(0.0858537942406949,-7.91363406139319,
118.860923137098));
#227539=CARTESIAN_POINT('Ctrl Pts',(0.30716799939464,-7.90503439715147,
118.869845557957));
#227540=CARTESIAN_POINT('Ctrl Pts',(0.522562911823992,-7.89666474042302,
118.87852933882));
#227541=CARTESIAN_POINT('Ctrl Pts',(0.73749935952798,-7.87949171753001,
118.887213119683));
#227542=CARTESIAN_POINT('Ctrl Pts',(0.951283084827622,-7.85359672331861,
118.895896900546));
#227543=CARTESIAN_POINT('Ctrl Pts',(1.17387933338185,-7.8266342940705,118.904938641402));
#227544=CARTESIAN_POINT('Ctrl Pts',(1.39522553407994,-7.79021568625419,
118.913980382258));
#227545=CARTESIAN_POINT('Ctrl Pts',(1.61454958687192,-7.74449163157478,
118.923022123114));
#227546=CARTESIAN_POINT('Ctrl Pts',(1.8338736396639,-7.69876757689536,118.93206386397));
#227547=CARTESIAN_POINT('Ctrl Pts',(2.05117527929417,-7.64373816321146,
118.941105604826));
#227548=CARTESIAN_POINT('Ctrl Pts',(2.26569821988195,-7.57961295690115,
118.950147345682));
#227549=CARTESIAN_POINT('Ctrl Pts',(2.46314455284439,-7.52059229085145,
118.958469339455));
#227550=CARTESIAN_POINT('Ctrl Pts',(2.65840469216121,-7.45381611622113,
118.966791333227));
#227551=CARTESIAN_POINT('Ctrl Pts',(2.85086500626089,-7.37946405344433,
118.975113327));
#227552=CARTESIAN_POINT('Ctrl Pts',(3.04315414282958,-7.30517812067772,
118.983427919047));
#227553=CARTESIAN_POINT('Ctrl Pts',(3.23264815010936,-7.22332984657303,
118.991742511094));
#227554=CARTESIAN_POINT('Ctrl Pts',(3.41874968624922,-7.13414827311368,
119.000057103142));
#227555=CARTESIAN_POINT('Ctrl Pts',(3.60469704984099,-7.04504058056206,
119.008364807111));
#227556=CARTESIAN_POINT('Ctrl Pts',(3.78725728609806,-6.94861183441135,
119.016672511081));
#227557=CARTESIAN_POINT('Ctrl Pts',(3.96585334813195,-6.84513902131364,
119.024980215051));
#227558=CARTESIAN_POINT('Ctrl Pts',(4.14426921478889,-6.74177060762063,
119.033279536921));
#227559=CARTESIAN_POINT('Ctrl Pts',(4.31872863852634,-6.63137245959264,
119.041578858792));
#227560=CARTESIAN_POINT('Ctrl Pts',(4.48867913574803,-6.51426746582456,
119.049878180663));
#227561=CARTESIAN_POINT('Ctrl Pts',(4.65852105146005,-6.39723729053139,
119.05817220009));
#227562=CARTESIAN_POINT('Ctrl Pts',(4.82385954666406,-6.27350898213789,
119.066466219518));
#227563=CARTESIAN_POINT('Ctrl Pts',(4.98416987967236,-6.1434494879153,119.074760238945));
#227564=CARTESIAN_POINT('Ctrl Pts',(5.14436133459422,-6.0134864392774,119.083048107945));
#227565=CARTESIAN_POINT('Ctrl Pts',(5.29953184239586,-5.87720175880035,
119.091335976944));
#227566=CARTESIAN_POINT('Ctrl Pts',(5.44918817656425,-5.73500385495881,
119.099623845943));
#227567=CARTESIAN_POINT('Ctrl Pts',(5.50623631990744,-5.68079882283283,
119.102783134465));
#227568=CARTESIAN_POINT('Ctrl Pts',(5.5624835365847,-5.62573496996465,119.105942422986));
#227569=CARTESIAN_POINT('Ctrl Pts',(5.61790377792052,-5.56983645559062,
119.109101711507));
#227570=CARTESIAN_POINT('Ctrl Pts',(5.76003450226718,-5.42647915243961,
119.117204021334));
#227571=CARTESIAN_POINT('Ctrl Pts',(5.89666373218884,-5.27768970130891,
119.12530633116));
#227572=CARTESIAN_POINT('Ctrl Pts',(6.02738087567515,-5.12392435341755,
119.133408640987));
#227573=CARTESIAN_POINT('Ctrl Pts',(6.15812687151884,-4.97012506588636,
119.141512739184));
#227574=CARTESIAN_POINT('Ctrl Pts',(6.28295797178841,-4.81134793413588,
119.149616837381));
#227575=CARTESIAN_POINT('Ctrl Pts',(6.40150390790828,-4.64808226229216,
119.157720935579));
#227576=CARTESIAN_POINT('Ctrl Pts',(6.5200908800299,-4.48476007420997,119.1658278391));
#227577=CARTESIAN_POINT('Ctrl Pts',(6.63238816147137,-4.31694650514095,
119.173934742622));
#227578=CARTESIAN_POINT('Ctrl Pts',(6.73806852270149,-4.14516026027696,
119.182041646144));
#227579=CARTESIAN_POINT('Ctrl Pts',(6.84384419164315,-3.97321909018674,
119.190155860867));
#227580=CARTESIAN_POINT('Ctrl Pts',(6.94299084829057,-3.79729835673636,
119.19827007559));
#227581=CARTESIAN_POINT('Ctrl Pts',(7.03522632795049,-3.61794299492299,
119.206384290313));
#227582=CARTESIAN_POINT('Ctrl Pts',(7.12750688606164,-3.43849997636449,
119.214502470715));
#227583=CARTESIAN_POINT('Ctrl Pts',(7.21286939000608,-3.25561926761517,
119.222620651116));
#227584=CARTESIAN_POINT('Ctrl Pts',(7.2910792737547,-3.0698671019809,119.230738831517));
#227585=CARTESIAN_POINT('Ctrl Pts',(7.36937326486342,-2.88391517739631,
119.238865742257));
#227586=CARTESIAN_POINT('Ctrl Pts',(7.44049914825659,-2.6950859220191,119.246992652996));
#227587=CARTESIAN_POINT('Ctrl Pts',(7.50427133008208,-2.50396341916333,
119.255119563735));
#227588=CARTESIAN_POINT('Ctrl Pts',(7.53810910369348,-2.40255305811633,
119.259431734934));
#227589=CARTESIAN_POINT('Ctrl Pts',(7.56987735906151,-2.30049729704032,
119.263743906133));
#227590=CARTESIAN_POINT('Ctrl Pts',(7.59955416871206,-2.19788476422472,
119.268056077332));
#227591=CARTESIAN_POINT('Ctrl Pts',(7.65459577772019,-2.00756919536555,
119.276053865636));
#227592=CARTESIAN_POINT('Ctrl Pts',(7.7025354397237,-1.81500738908132,119.284051653939));
#227593=CARTESIAN_POINT('Ctrl Pts',(7.74319318408437,-1.62076534820726,
119.292049442243));
#227594=CARTESIAN_POINT('Ctrl Pts',(7.78381773144638,-1.4266819057225,119.300040700362));
#227595=CARTESIAN_POINT('Ctrl Pts',(7.81717214194644,-1.23092128852819,
119.308031958481));
#227596=CARTESIAN_POINT('Ctrl Pts',(7.84312649034786,-1.03406375838421,
119.3160232166));
#227597=CARTESIAN_POINT('Ctrl Pts',(7.86906404820023,-0.83733358054227,
119.324009304964));
#227598=CARTESIAN_POINT('Ctrl Pts',(7.88761104186485,-0.639508234683549,
119.331995393329));
#227599=CARTESIAN_POINT('Ctrl Pts',(7.89868870566191,-0.441177663814656,
119.339981481693));
#227600=CARTESIAN_POINT('Ctrl Pts',(7.90976108068653,-0.242941781255309,
119.347963757286));
#227601=CARTESIAN_POINT('Ctrl Pts',(7.9133712155375,-0.0442014878576724,
119.355946032879));
#227602=CARTESIAN_POINT('Ctrl Pts',(7.9094921921131,0.154448253152782,119.363928308471));
#227603=CARTESIAN_POINT('Ctrl Pts',(7.90561436336275,0.353036813379822,
119.371908125657));
#227604=CARTESIAN_POINT('Ctrl Pts',(7.8942519812414,0.551534542692189,119.379887942843));
#227605=CARTESIAN_POINT('Ctrl Pts',(7.87543023136269,0.749346162289925,
119.387867760029));
#227606=CARTESIAN_POINT('Ctrl Pts',(7.85596167180673,0.953955580745488,
119.396121803735));
#227607=CARTESIAN_POINT('Ctrl Pts',(7.82851195718458,1.15783052104527,119.404375847442));
#227608=CARTESIAN_POINT('Ctrl Pts',(7.79316744696654,1.36031692760952,119.412629891148));
#227609=CARTESIAN_POINT('Ctrl Pts',(7.75899257665929,1.55610254298873,119.420610787514));
#227610=CARTESIAN_POINT('Ctrl Pts',(7.71743714391871,1.75058971130236,119.428591683881));
#227611=CARTESIAN_POINT('Ctrl Pts',(7.66863143007339,1.94319659059258,119.436572580247));
#227612=CARTESIAN_POINT('Ctrl Pts',(7.61981488073649,2.135846231069,119.444555248475));
#227613=CARTESIAN_POINT('Ctrl Pts',(7.56374492319702,2.32661442569172,119.452537916702));
#227614=CARTESIAN_POINT('Ctrl Pts',(7.50060213050016,2.5149331362755,119.46052058493));
#227615=CARTESIAN_POINT('Ctrl Pts',(7.43743561318835,2.70332260376921,119.468506252482));
#227616=CARTESIAN_POINT('Ctrl Pts',(7.36719106909571,2.8892604351785,119.476491920034));
#227617=CARTESIAN_POINT('Ctrl Pts',(7.29009788540409,3.07219690469652,119.484477587586));
#227618=CARTESIAN_POINT('Ctrl Pts',(7.21296388295768,3.25523023412526,119.492467483332));
#227619=CARTESIAN_POINT('Ctrl Pts',(7.12897414148497,3.43525872550265,119.500457379079));
#227620=CARTESIAN_POINT('Ctrl Pts',(7.03840497108245,3.61175531605365,119.508447274826));
#227621=CARTESIAN_POINT('Ctrl Pts',(6.94772851402123,3.78846098138571,119.516446635264));
#227622=CARTESIAN_POINT('Ctrl Pts',(6.85045721147659,3.96162609040045,119.524445995702));
#227623=CARTESIAN_POINT('Ctrl Pts',(6.74691250154266,4.13074965309293,119.53244535614));
#227624=CARTESIAN_POINT('Ctrl Pts',(6.64329540802179,4.29999144268578,119.540450308582));
#227625=CARTESIAN_POINT('Ctrl Pts',(6.53339634539518,4.46518577342108,119.548455261023));
#227626=CARTESIAN_POINT('Ctrl Pts',(6.41757865081015,4.62586265043244,119.556460213465));
#227627=CARTESIAN_POINT('Ctrl Pts',(6.30160980468221,4.78674922388056,119.564475613023));
#227628=CARTESIAN_POINT('Ctrl Pts',(6.17970710251706,4.94310630428356,119.572491012581));
#227629=CARTESIAN_POINT('Ctrl Pts',(6.05227327133962,5.09449793885796,119.580506412138));
#227630=CARTESIAN_POINT('Ctrl Pts',(6.02334626997655,5.12886327166815,119.582325877753));
#227631=CARTESIAN_POINT('Ctrl Pts',(5.99413441054198,5.16297290269607,119.584145343367));
#227632=CARTESIAN_POINT('Ctrl Pts',(5.96464265541942,5.19682200899272,119.585964808982));
#227633=CARTESIAN_POINT('Ctrl Pts',(5.83884770394008,5.3412029272023,119.593725608152));
#227634=CARTESIAN_POINT('Ctrl Pts',(5.70758380519134,5.48126989469719,119.601486407322));
#227635=CARTESIAN_POINT('Ctrl Pts',(5.5711817486657,5.61656967581941,119.609247206492));
#227636=CARTESIAN_POINT('Ctrl Pts',(5.434945282889,5.75170520434416,119.616998584128));
#227637=CARTESIAN_POINT('Ctrl Pts',(5.29358332630605,5.88208481622866,119.624749961765));
#227638=CARTESIAN_POINT('Ctrl Pts',(5.14746799382607,6.00728676296847,119.632501339401));
#227639=CARTESIAN_POINT('Ctrl Pts',(5.00150038414922,6.13236213036705,119.640244880384));
#227640=CARTESIAN_POINT('Ctrl Pts',(4.85078923511304,6.25227002160903,119.647988421367));
#227641=CARTESIAN_POINT('Ctrl Pts',(4.69574478683363,6.36662405808014,119.65573196235));
#227642=CARTESIAN_POINT('Ctrl Pts',(4.54082566327652,6.48088566049105,119.663469244115));
#227643=CARTESIAN_POINT('Ctrl Pts',(4.38158050125974,6.58960213416366,119.671206525879));
#227644=CARTESIAN_POINT('Ctrl Pts',(4.21845409622307,6.69242602036502,119.678943807643));
#227645=CARTESIAN_POINT('Ctrl Pts',(4.05542652010801,6.79518761147819,119.686676401833));
#227646=CARTESIAN_POINT('Ctrl Pts',(3.88852268591381,6.89206353305957,119.694408996022));
#227647=CARTESIAN_POINT('Ctrl Pts',(3.71821803993601,6.98274842791106,119.702141590212));
#227648=CARTESIAN_POINT('Ctrl Pts',(3.54798211470679,7.07339672990378,119.709871064171));
#227649=CARTESIAN_POINT('Ctrl Pts',(3.37434842720722,7.15785881222829,119.717600538131));
#227650=CARTESIAN_POINT('Ctrl Pts',(3.19781887402807,7.23587420073828,119.72533001209));
#227651=CARTESIAN_POINT('Ctrl Pts',(3.02129216768496,7.31388833111888,119.733059361399));
#227652=CARTESIAN_POINT('Ctrl Pts',(2.84187001253841,7.38545581951772,119.740788710708));
#227653=CARTESIAN_POINT('Ctrl Pts',(2.66007659322118,7.45036331451003,119.748518060017));
#227654=CARTESIAN_POINT('Ctrl Pts',(2.4782758242127,7.51527343363498,119.756247721814));
#227655=CARTESIAN_POINT('Ctrl Pts',(2.29410393821104,7.57352290139463,119.763977383611));
#227656=CARTESIAN_POINT('Ctrl Pts',(2.10810252566066,7.62494752383931,119.771707045408));
#227657=CARTESIAN_POINT('Ctrl Pts',(1.92205951152549,7.67638364805572,119.779438436043));
#227658=CARTESIAN_POINT('Ctrl Pts',(1.73418650220548,7.72099179136673,119.787169826677));
#227659=CARTESIAN_POINT('Ctrl Pts',(1.54503763079652,7.75865837109888,119.794901217311));
#227660=CARTESIAN_POINT('Ctrl Pts',(1.35581178450632,7.79634027939461,119.802635754266));
#227661=CARTESIAN_POINT('Ctrl Pts',(1.1653093941541,7.82707492893557,119.81037029122));
#227662=CARTESIAN_POINT('Ctrl Pts',(0.974092152111527,7.85080030819755,
119.818104828175));
#227663=CARTESIAN_POINT('Ctrl Pts',(0.78264972245639,7.87455362773027,119.825848473732));
#227664=CARTESIAN_POINT('Ctrl Pts',(0.590491116317506,7.89128114754464,
119.833592119289));
#227665=CARTESIAN_POINT('Ctrl Pts',(0.398181526491632,7.9009728813584,119.841335764847));
#227666=CARTESIAN_POINT('Ctrl Pts',(0.205748721035988,7.91067082481093,
119.849084371873));
#227667=CARTESIAN_POINT('Ctrl Pts',(0.0131650968569829,7.91332399779083,
119.8568329789));
#227668=CARTESIAN_POINT('Ctrl Pts',(-0.179006949978784,7.9089744917947,
119.864581585927));
#227669=CARTESIAN_POINT('Ctrl Pts',(-0.371470174448657,7.90461839545994,
119.872341933585));
#227670=CARTESIAN_POINT('Ctrl Pts',(-0.5635202191567,7.8932384500904,119.880102281242));
#227671=CARTESIAN_POINT('Ctrl Pts',(-0.754601381223256,7.8749284285926,
119.8878626289));
#227672=CARTESIAN_POINT('Ctrl Pts',(-0.886012315991531,7.8623362033066,
119.893199599477));
#227673=CARTESIAN_POINT('Ctrl Pts',(-1.01696519846024,7.84646738331229,
119.898536570054));
#227674=CARTESIAN_POINT('Ctrl Pts',(-1.14728311387771,7.82736625287274,
119.903873540631));
#227675=CARTESIAN_POINT('Ctrl Pts',(-1.34052922190157,7.79904152787639,
119.91178763893));
#227676=CARTESIAN_POINT('Ctrl Pts',(-1.53299881074559,7.76351608916653,
119.919701737229));
#227677=CARTESIAN_POINT('Ctrl Pts',(-1.72411413628818,7.72083877859467,
119.927615835527));
#227678=CARTESIAN_POINT('Ctrl Pts',(-1.91501000734958,7.67821047365344,
119.935520846201));
#227679=CARTESIAN_POINT('Ctrl Pts',(-2.10455437925534,7.62844672859773,
119.943425856875));
#227680=CARTESIAN_POINT('Ctrl Pts',(-2.29217510595005,7.57164805598246,
119.95133086755));
#227681=CARTESIAN_POINT('Ctrl Pts',(-2.47961523885351,7.51490405476626,
119.959228269278));
#227682=CARTESIAN_POINT('Ctrl Pts',(-2.66513508722515,7.45113871413749,
119.967125671007));
#227683=CARTESIAN_POINT('Ctrl Pts',(-2.84817289568144,7.38050351644829,
119.975023072736));
#227684=CARTESIAN_POINT('Ctrl Pts',(-3.03106850639844,7.30992319357163,
119.98291433916));
#227685=CARTESIAN_POINT('Ctrl Pts',(-3.21148559854803,7.2324837700926,119.990805605584));
#227686=CARTESIAN_POINT('Ctrl Pts',(-3.38887751257084,7.14838654556339,
119.998696872009));
#227687=CARTESIAN_POINT('Ctrl Pts',(-3.56616454321308,7.06433904371322,
120.006583472703));
#227688=CARTESIAN_POINT('Ctrl Pts',(-3.74042964897547,6.97364173176869,
120.014470073398));
#227689=CARTESIAN_POINT('Ctrl Pts',(-3.91114584112585,6.8765441327344,120.022356674093));
#227690=CARTESIAN_POINT('Ctrl Pts',(-4.0817927801578,6.77948592253278,120.030240075491));
#227691=CARTESIAN_POINT('Ctrl Pts',(-4.24889337540426,6.67603276987812,
120.03812347689));
#227692=CARTESIAN_POINT('Ctrl Pts',(-4.41194471236759,6.56648040087014,
120.046006878288));
#227693=CARTESIAN_POINT('Ctrl Pts',(-4.57498299938688,6.45693679997354,
120.053889648732));
#227694=CARTESIAN_POINT('Ctrl Pts',(-4.73397238391049,6.34129514199491,
120.061772419176));
#227695=CARTESIAN_POINT('Ctrl Pts',(-4.88843802027627,6.2198950732241,120.06965518962));
#227696=CARTESIAN_POINT('Ctrl Pts',(-5.04290404734862,6.09849469738302,
120.077537980003));
#227697=CARTESIAN_POINT('Ctrl Pts',(-5.19284603183183,5.97133609448737,
120.085420770386));
#227698=CARTESIAN_POINT('Ctrl Pts',(-5.33782130693576,5.8387999362217,120.093303560769));
#227699=CARTESIAN_POINT('Ctrl Pts',(-5.48282132859799,5.70624115469311,
120.101187696705));
#227700=CARTESIAN_POINT('Ctrl Pts',(-5.62285269699034,5.56830322160043,
120.10907183264));
#227701=CARTESIAN_POINT('Ctrl Pts',(-5.75750861486855,5.42540464386892,
120.116955968576));
#227702=CARTESIAN_POINT('Ctrl Pts',(-5.89221016245567,5.28245764330826,
120.124842776143));
#227703=CARTESIAN_POINT('Ctrl Pts',(-6.02153239375114,5.13454689976469,
120.132729583709));
#227704=CARTESIAN_POINT('Ctrl Pts',(-6.1451077480048,4.98212522578582,120.140616391275));
#227705=CARTESIAN_POINT('Ctrl Pts',(-6.26880385358569,4.82955461337547,
120.148510905414));
#227706=CARTESIAN_POINT('Ctrl Pts',(-6.38674164824982,4.67246453436258,
120.156405419553));
#227707=CARTESIAN_POINT('Ctrl Pts',(-6.49859537110552,4.51133895896174,
120.164299933692));
#227708=CARTESIAN_POINT('Ctrl Pts',(-6.61051164662823,4.3501232762832,120.172198862731));
#227709=CARTESIAN_POINT('Ctrl Pts',(-6.71633688107715,4.18486788757923,
120.180097791769));
#227710=CARTESIAN_POINT('Ctrl Pts',(-6.81579037075905,4.01608299489293,
120.187996720808));
#227711=CARTESIAN_POINT('Ctrl Pts',(-6.91536530335083,3.84709199854374,
120.195905295248));
#227712=CARTESIAN_POINT('Ctrl Pts',(-7.00855278642122,3.67456319215405,
120.203813869689));
#227713=CARTESIAN_POINT('Ctrl Pts',(-7.09511902650703,3.49902943681501,
120.21172244413));
#227714=CARTESIAN_POINT('Ctrl Pts',(-7.1318235554734,3.4246022259181,120.21507572018));
#227715=CARTESIAN_POINT('Ctrl Pts',(-7.16733831531233,3.34963501146115,
120.21842899623));
#227716=CARTESIAN_POINT('Ctrl Pts',(-7.20164816280539,3.27416932047837,
120.221782272281));
#227717=CARTESIAN_POINT('Ctrl Pts',(-7.29218645218861,3.07502723539373,
120.230631040189));
#227718=CARTESIAN_POINT('Ctrl Pts',(-7.37450316996348,2.87203455178348,
120.239479808097));
#227719=CARTESIAN_POINT('Ctrl Pts',(-7.44829984725901,2.6658489051935,120.248328576005));
#227720=CARTESIAN_POINT('Ctrl Pts',(-7.52428895885341,2.45353766460545,
120.257440233015));
#227721=CARTESIAN_POINT('Ctrl Pts',(-7.59124388804176,2.237840989881,120.266551890026));
#227722=CARTESIAN_POINT('Ctrl Pts',(-7.64889092479903,2.01950207242455,
120.275663547036));
#227723=CARTESIAN_POINT('Ctrl Pts',(-7.70459438214935,1.80852448778893,
120.284468003019));
#227724=CARTESIAN_POINT('Ctrl Pts',(-7.75160717027716,1.59508012271073,
120.293272459002));
#227725=CARTESIAN_POINT('Ctrl Pts',(-7.78973097277438,1.37985954785242,
120.302076914985));
#227726=CARTESIAN_POINT('Ctrl Pts',(-7.82776957822532,1.16511993648874,
120.310861695238));
#227727=CARTESIAN_POINT('Ctrl Pts',(-7.85695879704077,0.948612230775094,
120.319646475491));
#227728=CARTESIAN_POINT('Ctrl Pts',(-7.87715066373012,0.731039274523672,
120.328431255744));
#227729=CARTESIAN_POINT('Ctrl Pts',(-7.89727337150146,0.514211524769316,
120.337185947352));
#227730=CARTESIAN_POINT('Ctrl Pts',(-7.90846018411719,0.296326002315819,
120.345940638961));
#227731=CARTESIAN_POINT('Ctrl Pts',(-7.91061455199777,0.0780923153782337,
120.354695330569));
#227732=CARTESIAN_POINT('Ctrl Pts',(-7.91085842941872,0.053387960465725,
120.355686373756));
#227733=CARTESIAN_POINT('Ctrl Pts',(-7.91098661353903,0.0286791569209888,
120.356677416943));
#227734=CARTESIAN_POINT('Ctrl Pts',(-7.91099900539481,0.00396694370733382,
120.357668460131));
#227735=CARTESIAN_POINT('',(-7.90255836853663,-0.00601847252836551,122.357668497961));
#227736=CARTESIAN_POINT('Ctrl Pts',(-7.90626572818492,0.00396378192042368,
120.357668491763));
#227737=CARTESIAN_POINT('Ctrl Pts',(-7.90584785985939,-0.187660776584018,
120.365357873877));
#227738=CARTESIAN_POINT('Ctrl Pts',(-7.84915752905825,-1.70037946986372,
120.426032044598));
#227739=CARTESIAN_POINT('Ctrl Pts',(-6.53602975274865,-5.78311739899863,
120.592675792542));
#227740=CARTESIAN_POINT('Ctrl Pts',(-1.33164505529345,-8.62281587858876,
120.80461494697));
#227741=CARTESIAN_POINT('Ctrl Pts',(3.95079584577209,-7.22610140145887,
121.016554101405));
#227742=CARTESIAN_POINT('Ctrl Pts',(6.93730582468089,-4.47104709983874,
121.175508467229));
#227743=CARTESIAN_POINT('Ctrl Pts',(8.21337391138441,-0.604780945227029,
121.334462833054));
#227744=CARTESIAN_POINT('Ctrl Pts',(7.30159313550923,4.7675339096173,121.546401987488));
#227745=CARTESIAN_POINT('Ctrl Pts',(1.37451247778806,9.25621343198184,121.811325930528));
#227746=CARTESIAN_POINT('Ctrl Pts',(-6.27159982437673,6.44040648793863,
122.099409694823));
#227747=CARTESIAN_POINT('Ctrl Pts',(-7.88681031979375,1.88844581118687,
122.281523881901));
#227748=CARTESIAN_POINT('Ctrl Pts',(-7.90138446041817,-0.00601742412920814,
122.357668491763));
#227749=CARTESIAN_POINT('',(-7.92239988164926,-0.00247633632947917,124.357668806763));
#227750=CARTESIAN_POINT('Ctrl Pts',(-7.91099770491742,-0.00602600956896626,
122.357668542519));
#227751=CARTESIAN_POINT('Ctrl Pts',(-7.91082343745109,-0.234805853083792,
122.366852830167));
#227752=CARTESIAN_POINT('Ctrl Pts',(-7.90072110925209,-0.463199658241609,
122.376037117815));
#227753=CARTESIAN_POINT('Ctrl Pts',(-7.88081444583491,-0.690423544152256,
122.385221405463));
#227754=CARTESIAN_POINT('Ctrl Pts',(-7.86080562440018,-0.918813509040518,
122.394452825501));
#227755=CARTESIAN_POINT('Ctrl Pts',(-7.83089166989144,-1.14602143151767,
122.403684245539));
#227756=CARTESIAN_POINT('Ctrl Pts',(-7.79124766526346,-1.37126978327632,
122.412915665577));
#227757=CARTESIAN_POINT('Ctrl Pts',(-7.75137148169927,-1.59783732372909,
122.422201150317));
#227758=CARTESIAN_POINT('Ctrl Pts',(-7.7016510085194,-1.82242219111774,
122.431486635057));
#227759=CARTESIAN_POINT('Ctrl Pts',(-7.64231316787249,-2.04425302840983,
122.440772119796));
#227760=CARTESIAN_POINT('Ctrl Pts',(-7.62874153236439,-2.09498974608209,
122.442895877807));
#227761=CARTESIAN_POINT('Ctrl Pts',(-7.6146669917704,-2.14558247979062,
122.445019635817));
#227762=CARTESIAN_POINT('Ctrl Pts',(-7.60009261164581,-2.19602215253099,
122.447143393828));
#227763=CARTESIAN_POINT('Ctrl Pts',(-7.54111778509625,-2.4001248948534,
122.455737121948));
#227764=CARTESIAN_POINT('Ctrl Pts',(-7.47388082252246,-2.60197576896231,
122.464330850067));
#227765=CARTESIAN_POINT('Ctrl Pts',(-7.39856509941839,-2.80092046828683,
122.472924578187));
#227766=CARTESIAN_POINT('Ctrl Pts',(-7.32335811921021,-2.99957792582657,
122.481505898448));
#227767=CARTESIAN_POINT('Ctrl Pts',(-7.24009574407455,-3.19533735066757,
122.490087218708));
#227768=CARTESIAN_POINT('Ctrl Pts',(-7.14901080652297,-3.38756040362646,
122.498668538969));
#227769=CARTESIAN_POINT('Ctrl Pts',(-7.05398673524564,-3.58809649199087,
122.507620974026));
#227770=CARTESIAN_POINT('Ctrl Pts',(-6.95044854065877,-3.78478330039433,
122.516573409083));
#227771=CARTESIAN_POINT('Ctrl Pts',(-6.83871795396429,-3.97691560711646,
122.52552584414));
#227772=CARTESIAN_POINT('Ctrl Pts',(-6.73204100849876,-4.16035765474848,
122.534073355207));
#227773=CARTESIAN_POINT('Ctrl Pts',(-6.61789646909609,-4.33964779601734,
122.542620866275));
#227774=CARTESIAN_POINT('Ctrl Pts',(-6.49661316061465,-4.51419300000881,
122.551168377342));
#227775=CARTESIAN_POINT('Ctrl Pts',(-6.37551631531136,-4.68846985500919,
122.55970274731));
#227776=CARTESIAN_POINT('Ctrl Pts',(-6.24730273672162,-4.85801612224831,
122.568237117277));
#227777=CARTESIAN_POINT('Ctrl Pts',(-6.11234591069035,-5.02226527257043,
122.576771487245));
#227778=CARTESIAN_POINT('Ctrl Pts',(-5.97768291654091,-5.18615681492009,
122.585287275937));
#227779=CARTESIAN_POINT('Ctrl Pts',(-5.8363061281154,-5.34477406179062,
122.593803064629));
#227780=CARTESIAN_POINT('Ctrl Pts',(-5.68863092265281,-5.49758121593836,
122.602318853321));
#227781=CARTESIAN_POINT('Ctrl Pts',(-5.66678715342625,-5.52018409094987,
122.603578488765));
#227782=CARTESIAN_POINT('Ctrl Pts',(-5.64480565440291,-5.5426598950434,
122.604838124208));
#227783=CARTESIAN_POINT('Ctrl Pts',(-5.62268784985215,-5.5650069490635,
122.606097759652));
#227784=CARTESIAN_POINT('Ctrl Pts',(-5.48406843215521,-5.70506314715491,
122.613992301415));
#227785=CARTESIAN_POINT('Ctrl Pts',(-5.34022003012878,-5.83992976780298,
122.621886843178));
#227786=CARTESIAN_POINT('Ctrl Pts',(-5.19157519835085,-5.96920999461975,
122.629781384941));
#227787=CARTESIAN_POINT('Ctrl Pts',(-5.04289686831056,-6.0985193557354,
122.6376777058));
#227788=CARTESIAN_POINT('Ctrl Pts',(-4.88942021267008,-6.22223958920075,
122.645574026658));
#227789=CARTESIAN_POINT('Ctrl Pts',(-4.73161110841174,-6.34001398411349,
122.653470347517));
#227790=CARTESIAN_POINT('Ctrl Pts',(-4.57374042376016,-6.45783433704359,
122.661369749685));
#227791=CARTESIAN_POINT('Ctrl Pts',(-4.41153419555483,-6.56970402286812,
122.669269151852));
#227792=CARTESIAN_POINT('Ctrl Pts',(-4.24548774599272,-6.67530934104373,
122.67716855402));
#227793=CARTESIAN_POINT('Ctrl Pts',(-4.0792585813268,-6.78103086577915,
122.685076648575));
#227794=CARTESIAN_POINT('Ctrl Pts',(-3.90918104219986,-6.88047406748113,
122.69298474313));
#227795=CARTESIAN_POINT('Ctrl Pts',(-3.73577661790565,-6.9733703516384,
122.700892837685));
#227796=CARTESIAN_POINT('Ctrl Pts',(-3.56226888202774,-7.0663219819166,
122.708805643756));
#227797=CARTESIAN_POINT('Ctrl Pts',(-3.38543061583238,-7.1527187671374,
122.716718449827));
#227798=CARTESIAN_POINT('Ctrl Pts',(-3.20580410161825,-7.23233994375594,
122.724631255898));
#227799=CARTESIAN_POINT('Ctrl Pts',(-3.02592587066444,-7.3120726962355,
122.732555150454));
#227800=CARTESIAN_POINT('Ctrl Pts',(-2.84325190185535,-7.38501074096721,
122.740479045009));
#227801=CARTESIAN_POINT('Ctrl Pts',(-2.6583417859301,-7.4509824821414,122.748402939565));
#227802=CARTESIAN_POINT('Ctrl Pts',(-2.52883464035107,-7.49718769836549,
122.753952668202));
#227803=CARTESIAN_POINT('Ctrl Pts',(-2.39823091583697,-7.53997677735986,
122.75950239684));
#227804=CARTESIAN_POINT('Ctrl Pts',(-2.26672591224101,-7.57930568315958,
122.765052125477));
#227805=CARTESIAN_POINT('Ctrl Pts',(-2.07420992414844,-7.63688100693887,
122.773176618562));
#227806=CARTESIAN_POINT('Ctrl Pts',(-1.87933832265149,-7.68716533577582,
122.781301111647));
#227807=CARTESIAN_POINT('Ctrl Pts',(-1.68269142842093,-7.72997222224755,
122.789425604731));
#227808=CARTESIAN_POINT('Ctrl Pts',(-1.48621827120316,-7.7727412889479,
122.797542919848));
#227809=CARTESIAN_POINT('Ctrl Pts',(-1.28797326023693,-7.80804601663937,
122.805660234964));
#227810=CARTESIAN_POINT('Ctrl Pts',(-1.08855107457847,-7.83574996780998,
122.813777550081));
#227811=CARTESIAN_POINT('Ctrl Pts',(-0.889276683270306,-7.86343338722555,
122.82188884935));
#227812=CARTESIAN_POINT('Ctrl Pts',(-0.688827173348975,-7.88352721799388,
122.83000014862));
#227813=CARTESIAN_POINT('Ctrl Pts',(-0.48780716835004,-7.89594612231532,
122.83811144789));
#227814=CARTESIAN_POINT('Ctrl Pts',(-0.286907557755394,-7.90835758873729,
122.84621788916));
#227815=CARTESIAN_POINT('Ctrl Pts',(-0.0854384527376454,-7.91310327528335,
122.85432433043));
#227816=CARTESIAN_POINT('Ctrl Pts',(0.115990071895807,-7.91014963848483,
122.862430771701));
#227817=CARTESIAN_POINT('Ctrl Pts',(0.317326568464416,-7.90719735113509,
122.870533509324));
#227818=CARTESIAN_POINT('Ctrl Pts',(0.518622201490153,-7.89655276058245,
122.878636246948));
#227819=CARTESIAN_POINT('Ctrl Pts',(0.71926598195335,-7.87823441179587,
122.886738984571));
#227820=CARTESIAN_POINT('Ctrl Pts',(0.921721724629747,-7.85975063472773,
122.894914895928));
#227821=CARTESIAN_POINT('Ctrl Pts',(1.12351345260795,-7.83345380885929,
122.903090807284));
#227822=CARTESIAN_POINT('Ctrl Pts',(1.32401664272496,-7.79941670445857,
122.911266718641));
#227823=CARTESIAN_POINT('Ctrl Pts',(1.52264959289113,-7.76569708903358,
122.91936636729));
#227824=CARTESIAN_POINT('Ctrl Pts',(1.72001762199083,-7.72438104810107,
122.92746601594));
#227825=CARTESIAN_POINT('Ctrl Pts',(1.91552142449002,-7.67559109595604,
122.935565664589));
#227826=CARTESIAN_POINT('Ctrl Pts',(2.11102389835759,-7.62680147538449,
122.943665258194));
#227827=CARTESIAN_POINT('Ctrl Pts',(2.30466185975625,-7.57053812266403,
122.951764851798));
#227828=CARTESIAN_POINT('Ctrl Pts',(2.4958486122885,-7.50697413772937,122.959864445403));
#227829=CARTESIAN_POINT('Ctrl Pts',(2.68705874926596,-7.44340237815287,
122.967965029686));
#227830=CARTESIAN_POINT('Ctrl Pts',(2.87581677530425,-7.37252830720564,
122.976065613968));
#227831=CARTESIAN_POINT('Ctrl Pts',(3.06155298483146,-7.2945743070497,122.984166198251));
#227832=CARTESIAN_POINT('Ctrl Pts',(3.25032275769383,-7.21534711198306,
122.99239908649));
#227833=CARTESIAN_POINT('Ctrl Pts',(3.4359708315083,-7.12880684220308,123.00063197473));
#227834=CARTESIAN_POINT('Ctrl Pts',(3.6179220623365,-7.03523709272536,123.00886486297));
#227835=CARTESIAN_POINT('Ctrl Pts',(3.79712025935002,-6.9430831109958,123.016973182556));
#227836=CARTESIAN_POINT('Ctrl Pts',(3.97273242345603,-6.84411104754788,
123.025081502143));
#227837=CARTESIAN_POINT('Ctrl Pts',(4.14423535203928,-6.73863742509625,
123.03318982173));
#227838=CARTESIAN_POINT('Ctrl Pts',(4.3196904969638,-6.63073320523344,123.041484994296));
#227839=CARTESIAN_POINT('Ctrl Pts',(4.49084443242895,-6.51602435737667,
123.049780166862));
#227840=CARTESIAN_POINT('Ctrl Pts',(4.65716950940198,-6.39489586785403,
123.058075339428));
#227841=CARTESIAN_POINT('Ctrl Pts',(4.82349458637514,-6.27376737833129,
123.066370511994));
#227842=CARTESIAN_POINT('Ctrl Pts',(4.98499054108189,-6.14621948975367,
123.07466568456));
#227843=CARTESIAN_POINT('Ctrl Pts',(5.14116677031493,-6.01268037066744,
123.082960857126));
#227844=CARTESIAN_POINT('Ctrl Pts',(5.28854722988903,-5.88666211015046,
123.090788849587));
#227845=CARTESIAN_POINT('Ctrl Pts',(5.4314728055252,-5.75506676611666,123.098616842048));
#227846=CARTESIAN_POINT('Ctrl Pts',(5.56949181456856,-5.61824544919976,
123.10644483451));
#227847=CARTESIAN_POINT('Ctrl Pts',(5.70739425040121,-5.48153969390236,
123.114266215315));
#227848=CARTESIAN_POINT('Ctrl Pts',(5.84039812283548,-5.33961700065488,
123.12208759612));
#227849=CARTESIAN_POINT('Ctrl Pts',(5.96808476805478,-5.19286868708545,
123.129908976925));
#227850=CARTESIAN_POINT('Ctrl Pts',(6.09568611569148,-5.04621840472653,
123.13772513287));
#227851=CARTESIAN_POINT('Ctrl Pts',(6.21797707986872,-4.89474918651374,
123.145541288814));
#227852=CARTESIAN_POINT('Ctrl Pts',(6.33457572928104,-4.73888925065817,
123.153357444759));
#227853=CARTESIAN_POINT('Ctrl Pts',(6.45111836426451,-4.58310419050083,
123.161169845793));
#227854=CARTESIAN_POINT('Ctrl Pts',(6.56197392101166,-4.4229328955581,123.168982246827));
#227855=CARTESIAN_POINT('Ctrl Pts',(6.66680056193569,-4.25883684441819,
123.176794647862));
#227856=CARTESIAN_POINT('Ctrl Pts',(6.77159656318468,-4.09478875675054,
123.184604765417));
#227857=CARTESIAN_POINT('Ctrl Pts',(6.87036697022981,-3.92681849502103,
123.192414882972));
#227858=CARTESIAN_POINT('Ctrl Pts',(6.96281303026298,-3.75541684844707,
123.200225000527));
#227859=CARTESIAN_POINT('Ctrl Pts',(7.05526435759767,-3.58400543591711,
123.20803556308));
#227860=CARTESIAN_POINT('Ctrl Pts',(7.14139044505814,-3.40916255485171,
123.215846125632));
#227861=CARTESIAN_POINT('Ctrl Pts',(7.22093809887062,-3.23140433438446,
123.223656688185));
#227862=CARTESIAN_POINT('Ctrl Pts',(7.28292354456225,-3.09289085230257,
123.22974286644));
#227863=CARTESIAN_POINT('Ctrl Pts',(7.34091552061425,-2.95260775733558,
123.235829044696));
#227864=CARTESIAN_POINT('Ctrl Pts',(7.39481435040327,-2.81080801960395,
123.241915222951));
#227865=CARTESIAN_POINT('Ctrl Pts',(7.47133291377299,-2.6094991552019,123.250555588955));
#227866=CARTESIAN_POINT('Ctrl Pts',(7.53956441781505,-2.40522911851261,
123.259195954958));
#227867=CARTESIAN_POINT('Ctrl Pts',(7.59932669159849,-2.19867115193672,
123.267836320962));
#227868=CARTESIAN_POINT('Ctrl Pts',(7.65918837936401,-1.99176957812021,
123.276491060133));
#227869=CARTESIAN_POINT('Ctrl Pts',(7.71055261176152,-1.78257268759434,
123.285145799304));
#227870=CARTESIAN_POINT('Ctrl Pts',(7.75328795444121,-1.5717655345238,123.293800538475));
#227871=CARTESIAN_POINT('Ctrl Pts',(7.79734505487777,-1.35443834505475,
123.302722959334));
#227872=CARTESIAN_POINT('Ctrl Pts',(7.83223096106478,-1.13539997541228,
123.311645380192));
#227873=CARTESIAN_POINT('Ctrl Pts',(7.85785924489575,-0.915406514837176,
123.32056780105));
#227874=CARTESIAN_POINT('Ctrl Pts',(7.88280207198479,-0.701297022214343,
123.329251581914));
#227875=CARTESIAN_POINT('Ctrl Pts',(7.89897612254177,-0.486283093931356,
123.337935362777));
#227876=CARTESIAN_POINT('Ctrl Pts',(7.90635476831299,-0.271063235379707,
123.34661914364));
#227877=CARTESIAN_POINT('Ctrl Pts',(7.91403757422244,-0.0469716537561526,
123.355660884496));
#227878=CARTESIAN_POINT('Ctrl Pts',(7.91218454176299,0.177342906246704,
123.364702625352));
#227879=CARTESIAN_POINT('Ctrl Pts',(7.90082554757362,0.401094336544378,
123.373744366208));
#227880=CARTESIAN_POINT('Ctrl Pts',(7.88946655338425,0.624845766842052,
123.382786107064));
#227881=CARTESIAN_POINT('Ctrl Pts',(7.86860164337229,0.848033791804023,
123.39182784792));
#227882=CARTESIAN_POINT('Ctrl Pts',(7.83832126366524,1.06987885649423,123.400869588776));
#227883=CARTESIAN_POINT('Ctrl Pts',(7.81045128427076,1.27406445262936,123.409191582549));
#227884=CARTESIAN_POINT('Ctrl Pts',(7.77458145061864,1.47728584554186,123.417513576321));
#227885=CARTESIAN_POINT('Ctrl Pts',(7.73079461732031,1.67890904602105,123.425835570094));
#227886=CARTESIAN_POINT('Ctrl Pts',(7.6870467287885,1.8803529193401,123.434150162141));
#227887=CARTESIAN_POINT('Ctrl Pts',(7.63539594948841,2.08020115117116,123.442464754188));
#227888=CARTESIAN_POINT('Ctrl Pts',(7.57597647629685,2.2778282267539,123.450779346235));
#227889=CARTESIAN_POINT('Ctrl Pts',(7.5166062281239,2.47529158165804,123.459087050205));
#227890=CARTESIAN_POINT('Ctrl Pts',(7.44948020934234,2.67053717200129,123.467394754175));
#227891=CARTESIAN_POINT('Ctrl Pts',(7.37478311745651,2.8629521425407,123.475702458144));
#227892=CARTESIAN_POINT('Ctrl Pts',(7.30016139156988,3.05517297504677,123.484001780015));
#227893=CARTESIAN_POINT('Ctrl Pts',(7.21798394589666,3.24456861660356,123.492301101886));
#227894=CARTESIAN_POINT('Ctrl Pts',(7.12848461841886,3.43054340374315,123.500600423756));
#227895=CARTESIAN_POINT('Ctrl Pts',(7.03904247213368,3.61639937144105,123.508894443184));
#227896=CARTESIAN_POINT('Ctrl Pts',(6.94228790147491,3.79883858145367,123.517188462611));
#227897=CARTESIAN_POINT('Ctrl Pts',(6.83850255380036,3.97728598690941,123.525482482038));
#227898=CARTESIAN_POINT('Ctrl Pts',(6.73479416812338,4.15560106473805,123.533770351037));
#227899=CARTESIAN_POINT('Ctrl Pts',(6.62406555767608,4.32992999363992,123.542058220037));
#227900=CARTESIAN_POINT('Ctrl Pts',(6.5066441945941,4.49972247199256,123.550346089036));
#227901=CARTESIAN_POINT('Ctrl Pts',(6.46188383887172,4.5644463989729,123.553505377558));
#227902=CARTESIAN_POINT('Ctrl Pts',(6.41615143597175,4.62851140192374,123.556664666079));
#227903=CARTESIAN_POINT('Ctrl Pts',(6.36946683968058,4.691888018507,123.559823954601));
#227904=CARTESIAN_POINT('Ctrl Pts',(6.24973954643923,4.85442365897783,123.567926264428));
#227905=CARTESIAN_POINT('Ctrl Pts',(6.12379677769075,5.01236119801416,123.576028574254));
#227906=CARTESIAN_POINT('Ctrl Pts',(5.99202601781401,5.16522460323266,123.58413088408));
#227907=CARTESIAN_POINT('Ctrl Pts',(5.86022617302179,5.3181217490111,123.592234982278));
#227908=CARTESIAN_POINT('Ctrl Pts',(5.72259597978328,5.46594228571265,123.600339080475));
#227909=CARTESIAN_POINT('Ctrl Pts',(5.57956179768789,5.60824492562351,123.608443178672));
#227910=CARTESIAN_POINT('Ctrl Pts',(5.43647810270944,5.75059682518593,123.616550082194));
#227911=CARTESIAN_POINT('Ctrl Pts',(5.28798691399609,5.88742679360696,123.624656985716));
#227912=CARTESIAN_POINT('Ctrl Pts',(5.13455027690787,6.01833153406368,123.632763889237));
#227913=CARTESIAN_POINT('Ctrl Pts',(4.98097526316701,6.14935433080829,123.64087810396));
#227914=CARTESIAN_POINT('Ctrl Pts',(4.8224461313417,6.27444101413242,123.648992318683));
#227915=CARTESIAN_POINT('Ctrl Pts',(4.65945779159124,6.3932287686567,123.657106533407));
#227916=CARTESIAN_POINT('Ctrl Pts',(4.49638979418653,6.51207457858479,123.665224713808));
#227917=CARTESIAN_POINT('Ctrl Pts',(4.32885850323306,6.62461513689218,123.673342894209));
#227918=CARTESIAN_POINT('Ctrl Pts',(4.15738721186806,6.73053137356895,123.681461074611));
#227919=CARTESIAN_POINT('Ctrl Pts',(3.98573151928705,6.83656151317771,123.68958798535));
#227920=CARTESIAN_POINT('Ctrl Pts',(3.81012763456716,6.93595293457076,123.69771489609));
#227921=CARTESIAN_POINT('Ctrl Pts',(3.6311240385482,7.02843220189805,123.705841806829));
#227922=CARTESIAN_POINT('Ctrl Pts',(3.53614401773036,7.07750206938291,123.710153978028));
#227923=CARTESIAN_POINT('Ctrl Pts',(3.44020721014769,7.12462668468802,123.714466149226));
#227924=CARTESIAN_POINT('Ctrl Pts',(3.34339780309826,7.16977071671317,123.718778320425));
#227925=CARTESIAN_POINT('Ctrl Pts',(3.16384529748392,7.25349939877722,123.726776108728));
#227926=CARTESIAN_POINT('Ctrl Pts',(2.98097834721167,7.33055742192057,123.734773897032));
#227927=CARTESIAN_POINT('Ctrl Pts',(2.79532843593177,7.40067969414102,123.742771685335));
#227928=CARTESIAN_POINT('Ctrl Pts',(2.60983010757826,7.47074471161163,123.750762943454));
#227929=CARTESIAN_POINT('Ctrl Pts',(2.42155365801753,7.53388514623878,123.758754201573));
#227930=CARTESIAN_POINT('Ctrl Pts',(2.23105237594926,7.58988315428974,123.766745459692));
#227931=CARTESIAN_POINT('Ctrl Pts',(2.04067433415934,7.64584493575984,123.774731548057));
#227932=CARTESIAN_POINT('Ctrl Pts',(1.84807464843812,7.69467340592027,123.782717636421));
#227933=CARTESIAN_POINT('Ctrl Pts',(1.65382406139739,7.73619977598453,123.790703724786));
#227934=CARTESIAN_POINT('Ctrl Pts',(1.45966621477226,7.7777063202512,123.798686000379));
#227935=CARTESIAN_POINT('Ctrl Pts',(1.26385936444381,7.81191764378851,123.806668275971));
#227936=CARTESIAN_POINT('Ctrl Pts',(1.06698720773853,7.83871541124707,123.814650551564));
#227937=CARTESIAN_POINT('Ctrl Pts',(0.870175684351306,7.86550492544329,
123.82263036875));
#227938=CARTESIAN_POINT('Ctrl Pts',(0.672299839827818,7.88488539044696,
123.830610185936));
#227939=CARTESIAN_POINT('Ctrl Pts',(0.473951717323491,7.89678990284319,
123.838590003122));
#227940=CARTESIAN_POINT('Ctrl Pts',(0.268787359032186,7.90910351396139,
123.846844046828));
#227941=CARTESIAN_POINT('Ctrl Pts',(0.0631180567972388,7.91341816727462,
123.855098090534));
#227942=CARTESIAN_POINT('Ctrl Pts',(-0.142396639791706,7.90971833866264,
123.863352134241));
#227943=CARTESIAN_POINT('Ctrl Pts',(-0.341110331361759,7.90614094680762,
123.871333030607));
#227944=CARTESIAN_POINT('Ctrl Pts',(-0.539679135429459,7.89507104707969,
123.879313926974));
#227945=CARTESIAN_POINT('Ctrl Pts',(-0.737508079962727,7.87654764677963,
123.88729482334));
#227946=CARTESIAN_POINT('Ctrl Pts',(-0.935380945047946,7.85802013404816,
123.895277491568));
#227947=CARTESIAN_POINT('Ctrl Pts',(-1.13251328977988,7.83203585266932,
123.903260159795));
#227948=CARTESIAN_POINT('Ctrl Pts',(-1.32831602618527,7.79868562865432,
123.911242828023));
#227949=CARTESIAN_POINT('Ctrl Pts',(-1.52419233146929,7.76532287397387,
123.919228495575));
#227950=CARTESIAN_POINT('Ctrl Pts',(-1.71873770263018,7.72458871529149,
123.927214163127));
#227951=CARTESIAN_POINT('Ctrl Pts',(-1.91137361827227,7.6766250326151,123.935199830679));
#227952=CARTESIAN_POINT('Ctrl Pts',(-2.1041115294198,7.62863595446642,123.943189726425));
#227953=CARTESIAN_POINT('Ctrl Pts',(-2.29493764514277,7.57340980180064,
123.951179622172));
#227954=CARTESIAN_POINT('Ctrl Pts',(-2.4832886008591,7.5111383108583,123.959169517919));
#227955=CARTESIAN_POINT('Ctrl Pts',(-2.67186267383087,7.44879305419442,
123.967168878357));
#227956=CARTESIAN_POINT('Ctrl Pts',(-2.85795541194302,7.37938589245465,
123.975168238795));
#227957=CARTESIAN_POINT('Ctrl Pts',(-3.04102225315112,7.30315717041881,
123.983167599233));
#227958=CARTESIAN_POINT('Ctrl Pts',(-3.2242170683971,7.22687516021075,123.991172551675));
#227959=CARTESIAN_POINT('Ctrl Pts',(-3.40438146507005,7.1437622187103,123.999177504116));
#227960=CARTESIAN_POINT('Ctrl Pts',(-3.58099504504441,7.05410486790262,
124.007182456558));
#227961=CARTESIAN_POINT('Ctrl Pts',(-3.75783912015371,6.96433050693538,
124.015197856116));
#227962=CARTESIAN_POINT('Ctrl Pts',(-3.93112283067098,6.8679948382716,124.023213255674));
#227963=CARTESIAN_POINT('Ctrl Pts',(-4.10035333979208,6.76542855175161,
124.031228655232));
#227964=CARTESIAN_POINT('Ctrl Pts',(-4.13876803016639,6.74214638968775,
124.033048120846));
#227965=CARTESIAN_POINT('Ctrl Pts',(-4.17697399988309,6.71854334881586,
124.03486758646));
#227966=CARTESIAN_POINT('Ctrl Pts',(-4.21496571850726,6.69462358850806,
124.036687052075));
#227967=CARTESIAN_POINT('Ctrl Pts',(-4.37701665040925,6.5925955784805,124.044447851245));
#227968=CARTESIAN_POINT('Ctrl Pts',(-4.53564849664404,6.48449884468234,
124.052208650415));
#227969=CARTESIAN_POINT('Ctrl Pts',(-4.69036243648762,6.37059033484229,
124.059969449585));
#227970=CARTESIAN_POINT('Ctrl Pts',(-4.84488855513684,6.25682010880774,
124.067720827221));
#227971=CARTESIAN_POINT('Ctrl Pts',(-4.99550594919141,6.13725235992835,
124.075472204858));
#227972=CARTESIAN_POINT('Ctrl Pts',(-5.14174053642776,6.0121897222273,124.083223582494));
#227973=CARTESIAN_POINT('Ctrl Pts',(-5.2878272802938,5.88725352302624,124.090967123477));
#227974=CARTESIAN_POINT('Ctrl Pts',(-5.42953976775175,5.75683372497429,
124.09871066446));
#227975=CARTESIAN_POINT('Ctrl Pts',(-5.5664329848305,5.62127608514215,124.106454205443));
#227976=CARTESIAN_POINT('Ctrl Pts',(-5.70321554909599,5.48582801855642,
124.114191487207));
#227977=CARTESIAN_POINT('Ctrl Pts',(-5.83518634509595,5.34525062963367,
124.121928768972));
#227978=CARTESIAN_POINT('Ctrl Pts',(-5.96193348509867,5.19992981868594,
124.129666050736));
#227979=CARTESIAN_POINT('Ctrl Pts',(-6.08860383628698,5.05469704927337,
124.137398644925));
#227980=CARTESIAN_POINT('Ctrl Pts',(-6.21005659804115,4.90472684985828,
124.145131239115));
#227981=CARTESIAN_POINT('Ctrl Pts',(-6.32591675451383,4.75044189680931,
124.152863833304));
#227982=CARTESIAN_POINT('Ctrl Pts',(-6.44173015949393,4.59621920029491,
124.160593307264));
#227983=CARTESIAN_POINT('Ctrl Pts',(-6.55195523855155,4.43768550440512,
124.168322781223));
#227984=CARTESIAN_POINT('Ctrl Pts',(-6.6562572436728,4.27529654013067,124.176052255183));
#227985=CARTESIAN_POINT('Ctrl Pts',(-6.76055756674769,4.11291019465313,
124.183781604492));
#227986=CARTESIAN_POINT('Ctrl Pts',(-6.8589348028198,3.94666900067388,124.1915109538));
#227987=CARTESIAN_POINT('Ctrl Pts',(-6.95109732638403,3.77705797667137,
124.199240303109));
#227988=CARTESIAN_POINT('Ctrl Pts',(-7.0432635759693,3.6074400954972,124.206969964906));
#227989=CARTESIAN_POINT('Ctrl Pts',(-7.12921444026285,3.43445242826447,
124.214699626703));
#227990=CARTESIAN_POINT('Ctrl Pts',(-7.20870417949355,3.25860477084169,
124.222429288501));
#227991=CARTESIAN_POINT('Ctrl Pts',(-7.28821169761661,3.08271778285119,
124.230160679135));
#227992=CARTESIAN_POINT('Ctrl Pts',(-7.36125506484614,2.90396985815291,
124.237892069769));
#227993=CARTESIAN_POINT('Ctrl Pts',(-7.42763661342504,2.72289098917086,
124.245623460404));
#227994=CARTESIAN_POINT('Ctrl Pts',(-7.49404517623827,2.54173842942528,
124.253357997358));
#227995=CARTESIAN_POINT('Ctrl Pts',(-7.55378639849034,2.3582533734224,124.261092534313));
#227996=CARTESIAN_POINT('Ctrl Pts',(-7.60671240123349,2.17298123436918,
124.268827071267));
#227997=CARTESIAN_POINT('Ctrl Pts',(-7.65970073245708,1.98749090897474,
124.276570716824));
#227998=CARTESIAN_POINT('Ctrl Pts',(-7.70585771668609,1.80020964285619,
124.284314362382));
#227999=CARTESIAN_POINT('Ctrl Pts',(-7.7450863382906,1.61169432971156,124.292058007939));
#228000=CARTESIAN_POINT('Ctrl Pts',(-7.78434009425966,1.42305823198637,
124.299806614966));
#228001=CARTESIAN_POINT('Ctrl Pts',(-7.81665658514349,1.23318686488313,
124.307555221992));
#228002=CARTESIAN_POINT('Ctrl Pts',(-7.84199068151589,1.04264238884574,
124.315303829019));
#228003=CARTESIAN_POINT('Ctrl Pts',(-7.86736316391969,0.851809201257965,
124.323064176677));
#228004=CARTESIAN_POINT('Ctrl Pts',(-7.88573208784973,0.660301223715922,
124.330824524334));
#228005=CARTESIAN_POINT('Ctrl Pts',(-7.89710441926124,0.468681972434038,
124.338584871992));
#228006=CARTESIAN_POINT('Ctrl Pts',(-7.90492543460987,0.336900981259918,
124.343921842569));
#228007=CARTESIAN_POINT('Ctrl Pts',(-7.90943841241537,0.20506733643512,
124.349258813147));
#228008=CARTESIAN_POINT('Ctrl Pts',(-7.91065982831679,0.0733626652666543,
124.354595783724));
#228009=CARTESIAN_POINT('Ctrl Pts',(-7.91089423435946,0.0480867778846261,
124.355620019737));
#228010=CARTESIAN_POINT('Ctrl Pts',(-7.91100749162828,0.0228106579640831,
124.35664425575));
#228011=CARTESIAN_POINT('Ctrl Pts',(-7.91099961596495,-0.00246499540847172,
124.357668491763));
#228012=CARTESIAN_POINT('',(-7.90670614352357,0.00719251646262357,126.357668491763));
#228013=CARTESIAN_POINT('Ctrl Pts',(-7.9265347197683,-0.002480449643483,
124.357668921013));
#228014=CARTESIAN_POINT('Ctrl Pts',(-7.92370808336077,-2.59735768496362,
124.462614119133));
#228015=CARTESIAN_POINT('Ctrl Pts',(-5.80631166365505,-6.49188276010665,
124.620544105861));
#228016=CARTESIAN_POINT('Ctrl Pts',(-0.681732440644431,-8.19901426347268,
124.8314588812));
#228017=CARTESIAN_POINT('Ctrl Pts',(4.7061455593866,-7.34957997120415,125.04339803563));
#228018=CARTESIAN_POINT('Ctrl Pts',(8.31436308495323,-2.64529747305826,
125.255337190066));
#228019=CARTESIAN_POINT('Ctrl Pts',(7.74886771041429,2.78933298220472,125.467276344498));
#228020=CARTESIAN_POINT('Ctrl Pts',(5.48726075163886,6.16493663533192,125.626230710322));
#228021=CARTESIAN_POINT('Ctrl Pts',(1.86399302745116,8.02189509988344,125.785185076148));
#228022=CARTESIAN_POINT('Ctrl Pts',(-3.58466317121117,7.94939191666906,
125.99712423058));
#228023=CARTESIAN_POINT('Ctrl Pts',(-7.43754732069607,4.2296490490804,126.187952035785));
#228024=CARTESIAN_POINT('Ctrl Pts',(-7.91164687381234,0.804141605855872,
126.325795052383));
#228025=CARTESIAN_POINT('Ctrl Pts',(-7.90514438368602,0.00980857580332107,
126.357668491763));
#228026=CARTESIAN_POINT('',(-7.911,-2.14273043752655E-13,128.357668491763));
#228027=CARTESIAN_POINT('Ctrl Pts',(-7.911,-3.84692278032617E-13,126.357668491763));
#228028=CARTESIAN_POINT('Ctrl Pts',(-7.91099999999989,-2.20167589666733,
126.446255927496));
#228029=CARTESIAN_POINT('Ctrl Pts',(-6.94214576672333,-4.38610418338752,
126.534843363228));
#228030=CARTESIAN_POINT('Ctrl Pts',(-3.67820201488187,-7.34180684107687,
126.712018234694));
#228031=CARTESIAN_POINT('Ctrl Pts',(-1.40868175871612,-8.08992666571364,
126.800605670427));
#228032=CARTESIAN_POINT('Ctrl Pts',(2.97309270521433,-7.654542280252,126.977780541892));
#228033=CARTESIAN_POINT('Ctrl Pts',(5.05102072675755,-6.47444880834112,
127.066367977625));
#228034=CARTESIAN_POINT('Ctrl Pts',(7.66951518847956,-2.93425195367499,
127.24354284909));
#228035=CARTESIAN_POINT('Ctrl Pts',(8.18956872247094,-0.601881960096723,
127.332130284823));
#228036=CARTESIAN_POINT('Ctrl Pts',(7.3230668976122,3.71537198232701,127.509305156289));
#228037=CARTESIAN_POINT('Ctrl Pts',(5.94329958849997,5.66643518936732,127.597892592021));
#228038=CARTESIAN_POINT('Ctrl Pts',(2.16154501637526,7.92205913233091,127.775067463487));
#228039=CARTESIAN_POINT('Ctrl Pts',(-0.210816529303931,8.20894963712998,
127.863654899219));
#228040=CARTESIAN_POINT('Ctrl Pts',(-4.42123908576769,6.91982244717625,
128.040829770685));
#228041=CARTESIAN_POINT('Ctrl Pts',(-6.2263162563446,5.35390358803212,128.129417206418));
#228042=CARTESIAN_POINT('Ctrl Pts',(-7.65317280859554,2.31334857514237,
128.264559258688));
#228043=CARTESIAN_POINT('Ctrl Pts',(-7.91100000000003,1.15702837836367,
128.311113875225));
#228044=CARTESIAN_POINT('Ctrl Pts',(-7.911,-2.14273043752655E-13,128.357668491763));
#228045=CARTESIAN_POINT('',(-7.90996818647143,0.00413822696500661,132.357668491763));
#228046=CARTESIAN_POINT('Ctrl Pts',(-7.91099890900509,-0.0041547226431693,
128.364649935517));
#228047=CARTESIAN_POINT('Ctrl Pts',(-7.91056187092003,-0.836318048842218,
128.394870332571));
#228048=CARTESIAN_POINT('Ctrl Pts',(-7.77883880110308,-1.6631115170934,
128.42100714115));
#228049=CARTESIAN_POINT('Ctrl Pts',(-7.46272976525518,-2.63182852547884,
128.45823722325));
#228050=CARTESIAN_POINT('Ctrl Pts',(-7.3984705521292,-2.80739774204712,
128.465296010569));
#228051=CARTESIAN_POINT('Ctrl Pts',(-7.31776670017044,-3.00582065284319,
128.473795593309));
#228052=CARTESIAN_POINT('Ctrl Pts',(-7.30734358154125,-3.03107192632827,
128.474887121511));
#228053=CARTESIAN_POINT('Ctrl Pts',(-7.29394783665126,-3.06305404438618,
128.476282719078));
#228054=CARTESIAN_POINT('Ctrl Pts',(-7.29109621518518,-3.0698356801046,
128.476579399161));
#228055=CARTESIAN_POINT('Ctrl Pts',(-7.28652477886291,-3.08066502378771,
128.477054371261));
#228056=CARTESIAN_POINT('Ctrl Pts',(-7.28481103539682,-3.08471530618037,
128.477232287388));
#228057=CARTESIAN_POINT('Ctrl Pts',(-7.28156578967879,-3.09236737289993,
128.477568935933));
#228058=CARTESIAN_POINT('Ctrl Pts',(-7.28003498956775,-3.09596945543065,
128.477727624505));
#228059=CARTESIAN_POINT('Ctrl Pts',(-7.27657369197578,-3.10409737529657,
128.47808619001));
#228060=CARTESIAN_POINT('Ctrl Pts',(-7.27464164554164,-3.10862254685501,
128.478286164305));
#228061=CARTESIAN_POINT('Ctrl Pts',(-7.26969315929526,-3.12018284106618,
128.478797920278));
#228062=CARTESIAN_POINT('Ctrl Pts',(-7.26667072849489,-3.12721539319168,
128.479110082397));
#228063=CARTESIAN_POINT('Ctrl Pts',(-7.2485528224437,-3.16920380625505,
128.480978960651));
#228064=CARTESIAN_POINT('Ctrl Pts',(-7.23321559758548,-3.20405412042349,
128.482551181611));
#228065=CARTESIAN_POINT('Ctrl Pts',(-6.9583412619347,-3.81660989797856,
128.510538015696));
#228066=CARTESIAN_POINT('Ctrl Pts',(-6.63062074787241,-4.36117418717565,
128.540764195017));
#228067=CARTESIAN_POINT('Ctrl Pts',(-6.03500992369722,-5.12596545496245,
128.58556986693));
#228068=CARTESIAN_POINT('Ctrl Pts',(-5.81181518423438,-5.37770409948623,
128.600831636801));
#228069=CARTESIAN_POINT('Ctrl Pts',(-5.45068436703809,-5.73618295584506,
128.622980773011));
#228070=CARTESIAN_POINT('Ctrl Pts',(-5.32414308190378,-5.85382444858474,
128.630331092741));
#228071=CARTESIAN_POINT('Ctrl Pts',(-5.14801074177935,-6.0071290000049,
128.640014410502));
#228072=CARTESIAN_POINT('Ctrl Pts',(-5.10171692454457,-6.04649469325223,
128.642511030369));
#228073=CARTESIAN_POINT('Ctrl Pts',(-5.03535662851792,-6.10161904559869,
128.646022062702));
#228074=CARTESIAN_POINT('Ctrl Pts',(-5.01566106563755,-6.11781950091623,
128.647055805111));
#228075=CARTESIAN_POINT('Ctrl Pts',(-4.98549722024487,-6.14238699818202,
128.648626397462));
#228076=CARTESIAN_POINT('Ctrl Pts',(-4.97508554255796,-6.15082306811171,
128.649166250643));
#228077=CARTESIAN_POINT('Ctrl Pts',(-4.95578341122672,-6.16638156031196,
128.650162902403));
#228078=CARTESIAN_POINT('Ctrl Pts',(-4.9468989219567,-6.17351130425842,
128.650620018083));
#228079=CARTESIAN_POINT('Ctrl Pts',(-4.93241474997797,-6.18508341285493,
128.651362604191));
#228080=CARTESIAN_POINT('Ctrl Pts',(-4.92682440817282,-6.18953740930448,
128.651648577074));
#228081=CARTESIAN_POINT('Ctrl Pts',(-4.91623889908605,-6.19794778062934,
128.652188874966));
#228082=CARTESIAN_POINT('Ctrl Pts',(-4.91124497525431,-6.20190570692576,
128.652443266777));
#228083=CARTESIAN_POINT('Ctrl Pts',(-4.89961116298036,-6.21110320253402,
128.653034725391));
#228084=CARTESIAN_POINT('Ctrl Pts',(-4.89296763677944,-6.21633817025545,
128.653371594195));
#228085=CARTESIAN_POINT('Ctrl Pts',(-4.87280680605442,-6.23217216440233,
128.654391201656));
#228086=CARTESIAN_POINT('Ctrl Pts',(-4.85926332163606,-6.24273786347078,
128.655072511054));
#228087=CARTESIAN_POINT('Ctrl Pts',(-4.76484084223335,-6.31590636751635,
128.65979738694));
#228088=CARTESIAN_POINT('Ctrl Pts',(-4.68278712545681,-6.37698104705263,
128.663775614509));
#228089=CARTESIAN_POINT('Ctrl Pts',(-4.32708719123494,-6.6311688338786,
128.680506519401));
#228090=CARTESIAN_POINT('Ctrl Pts',(-4.04250279138282,-6.80839779726759,
128.692599434196));
#228091=CARTESIAN_POINT('Ctrl Pts',(-3.57710466557525,-7.05873135385175,
128.711006125476));
#228092=CARTESIAN_POINT('Ctrl Pts',(-3.40337814026,-7.14411545477539,128.717602712292));
#228093=CARTESIAN_POINT('Ctrl Pts',(-2.89711559888655,-7.37027408506629,
128.736371798973));
#228094=CARTESIAN_POINT('Ctrl Pts',(-2.55785952689693,-7.4947686166418,
128.748392646314));
#228095=CARTESIAN_POINT('Ctrl Pts',(-2.0758577420648,-7.63509238835664,
128.766027324354));
#228096=CARTESIAN_POINT('Ctrl Pts',(-1.93938679515738,-7.67089286401137,
128.771082890438));
#228097=CARTESIAN_POINT('Ctrl Pts',(-1.66137032994446,-7.73593171881953,
128.781639553966));
#228098=CARTESIAN_POINT('Ctrl Pts',(-1.51983615823292,-7.76497807917405,
128.787146527096));
#228099=CARTESIAN_POINT('Ctrl Pts',(-1.35516060573402,-7.79409903275928,
128.793790967958));
#228100=CARTESIAN_POINT('Ctrl Pts',(-1.3327103061836,-7.79796917268563,
128.794701879188));
#228101=CARTESIAN_POINT('Ctrl Pts',(-1.30374611714872,-7.80283349003321,
128.7958839942));
#228102=CARTESIAN_POINT('Ctrl Pts',(-1.29724704627652,-7.80391661359336,
128.796149688475));
#228103=CARTESIAN_POINT('Ctrl Pts',(-1.28672527082612,-7.80565664701212,
128.796580574145));
#228104=CARTESIAN_POINT('Ctrl Pts',(-1.28270340212337,-7.80631856867759,
128.796745450504));
#228105=CARTESIAN_POINT('Ctrl Pts',(-1.27498419211388,-7.80758287455877,
128.797062229841));
#228106=CARTESIAN_POINT('Ctrl Pts',(-1.27128692971231,-7.80818574161039,
128.797214102828));
#228107=CARTESIAN_POINT('Ctrl Pts',(-1.26285561166517,-7.80955438561218,
128.797560766761));
#228108=CARTESIAN_POINT('Ctrl Pts',(-1.25812128919059,-7.81031848385381,
128.797755660965));
#228109=CARTESIAN_POINT('Ctrl Pts',(-1.24337808743088,-7.81268421701364,
128.798363313542));
#228110=CARTESIAN_POINT('Ctrl Pts',(-1.23336685890424,-7.81427091496779,
128.798776982208));
#228111=CARTESIAN_POINT('Ctrl Pts',(-1.15686969770765,-7.82624442324337,
128.80194573346));
#228112=CARTESIAN_POINT('Ctrl Pts',(-1.0902585973341,-7.8358014861306,128.80475026061));
#228113=CARTESIAN_POINT('Ctrl Pts',(-0.19853192973562,-7.95215220450645,
128.842822023939));
#228114=CARTESIAN_POINT('Ctrl Pts',(0.638291672826344,-7.9289895672604,
128.884004691237));
#228115=CARTESIAN_POINT('Ctrl Pts',(1.71543711493337,-7.7272748975085,128.933930010972));
#228116=CARTESIAN_POINT('Ctrl Pts',(1.97213451803535,-7.66578139660503,
128.945645356666));
#228117=CARTESIAN_POINT('Ctrl Pts',(2.35427287560337,-7.55376624151274,
128.962712732675));
#228118=CARTESIAN_POINT('Ctrl Pts',(2.48226864710161,-7.51267795379807,
128.968365977846));
#228119=CARTESIAN_POINT('Ctrl Pts',(2.65338786730291,-7.45289532165581,
128.975840211399));
#228120=CARTESIAN_POINT('Ctrl Pts',(2.69747805664161,-7.43705103435778,
128.977758464128));
#228121=CARTESIAN_POINT('Ctrl Pts',(2.76135742078552,-7.41345248165311,
128.980527097822));
#228122=CARTESIAN_POINT('Ctrl Pts',(2.78125976513068,-7.40600881929687,
128.981388194214));
#228123=CARTESIAN_POINT('Ctrl Pts',(2.81682577116757,-7.39254321427327,
128.98292436005));
#228124=CARTESIAN_POINT('Ctrl Pts',(2.83250067671713,-7.38655146337526,
128.983600470272));
#228125=CARTESIAN_POINT('Ctrl Pts',(2.85611137178011,-7.37744003949338,
128.984617515344));
#228126=CARTESIAN_POINT('Ctrl Pts',(2.86406132761681,-7.37435735617696,
128.984959731137));
#228127=CARTESIAN_POINT('Ctrl Pts',(2.87784440894416,-7.36898716347637,
128.985552640318));
#228128=CARTESIAN_POINT('Ctrl Pts',(2.88367982105365,-7.36670556948244,
128.985803538423));
#228129=CARTESIAN_POINT('Ctrl Pts',(2.89569304677875,-7.3619920441611,128.986319801379));
#228130=CARTESIAN_POINT('Ctrl Pts',(2.90187052221981,-7.35955926343366,
128.986585136479));
#228131=CARTESIAN_POINT('Ctrl Pts',(2.9167361504912,-7.35368333336157,128.987223313316));
#228132=CARTESIAN_POINT('Ctrl Pts',(2.92542128910286,-7.35023255557451,
128.987595890229));
#228133=CARTESIAN_POINT('Ctrl Pts',(2.95205758337775,-7.33959473816933,
128.988737711222));
#228134=CARTESIAN_POINT('Ctrl Pts',(2.96998858247982,-7.3323572419146,128.989505204854));
#228135=CARTESIAN_POINT('Ctrl Pts',(3.17456864909349,-7.24890893759965,
128.998248929923));
#228136=CARTESIAN_POINT('Ctrl Pts',(3.35827186305671,-7.16565307873128,
129.005975281876));
#228137=CARTESIAN_POINT('Ctrl Pts',(3.93435451042694,-6.877540937294,129.029983956261));
#228138=CARTESIAN_POINT('Ctrl Pts',(4.31281672067203,-6.64675511712714,
129.045372360403));
#228139=CARTESIAN_POINT('Ctrl Pts',(4.95140949284133,-6.17972572264137,
129.072672902979));
#228140=CARTESIAN_POINT('Ctrl Pts',(5.21889344529578,-5.95555199761565,
129.08461894903));
#228141=CARTESIAN_POINT('Ctrl Pts',(5.63568574651383,-5.55653933214197,
129.105482985821));
#228142=CARTESIAN_POINT('Ctrl Pts',(5.79374395211244,-5.39153193491925,
129.114031790362));
#228143=CARTESIAN_POINT('Ctrl Pts',(5.96911166185044,-5.19182283514702,
129.124549050813));
#228144=CARTESIAN_POINT('Ctrl Pts',(5.99357745023262,-5.16355959249529,
129.126039824246));
#228145=CARTESIAN_POINT('Ctrl Pts',(6.02476760592542,-5.12700791292681,
129.12796978757));
#228146=CARTESIAN_POINT('Ctrl Pts',(6.03167705028848,-5.11887749454685,
129.128399207953));
#228147=CARTESIAN_POINT('Ctrl Pts',(6.04277749584214,-5.10576179948299,
129.129092108232));
#228148=CARTESIAN_POINT('Ctrl Pts',(6.04697884011277,-5.10078526544848,
129.129355058217));
#228149=CARTESIAN_POINT('Ctrl Pts',(6.05496431272556,-5.09130266198775,
129.129856168986));
#228150=CARTESIAN_POINT('Ctrl Pts',(6.05874957008869,-5.08679754571132,
129.130094272729));
#228151=CARTESIAN_POINT('Ctrl Pts',(6.06736076284103,-5.07652547723436,
129.130637231328));
#228152=CARTESIAN_POINT('Ctrl Pts',(6.07218350506904,-5.07075586355209,
129.130942243732));
#228153=CARTESIAN_POINT('Ctrl Pts',(6.08651380507773,-5.05356226852524,
129.13185129953));
#228154=CARTESIAN_POINT('Ctrl Pts',(6.09599737370257,-5.04211839581,129.132456502953));
#228155=CARTESIAN_POINT('Ctrl Pts',(6.16210077008492,-4.96189197258841,
129.136699924102));
#228156=CARTESIAN_POINT('Ctrl Pts',(6.21758625226706,-4.89218543582551,
129.140390386949));
#228157=CARTESIAN_POINT('Ctrl Pts',(6.39621230611836,-4.65982872987308,
129.15267116211));
#228158=CARTESIAN_POINT('Ctrl Pts',(6.51423746133555,-4.49335518141653,
129.16143543403));
#228159=CARTESIAN_POINT('Ctrl Pts',(6.8393047016571,-3.99508117137071,129.187272154833));
#228160=CARTESIAN_POINT('Ctrl Pts',(7.02835188804369,-3.65226481004147,
129.204537393867));
#228161=CARTESIAN_POINT('Ctrl Pts',(7.29706880874307,-3.06612835281899,
129.232514751419));
#228162=CARTESIAN_POINT('Ctrl Pts',(7.39169148306106,-2.83041709841477,
129.243393096487));
#228163=CARTESIAN_POINT('Ctrl Pts',(7.54724344703225,-2.38158595348237,
129.263368775281));
#228164=CARTESIAN_POINT('Ctrl Pts',(7.61087378349197,-2.16966389593463,
129.272507438292));
#228165=CARTESIAN_POINT('Ctrl Pts',(7.67797864688371,-1.90659292153293,
129.283529821171));
#228166=CARTESIAN_POINT('Ctrl Pts',(7.68994976157265,-1.85772048329132,
129.285564339855));
#228167=CARTESIAN_POINT('Ctrl Pts',(7.70589318839512,-1.78983467758121,
129.288372684894));
#228168=CARTESIAN_POINT('Ctrl Pts',(7.71026292040913,-1.77091606410035,
129.289153410071));
#228169=CARTESIAN_POINT('Ctrl Pts',(7.71751234138909,-1.73899442882002,
129.290467506746));
#228170=CARTESIAN_POINT('Ctrl Pts',(7.72042891959213,-1.72599990201667,
129.291001542816));
#228171=CARTESIAN_POINT('Ctrl Pts',(7.72611362560204,-1.7003695389147,129.292053096799));
#228172=CARTESIAN_POINT('Ctrl Pts',(7.72888360267606,-1.68773415621328,
129.292570647105));
#228173=CARTESIAN_POINT('Ctrl Pts',(7.7349371507878,-1.65979315423455,129.293713243481));
#228174=CARTESIAN_POINT('Ctrl Pts',(7.73820631103835,-1.64448445763401,
129.294338020872));
#228175=CARTESIAN_POINT('Ctrl Pts',(7.74898220148479,-1.59327985640897,
129.296423626402));
#228176=CARTESIAN_POINT('Ctrl Pts',(7.7562847979623,-1.55734133066358,129.297880615199));
#228177=CARTESIAN_POINT('Ctrl Pts',(7.83496790036148,-1.15582806876709,
129.314082903022));
#228178=CARTESIAN_POINT('Ctrl Pts',(7.88069636440455,-0.785690813013254,
129.328286311182));
#228179=CARTESIAN_POINT('Ctrl Pts',(7.92257113302998,0.0139858436980569,
129.358012417013));
#228180=CARTESIAN_POINT('Ctrl Pts',(7.91020120737385,0.442764543545203,
129.373355070737));
#228181=CARTESIAN_POINT('Ctrl Pts',(7.82792519090264,1.18773038202908,129.400866729264));
#228182=CARTESIAN_POINT('Ctrl Pts',(7.77324715621524,1.50456557210768,129.412862219009));
#228183=CARTESIAN_POINT('Ctrl Pts',(7.69459519072899,1.83781820207173,129.426509384832));
#228184=CARTESIAN_POINT('Ctrl Pts',(7.68964007831451,1.85844191375176,129.427358275959));
#228185=CARTESIAN_POINT('Ctrl Pts',(7.68272195800677,1.88673447370437,129.428529055246));
#228186=CARTESIAN_POINT('Ctrl Pts',(7.6808302617933,1.89442079463921,129.428847756864));
#228187=CARTESIAN_POINT('Ctrl Pts',(7.67763257676687,1.90733007135076,129.429384102417));
#228188=CARTESIAN_POINT('Ctrl Pts',(7.67633278405058,1.91255456738065,129.429601464126));
#228189=CARTESIAN_POINT('Ctrl Pts',(7.67376218915766,1.92284219700226,129.43003006821));
#228190=CARTESIAN_POINT('Ctrl Pts',(7.67249170635665,1.92790540899385,129.4302412958));
#228191=CARTESIAN_POINT('Ctrl Pts',(7.66969557617082,1.93900219198646,129.430704861462));
#228192=CARTESIAN_POINT('Ctrl Pts',(7.66816781978634,1.94503522304873,129.430957297891));
#228193=CARTESIAN_POINT('Ctrl Pts',(7.66288293442325,1.96580195635749,129.431827651203));
#228194=CARTESIAN_POINT('Ctrl Pts',(7.65909046459879,1.98052655834565,129.43244724182));
#228195=CARTESIAN_POINT('Ctrl Pts',(7.61456441630623,2.15136228279456,129.439665379117));
#228196=CARTESIAN_POINT('Ctrl Pts',(7.56911161931509,2.30618498420136,129.446509692779));
#228197=CARTESIAN_POINT('Ctrl Pts',(7.38674054891172,2.86371458039327,129.472047860212));
#228198=CARTESIAN_POINT('Ctrl Pts',(7.22214316172528,3.25659528591906,129.491720937577));
#228199=CARTESIAN_POINT('Ctrl Pts',(6.83393336215497,4.00717968178939,129.530684589541));
#228200=CARTESIAN_POINT('Ctrl Pts',(6.61170364121456,4.364121204987,129.549905582059));
#228201=CARTESIAN_POINT('Ctrl Pts',(6.19941041373206,4.92201592749204,129.580282507631));
#228202=CARTESIAN_POINT('Ctrl Pts',(6.02529962231773,5.13368419490476,129.591909539464));
#228203=CARTESIAN_POINT('Ctrl Pts',(5.82034681200733,5.35802024933356,129.604335771708));
#228204=CARTESIAN_POINT('Ctrl Pts',(5.8000202062194,5.38001706656734,129.605555472827));
#228205=CARTESIAN_POINT('Ctrl Pts',(5.76424083456069,5.41829793479299,129.607680452746));
#228206=CARTESIAN_POINT('Ctrl Pts',(5.74884282671335,5.43463256100433,129.608587948841));
#228207=CARTESIAN_POINT('Ctrl Pts',(5.72639942560201,5.45823901289664,129.609900591646));
#228208=CARTESIAN_POINT('Ctrl Pts',(5.7194093351351,5.46556313306869,129.610308012999));
#228209=CARTESIAN_POINT('Ctrl Pts',(5.70712460314805,5.47838553111681,129.611021578854));
#228210=CARTESIAN_POINT('Ctrl Pts',(5.70183603547348,5.48388959483867,129.611327973871));
#228211=CARTESIAN_POINT('Ctrl Pts',(5.6916354340797,5.49447513732278,129.611917424181));
#228212=CARTESIAN_POINT('Ctrl Pts',(5.68672454250177,5.49955770286471,129.612200526311));
#228213=CARTESIAN_POINT('Ctrl Pts',(5.67511487104764,5.51154104533416,129.612868203183));
#228214=CARTESIAN_POINT('Ctrl Pts',(5.66841029815454,5.51843620843801,129.613252536329));
#228215=CARTESIAN_POINT('Ctrl Pts',(5.64506487534329,5.54235783487604,129.614586466451));
#228216=CARTESIAN_POINT('Ctrl Pts',(5.62835967856365,5.55932146556517,129.615533372154));
#228217=CARTESIAN_POINT('Ctrl Pts',(5.42982145560681,5.75911896850382,129.626698178582));
#228218=CARTESIAN_POINT('Ctrl Pts',(5.23922370564749,5.93303975847275,129.636531279462));
#228219=CARTESIAN_POINT('Ctrl Pts',(4.69071232634645,6.38647440461411,129.662807833496));
#228220=CARTESIAN_POINT('Ctrl Pts',(4.31672502951896,6.6449790715276,129.678512860951));
#228221=CARTESIAN_POINT('Ctrl Pts',(3.59903318321788,7.05476708264577,129.707030019479));
#228222=CARTESIAN_POINT('Ctrl Pts',(3.26279447726962,7.21643458756564,129.719841866464));
#228223=CARTESIAN_POINT('Ctrl Pts',(2.7640030883237,7.41424960547021,129.739418952232));
#228224=CARTESIAN_POINT('Ctrl Pts',(2.60973700464503,7.4699450087469,129.745550763118));
#228225=CARTESIAN_POINT('Ctrl Pts',(2.38187893319387,7.54428965627332,129.754844284878));
#228226=CARTESIAN_POINT('Ctrl Pts',(2.30956975471727,7.56673906792916,129.757829598441));
#228227=CARTESIAN_POINT('Ctrl Pts',(2.22382234453675,7.59201702819807,129.761404961232));
#228228=CARTESIAN_POINT('Ctrl Pts',(2.21068245770068,7.59585356920209,129.761953806811));
#228229=CARTESIAN_POINT('Ctrl Pts',(2.19048857530311,7.60169287531331,129.762798700322));
#228230=CARTESIAN_POINT('Ctrl Pts',(2.18344160423823,7.60371997969149,129.763093801772));
#228231=CARTESIAN_POINT('Ctrl Pts',(2.17056123802547,7.60740571361684,129.763633652466));
#228232=CARTESIAN_POINT('Ctrl Pts',(2.16472872954231,7.6090674400245,129.763878283658));
#228233=CARTESIAN_POINT('Ctrl Pts',(2.15297506109052,7.6124015424406,129.764371609715));
#228234=CARTESIAN_POINT('Ctrl Pts',(2.14705384957303,7.61407372067037,129.764620311764));
#228235=CARTESIAN_POINT('Ctrl Pts',(2.13013549411853,7.61883024008114,129.765331407609));
#228236=CARTESIAN_POINT('Ctrl Pts',(2.11913363642794,7.6218976692058,129.765794421546));
#228237=CARTESIAN_POINT('Ctrl Pts',(2.07175039714012,7.63499807193604,129.767791003711));
#228238=CARTESIAN_POINT('Ctrl Pts',(2.03530442199564,7.64479438065512,129.76933294534));
#228239=CARTESIAN_POINT('Ctrl Pts',(1.86715990434793,7.6887022893419,129.776471483367));
#228240=CARTESIAN_POINT('Ctrl Pts',(1.73466802360506,7.71967317729758,129.78216561357));
#228241=CARTESIAN_POINT('Ctrl Pts',(1.18074385469772,7.83417635993924,129.8061114203));
#228242=CARTESIAN_POINT('Ctrl Pts',(0.753657426327338,7.88672796529521,
129.824851198811));
#228243=CARTESIAN_POINT('Ctrl Pts',(-0.10329475129395,7.92189989176989,
129.86171757323));
#228244=CARTESIAN_POINT('Ctrl Pts',(-0.531739692208522,7.90471047675374,
129.879782875525));
#228245=CARTESIAN_POINT('Ctrl Pts',(-1.27556625247278,7.81409206508833,
129.910739577785));
#228246=CARTESIAN_POINT('Ctrl Pts',(-1.59177649401483,7.75585960544128,
129.923832175341));
#228247=CARTESIAN_POINT('Ctrl Pts',(-1.95921065679009,7.66477010664329,
129.939157039336));
#228248=CARTESIAN_POINT('Ctrl Pts',(-2.01470023209559,7.65037189980341,
129.941473024668));
#228249=CARTESIAN_POINT('Ctrl Pts',(-2.0985775730029,7.62763188156648,129.94497638038));
#228250=CARTESIAN_POINT('Ctrl Pts',(-2.12708297004477,7.61973188476867,
129.94616743269));
#228251=CARTESIAN_POINT('Ctrl Pts',(-2.17652852498675,7.60572943706828,
129.948234254787));
#228252=CARTESIAN_POINT('Ctrl Pts',(-2.19748897189781,7.59969992243665,
129.949110657456));
#228253=CARTESIAN_POINT('Ctrl Pts',(-2.24450538002941,7.58596433426751,
129.951077122105));
#228254=CARTESIAN_POINT('Ctrl Pts',(-2.27054713296442,7.578210541027,129.952166738374));
#228255=CARTESIAN_POINT('Ctrl Pts',(-2.34032906498078,7.5570413524738,129.95508769805));
#228256=CARTESIAN_POINT('Ctrl Pts',(-2.38399375773189,7.54338040434978,
129.956916703571));
#228257=CARTESIAN_POINT('Ctrl Pts',(-2.58419937770159,7.47883203969176,
129.96530957834));
#228258=CARTESIAN_POINT('Ctrl Pts',(-2.73924811821045,7.42344502553817,
129.971827676718));
#228259=CARTESIAN_POINT('Ctrl Pts',(-2.91680045747469,7.35369839627158,
129.979331609379));
#228260=CARTESIAN_POINT('Ctrl Pts',(-2.94109573515341,7.34401531133811,
129.9803593054));
#228261=CARTESIAN_POINT('Ctrl Pts',(-3.08790237325577,7.28465897130143,
129.986575254708));
#228262=CARTESIAN_POINT('Ctrl Pts',(-3.20920157800645,7.23204142069894,
129.991736183988));
#228263=CARTESIAN_POINT('Ctrl Pts',(-3.67902000432681,7.01409330374899,
130.011879698824));
#228264=CARTESIAN_POINT('Ctrl Pts',(-4.0165722542617,6.82640736964534,130.026670153766));
#228265=CARTESIAN_POINT('Ctrl Pts',(-4.5213793949347,6.49527367366471,130.050165149765));
#228266=CARTESIAN_POINT('Ctrl Pts',(-4.69864996365079,6.36821292940971,
130.058715309478));
#228267=CARTESIAN_POINT('Ctrl Pts',(-4.89042197340382,6.2183869931454,130.068458733938));
#228268=CARTESIAN_POINT('Ctrl Pts',(-4.91032686411225,6.20268119058127,
130.069476245164));
#228269=CARTESIAN_POINT('Ctrl Pts',(-4.94011874340805,6.1789408551341,130.071008853701));
#228270=CARTESIAN_POINT('Ctrl Pts',(-4.95006244745346,6.1709776417661,130.071522030045));
#228271=CARTESIAN_POINT('Ctrl Pts',(-4.96713987380967,6.1572336954251,130.072406232153));
#228272=CARTESIAN_POINT('Ctrl Pts',(-4.97428285649951,6.15146448978461,
130.072776935103));
#228273=CARTESIAN_POINT('Ctrl Pts',(-4.98898736199602,6.13954567505202,
130.073541875344));
#228274=CARTESIAN_POINT('Ctrl Pts',(-4.99654759509067,6.13339450252123,
130.073936157213));
#228275=CARTESIAN_POINT('Ctrl Pts',(-5.01476880137936,6.11851327846581,
130.07488886193));
#228276=CARTESIAN_POINT('Ctrl Pts',(-5.02541832663489,6.10976935012077,
130.075447696393));
#228277=CARTESIAN_POINT('Ctrl Pts',(-5.06847217445395,6.0742307171994,130.077715260372));
#228278=CARTESIAN_POINT('Ctrl Pts',(-5.10068521770798,6.04720590428966,
130.07943091401));
#228279=CARTESIAN_POINT('Ctrl Pts',(-5.4145561294069,5.77959475056108,130.096327834523));
#228280=CARTESIAN_POINT('Ctrl Pts',(-5.67919828794121,5.51976723743063,
130.111988896187));
#228281=CARTESIAN_POINT('Ctrl Pts',(-6.24671695867545,4.87838608170758,
130.14811202078));
#228282=CARTESIAN_POINT('Ctrl Pts',(-6.53456480729434,4.48549027533,130.168433166312));
#228283=CARTESIAN_POINT('Ctrl Pts',(-6.81429437817311,4.01903724463986,
130.190529702024));
#228284=CARTESIAN_POINT('Ctrl Pts',(-6.84350456336735,3.96909480972181,
130.192872426639));
#228285=CARTESIAN_POINT('Ctrl Pts',(-6.88533379836675,3.89574206738144,
130.196280723487));
#228286=CARTESIAN_POINT('Ctrl Pts',(-6.89838670088746,3.87258165857005,
130.19735218012));
#228287=CARTESIAN_POINT('Ctrl Pts',(-6.92114982179581,3.83171163264294,
130.199234849875));
#228288=CARTESIAN_POINT('Ctrl Pts',(-6.93090941794958,3.81402982874741,
130.20004671747));
#228289=CARTESIAN_POINT('Ctrl Pts',(-6.94980348913918,3.77948676315984,
130.201627710446));
#228290=CARTESIAN_POINT('Ctrl Pts',(-6.95894457708538,3.76262928097667,
130.202396918238));
#228291=CARTESIAN_POINT('Ctrl Pts',(-6.98079279379227,3.72198605489603,
130.204245936735));
#228292=CARTESIAN_POINT('Ctrl Pts',(-6.99343978463542,3.69816822332976,
130.205324963003));
#228293=CARTESIAN_POINT('Ctrl Pts',(-7.0398361039095,3.6097017930393,130.20931638759));
#228294=CARTESIAN_POINT('Ctrl Pts',(-7.07281294742987,3.54465182177587,
130.212218993939));
#228295=CARTESIAN_POINT('Ctrl Pts',(-7.48334848831802,2.70628494892475,
130.249246710995));
#228296=CARTESIAN_POINT('Ctrl Pts',(-7.73319894900463,1.87676860163868,
130.281950644593));
#228297=CARTESIAN_POINT('Ctrl Pts',(-7.88891258386936,0.683148131472218,
130.326963227141));
#228298=CARTESIAN_POINT('Ctrl Pts',(-7.91111459673225,0.340420927446174,
130.339740904145));
#228299=CARTESIAN_POINT('Ctrl Pts',(-7.91094715504957,-0.158919179004584,
130.358948104736));
#228300=CARTESIAN_POINT('Ctrl Pts',(-7.90626464627182,-0.31514545146595,
130.365044852001));
#228301=CARTESIAN_POINT('Ctrl Pts',(-7.8959248475961,-0.488460202016362,
130.371980140228));
#228302=CARTESIAN_POINT('Ctrl Pts',(-7.894833592724,-0.505791563732877,
130.372675583515));
#228303=CARTESIAN_POINT('Ctrl Pts',(-7.89310764544519,-0.531835507013181,
130.373723662075));
#228304=CARTESIAN_POINT('Ctrl Pts',(-7.89251556967546,-0.540550914221878,
130.374074904111));
#228305=CARTESIAN_POINT('Ctrl Pts',(-7.89146638534851,-0.555625719132479,
130.374683342913));
#228306=CARTESIAN_POINT('Ctrl Pts',(-7.89101602141004,-0.561985587401749,
130.374940314203));
#228307=CARTESIAN_POINT('Ctrl Pts',(-7.89006612743187,-0.57517334290341,
130.375473755316));
#228308=CARTESIAN_POINT('Ctrl Pts',(-7.88956542179449,-0.582001137892017,
130.375750264801));
#228309=CARTESIAN_POINT('Ctrl Pts',(-7.8883708615974,-0.598005723140507,
130.376399193497));
#228310=CARTESIAN_POINT('Ctrl Pts',(-7.88766985631753,-0.607181959476842,
130.37677185914));
#228311=CARTESIAN_POINT('Ctrl Pts',(-7.88534843961067,-0.636886994390217,
130.377980238666));
#228312=CARTESIAN_POINT('Ctrl Pts',(-7.88366389126807,-0.657410600373982,
130.378818213768));
#228313=CARTESIAN_POINT('Ctrl Pts',(-7.85574887837748,-0.981963582256113,
130.392121191229));
#228314=CARTESIAN_POINT('Ctrl Pts',(-7.81203550088187,-1.28416447278493,
130.405368504632));
#228315=CARTESIAN_POINT('Ctrl Pts',(-7.60526204055151,-2.29657986755635,
130.451737270648));
#228316=CARTESIAN_POINT('Ctrl Pts',(-7.36166477587235,-2.98670651743664,
130.486064968325));
#228317=CARTESIAN_POINT('Ctrl Pts',(-6.92138990662583,-3.8381279818609,
130.527355029864));
#228318=CARTESIAN_POINT('Ctrl Pts',(-6.80682966955358,-4.03781449679715,
130.536989878815));
#228319=CARTESIAN_POINT('Ctrl Pts',(-6.67169625797304,-4.25122278565904,
130.54722595989));
#228320=CARTESIAN_POINT('Ctrl Pts',(-6.65959155835353,-4.27015999918037,
130.548133780671));
#228321=CARTESIAN_POINT('Ctrl Pts',(-6.64242977747168,-4.29675830184028,
130.549408192292));
#228322=CARTESIAN_POINT('Ctrl Pts',(-6.63743986873736,-4.30446248011,130.549777245159));
#228323=CARTESIAN_POINT('Ctrl Pts',(-6.62873999585265,-4.31784356570039,
130.550418103538));
#228324=CARTESIAN_POINT('Ctrl Pts',(-6.62503612423523,-4.32352441225514,
130.550690133039));
#228325=CARTESIAN_POINT('Ctrl Pts',(-6.61729763272182,-4.33536010037516,
130.551256802566));
#228326=CARTESIAN_POINT('Ctrl Pts',(-6.61326171877062,-4.34151409065737,
130.551551394426));
#228327=CARTESIAN_POINT('Ctrl Pts',(-6.6037086360126,-4.35603646900358,
130.552246467948));
#228328=CARTESIAN_POINT('Ctrl Pts',(-6.59818413273516,-4.36440002979814,
130.552646677419));
#228329=CARTESIAN_POINT('Ctrl Pts',(-6.57994574852593,-4.39189739061122,
130.553962184657));
#228330=CARTESIAN_POINT('Ctrl Pts',(-6.56716436534541,-4.41098639229762,
130.554874970822));
#228331=CARTESIAN_POINT('Ctrl Pts',(-6.33239244413116,-4.75833600826952,
130.571476716409));
#228332=CARTESIAN_POINT('Ctrl Pts',(-6.08612144810702,-5.06952919780342,
130.586185620073));
#228333=CARTESIAN_POINT('Ctrl Pts',(-5.40931165844547,-5.80397849971194,
130.621624330112));
#228334=CARTESIAN_POINT('Ctrl Pts',(-4.95184523238778,-6.19887101719241,
130.641308498791));
#228335=CARTESIAN_POINT('Ctrl Pts',(-4.36253865693198,-6.60033556069919,
130.666325569196));
#228336=CARTESIAN_POINT('Ctrl Pts',(-4.26976414064126,-6.66072715354705,
130.670260277475));
#228337=CARTESIAN_POINT('Ctrl Pts',(-4.13358030302506,-6.74536141243194,
130.676071222838));
#228338=CARTESIAN_POINT('Ctrl Pts',(-4.09116010634702,-6.77117386944939,
130.677886126856));
#228339=CARTESIAN_POINT('Ctrl Pts',(-3.9610349422242,-6.84868511425587,
130.683475983347));
#228340=CARTESIAN_POINT('Ctrl Pts',(-3.87257475343541,-6.89909045433856,
130.687306948206));
#228341=CARTESIAN_POINT('Ctrl Pts',(-3.73249063600178,-6.97536841249642,
130.69345706889));
#228342=CARTESIAN_POINT('Ctrl Pts',(-3.68151258041225,-7.00240784800352,
130.695712104521));
#228343=CARTESIAN_POINT('Ctrl Pts',(-3.60600701792215,-7.04140458558351,
130.699083059605));
#228344=CARTESIAN_POINT('Ctrl Pts',(-3.58170532336805,-7.05379699835596,
130.700172679809));
#228345=CARTESIAN_POINT('Ctrl Pts',(-3.55054418252642,-7.06948476915608,
130.701576374706));
#228346=CARTESIAN_POINT('Ctrl Pts',(-3.54374315800858,-7.07289638851776,
130.701883131242));
#228347=CARTESIAN_POINT('Ctrl Pts',(-3.53291341633145,-7.07830940471843,
130.702372244711));
#228348=CARTESIAN_POINT('Ctrl Pts',(-3.52888788124158,-7.08031719329628,
130.70255419494));
#228349=CARTESIAN_POINT('Ctrl Pts',(-3.5213671453463,-7.0840602520952,130.702894392296));
#228350=CARTESIAN_POINT('Ctrl Pts',(-3.51787236697227,-7.08579637283116,
130.70305258488));
#228351=CARTESIAN_POINT('Ctrl Pts',(-3.51009740587929,-7.08965161428452,
130.703404764067));
#228352=CARTESIAN_POINT('Ctrl Pts',(-3.50581658887822,-7.09176944461953,
130.703598833655));
#228353=CARTESIAN_POINT('Ctrl Pts',(-3.49338332400954,-7.09790649193071,
130.704162972476));
#228354=CARTESIAN_POINT('Ctrl Pts',(-3.48522587417126,-7.10191553193301,
130.704533703228));
#228355=CARTESIAN_POINT('Ctrl Pts',(-3.42282419987054,-7.13244989618076,
130.707374348834));
#228356=CARTESIAN_POINT('Ctrl Pts',(-3.36828620527822,-7.15836676088272,
130.709883861813));
#228357=CARTESIAN_POINT('Ctrl Pts',(-3.18242524124949,-7.24409505234318,
130.718511162981));
#228358=CARTESIAN_POINT('Ctrl Pts',(-3.04976919386851,-7.30093468406857,
130.724794313426));
#228359=CARTESIAN_POINT('Ctrl Pts',(-2.74491364720468,-7.42179891708394,
130.739381180108));
#228360=CARTESIAN_POINT('Ctrl Pts',(-2.57188746323626,-7.48351789944077,
130.747763540692));
#228361=CARTESIAN_POINT('Ctrl Pts',(-1.87024865897849,-7.70658555893855,
130.781729527731));
#228362=CARTESIAN_POINT('Ctrl Pts',(-1.32746337206994,-7.81839083765405,
130.807805887729));
#228363=CARTESIAN_POINT('Ctrl Pts',(-0.605502295850416,-7.88968564964103,
130.839885127073));
#228364=CARTESIAN_POINT('Ctrl Pts',(-0.43304584130309,-7.90102835415054,
130.847370768208));
#228365=CARTESIAN_POINT('Ctrl Pts',(-0.108900807741692,-7.91170164029605,
130.861081545278));
#228366=CARTESIAN_POINT('Ctrl Pts',(0.0426639127485166,-7.91233629472284,
130.867345853968));
#228367=CARTESIAN_POINT('Ctrl Pts',(0.213453486238489,-7.90814333950836,
130.874242794877));
#228368=CARTESIAN_POINT('Ctrl Pts',(0.23274542477781,-7.90759906948013,
130.875019539904));
#228369=CARTESIAN_POINT('Ctrl Pts',(0.260806475700599,-7.90670462293567,
130.876146013363));
#228370=CARTESIAN_POINT('Ctrl Pts',(0.269577224197976,-7.90641044551862,
130.876497628714));
#228371=CARTESIAN_POINT('Ctrl Pts',(0.285051348138922,-7.9058656531978,
130.877117145507));
#228372=CARTESIAN_POINT('Ctrl Pts',(0.29175491991475,-7.90562110554905,
130.877385251292));
#228373=CARTESIAN_POINT('Ctrl Pts',(0.305608344632387,-7.90509808524587,
130.877938742926));
#228374=CARTESIAN_POINT('Ctrl Pts',(0.31275814860346,-7.90481843804919,
130.878224088902));
#228375=CARTESIAN_POINT('Ctrl Pts',(0.331047414985672,-7.90407824532979,
130.878953208763));
#228376=CARTESIAN_POINT('Ctrl Pts',(0.342186319213008,-7.90360385037199,
130.879396515041));
#228377=CARTESIAN_POINT('Ctrl Pts',(0.3874866545255,-7.90157860794142,130.881196318539));
#228378=CARTESIAN_POINT('Ctrl Pts',(0.4216391151913,-7.89982980206562,130.882546130952));
#228379=CARTESIAN_POINT('Ctrl Pts',(0.642704926114706,-7.88707226245944,
130.891238545469));
#228380=CARTESIAN_POINT('Ctrl Pts',(0.829194890535647,-7.86965185391553,
130.898361753168));
#228381=CARTESIAN_POINT('Ctrl Pts',(1.16429993988588,-7.82630311803096,
130.910859990856));
#228382=CARTESIAN_POINT('Ctrl Pts',(1.31312090800703,-7.80271304095509,
130.916302435787));
#228383=CARTESIAN_POINT('Ctrl Pts',(1.94282853979077,-7.68436825528129,
130.939018531948));
#228384=CARTESIAN_POINT('Ctrl Pts',(2.4150306847506,-7.54928621885128,130.955190881259));
#228385=CARTESIAN_POINT('Ctrl Pts',(3.06268251901901,-7.29697992622877,
130.978878383457));
#228386=CARTESIAN_POINT('Ctrl Pts',(3.2507162750062,-7.21517695087289,130.985960865659));
#228387=CARTESIAN_POINT('Ctrl Pts',(3.49069392962469,-7.09948949748859,
130.995517325331));
#228388=CARTESIAN_POINT('Ctrl Pts',(3.54572043577076,-7.07216809678589,
130.997745173024));
#228389=CARTESIAN_POINT('Ctrl Pts',(3.6842575373213,-7.0013592862187,131.003460988402));
#228390=CARTESIAN_POINT('Ctrl Pts',(3.76731868403214,-6.95701762966985,
131.006987661926));
#228391=CARTESIAN_POINT('Ctrl Pts',(3.92066106283459,-6.8716053810305,131.013723306125));
#228392=CARTESIAN_POINT('Ctrl Pts',(3.99113846528694,-6.8309118381627,131.016910111055));
#228393=CARTESIAN_POINT('Ctrl Pts',(4.06913227931461,-6.78425927305019,
131.020554014006));
#228394=CARTESIAN_POINT('Ctrl Pts',(4.07728258699863,-6.77936413645787,
131.020936245805));
#228395=CARTESIAN_POINT('Ctrl Pts',(4.08950222005293,-6.77199492562322,
131.021511524471));
#228396=CARTESIAN_POINT('Ctrl Pts',(4.09357818913035,-6.76953183683631,
131.021703783102));
#228397=CARTESIAN_POINT('Ctrl Pts',(4.10064421631865,-6.76525315475101,
131.022037722703));
#228398=CARTESIAN_POINT('Ctrl Pts',(4.1036352811846,-6.7634392667957,131.022179279961));
#228399=CARTESIAN_POINT('Ctrl Pts',(4.10986349334535,-6.75965660527918,
131.02247445561));
#228400=CARTESIAN_POINT('Ctrl Pts',(4.11310043046326,-6.75768748937437,
131.022628098535));
#228401=CARTESIAN_POINT('Ctrl Pts',(4.12073008184018,-6.75303865452489,
131.022990792916));
#228402=CARTESIAN_POINT('Ctrl Pts',(4.12512159400354,-6.7503569765844,131.023199983893));
#228403=CARTESIAN_POINT('Ctrl Pts',(4.13950967279792,-6.74155160923391,
131.023886764865));
#228404=CARTESIAN_POINT('Ctrl Pts',(4.14949520089733,-6.73541001023058,
131.024365619414));
#228405=CARTESIAN_POINT('Ctrl Pts',(4.50425717106616,-6.51612531719592,
131.04145614003));
#228406=CARTESIAN_POINT('Ctrl Pts',(4.83212219284879,-6.27684185932895,
131.059854790864));
#228407=CARTESIAN_POINT('Ctrl Pts',(5.46436521001771,-5.73642090136131,
131.098573312149));
#228408=CARTESIAN_POINT('Ctrl Pts',(5.76563343454988,-5.43353517267719,
131.118861876848));
#228409=CARTESIAN_POINT('Ctrl Pts',(6.36707653687011,-4.72221163336846,
131.161751988428));
#228410=CARTESIAN_POINT('Ctrl Pts',(6.65549635243849,-4.30620995182937,
131.183953658628));
#228411=CARTESIAN_POINT('Ctrl Pts',(6.91910937631706,-3.8354958025182,131.205915473879));
#228412=CARTESIAN_POINT('Ctrl Pts',(6.93571003823924,-3.80539471262152,
131.207307472985));
#228413=CARTESIAN_POINT('Ctrl Pts',(6.9577906603516,-3.76473261010134,131.209171402791));
#228414=CARTESIAN_POINT('Ctrl Pts',(6.96344362836989,-3.75426628451074,
131.209649715423));
#228415=CARTESIAN_POINT('Ctrl Pts',(6.97227729335187,-3.73782238628518,
131.210398928716));
#228416=CARTESIAN_POINT('Ctrl Pts',(6.97547394770028,-3.73185343389311,
131.210670415605));
#228417=CARTESIAN_POINT('Ctrl Pts',(6.98159595285452,-3.72038677200616,
131.211191058068));
#228418=CARTESIAN_POINT('Ctrl Pts',(6.9845224821248,-3.71488969946119,131.211440256731));
#228419=CARTESIAN_POINT('Ctrl Pts',(6.99138177683038,-3.70196872371084,
131.212025077482));
#228420=CARTESIAN_POINT('Ctrl Pts',(6.99530921698123,-3.69454199328287,
131.212360504682));
#228421=CARTESIAN_POINT('Ctrl Pts',(7.0066246321403,-3.67306198425774,131.213328584568));
#228422=CARTESIAN_POINT('Ctrl Pts',(7.01398216103787,-3.65899266526142,
131.21396012719));
#228423=CARTESIAN_POINT('Ctrl Pts',(7.06360765230317,-3.56339739235665,
131.218234084477));
#228424=CARTESIAN_POINT('Ctrl Pts',(7.10449645715328,-3.48116142289665,
131.221826367483));
#228425=CARTESIAN_POINT('Ctrl Pts',(7.18096130069846,-3.32041285917845,
131.228694820407));
#228426=CARTESIAN_POINT('Ctrl Pts',(7.21670418007605,-3.2419944602089,131.231976363417));
#228427=CARTESIAN_POINT('Ctrl Pts',(7.37733024898325,-2.87376084165445,
131.247088627686));
#228428=CARTESIAN_POINT('Ctrl Pts',(7.48608588906328,-2.57721515750595,
131.258395927004));
#228429=CARTESIAN_POINT('Ctrl Pts',(7.69998956580586,-1.86479861383034,
131.284430489986));
#228430=CARTESIAN_POINT('Ctrl Pts',(7.78962790029915,-1.44533534284104,
131.298880235897));
#228431=CARTESIAN_POINT('Ctrl Pts',(7.88680415239507,-0.698452646272621,
131.325551606683));
#228432=CARTESIAN_POINT('Ctrl Pts',(7.90883663642662,-0.373937185808327,
131.337495310781));
#228433=CARTESIAN_POINT('Ctrl Pts',(7.91099372363021,-0.0255011837131471,
131.351379417631));
#228434=CARTESIAN_POINT('Ctrl Pts',(7.91103456431694,-0.00202776225569635,
131.352319127705));
#228435=CARTESIAN_POINT('Ctrl Pts',(7.91094843688656,0.0297438130795243,
131.353596689119));
#228436=CARTESIAN_POINT('Ctrl Pts',(7.91091288363323,0.0380422450148598,
131.353930897875));
#228437=CARTESIAN_POINT('Ctrl Pts',(7.91083067877513,0.0520755478662569,
131.354496939756));
#228438=CARTESIAN_POINT('Ctrl Pts',(7.91079084802368,0.057810461949476,
131.354728506332));
#228439=CARTESIAN_POINT('Ctrl Pts',(7.91070232387717,0.0688308166460872,
131.35517395658));
#228440=CARTESIAN_POINT('Ctrl Pts',(7.91065456947036,0.0741162644690045,
131.355387804022));
#228441=CARTESIAN_POINT('Ctrl Pts',(7.91052977514755,0.0865492319514098,
131.355891317345));
#228442=CARTESIAN_POINT('Ctrl Pts',(7.91044834517563,0.0936966964467147,
131.356181149983));
#228443=CARTESIAN_POINT('Ctrl Pts',(7.91018433197714,0.114406289302989,
131.35702199774));
#228444=CARTESIAN_POINT('Ctrl Pts',(7.90997655776122,0.127968034002399,
131.357573953337));
#228445=CARTESIAN_POINT('Ctrl Pts',(7.90832600963994,0.220213333147443,
131.361337047475));
#228446=CARTESIAN_POINT('Ctrl Pts',(7.90574411678412,0.298870625549505,
131.364589157162));
#228447=CARTESIAN_POINT('Ctrl Pts',(7.89362925044877,0.552481152398151,
131.375192762896));
#228448=CARTESIAN_POINT('Ctrl Pts',(7.87945794921925,0.727156734810832,
131.382676654555));
#228449=CARTESIAN_POINT('Ctrl Pts',(7.7716684952341,1.6671923623803,131.423568638727));
#228450=CARTESIAN_POINT('Ctrl Pts',(7.57230951313802,2.41634109516279,131.457891496573));
#228451=CARTESIAN_POINT('Ctrl Pts',(7.20290668976725,3.27551191870523,131.496712989455));
#228452=CARTESIAN_POINT('Ctrl Pts',(7.13342156389494,3.4241995096306,131.503432513099));
#228453=CARTESIAN_POINT('Ctrl Pts',(7.04622159119718,3.5965997524717,131.511242978615));
#228454=CARTESIAN_POINT('Ctrl Pts',(7.03293867726194,3.62250494389511,131.512417171674));
#228455=CARTESIAN_POINT('Ctrl Pts',(7.01164104571621,3.66348225247664,131.514275431587));
#228456=CARTESIAN_POINT('Ctrl Pts',(7.00372003802315,3.67860272383894,131.514961316352));
#228457=CARTESIAN_POINT('Ctrl Pts',(6.98971296462401,3.70513169279424,131.516165040947));
#228458=CARTESIAN_POINT('Ctrl Pts',(6.98364775887051,3.71655111225107,131.516683294972));
#228459=CARTESIAN_POINT('Ctrl Pts',(6.97196187460413,3.73842339381317,131.51767614622));
#228460=CARTESIAN_POINT('Ctrl Pts',(6.96634561878001,3.74887857538239,131.518150831547));
#228461=CARTESIAN_POINT('Ctrl Pts',(6.95155944863181,3.77625643920008,131.519394080109));
#228462=CARTESIAN_POINT('Ctrl Pts',(6.94235125094906,3.79315839042393,131.520161851769));
#228463=CARTESIAN_POINT('Ctrl Pts',(6.90869572393306,3.85440114100887,131.522944692225));
#228464=CARTESIAN_POINT('Ctrl Pts',(6.88388438649135,3.89854082803961,131.524952060594));
#228465=CARTESIAN_POINT('Ctrl Pts',(6.82282275927925,4.00476956525558,131.529787516396));
#228466=CARTESIAN_POINT('Ctrl Pts',(6.78614636501044,4.06660883263131,131.532606076452));
#228467=CARTESIAN_POINT('Ctrl Pts',(6.62755730968866,4.32588078857785,131.544442900794));
#228468=CARTESIAN_POINT('Ctrl Pts',(6.49783043401172,4.51840307414474,131.553275960361));
#228469=CARTESIAN_POINT('Ctrl Pts',(6.11657028029414,5.0337639721956,131.577246613157));
#228470=CARTESIAN_POINT('Ctrl Pts',(5.84818566009107,5.34321433293493,131.591986630454));
#228471=CARTESIAN_POINT('Ctrl Pts',(5.32500385328593,5.85957107808733,131.618797505408));
#228472=CARTESIAN_POINT('Ctrl Pts',(5.07900515266533,6.0740368180053,131.630791900848));
#228473=CARTESIAN_POINT('Ctrl Pts',(4.76057620459584,6.31874555688031,131.646428534573));
#228474=CARTESIAN_POINT('Ctrl Pts',(4.70000391809516,6.3639291230061,131.649408269933));
#228475=CARTESIAN_POINT('Ctrl Pts',(4.62835075171268,6.41579742219139,131.652950318863));
#228476=CARTESIAN_POINT('Ctrl Pts',(4.6178880243812,6.42333226876395,131.653467949892));
#228477=CARTESIAN_POINT('Ctrl Pts',(4.60207960846132,6.43465828356091,131.654250763827));
#228478=CARTESIAN_POINT('Ctrl Pts',(4.59674751986884,6.43846846594865,131.654514924134));
#228479=CARTESIAN_POINT('Ctrl Pts',(4.58722308571632,6.44525653527459,131.654987008186));
#228480=CARTESIAN_POINT('Ctrl Pts',(4.58303255505015,6.44823697166854,131.655194792889));
#228481=CARTESIAN_POINT('Ctrl Pts',(4.57418602009187,6.45451592392825,131.655633614745));
#228482=CARTESIAN_POINT('Ctrl Pts',(4.56952934885523,6.45781349129409,131.655864703849));
#228483=CARTESIAN_POINT('Ctrl Pts',(4.55720824186382,6.46651853974445,131.656476420007));
#228484=CARTESIAN_POINT('Ctrl Pts',(4.54953776548107,6.47191742097055,131.656857524846));
#228485=CARTESIAN_POINT('Ctrl Pts',(4.51532689407749,6.49590594206585,131.658558618974));
#228486=CARTESIAN_POINT('Ctrl Pts',(4.4886821612934,6.51434596906616,131.659887086957));
#228487=CARTESIAN_POINT('Ctrl Pts',(4.41854378725765,6.56225202832388,131.663395425983));
#228488=CARTESIAN_POINT('Ctrl Pts',(4.37486935980116,6.59144891154052,131.665591119698));
#228489=CARTESIAN_POINT('Ctrl Pts',(4.18222597206528,6.71747528828708,131.675314119173));
#228490=CARTESIAN_POINT('Ctrl Pts',(4.030316427061,6.80970126991515,131.683079322232));
#228491=CARTESIAN_POINT('Ctrl Pts',(3.57064907029234,7.06799947699284,131.706603090643));
#228492=CARTESIAN_POINT('Ctrl Pts',(3.25484851122357,7.21887109479932,131.722785671932));
#228493=CARTESIAN_POINT('Ctrl Pts',(2.30051042776497,7.59940805275421,131.770143569925));
#228494=CARTESIAN_POINT('Ctrl Pts',(1.6411541164364,7.76854150435772,131.800685987257));
#228495=CARTESIAN_POINT('Ctrl Pts',(0.923734459519948,7.8570125549352,131.830250308261));
#228496=CARTESIAN_POINT('Ctrl Pts',(0.879185110662258,7.86212218579703,
131.832072835756));
#228497=CARTESIAN_POINT('Ctrl Pts',(0.820769300509547,7.86831951791108,
131.834445501075));
#228498=CARTESIAN_POINT('Ctrl Pts',(0.806940458294124,7.86974976602352,
131.835005928705));
#228499=CARTESIAN_POINT('Ctrl Pts',(0.785596700086403,7.87190039414498,
131.835868980404));
#228500=CARTESIAN_POINT('Ctrl Pts',(0.778084434378132,7.87264648030756,
131.836172376977));
#228501=CARTESIAN_POINT('Ctrl Pts',(0.763125459445799,7.8741105213042,131.836775793019));
#228502=CARTESIAN_POINT('Ctrl Pts',(0.755678777170742,7.8748286682747,131.837075817971));
#228503=CARTESIAN_POINT('Ctrl Pts',(0.739173761606479,7.87639676029255,
131.83774000679));
#228504=CARTESIAN_POINT('Ctrl Pts',(0.730114952277006,7.87724164492489,
131.838104018211));
#228505=CARTESIAN_POINT('Ctrl Pts',(0.703990730607179,7.87963271155895,
131.839152251478));
#228506=CARTESIAN_POINT('Ctrl Pts',(0.686921680075027,7.88113908187342,
131.839835276647));
#228507=CARTESIAN_POINT('Ctrl Pts',(0.572489277602448,7.89086333412594,
131.844401935068));
#228508=CARTESIAN_POINT('Ctrl Pts',(0.474983928235118,7.89733241114043,
131.848232796594));
#228509=CARTESIAN_POINT('Ctrl Pts',(0.209217416272467,7.91002482681946,
131.85852275347));
#228510=CARTESIAN_POINT('Ctrl Pts',(0.040835140910128,7.91268606893869,
131.864876189681));
#228511=CARTESIAN_POINT('Ctrl Pts',(-0.297661556367035,7.90722946366799,
131.877385067391));
#228512=CARTESIAN_POINT('Ctrl Pts',(-0.467684352132172,7.89899704895067,
131.883534334743));
#228513=CARTESIAN_POINT('Ctrl Pts',(-0.850894902728228,7.86802477374352,
131.897206312108));
#228514=CARTESIAN_POINT('Ctrl Pts',(-1.06368980779961,7.84209173778786,
131.904665435726));
#228515=CARTESIAN_POINT('Ctrl Pts',(-1.46461698824881,7.77661010817831,
131.918716868003));
#228516=CARTESIAN_POINT('Ctrl Pts',(-1.6528722614479,7.73878418070761,131.925314438363));
#228517=CARTESIAN_POINT('Ctrl Pts',(-2.29167004799866,7.58605647036536,
131.948093758971));
#228518=CARTESIAN_POINT('Ctrl Pts',(-2.73336750502716,7.43832651494931,
131.964526792273));
#228519=CARTESIAN_POINT('Ctrl Pts',(-3.18963915183753,7.23955812774204,
131.984222122834));
#228520=CARTESIAN_POINT('Ctrl Pts',(-3.21966877286616,7.22625302312937,
131.985530418814));
#228521=CARTESIAN_POINT('Ctrl Pts',(-3.25948427929215,7.20831467279348,
131.987280321433));
#228522=CARTESIAN_POINT('Ctrl Pts',(-3.26934502896877,7.20384767114533,
131.987714955105));
#228523=CARTESIAN_POINT('Ctrl Pts',(-3.28468332133363,7.19686131788961,
131.988392940262));
#228524=CARTESIAN_POINT('Ctrl Pts',(-3.29016722678858,7.19435591070613,
131.988635722847));
#228525=CARTESIAN_POINT('Ctrl Pts',(-3.30117281597283,7.1893126214522,131.989123721389));
#228526=CARTESIAN_POINT('Ctrl Pts',(-3.30669445001531,7.18677464123304,
131.98936894119));
#228527=CARTESIAN_POINT('Ctrl Pts',(-3.31906022764567,7.18107353068025,
131.989918969774));
#228528=CARTESIAN_POINT('Ctrl Pts',(-3.32590278035102,7.17790697508421,
131.990223913795));
#228529=CARTESIAN_POINT('Ctrl Pts',(-3.34604527187692,7.16855056768209,
131.991123293318));
#228530=CARTESIAN_POINT('Ctrl Pts',(-3.35933249525944,7.16233351539971,
131.991718781771));
#228531=CARTESIAN_POINT('Ctrl Pts',(-3.46030491137074,7.11474603410072,
131.99626042358));
#228532=CARTESIAN_POINT('Ctrl Pts',(-3.54723846981561,7.07180455258907,
132.000264749638));
#228533=CARTESIAN_POINT('Ctrl Pts',(-3.84895828295636,6.91580439792312,
132.014447614189));
#228534=CARTESIAN_POINT('Ctrl Pts',(-4.05930867461679,6.79447110254698,
132.024845285061));
#228535=CARTESIAN_POINT('Ctrl Pts',(-4.48271654169488,6.52355379602759,
132.04651220676));
#228536=CARTESIAN_POINT('Ctrl Pts',(-4.694653459865,6.37273349570443,132.057776401105));
#228537=CARTESIAN_POINT('Ctrl Pts',(-5.20093430068734,5.97346481957138,
132.0854879719));
#228538=CARTESIAN_POINT('Ctrl Pts',(-5.48530798932626,5.71344167026328,
132.101766426826));
#228539=CARTESIAN_POINT('Ctrl Pts',(-5.98411674809319,5.18563482811866,
132.131884562175));
#228540=CARTESIAN_POINT('Ctrl Pts',(-6.20229657354122,4.92259953994062,
132.145810219661));
#228541=CARTESIAN_POINT('Ctrl Pts',(-6.44389387263535,4.58966749226703,
132.162486407668));
#228542=CARTESIAN_POINT('Ctrl Pts',(-6.48423221442287,4.53249915616988,
132.165316053974));
#228543=CARTESIAN_POINT('Ctrl Pts',(-6.54197736644485,4.44831260587567,
132.169434076157));
#228544=CARTESIAN_POINT('Ctrl Pts',(-6.55998617648189,4.4217116906728,132.170728270737));
#228545=CARTESIAN_POINT('Ctrl Pts',(-6.59144070679422,4.37463488785543,
132.173006415794));
#228546=CARTESIAN_POINT('Ctrl Pts',(-6.60495426721267,4.35420487863197,
132.173991043116));
#228547=CARTESIAN_POINT('Ctrl Pts',(-6.63069672704732,4.31489142663367,
132.175878096419));
#228548=CARTESIAN_POINT('Ctrl Pts',(-6.64294038764321,4.29601793745975,
132.176780667927));
#228549=CARTESIAN_POINT('Ctrl Pts',(-6.66894044328155,4.2555621697856,132.178708224298));
#228550=CARTESIAN_POINT('Ctrl Pts',(-6.68267295521114,4.23396483159602,
132.179732948371));
#228551=CARTESIAN_POINT('Ctrl Pts',(-6.73280024654331,4.15427741431908,
132.183498189338));
#228552=CARTESIAN_POINT('Ctrl Pts',(-6.7685445050632,4.09578141101457,132.18623164309));
#228553=CARTESIAN_POINT('Ctrl Pts',(-6.93598247194728,3.81358750531054,
132.199277272731));
#228554=CARTESIAN_POINT('Ctrl Pts',(-7.05737464637724,3.58396006838076,
132.209468635308));
#228555=CARTESIAN_POINT('Ctrl Pts',(-7.25448840815833,3.16208503612219,
132.227604503703));
#228556=CARTESIAN_POINT('Ctrl Pts',(-7.33438974739932,2.97205513817852,
132.235573410499));
#228557=CARTESIAN_POINT('Ctrl Pts',(-7.54507205021783,2.41055488400625,
132.258754609685));
#228558=CARTESIAN_POINT('Ctrl Pts',(-7.65565638841629,2.03218969031106,
132.273909238018));
#228559=CARTESIAN_POINT('Ctrl Pts',(-7.74662623168385,1.60485990944624,
132.291318220727));
#228560=CARTESIAN_POINT('Ctrl Pts',(-7.75528824480562,1.56246519802373,
132.293048720586));
#228561=CARTESIAN_POINT('Ctrl Pts',(-7.76673552693982,1.50399675412808,
132.295441524756));
#228562=CARTESIAN_POINT('Ctrl Pts',(-7.76981958350817,1.48798206266565,
132.296097559713));
#228563=CARTESIAN_POINT('Ctrl Pts',(-7.77466025913748,1.46242028333684,
132.297145802009));
#228564=CARTESIAN_POINT('Ctrl Pts',(-7.77644887100753,1.4528792744493,132.297537308999));
#228565=CARTESIAN_POINT('Ctrl Pts',(-7.77998983362453,1.4337968121707,132.298320861744));
#228566=CARTESIAN_POINT('Ctrl Pts',(-7.78174220361343,1.42425537940682,
132.298712906321));
#228567=CARTESIAN_POINT('Ctrl Pts',(-7.78523658949436,1.40502991446249,
132.299503404207));
#228568=CARTESIAN_POINT('Ctrl Pts',(-7.78697809747688,1.39534580791992,
132.299901868415));
#228569=CARTESIAN_POINT('Ctrl Pts',(-7.79091587444081,1.37321180477954,
132.300813270469));
#228570=CARTESIAN_POINT('Ctrl Pts',(-7.79310036643597,1.36075989811202,
132.301326489492));
#228571=CARTESIAN_POINT('Ctrl Pts',(-7.79871935068607,1.32827356421151,
132.302666729167));
#228572=CARTESIAN_POINT('Ctrl Pts',(-7.80210647919657,1.30823111629935,
132.303494843883));
#228573=CARTESIAN_POINT('Ctrl Pts',(-7.81212380183295,1.24753337073086,
132.30600627133));
#228574=CARTESIAN_POINT('Ctrl Pts',(-7.81851370903775,1.20683932001855,
132.307694791727));
#228575=CARTESIAN_POINT('Ctrl Pts',(-7.88191327525664,0.781424354597747,
132.32538857553));
#228576=CARTESIAN_POINT('Ctrl Pts',(-7.91079421575543,0.393060249264107,
132.341872565054));
#228577=CARTESIAN_POINT('Ctrl Pts',(-7.91099890422817,0.00416380844229285,
132.358262606746));
#228578=CARTESIAN_POINT('',(-7.90831251326435,6.9057182936028E-7,134.357573016214));
#228579=CARTESIAN_POINT('Ctrl Pts',(-7.90996818647143,0.00413822696500661,
132.357668491763));
#228580=CARTESIAN_POINT('Ctrl Pts',(-7.90766063577685,-0.852908314836981,
132.392201808104));
#228581=CARTESIAN_POINT('Ctrl Pts',(-7.55022317271499,-3.02898935298784,
132.479719913055));
#228582=CARTESIAN_POINT('Ctrl Pts',(-4.88042203922493,-7.22662596088967,
132.67320759522));
#228583=CARTESIAN_POINT('Ctrl Pts',(2.32377147178489,-9.06459362976759,
132.938131538262));
#228584=CARTESIAN_POINT('Ctrl Pts',(8.89536617229082,-2.9274547798747,133.256040269912));
#228585=CARTESIAN_POINT('Ctrl Pts',(7.52945874066786,4.39853555416276,133.520964212952));
#228586=CARTESIAN_POINT('Ctrl Pts',(3.14753813267379,7.60142069634967,133.732903367385));
#228587=CARTESIAN_POINT('Ctrl Pts',(-2.24296169861593,8.43405333923822,
133.944842521819));
#228588=CARTESIAN_POINT('Ctrl Pts',(-7.0276043223463,5.11216238889513,134.153065738094));
#228589=CARTESIAN_POINT('Ctrl Pts',(-7.91025855294315,1.22824022493078,
134.308304165763));
#228590=CARTESIAN_POINT('Ctrl Pts',(-7.90831251326434,6.90571829360795E-7,
134.357573016214));
#228591=CARTESIAN_POINT('',(-3.42280818030014,7.13531452195942,137.99828572006));
#228592=CARTESIAN_POINT('Ctrl Pts',(-7.91099999973896,6.42667422549036E-5,
134.359122557131));
#228593=CARTESIAN_POINT('Ctrl Pts',(-7.91100135031142,-0.166186245076805,
134.365941313037));
#228594=CARTESIAN_POINT('Ctrl Pts',(-7.90576200601237,-0.33239889165738,
134.372723415823));
#228595=CARTESIAN_POINT('Ctrl Pts',(-7.88937324703694,-0.592057096643569,
134.383300304956));
#228596=CARTESIAN_POINT('Ctrl Pts',(-7.88178839485409,-0.685677559252165,
134.3871077824));
#228597=CARTESIAN_POINT('Ctrl Pts',(-7.86946744438583,-0.810169954690298,
134.392162194791));
#228598=CARTESIAN_POINT('Ctrl Pts',(-7.86621312090279,-0.841180336018112,
134.393420517128));
#228599=CARTESIAN_POINT('Ctrl Pts',(-7.86014286011769,-0.89590482591113,
134.395639873494));
#228600=CARTESIAN_POINT('Ctrl Pts',(-7.85740272414143,-0.919626920377347,
134.396601518469));
#228601=CARTESIAN_POINT('Ctrl Pts',(-7.85176327288654,-0.966583008271905,
134.398504236969));
#228602=CARTESIAN_POINT('Ctrl Pts',(-7.8488681346898,-0.989817262399845,
134.399445336393));
#228603=CARTESIAN_POINT('Ctrl Pts',(-7.84290721123858,-1.03598395442221,
134.401314580324));
#228604=CARTESIAN_POINT('Ctrl Pts',(-7.83984388676748,-1.05891648034513,
134.402242737066));
#228605=CARTESIAN_POINT('Ctrl Pts',(-7.83134082075238,-1.12051163170326,
134.404734784321));
#228606=CARTESIAN_POINT('Ctrl Pts',(-7.82571538047249,-1.15914803525641,
134.406296981637));
#228607=CARTESIAN_POINT('Ctrl Pts',(-7.8036641938834,-1.30311565030008,
134.41211485197));
#228608=CARTESIAN_POINT('Ctrl Pts',(-7.78539586097027,-1.40815370973349,
134.416352972435));
#228609=CARTESIAN_POINT('Ctrl Pts',(-7.73609108725339,-1.66123031908117,
134.426556913989));
#228610=CARTESIAN_POINT('Ctrl Pts',(-7.70292122824836,-1.80881090519743,
134.432500884393));
#228611=CARTESIAN_POINT('Ctrl Pts',(-7.53848515129802,-2.4534477816681,
134.458509361132));
#228612=CARTESIAN_POINT('Ctrl Pts',(-7.36318540038592,-2.93796781686119,
134.478107978626));
#228613=CARTESIAN_POINT('Ctrl Pts',(-7.07122565761197,-3.5508975194716,
134.504645549634));
#228614=CARTESIAN_POINT('Ctrl Pts',(-6.9956869956998,-3.69749468422313,
134.51114146088));
#228615=CARTESIAN_POINT('Ctrl Pts',(-6.90622925658279,-3.85853505902265,
134.518512217244));
#228616=CARTESIAN_POINT('Ctrl Pts',(-6.89677176691106,-3.87541411167201,
134.519287716281));
#228617=CARTESIAN_POINT('Ctrl Pts',(-6.88109707876542,-3.90315007570101,
134.520567065991));
#228618=CARTESIAN_POINT('Ctrl Pts',(-6.87491586138241,-3.91402726338345,
134.52107006877));
#228619=CARTESIAN_POINT('Ctrl Pts',(-6.86382403384081,-3.93343839076604,
134.521970055588));
#228620=CARTESIAN_POINT('Ctrl Pts',(-6.85892324040459,-3.94197792016819,
134.522366799251));
#228621=CARTESIAN_POINT('Ctrl Pts',(-6.84942366647437,-3.95845937960376,
134.523134120481));
#228622=CARTESIAN_POINT('Ctrl Pts',(-6.84482698210708,-3.96640250193163,
134.523504644923));
#228623=CARTESIAN_POINT('Ctrl Pts',(-6.83531418929179,-3.9827749314889,
134.524269881455));
#228624=CARTESIAN_POINT('Ctrl Pts',(-6.83039628642708,-3.99120317585423,
134.524664639442));
#228625=CARTESIAN_POINT('Ctrl Pts',(-6.81847338446442,-4.01154992815681,
134.525619664446));
#228626=CARTESIAN_POINT('Ctrl Pts',(-6.81145274279046,-4.0234591650426,
134.526180347718));
#228627=CARTESIAN_POINT('Ctrl Pts',(-6.78278890587306,-4.07179208252226,
134.528462856215));
#228628=CARTESIAN_POINT('Ctrl Pts',(-6.7608846584911,-4.10805972308446,
134.530191716958));
#228629=CARTESIAN_POINT('Ctrl Pts',(-6.53522830863079,-4.47499346788989,
134.547839724681));
#228630=CARTESIAN_POINT('Ctrl Pts',(-6.30768135718817,-4.79039886381559,
134.564282588085));
#228631=CARTESIAN_POINT('Ctrl Pts',(-5.87855850299361,-5.3013422968962,
134.592418756284));
#228632=CARTESIAN_POINT('Ctrl Pts',(-5.68805156497539,-5.50524793590822,
134.604130439029));
#228633=CARTESIAN_POINT('Ctrl Pts',(-5.38595783210295,-5.79612992460482,
134.621512368895));
#228634=CARTESIAN_POINT('Ctrl Pts',(-5.28216258152839,-5.89087627759218,
134.627295686004));
#228635=CARTESIAN_POINT('Ctrl Pts',(-5.12911411459645,-6.02328284519411,
134.635561606678));
#228636=CARTESIAN_POINT('Ctrl Pts',(-5.08185713907819,-6.06320673731213,
134.638079570315));
#228637=CARTESIAN_POINT('Ctrl Pts',(-4.99669224683271,-6.13346099381015,
134.642557827776));
#228638=CARTESIAN_POINT('Ctrl Pts',(-4.9589643454751,-6.16400436683672,
134.644521355583));
#228639=CARTESIAN_POINT('Ctrl Pts',(-4.90164342481219,-6.2095427538191,
134.647474763863));
#228640=CARTESIAN_POINT('Ctrl Pts',(-4.88225758519829,-6.2247964105413,
134.648468533251));
#228641=CARTESIAN_POINT('Ctrl Pts',(-4.84740815567947,-6.25195457368229,
134.650246073611));
#228642=CARTESIAN_POINT('Ctrl Pts',(-4.83197127673987,-6.26389299098627,
134.651030341599));
#228643=CARTESIAN_POINT('Ctrl Pts',(-4.79870436322047,-6.28942446540238,
134.652713869104));
#228644=CARTESIAN_POINT('Ctrl Pts',(-4.78086038859333,-6.30299909727791,
134.653612855211));
#228645=CARTESIAN_POINT('Ctrl Pts',(-4.73299708855017,-6.33909044755376,
134.656013610461));
#228646=CARTESIAN_POINT('Ctrl Pts',(-4.70287480087382,-6.36146978044476,
134.657513413464));
#228647=CARTESIAN_POINT('Ctrl Pts',(-4.56562549428634,-6.46193141879186,
134.664298402505));
#228648=CARTESIAN_POINT('Ctrl Pts',(-4.45670463711384,-6.5375284517388,
134.669549160093));
#228649=CARTESIAN_POINT('Ctrl Pts',(-3.73793401218352,-7.01007960313806,
134.703446782646));
#228650=CARTESIAN_POINT('Ctrl Pts',(-3.07765217161356,-7.3240368551536,
134.731236723278));
#228651=CARTESIAN_POINT('Ctrl Pts',(-2.24389990383895,-7.58751308993906,
134.763969942717));
#228652=CARTESIAN_POINT('Ctrl Pts',(-2.10281662481511,-7.62781776620551,
134.769447627685));
#228653=CARTESIAN_POINT('Ctrl Pts',(-1.6643911332303,-7.73997834690071,
134.786388741539));
#228654=CARTESIAN_POINT('Ctrl Pts',(-1.36395009197624,-7.79853131933149,
134.797875582633));
#228655=CARTESIAN_POINT('Ctrl Pts',(-0.953415629191189,-7.85408690543955,
134.813984170946));
#228656=CARTESIAN_POINT('Ctrl Pts',(-0.845659419824983,-7.86641859941681,
134.818251591967));
#228657=CARTESIAN_POINT('Ctrl Pts',(-0.721552434783314,-7.87804199477941,
134.823237870058));
#228658=CARTESIAN_POINT('Ctrl Pts',(-0.705413942137415,-7.87950345857654,
134.823887656261));
#228659=CARTESIAN_POINT('Ctrl Pts',(-0.680958359230041,-7.88164236335777,
134.824874533965));
#228660=CARTESIAN_POINT('Ctrl Pts',(-0.672644452873165,-7.88235625116694,
134.825210420756));
#228661=CARTESIAN_POINT('Ctrl Pts',(-0.657619025430322,-7.88362249013696,
134.825818178533));
#228662=CARTESIAN_POINT('Ctrl Pts',(-0.650907892432978,-7.88417942875896,
134.826089894606));
#228663=CARTESIAN_POINT('Ctrl Pts',(-0.637529901924567,-7.88527243401025,
134.826632063879));
#228664=CARTESIAN_POINT('Ctrl Pts',(-0.630863059777419,-7.88580861636203,
134.826902512852));
#228665=CARTESIAN_POINT('Ctrl Pts',(-0.612202229786365,-7.88728560221123,
134.827660262755));
#228666=CARTESIAN_POINT('Ctrl Pts',(-0.600206791140009,-7.88820749898139,
134.828148221189));
#228667=CARTESIAN_POINT('Ctrl Pts',(-0.551640206178058,-7.89182861055798,
134.830127486014));
#228668=CARTESIAN_POINT('Ctrl Pts',(-0.515052943072718,-7.89430086481496,
134.831626903635));
#228669=CARTESIAN_POINT('Ctrl Pts',(0.0260200785681229,-7.92708448936865,
134.853938646844));
#228670=CARTESIAN_POINT('Ctrl Pts',(0.532149369880393,-7.90923143889126,
134.87696000699));
#228671=CARTESIAN_POINT('Ctrl Pts',(1.38991095178326,-7.79625953824765,
134.916625184714));
#228672=CARTESIAN_POINT('Ctrl Pts',(1.74321151562132,-7.72494337933138,
134.933135060912));
#228673=CARTESIAN_POINT('Ctrl Pts',(2.44472697546279,-7.53274022151604,
134.965431384782));
#228674=CARTESIAN_POINT('Ctrl Pts',(2.79184994556288,-7.4111054916239,134.981153613398));
#228675=CARTESIAN_POINT('Ctrl Pts',(3.15554056877153,-7.2544676878701,134.997237081378));
#228676=CARTESIAN_POINT('Ctrl Pts',(3.18172666356277,-7.24302099789654,
134.998393043265));
#228677=CARTESIAN_POINT('Ctrl Pts',(3.2178601992871,-7.22699222719772,134.999985329666));
#228678=CARTESIAN_POINT('Ctrl Pts',(3.2278608576596,-7.22253107981955,135.000425728474));
#228679=CARTESIAN_POINT('Ctrl Pts',(3.2447306417561,-7.21496367939714,135.001168125615));
#228680=CARTESIAN_POINT('Ctrl Pts',(3.25160463477087,-7.2118683523835,135.001470493216));
#228681=CARTESIAN_POINT('Ctrl Pts',(3.26519969990462,-7.2057231693844,135.002068227434));
#228682=CARTESIAN_POINT('Ctrl Pts',(3.27192094805435,-7.20267372467324,
135.00236360755));
#228683=CARTESIAN_POINT('Ctrl Pts',(3.28672622808175,-7.19593153727496,
135.00301396745));
#228684=CARTESIAN_POINT('Ctrl Pts',(3.29480833022685,-7.19223456620105,
135.003368803039));
#228685=CARTESIAN_POINT('Ctrl Pts',(3.32301348611423,-7.17927524880641,
135.004606456555));
#228686=CARTESIAN_POINT('Ctrl Pts',(3.34310393581234,-7.1699419670949,135.005486854537));
#228687=CARTESIAN_POINT('Ctrl Pts',(3.54418053598472,-7.07550031135375,
135.014286883686));
#228688=CARTESIAN_POINT('Ctrl Pts',(3.7219230775093,-6.9836391533939,135.021969477154));
#228689=CARTESIAN_POINT('Ctrl Pts',(4.23037865769221,-6.6959260598306,135.043788102178));
#228690=CARTESIAN_POINT('Ctrl Pts',(4.55054102467892,-6.48260231058685,
135.057298321681));
#228691=CARTESIAN_POINT('Ctrl Pts',(5.13046800663816,-6.03198547380571,
135.082515338386));
#228692=CARTESIAN_POINT('Ctrl Pts',(5.39241210110661,-5.79900305097784,
135.094256470895));
#228693=CARTESIAN_POINT('Ctrl Pts',(5.85705839497631,-5.32693689978065,
135.117179368428));
#228694=CARTESIAN_POINT('Ctrl Pts',(6.06268411110129,-5.09168185821444,
135.128270681824));
#228695=CARTESIAN_POINT('Ctrl Pts',(6.31233972803033,-4.76942417912666,
135.143879284295));
#228696=CARTESIAN_POINT('Ctrl Pts',(6.36944829871924,-4.69288470917488,
135.147615314876));
#228697=CARTESIAN_POINT('Ctrl Pts',(6.43120643581712,-4.60690919794417,
135.151864360133));
#228698=CARTESIAN_POINT('Ctrl Pts',(6.43724092891516,-4.59847342053661,
135.152281820214));
#228699=CARTESIAN_POINT('Ctrl Pts',(6.4461833313349,-4.5859205036222,135.152903877567));
#228700=CARTESIAN_POINT('Ctrl Pts',(6.44910394347002,-4.58181238515924,
135.153107589957));
#228701=CARTESIAN_POINT('Ctrl Pts',(6.45408247280646,-4.57479541954229,
135.153455781213));
#228702=CARTESIAN_POINT('Ctrl Pts',(6.45614235861604,-4.57188796250278,
135.15360012208));
#228703=CARTESIAN_POINT('Ctrl Pts',(6.46034618754733,-4.56594589788487,
135.153895258978));
#228704=CARTESIAN_POINT('Ctrl Pts',(6.4624899583663,-4.56291116977931,135.154046067096));
#228705=CARTESIAN_POINT('Ctrl Pts',(6.46759000682828,-4.55568072270925,
135.154405561177));
#228706=CARTESIAN_POINT('Ctrl Pts',(6.4705443373088,-4.55148363968955,135.154614384883));
#228707=CARTESIAN_POINT('Ctrl Pts',(6.48109655754965,-4.53646154186808,
135.15536233719));
#228708=CARTESIAN_POINT('Ctrl Pts',(6.48867123166355,-4.52562057065816,
135.155903118517));
#228709=CARTESIAN_POINT('Ctrl Pts',(6.60836805040142,-4.35339068464051,
135.164510149394));
#228710=CARTESIAN_POINT('Ctrl Pts',(6.71445809463561,-4.18790880472618,
135.172994701151));
#228711=CARTESIAN_POINT('Ctrl Pts',(6.97020831420628,-3.75424437952543,
135.195378908409));
#228712=CARTESIAN_POINT('Ctrl Pts',(7.11061834884796,-3.48098363525993,
135.209614305358));
#228713=CARTESIAN_POINT('Ctrl Pts',(7.34807697728012,-2.9441652071837,135.236909989157));
#228714=CARTESIAN_POINT('Ctrl Pts',(7.44768783174739,-2.68221898989426,
135.249945455162));
#228715=CARTESIAN_POINT('Ctrl Pts',(7.62617617529547,-2.12557732816804,
135.276562343962));
#228716=CARTESIAN_POINT('Ctrl Pts',(7.70233927235807,-1.83047479559133,
135.290066990104));
#228717=CARTESIAN_POINT('Ctrl Pts',(7.79133006981822,-1.37954597757157,
135.30960242964));
#228718=CARTESIAN_POINT('Ctrl Pts',(7.81687702637453,-1.2265434328895,135.316047255831));
#228719=CARTESIAN_POINT('Ctrl Pts',(7.84066047342695,-1.05279410472832,
135.323161311835));
#228720=CARTESIAN_POINT('Ctrl Pts',(7.84333296366554,-1.03269555833407,
135.323981172133));
#228721=CARTESIAN_POINT('Ctrl Pts',(7.84799005513257,-0.996610549900073,
135.32544769685));
#228722=CARTESIAN_POINT('Ctrl Pts',(7.85000314512618,-0.980627920997422,
135.326095326149));
#228723=CARTESIAN_POINT('Ctrl Pts',(7.8529721526951,-0.956460801343032,
135.327071717635));
#228724=CARTESIAN_POINT('Ctrl Pts',(7.85396411744352,-0.948280832873142,
135.327401703516));
#228725=CARTESIAN_POINT('Ctrl Pts',(7.85565532261476,-0.934150069707103,
135.327970891243));
#228726=CARTESIAN_POINT('Ctrl Pts',(7.85636058485882,-0.928200011500118,
135.328210297356));
#228727=CARTESIAN_POINT('Ctrl Pts',(7.85780563427802,-0.915888979619091,
135.32870510166));
#228728=CARTESIAN_POINT('Ctrl Pts',(7.8585444591157,-0.909527895918776,
135.328960467034));
#228729=CARTESIAN_POINT('Ctrl Pts',(7.86052777928438,-0.892269206758298,
135.32965250777));
#228730=CARTESIAN_POINT('Ctrl Pts',(7.86175733811396,-0.881369879325183,
135.330088675999));
#228731=CARTESIAN_POINT('Ctrl Pts',(7.86626409963879,-0.840660163769034,
135.331714547681));
#228732=CARTESIAN_POINT('Ctrl Pts',(7.86939446933841,-0.81083358897632,
135.332899268815));
#228733=CARTESIAN_POINT('Ctrl Pts',(7.91639991495052,-0.337019964131563,
135.351617935601));
#228734=CARTESIAN_POINT('Ctrl Pts',(7.9228120426035,0.1099035309372,135.367791207442));
#228735=CARTESIAN_POINT('Ctrl Pts',(7.85818389820049,1.02881400171604,135.399695337205));
#228736=CARTESIAN_POINT('Ctrl Pts',(7.78226300692866,1.49862351932244,135.4152691391));
#228737=CARTESIAN_POINT('Ctrl Pts',(7.61696664535482,2.14542625895294,135.438402298407));
#228738=CARTESIAN_POINT('Ctrl Pts',(7.56246620561757,2.33026464255066,135.445225558587));
#228739=CARTESIAN_POINT('Ctrl Pts',(7.45528153936251,2.65021975220097,135.457699449453));
#228740=CARTESIAN_POINT('Ctrl Pts',(7.40552796349576,2.78622301804474,135.463218513244));
#228741=CARTESIAN_POINT('Ctrl Pts',(7.34365033451669,2.9419791381574,135.469877372092));
#228742=CARTESIAN_POINT('Ctrl Pts',(7.33513566111852,2.96314466343925,135.470789573347));
#228743=CARTESIAN_POINT('Ctrl Pts',(7.32404282390114,2.99037809851655,135.471973138509));
#228744=CARTESIAN_POINT('Ctrl Pts',(7.32154837806681,2.99648023619336,135.472238976491));
#228745=CARTESIAN_POINT('Ctrl Pts',(7.31749875947206,3.00635153137009,135.47267006261));
#228746=CARTESIAN_POINT('Ctrl Pts',(7.31594829686062,3.01012261254933,135.472834995253));
#228747=CARTESIAN_POINT('Ctrl Pts',(7.31296759263189,3.01735646311849,135.473151847765));
#228748=CARTESIAN_POINT('Ctrl Pts',(7.31153780473852,3.02081941965885,135.473303737552));
#228749=CARTESIAN_POINT('Ctrl Pts',(7.30827250898547,3.0287120902976,135.473650391464));
#228750=CARTESIAN_POINT('Ctrl Pts',(7.30643543424889,3.03314115010401,135.473845258723));
#228751=CARTESIAN_POINT('Ctrl Pts',(7.30070459878669,3.04692237936565,135.474452645163));
#228752=CARTESIAN_POINT('Ctrl Pts',(7.29679691425301,3.05626870789418,135.474866073205));
#228753=CARTESIAN_POINT('Ctrl Pts',(7.26685467473443,3.12749925590691,135.478028227449));
#228754=CARTESIAN_POINT('Ctrl Pts',(7.24005197045764,3.18905556512344,135.480826159479));
#228755=CARTESIAN_POINT('Ctrl Pts',(7.05303728994141,3.60404918025981,135.500095106783));
#228756=CARTESIAN_POINT('Ctrl Pts',(6.86780251044484,3.94559768628711,135.517947337373));
#228757=CARTESIAN_POINT('Ctrl Pts',(6.47681462644036,4.55496560805641,135.551815270665));
#228758=CARTESIAN_POINT('Ctrl Pts',(6.27750725066601,4.8259455938197,135.567722543651));
#228759=CARTESIAN_POINT('Ctrl Pts',(5.86965037000293,5.31228119662681,135.597122305045));
#228760=CARTESIAN_POINT('Ctrl Pts',(5.66491302108104,5.53009131863548,135.610665465629));
#228761=CARTESIAN_POINT('Ctrl Pts',(5.31621938830087,5.86130833265701,135.6316712657));
#228762=CARTESIAN_POINT('Ctrl Pts',(5.17980287188342,5.98220463318566,135.63944227536));
#228763=CARTESIAN_POINT('Ctrl Pts',(4.9672225430096,6.1578705913434,135.65089461044));
#228764=CARTESIAN_POINT('Ctrl Pts',(4.89406648975625,6.21617117126574,135.654724984464));
#228765=CARTESIAN_POINT('Ctrl Pts',(4.80723660688551,6.28288563550633,135.659146050707));
#228766=CARTESIAN_POINT('Ctrl Pts',(4.79455186031634,6.29257087097112,135.659788844367));
#228767=CARTESIAN_POINT('Ctrl Pts',(4.77513040741212,6.30730699132631,135.66076836519));
#228768=CARTESIAN_POINT('Ctrl Pts',(4.76841483901869,6.3123855882095,135.661106219152));
#228769=CARTESIAN_POINT('Ctrl Pts',(4.75671558517504,6.32120373525802,135.661693332175));
#228770=CARTESIAN_POINT('Ctrl Pts',(4.75173557236388,6.32494813191816,135.661942787487));
#228771=CARTESIAN_POINT('Ctrl Pts',(4.74133999860546,6.33274520013675,135.662462557511));
#228772=CARTESIAN_POINT('Ctrl Pts',(4.73592365241508,6.33679681787336,135.662732829565));
#228773=CARTESIAN_POINT('Ctrl Pts',(4.72264983563816,6.34669957578501,135.663393864796));
#228774=CARTESIAN_POINT('Ctrl Pts',(4.71478666975881,6.35254308406698,135.663784320629));
#228775=CARTESIAN_POINT('Ctrl Pts',(4.6846008558908,6.37488873944882,135.665278929766));
#228776=CARTESIAN_POINT('Ctrl Pts',(4.66220213360857,6.39128804743691,135.66637896227));
#228777=CARTESIAN_POINT('Ctrl Pts',(4.29282268592522,6.65875550520183,135.684373993808));
#228778=CARTESIAN_POINT('Ctrl Pts',(3.92608512076348,6.88137029383959,135.70008173474));
#228779=CARTESIAN_POINT('Ctrl Pts',(3.05739626052743,7.31651233308555,135.734348940853));
#228780=CARTESIAN_POINT('Ctrl Pts',(2.54795303195255,7.50912174039579,135.75242965059));
#228781=CARTESIAN_POINT('Ctrl Pts',(1.92611649079876,7.67359124157175,135.775607093459));
#228782=CARTESIAN_POINT('Ctrl Pts',(1.82893614968746,7.69733193613248,135.77926324371));
#228783=CARTESIAN_POINT('Ctrl Pts',(1.58470292792323,7.7521106762175,135.788590460571));
#228784=CARTESIAN_POINT('Ctrl Pts',(1.43718633442356,7.78080959042918,135.794358266909));
#228785=CARTESIAN_POINT('Ctrl Pts',(1.26010355083917,7.81005206466047,135.801490118031));
#228786=CARTESIAN_POINT('Ctrl Pts',(1.23125819146574,7.81465146032297,135.802657684146));
#228787=CARTESIAN_POINT('Ctrl Pts',(1.19276967484345,7.82057006926553,135.804222868699));
#228788=CARTESIAN_POINT('Ctrl Pts',(1.18314836728234,7.8220314270274,135.804614738344));
#228789=CARTESIAN_POINT('Ctrl Pts',(1.16729194444085,7.82440989686345,135.805261537706));
#228790=CARTESIAN_POINT('Ctrl Pts',(1.16105836948133,7.82533732052821,135.805516060217));
#228791=CARTESIAN_POINT('Ctrl Pts',(1.1489379974558,7.82712577347588,135.806011422399));
#228792=CARTESIAN_POINT('Ctrl Pts',(1.14305132265721,7.82798761300329,135.806252230412));
#228793=CARTESIAN_POINT('Ctrl Pts',(1.12940061227412,7.82997042101067,135.806811143335));
#228794=CARTESIAN_POINT('Ctrl Pts',(1.12163587761646,7.83108648237224,135.807129435833));
#228795=CARTESIAN_POINT('Ctrl Pts',(1.10067208771137,7.83406788648908,135.807989775922));
#228796=CARTESIAN_POINT('Ctrl Pts',(1.08746998853076,7.83591141579306,135.80853264134));
#228797=CARTESIAN_POINT('Ctrl Pts',(0.99057835584056,7.84919169481745,135.8125243142));
#228798=CARTESIAN_POINT('Ctrl Pts',(0.906716750533531,7.85932057302182,
135.816020312002));
#228799=CARTESIAN_POINT('Ctrl Pts',(0.12530905933518,7.94102673852782,135.848899516));
#228800=CARTESIAN_POINT('Ctrl Pts',(-0.578699863589856,7.92090747917323,
135.880462514738));
#228801=CARTESIAN_POINT('Ctrl Pts',(-1.6190286759695,7.75158783938078,135.925720603467));
#228802=CARTESIAN_POINT('Ctrl Pts',(-1.96305030272363,7.67168982855214,
135.94051103658));
#228803=CARTESIAN_POINT('Ctrl Pts',(-2.364542964997,7.54965715686852,135.957607531542));
#228804=CARTESIAN_POINT('Ctrl Pts',(-2.42823179576967,7.52941412714909,
135.960315343433));
#228805=CARTESIAN_POINT('Ctrl Pts',(-2.51240645063944,7.5014807060306,135.963890150371));
#228806=CARTESIAN_POINT('Ctrl Pts',(-2.53312739965129,7.49450895915408,
135.964769801805));
#228807=CARTESIAN_POINT('Ctrl Pts',(-2.56692476538192,7.48298135670251,
135.966203997449));
#228808=CARTESIAN_POINT('Ctrl Pts',(-2.58001855323884,7.47847691727818,
135.966759491648));
#228809=CARTESIAN_POINT('Ctrl Pts',(-2.6052647283038,7.46971769724389,135.967830264257));
#228810=CARTESIAN_POINT('Ctrl Pts',(-2.61741868436853,7.46546758166851,
135.968345628704));
#228811=CARTESIAN_POINT('Ctrl Pts',(-2.64533082442786,7.45563044698993,
135.969528900518));
#228812=CARTESIAN_POINT('Ctrl Pts',(-2.6610817957033,7.45002310143388,135.970196416241));
#228813=CARTESIAN_POINT('Ctrl Pts',(-2.71109014358489,7.43204130233371,
135.972315067849));
#228814=CARTESIAN_POINT('Ctrl Pts',(-2.74528002055947,7.41948012477288,
135.973762552049));
#228815=CARTESIAN_POINT('Ctrl Pts',(-3.07908234330066,7.29421971115853,
135.987885133593));
#228816=CARTESIAN_POINT('Ctrl Pts',(-3.3716886044844,7.16366679148435,136.000170418465));
#228817=CARTESIAN_POINT('Ctrl Pts',(-4.05049948940648,6.80996819382163,
136.02881242978));
#228818=CARTESIAN_POINT('Ctrl Pts',(-4.42732071333323,6.57122850769228,
136.0448014499));
#228819=CARTESIAN_POINT('Ctrl Pts',(-5.07278384057463,6.08144523990192,
136.074429077218));
#228820=CARTESIAN_POINT('Ctrl Pts',(-5.34787889823811,5.84099854693965,
136.087956554177));
#228821=CARTESIAN_POINT('Ctrl Pts',(-5.61693445560959,5.57083806738167,
136.103193525049));
#228822=CARTESIAN_POINT('Ctrl Pts',(-5.62846012187602,5.55919293624044,
136.103850414269));
#228823=CARTESIAN_POINT('Ctrl Pts',(-5.64495206860732,5.542426186801,136.104796502856));
#228824=CARTESIAN_POINT('Ctrl Pts',(-5.64994777681369,5.5373334748598,136.105083905422));
#228825=CARTESIAN_POINT('Ctrl Pts',(-5.65859556898588,5.5284938784054,136.10558284125));
#228826=CARTESIAN_POINT('Ctrl Pts',(-5.6622508426639,5.52475010941454,136.105794177035));
#228827=CARTESIAN_POINT('Ctrl Pts',(-5.66926371262448,5.51755318547138,
136.106200497935));
#228828=CARTESIAN_POINT('Ctrl Pts',(-5.67262187624312,5.51410058366853,
136.106395447493));
#228829=CARTESIAN_POINT('Ctrl Pts',(-5.68051234425018,5.50597338356774,
136.106854408435));
#228830=CARTESIAN_POINT('Ctrl Pts',(-5.68504202946672,5.50129625783993,
136.107118584469));
#228831=CARTESIAN_POINT('Ctrl Pts',(-5.70061727081034,5.48517426535884,
136.10802938381));
#228832=CARTESIAN_POINT('Ctrl Pts',(-5.71163402892843,5.47370173679395,
136.108677840654));
#228833=CARTESIAN_POINT('Ctrl Pts',(-5.87354533996715,5.30407101586759,
136.118271932449));
#228834=CARTESIAN_POINT('Ctrl Pts',(-6.01783649188541,5.13977862894329,
136.127670612993));
#228835=CARTESIAN_POINT('Ctrl Pts',(-6.3498201743387,4.72861047932357,136.151061288945));
#228836=CARTESIAN_POINT('Ctrl Pts',(-6.5301708020188,4.47625162722608,136.16530028286));
#228837=CARTESIAN_POINT('Ctrl Pts',(-6.83991037814008,3.98413143818814,
136.192105527461));
#228838=CARTESIAN_POINT('Ctrl Pts',(-6.97264574394831,3.74698473587029,
136.204643819333));
#228839=CARTESIAN_POINT('Ctrl Pts',(-7.31175402719853,3.0604472068842,136.239381899073));
#228840=CARTESIAN_POINT('Ctrl Pts',(-7.48861622076895,2.59784885706755,
136.260936847229));
#228841=CARTESIAN_POINT('Ctrl Pts',(-7.62973372409618,2.0909576440689,136.282357759272));
#228842=CARTESIAN_POINT('Ctrl Pts',(-7.6381112372613,2.06014497719628,136.283651903632));
#228843=CARTESIAN_POINT('Ctrl Pts',(-7.64940708068612,2.01758242461873,
136.285428677968));
#228844=CARTESIAN_POINT('Ctrl Pts',(-7.65248528253231,2.00587550172729,
136.285916252954));
#228845=CARTESIAN_POINT('Ctrl Pts',(-7.65734903800562,1.98720366517646,
136.286692113057));
#228846=CARTESIAN_POINT('Ctrl Pts',(-7.65915198134217,1.98024332438444,
136.28698093557));
#228847=CARTESIAN_POINT('Ctrl Pts',(-7.66264362922107,1.96668756099512,
136.287542668744));
#228848=CARTESIAN_POINT('Ctrl Pts',(-7.66433331369956,1.96009239778099,
136.28781560951));
#228849=CARTESIAN_POINT('Ctrl Pts',(-7.66835822379588,1.94429762057987,
136.288468431015));
#228850=CARTESIAN_POINT('Ctrl Pts',(-7.6706854134382,1.93509596006992,136.288848063341));
#228851=CARTESIAN_POINT('Ctrl Pts',(-7.67762677053578,1.90744069295049,
136.289986984329));
#228852=CARTESIAN_POINT('Ctrl Pts',(-7.6821909615888,1.88897455267583,136.290744730917));
#228853=CARTESIAN_POINT('Ctrl Pts',(-7.72203369099223,1.72524295548827,
136.29743932926));
#228854=CARTESIAN_POINT('Ctrl Pts',(-7.75325577563833,1.5790171933201,136.303250033498));
#228855=CARTESIAN_POINT('Ctrl Pts',(-7.82274384609175,1.20147310293162,
136.317869998403));
#228856=CARTESIAN_POINT('Ctrl Pts',(-7.85490690069484,0.969177476494734,
136.326498305678));
#228857=CARTESIAN_POINT('Ctrl Pts',(-7.91489028185631,0.327046568713605,
136.34966155197));
#228858=CARTESIAN_POINT('Ctrl Pts',(-7.92119887124829,-0.0840536765173626,
136.363705962504));
#228859=CARTESIAN_POINT('Ctrl Pts',(-7.86376164364314,-1.00247119054195,
136.395516433555));
#228860=CARTESIAN_POINT('Ctrl Pts',(-7.78286352958253,-1.50689096754052,
136.413322594698));
#228861=CARTESIAN_POINT('Ctrl Pts',(-7.64576571696238,-2.03156382264371,
136.434783901456));
#228862=CARTESIAN_POINT('Ctrl Pts',(-7.63732431421645,-2.06307107042614,
136.436083210584));
#228863=CARTESIAN_POINT('Ctrl Pts',(-7.62584104193559,-2.10489549858869,
136.437821233071));
#228864=CARTESIAN_POINT('Ctrl Pts',(-7.62297256340687,-2.11526025655475,
136.438253027805));
#228865=CARTESIAN_POINT('Ctrl Pts',(-7.61847339832232,-2.13138920986506,
136.438926616887));
#228866=CARTESIAN_POINT('Ctrl Pts',(-7.61685727801344,-2.13715747922644,
136.439167846251));
#228867=CARTESIAN_POINT('Ctrl Pts',(-7.61359892450181,-2.1487365775127,
136.439652742026));
#228868=CARTESIAN_POINT('Ctrl Pts',(-7.61195658692626,-2.15454737270082,
136.439896412298));
#228869=CARTESIAN_POINT('Ctrl Pts',(-7.60826150100246,-2.16756408705518,
136.440442993725));
#228870=CARTESIAN_POINT('Ctrl Pts',(-7.60620516644946,-2.17476897728105,
136.440746039376));
#228871=CARTESIAN_POINT('Ctrl Pts',(-7.60011720058397,-2.19598545446804,
136.441639902043));
#228872=CARTESIAN_POINT('Ctrl Pts',(-7.59605707725077,-2.20998879062601,
136.442231766446));
#228873=CARTESIAN_POINT('Ctrl Pts',(-7.5643613783558,-2.31818775854298,
136.44681918667));
#228874=CARTESIAN_POINT('Ctrl Pts',(-7.53501394362846,-2.41187096711469,
136.45087485795));
#228875=CARTESIAN_POINT('Ctrl Pts',(-7.42301395737386,-2.74737852250292,
136.465651543895));
#228876=CARTESIAN_POINT('Ctrl Pts',(-7.33040058904106,-2.98570689433657,
136.476619057148));
#228877=CARTESIAN_POINT('Ctrl Pts',(-6.99494608645096,-3.73874777956843,
136.512195213584));
#228878=CARTESIAN_POINT('Ctrl Pts',(-6.7080859060453,-4.2319208089412,136.536776651183));
#228879=CARTESIAN_POINT('Ctrl Pts',(-6.14303244215255,-4.99946877119786,
136.576556068512));
#228880=CARTESIAN_POINT('Ctrl Pts',(-5.89301322822294,-5.29187498704281,
136.592243489285));
#228881=CARTESIAN_POINT('Ctrl Pts',(-5.57018057078227,-5.61805937193414,
136.610856059387));
#228882=CARTESIAN_POINT('Ctrl Pts',(-5.51687581407221,-5.67041304011356,
136.6138786558));
#228883=CARTESIAN_POINT('Ctrl Pts',(-5.44086927406208,-5.74297701562394,
136.618118235123));
#228884=CARTESIAN_POINT('Ctrl Pts',(-5.41878064099899,-5.76382336918695,
136.619342177075));
#228885=CARTESIAN_POINT('Ctrl Pts',(-5.37838622168782,-5.80150853241021,
136.621565751023));
#228886=CARTESIAN_POINT('Ctrl Pts',(-5.3601200379922,-5.81838919148437,
136.622565851215));
#228887=CARTESIAN_POINT('Ctrl Pts',(-5.32315907846042,-5.8522248220921,
136.624578735194));
#228888=CARTESIAN_POINT('Ctrl Pts',(-5.30446216271045,-5.86917703869629,
136.625591477542));
#228889=CARTESIAN_POINT('Ctrl Pts',(-5.25841682209093,-5.91052591825176,
136.62807223936));
#228890=CARTESIAN_POINT('Ctrl Pts',(-5.23097933893577,-5.93482259837594,
136.629539049168));
#228891=CARTESIAN_POINT('Ctrl Pts',(-5.12931303552639,-6.02359826606543,
136.634932639878));
#228892=CARTESIAN_POINT('Ctrl Pts',(-5.05405244671255,-6.08688281599496,
136.638844652628));
#228893=CARTESIAN_POINT('Ctrl Pts',(-4.91460939214823,-6.19976694474039,
136.645952696338));
#228894=CARTESIAN_POINT('Ctrl Pts',(-4.85080651237334,-6.2498137546493,
136.649153601768));
#228895=CARTESIAN_POINT('Ctrl Pts',(-4.54906517694144,-6.47909420673662,
136.664064289952));
#228896=CARTESIAN_POINT('Ctrl Pts',(-4.30189310048057,-6.6457787902255,
136.675621276554));
#228897=CARTESIAN_POINT('Ctrl Pts',(-3.65918256189946,-7.02828810808652,
136.704537217785));
#228898=CARTESIAN_POINT('Ctrl Pts',(-3.25353448819647,-7.22502177655864,
136.721773360009));
#228899=CARTESIAN_POINT('Ctrl Pts',(-2.79295025801972,-7.4017042008739,
136.741427820764));
#228900=CARTESIAN_POINT('Ctrl Pts',(-2.75239274391208,-7.41688144414838,
136.743159540706));
#228901=CARTESIAN_POINT('Ctrl Pts',(-2.69674102015199,-7.43718783363369,
136.745538670695));
#228902=CARTESIAN_POINT('Ctrl Pts',(-2.68175267251557,-7.44260556548389,
136.746179716044));
#228903=CARTESIAN_POINT('Ctrl Pts',(-2.65679301006792,-7.45154237124322,
136.747247804158));
#228904=CARTESIAN_POINT('Ctrl Pts',(-2.64683080675357,-7.45508681964258,
136.747674264132));
#228905=CARTESIAN_POINT('Ctrl Pts',(-2.62742337876813,-7.46194797631548,
136.748505380958));
#228906=CARTESIAN_POINT('Ctrl Pts',(-2.61797890400205,-7.46526675143261,
136.748909988256));
#228907=CARTESIAN_POINT('Ctrl Pts',(-2.59570038724173,-7.47304791400891,
136.749864802684));
#228908=CARTESIAN_POINT('Ctrl Pts',(-2.58286111204484,-7.47749517549158,
136.750415372867));
#228909=CARTESIAN_POINT('Ctrl Pts',(-2.53997095268429,-7.49222779974579,
136.752255708096));
#228910=CARTESIAN_POINT('Ctrl Pts',(-2.50986988989184,-7.50236515654474,
136.753549234786));
#228911=CARTESIAN_POINT('Ctrl Pts',(-2.43660169230001,-7.52654993232625,
136.756701780051));
#228912=CARTESIAN_POINT('Ctrl Pts',(-2.39337318469666,-7.54040757721394,
136.758565111757));
#228913=CARTESIAN_POINT('Ctrl Pts',(-1.7182118370628,-7.75045136583826,
136.787703291497));
#228914=CARTESIAN_POINT('Ctrl Pts',(-1.06422114946391,-7.86697108315226,
136.816167969104));
#228915=CARTESIAN_POINT('Ctrl Pts',(-0.208718193763188,-7.91064730273531,
136.85163425675));
#228916=CARTESIAN_POINT('Ctrl Pts',(-0.0137754869546448,-7.91338846755851,
136.859619190027));
#228917=CARTESIAN_POINT('Ctrl Pts',(0.21895698198812,-7.90806011575726,
136.869051175369));
#228918=CARTESIAN_POINT('Ctrl Pts',(0.256834453835736,-7.90692057872124,
136.870583124002));
#228919=CARTESIAN_POINT('Ctrl Pts',(0.318967926994052,-7.90460436044039,
136.873091311122));
#228920=CARTESIAN_POINT('Ctrl Pts',(0.343229203732085,-7.90358806824807,
136.874069484961));
#228921=CARTESIAN_POINT('Ctrl Pts',(0.386817111690746,-7.90156111427252,
136.875824828444));
#228922=CARTESIAN_POINT('Ctrl Pts',(0.406145422111844,-7.90059120694265,
136.876602481624));
#228923=CARTESIAN_POINT('Ctrl Pts',(0.447305124695851,-7.89837434416711,
136.878257024626));
#228924=CARTESIAN_POINT('Ctrl Pts',(0.469135308630685,-7.89710777570572,
136.879133674533));
#228925=CARTESIAN_POINT('Ctrl Pts',(0.528008561126827,-7.89344702028305,
136.881495644447));
#228926=CARTESIAN_POINT('Ctrl Pts',(0.565040561878516,-7.89088259219176,
136.882978952819));
#228927=CARTESIAN_POINT('Ctrl Pts',(0.75705964232581,-7.8762268025133,136.890659197131));
#228928=CARTESIAN_POINT('Ctrl Pts',(0.911685126250312,-7.85982946680961,
136.896805744961));
#228929=CARTESIAN_POINT('Ctrl Pts',(1.38630023125547,-7.79530360363674,
136.915634452173));
#228930=CARTESIAN_POINT('Ctrl Pts',(1.70390788228406,-7.73209504900646,
136.92822794354));
#228931=CARTESIAN_POINT('Ctrl Pts',(2.69532085798193,-7.47071785265343,
136.967639385243));
#228932=CARTESIAN_POINT('Ctrl Pts',(3.34704192321646,-7.20233557902392,
136.993278448167));
#228933=CARTESIAN_POINT('Ctrl Pts',(3.99569409638519,-6.82792655369442,
137.021745442572));
#228934=CARTESIAN_POINT('Ctrl Pts',(4.0363924810619,-6.80394650378785,137.023546675736));
#228935=CARTESIAN_POINT('Ctrl Pts',(4.16755765722972,-6.72507112128776,
137.029406375802));
#228936=CARTESIAN_POINT('Ctrl Pts',(4.25713721417319,-6.66872554701499,
137.033493142118));
#228937=CARTESIAN_POINT('Ctrl Pts',(4.41535617473172,-6.56471841439059,
137.040900350845));
#228938=CARTESIAN_POINT('Ctrl Pts',(4.48442213792002,-6.51773393193075,
137.044200475582));
#228939=CARTESIAN_POINT('Ctrl Pts',(4.56469019830904,-6.46124897223342,
137.048127319956));
#228940=CARTESIAN_POINT('Ctrl Pts',(4.57662712976933,-6.4527993150065,137.048713708165));
#228941=CARTESIAN_POINT('Ctrl Pts',(4.59573949504721,-6.43919075610921,
137.049656554245));
#228942=CARTESIAN_POINT('Ctrl Pts',(4.60292986082819,-6.43405282815602,
137.050012173495));
#228943=CARTESIAN_POINT('Ctrl Pts',(4.61567243837084,-6.42491523415001,
137.050644024843));
#228944=CARTESIAN_POINT('Ctrl Pts',(4.62122810470296,-6.42092038794469,
137.050920059408));
#228945=CARTESIAN_POINT('Ctrl Pts',(4.63229182212711,-6.41294313656981,
137.051470876406));
#228946=CARTESIAN_POINT('Ctrl Pts',(4.63779993799344,-6.40896083098058,
137.051745654589));
#228947=CARTESIAN_POINT('Ctrl Pts',(4.65224295404536,-6.39849032396414,
137.052467624567));
#228948=CARTESIAN_POINT('Ctrl Pts',(4.66116939749716,-6.39199051749304,
137.052915309406));
#228949=CARTESIAN_POINT('Ctrl Pts',(4.68029442962054,-6.37800322402905,
137.053877703446));
#228950=CARTESIAN_POINT('Ctrl Pts',(4.6904887150439,-6.37050992350434,137.054392666714));
#228951=CARTESIAN_POINT('Ctrl Pts',(4.71932449286379,-6.34920747252993,
137.055855017416));
#228952=CARTESIAN_POINT('Ctrl Pts',(4.73792319015151,-6.33534079808741,
137.056805006622));
#228953=CARTESIAN_POINT('Ctrl Pts',(4.90231168372407,-6.21164853215248,
137.06526422718));
#228954=CARTESIAN_POINT('Ctrl Pts',(5.04429738329768,-6.09690809464115,
137.073040935022));
#228955=CARTESIAN_POINT('Ctrl Pts',(5.43300599863429,-5.75991014362268,
137.095588621291));
#228956=CARTESIAN_POINT('Ctrl Pts',(5.66988261999473,-5.52689183402546,
137.110777865977));
#228957=CARTESIAN_POINT('Ctrl Pts',(6.05955294442313,-5.09207349950693,
137.137543211365));
#228958=CARTESIAN_POINT('Ctrl Pts',(6.21863871113789,-4.89652245716874,
137.149095208133));
#228959=CARTESIAN_POINT('Ctrl Pts',(6.64018019627438,-4.32460211367056,
137.181124636086));
#228960=CARTESIAN_POINT('Ctrl Pts',(6.87965411248884,-3.93250857936813,
137.201040943593));
#228961=CARTESIAN_POINT('Ctrl Pts',(7.09732896970311,-3.49467625493419,
137.220914748124));
#228962=CARTESIAN_POINT('Ctrl Pts',(7.11067312990908,-3.46744405826491,
137.222141913801));
#228963=CARTESIAN_POINT('Ctrl Pts',(7.12887059784851,-3.42976059533592,
137.223827814578));
#228964=CARTESIAN_POINT('Ctrl Pts',(7.13385806678806,-3.41937462506903,
137.224291191499));
#228965=CARTESIAN_POINT('Ctrl Pts',(7.14177492682433,-3.40279573687417,
137.225028843222));
#228966=CARTESIAN_POINT('Ctrl Pts',(7.14471898415316,-3.39660986427426,
137.225303625158));
#228967=CARTESIAN_POINT('Ctrl Pts',(7.15043705443133,-3.38455507706051,
137.22583823751));
#228968=CARTESIAN_POINT('Ctrl Pts',(7.15321188610707,-3.37868655719622,
137.22609809612));
#228969=CARTESIAN_POINT('Ctrl Pts',(7.15984091569622,-3.36462198348927,
137.226719916768));
#228970=CARTESIAN_POINT('Ctrl Pts',(7.16368827171385,-3.35642270524064,
137.227081642171));
#228971=CARTESIAN_POINT('Ctrl Pts',(7.17521486090875,-3.33174775709674,
137.228167883753));
#228972=CARTESIAN_POINT('Ctrl Pts',(7.18285142225183,-3.31525215762523,
137.228890926097));
#228973=CARTESIAN_POINT('Ctrl Pts',(7.25041497574915,-3.16798001657772,
137.235318552345));
#228974=CARTESIAN_POINT('Ctrl Pts',(7.30682307210091,-3.03561426708979,
137.240900778931));
#228975=CARTESIAN_POINT('Ctrl Pts',(7.44197216408833,-2.69284450122335,
137.254899267162));
#228976=CARTESIAN_POINT('Ctrl Pts',(7.51542027370736,-2.48048937822177,
137.263139143102));
#228977=CARTESIAN_POINT('Ctrl Pts',(7.66831896238124,-1.96888464999519,
137.282204346993));
#228978=CARTESIAN_POINT('Ctrl Pts',(7.73944191938007,-1.66753438224366,
137.292809423382));
#228979=CARTESIAN_POINT('Ctrl Pts',(7.84521605560998,-1.06269310231812,
137.313660076921));
#228980=CARTESIAN_POINT('Ctrl Pts',(7.88031673336665,-0.759824242257206,
137.32389377151));
#228981=CARTESIAN_POINT('Ctrl Pts',(7.91830544702248,-0.101421171746311,
137.346809635786));
#228982=CARTESIAN_POINT('Ctrl Pts',(7.91488398956741,0.253793123182802,
137.359594946649));
#228983=CARTESIAN_POINT('Ctrl Pts',(7.88583301257502,0.630959979855571,
137.37463518708));
#228984=CARTESIAN_POINT('Ctrl Pts',(7.88392473719205,0.654372611468432,
137.37557488224));
#228985=CARTESIAN_POINT('Ctrl Pts',(7.88129577818577,0.6849449822814,137.376810248428));
#228986=CARTESIAN_POINT('Ctrl Pts',(7.88066954363933,0.692112935365577,
137.377100487385));
#228987=CARTESIAN_POINT('Ctrl Pts',(7.87968992919449,0.703151996484756,
137.377548404027));
#228988=CARTESIAN_POINT('Ctrl Pts',(7.8793434722941,0.707023730801474,137.377705678623));
#228989=CARTESIAN_POINT('Ctrl Pts',(7.87864924257936,0.714718018030574,
137.378018583591));
#228990=CARTESIAN_POINT('Ctrl Pts',(7.87830154109193,0.718540576742255,
137.378174209754));
#228991=CARTESIAN_POINT('Ctrl Pts',(7.87752662362451,0.72699167812077,137.378518662073));
#228992=CARTESIAN_POINT('Ctrl Pts',(7.87709811029137,0.731620097203008,
137.378707564711));
#228993=CARTESIAN_POINT('Ctrl Pts',(7.87587255549259,0.744731553629492,
137.379243423262));
#228994=CARTESIAN_POINT('Ctrl Pts',(7.87506589031872,0.753213661141762,
137.379590951245));
#228995=CARTESIAN_POINT('Ctrl Pts',(7.8695838669992,0.809885728993842,137.381918808303));
#228996=CARTESIAN_POINT('Ctrl Pts',(7.86448006579414,0.858031531406276,
137.383925185326));
#228997=CARTESIAN_POINT('Ctrl Pts',(7.84787564778091,1.0020435773276,137.390005790461));
#228998=CARTESIAN_POINT('Ctrl Pts',(7.83506177681284,1.09774726148733,137.394151876249));
#228999=CARTESIAN_POINT('Ctrl Pts',(7.79131402430223,1.38448256494346,137.406835761854));
#229000=CARTESIAN_POINT('Ctrl Pts',(7.75512035563487,1.57463233182598,137.415597058033));
#229001=CARTESIAN_POINT('Ctrl Pts',(7.67063808499086,1.94413500329999,137.43304803864));
#229002=CARTESIAN_POINT('Ctrl Pts',(7.62293138154975,2.12350287717563,137.441720603128));
#229003=CARTESIAN_POINT('Ctrl Pts',(7.45696342516364,2.66943605686101,137.468434527694));
#229004=CARTESIAN_POINT('Ctrl Pts',(7.3182078153177,3.02920128498578,137.486457865711));
#229005=CARTESIAN_POINT('Ctrl Pts',(6.99222649849499,3.71966514697358,137.520767924053));
#229006=CARTESIAN_POINT('Ctrl Pts',(6.80629825478973,4.04987672366209,137.537034440507));
#229007=CARTESIAN_POINT('Ctrl Pts',(6.58441351938915,4.38519954921796,137.553302836553));
#229008=CARTESIAN_POINT('Ctrl Pts',(6.57131973557064,4.40479663860583,137.554252796586));
#229009=CARTESIAN_POINT('Ctrl Pts',(6.55320411359318,4.43164920662849,137.55555340553));
#229010=CARTESIAN_POINT('Ctrl Pts',(6.54825749620984,4.43895512582095,137.55590716099));
#229011=CARTESIAN_POINT('Ctrl Pts',(6.5397838802022,4.45142526710199,137.556510789117));
#229012=CARTESIAN_POINT('Ctrl Pts',(6.53626296687371,4.45659360234842,137.556760913652));
#229013=CARTESIAN_POINT('Ctrl Pts',(6.52941406527846,4.46662150342126,137.557246117771));
#229014=CARTESIAN_POINT('Ctrl Pts',(6.52608677144406,4.47148153775562,137.557481225956));
#229015=CARTESIAN_POINT('Ctrl Pts',(6.51813646202759,4.48306643473186,137.558041545496));
#229016=CARTESIAN_POINT('Ctrl Pts',(6.51350845792592,4.48978787526941,137.558366549107));
#229017=CARTESIAN_POINT('Ctrl Pts',(6.49967936195226,4.5098060550648,137.559334236502));
#229018=CARTESIAN_POINT('Ctrl Pts',(6.49044786692956,4.52308179823314,137.559975652733));
#229019=CARTESIAN_POINT('Ctrl Pts',(6.41326131149601,4.63336030866507,137.565301062576));
#229020=CARTESIAN_POINT('Ctrl Pts',(6.34317475645783,4.72885652544241,137.569894923436));
#229021=CARTESIAN_POINT('Ctrl Pts',(6.09084953000408,5.05695248063119,137.585647244255));
#229022=CARTESIAN_POINT('Ctrl Pts',(5.89774461613417,5.28089416286222,137.596331835361));
#229023=CARTESIAN_POINT('Ctrl Pts',(5.5234011833854,5.66880018543502,137.615183317774));
#229024=CARTESIAN_POINT('Ctrl Pts',(5.34624178723412,5.83617675071304,137.623455919542));
#229025=CARTESIAN_POINT('Ctrl Pts',(4.98453158520127,6.14759992167587,137.639572086774));
#229026=CARTESIAN_POINT('Ctrl Pts',(4.80075605714054,6.29216008422309,137.647412408225));
#229027=CARTESIAN_POINT('Ctrl Pts',(4.30277394768891,6.64934587014393,137.66843927089));
#229028=CARTESIAN_POINT('Ctrl Pts',(3.97923706212365,6.84786652533176,137.681882561439));
#229029=CARTESIAN_POINT('Ctrl Pts',(3.62159537579133,7.03338726050776,137.697879336629));
#229030=CARTESIAN_POINT('Ctrl Pts',(3.60038307126351,7.04426938324619,137.698832313249));
#229031=CARTESIAN_POINT('Ctrl Pts',(3.57260357140288,7.05836228434764,137.700085882373));
#229032=CARTESIAN_POINT('Ctrl Pts',(3.56608118831309,7.06165981715079,137.700380600865));
#229033=CARTESIAN_POINT('Ctrl Pts',(3.55600394518907,7.06673706503045,137.700836541252));
#229034=CARTESIAN_POINT('Ctrl Pts',(3.55245228240092,7.06852315449443,137.700997348227));
#229035=CARTESIAN_POINT('Ctrl Pts',(3.54537413565968,7.07207598910778,137.701318046062));
#229036=CARTESIAN_POINT('Ctrl Pts',(3.54184767332189,7.07384277577609,137.701477934189));
#229037=CARTESIAN_POINT('Ctrl Pts',(3.53402518050049,7.07775459313704,137.70183284497));
#229038=CARTESIAN_POINT('Ctrl Pts',(3.52972851852906,7.07989834972029,137.702027949012));
#229039=CARTESIAN_POINT('Ctrl Pts',(3.52085560428013,7.08431527554123,137.702431183201));
#229040=CARTESIAN_POINT('Ctrl Pts',(3.51627909715017,7.08658792509975,137.702639346111));
#229041=CARTESIAN_POINT('Ctrl Pts',(3.4920512833741,7.09858997758302,137.703742296214));
#229042=CARTESIAN_POINT('Ctrl Pts',(3.47236196283464,7.1082419919824,137.704641924229));
#229043=CARTESIAN_POINT('Ctrl Pts',(3.27506504298794,7.20394469581716,137.713687572718));
#229044=CARTESIAN_POINT('Ctrl Pts',(3.09434773587105,7.28339698755708,137.722222219025));
#229045=CARTESIAN_POINT('Ctrl Pts',(2.78805009204316,7.40460278664932,137.736873241804));
#229046=CARTESIAN_POINT('Ctrl Pts',(2.66404305751848,7.4501166653912,137.742854046942));
#229047=CARTESIAN_POINT('Ctrl Pts',(2.42521066295268,7.53104897139772,137.754396289446));
#229048=CARTESIAN_POINT('Ctrl Pts',(2.31060110278897,7.56699855355914,137.75994519524));
#229049=CARTESIAN_POINT('Ctrl Pts',(1.68119686727785,7.74879083909839,137.790338903395));
#229050=CARTESIAN_POINT('Ctrl Pts',(1.15338828676953,7.84474141608955,137.815420862829));
#229051=CARTESIAN_POINT('Ctrl Pts',(0.587116279381268,7.8892520506006,137.84051973687));
#229052=CARTESIAN_POINT('Ctrl Pts',(0.554300954743872,7.89162555658072,
137.841968314981));
#229053=CARTESIAN_POINT('Ctrl Pts',(0.224501951515393,7.913412391737,137.856466433581));
#229054=CARTESIAN_POINT('Ctrl Pts',(-0.0733546393494361,7.91625801729728,
137.869056190157));
#229055=CARTESIAN_POINT('Ctrl Pts',(-0.39500889416899,7.90116965032467,
137.882114690229));
#229056=CARTESIAN_POINT('Ctrl Pts',(-0.41932580395055,7.89991643964552,
137.883098666567));
#229057=CARTESIAN_POINT('Ctrl Pts',(-0.453222669692455,7.89801255967257,
137.884465844585));
#229058=CARTESIAN_POINT('Ctrl Pts',(-0.462807690714998,7.8974566933462,
137.884851945608));
#229059=CARTESIAN_POINT('Ctrl Pts',(-0.479352537662126,7.8964669803212,
137.885517549711));
#229060=CARTESIAN_POINT('Ctrl Pts',(-0.486312836084989,7.89604137859354,
137.88579730464));
#229061=CARTESIAN_POINT('Ctrl Pts',(-0.500711914334743,7.89514180611295,
137.886375511041));
#229062=CARTESIAN_POINT('Ctrl Pts',(-0.50815060715982,7.89466652371237,
137.886673922148));
#229063=CARTESIAN_POINT('Ctrl Pts',(-0.525521806858425,7.89353196733937,
137.887370100198));
#229064=CARTESIAN_POINT('Ctrl Pts',(-0.535453772929936,7.89286445765136,
137.887767615255));
#229065=CARTESIAN_POINT('Ctrl Pts',(-0.56732404589184,7.89066208060671,
137.889041516466));
#229066=CARTESIAN_POINT('Ctrl Pts',(-0.58925730682568,7.88905447309326,
137.889915682906));
#229067=CARTESIAN_POINT('Ctrl Pts',(-1.06335697122926,7.85231693977553,
137.908757453707));
#229068=CARTESIAN_POINT('Ctrl Pts',(-1.51170353755009,7.77845852054929,
137.925450237707));
#229069=CARTESIAN_POINT('Ctrl Pts',(-2.4575557918196,7.53772252052056,137.960068866455));
#229070=CARTESIAN_POINT('Ctrl Pts',(-2.94978943986607,7.3590436259296,137.977712341762));
#229071=CARTESIAN_POINT('Ctrl Pts',(-3.42078955582569,7.13317039013887,
137.996634350838));
#229072=CARTESIAN_POINT('',(3.42067962509738,7.13322310757512,138.));
#229073=CARTESIAN_POINT('Origin',(0.,0.,138.));
#229074=CARTESIAN_POINT('',(-7.91099871838666,-0.0025630630418797,136.642331508237));
#229075=CARTESIAN_POINT('Ctrl Pts',(3.42067962509738,7.13322310757512,138.));
#229076=CARTESIAN_POINT('Ctrl Pts',(3.61450323792865,7.04027655686782,137.991350898295));
#229077=CARTESIAN_POINT('Ctrl Pts',(3.80449053363425,6.9394483670193,137.982701796591));
#229078=CARTESIAN_POINT('Ctrl Pts',(3.99003223922227,6.83107339515299,137.974052694886));
#229079=CARTESIAN_POINT('Ctrl Pts',(4.17562869260824,6.72266644507969,137.96540104109));
#229080=CARTESIAN_POINT('Ctrl Pts',(4.35677673418512,6.60670838442162,137.956749387295));
#229081=CARTESIAN_POINT('Ctrl Pts',(4.53289396587659,6.48357874126008,137.948097733499));
#229082=CARTESIAN_POINT('Ctrl Pts',(4.71449430712678,6.35661566671367,137.939176725222));
#229083=CARTESIAN_POINT('Ctrl Pts',(4.89074533052145,6.22202742493026,137.930255716945));
#229084=CARTESIAN_POINT('Ctrl Pts',(5.06104230700313,6.08027727712515,137.921334708668));
#229085=CARTESIAN_POINT('Ctrl Pts',(5.22620278543872,5.94280259781207,137.912682775876));
#229086=CARTESIAN_POINT('Ctrl Pts',(5.38576295710407,5.79859189864489,137.904030843084));
#229087=CARTESIAN_POINT('Ctrl Pts',(5.53920484348363,5.64810859508982,137.895378910293));
#229088=CARTESIAN_POINT('Ctrl Pts',(5.69980480385011,5.49060523562916,137.886323364273));
#229089=CARTESIAN_POINT('Ctrl Pts',(5.85370181180418,5.32623024217355,137.877267818253));
#229090=CARTESIAN_POINT('Ctrl Pts',(6.00034404570054,5.1555593618177,137.868212272234));
#229091=CARTESIAN_POINT('Ctrl Pts',(6.1469862795968,4.98488848146197,137.859156726214));
#229092=CARTESIAN_POINT('Ctrl Pts',(6.28637353306249,4.80792192525416,137.850101180194));
#229093=CARTESIAN_POINT('Ctrl Pts',(6.41800015970126,4.62527782409605,137.841045634175));
#229094=CARTESIAN_POINT('Ctrl Pts',(6.53225023542455,4.46674529218672,137.833185546555));
#229095=CARTESIAN_POINT('Ctrl Pts',(6.64068733369427,4.30388758917187,137.825325458936));
#229096=CARTESIAN_POINT('Ctrl Pts',(6.74297429743848,4.13717519862092,137.817465371316));
#229097=CARTESIAN_POINT('Ctrl Pts',(6.84522917872496,3.97051509765826,137.809607749024));
#229098=CARTESIAN_POINT('Ctrl Pts',(6.94133758611483,3.80000301422222,137.801750126733));
#229099=CARTESIAN_POINT('Ctrl Pts',(7.03100584644683,3.62613813681035,137.793892504441));
#229100=CARTESIAN_POINT('Ctrl Pts',(7.12066144242633,3.45229781531256,137.786035991926));
#229101=CARTESIAN_POINT('Ctrl Pts',(7.203878544636,3.27510595323246,137.778179479411));
#229102=CARTESIAN_POINT('Ctrl Pts',(7.28040948782943,3.09508621681581,137.770322966896));
#229103=CARTESIAN_POINT('Ctrl Pts',(7.35696442839242,2.9150100326414,137.762463990859));
#229104=CARTESIAN_POINT('Ctrl Pts',(7.42682888092052,2.73210452182045,137.754605014822));
#229105=CARTESIAN_POINT('Ctrl Pts',(7.48980312788921,2.54691383942628,137.746746038785));
#229106=CARTESIAN_POINT('Ctrl Pts',(7.55278699150612,2.36169487700123,137.738885862622));
#229107=CARTESIAN_POINT('Ctrl Pts',(7.60887844677386,2.17419037968845,137.73102568646));
#229108=CARTESIAN_POINT('Ctrl Pts',(7.6579276241108,1.98495982424852,137.723165510297));
#229109=CARTESIAN_POINT('Ctrl Pts',(7.7070131150093,1.79558917195487,137.715299514853));
#229110=CARTESIAN_POINT('Ctrl Pts',(7.74904583020806,1.60449024757822,137.707433519408));
#229111=CARTESIAN_POINT('Ctrl Pts',(7.78392682092784,1.41223377896162,137.699567523964));
#229112=CARTESIAN_POINT('Ctrl Pts',(7.8097590720885,1.26985200361403,137.693742105426));
#229113=CARTESIAN_POINT('Ctrl Pts',(7.83166993231325,1.1268355922756,137.687916686889));
#229114=CARTESIAN_POINT('Ctrl Pts',(7.84963754731252,0.983418210031437,
137.682091268351));
#229115=CARTESIAN_POINT('Ctrl Pts',(7.87718026824534,0.763572396537256,
137.673161431135));
#229116=CARTESIAN_POINT('Ctrl Pts',(7.89547509537865,0.542630538372062,
137.664231593919));
#229117=CARTESIAN_POINT('Ctrl Pts',(7.90447130504336,0.321332207763367,
137.655301756703));
#229118=CARTESIAN_POINT('Ctrl Pts',(7.91346938005995,0.0999879912458073,
137.646370067898));
#229119=CARTESIAN_POINT('Ctrl Pts',(7.9131649801128,-0.121712667043669,
137.637438379092));
#229120=CARTESIAN_POINT('Ctrl Pts',(7.90355947844026,-0.343028527614233,
137.628506690287));
#229121=CARTESIAN_POINT('Ctrl Pts',(7.89396064943931,-0.564190646287026,
137.619581206074));
#229122=CARTESIAN_POINT('Ctrl Pts',(7.87507364340439,-0.784968323718609,
137.610655721861));
#229123=CARTESIAN_POINT('Ctrl Pts',(7.84695182636227,-1.00462332978574,
137.601730237649));
#229124=CARTESIAN_POINT('Ctrl Pts',(7.81885546307165,-1.22407952067923,
137.592812832112));
#229125=CARTESIAN_POINT('Ctrl Pts',(7.78154100710172,-1.44241489332641,
137.583895426576));
#229126=CARTESIAN_POINT('Ctrl Pts',(7.73511348190396,-1.65889735127513,
137.574978021039));
#229127=CARTESIAN_POINT('Ctrl Pts',(7.68879188541431,-1.87488588440226,
137.566080961391));
#229128=CARTESIAN_POINT('Ctrl Pts',(7.63339877760798,-2.08902977067117,
137.557183901744));
#229129=CARTESIAN_POINT('Ctrl Pts',(7.56908981737375,-2.30060868826689,
137.548286842096));
#229130=CARTESIAN_POINT('Ctrl Pts',(7.5084942750378,-2.49997032017428,137.539903528906));
#229131=CARTESIAN_POINT('Ctrl Pts',(7.43998324254046,-2.69705457975007,
137.531520215716));
#229132=CARTESIAN_POINT('Ctrl Pts',(7.3637285946372,-2.89126653640277,137.523136902526));
#229133=CARTESIAN_POINT('Ctrl Pts',(7.29141407464606,-3.07544343326152,
137.515186760653));
#229134=CARTESIAN_POINT('Ctrl Pts',(7.21216691845961,-3.25695364429777,
137.507236618781));
#229135=CARTESIAN_POINT('Ctrl Pts',(7.1262167607559,-3.4352519090631,137.499286476908));
#229136=CARTESIAN_POINT('Ctrl Pts',(7.04027424968884,-3.61353431135555,
137.491337042328));
#229137=CARTESIAN_POINT('Ctrl Pts',(6.94763007264582,-3.78860503235103,
137.483387607747));
#229138=CARTESIAN_POINT('Ctrl Pts',(6.84856099919256,-3.95994106526078,
137.475438173166));
#229139=CARTESIAN_POINT('Ctrl Pts',(6.74948496992316,-4.13128912797861,
137.467488180442));
#229140=CARTESIAN_POINT('Ctrl Pts',(6.64398331521634,-4.29890168764394,
137.459538187717));
#229141=CARTESIAN_POINT('Ctrl Pts',(6.53237769691227,-4.46228222156366,
137.451588194993));
#229142=CARTESIAN_POINT('Ctrl Pts',(6.4207063793305,-4.62575893328549,137.443633522317));
#229143=CARTESIAN_POINT('Ctrl Pts',(6.30292410901325,-4.78499836153753,
137.435678849642));
#229144=CARTESIAN_POINT('Ctrl Pts',(6.17939520875281,-4.93953397134212,
137.427724176967));
#229145=CARTESIAN_POINT('Ctrl Pts',(6.05582777813717,-5.09411778291913,
137.419767023121));
#229146=CARTESIAN_POINT('Ctrl Pts',(5.92651036112141,-5.2439945915914,137.411809869274));
#229147=CARTESIAN_POINT('Ctrl Pts',(5.79184650745455,-5.38873222883514,
137.403852715428));
#229148=CARTESIAN_POINT('Ctrl Pts',(5.65705792690499,-5.5336039233913,137.395888191593));
#229149=CARTESIAN_POINT('Ctrl Pts',(5.51691325199007,-5.67332669388599,
137.387923667759));
#229150=CARTESIAN_POINT('Ctrl Pts',(5.37185250905003,-5.80750562815163,
137.379959143924));
#229151=CARTESIAN_POINT('Ctrl Pts',(5.27607083134976,-5.89610219242892,
137.37470027485));
#229152=CARTESIAN_POINT('Ctrl Pts',(5.17814657378654,-5.98228256059462,
137.369441405775));
#229153=CARTESIAN_POINT('Ctrl Pts',(5.07821400434164,-6.06594292143509,
137.364182536701));
#229154=CARTESIAN_POINT('Ctrl Pts',(4.92603880247249,-6.19333914841155,
137.356174442168));
#229155=CARTESIAN_POINT('Ctrl Pts',(4.76893302042205,-6.31511772874101,
137.348166347636));
#229156=CARTESIAN_POINT('Ctrl Pts',(4.60734473284941,-6.43088605968764,
137.340158253103));
#229157=CARTESIAN_POINT('Ctrl Pts',(4.44588202042821,-6.54656442355863,
137.332156381903));
#229158=CARTESIAN_POINT('Ctrl Pts',(4.27994401469346,-6.65624165372637,
137.324154510703));
#229159=CARTESIAN_POINT('Ctrl Pts',(4.11001185674365,-6.75956533642708,
137.316152639504));
#229160=CARTESIAN_POINT('Ctrl Pts',(3.94018336624525,-6.86282598630938,
137.308155649861));
#229161=CARTESIAN_POINT('Ctrl Pts',(3.76636586409051,-6.95974064185519,
137.300158660219));
#229162=CARTESIAN_POINT('Ctrl Pts',(3.58906981975408,-7.04999991694542,
137.292161670577));
#229163=CARTESIAN_POINT('Ctrl Pts',(3.4118523266209,-7.14021920256668,137.284168224009));
#229164=CARTESIAN_POINT('Ctrl Pts',(3.23115965990965,-7.22378883490069,
137.276174777441));
#229165=CARTESIAN_POINT('Ctrl Pts',(3.0475276347068,-7.30044493957035,137.268181330874));
#229166=CARTESIAN_POINT('Ctrl Pts',(2.86394631192219,-7.3770798788149,137.260190091367));
#229167=CARTESIAN_POINT('Ctrl Pts',(2.67742755588218,-7.44680496804883,
137.252198851861));
#229168=CARTESIAN_POINT('Ctrl Pts',(2.48852833353138,-7.50940395325831,
137.244207612354));
#229169=CARTESIAN_POINT('Ctrl Pts',(2.29357765115322,-7.57400832129591,
137.235960370383));
#229170=CARTESIAN_POINT('Ctrl Pts',(2.09609179479209,-7.63102228981386,
137.227713128412));
#229171=CARTESIAN_POINT('Ctrl Pts',(1.89670189544186,-7.68026320641599,
137.219465886441));
#229172=CARTESIAN_POINT('Ctrl Pts',(1.70346233245657,-7.72798524868694,
137.211473037057));
#229173=CARTESIAN_POINT('Ctrl Pts',(1.50843478373704,-7.76840656863684,
137.203480187672));
#229174=CARTESIAN_POINT('Ctrl Pts',(1.31220603019056,-7.80141245764711,
137.195487338288));
#229175=CARTESIAN_POINT('Ctrl Pts',(1.11592948169991,-7.83442638581879,
137.187492542105));
#229176=CARTESIAN_POINT('Ctrl Pts',(0.918451473767237,-7.86002122647965,
137.179497745922));
#229177=CARTESIAN_POINT('Ctrl Pts',(0.720366334600081,-7.87813387446385,
137.17150294974));
#229178=CARTESIAN_POINT('Ctrl Pts',(0.522202939233237,-7.89625367809337,
137.163504995105));
#229179=CARTESIAN_POINT('Ctrl Pts',(0.323432266201273,-7.90688536532492,
137.15550704047));
#229180=CARTESIAN_POINT('Ctrl Pts',(0.124651486185002,-7.91001788917016,
137.147509085836));
#229181=CARTESIAN_POINT('Ctrl Pts',(-0.074237946007496,-7.91315212523089,
137.139506759576));
#229182=CARTESIAN_POINT('Ctrl Pts',(-0.273137163426149,-7.90877902027729,
137.131504433315));
#229183=CARTESIAN_POINT('Ctrl Pts',(-0.471450878998735,-7.89693960143367,
137.123502107055));
#229184=CARTESIAN_POINT('Ctrl Pts',(-0.670002770870968,-7.88508596335683,
137.115490169939));
#229185=CARTESIAN_POINT('Ctrl Pts',(-0.867967423520542,-7.86574811784401,
137.107478232823));
#229186=CARTESIAN_POINT('Ctrl Pts',(-1.06475525431146,-7.83901889578129,
137.099466295708));
#229187=CARTESIAN_POINT('Ctrl Pts',(-1.26168279717544,-7.81227069696066,
137.091448670413));
#229188=CARTESIAN_POINT('Ctrl Pts',(-1.45743152451879,-7.77812071217562,
137.083431045119));
#229189=CARTESIAN_POINT('Ctrl Pts',(-1.6514233551077,-7.73671260305078,
137.075413419824));
#229190=CARTESIAN_POINT('Ctrl Pts',(-1.84566907495877,-7.69525030053934,
137.067385301361));
#229191=CARTESIAN_POINT('Ctrl Pts',(-2.03815298324123,-7.6465109805656,
137.059357182898));
#229192=CARTESIAN_POINT('Ctrl Pts',(-2.22831228863559,-7.59068806791029,
137.051329064435));
#229193=CARTESIAN_POINT('Ctrl Pts',(-2.26822635722923,-7.57897094704576,
137.049643977974));
#229194=CARTESIAN_POINT('Ctrl Pts',(-2.3080380813465,-7.56694191164845,
137.047958891513));
#229195=CARTESIAN_POINT('Ctrl Pts',(-2.34774237437529,-7.55460301694025,
137.046273805051));
#229196=CARTESIAN_POINT('Ctrl Pts',(-2.53019976867307,-7.4979007712828,
137.038530146584));
#229197=CARTESIAN_POINT('Ctrl Pts',(-2.71093239789151,-7.43448165792094,
137.030786488117));
#229198=CARTESIAN_POINT('Ctrl Pts',(-2.88939377760752,-7.36446363273816,
137.02304282965));
#229199=CARTESIAN_POINT('Ctrl Pts',(-3.0676382729918,-7.29453070054651,
137.01530858206));
#229200=CARTESIAN_POINT('Ctrl Pts',(-3.2436166815152,-7.2180149475349,137.007574334471));
#229201=CARTESIAN_POINT('Ctrl Pts',(-3.41679451805204,-7.13508487836056,
136.999840086881));
#229202=CARTESIAN_POINT('Ctrl Pts',(-3.58979732104159,-7.05223862790388,
136.992113656417));
#229203=CARTESIAN_POINT('Ctrl Pts',(-3.76000486430489,-6.96299112005469,
136.984387225952));
#229204=CARTESIAN_POINT('Ctrl Pts',(-3.92689952899846,-6.86756005355262,
136.976660795487));
#229205=CARTESIAN_POINT('Ctrl Pts',(-4.09365959479012,-6.77220595126497,
136.968940596313));
#229206=CARTESIAN_POINT('Ctrl Pts',(-4.25711178994332,-6.67067839616624,
136.961220397138));
#229207=CARTESIAN_POINT('Ctrl Pts',(-4.41676007373928,-6.56324244950791,
136.953500197963));
#229208=CARTESIAN_POINT('Ctrl Pts',(-4.5763121659837,-6.45587123533624,
136.945784650376));
#229209=CARTESIAN_POINT('Ctrl Pts',(-4.73206461227333,-6.34259891835515,
136.938069102789));
#229210=CARTESIAN_POINT('Ctrl Pts',(-4.88354745926241,-6.2237356316871,
136.930353555202));
#229211=CARTESIAN_POINT('Ctrl Pts',(-5.03496990566085,-6.10491973924792,
136.922641084026));
#229212=CARTESIAN_POINT('Ctrl Pts',(-5.18212585994934,-5.98051753896768,
136.914928612851));
#229213=CARTESIAN_POINT('Ctrl Pts',(-5.32457571748206,-5.85088150869596,
136.907216141675));
#229214=CARTESIAN_POINT('Ctrl Pts',(-5.46702519221316,-5.72124582679163,
136.899503691226));
#229215=CARTESIAN_POINT('Ctrl Pts',(-5.60476832086258,-5.58637657686959,
136.891791240776));
#229216=CARTESIAN_POINT('Ctrl Pts',(-5.73739958768388,-5.4466656746348,
136.884078790326));
#229217=CARTESIAN_POINT('Ctrl Pts',(-5.87003721824548,-5.30694806897387,
136.876365969827));
#229218=CARTESIAN_POINT('Ctrl Pts',(-5.99756224937468,-5.16238860943103,
136.868653149329));
#229219=CARTESIAN_POINT('Ctrl Pts',(-6.11960711221558,-5.01341498303507,
136.86094032883));
#229220=CARTESIAN_POINT('Ctrl Pts',(-6.24168035510818,-4.86440671463026,
136.853225714809));
#229221=CARTESIAN_POINT('Ctrl Pts',(-6.35827066347908,-4.71098251444336,
136.845511100787));
#229222=CARTESIAN_POINT('Ctrl Pts',(-6.46905172182266,-4.5536019611274,
136.837796486766));
#229223=CARTESIAN_POINT('Ctrl Pts',(-6.57987899456815,-4.39615575355382,
136.830078654448));
#229224=CARTESIAN_POINT('Ctrl Pts',(-6.68489198454414,-4.23475020122318,
136.82236082213));
#229225=CARTESIAN_POINT('Ctrl Pts',(-6.78380852903311,-4.06987258294625,
136.814642989813));
#229226=CARTESIAN_POINT('Ctrl Pts',(-6.8828441955438,-3.90479640784218,
136.806915863157));
#229227=CARTESIAN_POINT('Ctrl Pts',(-6.97576856889581,-3.73624012568704,
136.799188736502));
#229228=CARTESIAN_POINT('Ctrl Pts',(-7.06234569075244,-3.56471518417818,
136.791461609846));
#229229=CARTESIAN_POINT('Ctrl Pts',(-7.14897920919224,-3.39307851083505,
136.783729449718));
#229230=CARTESIAN_POINT('Ctrl Pts',(-7.22925709111192,-3.21846965281537,
136.77599728959));
#229231=CARTESIAN_POINT('Ctrl Pts',(-7.30299218554266,-3.04141844176411,
136.768265129462));
#229232=CARTESIAN_POINT('Ctrl Pts',(-7.37684175556544,-2.86409235424645,
136.760520964961));
#229233=CARTESIAN_POINT('Ctrl Pts',(-7.44412812516747,-2.68431667691066,
136.75277680046));
#229234=CARTESIAN_POINT('Ctrl Pts',(-7.50471415038671,-2.50263591458795,
136.745032635958));
#229235=CARTESIAN_POINT('Ctrl Pts',(-7.54818005581054,-2.37229366480557,
136.739476781773));
#229236=CARTESIAN_POINT('Ctrl Pts',(-7.58819837098074,-2.24097114054649,
136.733920927587));
#229237=CARTESIAN_POINT('Ctrl Pts',(-7.6247348206606,-2.10887171601445,
136.728365073402));
#229238=CARTESIAN_POINT('Ctrl Pts',(-7.69817641599759,-1.84333982756507,
136.717197299893));
#229239=CARTESIAN_POINT('Ctrl Pts',(-7.75774424075977,-1.57396649721242,
136.706029526384));
#229240=CARTESIAN_POINT('Ctrl Pts',(-7.80312831751188,-1.30196369398084,
136.694861752875));
#229241=CARTESIAN_POINT('Ctrl Pts',(-7.84692604597825,-1.03946843637983,
136.684084336065));
#229242=CARTESIAN_POINT('Ctrl Pts',(-7.87751447532542,-0.77452376069535,
136.673306919254));
#229243=CARTESIAN_POINT('Ctrl Pts',(-7.89465718412611,-0.508241030541709,
136.662529502443));
#229244=CARTESIAN_POINT('Ctrl Pts',(-7.90536625412329,-0.341893901309606,
136.655796837708));
#229245=CARTESIAN_POINT('Ctrl Pts',(-7.91082891972596,-0.175025061706264,
136.649064172972));
#229246=CARTESIAN_POINT('Ctrl Pts',(-7.91099604399589,-0.00791150310789744,
136.642331508237));
#229247=CARTESIAN_POINT('',(-7.911,6.23723295234413E-12,134.642331508237));
#229248=CARTESIAN_POINT('Ctrl Pts',(-7.911,6.85784762310959E-12,136.642331508237));
#229249=CARTESIAN_POINT('Ctrl Pts',(-7.91099999999809,2.20167589667335,
136.553744072504));
#229250=CARTESIAN_POINT('Ctrl Pts',(-6.94214576672016,4.38610418339232,
136.465156636771));
#229251=CARTESIAN_POINT('Ctrl Pts',(-3.67820201487745,7.34180684107895,
136.287981765306));
#229252=CARTESIAN_POINT('Ctrl Pts',(-1.40868175871181,8.08992666571427,
136.199394329573));
#229253=CARTESIAN_POINT('Ctrl Pts',(2.97309270521754,7.65454228025063,136.022219458108));
#229254=CARTESIAN_POINT('Ctrl Pts',(5.05102072675981,6.47444880833921,135.933632022375));
#229255=CARTESIAN_POINT('Ctrl Pts',(7.66951518848019,2.934251953673,135.75645715091));
#229256=CARTESIAN_POINT('Ctrl Pts',(8.18956872247094,0.601881960095167,
135.667869715177));
#229257=CARTESIAN_POINT('Ctrl Pts',(7.32306689761179,-3.71537198232757,
135.490694843711));
#229258=CARTESIAN_POINT('Ctrl Pts',(5.94329958849978,-5.66643518936734,
135.402107407979));
#229259=CARTESIAN_POINT('Ctrl Pts',(2.16154501637591,-7.9220591323306,135.224932536513));
#229260=CARTESIAN_POINT('Ctrl Pts',(-0.210816529302679,-8.20894963712989,
135.136345100781));
#229261=CARTESIAN_POINT('Ctrl Pts',(-4.42123908576584,-6.91982244717729,
134.959170229315));
#229262=CARTESIAN_POINT('Ctrl Pts',(-6.22631625634278,-5.35390358803405,
134.870582793582));
#229263=CARTESIAN_POINT('Ctrl Pts',(-7.65317280859594,-2.31334857514253,
134.735440741312));
#229264=CARTESIAN_POINT('Ctrl Pts',(-7.91100000000091,-1.15702837836065,
134.688886124774));
#229265=CARTESIAN_POINT('Ctrl Pts',(-7.911,6.23723295234413E-12,134.642331508237));
#229266=CARTESIAN_POINT('',(-7.91099763196637,-0.00612103116663704,130.642331508237));
#229267=CARTESIAN_POINT('Ctrl Pts',(-7.91099965031895,0.00235215931849442,
134.634842937691));
#229268=CARTESIAN_POINT('Ctrl Pts',(-7.91070729992585,0.985612025887326,
134.597355279287));
#229269=CARTESIAN_POINT('Ctrl Pts',(-7.72714776753475,1.95996465666296,
134.567471101788));
#229270=CARTESIAN_POINT('Ctrl Pts',(-7.31415261496248,3.01836535369072,
134.525553036253));
#229271=CARTESIAN_POINT('Ctrl Pts',(-7.25437688176638,3.15933044397698,
134.519727960306));
#229272=CARTESIAN_POINT('Ctrl Pts',(-7.18066625036259,3.32001739034016,
134.512704803826));
#229273=CARTESIAN_POINT('Ctrl Pts',(-7.17068269178165,3.34152554982886,
134.511756670364));
#229274=CARTESIAN_POINT('Ctrl Pts',(-7.15767334640095,3.36922554119806,
134.510524739347));
#229275=CARTESIAN_POINT('Ctrl Pts',(-7.15473596741449,3.37545874174651,
134.510246816222));
#229276=CARTESIAN_POINT('Ctrl Pts',(-7.14995802542409,3.38556341111709,
134.509795135232));
#229277=CARTESIAN_POINT('Ctrl Pts',(-7.14812244722044,3.38943724760068,
134.509621702051));
#229278=CARTESIAN_POINT('Ctrl Pts',(-7.14459970572387,3.39685611393449,
134.509289038257));
#229279=CARTESIAN_POINT('Ctrl Pts',(-7.14291304972564,3.40040138480072,
134.509129840455));
#229280=CARTESIAN_POINT('Ctrl Pts',(-7.139069267868,3.40846535268475,134.508767219703));
#229281=CARTESIAN_POINT('Ctrl Pts',(-7.13691049146306,3.41298325640359,
134.508563690786));
#229282=CARTESIAN_POINT('Ctrl Pts',(-7.13020554840639,3.42698123384001,
134.507931956892));
#229283=CARTESIAN_POINT('Ctrl Pts',(-7.12564478750139,3.43645426274363,
134.507502823043));
#229284=CARTESIAN_POINT('Ctrl Pts',(-7.09139987360813,3.50722212627631,
134.504285084167));
#229285=CARTESIAN_POINT('Ctrl Pts',(-7.06094499922386,3.56813878738974,
134.501448365001));
#229286=CARTESIAN_POINT('Ctrl Pts',(-6.94142129914273,3.79968938528309,
134.490429767277));
#229287=CARTESIAN_POINT('Ctrl Pts',(-6.84692660120395,3.96743699089044,
134.481952306651));
#229288=CARTESIAN_POINT('Ctrl Pts',(-6.35550715057569,4.7698745756642,134.439527352387));
#229289=CARTESIAN_POINT('Ctrl Pts',(-5.87597847899331,5.34951237034305,
134.403378010267));
#229290=CARTESIAN_POINT('Ctrl Pts',(-5.19235134669754,5.97110921833049,
134.362495107838));
#229291=CARTESIAN_POINT('Ctrl Pts',(-5.05874729136224,6.08471352498639,
134.354890940838));
#229292=CARTESIAN_POINT('Ctrl Pts',(-4.83613591494947,6.26159648918448,
134.342843428782));
#229293=CARTESIAN_POINT('Ctrl Pts',(-4.74940477550864,6.32763437006564,
134.338293640868));
#229294=CARTESIAN_POINT('Ctrl Pts',(-4.62873102055958,6.41563702386578,
134.332155401607));
#229295=CARTESIAN_POINT('Ctrl Pts',(-4.59594603103169,6.43916372101804,
134.3305066431));
#229296=CARTESIAN_POINT('Ctrl Pts',(-4.53985110592844,6.4787710813844,134.327717306397));
#229297=CARTESIAN_POINT('Ctrl Pts',(-4.51663239555363,6.4949791850433,134.326571864853));
#229298=CARTESIAN_POINT('Ctrl Pts',(-4.48437192529442,6.51724234787714,
134.324992834236));
#229299=CARTESIAN_POINT('Ctrl Pts',(-4.47540408339446,6.52340384131562,
134.324555216067));
#229300=CARTESIAN_POINT('Ctrl Pts',(-4.46087077750231,6.53334509775676,
134.323848143605));
#229301=CARTESIAN_POINT('Ctrl Pts',(-4.45531316819409,6.53713628690428,
134.323578258616));
#229302=CARTESIAN_POINT('Ctrl Pts',(-4.44370971825894,6.54503004751404,
134.3230158255));
#229303=CARTESIAN_POINT('Ctrl Pts',(-4.43766301505954,6.54913134302183,
134.322723325478));
#229304=CARTESIAN_POINT('Ctrl Pts',(-4.42363768719583,6.55861595541005,
134.32204623608));
#229305=CARTESIAN_POINT('Ctrl Pts',(-4.4156548952219,6.56399310521258,134.321661878074));
#229306=CARTESIAN_POINT('Ctrl Pts',(-4.38985596927511,6.58130271037187,
134.320422981844));
#229307=CARTESIAN_POINT('Ctrl Pts',(-4.37200105934812,6.59317734804389,
134.319570602593));
#229308=CARTESIAN_POINT('Ctrl Pts',(-4.20428424590407,6.70373870007293,
134.311610559462));
#229309=CARTESIAN_POINT('Ctrl Pts',(-4.05114905908561,6.79737558017027,
134.304691823014));
#229310=CARTESIAN_POINT('Ctrl Pts',(-3.65788389168276,7.01982852255921,
134.287689075509));
#229311=CARTESIAN_POINT('Ctrl Pts',(-3.41403731740536,7.14160119837584,
134.277837359741));
#229312=CARTESIAN_POINT('Ctrl Pts',(-3.00391008688681,7.32059442494948,
134.262012632256));
#229313=CARTESIAN_POINT('Ctrl Pts',(-2.84115202323861,7.38528503494512,
134.25591347262));
#229314=CARTESIAN_POINT('Ctrl Pts',(-2.36201510346746,7.55753953663914,
134.238248325779));
#229315=CARTESIAN_POINT('Ctrl Pts',(-2.04081550068744,7.65052808493037,
134.226772596442));
#229316=CARTESIAN_POINT('Ctrl Pts',(-1.42065228693337,7.78822194147042,
134.204015471019));
#229317=CARTESIAN_POINT('Ctrl Pts',(-1.12316738090208,7.83665441464296,
134.192789956154));
#229318=CARTESIAN_POINT('Ctrl Pts',(-0.801294635919355,7.87034624121721,
134.179894009537));
#229319=CARTESIAN_POINT('Ctrl Pts',(-0.779000233120226,7.87258418023723,
134.178997701949));
#229320=CARTESIAN_POINT('Ctrl Pts',(-0.747228429024424,7.87563719021797,
134.177716225397));
#229321=CARTESIAN_POINT('Ctrl Pts',(-0.737758487662745,7.87652993964204,
134.177333742565));
#229322=CARTESIAN_POINT('Ctrl Pts',(-0.721428555241354,7.87803968508456,
134.176673307624));
#229323=CARTESIAN_POINT('Ctrl Pts',(-0.714569314518207,7.87866480658477,
134.17639562941));
#229324=CARTESIAN_POINT('Ctrl Pts',(-0.701450640028202,7.87984311304252,
134.175864050023));
#229325=CARTESIAN_POINT('Ctrl Pts',(-0.695191344606962,7.88039779964692,
134.175610198683));
#229326=CARTESIAN_POINT('Ctrl Pts',(-0.680550704538279,7.88167764574459,
134.175015929004));
#229327=CARTESIAN_POINT('Ctrl Pts',(-0.672168857583668,7.88239689429476,
134.174675319079));
#229328=CARTESIAN_POINT('Ctrl Pts',(-0.642411189064694,7.88490259810949,
134.173464722853));
#229329=CARTESIAN_POINT('Ctrl Pts',(-0.621029356463556,7.88661547475162,
134.172592407784));
#229330=CARTESIAN_POINT('Ctrl Pts',(-0.253090550480812,7.9145851017779,
134.157541563156));
#229331=CARTESIAN_POINT('Ctrl Pts',(0.0948079532204345,7.91806201106853,
134.142720512965));
#229332=CARTESIAN_POINT('Ctrl Pts',(0.559162513855125,7.89208955629123,
134.122747046785));
#229333=CARTESIAN_POINT('Ctrl Pts',(0.67637341337458,7.88290931110074,134.117686834216));
#229334=CARTESIAN_POINT('Ctrl Pts',(1.69832656368766,7.77990591646846,134.073493473426));
#229335=CARTESIAN_POINT('Ctrl Pts',(2.58087950293275,7.53328953772175,134.035568794168));
#229336=CARTESIAN_POINT('Ctrl Pts',(3.45796295061826,7.11549290833311,133.996144003404));
#229337=CARTESIAN_POINT('Ctrl Pts',(3.51349273445849,7.08823786101105,133.993640896697));
#229338=CARTESIAN_POINT('Ctrl Pts',(3.59300282443886,7.04804890630641,133.990046534826));
#229339=CARTESIAN_POINT('Ctrl Pts',(3.61724467631051,7.03563811180938,133.988949251469));
#229340=CARTESIAN_POINT('Ctrl Pts',(3.65940401583432,7.0137788338023,133.987038472488));
#229341=CARTESIAN_POINT('Ctrl Pts',(3.67735017555703,7.00438626645202,133.986224313934));
#229342=CARTESIAN_POINT('Ctrl Pts',(3.71379968247048,6.98513081896998,133.984569087552));
#229343=CARTESIAN_POINT('Ctrl Pts',(3.73230029191427,6.97526308992605,133.983728086593));
#229344=CARTESIAN_POINT('Ctrl Pts',(3.77872308343237,6.95026484566663,133.981615589364));
#229345=CARTESIAN_POINT('Ctrl Pts',(3.80659383434492,6.93503950653828,133.980345294921));
#229346=CARTESIAN_POINT('Ctrl Pts',(3.91146992995167,6.8769246916588,133.975557335384));
#229347=CARTESIAN_POINT('Ctrl Pts',(3.98784878023691,6.83291684146512,133.972054252011));
#229348=CARTESIAN_POINT('Ctrl Pts',(4.57845825960972,6.47934367071942,133.944822035303));
#229349=CARTESIAN_POINT('Ctrl Pts',(5.05667537576387,6.11344492418261,133.922074582275));
#229350=CARTESIAN_POINT('Ctrl Pts',(5.60901817140684,5.58127707323018,133.892429913593));
#229351=CARTESIAN_POINT('Ctrl Pts',(5.72543544308371,5.46178778410835,133.885944362167));
#229352=CARTESIAN_POINT('Ctrl Pts',(5.89284034526309,5.27872717451378,133.87615645709));
#229353=CARTESIAN_POINT('Ctrl Pts',(5.94676546202799,5.21790265562518,133.872927112294));
#229354=CARTESIAN_POINT('Ctrl Pts',(6.01172370144999,5.14231825285087,133.868931546136));
#229355=CARTESIAN_POINT('Ctrl Pts',(6.02365567218836,5.12833610587973,133.868193113736));
#229356=CARTESIAN_POINT('Ctrl Pts',(6.04275714719806,5.10579393722438,133.867003683716));
#229357=CARTESIAN_POINT('Ctrl Pts',(6.0499574054631,5.09726015232854,133.866553655817));
#229358=CARTESIAN_POINT('Ctrl Pts',(6.06367642953856,5.08093027219427,133.865693012521));
#229359=CARTESIAN_POINT('Ctrl Pts',(6.07019829018416,5.07313679986769,133.865282489572));
#229360=CARTESIAN_POINT('Ctrl Pts',(6.08509601278354,5.0552645086772,133.864341590493));
#229361=CARTESIAN_POINT('Ctrl Pts',(6.09346187737195,5.04517740867602,133.863810931039));
#229362=CARTESIAN_POINT('Ctrl Pts',(6.11916652746654,5.01402695513974,133.862173418814));
#229363=CARTESIAN_POINT('Ctrl Pts',(6.13642139375905,4.99289472784215,133.861064287228));
#229364=CARTESIAN_POINT('Ctrl Pts',(6.34265325608749,4.73763632870868,133.847690102012));
#229365=CARTESIAN_POINT('Ctrl Pts',(6.51823038483631,4.49300710983339,133.835113530052));
#229366=CARTESIAN_POINT('Ctrl Pts',(6.87405300120233,3.9323305228053,133.807240717542));
#229367=CARTESIAN_POINT('Ctrl Pts',(7.04731747628843,3.61263778420711,133.791961776323));
#229368=CARTESIAN_POINT('Ctrl Pts',(7.26674204946458,3.1314262023491,133.770028037084));
#229369=CARTESIAN_POINT('Ctrl Pts',(7.3307278590558,2.97855678215018,133.763203941213));
#229370=CARTESIAN_POINT('Ctrl Pts',(7.41585392593125,2.75578154225637,133.753457413638));
#229371=CARTESIAN_POINT('Ctrl Pts',(7.44090088381112,2.68741800260095,133.75049258707));
#229372=CARTESIAN_POINT('Ctrl Pts',(7.48416387073204,2.5640911608469,133.745188889147));
#229373=CARTESIAN_POINT('Ctrl Pts',(7.50272685477848,2.50925529376175,133.742846356551));
#229374=CARTESIAN_POINT('Ctrl Pts',(7.5298989167658,2.42598952085995,133.739311936622));
#229375=CARTESIAN_POINT('Ctrl Pts',(7.53895246049939,2.39770695842284,133.738115329271));
#229376=CARTESIAN_POINT('Ctrl Pts',(7.55499794020347,2.34659269046629,133.735959587966));
#229377=CARTESIAN_POINT('Ctrl Pts',(7.56204615435491,2.32377905467626,133.734999875491));
#229378=CARTESIAN_POINT('Ctrl Pts',(7.57704736052552,2.27443213586511,133.732929127839));
#229379=CARTESIAN_POINT('Ctrl Pts',(7.58496450688547,2.24788827120917,133.731818472487));
#229380=CARTESIAN_POINT('Ctrl Pts',(7.60577576594224,2.17675232082948,133.728850270435));
#229381=CARTESIAN_POINT('Ctrl Pts',(7.61841711327296,2.13208733031883,133.726995276738));
#229382=CARTESIAN_POINT('Ctrl Pts',(7.6813222812751,1.90212271964092,133.717486283887));
#229383=CARTESIAN_POINT('Ctrl Pts',(7.72522185659126,1.71514757806987,133.709892612196));
#229384=CARTESIAN_POINT('Ctrl Pts',(7.84100751703233,1.12647591692705,133.686280670193));
#229385=CARTESIAN_POINT('Ctrl Pts',(7.88866097942817,0.720691615053063,
133.670522200799));
#229386=CARTESIAN_POINT('Ctrl Pts',(7.91876629570847,-0.0395408363007919,
133.641787822611));
#229387=CARTESIAN_POINT('Ctrl Pts',(7.90912452918413,-0.392651176533162,
133.628744523392));
#229388=CARTESIAN_POINT('Ctrl Pts',(7.84733411201154,-1.04681399129394,
133.604330554539));
#229389=CARTESIAN_POINT('Ctrl Pts',(7.80127938114409,-1.34777551333776,
133.592990423676));
#229390=CARTESIAN_POINT('Ctrl Pts',(7.71584317862537,-1.74958475678387,
133.577072051011));
#229391=CARTESIAN_POINT('Ctrl Pts',(7.69156990597228,-1.85338448485048,
133.572886854609));
#229392=CARTESIAN_POINT('Ctrl Pts',(7.66151993466688,-1.97110516497737,
133.568029101787));
#229393=CARTESIAN_POINT('Ctrl Pts',(7.65779159723041,-1.98554051342504,
133.567431503542));
#229394=CARTESIAN_POINT('Ctrl Pts',(7.65210661151424,-2.0072973965174,133.566527800184));
#229395=CARTESIAN_POINT('Ctrl Pts',(7.65018020112903,-2.0146268443092,133.56622284566));
#229396=CARTESIAN_POINT('Ctrl Pts',(7.64683971670512,-2.02726256394383,
133.565696209394));
#229397=CARTESIAN_POINT('Ctrl Pts',(7.64543064191786,-2.03257016006475,
133.565474721768));
#229398=CARTESIAN_POINT('Ctrl Pts',(7.6425084731209,-2.04353113224334,133.565016740222));
#229399=CARTESIAN_POINT('Ctrl Pts',(7.64099463032019,-2.04918430341032,
133.564780216944));
#229400=CARTESIAN_POINT('Ctrl Pts',(7.63688040825467,-2.06448017033174,
133.564139382174));
#229401=CARTESIAN_POINT('Ctrl Pts',(7.63426804489553,-2.07411961110434,
133.563734591974));
#229402=CARTESIAN_POINT('Ctrl Pts',(7.62450382469438,-2.1098805438719,133.562229321277));
#229403=CARTESIAN_POINT('Ctrl Pts',(7.61723614995478,-2.13597001216449,
133.561124096314));
#229404=CARTESIAN_POINT('Ctrl Pts',(7.50475422953521,-2.53188136403538,
133.544238339615));
#229405=CARTESIAN_POINT('Ctrl Pts',(7.37287032290911,-2.89351464806571,
133.527128447268));
#229406=CARTESIAN_POINT('Ctrl Pts',(7.00605023781762,-3.70937581191444,
133.486318696312));
#229407=CARTESIAN_POINT('Ctrl Pts',(6.75230222157421,-4.15339250603831,
133.462483465425));
#229408=CARTESIAN_POINT('Ctrl Pts',(6.22613584299422,-4.89690262860306,
133.421778811307));
#229409=CARTESIAN_POINT('Ctrl Pts',(5.97018612154915,-5.20589648393161,
133.404554765575));
#229410=CARTESIAN_POINT('Ctrl Pts',(5.67758223457798,-5.50902949833257,
133.387415659092));
#229411=CARTESIAN_POINT('Ctrl Pts',(5.66320599660458,-5.52380701074462,
133.386579379995));
#229412=CARTESIAN_POINT('Ctrl Pts',(5.63718616773183,-5.55034476175778,
133.385076157805));
#229413=CARTESIAN_POINT('Ctrl Pts',(5.62556315584081,-5.56212495794752,
133.384408364525));
#229414=CARTESIAN_POINT('Ctrl Pts',(5.60762225853358,-5.58019471661327,
133.383383225783));
#229415=CARTESIAN_POINT('Ctrl Pts',(5.60133059520238,-5.58651018379219,
133.383024782751));
#229416=CARTESIAN_POINT('Ctrl Pts',(5.58975131153417,-5.59809404972464,
133.382367040442));
#229417=CARTESIAN_POINT('Ctrl Pts',(5.58446688802854,-5.60336562177147,
133.382067607274));
#229418=CARTESIAN_POINT('Ctrl Pts',(5.57304962634139,-5.61472292368488,
133.381422258032));
#229419=CARTESIAN_POINT('Ctrl Pts',(5.56691426036116,-5.62080610462478,
133.381076449332));
#229420=CARTESIAN_POINT('Ctrl Pts',(5.55031288731839,-5.63721242783764,
133.380143398481));
#229421=CARTESIAN_POINT('Ctrl Pts',(5.53982802947232,-5.64751649049666,
133.379556956423));
#229422=CARTESIAN_POINT('Ctrl Pts',(5.49096890530847,-5.69526612424974,
133.376837266112));
#229423=CARTESIAN_POINT('Ctrl Pts',(5.45224291384226,-5.73235057283614,
133.374719067983));
#229424=CARTESIAN_POINT('Ctrl Pts',(4.79460626787116,-6.34941710530771,
133.339360709573));
#229425=CARTESIAN_POINT('Ctrl Pts',(4.08682396485852,-6.82650753453245,
133.311041472194));
#229426=CARTESIAN_POINT('Ctrl Pts',(3.13105028480155,-7.26789524810983,
133.274251508648));
#229427=CARTESIAN_POINT('Ctrl Pts',(2.9420600289252,-7.34643143552284,133.267002245191));
#229428=CARTESIAN_POINT('Ctrl Pts',(2.56533779673298,-7.48611074256786,
133.252282692327));
#229429=CARTESIAN_POINT('Ctrl Pts',(2.37794176554221,-7.54772788883545,
133.244834406396));
#229430=CARTESIAN_POINT('Ctrl Pts',(2.1587941132795,-7.61081345082955,133.235804191481));
#229431=CARTESIAN_POINT('Ctrl Pts',(2.129088041258,-7.61917695493053,133.234573398669));
#229432=CARTESIAN_POINT('Ctrl Pts',(2.09053706622166,-7.62978761346753,
133.232968143788));
#229433=CARTESIAN_POINT('Ctrl Pts',(2.08173579709158,-7.63219367691513,
133.232601121995));
#229434=CARTESIAN_POINT('Ctrl Pts',(2.0674874736476,-7.63606235935512,133.232006103539));
#229435=CARTESIAN_POINT('Ctrl Pts',(2.06204296605477,-7.63753439373948,
133.231778537279));
#229436=CARTESIAN_POINT('Ctrl Pts',(2.05163158021397,-7.640337381323,133.231342991638));
#229437=CARTESIAN_POINT('Ctrl Pts',(2.04666496741692,-7.64166931712836,
133.231135056612));
#229438=CARTESIAN_POINT('Ctrl Pts',(2.03528565281477,-7.64470910833343,
133.230658274311));
#229439=CARTESIAN_POINT('Ctrl Pts',(2.02887209892744,-7.64641373752436,
133.230389284008));
#229440=CARTESIAN_POINT('Ctrl Pts',(2.00912226465456,-7.65163635822852,
133.229560147507));
#229441=CARTESIAN_POINT('Ctrl Pts',(1.99577896739489,-7.65512753276163,
133.228998833104));
#229442=CARTESIAN_POINT('Ctrl Pts',(1.8940200609301,-7.68146785568417,133.224709823971));
#229443=CARTESIAN_POINT('Ctrl Pts',(1.80522598327546,-7.70281888062695,
133.220919620551));
#229444=CARTESIAN_POINT('Ctrl Pts',(1.68105091908591,-7.73041245831064,
133.215571143747));
#229445=CARTESIAN_POINT('Ctrl Pts',(1.64596491820787,-7.7379589306676,133.214054601859));
#229446=CARTESIAN_POINT('Ctrl Pts',(1.58843284128214,-7.74992421876095,
133.211560385568));
#229447=CARTESIAN_POINT('Ctrl Pts',(1.56601660242534,-7.75448491381215,
133.210586710666));
#229448=CARTESIAN_POINT('Ctrl Pts',(1.53012554898418,-7.76162515323484,
133.209025078937));
#229449=CARTESIAN_POINT('Ctrl Pts',(1.51666318428827,-7.76426699684858,
133.208438728657));
#229450=CARTESIAN_POINT('Ctrl Pts',(1.49458726240653,-7.76853955171889,
133.207476301363));
#229451=CARTESIAN_POINT('Ctrl Pts',(1.48597772331084,-7.77019099230378,
133.207100729824));
#229452=CARTESIAN_POINT('Ctrl Pts',(0.968007310495516,-7.86865323204229,
133.18449235496));
#229453=CARTESIAN_POINT('Ctrl Pts',(0.450363337993549,-7.91517129740445,
133.161258006488));
#229454=CARTESIAN_POINT('Ctrl Pts',(-0.506622248122634,-7.90693083020566,
133.119693833949));
#229455=CARTESIAN_POINT('Ctrl Pts',(-0.944074815662322,-7.86670157855124,
133.10121159228));
#229456=CARTESIAN_POINT('Ctrl Pts',(-1.41494310503345,-7.78353541275905,
133.081836339441));
#229457=CARTESIAN_POINT('Ctrl Pts',(-1.45386701724515,-7.77635893222157,
133.080238064113));
#229458=CARTESIAN_POINT('Ctrl Pts',(-1.50987809959367,-7.7655968113854,
133.07794248971));
#229459=CARTESIAN_POINT('Ctrl Pts',(-1.5270096387014,-7.76224627790212,
133.077240949834));
#229460=CARTESIAN_POINT('Ctrl Pts',(-1.55680197414965,-7.75631713847533,
133.076021904543));
#229461=CARTESIAN_POINT('Ctrl Pts',(-1.56946778405745,-7.75376417072802,
133.075503945207));
#229462=CARTESIAN_POINT('Ctrl Pts',(-1.59388259695865,-7.7487807564321,
133.074506071615));
#229463=CARTESIAN_POINT('Ctrl Pts',(-1.60563243399604,-7.74635458986578,
133.074026083752));
#229464=CARTESIAN_POINT('Ctrl Pts',(-1.63343359860102,-7.74054809098502,
133.072890946134));
#229465=CARTESIAN_POINT('Ctrl Pts',(-1.64948003606043,-7.73714454322557,
133.072236200578));
#229466=CARTESIAN_POINT('Ctrl Pts',(-1.70531399080936,-7.72512022872451,
133.069959415842));
#229467=CARTESIAN_POINT('Ctrl Pts',(-1.74504570474384,-7.71624221216602,
133.068341700819));
#229468=CARTESIAN_POINT('Ctrl Pts',(-2.31842962929609,-7.5834648993405,
133.045026853933));
#229469=CARTESIAN_POINT('Ctrl Pts',(-2.83788091781876,-7.404764578742,133.024437070825));
#229470=CARTESIAN_POINT('Ctrl Pts',(-3.70050535140613,-7.00377711255711,
132.98935913984));
#229471=CARTESIAN_POINT('Ctrl Pts',(-4.05274236678752,-6.80601913273081,
132.974707058697));
#229472=CARTESIAN_POINT('Ctrl Pts',(-4.51532203922729,-6.49762074068063,
132.95371295952));
#229473=CARTESIAN_POINT('Ctrl Pts',(-4.63981385001518,-6.4093161283117,
132.947868090166));
#229474=CARTESIAN_POINT('Ctrl Pts',(-4.81855291739327,-6.27459501774054,
132.939093320269));
#229475=CARTESIAN_POINT('Ctrl Pts',(-4.8748530202892,-6.23095518493975,
132.936271198236));
#229476=CARTESIAN_POINT('Ctrl Pts',(-4.94080434151334,-6.17839341817899,
132.93288776733));
#229477=CARTESIAN_POINT('Ctrl Pts',(-4.95103325520092,-6.1701995489811,
132.932360763013));
#229478=CARTESIAN_POINT('Ctrl Pts',(-4.96672536427735,-6.15756524278659,
132.93154877244));
#229479=CARTESIAN_POINT('Ctrl Pts',(-4.9722030998187,-6.1531428471209,132.931264664718));
#229480=CARTESIAN_POINT('Ctrl Pts',(-4.98216508254784,-6.14507814963483,
132.930746759957));
#229481=CARTESIAN_POINT('Ctrl Pts',(-4.98665126082799,-6.14143823363323,
132.930513081179));
#229482=CARTESIAN_POINT('Ctrl Pts',(-4.99640521975191,-6.13350650519537,
132.930004021262));
#229483=CARTESIAN_POINT('Ctrl Pts',(-5.00167146319756,-6.12921281594096,
132.92972854583));
#229484=CARTESIAN_POINT('Ctrl Pts',(-5.01596277626851,-6.11753009611935,
132.928979243361));
#229485=CARTESIAN_POINT('Ctrl Pts',(-5.0249770248426,-6.11012789945369,
132.92850474358));
#229486=CARTESIAN_POINT('Ctrl Pts',(-5.06756018200102,-6.07500208019946,
132.926254173087));
#229487=CARTESIAN_POINT('Ctrl Pts',(-5.10091578014011,-6.04702195858714,
132.924464624876));
#229488=CARTESIAN_POINT('Ctrl Pts',(-5.74071032088883,-5.50127414999527,
132.889590353419));
#229489=CARTESIAN_POINT('Ctrl Pts',(-6.26558824262071,-4.89509781934732,
132.851114189951));
#229490=CARTESIAN_POINT('Ctrl Pts',(-6.79381420856736,-4.05772977819765,
132.806695808827));
#229491=CARTESIAN_POINT('Ctrl Pts',(-6.89067463871677,-3.89097563987157,
132.798192330299));
#229492=CARTESIAN_POINT('Ctrl Pts',(-7.06894195865911,-3.55649584051316,
132.781862440196));
#229493=CARTESIAN_POINT('Ctrl Pts',(-7.15070641823623,-3.38910122292492,
132.774027862526));
#229494=CARTESIAN_POINT('Ctrl Pts',(-7.24726399696753,-3.17233227011671,
132.764313071881));
#229495=CARTESIAN_POINT('Ctrl Pts',(-7.26758592360581,-3.12549555249587,
132.762238864005));
#229496=CARTESIAN_POINT('Ctrl Pts',(-7.2926000190712,-3.06628128004778,
132.759647391238));
#229497=CARTESIAN_POINT('Ctrl Pts',(-7.29771619536364,-3.05408484832029,
132.75911526137));
#229498=CARTESIAN_POINT('Ctrl Pts',(-7.30580459412044,-3.03466657468794,
132.758270638272));
#229499=CARTESIAN_POINT('Ctrl Pts',(-7.3087967393643,-3.02745308966572,
132.757957446682));
#229500=CARTESIAN_POINT('Ctrl Pts',(-7.31440893042893,-3.01386636745109,
132.757368611941));
#229501=CARTESIAN_POINT('Ctrl Pts',(-7.31703133887523,-3.00749411780485,
132.757092886149));
#229502=CARTESIAN_POINT('Ctrl Pts',(-7.32290257600748,-2.99317433174094,
132.756474260389));
#229503=CARTESIAN_POINT('Ctrl Pts',(-7.32614680117663,-2.98522491047493,
132.756131521948));
#229504=CARTESIAN_POINT('Ctrl Pts',(-7.33435331598121,-2.96502229344952,
132.755262216481));
#229505=CARTESIAN_POINT('Ctrl Pts',(-7.33929785405295,-2.95276188949425,
132.754736271418));
#229506=CARTESIAN_POINT('Ctrl Pts',(-7.36632075766717,-2.88526906219566,
132.751849792611));
#229507=CARTESIAN_POINT('Ctrl Pts',(-7.38780667218553,-2.82980067198163,
132.749510017625));
#229508=CARTESIAN_POINT('Ctrl Pts',(-7.74144172349002,-1.88536139352956,
132.710205925155));
#229509=CARTESIAN_POINT('Ctrl Pts',(-7.91156124447503,-0.944180572107552,
132.6802555473));
#229510=CARTESIAN_POINT('Ctrl Pts',(-7.91079403691426,0.349697463186542,
132.635479842313));
#229511=CARTESIAN_POINT('Ctrl Pts',(-7.88802041595599,0.69428979537607,
132.623065240056));
#229512=CARTESIAN_POINT('Ctrl Pts',(-7.8399067843408,1.05843422534096,132.608464906672));
#229513=CARTESIAN_POINT('Ctrl Pts',(-7.83688259007172,1.08059828160568,
132.607570325048));
#229514=CARTESIAN_POINT('Ctrl Pts',(-7.83280230077181,1.10958404852886,
132.606392331632));
#229515=CARTESIAN_POINT('Ctrl Pts',(-7.8318311968387,1.11641781934443,132.606114016469));
#229516=CARTESIAN_POINT('Ctrl Pts',(-7.83032011123745,1.12695250296761,
132.605684058254));
#229517=CARTESIAN_POINT('Ctrl Pts',(-7.8297864445307,1.13065433326774,132.605532798433));
#229518=CARTESIAN_POINT('Ctrl Pts',(-7.82871960159197,1.13801761417929,
132.605231578536));
#229519=CARTESIAN_POINT('Ctrl Pts',(-7.82818648131557,1.14167907232754,
132.605081621898));
#229520=CARTESIAN_POINT('Ctrl Pts',(-7.82700032130464,1.14978570017987,
132.604749227264));
#229521=CARTESIAN_POINT('Ctrl Pts',(-7.82634606344601,1.15423068804853,
132.60456671424));
#229522=CARTESIAN_POINT('Ctrl Pts',(-7.82442888579746,1.16717929963073,
132.604034288818));
#229523=CARTESIAN_POINT('Ctrl Pts',(-7.82315589737849,1.17568138137508,
132.603683756536));
#229524=CARTESIAN_POINT('Ctrl Pts',(-7.81384825565771,1.23716111636876,
132.601142298232));
#229525=CARTESIAN_POINT('Ctrl Pts',(-7.80528957724058,1.29005679416012,
132.598919640146));
#229526=CARTESIAN_POINT('Ctrl Pts',(-7.77629181563464,1.45840804539193,
132.591740579816));
#229527=CARTESIAN_POINT('Ctrl Pts',(-7.75382367888209,1.57349431919397,
132.586675066249));
#229528=CARTESIAN_POINT('Ctrl Pts',(-7.68718367562894,1.87861135635095,
132.572908619207));
#229529=CARTESIAN_POINT('Ctrl Pts',(-7.63852693029445,2.06757660174795,
132.564032356975));
#229530=CARTESIAN_POINT('Ctrl Pts',(-7.4032556108462,2.85888983844256,132.525931213477));
#229531=CARTESIAN_POINT('Ctrl Pts',(-7.15193399510597,3.43968874569621,
132.495888226658));
#229532=CARTESIAN_POINT('Ctrl Pts',(-6.68726901109647,4.23669451729892,
132.455320214001));
#229533=CARTESIAN_POINT('Ctrl Pts',(-6.52637555043864,4.48057979793452,
132.442964007059));
#229534=CARTESIAN_POINT('Ctrl Pts',(-6.33897517602841,4.733055937788,132.430249526307));
#229535=CARTESIAN_POINT('Ctrl Pts',(-6.32552082676708,4.75102210838096,
132.429345124625));
#229536=CARTESIAN_POINT('Ctrl Pts',(-6.3067318518487,4.7758905384318,132.428093721272));
#229537=CARTESIAN_POINT('Ctrl Pts',(-6.30146206687178,4.78284150967167,
132.427743990978));
#229538=CARTESIAN_POINT('Ctrl Pts',(-6.29237171337033,4.79479079837239,
132.427142856981));
#229539=CARTESIAN_POINT('Ctrl Pts',(-6.28855666442385,4.79979329325549,
132.426891220509));
#229540=CARTESIAN_POINT('Ctrl Pts',(-6.28067634582337,4.81010086266624,
132.426372775902));
#229541=CARTESIAN_POINT('Ctrl Pts',(-6.27661031155478,4.8154053481719,132.426106000436));
#229542=CARTESIAN_POINT('Ctrl Pts',(-6.2671414787767,4.82772587246902,132.42548643089));
#229543=CARTESIAN_POINT('Ctrl Pts',(-6.26173360756573,4.83473801185716,
132.425133852276));
#229544=CARTESIAN_POINT('Ctrl Pts',(-6.24451420314792,4.85698827238664,
132.424015217613));
#229545=CARTESIAN_POINT('Ctrl Pts',(-6.2326586894807,4.87219235858723,132.423251031534));
#229546=CARTESIAN_POINT('Ctrl Pts',(-6.03266174936424,5.12675356772148,
132.41045918577));
#229547=CARTESIAN_POINT('Ctrl Pts',(-5.83090562105139,5.35510718071116,
132.39904283836));
#229548=CARTESIAN_POINT('Ctrl Pts',(-5.37409704208839,5.81562124434117,
132.375682576322));
#229549=CARTESIAN_POINT('Ctrl Pts',(-5.1160291526152,6.04389177312378,132.363892858781));
#229550=CARTESIAN_POINT('Ctrl Pts',(-4.72459843231501,6.34703584617935,
132.347059890264));
#229551=CARTESIAN_POINT('Ctrl Pts',(-4.60266736571015,6.43600397450812,
132.341945763408));
#229552=CARTESIAN_POINT('Ctrl Pts',(-4.32907020419059,6.62388319103574,
132.330604430325));
#229553=CARTESIAN_POINT('Ctrl Pts',(-4.17640482476983,6.72118419779869,
132.324362193736));
#229554=CARTESIAN_POINT('Ctrl Pts',(-3.78522390914374,6.95202548985871,
132.308258022734));
#229555=CARTESIAN_POINT('Ctrl Pts',(-3.54288907325115,7.07859378672325,
132.298185098513));
#229556=CARTESIAN_POINT('Ctrl Pts',(-3.27938054635856,7.19929589736811,
132.286617318392));
#229557=CARTESIAN_POINT('Ctrl Pts',(-3.26422227536739,7.20618145228941,
132.285949766988));
#229558=CARTESIAN_POINT('Ctrl Pts',(-3.24391566411867,7.21532839023156,
132.285052540998));
#229559=CARTESIAN_POINT('Ctrl Pts',(-3.23878659945979,7.21763215865377,
132.284825670729));
#229560=CARTESIAN_POINT('Ctrl Pts',(-3.23014665842847,7.22150180664221,
132.284443094412));
#229561=CARTESIAN_POINT('Ctrl Pts',(-3.22663708181063,7.22307060193075,
132.284287576152));
#229562=CARTESIAN_POINT('Ctrl Pts',(-3.21991977061475,7.22606739517272,
132.28398969833));
#229563=CARTESIAN_POINT('Ctrl Pts',(-3.21671222507537,7.22749581734567,
132.283847365915));
#229564=CARTESIAN_POINT('Ctrl Pts',(-3.20920875403746,7.23083136749603,
132.283514186062));
#229565=CARTESIAN_POINT('Ctrl Pts',(-3.20491208181411,7.23273680150267,
132.283323231333));
#229566=CARTESIAN_POINT('Ctrl Pts',(-3.19260203803161,7.23818278136748,
132.282775667751));
#229567=CARTESIAN_POINT('Ctrl Pts',(-3.18458450179376,7.24171383717131,
132.282418463611));
#229568=CARTESIAN_POINT('Ctrl Pts',(-3.13303703051839,7.26431403887533,
132.280118258212));
#229569=CARTESIAN_POINT('Ctrl Pts',(-3.08934271334617,7.28300356365285,
132.278151924914));
#229570=CARTESIAN_POINT('Ctrl Pts',(-2.95642056211746,7.33844743554331,
132.272126017307));
#229571=CARTESIAN_POINT('Ctrl Pts',(-2.86668841021329,7.37396294596851,
132.267998293921));
#229572=CARTESIAN_POINT('Ctrl Pts',(-2.60328017229208,7.47268404788839,
132.255754521818));
#229573=CARTESIAN_POINT('Ctrl Pts',(-2.42801615920669,7.53145441302817,
132.247450145728));
#229574=CARTESIAN_POINT('Ctrl Pts',(-1.74424682103745,7.73439030001617,
132.21485060008));
#229575=CARTESIAN_POINT('Ctrl Pts',(-1.22383344923151,7.83361095620723,
132.189715163654));
#229576=CARTESIAN_POINT('Ctrl Pts',(-0.226539098790644,7.921871171148,132.144098731499));
#229577=CARTESIAN_POINT('Ctrl Pts',(0.247145662952985,7.92126144670701,
132.123490759275));
#229578=CARTESIAN_POINT('Ctrl Pts',(0.750324467869314,7.8754039834075,132.102930204537));
#229579=CARTESIAN_POINT('Ctrl Pts',(0.782633188062952,7.8722588902326,132.101615536776));
#229580=CARTESIAN_POINT('Ctrl Pts',(0.826759997879149,7.867689022179,132.099827361748));
#229581=CARTESIAN_POINT('Ctrl Pts',(0.838595356555082,7.86643632615018,
132.099348477133));
#229582=CARTESIAN_POINT('Ctrl Pts',(0.857344604591703,7.86440904514893,
132.098590982286));
#229583=CARTESIAN_POINT('Ctrl Pts',(0.864260353740726,7.86365204225786,
132.098311822802));
#229584=CARTESIAN_POINT('Ctrl Pts',(0.877650463942954,7.86216847365358,
132.097771794848));
#229585=CARTESIAN_POINT('Ctrl Pts',(0.884124942638113,7.86144303108823,
132.097510891505));
#229586=CARTESIAN_POINT('Ctrl Pts',(0.899510131258267,7.8596999281053,132.096891419214));
#229587=CARTESIAN_POINT('Ctrl Pts',(0.908420029922871,7.85867511009371,
132.096533074161));
#229588=CARTESIAN_POINT('Ctrl Pts',(0.934776141358874,7.85559820419946,
132.095474253243));
#229589=CARTESIAN_POINT('Ctrl Pts',(0.952217334701166,7.85350315036705,
132.09477511933));
#229590=CARTESIAN_POINT('Ctrl Pts',(1.08984254290069,7.83650626623499,132.089270371984));
#229591=CARTESIAN_POINT('Ctrl Pts',(1.2096797759489,7.8189042478654,132.08454966325));
#229592=CARTESIAN_POINT('Ctrl Pts',(1.64560612518417,7.74461150401348,132.067605100019));
#229593=CARTESIAN_POINT('Ctrl Pts',(1.95857765065799,7.67144187293376,132.055893933596));
#229594=CARTESIAN_POINT('Ctrl Pts',(2.85140327374869,7.40448746549866,132.022850996708));
#229595=CARTESIAN_POINT('Ctrl Pts',(3.4142831269127,7.1623684162658,132.002577571574));
#229596=CARTESIAN_POINT('Ctrl Pts',(4.13398663289207,6.74850145176339,131.972108594253));
#229597=CARTESIAN_POINT('Ctrl Pts',(4.31962790377202,6.63120862147032,131.963739602068));
#229598=CARTESIAN_POINT('Ctrl Pts',(4.51651536554941,6.49502922704184,131.954188071791));
#229599=CARTESIAN_POINT('Ctrl Pts',(4.53281228473271,6.48366628462464,131.953392696322));
#229600=CARTESIAN_POINT('Ctrl Pts',(4.55639436143299,6.46709143708528,131.9522349934));
#229601=CARTESIAN_POINT('Ctrl Pts',(4.56371381295691,6.46192830857818,131.951874711739));
#229602=CARTESIAN_POINT('Ctrl Pts',(4.57658980688718,6.45281281580426,131.951239263243));
#229603=CARTESIAN_POINT('Ctrl Pts',(4.58215004508853,6.448865672371,131.95096431078));
#229604=CARTESIAN_POINT('Ctrl Pts',(4.59360954550264,6.4407084136673,131.950396521291));
#229605=CARTESIAN_POINT('Ctrl Pts',(4.59950813854067,6.43649737120558,131.950103646945));
#229606=CARTESIAN_POINT('Ctrl Pts',(4.61435866019226,6.42586465233883,131.94936476027));
#229607=CARTESIAN_POINT('Ctrl Pts',(4.62330296340256,6.41943238007525,131.948918328128));
#229608=CARTESIAN_POINT('Ctrl Pts',(4.65814253861303,6.39426700917826,131.94717396696));
#229609=CARTESIAN_POINT('Ctrl Pts',(4.68393746444788,6.37539585388859,131.945870720368));
#229610=CARTESIAN_POINT('Ctrl Pts',(4.85909023635991,6.24562011416577,131.936944023274));
#229611=CARTESIAN_POINT('Ctrl Pts',(5.00460634244275,6.12963618916547,131.929143226832));
#229612=CARTESIAN_POINT('Ctrl Pts',(5.45341490891541,5.74526914859836,131.90406991572));
#229613=CARTESIAN_POINT('Ctrl Pts',(5.74026290325166,5.45868436433307,131.886523642141));
#229614=CARTESIAN_POINT('Ctrl Pts',(6.49147055438085,4.58315901219154,131.837112421992));
#229615=CARTESIAN_POINT('Ctrl Pts',(6.89590685858335,3.94855326766262,131.80610909589));
#229616=CARTESIAN_POINT('Ctrl Pts',(7.23579345135852,3.19886572087348,131.772648042261));
#229617=CARTESIAN_POINT('Ctrl Pts',(7.26553740029913,3.13072119171093,131.769635568221));
#229618=CARTESIAN_POINT('Ctrl Pts',(7.30481613030589,3.03715625033907,131.765538700701));
#229619=CARTESIAN_POINT('Ctrl Pts',(7.31518706292799,3.01209147061176,131.764445017148));
#229620=CARTESIAN_POINT('Ctrl Pts',(7.33267435491359,2.96920461489199,131.762580144618));
#229621=CARTESIAN_POINT('Ctrl Pts',(7.33985514392959,2.95140910562158,131.7618082234));
#229622=CARTESIAN_POINT('Ctrl Pts',(7.35443249590867,2.91490111676169,131.760228454238));
#229623=CARTESIAN_POINT('Ctrl Pts',(7.36182256156905,2.89618618739312,131.759420686857));
#229624=CARTESIAN_POINT('Ctrl Pts',(7.37853063235474,2.85339676567689,131.757578496812));
#229625=CARTESIAN_POINT('Ctrl Pts',(7.38780236925084,2.82930442929286,131.756544626275));
#229626=CARTESIAN_POINT('Ctrl Pts',(7.41591676594756,2.75516946705602,131.753373492314));
#229627=CARTESIAN_POINT('Ctrl Pts',(7.43437017387719,2.70498067291312,131.751240901248));
#229628=CARTESIAN_POINT('Ctrl Pts',(7.47592236043535,2.58833073156207,131.746316203503));
#229629=CARTESIAN_POINT('Ctrl Pts',(7.49864622569285,2.52174067108512,131.74352871091));
#229630=CARTESIAN_POINT('Ctrl Pts',(7.57285617297698,2.29439766118438,131.734088138855));
#229631=CARTESIAN_POINT('Ctrl Pts',(7.62008521338192,2.13230250028844,131.727486273193));
#229632=CARTESIAN_POINT('Ctrl Pts',(7.74578638703014,1.64310860448985,131.707863231883));
#229633=CARTESIAN_POINT('Ctrl Pts',(7.80862585530429,1.31239342305064,131.695005132221));
#229634=CARTESIAN_POINT('Ctrl Pts',(7.88874083073698,0.669774016502942,
131.67008307852));
#229635=CARTESIAN_POINT('Ctrl Pts',(7.90898404229305,0.358870257901192,
131.658048801793));
#229636=CARTESIAN_POINT('Ctrl Pts',(7.91100561999111,0.022863898115329,
131.644609063699));
#229637=CARTESIAN_POINT('Ctrl Pts',(7.9110384389916,-0.00186825295649431,
131.643617217254));
#229638=CARTESIAN_POINT('Ctrl Pts',(7.910913695667,-0.0389672512191592,
131.642125210408));
#229639=CARTESIAN_POINT('Ctrl Pts',(7.91084311209925,-0.0513342124840412,
131.641627160103));
#229640=CARTESIAN_POINT('Ctrl Pts',(7.91066228089055,-0.0737908597183481,
131.640721552485));
#229641=CARTESIAN_POINT('Ctrl Pts',(7.91056172824003,-0.0838806072956481,
131.640314217099));
#229642=CARTESIAN_POINT('Ctrl Pts',(7.91031217804911,-0.104887841697685,
131.639465219423));
#229643=CARTESIAN_POINT('Ctrl Pts',(7.91015988163277,-0.115805266141546,
131.63902348495));
#229644=CARTESIAN_POINT('Ctrl Pts',(7.90968103930422,-0.145694520238988,
131.63781275561));
#229645=CARTESIAN_POINT('Ctrl Pts',(7.90930883850215,-0.164665508150562,
131.637042785688));
#229646=CARTESIAN_POINT('Ctrl Pts',(7.9083313712687,-0.206763492154223,
131.635330959316));
#229647=CARTESIAN_POINT('Ctrl Pts',(7.90769290117543,-0.229889522892169,
131.634388438799));
#229648=CARTESIAN_POINT('Ctrl Pts',(7.90544734029276,-0.300066117807757,
131.631522152174));
#229649=CARTESIAN_POINT('Ctrl Pts',(7.90352169791984,-0.347105228659188,
131.629592458698));
#229650=CARTESIAN_POINT('Ctrl Pts',(7.89473012600363,-0.523353701474114,
131.622333982576));
#229651=CARTESIAN_POINT('Ctrl Pts',(7.88511450197023,-0.652404277715379,
131.616962635147));
#229652=CARTESIAN_POINT('Ctrl Pts',(7.82961522751308,-1.21171291406717,
131.593509734169));
#229653=CARTESIAN_POINT('Ctrl Pts',(7.75164243637642,-1.63803824784402,
131.575222896025));
#229654=CARTESIAN_POINT('Ctrl Pts',(7.60537040176252,-2.18156141667359,
131.551801021626));
#229655=CARTESIAN_POINT('Ctrl Pts',(7.56844065687543,-2.30642056003329,
131.546409455486));
#229656=CARTESIAN_POINT('Ctrl Pts',(7.4751336948425,-2.59546011176246,131.533902623202));
#229657=CARTESIAN_POINT('Ctrl Pts',(7.41640084691425,-2.75881081020412,
131.526815085619));
#229658=CARTESIAN_POINT('Ctrl Pts',(7.33517263694406,-2.96333040274327,
131.51790203419));
#229659=CARTESIAN_POINT('Ctrl Pts',(7.317621882762,-3.00640893796247,131.516022327462));
#229660=CARTESIAN_POINT('Ctrl Pts',(7.28917046476299,-3.07451785698646,
131.51304612913));
#229661=CARTESIAN_POINT('Ctrl Pts',(7.27851846164613,-3.09965080727473,
131.511946939756));
#229662=CARTESIAN_POINT('Ctrl Pts',(7.25828736265001,-3.14670587568004,
131.509887057419));
#229663=CARTESIAN_POINT('Ctrl Pts',(7.24873849711079,-3.16864064094754,
131.508926049696));
#229664=CARTESIAN_POINT('Ctrl Pts',(7.22712193644164,-3.21768708336256,
131.506775303689));
#229665=CARTESIAN_POINT('Ctrl Pts',(7.21500087931375,-3.24477487196806,
131.505586150802));
#229666=CARTESIAN_POINT('Ctrl Pts',(7.17910225894761,-3.32380429619657,
131.502112507688));
#229667=CARTESIAN_POINT('Ctrl Pts',(7.15491410946176,-3.37555749187765,
131.499832363477));
#229668=CARTESIAN_POINT('Ctrl Pts',(7.09718637547597,-3.49566343932966,
131.494525656358));
#229669=CARTESIAN_POINT('Ctrl Pts',(7.06321631101485,-3.56380313401105,
131.491503479813));
#229670=CARTESIAN_POINT('Ctrl Pts',(6.94248366995176,-3.79746824550364,
131.481089900985));
#229671=CARTESIAN_POINT('Ctrl Pts',(6.85084169358579,-3.96040583485297,
131.47373081443));
#229672=CARTESIAN_POINT('Ctrl Pts',(6.2677679034555,-4.91619466639724,131.429982353456));
#229673=CARTESIAN_POINT('Ctrl Pts',(5.64508723852377,-5.62019479616323,
131.396777274658));
#229674=CARTESIAN_POINT('Ctrl Pts',(4.89693951136714,-6.21324342706174,
131.360168149402));
#229675=CARTESIAN_POINT('Ctrl Pts',(4.87954456824737,-6.22691378302315,
131.359317751109));
#229676=CARTESIAN_POINT('Ctrl Pts',(4.84028492855138,-6.25750166349224,
131.357399750589));
#229677=CARTESIAN_POINT('Ctrl Pts',(4.81838847758797,-6.27437787527741,
131.356330923647));
#229678=CARTESIAN_POINT('Ctrl Pts',(4.71688998157077,-6.35176097156591,
131.351378805897));
#229679=CARTESIAN_POINT('Ctrl Pts',(4.63623539545467,-6.41086881593325,
131.347450287076));
#229680=CARTESIAN_POINT('Ctrl Pts',(4.54164443685752,-6.47747121965408,
131.342827264503));
#229681=CARTESIAN_POINT('Ctrl Pts',(4.52877783052257,-6.48647353727907,
131.342198091247));
#229682=CARTESIAN_POINT('Ctrl Pts',(4.50944011063742,-6.49991788362271,
131.341251862765));
#229683=CARTESIAN_POINT('Ctrl Pts',(4.50298900946952,-6.50438871726726,
131.340936096072));
#229684=CARTESIAN_POINT('Ctrl Pts',(4.49151488482207,-6.51231542642754,
131.34037426288));
#229685=CARTESIAN_POINT('Ctrl Pts',(4.48649449395881,-6.51577511346732,
131.340128370093));
#229686=CARTESIAN_POINT('Ctrl Pts',(4.47594576456272,-6.52302655618528,
131.339611552756));
#229687=CARTESIAN_POINT('Ctrl Pts',(4.47041659772165,-6.52681709430147,
131.339340572405));
#229688=CARTESIAN_POINT('Ctrl Pts',(4.45921723363772,-6.53447394690843,
131.338791508869));
#229689=CARTESIAN_POINT('Ctrl Pts',(4.45354681055171,-6.53833991969169,
131.33851341008));
#229690=CARTESIAN_POINT('Ctrl Pts',(4.43005013245647,-6.55431470277271,
131.337360607571));
#229691=CARTESIAN_POINT('Ctrl Pts',(4.41217957483781,-6.56635795444614,
131.336482795221));
#229692=CARTESIAN_POINT('Ctrl Pts',(4.36951433603597,-6.59485792588513,
131.334384070834));
#229693=CARTESIAN_POINT('Ctrl Pts',(4.34467568579787,-6.61124797185816,
131.333159863127));
#229694=CARTESIAN_POINT('Ctrl Pts',(4.25661271117346,-6.66864665671793,
131.32880914566));
#229695=CARTESIAN_POINT('Ctrl Pts',(4.19289993568851,-6.7088888044265,131.325640303226));
#229696=CARTESIAN_POINT('Ctrl Pts',(4.03027579555711,-6.80838386128025,
131.317508945766));
#229697=CARTESIAN_POINT('Ctrl Pts',(3.93062737874045,-6.86639500934533,
131.312488969125));
#229698=CARTESIAN_POINT('Ctrl Pts',(3.53662037802923,-7.0843816600019,131.29258696103));
#229699=CARTESIAN_POINT('Ctrl Pts',(3.23349542915775,-7.22776855108928,
131.277172752162));
#229700=CARTESIAN_POINT('Ctrl Pts',(2.67834396708993,-7.44844018590403,
131.24964654932));
#229701=CARTESIAN_POINT('Ctrl Pts',(2.42980142330698,-7.53318382762938,
131.237557371073));
#229702=CARTESIAN_POINT('Ctrl Pts',(1.71404280037865,-7.73811223118917,
131.203853927677));
#229703=CARTESIAN_POINT('Ctrl Pts',(1.23938359919552,-7.82817675642457,
131.182867223469));
#229704=CARTESIAN_POINT('Ctrl Pts',(0.727460526266421,-7.87754742711526,
131.161929216356));
#229705=CARTESIAN_POINT('Ctrl Pts',(0.695476526050218,-7.8804355663749,
131.16062764941));
#229706=CARTESIAN_POINT('Ctrl Pts',(0.651402085719223,-7.88414504716499,
131.158843038747));
#229707=CARTESIAN_POINT('Ctrl Pts',(0.639326232371146,-7.88513346572133,
131.158355003629));
#229708=CARTESIAN_POINT('Ctrl Pts',(0.620090460192549,-7.88666345024435,
131.157579072929));
#229709=CARTESIAN_POINT('Ctrl Pts',(0.612932014899007,-7.88722301584542,
131.157290639534));
#229710=CARTESIAN_POINT('Ctrl Pts',(0.599004739605401,-7.88829261620159,
131.156730097936));
#229711=CARTESIAN_POINT('Ctrl Pts',(0.592235995971775,-7.88880368638161,
131.156457958983));
#229712=CARTESIAN_POINT('Ctrl Pts',(0.576046652408271,-7.89000510001128,
131.155807748297));
#229713=CARTESIAN_POINT('Ctrl Pts',(0.566625448200215,-7.89068728477801,
131.155429920772));
#229714=CARTESIAN_POINT('Ctrl Pts',(0.538383010215264,-7.89268146406173,
131.154298942482));
#229715=CARTESIAN_POINT('Ctrl Pts',(0.519558223772725,-7.89394300821675,
131.153547300121));
#229716=CARTESIAN_POINT('Ctrl Pts',(0.355731484426099,-7.904333303052,131.147024913684));
#229717=CARTESIAN_POINT('Ctrl Pts',(0.210504213934108,-7.90953351565325,
131.141372785188));
#229718=CARTESIAN_POINT('Ctrl Pts',(-0.31897172246396,-7.91389819751642,
131.121178961891));
#229719=CARTESIAN_POINT('Ctrl Pts',(-0.702890991865361,-7.88907481284543,
131.10735565344));
#229720=CARTESIAN_POINT('Ctrl Pts',(-1.38764628191403,-7.7943973045146,
131.083146187415));
#229721=CARTESIAN_POINT('Ctrl Pts',(-1.68908339619839,-7.73467446966547,
131.072638801583));
#229722=CARTESIAN_POINT('Ctrl Pts',(-2.11774384123277,-7.62348519771749,
131.057266002313));
#229723=CARTESIAN_POINT('Ctrl Pts',(-2.24830252227199,-7.58600687782166,
131.052522953512));
#229724=CARTESIAN_POINT('Ctrl Pts',(-2.59016459989613,-7.47827066918614,
131.039821436862));
#229725=CARTESIAN_POINT('Ctrl Pts',(-2.79957066622585,-7.40242391479314,
131.03175211285));
#229726=CARTESIAN_POINT('Ctrl Pts',(-3.11860071292908,-7.27139622176705,
131.018671875407));
#229727=CARTESIAN_POINT('Ctrl Pts',(-3.23061831025314,-7.22232502982957,
131.013921305264));
#229728=CARTESIAN_POINT('Ctrl Pts',(-3.35308793643955,-7.16525554224267,
131.00851748926));
#229729=CARTESIAN_POINT('Ctrl Pts',(-3.36470707218285,-7.15980670204315,
131.008002786386));
#229730=CARTESIAN_POINT('Ctrl Pts',(-3.38223554820827,-7.15153456170686,
131.007223311176));
#229731=CARTESIAN_POINT('Ctrl Pts',(-3.388154764195,-7.14873213824349,131.006959570978));
#229732=CARTESIAN_POINT('Ctrl Pts',(-3.39842135530475,-7.14385585607813,
131.006501235615));
#229733=CARTESIAN_POINT('Ctrl Pts',(-3.40277033442436,-7.14178536863234,
131.006306804637));
#229734=CARTESIAN_POINT('Ctrl Pts',(-3.41181567168698,-7.13746887368505,
131.005901838137));
#229735=CARTESIAN_POINT('Ctrl Pts',(-3.41651170892208,-7.13522219997365,
131.005691270577));
#229736=CARTESIAN_POINT('Ctrl Pts',(-3.42756238649814,-7.12992193453942,
131.005195011086));
#229737=CARTESIAN_POINT('Ctrl Pts',(-3.43391516303344,-7.12686448296829,
131.004909135728));
#229738=CARTESIAN_POINT('Ctrl Pts',(-3.44727899788268,-7.12041074661861,
131.0043065383));
#229739=CARTESIAN_POINT('Ctrl Pts',(-3.45428914101289,-7.11701259093155,
131.003989728918));
#229740=CARTESIAN_POINT('Ctrl Pts',(-3.50648886076114,-7.09161356862683,
131.001625432121));
#229741=CARTESIAN_POINT('Ctrl Pts',(-3.5514722307191,-7.06919316327819,
130.999558731628));
#229742=CARTESIAN_POINT('Ctrl Pts',(-3.68354154049401,-7.00178905092022,
130.993410785228));
#229743=CARTESIAN_POINT('Ctrl Pts',(-3.77000729171713,-6.95561444443585,
130.989281923224));
#229744=CARTESIAN_POINT('Ctrl Pts',(-4.08237750706112,-6.78126609055553,
130.974039262031));
#229745=CARTESIAN_POINT('Ctrl Pts',(-4.30278790584083,-6.64359731019736,
130.962655395159));
#229746=CARTESIAN_POINT('Ctrl Pts',(-4.71324885921859,-6.35821583549561,
130.940654172516));
#229747=CARTESIAN_POINT('Ctrl Pts',(-4.90413092883447,-6.2121756077295,
130.930054152948));
#229748=CARTESIAN_POINT('Ctrl Pts',(-5.46153231658274,-5.74399289965348,
130.898286643073));
#229749=CARTESIAN_POINT('Ctrl Pts',(-5.80520533106435,-5.39642930886564,
130.877632599852));
#229750=CARTESIAN_POINT('Ctrl Pts',(-6.13907950793423,-4.9896994243265,
130.856316269144));
#229751=CARTESIAN_POINT('Ctrl Pts',(-6.16324351830985,-4.95982125840603,
130.854764859031));
#229752=CARTESIAN_POINT('Ctrl Pts',(-6.19685941828311,-4.91763105303388,
130.8525938834));
#229753=CARTESIAN_POINT('Ctrl Pts',(-6.20649411136275,-4.90546559170052,
130.851970165368));
#229754=CARTESIAN_POINT('Ctrl Pts',(-6.22410847384288,-4.88308945597198,
130.85082707706));
#229755=CARTESIAN_POINT('Ctrl Pts',(-6.23209896415351,-4.8728873813514,
130.850307466962));
#229756=CARTESIAN_POINT('Ctrl Pts',(-6.24825321342879,-4.8521572795058,
130.849254781945));
#229757=CARTESIAN_POINT('Ctrl Pts',(-6.25641551858542,-4.84162817079275,
130.848721739929));
#229758=CARTESIAN_POINT('Ctrl Pts',(-6.27274840236682,-4.82044901023082,
130.847652768087));
#229759=CARTESIAN_POINT('Ctrl Pts',(-6.28091854977015,-4.80979868102738,
130.847116848675));
#229760=CARTESIAN_POINT('Ctrl Pts',(-6.30041873004687,-4.78424448769462,
130.845834833276));
#229761=CARTESIAN_POINT('Ctrl Pts',(-6.31172305385114,-4.769321082365,130.845089277373));
#229762=CARTESIAN_POINT('Ctrl Pts',(-6.3842234420301,-4.67290046656368,
130.840291995193));
#229763=CARTESIAN_POINT('Ctrl Pts',(-6.44389362357367,-4.59026614137918,
130.836271200349));
#229764=CARTESIAN_POINT('Ctrl Pts',(-6.67740422913668,-4.25335851368372,
130.820228282927));
#229765=CARTESIAN_POINT('Ctrl Pts',(-6.83792819962555,-3.99017991628767,
130.808492775632));
#229766=CARTESIAN_POINT('Ctrl Pts',(-7.0294306256028,-3.63055226294356,
130.793249472181));
#229767=CARTESIAN_POINT('Ctrl Pts',(-7.07450010450672,-3.54192789263511,
130.78955221141));
#229768=CARTESIAN_POINT('Ctrl Pts',(-7.16640534116194,-3.35244911203576,
130.781752297394));
#229769=CARTESIAN_POINT('Ctrl Pts',(-7.21280939127133,-3.25140914994615,
130.777654321761));
#229770=CARTESIAN_POINT('Ctrl Pts',(-7.45709445231892,-2.68851471465759,
130.755075806522));
#229771=CARTESIAN_POINT('Ctrl Pts',(-7.61274357434249,-2.20962509032041,
130.736853953726));
#229772=CARTESIAN_POINT('Ctrl Pts',(-7.73822630616955,-1.64602622079661,
130.71425593118));
#229773=CARTESIAN_POINT('Ctrl Pts',(-7.7534868193402,-1.5725744502583,130.711287581794));
#229774=CARTESIAN_POINT('Ctrl Pts',(-7.77012955626127,-1.48632839059519,
130.707765944901));
#229775=CARTESIAN_POINT('Ctrl Pts',(-7.77252836955353,-1.4737327260642,
130.707250730951));
#229776=CARTESIAN_POINT('Ctrl Pts',(-7.77631643710953,-1.45357585672041,
130.70642472723));
#229777=CARTESIAN_POINT('Ctrl Pts',(-7.77772531533506,-1.44601833320615,
130.706114690963));
#229778=CARTESIAN_POINT('Ctrl Pts',(-7.78019852367665,-1.43264332898656,
130.705565387729));
#229779=CARTESIAN_POINT('Ctrl Pts',(-7.78126735200993,-1.42682667910636,
130.705326296364));
#229780=CARTESIAN_POINT('Ctrl Pts',(-7.78346957776464,-1.41476591900512,
130.704830109819));
#229781=CARTESIAN_POINT('Ctrl Pts',(-7.78460198593676,-1.40852163412866,
130.704572975809));
#229782=CARTESIAN_POINT('Ctrl Pts',(-7.78687076068286,-1.39592492673905,
130.704053759958));
#229783=CARTESIAN_POINT('Ctrl Pts',(-7.78800687040367,-1.38957246334485,
130.703791668081));
#229784=CARTESIAN_POINT('Ctrl Pts',(-7.79075785756785,-1.37408119500227,
130.703151893961));
#229785=CARTESIAN_POINT('Ctrl Pts',(-7.79236442671566,-1.36494093863996,
130.702773875558));
#229786=CARTESIAN_POINT('Ctrl Pts',(-7.79669698786827,-1.34003472941215,
130.701742318702));
#229787=CARTESIAN_POINT('Ctrl Pts',(-7.79939123011584,-1.32426335409457,
130.701087471629));
#229788=CARTESIAN_POINT('Ctrl Pts',(-7.87423464476727,-0.877997953164491,
130.682509602445));
#229789=CARTESIAN_POINT('Ctrl Pts',(-7.91066124806279,-0.442382604334897,
130.662818762618));
#229790=CARTESIAN_POINT('Ctrl Pts',(-7.91099764832253,-0.00609985535713557,
130.642792890452));
#229791=CARTESIAN_POINT('',(-7.91099997694602,-0.000603953663847722,128.642331508237));
#229792=CARTESIAN_POINT('Ctrl Pts',(-7.91099763196637,-0.00612103116663704,
130.642331508237));
#229793=CARTESIAN_POINT('Ctrl Pts',(-7.91114782317046,0.18799042285764,
130.634504138835));
#229794=CARTESIAN_POINT('Ctrl Pts',(-7.90414951540968,0.382321771707403,
130.626676769434));
#229795=CARTESIAN_POINT('Ctrl Pts',(-7.88998090783303,0.576300506706553,
130.618849400032));
#229796=CARTESIAN_POINT('Ctrl Pts',(-7.87582335202878,0.770127934753637,
130.611028136121));
#229797=CARTESIAN_POINT('Ctrl Pts',(-7.85450666116262,0.963602947557249,
130.60320687221));
#229798=CARTESIAN_POINT('Ctrl Pts',(-7.82606108445803,1.15615262934077,
130.5953856083));
#229799=CARTESIAN_POINT('Ctrl Pts',(-7.79763215742691,1.34858960856388,
130.587568922306));
#229800=CARTESIAN_POINT('Ctrl Pts',(-7.7620827075776,1.54010198851846,130.579752236312));
#229801=CARTESIAN_POINT('Ctrl Pts',(-7.71949486697746,1.73012138265169,
130.571935550318));
#229802=CARTESIAN_POINT('Ctrl Pts',(-7.67692366416245,1.92006654193748,
130.564121918068));
#229803=CARTESIAN_POINT('Ctrl Pts',(-7.62731962579182,2.10851953455246,
130.556308285818));
#229804=CARTESIAN_POINT('Ctrl Pts',(-7.57081612274288,2.29492140074916,
130.548494653568));
#229805=CARTESIAN_POINT('Ctrl Pts',(-7.51431398949648,2.48131874804463,
130.540681210742));
#229806=CARTESIAN_POINT('Ctrl Pts',(-7.45091281772856,2.66566472846678,
130.532867767916));
#229807=CARTESIAN_POINT('Ctrl Pts',(-7.38079620123127,2.84741434215151,
130.52505432509));
#229808=CARTESIAN_POINT('Ctrl Pts',(-7.31067703841428,3.02917055616359,
130.517240598515));
#229809=CARTESIAN_POINT('Ctrl Pts',(-7.23384207105125,3.20832988672088,
130.50942687194));
#229810=CARTESIAN_POINT('Ctrl Pts',(-7.15052350236325,3.38436620981696,
130.501613145365));
#229811=CARTESIAN_POINT('Ctrl Pts',(-7.0671872167759,3.56043996535899,130.493797757275));
#229812=CARTESIAN_POINT('Ctrl Pts',(-6.97736473405849,3.73338907226283,
130.485982369186));
#229813=CARTESIAN_POINT('Ctrl Pts',(-6.88133484139416,3.90271082718343,
130.478166981096));
#229814=CARTESIAN_POINT('Ctrl Pts',(-6.78526759506394,4.07209844480666,
130.47034855298));
#229815=CARTESIAN_POINT('Ctrl Pts',(-6.6829883026622,4.23785559386953,130.462530124865));
#229816=CARTESIAN_POINT('Ctrl Pts',(-6.57481987435693,4.39950731557082,
130.454711696749));
#229817=CARTESIAN_POINT('Ctrl Pts',(-6.46653145304692,4.56133836016801,
130.446884595523));
#229818=CARTESIAN_POINT('Ctrl Pts',(-6.35234104332711,4.71905458844504,
130.439057494297));
#229819=CARTESIAN_POINT('Ctrl Pts',(-6.23261341089965,4.87221213313561,
130.431230393072));
#229820=CARTESIAN_POINT('Ctrl Pts',(-6.11281218343387,5.02546382180232,
130.423398480627));
#229821=CARTESIAN_POINT('Ctrl Pts',(-5.98746717643063,5.17415097421666,
130.415566568183));
#229822=CARTESIAN_POINT('Ctrl Pts',(-5.85698107581138,5.31786551894531,
130.407734655738));
#229823=CARTESIAN_POINT('Ctrl Pts',(-5.72631141641576,5.46178223130598,
130.399891725904));
#229824=CARTESIAN_POINT('Ctrl Pts',(-5.59048646306852,5.60071211292389,
130.392048796069));
#229825=CARTESIAN_POINT('Ctrl Pts',(-5.44994399259742,5.73428561178734,
130.384205866235));
#229826=CARTESIAN_POINT('Ctrl Pts',(-5.36622686938654,5.81385151826796,
130.379534057627));
#229827=CARTESIAN_POINT('Ctrl Pts',(-5.28083647453102,5.89151763492538,
130.37486224902));
#229828=CARTESIAN_POINT('Ctrl Pts',(-5.19387032345218,5.96721309014206,
130.370190440412));
#229829=CARTESIAN_POINT('Ctrl Pts',(-5.04941193573323,6.09294986568753,
130.362430157465));
#229830=CARTESIAN_POINT('Ctrl Pts',(-4.90013023472339,6.21365931778303,
130.354669874518));
#229831=CARTESIAN_POINT('Ctrl Pts',(-4.74641559371106,6.32893830051901,
130.346909591571));
#229832=CARTESIAN_POINT('Ctrl Pts',(-4.59288595595854,6.44407853923261,
130.339158648512));
#229833=CARTESIAN_POINT('Ctrl Pts',(-4.43493428100679,6.55380110512324,
130.331407705454));
#229834=CARTESIAN_POINT('Ctrl Pts',(-4.27298750711932,6.65773976391405,
130.323656762396));
#229835=CARTESIAN_POINT('Ctrl Pts',(-4.11120277393074,6.76157442376429,
130.315913574776));
#229836=CARTESIAN_POINT('Ctrl Pts',(-3.94543119870691,6.85963650494034,
130.308170387156));
#229837=CARTESIAN_POINT('Ctrl Pts',(-3.77613257696021,6.9516000863988,130.300427199536));
#229838=CARTESIAN_POINT('Ctrl Pts',(-3.60696903974555,7.04349028948455,
130.292690190258));
#229839=CARTESIAN_POINT('Ctrl Pts',(-3.43428437265227,7.1292915105122,130.284953180981));
#229840=CARTESIAN_POINT('Ctrl Pts',(-3.25856720076424,7.20872116246034,
130.277216171703));
#229841=CARTESIAN_POINT('Ctrl Pts',(-3.08295465862199,7.28810351849424,
130.269483769382));
#229842=CARTESIAN_POINT('Ctrl Pts',(-2.90431353333025,7.36112171272404,
130.261751367061));
#229843=CARTESIAN_POINT('Ctrl Pts',(-2.72315697160088,7.42753910174975,
130.25401896474));
#229844=CARTESIAN_POINT('Ctrl Pts',(-2.54207162691524,7.49393038048692,
130.246289602214));
#229845=CARTESIAN_POINT('Ctrl Pts',(-2.35847315188261,7.55372589889675,
130.238560239688));
#229846=CARTESIAN_POINT('Ctrl Pts',(-2.17289466916262,7.60673712946127,
130.230830877161));
#229847=CARTESIAN_POINT('Ctrl Pts',(-1.98731625884801,7.65974833934291,
130.223101517651));
#229848=CARTESIAN_POINT('Ctrl Pts',(-1.79975818442748,7.70597515703875,
130.215372158141));
#229849=CARTESIAN_POINT('Ctrl Pts',(-1.61076912072071,7.74527880968353,
130.20764279863));
#229850=CARTESIAN_POINT('Ctrl Pts',(-1.42177058420322,7.78458443236855,
130.199913051696));
#229851=CARTESIAN_POINT('Ctrl Pts',(-1.23134126718937,7.8169661248216,130.192183304763));
#229852=CARTESIAN_POINT('Ctrl Pts',(-1.04004026967997,7.84233621043143,
130.184453557829));
#229853=CARTESIAN_POINT('Ctrl Pts',(-0.84869463012058,7.86771221641097,
130.17672200708));
#229854=CARTESIAN_POINT('Ctrl Pts',(-0.656477261096092,7.88607330984533,
130.16899045633));
#229855=CARTESIAN_POINT('Ctrl Pts',(-0.463952669895659,7.89738367562933,
130.161258905581));
#229856=CARTESIAN_POINT('Ctrl Pts',(-0.271347862168685,7.90869875394513,
130.153524133434));
#229857=CARTESIAN_POINT('Ctrl Pts',(-0.0784359355669855,7.91295723374037,
130.145789361288));
#229858=CARTESIAN_POINT('Ctrl Pts',(0.11421826373655,7.91017542082532,130.138054589142));
#229859=CARTESIAN_POINT('Ctrl Pts',(0.30710220327139,7.90739029059694,130.130310593275));
#229860=CARTESIAN_POINT('Ctrl Pts',(0.499727442556436,7.89754810592534,
130.122566597409));
#229861=CARTESIAN_POINT('Ctrl Pts',(0.691532870580185,7.8807171811268,130.114822601543));
#229862=CARTESIAN_POINT('Ctrl Pts',(0.883462789948739,7.86387533221373,
130.107073579435));
#229863=CARTESIAN_POINT('Ctrl Pts',(1.07457148325651,7.84003575197567,130.099324557327));
#229864=CARTESIAN_POINT('Ctrl Pts',(1.26430782929928,7.80931794158572,130.091575535219));
#229865=CARTESIAN_POINT('Ctrl Pts',(1.45433413717369,7.7785531871455,130.08381467078));
#229866=CARTESIAN_POINT('Ctrl Pts',(1.6429835585206,7.74088927881033,130.076053806341));
#229867=CARTESIAN_POINT('Ctrl Pts',(1.82971875817401,7.69649597323263,130.068292941902));
#229868=CARTESIAN_POINT('Ctrl Pts',(1.9581349004912,7.66596709031406,130.062955864189));
#229869=CARTESIAN_POINT('Ctrl Pts',(2.08564611180101,7.6322567852051,130.057618786476));
#229870=CARTESIAN_POINT('Ctrl Pts',(2.21208335260762,7.59543338073057,130.052281708762));
#229871=CARTESIAN_POINT('Ctrl Pts',(2.40193308980169,7.54014180984939,130.044267908439));
#229872=CARTESIAN_POINT('Ctrl Pts',(2.58994300467057,7.4776598214353,130.036254108116));
#229873=CARTESIAN_POINT('Ctrl Pts',(2.77553686750707,7.40812500549964,130.028240307793));
#229874=CARTESIAN_POINT('Ctrl Pts',(2.96091917524786,7.3386694510461,130.020235642257));
#229875=CARTESIAN_POINT('Ctrl Pts',(3.14389060797537,7.26217720475818,130.01223097672));
#229876=CARTESIAN_POINT('Ctrl Pts',(3.32388829368905,7.17883609027793,130.004226311184));
#229877=CARTESIAN_POINT('Ctrl Pts',(3.50371136086772,7.09557582630005,129.996229411097));
#229878=CARTESIAN_POINT('Ctrl Pts',(3.680566128368,7.00548007450622,129.98823251101));
#229879=CARTESIAN_POINT('Ctrl Pts',(3.85390758861673,6.90878551544353,129.980235610923));
#229880=CARTESIAN_POINT('Ctrl Pts',(4.02711029629211,6.81216835632244,129.972245112019));
#229881=CARTESIAN_POINT('Ctrl Pts',(4.19680501077975,6.70896307964677,129.964254613116));
#229882=CARTESIAN_POINT('Ctrl Pts',(4.36246894971703,6.59945343666843,129.956264114212));
#229883=CARTESIAN_POINT('Ctrl Pts',(4.52802837277728,6.49001288233095,129.948278656442));
#229884=CARTESIAN_POINT('Ctrl Pts',(4.68956181093357,6.37427607378451,129.940293198671));
#229885=CARTESIAN_POINT('Ctrl Pts',(4.84657288472726,6.25257165277028,129.932307740901));
#229886=CARTESIAN_POINT('Ctrl Pts',(5.00873197596496,6.12687683498176,129.924060459076));
#229887=CARTESIAN_POINT('Ctrl Pts',(5.16606679754621,5.99481661610349,129.915813177252));
#229888=CARTESIAN_POINT('Ctrl Pts',(5.31806385291161,5.85680099169802,129.907565895427));
#229889=CARTESIAN_POINT('Ctrl Pts',(5.46513583305697,5.72325741005749,129.899585845644));
#229890=CARTESIAN_POINT('Ctrl Pts',(5.6072102771621,5.58413855917991,129.891605795861));
#229891=CARTESIAN_POINT('Ctrl Pts',(5.74385632493325,5.43985620384623,129.883625746077));
#229892=CARTESIAN_POINT('Ctrl Pts',(5.88049152130627,5.29558530632861,129.875646330009));
#229893=CARTESIAN_POINT('Ctrl Pts',(6.01169895042716,5.14615196445618,129.867666913941));
#229894=CARTESIAN_POINT('Ctrl Pts',(6.13708532179537,4.99200408182965,129.859687497873));
#229895=CARTESIAN_POINT('Ctrl Pts',(6.26248100585716,4.83784475033526,129.851707489158));
#229896=CARTESIAN_POINT('Ctrl Pts',(6.38205455954969,4.67897043992738,129.843727480443));
#229897=CARTESIAN_POINT('Ctrl Pts',(6.49545339007537,4.51586162956289,129.835747471728));
#229898=CARTESIAN_POINT('Ctrl Pts',(6.60887807083673,4.35271563714662,129.827765643901));
#229899=CARTESIAN_POINT('Ctrl Pts',(6.71612503229753,4.18533349565868,129.819783816075));
#229900=CARTESIAN_POINT('Ctrl Pts',(6.81688516144929,4.01422442018537,129.811801988248));
#229901=CARTESIAN_POINT('Ctrl Pts',(6.91772021028737,3.84298811742116,129.803814225574));
#229902=CARTESIAN_POINT('Ctrl Pts',(7.01205862217755,3.66801963360344,129.7958264629));
#229903=CARTESIAN_POINT('Ctrl Pts',(7.09963689854132,3.48985342226155,129.787838700225));
#229904=CARTESIAN_POINT('Ctrl Pts',(7.18725374749185,3.31160874018547,129.779847419456));
#229905=CARTESIAN_POINT('Ctrl Pts',(7.26810438443607,3.13016382595912,129.771856138687));
#229906=CARTESIAN_POINT('Ctrl Pts',(7.34197335188398,2.94607336979675,129.763864857918));
#229907=CARTESIAN_POINT('Ctrl Pts',(7.41591182020932,2.76180970899007,129.755866058416));
#229908=CARTESIAN_POINT('Ctrl Pts',(7.48285538381998,2.57489584831195,129.747867258915));
#229909=CARTESIAN_POINT('Ctrl Pts',(7.54263804339973,2.38590283671803,129.739868459413));
#229910=CARTESIAN_POINT('Ctrl Pts',(7.55632903738414,2.34262101882939,129.738036631979));
#229911=CARTESIAN_POINT('Ctrl Pts',(7.56964467461467,2.29923020566681,129.736204804546));
#229912=CARTESIAN_POINT('Ctrl Pts',(7.58258333712301,2.25573733745409,129.734372977112));
#229913=CARTESIAN_POINT('Ctrl Pts',(7.63998395193699,2.06278714852815,129.72624632408));
#229914=CARTESIAN_POINT('Ctrl Pts',(7.69006241361648,1.86748726185573,129.718119671047));
#229915=CARTESIAN_POINT('Ctrl Pts',(7.73263321854928,1.67042045826439,129.709993018014));
#229916=CARTESIAN_POINT('Ctrl Pts',(7.77516778530392,1.47352140677331,129.701873282753));
#229917=CARTESIAN_POINT('Ctrl Pts',(7.81020736932014,1.27485874716274,129.693753547492));
#229918=CARTESIAN_POINT('Ctrl Pts',(7.83761650697373,1.07502952964691,129.685633812231));
#229919=CARTESIAN_POINT('Ctrl Pts',(7.8650057643388,0.875345251477647,129.677519966344));
#229920=CARTESIAN_POINT('Ctrl Pts',(7.88477556718692,0.674496417318688,
129.669406120458));
#229921=CARTESIAN_POINT('Ctrl Pts',(7.89684157865705,0.473089929710325,
129.661292274571));
#229922=CARTESIAN_POINT('Ctrl Pts',(7.90889901677679,0.27182654890996,129.653184193874));
#229923=CARTESIAN_POINT('Ctrl Pts',(7.91326356495437,0.0700066226631564,
129.645076113177));
#229924=CARTESIAN_POINT('Ctrl Pts',(7.90990271011032,-0.131757795175419,
129.63696803248));
#229925=CARTESIAN_POINT('Ctrl Pts',(7.90654329877035,-0.333435554179994,
129.628863434245));
#229926=CARTESIAN_POINT('Ctrl Pts',(7.89546510567637,-0.535057534099425,
129.62075883601));
#229927=CARTESIAN_POINT('Ctrl Pts',(7.8766877001253,-0.736010784360424,
129.612654237774));
#229928=CARTESIAN_POINT('Ctrl Pts',(7.85791616384324,-0.936901222499596,
129.604552172799));
#229929=CARTESIAN_POINT('Ctrl Pts',(7.83145024429911,-1.13712303074794,
129.596450107825));
#229930=CARTESIAN_POINT('Ctrl Pts',(7.79736148799388,-1.33606692405356,
129.58834804285));
#229931=CARTESIAN_POINT('Ctrl Pts',(7.77922832305013,-1.44189309147248,
129.584038232329));
#229932=CARTESIAN_POINT('Ctrl Pts',(7.75893907923601,-1.54735774143948,
129.579728421809));
#229933=CARTESIAN_POINT('Ctrl Pts',(7.73651047970317,-1.6523699941124,129.575418611288));
#229934=CARTESIAN_POINT('Ctrl Pts',(7.69337535876219,-1.85433161069477,
129.567129899468));
#229935=CARTESIAN_POINT('Ctrl Pts',(7.64234282627787,-2.05453237315838,
129.558841187648));
#229936=CARTESIAN_POINT('Ctrl Pts',(7.58358851097656,-2.25235572150234,
129.550552475828));
#229937=CARTESIAN_POINT('Ctrl Pts',(7.52480032438705,-2.45029311307207,
129.542258985647));
#229938=CARTESIAN_POINT('Ctrl Pts',(7.45828155278369,-2.64585007437836,
129.533965495466));
#229939=CARTESIAN_POINT('Ctrl Pts',(7.38425724951933,-2.83842665449034,
129.525672005284));
#229940=CARTESIAN_POINT('Ctrl Pts',(7.31018580901054,-3.03112586364343,
129.517373233969));
#229941=CARTESIAN_POINT('Ctrl Pts',(7.22859940157151,-3.2208406303884,129.509074462654));
#229942=CARTESIAN_POINT('Ctrl Pts',(7.13977095373429,-3.40699159497234,
129.500775691338));
#229943=CARTESIAN_POINT('Ctrl Pts',(7.05083910445851,-3.59335925001971,
129.492467259774));
#229944=CARTESIAN_POINT('Ctrl Pts',(6.95464849006075,-3.77615454630648,
129.48415882821));
#229945=CARTESIAN_POINT('Ctrl Pts',(6.8515184930998,-3.95482178343241,129.475850396646));
#229946=CARTESIAN_POINT('Ctrl Pts',(6.74832487856208,-4.13359923462803,
129.467536839878));
#229947=CARTESIAN_POINT('Ctrl Pts',(6.63818348852295,-4.30824329374038,
129.45922328311));
#229948=CARTESIAN_POINT('Ctrl Pts',(6.52145744518215,-4.47822663458186,
129.450909726342));
#229949=CARTESIAN_POINT('Ctrl Pts',(6.40460378620328,-4.64839581683355,
129.44258708043));
#229950=CARTESIAN_POINT('Ctrl Pts',(6.28115125632881,-4.81389385895475,
129.434264434518));
#229951=CARTESIAN_POINT('Ctrl Pts',(6.15150470580301,-4.97422464857423,
129.425941788605));
#229952=CARTESIAN_POINT('Ctrl Pts',(6.10229236040166,-5.03508437962935,
129.422782607558));
#229953=CARTESIAN_POINT('Ctrl Pts',(6.05218793563885,-5.09519993015592,
129.41962342651));
#229954=CARTESIAN_POINT('Ctrl Pts',(6.00121501131736,-5.15454550740793,
129.416464245463));
#229955=CARTESIAN_POINT('Ctrl Pts',(5.86087052655006,-5.3179425377631,129.407766026903));
#229956=CARTESIAN_POINT('Ctrl Pts',(5.71381491466608,-5.47564514668322,
129.399067808342));
#229957=CARTESIAN_POINT('Ctrl Pts',(5.56051322480689,-5.62713192281358,
129.390369589782));
#229958=CARTESIAN_POINT('Ctrl Pts',(5.40734623103258,-5.77848559750407,
129.381679013773));
#229959=CARTESIAN_POINT('Ctrl Pts',(5.24794428011976,-5.9236341839293,129.372988437764));
#229960=CARTESIAN_POINT('Ctrl Pts',(5.08280978380573,-6.06209251840062,
129.364297861755));
#229961=CARTESIAN_POINT('Ctrl Pts',(4.91371493496276,-6.20387144201179,
129.355398863245));
#229962=CARTESIAN_POINT('Ctrl Pts',(4.73860929424641,-6.33863502031817,
129.346499864736));
#229963=CARTESIAN_POINT('Ctrl Pts',(4.55807175947969,-6.46590309511624,
129.337600866226));
#229964=CARTESIAN_POINT('Ctrl Pts',(4.38228206693546,-6.58982422746335,
129.328935896839));
#229965=CARTESIAN_POINT('Ctrl Pts',(4.20134274486011,-6.70663892205821,
129.320270927452));
#229966=CARTESIAN_POINT('Ctrl Pts',(4.01582217827375,-6.81594404558053,
129.311605958064));
#229967=CARTESIAN_POINT('Ctrl Pts',(3.8227856217016,-6.92967744478627,129.302589944993));
#229968=CARTESIAN_POINT('Ctrl Pts',(3.62478906884573,-7.03527998402457,
129.293573931922));
#229969=CARTESIAN_POINT('Ctrl Pts',(3.42250840623855,-7.13234584195316,
129.284557918851));
#229970=CARTESIAN_POINT('Ctrl Pts',(3.22022774363136,-7.22941169988175,
129.27554190578));
#229971=CARTESIAN_POINT('Ctrl Pts',(3.01366319431664,-7.31794069493331,
129.266525892709));
#229972=CARTESIAN_POINT('Ctrl Pts',(2.80352372497274,-7.39757904476289,
129.257509879638));
#229973=CARTESIAN_POINT('Ctrl Pts',(2.6214829541078,-7.46656859079464,129.249699438436));
#229974=CARTESIAN_POINT('Ctrl Pts',(2.43683770602419,-7.52885590885969,
129.241888997233));
#229975=CARTESIAN_POINT('Ctrl Pts',(2.25012971134512,-7.58424928929172,
129.234078556031));
#229976=CARTESIAN_POINT('Ctrl Pts',(2.06343517793614,-7.63963867597266,
129.226268677946));
#229977=CARTESIAN_POINT('Ctrl Pts',(1.87467853179391,-7.68813501490881,
129.218458799861));
#229978=CARTESIAN_POINT('Ctrl Pts',(1.6844167269518,-7.72959645065413,129.210648921776));
#229979=CARTESIAN_POINT('Ctrl Pts',(1.49413505736912,-7.77106221528021,
129.202838228281));
#229980=CARTESIAN_POINT('Ctrl Pts',(1.30234826035644,-7.80549153953602,
129.195027534787));
#229981=CARTESIAN_POINT('Ctrl Pts',(1.10962368973367,-7.83279364385286,
129.187216841293));
#229982=CARTESIAN_POINT('Ctrl Pts',(0.916762351033343,-7.86011512326189,
129.179400604896));
#229983=CARTESIAN_POINT('Ctrl Pts',(0.722962258273764,-7.88029922835287,
129.171584368499));
#229984=CARTESIAN_POINT('Ctrl Pts',(0.528796982780863,-7.89330695912695,
129.163768132102));
#229985=CARTESIAN_POINT('Ctrl Pts',(0.3345599215757,-7.90631949904733,129.15594900593));
#229986=CARTESIAN_POINT('Ctrl Pts',(0.139957760356455,-7.91215036391374,
129.148129879757));
#229987=CARTESIAN_POINT('Ctrl Pts',(-0.0544355691391259,-7.91081271228263,
129.140310753584));
#229988=CARTESIAN_POINT('Ctrl Pts',(-0.249045058317264,-7.90947357322214,
129.132482932773));
#229989=CARTESIAN_POINT('Ctrl Pts',(-0.443444899973684,-7.90095000545172,
129.124655111961));
#229990=CARTESIAN_POINT('Ctrl Pts',(-0.637064811594767,-7.88530718652278,
129.116827291149));
#229991=CARTESIAN_POINT('Ctrl Pts',(-0.787714653910383,-7.87313597858612,
129.110736698704));
#229992=CARTESIAN_POINT('Ctrl Pts',(-0.937892393890127,-7.85665587907517,
129.104646106259));
#229993=CARTESIAN_POINT('Ctrl Pts',(-1.08733377287872,-7.83591898033392,
129.098555513814));
#229994=CARTESIAN_POINT('Ctrl Pts',(-1.28649543838022,-7.80828275723028,
129.090438534812));
#229995=CARTESIAN_POINT('Ctrl Pts',(-1.48474480775886,-7.77302955959852,
129.08232155581));
#229996=CARTESIAN_POINT('Ctrl Pts',(-1.68147669854351,-7.73023654956659,
129.074204576808));
#229997=CARTESIAN_POINT('Ctrl Pts',(-1.8780646867795,-7.68747484113596,
129.066093535094));
#229998=CARTESIAN_POINT('Ctrl Pts',(-2.07313709734138,-7.63718438462703,
129.057982493381));
#229999=CARTESIAN_POINT('Ctrl Pts',(-2.26609703542969,-7.57949373151115,
129.049871451667));
#230000=CARTESIAN_POINT('Ctrl Pts',(-2.45894326550832,-7.52183707451595,
129.041765189653));
#230001=CARTESIAN_POINT('Ctrl Pts',(-2.64967919891987,-7.45678900823411,
129.033658927638));
#230002=CARTESIAN_POINT('Ctrl Pts',(-2.83772068544547,-7.38452857746484,
129.025552665623));
#230003=CARTESIAN_POINT('Ctrl Pts',(-3.02567806992521,-7.31230046536192,
129.017450029155));
#230004=CARTESIAN_POINT('Ctrl Pts',(-3.21094311195377,-7.2328665366034,
129.009347392688));
#230005=CARTESIAN_POINT('Ctrl Pts',(-3.39294876614398,-7.14645504220953,
129.00124475622));
#230006=CARTESIAN_POINT('Ctrl Pts',(-3.57489884682694,-7.06006993265427,
128.993144593807));
#230007=CARTESIAN_POINT('Ctrl Pts',(-3.75359123527485,-6.96671164425574,
128.985044431393));
#230008=CARTESIAN_POINT('Ctrl Pts',(-3.92848022020225,-6.86665596629682,
128.97694426898));
#230009=CARTESIAN_POINT('Ctrl Pts',(-4.10507270924634,-6.76562569717441,
128.968765207029));
#230010=CARTESIAN_POINT('Ctrl Pts',(-4.27778700634479,-6.65776701350228,
128.960586145079));
#230011=CARTESIAN_POINT('Ctrl Pts',(-4.44608732466862,-6.54341107538117,
128.952407083128));
#230012=CARTESIAN_POINT('Ctrl Pts',(-4.6127632151291,-6.43015889614818,
128.944306965152));
#230013=CARTESIAN_POINT('Ctrl Pts',(-4.77510970111102,-6.31053453282727,
128.936206847177));
#230014=CARTESIAN_POINT('Ctrl Pts',(-4.93263578576802,-6.18490300691617,
128.928106729201));
#230015=CARTESIAN_POINT('Ctrl Pts',(-5.09018307066639,-6.05925457321054,
128.920005521092));
#230016=CARTESIAN_POINT('Ctrl Pts',(-5.24290840960802,-5.92759756459862,
128.911904312983));
#230017=CARTESIAN_POINT('Ctrl Pts',(-5.39035375721154,-5.79033741435812,
128.903803104874));
#230018=CARTESIAN_POINT('Ctrl Pts',(-5.53783799082539,-5.65304106426657,
128.895699760219));
#230019=CARTESIAN_POINT('Ctrl Pts',(-5.68003922133437,-5.51013884410502,
128.887596415565));
#230020=CARTESIAN_POINT('Ctrl Pts',(-5.81653576125156,-5.36207354836557,
128.879493070911));
#230021=CARTESIAN_POINT('Ctrl Pts',(-5.95528686725633,-5.21156260092883,
128.871255880182));
#230022=CARTESIAN_POINT('Ctrl Pts',(-6.08814294612623,-5.05571677712489,
128.863018689453));
#230023=CARTESIAN_POINT('Ctrl Pts',(-6.21470335965031,-4.89503658326995,
128.854781498724));
#230024=CARTESIAN_POINT('Ctrl Pts',(-6.33936942420691,-4.73676144128587,
128.84666760179));
#230025=CARTESIAN_POINT('Ctrl Pts',(-6.45792680946358,-4.57379591904472,
128.838553704857));
#230026=CARTESIAN_POINT('Ctrl Pts',(-6.57003591656469,-4.40664827902682,
128.830439807924));
#230027=CARTESIAN_POINT('Ctrl Pts',(-6.68470033539451,-4.23569082965436,
128.822140970297));
#230028=CARTESIAN_POINT('Ctrl Pts',(-6.79261883201481,-4.06035864948025,
128.81384213267));
#230029=CARTESIAN_POINT('Ctrl Pts',(-6.89347722352456,-3.88122310216099,
128.805543295044));
#230030=CARTESIAN_POINT('Ctrl Pts',(-6.99433561503423,-3.70208755484186,
128.797244457417));
#230031=CARTESIAN_POINT('Ctrl Pts',(-7.08813377025222,-3.51914897332756,
128.78894561979));
#230032=CARTESIAN_POINT('Ctrl Pts',(-7.1746094353811,-3.33300171763239,
128.780646782164));
#230033=CARTESIAN_POINT('Ctrl Pts',(-7.2587303778006,-3.15192323093279,
128.772573920959));
#230034=CARTESIAN_POINT('Ctrl Pts',(-7.3360950640958,-2.96743665300502,
128.764501059755));
#230035=CARTESIAN_POINT('Ctrl Pts',(-7.40642284997545,-2.78007582043394,
128.756428198551));
#230036=CARTESIAN_POINT('Ctrl Pts',(-7.47666360158173,-2.59294685658613,
128.74836532793));
#230037=CARTESIAN_POINT('Ctrl Pts',(-7.53988469464196,-2.40295102848861,
128.740302457309));
#230038=CARTESIAN_POINT('Ctrl Pts',(-7.59585206049751,-2.21064526214312,
128.732239586688));
#230039=CARTESIAN_POINT('Ctrl Pts',(-7.65173768266623,-2.01862036987662,
128.724188492372));
#230040=CARTESIAN_POINT('Ctrl Pts',(-7.70039061785201,-1.82429257827295,
128.716137398056));
#230041=CARTESIAN_POINT('Ctrl Pts',(-7.74162547949035,-1.62823706360768,
128.70808630374));
#230042=CARTESIAN_POINT('Ctrl Pts',(-7.78282540607073,-1.43234765137363,
128.700042030483));
#230043=CARTESIAN_POINT('Ctrl Pts',(-7.81661971546128,-1.2347337488063,
128.691997757227));
#230044=CARTESIAN_POINT('Ctrl Pts',(-7.84287291842816,-1.03598522450182,
128.683953483971));
#230045=CARTESIAN_POINT('Ctrl Pts',(-7.86910184996185,-0.837420445835432,
128.675916647751));
#230046=CARTESIAN_POINT('Ctrl Pts',(-7.88780353659961,-0.637723458176799,
128.667879811532));
#230047=CARTESIAN_POINT('Ctrl Pts',(-7.89889359558828,-0.43749396061485,
128.659842975312));
#230048=CARTESIAN_POINT('Ctrl Pts',(-7.9069483075645,-0.29206723802905,
128.654005819621));
#230049=CARTESIAN_POINT('Ctrl Pts',(-7.91098884942515,-0.146359866205317,
128.648168663929));
#230050=CARTESIAN_POINT('Ctrl Pts',(-7.91099997694602,-0.000603953663847722,
128.642331508237));
#230051=CARTESIAN_POINT('',(-7.9109999966855,0.000229002203636593,124.647722132928));
#230052=CARTESIAN_POINT('Ctrl Pts',(-7.91099999894138,-0.000129419717556176,
128.639166935561));
#230053=CARTESIAN_POINT('Ctrl Pts',(-7.91100121127412,0.0739764775597892,
128.636136268948));
#230054=CARTESIAN_POINT('Ctrl Pts',(-7.90996114968628,0.148079691724727,
128.633125555382));
#230055=CARTESIAN_POINT('Ctrl Pts',(-7.90735126112598,0.240980462184097,
128.629373408072));
#230056=CARTESIAN_POINT('Ctrl Pts',(-7.90675528800012,0.259800633819714,
128.628614428807));
#230057=CARTESIAN_POINT('Ctrl Pts',(-7.9056179254174,0.29207448438457,128.627314782394));
#230058=CARTESIAN_POINT('Ctrl Pts',(-7.90510937232408,0.305529213036417,
128.626773533638));
#230059=CARTESIAN_POINT('Ctrl Pts',(-7.90408917295933,0.330810321266307,
128.625757570898));
#230060=CARTESIAN_POINT('Ctrl Pts',(-7.903585327482,0.342636972377066,128.625282721452));
#230061=CARTESIAN_POINT('Ctrl Pts',(-7.90249553643135,0.366934829989268,
128.624307991145));
#230062=CARTESIAN_POINT('Ctrl Pts',(-7.90190660906471,0.379405871607893,
128.623808163293));
#230063=CARTESIAN_POINT('Ctrl Pts',(-7.90046935423753,0.408384883873768,
128.622647746519));
#230064=CARTESIAN_POINT('Ctrl Pts',(-7.89959880433447,0.424891707948672,
128.621987539022));
#230065=CARTESIAN_POINT('Ctrl Pts',(-7.89669893936198,0.476784135723711,
128.619914399464));
#230066=CARTESIAN_POINT('Ctrl Pts',(-7.89448354223286,0.51215902917028,
128.618504568365));
#230067=CARTESIAN_POINT('Ctrl Pts',(-7.88629008874091,0.630261068471869,
128.613808219431));
#230068=CARTESIAN_POINT('Ctrl Pts',(-7.87924873140524,0.712909591018122,
128.610539195005));
#230069=CARTESIAN_POINT('Ctrl Pts',(-7.78697011253223,1.62601811823754,
128.5746030605));
#230070=CARTESIAN_POINT('Ctrl Pts',(-7.57210414134284,2.43803142597582,
128.544969408907));
#230071=CARTESIAN_POINT('Ctrl Pts',(-7.15984653287076,3.36962347645104,
128.506794549435));
#230072=CARTESIAN_POINT('Ctrl Pts',(-7.07955622243845,3.53520073623228,
128.499802380294));
#230073=CARTESIAN_POINT('Ctrl Pts',(-6.95491557586082,3.77092947282715,
128.489386740156));
#230074=CARTESIAN_POINT('Ctrl Pts',(-6.91511762839045,3.8434239131052,128.486117981144));
#230075=CARTESIAN_POINT('Ctrl Pts',(-6.86743686486009,3.92713867459256,
128.482254085106));
#230076=CARTESIAN_POINT('Ctrl Pts',(-6.86065170309211,3.93898025741314,
128.481705425953));
#230077=CARTESIAN_POINT('Ctrl Pts',(-6.85026247888206,3.95700343327686,
128.480867067355));
#230078=CARTESIAN_POINT('Ctrl Pts',(-6.84668059675476,3.96319782576374,
128.480578338063));
#230079=CARTESIAN_POINT('Ctrl Pts',(-6.84016119063358,3.97443706274176,
128.480053370482));
#230080=CARTESIAN_POINT('Ctrl Pts',(-6.83722647476021,3.97948353585577,
128.479817257192));
#230081=CARTESIAN_POINT('Ctrl Pts',(-6.83090079366699,3.9903333851911,128.47930874711));
#230082=CARTESIAN_POINT('Ctrl Pts',(-6.82750801449153,3.99613569459031,
128.479036268582));
#230083=CARTESIAN_POINT('Ctrl Pts',(-6.81836635055561,4.01172408408465,
128.478302774026));
#230084=CARTESIAN_POINT('Ctrl Pts',(-6.81260380694788,4.02150210555337,
128.477841132327));
#230085=CARTESIAN_POINT('Ctrl Pts',(-6.78617524140649,4.06612690119456,
128.475727091229));
#230086=CARTESIAN_POINT('Ctrl Pts',(-6.76526301596299,4.1008265777983,128.474063117669));
#230087=CARTESIAN_POINT('Ctrl Pts',(-6.42824960169078,4.65043901203498,
128.447365444081));
#230088=CARTESIAN_POINT('Ctrl Pts',(-6.0545011462509,5.12754827620941,128.419079539236));
#230089=CARTESIAN_POINT('Ctrl Pts',(-5.49870413874924,5.69062479448512,
128.382759735616));
#230090=CARTESIAN_POINT('Ctrl Pts',(-5.36252161189191,5.81913421414582,
128.37422098809));
#230091=CARTESIAN_POINT('Ctrl Pts',(-5.03073695829835,6.1106767293155,128.354376293751));
#230092=CARTESIAN_POINT('Ctrl Pts',(-4.83156501548559,6.26934431935141,
128.343194039817));
#230093=CARTESIAN_POINT('Ctrl Pts',(-4.5293528194415,6.48712618490164,128.32736051447));
#230094=CARTESIAN_POINT('Ctrl Pts',(-4.43209288467012,6.55396043425648,
128.322424245819));
#230095=CARTESIAN_POINT('Ctrl Pts',(-4.29805063652521,6.64172146817376,
128.315835424086));
#230096=CARTESIAN_POINT('Ctrl Pts',(-4.26254504276058,6.66456398934121,
128.314110017186));
#230097=CARTESIAN_POINT('Ctrl Pts',(-4.21026732610536,6.69760817471524,
128.31159838707));
#230098=CARTESIAN_POINT('Ctrl Pts',(-4.19363768819147,6.70803318171213,
128.310803662887));
#230099=CARTESIAN_POINT('Ctrl Pts',(-4.16354986777803,6.7267394173849,128.309373370625));
#230100=CARTESIAN_POINT('Ctrl Pts',(-4.15010537281631,6.73504239699292,
128.308736976536));
#230101=CARTESIAN_POINT('Ctrl Pts',(-4.12949887517224,6.7476833171155,128.307765710601));
#230102=CARTESIAN_POINT('Ctrl Pts',(-4.12235475136984,6.75205023770998,
128.30742973828));
#230103=CARTESIAN_POINT('Ctrl Pts',(-4.10989864132629,6.75963702740896,
128.306845272573));
#230104=CARTESIAN_POINT('Ctrl Pts',(-4.10458977755371,6.76286199345599,
128.306596585905));
#230105=CARTESIAN_POINT('Ctrl Pts',(-4.09349665681893,6.76958283790018,
128.3060778099));
#230106=CARTESIAN_POINT('Ctrl Pts',(-4.08771170555547,6.7730775642357,128.305807764335));
#230107=CARTESIAN_POINT('Ctrl Pts',(-4.07174047653524,6.78269797171888,
128.30506356717));
#230108=CARTESIAN_POINT('Ctrl Pts',(-4.06154484096062,6.78880812737592,
128.304590003717));
#230109=CARTESIAN_POINT('Ctrl Pts',(-4.02176220371625,6.81252781711409,
128.302748063967));
#230110=CARTESIAN_POINT('Ctrl Pts',(-3.99207393047296,6.8299672221038,128.301386120921));
#230111=CARTESIAN_POINT('Ctrl Pts',(-3.50928213737817,7.10934407385299,
128.279439688606));
#230112=CARTESIAN_POINT('Ctrl Pts',(-3.03138836506622,7.3258858474412,128.260704198303));
#230113=CARTESIAN_POINT('Ctrl Pts',(-2.2931515475015,7.57567577855633,128.234052269651));
#230114=CARTESIAN_POINT('Ctrl Pts',(-2.04690949239423,7.64588586348729,
128.225493231206));
#230115=CARTESIAN_POINT('Ctrl Pts',(-1.76605233908665,7.71142244367132,
128.215790663973));
#230116=CARTESIAN_POINT('Ctrl Pts',(-1.73436162607159,7.71861170900182,
128.214696619827));
#230117=CARTESIAN_POINT('Ctrl Pts',(-1.6659907971715,7.73367979101778,128.212336532435));
#230118=CARTESIAN_POINT('Ctrl Pts',(-1.62929714106727,7.74149334822053,
128.211070060516));
#230119=CARTESIAN_POINT('Ctrl Pts',(-1.48467495034829,7.77121545747075,
128.20607511708));
#230120=CARTESIAN_POINT('Ctrl Pts',(-1.37635048005621,7.7911300987996,128.202326632114));
#230121=CARTESIAN_POINT('Ctrl Pts',(-1.07345989407446,7.84030019825425,
128.191751208123));
#230122=CARTESIAN_POINT('Ctrl Pts',(-0.878171960371177,7.86456807998093,
128.184825899124));
#230123=CARTESIAN_POINT('Ctrl Pts',(-0.51927092236274,7.89563301418451,
128.171605098645));
#230124=CARTESIAN_POINT('Ctrl Pts',(-0.355961363407117,7.90467889214603,
128.165403245937));
#230125=CARTESIAN_POINT('Ctrl Pts',(-0.167723119136127,7.90926065743318,
128.157928234554));
#230126=CARTESIAN_POINT('Ctrl Pts',(-0.142945135043231,7.90974726862364,
128.156937782592));
#230127=CARTESIAN_POINT('Ctrl Pts',(-0.111295951826042,7.91022006096811,
128.155663918323));
#230128=CARTESIAN_POINT('Ctrl Pts',(-0.1044262498859,7.91031373332172,128.155386889707));
#230129=CARTESIAN_POINT('Ctrl Pts',(-0.09340881010094,7.91044960794139,
128.154941742852));
#230130=CARTESIAN_POINT('Ctrl Pts',(-0.089261132376909,7.91049749735751,
128.154773966207));
#230131=CARTESIAN_POINT('Ctrl Pts',(-0.0813962377484495,7.91058211964043,
128.154455453445));
#230132=CARTESIAN_POINT('Ctrl Pts',(-0.0776790273551331,7.91061949455969,
128.154304756198));
#230133=CARTESIAN_POINT('Ctrl Pts',(-0.0692478609497113,7.91069832296132,
128.153962593291));
#230134=CARTESIAN_POINT('Ctrl Pts',(-0.0645339224007235,7.9107381827475,
128.153771031442));
#230135=CARTESIAN_POINT('Ctrl Pts',(-0.0522928525898666,7.91083074762393,
128.153272920988));
#230136=CARTESIAN_POINT('Ctrl Pts',(-0.0447657354246197,7.91087692282478,
128.152965977143));
#230137=CARTESIAN_POINT('Ctrl Pts',(0.00162847907137823,7.91109531169428,
128.151070129017));
#230138=CARTESIAN_POINT('Ctrl Pts',(0.0404956967984957,7.91099182627501,
128.149464708376));
#230139=CARTESIAN_POINT('Ctrl Pts',(0.734275082004543,7.9040317681045,128.120523403488));
#230140=CARTESIAN_POINT('Ctrl Pts',(1.38580846036759,7.81616030339117,128.089042961505));
#230141=CARTESIAN_POINT('Ctrl Pts',(2.21805256030406,7.59648167987469,128.049116846429));
#230142=CARTESIAN_POINT('Ctrl Pts',(2.41495582983533,7.53619833059681,128.03967026914));
#230143=CARTESIAN_POINT('Ctrl Pts',(2.83017952890383,7.39112662353034,128.019900972368));
#230144=CARTESIAN_POINT('Ctrl Pts',(3.04754656824602,7.30418656388955,128.009646008333));
#230145=CARTESIAN_POINT('Ctrl Pts',(3.36033381813377,7.16268269707147,127.995091978784));
#230146=CARTESIAN_POINT('Ctrl Pts',(3.45897267658545,7.11557279319726,127.990532072382));
#230147=CARTESIAN_POINT('Ctrl Pts',(3.59194910385011,7.04864441884482,127.984424766662));
#230148=CARTESIAN_POINT('Ctrl Pts',(3.62715794216121,7.03059114406723,127.982811558872));
#230149=CARTESIAN_POINT('Ctrl Pts',(3.67864334010268,7.00370238118153,127.980458064688));
#230150=CARTESIAN_POINT('Ctrl Pts',(3.69502638163961,6.99507283117162,127.979709984645));
#230151=CARTESIAN_POINT('Ctrl Pts',(3.72448251138582,6.97942484577755,127.978366409201));
#230152=CARTESIAN_POINT('Ctrl Pts',(3.73756640917296,6.97242701617256,127.977770132838));
#230153=CARTESIAN_POINT('Ctrl Pts',(3.75769598649603,6.96158791274822,127.976853542057));
#230154=CARTESIAN_POINT('Ctrl Pts',(3.7647556022566,6.95777267878535,127.976532234144));
#230155=CARTESIAN_POINT('Ctrl Pts',(3.77704306051581,6.95110798134977,127.975973244228));
#230156=CARTESIAN_POINT('Ctrl Pts',(3.78227350725494,6.9482633489173,127.975735377772));
#230157=CARTESIAN_POINT('Ctrl Pts',(3.79318888994037,6.94231092806197,127.975239143143));
#230158=CARTESIAN_POINT('Ctrl Pts',(3.79887323035141,6.93920205474923,127.974980816798));
#230159=CARTESIAN_POINT('Ctrl Pts',(3.81280409051244,6.93156075606482,127.974347955491));
#230160=CARTESIAN_POINT('Ctrl Pts',(3.82104636545572,6.92702058763709,127.973973717626));
#230161=CARTESIAN_POINT('Ctrl Pts',(3.85276248305608,6.9094762736656,127.972534408928));
#230162=CARTESIAN_POINT('Ctrl Pts',(3.87617833351463,6.89636735340833,127.971473363667));
#230163=CARTESIAN_POINT('Ctrl Pts',(4.2633728756836,6.67700878084544,127.95395339055));
#230164=CARTESIAN_POINT('Ctrl Pts',(4.61032093100209,6.44234319828263,127.938676841411));
#230165=CARTESIAN_POINT('Ctrl Pts',(5.31584473587302,5.8788311362351,127.907110024825));
#230166=CARTESIAN_POINT('Ctrl Pts',(5.66595488929413,5.54218307766664,127.891121907487));
#230167=CARTESIAN_POINT('Ctrl Pts',(6.03005812778953,5.12127747317954,127.871733860245));
#230168=CARTESIAN_POINT('Ctrl Pts',(6.07632406315281,5.0662974266392,127.869210259617));
#230169=CARTESIAN_POINT('Ctrl Pts',(6.18421386044982,4.93448270397832,127.863161202208));
#230170=CARTESIAN_POINT('Ctrl Pts',(6.24516367136208,4.85711338707234,127.859611706086));
#230171=CARTESIAN_POINT('Ctrl Pts',(6.40141946301403,4.65095833923383,127.850098225546));
#230172=CARTESIAN_POINT('Ctrl Pts',(6.49428166457669,4.52038543862774,127.844017516621));
#230173=CARTESIAN_POINT('Ctrl Pts',(6.5966257938236,4.36681154544922,127.836689064041));
#230174=CARTESIAN_POINT('Ctrl Pts',(6.61004693563552,4.34646919228543,127.835714853272));
#230175=CARTESIAN_POINT('Ctrl Pts',(6.62717794131313,4.32024095702252,127.834453856382));
#230176=CARTESIAN_POINT('Ctrl Pts',(6.63097433720514,4.31441174799988,127.834173294221));
#230177=CARTESIAN_POINT('Ctrl Pts',(6.63710578622756,4.30496995178391,127.833718371256));
#230178=CARTESIAN_POINT('Ctrl Pts',(6.63944559764473,4.30136044282628,127.833544343911));
#230179=CARTESIAN_POINT('Ctrl Pts',(6.64391323737766,4.2944561096564,127.833211245041));
#230180=CARTESIAN_POINT('Ctrl Pts',(6.64604156240506,4.29116160663332,127.833052208073));
#230181=CARTESIAN_POINT('Ctrl Pts',(6.65091085556426,4.28361195844812,127.832687547952));
#230182=CARTESIAN_POINT('Ctrl Pts',(6.65365018934629,4.2793557665616,127.832481812484));
#230183=CARTESIAN_POINT('Ctrl Pts',(6.66206729161779,4.26625022124334,127.831847849524));
#230184=CARTESIAN_POINT('Ctrl Pts',(6.66773148423367,4.25739220655312,127.831418699046));
#230185=CARTESIAN_POINT('Ctrl Pts',(6.70995470088925,4.19106998440169,127.828200797184));
#230186=CARTESIAN_POINT('Ctrl Pts',(6.74578694018977,4.13314864689467,127.825363928082));
#230187=CARTESIAN_POINT('Ctrl Pts',(7.0450362889,3.6351652238909,127.800797190376));
#230188=CARTESIAN_POINT('Ctrl Pts',(7.26581208746858,3.17094018161968,127.776795965506));
#230189=CARTESIAN_POINT('Ctrl Pts',(7.53520571427323,2.42547142535818,127.739808659456));
#230190=CARTESIAN_POINT('Ctrl Pts',(7.6162868986103,2.15741054967077,127.726783426014));
#230191=CARTESIAN_POINT('Ctrl Pts',(7.75515812895008,1.59157410622988,127.700264519393));
#230192=CARTESIAN_POINT('Ctrl Pts',(7.81038753440492,1.29362162286276,127.686844109572));
#230193=CARTESIAN_POINT('Ctrl Pts',(7.86901738905358,0.830327424531193,
127.666950089259));
#230194=CARTESIAN_POINT('Ctrl Pts',(7.88455565284768,0.666831886836047,
127.660110732551));
#230195=CARTESIAN_POINT('Ctrl Pts',(7.89637673781107,0.481277105799719,
127.652546478748));
#230196=CARTESIAN_POINT('Ctrl Pts',(7.89766899155654,0.459584320521321,
127.65166519196));
#230197=CARTESIAN_POINT('Ctrl Pts',(7.89983054064649,0.420592928296198,
127.650086525196));
#230198=CARTESIAN_POINT('Ctrl Pts',(7.90073243890115,0.403296313038426,
127.649388131948));
#230199=CARTESIAN_POINT('Ctrl Pts',(7.90201263261451,0.377090008239126,
127.648332844756));
#230200=CARTESIAN_POINT('Ctrl Pts',(7.90243267565847,0.368182465184135,
127.647974651587));
#230201=CARTESIAN_POINT('Ctrl Pts',(7.90313323640022,0.352772459050454,
127.647355838861));
#230202=CARTESIAN_POINT('Ctrl Pts',(7.90342079204526,0.346270334101139,
127.647095000653));
#230203=CARTESIAN_POINT('Ctrl Pts',(7.90400006973454,0.332795141442946,
127.64655497823));
#230204=CARTESIAN_POINT('Ctrl Pts',(7.90429058900953,0.325822027069712,
127.646275831647));
#230205=CARTESIAN_POINT('Ctrl Pts',(7.90497338961275,0.308894721436374,
127.645598932737));
#230206=CARTESIAN_POINT('Ctrl Pts',(7.90535609766465,0.298940143658653,
127.645201477888));
#230207=CARTESIAN_POINT('Ctrl Pts',(7.9067174889718,0.261696742733594,127.643716749595));
#230208=CARTESIAN_POINT('Ctrl Pts',(7.90757368963916,0.234403491987286,
127.642633275133));
#230209=CARTESIAN_POINT('Ctrl Pts',(7.91945394396499,-0.219240524756486,
127.624699341592));
#230210=CARTESIAN_POINT('Ctrl Pts',(7.89612500699176,-0.645814099276256,
127.60898279469));
#230211=CARTESIAN_POINT('Ctrl Pts',(7.76791458401909,-1.58640449193305,
127.575318675768));
#230212=CARTESIAN_POINT('Ctrl Pts',(7.64615516803898,-2.09605719926854,
127.557762258673));
#230213=CARTESIAN_POINT('Ctrl Pts',(7.37543293457946,-2.87740399458092,
127.528161550649));
#230214=CARTESIAN_POINT('Ctrl Pts',(7.25936692570651,-3.15880679583878,
127.516833759523));
#230215=CARTESIAN_POINT('Ctrl Pts',(7.11760984898295,-3.45312256546041,
127.503816847697));
#230216=CARTESIAN_POINT('Ctrl Pts',(7.10777788190242,-3.47331527273461,
127.502918446733));
#230217=CARTESIAN_POINT('Ctrl Pts',(7.09365552708116,-3.50200841224156,
127.501634486217));
#230218=CARTESIAN_POINT('Ctrl Pts',(7.08943552405788,-3.51054349148853,
127.501251627071));
#230219=CARTESIAN_POINT('Ctrl Pts',(7.0821353710373,-3.52524141786543,127.500590734554));
#230220=CARTESIAN_POINT('Ctrl Pts',(7.07906255460162,-3.53140790842009,
127.500312976034));
#230221=CARTESIAN_POINT('Ctrl Pts',(7.07317239281364,-3.54318963221742,
127.499781375778));
#230222=CARTESIAN_POINT('Ctrl Pts',(7.07035640564869,-3.54880554062257,
127.499527584161));
#230223=CARTESIAN_POINT('Ctrl Pts',(7.0637569968915,-3.5619276728514,127.498933652611));
#230224=CARTESIAN_POINT('Ctrl Pts',(7.05996829840127,-3.56943122678449,
127.498593321691));
#230225=CARTESIAN_POINT('Ctrl Pts',(7.04648903191586,-3.59602162649467,
127.497384810311));
#230226=CARTESIAN_POINT('Ctrl Pts',(7.03673300246097,-3.61507508330517,
127.496514311783));
#230227=CARTESIAN_POINT('Ctrl Pts',(6.89280533789541,-3.89337464818352,
127.483735041236));
#230228=CARTESIAN_POINT('Ctrl Pts',(6.74446685989942,-4.1450314520681,127.471367495351));
#230229=CARTESIAN_POINT('Ctrl Pts',(6.21520984343613,-4.93900298755645,
127.430517156432));
#230230=CARTESIAN_POINT('Ctrl Pts',(5.7800638917804,-5.44183145675548,127.401932221355));
#230231=CARTESIAN_POINT('Ctrl Pts',(4.96201057748446,-6.17686648437265,
127.356067753393));
#230232=CARTESIAN_POINT('Ctrl Pts',(4.61296617694909,-6.4417225915335,127.338096220104));
#230233=CARTESIAN_POINT('Ctrl Pts',(4.20163165313136,-6.70318668381087,
127.318349471264));
#230234=CARTESIAN_POINT('Ctrl Pts',(4.15918767725659,-6.72960460733497,
127.316328772945));
#230235=CARTESIAN_POINT('Ctrl Pts',(4.09513266996374,-6.76863614507779,
127.313304309528));
#230236=CARTESIAN_POINT('Ctrl Pts',(4.07370768947117,-6.78155236762812,
127.312296857622));
#230237=CARTESIAN_POINT('Ctrl Pts',(4.0367000966844,-6.80362403049173,127.310563797947));
#230238=CARTESIAN_POINT('Ctrl Pts',(4.02114673500226,-6.81282808798094,
127.309837588312));
#230239=CARTESIAN_POINT('Ctrl Pts',(3.98894776163817,-6.83173389032634,
127.308338589413));
#230240=CARTESIAN_POINT('Ctrl Pts',(3.97229796922217,-6.84142828942935,
127.307565896845));
#230241=CARTESIAN_POINT('Ctrl Pts',(3.92699091822985,-6.86758732303617,
127.305469802101));
#230242=CARTESIAN_POINT('Ctrl Pts',(3.89826557889077,-6.88393338142764,
127.304147919869));
#230243=CARTESIAN_POINT('Ctrl Pts',(3.78858369651143,-6.94544080420906,
127.299127093602));
#230244=CARTESIAN_POINT('Ctrl Pts',(3.70693751791876,-6.98935826053939,
127.295444353657));
#230245=CARTESIAN_POINT('Ctrl Pts',(3.5264138297107,-7.08240869392595,127.287414677762));
#230246=CARTESIAN_POINT('Ctrl Pts',(3.42724124136173,-7.13092737967312,
127.283076051168));
#230247=CARTESIAN_POINT('Ctrl Pts',(2.88398997815055,-7.3827531656119,127.259663011855));
#230248=CARTESIAN_POINT('Ctrl Pts',(2.42283147915567,-7.54667662001762,
127.241119188796));
#230249=CARTESIAN_POINT('Ctrl Pts',(1.79130519476014,-7.70725587816562,
127.21592414503));
#230250=CARTESIAN_POINT('Ctrl Pts',(1.63189710549168,-7.7425756436185,127.209573584054));
#230251=CARTESIAN_POINT('Ctrl Pts',(1.39275569657107,-7.78784807750668,
127.19996801373));
#230252=CARTESIAN_POINT('Ctrl Pts',(1.31377670325269,-7.80155988004134,
127.196782916753));
#230253=CARTESIAN_POINT('Ctrl Pts',(1.2165217250263,-7.81692593190561,127.192835372436));
#230254=CARTESIAN_POINT('Ctrl Pts',(1.19842970397341,-7.81972009555002,
127.192099926928));
#230255=CARTESIAN_POINT('Ctrl Pts',(1.16930234122253,-7.82411511738605,
127.190914092964));
#230256=CARTESIAN_POINT('Ctrl Pts',(1.15827309312231,-7.82575547637889,
127.1904646628));
#230257=CARTESIAN_POINT('Ctrl Pts',(1.137181307991,-7.82884685202697,127.189604442218));
#230258=CARTESIAN_POINT('Ctrl Pts',(1.12711936506956,-7.8303018010742,127.189193742428));
#230259=CARTESIAN_POINT('Ctrl Pts',(1.10405064384642,-7.83359213391723,
127.188251416144));
#230260=CARTESIAN_POINT('Ctrl Pts',(1.09104205326145,-7.83541452517142,
127.187719503395));
#230261=CARTESIAN_POINT('Ctrl Pts',(1.05084674145612,-7.84094350074853,
127.186074374704));
#230262=CARTESIAN_POINT('Ctrl Pts',(1.02364531663509,-7.84454103876331,
127.184958849807));
#230263=CARTESIAN_POINT('Ctrl Pts',(0.728891764564894,-7.88196460789007,
127.172849153586));
#230264=CARTESIAN_POINT('Ctrl Pts',(0.459801317816734,-7.90222915293735,
127.161603385505));
#230265=CARTESIAN_POINT('Ctrl Pts',(-0.0547559478940852,-7.91460457148811,
127.140021188502));
#230266=CARTESIAN_POINT('Ctrl Pts',(-0.299863770029728,-7.90911158751756,
127.129706749688));
#230267=CARTESIAN_POINT('Ctrl Pts',(-0.898554161588049,-7.86782052009627,
127.104583651413));
#230268=CARTESIAN_POINT('Ctrl Pts',(-1.25074927542086,-7.81956765641137,
127.089875604971));
#230269=CARTESIAN_POINT('Ctrl Pts',(-1.67626220352074,-7.73177647893193,
127.072188351917));
#230270=CARTESIAN_POINT('Ctrl Pts',(-1.75376135362985,-7.71456698522073,
127.068969444003));
#230271=CARTESIAN_POINT('Ctrl Pts',(-1.8637342825626,-7.68840350646528,
127.064402981761));
#230272=CARTESIAN_POINT('Ctrl Pts',(-1.89642975140006,-7.68040416671623,
127.063045500704));
#230273=CARTESIAN_POINT('Ctrl Pts',(-1.95294211941689,-7.66619487222827,
127.060699158801));
#230274=CARTESIAN_POINT('Ctrl Pts',(-1.97678288955216,-7.66008199387467,
127.059709308781));
#230275=CARTESIAN_POINT('Ctrl Pts',(-2.02259379101185,-7.64810776449011,
127.05780714235));
#230276=CARTESIAN_POINT('Ctrl Pts',(-2.04456793619461,-7.64226275251456,
127.056894669422));
#230277=CARTESIAN_POINT('Ctrl Pts',(-2.09650191950617,-7.62820854890854,
127.05473784476));
#230278=CARTESIAN_POINT('Ctrl Pts',(-2.12643923724366,-7.61991746300815,
127.053494328278));
#230279=CARTESIAN_POINT('Ctrl Pts',(-2.23252328786504,-7.5898638074851,
127.04908656302));
#230280=CARTESIAN_POINT('Ctrl Pts',(-2.30839150132203,-7.56713430920068,
127.045931880051));
#230281=CARTESIAN_POINT('Ctrl Pts',(-3.03914081070575,-7.33619496612101,
127.01549514784));
#230282=CARTESIAN_POINT('Ctrl Pts',(-3.66464783006157,-7.04461455593648,
126.989021916552));
#230283=CARTESIAN_POINT('Ctrl Pts',(-4.59368502364438,-6.45392132999017,
126.947938407626));
#230284=CARTESIAN_POINT('Ctrl Pts',(-4.92481142097114,-6.20493822861273,
126.93278793703));
#230285=CARTESIAN_POINT('Ctrl Pts',(-5.36753093011396,-5.81419018685479,
126.910404200392));
#230286=CARTESIAN_POINT('Ctrl Pts',(-5.49615527167176,-5.6927558299386,
126.903602584133));
#230287=CARTESIAN_POINT('Ctrl Pts',(-5.6395138915521,-5.54802006408539,
126.89554647607));
#230288=CARTESIAN_POINT('Ctrl Pts',(-5.65833265448537,-5.52882583521377,
126.894479062799));
#230289=CARTESIAN_POINT('Ctrl Pts',(-5.69073115102466,-5.49544226563643,
126.892623513879));
#230290=CARTESIAN_POINT('Ctrl Pts',(-5.70435660203371,-5.48129751763507,
126.89183760204));
#230291=CARTESIAN_POINT('Ctrl Pts',(-5.72379092210334,-5.46097156425398,
126.890708438992));
#230292=CARTESIAN_POINT('Ctrl Pts',(-5.72964280082457,-5.45483146575721,
126.890367364076));
#230293=CARTESIAN_POINT('Ctrl Pts',(-5.73975253569239,-5.44418958380439,
126.889776240866));
#230294=CARTESIAN_POINT('Ctrl Pts',(-5.74401500532617,-5.43969218005195,
126.889526430404));
#230295=CARTESIAN_POINT('Ctrl Pts',(-5.75217934210085,-5.43105755424641,
126.889046818237));
#230296=CARTESIAN_POINT('Ctrl Pts',(-5.75608204260536,-5.42692112157854,
126.88881706019));
#230297=CARTESIAN_POINT('Ctrl Pts',(-5.7652332045074,-5.41720092137577,
126.888277145113));
#230298=CARTESIAN_POINT('Ctrl Pts',(-5.7704780132899,-5.41161373552023,
126.887966795852));
#230299=CARTESIAN_POINT('Ctrl Pts',(-5.78842963191154,-5.39243447843413,
126.886901402197));
#230300=CARTESIAN_POINT('Ctrl Pts',(-5.80109654213844,-5.37880526777141,
126.886144222325));
#230301=CARTESIAN_POINT('Ctrl Pts',(-5.95525445125142,-5.21175807362279,
126.876861053795));
#230302=CARTESIAN_POINT('Ctrl Pts',(-6.09064397040441,-5.05287151888935,
126.867955198233));
#230303=CARTESIAN_POINT('Ctrl Pts',(-6.61329874990684,-4.38794922039038,
126.830730231465));
#230304=CARTESIAN_POINT('Ctrl Pts',(-6.94506665078206,-3.84134086028336,
126.800556618191));
#230305=CARTESIAN_POINT('Ctrl Pts',(-7.31101016087678,-3.0324721531888,
126.760497488015));
#230306=CARTESIAN_POINT('Ctrl Pts',(-7.40342598805415,-2.79929506686485,
126.749404632981));
#230307=CARTESIAN_POINT('Ctrl Pts',(-7.55002935522304,-2.37102711631056,
126.729951183344));
#230308=CARTESIAN_POINT('Ctrl Pts',(-7.60810174612933,-2.17750045052778,
126.721484453114));
#230309=CARTESIAN_POINT('Ctrl Pts',(-7.66808127750534,-1.94572629862531,
126.71172144012));
#230310=CARTESIAN_POINT('Ctrl Pts',(-7.67719924844319,-1.90943265273781,
126.710203361392));
#230311=CARTESIAN_POINT('Ctrl Pts',(-7.68900508906434,-1.86098804947727,
126.708191115238));
#230312=CARTESIAN_POINT('Ctrl Pts',(-7.69192223051535,-1.84889377234421,
126.707689920086));
#230313=CARTESIAN_POINT('Ctrl Pts',(-7.69667972412839,-1.82896337147814,
126.706865899581));
#230314=CARTESIAN_POINT('Ctrl Pts',(-7.69853666327623,-1.82113125136086,
126.706542566226));
#230315=CARTESIAN_POINT('Ctrl Pts',(-7.7021220354579,-1.80590553551546,
126.70591494185));
#230316=CARTESIAN_POINT('Ctrl Pts',(-7.70385178353016,-1.7985122601993,
126.705610610834));
#230317=CARTESIAN_POINT('Ctrl Pts',(-7.70783537877509,-1.78137441591975,
126.704906153957));
#230318=CARTESIAN_POINT('Ctrl Pts',(-7.71008139752591,-1.77162803105467,
126.704506268054));
#230319=CARTESIAN_POINT('Ctrl Pts',(-7.71727126903328,-1.74015563091299,
126.703217366535));
#230320=CARTESIAN_POINT('Ctrl Pts',(-7.7221418392687,-1.71841289676821,
126.702330592599));
#230321=CARTESIAN_POINT('Ctrl Pts',(-7.76689541662674,-1.51459514854758,
126.694051812421));
#230322=CARTESIAN_POINT('Ctrl Pts',(-7.80042507303443,-1.33117876678049,
126.686856591788));
#230323=CARTESIAN_POINT('Ctrl Pts',(-7.88306478053682,-0.76709537174334,
126.665387565063));
#230324=CARTESIAN_POINT('Ctrl Pts',(-7.91099226863457,-0.383891627020796,
126.651734473559));
#230325=CARTESIAN_POINT('Ctrl Pts',(-7.91101426730382,0.708199051772036,
126.613702437656));
#230326=CARTESIAN_POINT('Ctrl Pts',(-7.81588990038079,1.41326583717628,
126.590301005153));
#230327=CARTESIAN_POINT('Ctrl Pts',(-7.61746168952565,2.13538151381546,
126.560816417889));
#230328=CARTESIAN_POINT('Ctrl Pts',(-7.6063777508781,2.17453308484879,126.55919916733));
#230329=CARTESIAN_POINT('Ctrl Pts',(-7.59208350190564,2.22357756120768,
126.55715056772));
#230330=CARTESIAN_POINT('Ctrl Pts',(-7.58915499447128,2.23355222436618,
126.556732752421));
#230331=CARTESIAN_POINT('Ctrl Pts',(-7.58450896284928,2.24926224272562,
126.556072881872));
#230332=CARTESIAN_POINT('Ctrl Pts',(-7.58280456724606,2.25500149418048,
126.555831432977));
#230333=CARTESIAN_POINT('Ctrl Pts',(-7.57978263261094,2.26513515914518,
126.555404443827));
#230334=CARTESIAN_POINT('Ctrl Pts',(-7.57846778156442,2.26953037664025,
126.555219025959));
#230335=CARTESIAN_POINT('Ctrl Pts',(-7.57544770128083,2.2795938590567,126.554793979892));
#230336=CARTESIAN_POINT('Ctrl Pts',(-7.5737399334249,2.2852613543439,126.554554237531));
#230337=CARTESIAN_POINT('Ctrl Pts',(-7.56902133132096,2.30085738958276,
126.553893503882));
#230338=CARTESIAN_POINT('Ctrl Pts',(-7.56599733051227,2.3107819097504,126.553471928932));
#230339=CARTESIAN_POINT('Ctrl Pts',(-7.54981573579065,2.363516270765,126.551226031607));
#230340=CARTESIAN_POINT('Ctrl Pts',(-7.53631446872862,2.40621921828136,
126.549386881569));
#230341=CARTESIAN_POINT('Ctrl Pts',(-7.39096090504319,2.85272896677761,
126.529957533555));
#230342=CARTESIAN_POINT('Ctrl Pts',(-7.22715509754713,3.2453918524543,126.511208152868));
#230343=CARTESIAN_POINT('Ctrl Pts',(-6.86000178534438,3.95807821467675,
126.475898437962));
#230344=CARTESIAN_POINT('Ctrl Pts',(-6.66363747992839,4.28041658329275,
126.45936982166));
#230345=CARTESIAN_POINT('Ctrl Pts',(-6.27435983061465,4.82731319347053,
126.43079429022));
#230346=CARTESIAN_POINT('Ctrl Pts',(-6.09043360899482,5.05738840377083,
126.41857293624));
#230347=CARTESIAN_POINT('Ctrl Pts',(-5.87027557670261,5.30330670016279,
126.405211577054));
#230348=CARTESIAN_POINT('Ctrl Pts',(-5.84626637383349,5.32976235996558,
126.403769856501));
#230349=CARTESIAN_POINT('Ctrl Pts',(-5.81086544632176,5.36824348084719,
126.401666042111));
#230350=CARTESIAN_POINT('Ctrl Pts',(-5.79961395061265,5.38039713508329,
126.401000586597));
#230351=CARTESIAN_POINT('Ctrl Pts',(-5.77958303694581,5.4018983115835,126.399821490751));
#230352=CARTESIAN_POINT('Ctrl Pts',(-5.77081891160866,5.41125997713755,
126.399307489167));
#230353=CARTESIAN_POINT('Ctrl Pts',(-5.75253539013836,5.430695137577,126.39823907915));
#230354=CARTESIAN_POINT('Ctrl Pts',(-5.74301220427366,5.44076501192947,
126.397684762572));
#230355=CARTESIAN_POINT('Ctrl Pts',(-5.71828436490337,5.46677511802796,
126.396251000655));
#230356=CARTESIAN_POINT('Ctrl Pts',(-5.7030394825771,5.48267698615574,126.395372498548));
#230357=CARTESIAN_POINT('Ctrl Pts',(-5.64018706117961,5.54769226704856,
126.3917723908));
#230358=CARTESIAN_POINT('Ctrl Pts',(-5.59200937496956,5.59625150501233,
126.389063644655));
#230359=CARTESIAN_POINT('Ctrl Pts',(-5.28132847130631,5.9013744344875,126.371910686583));
#230360=CARTESIAN_POINT('Ctrl Pts',(-5.00186045676111,6.14003766881747,
126.357914364024));
#230361=CARTESIAN_POINT('Ctrl Pts',(-4.20805161089058,6.72765252395125,
126.321041319045));
#230362=CARTESIAN_POINT('Ctrl Pts',(-3.66760652037844,7.03687367189595,
126.298944615369));
#230363=CARTESIAN_POINT('Ctrl Pts',(-3.03316223698029,7.30675061343535,
126.272497743083));
#230364=CARTESIAN_POINT('Ctrl Pts',(-2.9693473124092,7.33291578826961,126.269830195637));
#230365=CARTESIAN_POINT('Ctrl Pts',(-2.83060933891404,7.38769265284646,
126.264002142958));
#230366=CARTESIAN_POINT('Ctrl Pts',(-2.75557729732104,7.41600601436807,
126.260832426404));
#230367=CARTESIAN_POINT('Ctrl Pts',(-2.66780466630403,7.44761108379233,
126.257092841365));
#230368=CARTESIAN_POINT('Ctrl Pts',(-2.65546900418735,7.45201831440564,
126.256566553534));
#230369=CARTESIAN_POINT('Ctrl Pts',(-2.63579973910678,7.45899062179729,
126.255726168407));
#230370=CARTESIAN_POINT('Ctrl Pts',(-2.62847317615797,7.46157557908572,
126.255412866643));
#230371=CARTESIAN_POINT('Ctrl Pts',(-2.61555026313918,7.46611364464712,
126.254859762644));
#230372=CARTESIAN_POINT('Ctrl Pts',(-2.60995549682393,7.46807126627389,
126.254620143966));
#230373=CARTESIAN_POINT('Ctrl Pts',(-2.59839782086855,7.4721007496869,126.254124798445));
#230374=CARTESIAN_POINT('Ctrl Pts',(-2.59243462225202,7.47417176535386,
126.253869037066));
#230375=CARTESIAN_POINT('Ctrl Pts',(-2.57719177669453,7.47944516079605,
126.253214781764));
#230376=CARTESIAN_POINT('Ctrl Pts',(-2.56790865275239,7.48263740382877,
126.25281586661));
#230377=CARTESIAN_POINT('Ctrl Pts',(-2.53025175244799,7.49550837629793,
126.251195719941));
#230378=CARTESIAN_POINT('Ctrl Pts',(-2.50182925168449,7.50504297860175,
126.249968387091));
#230379=CARTESIAN_POINT('Ctrl Pts',(-1.96233797832857,7.68261535319951,
126.226577702406));
#230380=CARTESIAN_POINT('Ctrl Pts',(-1.43560690508122,7.79821362571434,
126.201763077198));
#230381=CARTESIAN_POINT('Ctrl Pts',(-0.242384383227391,7.93505644900924,
126.146467779436));
#230382=CARTESIAN_POINT('Ctrl Pts',(0.423580290964235,7.92746650860418,
126.116472646456));
#230383=CARTESIAN_POINT('Ctrl Pts',(1.1191512611547,7.83153344762973,126.087793321047));
#230384=CARTESIAN_POINT('Ctrl Pts',(1.15741101766778,7.82597057751608,126.086223319548));
#230385=CARTESIAN_POINT('Ctrl Pts',(1.20974125700984,7.81796974329931,126.084086086151));
#230386=CARTESIAN_POINT('Ctrl Pts',(1.22384786437571,7.81577387235536,126.083510966305));
#230387=CARTESIAN_POINT('Ctrl Pts',(1.24675004053743,7.81214533582886,126.082578889327));
#230388=CARTESIAN_POINT('Ctrl Pts',(1.25554923730463,7.8107359784526,126.082221170149));
#230389=CARTESIAN_POINT('Ctrl Pts',(1.2711831518416,7.80820481069186,126.08158628911));
#230390=CARTESIAN_POINT('Ctrl Pts',(1.2780188052648,7.80708888798852,126.081308934571));
#230391=CARTESIAN_POINT('Ctrl Pts',(1.29236970587251,7.80472674569952,126.08072714508));
#230392=CARTESIAN_POINT('Ctrl Pts',(1.29988463863055,7.80347864470588,126.080422772211));
#230393=CARTESIAN_POINT('Ctrl Pts',(1.31959816694817,7.80017529975924,126.079625070633));
#230394=CARTESIAN_POINT('Ctrl Pts',(1.33179378740152,7.79810229087045,126.079132326472));
#230395=CARTESIAN_POINT('Ctrl Pts',(1.38563700533262,7.78882003769183,126.076960158398));
#230396=CARTESIAN_POINT('Ctrl Pts',(1.42723167206808,7.78130563064428,126.075290803443));
#230397=CARTESIAN_POINT('Ctrl Pts',(1.71886458447717,7.72620273096711,126.063645608632));
#230398=CARTESIAN_POINT('Ctrl Pts',(1.96654838197397,7.66690325542648,126.054068337391));
#230399=CARTESIAN_POINT('Ctrl Pts',(2.49584048831774,7.51283806250312,126.034052310584));
#230400=CARTESIAN_POINT('Ctrl Pts',(2.77584130099618,7.41395125901815,126.023752515233));
#230401=CARTESIAN_POINT('Ctrl Pts',(3.61632879469066,7.06280977758361,125.992773847716));
#230402=CARTESIAN_POINT('Ctrl Pts',(4.15346714379324,6.76089412248895,125.972994549617));
#230403=CARTESIAN_POINT('Ctrl Pts',(4.78049522831162,6.30529257617258,125.944337511789));
#230404=CARTESIAN_POINT('Ctrl Pts',(4.90783321278726,6.2066912423356,125.93818072848));
#230405=CARTESIAN_POINT('Ctrl Pts',(5.04180582154404,6.09625084585802,125.931230435219));
#230406=CARTESIAN_POINT('Ctrl Pts',(5.05152600353584,6.08819885924942,125.930723405208));
#230407=CARTESIAN_POINT('Ctrl Pts',(5.06499450138001,6.0769873895547,125.930016948436));
#230408=CARTESIAN_POINT('Ctrl Pts',(5.06875925986301,6.07384759416623,125.929819052233));
#230409=CARTESIAN_POINT('Ctrl Pts',(5.07523295571971,6.06843834392309,125.92947802287));
#230410=CARTESIAN_POINT('Ctrl Pts',(5.07794329912441,6.06617056631375,125.929335021411));
#230411=CARTESIAN_POINT('Ctrl Pts',(5.0832410797306,6.06173180975138,125.929055065595));
#230412=CARTESIAN_POINT('Ctrl Pts',(5.08582864712844,6.0595609890459,125.928918123732));
#230413=CARTESIAN_POINT('Ctrl Pts',(5.09198807914528,6.05438685417333,125.928591658655));
#230414=CARTESIAN_POINT('Ctrl Pts',(5.09555865380275,6.05138205567481,125.928402016528));
#230415=CARTESIAN_POINT('Ctrl Pts',(5.10646400061859,6.04218822222675,125.927821602148));
#230416=CARTESIAN_POINT('Ctrl Pts',(5.11379011570926,6.03598904515685,125.927430020175));
#230417=CARTESIAN_POINT('Ctrl Pts',(5.13061987867352,6.02169548379129,125.926526672995));
#230418=CARTESIAN_POINT('Ctrl Pts',(5.14011566234969,6.01359192272387,125.926014187021));
#230419=CARTESIAN_POINT('Ctrl Pts',(5.22977800981316,5.93670787657084,125.92114901409));
#230420=CARTESIAN_POINT('Ctrl Pts',(5.30857532463509,5.8663535969376,125.916675488758));
#230421=CARTESIAN_POINT('Ctrl Pts',(5.56386229537344,5.629064390629,125.901596668344));
#230422=CARTESIAN_POINT('Ctrl Pts',(5.73406596567516,5.4555845485758,125.890590673001));
#230423=CARTESIAN_POINT('Ctrl Pts',(6.48542865046835,4.61569677749745,125.838603978893));
#230424=CARTESIAN_POINT('Ctrl Pts',(6.96044867438516,3.86243057686019,125.796530733588));
#230425=CARTESIAN_POINT('Ctrl Pts',(7.3227405149124,2.99408999409558,125.757970640054));
#230426=CARTESIAN_POINT('Ctrl Pts',(7.34390566987932,2.94179422116596,125.755678995068));
#230427=CARTESIAN_POINT('Ctrl Pts',(7.36912031472889,2.87752430720629,125.752899412685));
#230428=CARTESIAN_POINT('Ctrl Pts',(7.37370256471094,2.86576182554553,125.752392199559));
#230429=CARTESIAN_POINT('Ctrl Pts',(7.38122018740419,2.8463269357938,125.751556601288));
#230430=CARTESIAN_POINT('Ctrl Pts',(7.38417178995237,2.83866085635588,125.751227630263));
#230431=CARTESIAN_POINT('Ctrl Pts',(7.38947458345409,2.82482388619503,125.750634983135));
#230432=CARTESIAN_POINT('Ctrl Pts',(7.39182999628302,2.81865462834243,125.750371154981));
#230433=CARTESIAN_POINT('Ctrl Pts',(7.39684247611021,2.80547653121,125.749808457064));
#230434=CARTESIAN_POINT('Ctrl Pts',(7.39949731320232,2.7984668473823,125.749509667759));
#230435=CARTESIAN_POINT('Ctrl Pts',(7.40663135107487,2.77954940353425,125.748704706606));
#230436=CARTESIAN_POINT('Ctrl Pts',(7.41109180531551,2.76763456993157,125.74819920882));
#230437=CARTESIAN_POINT('Ctrl Pts',(7.43274263263046,2.70937289584864,125.745734652526));
#230438=CARTESIAN_POINT('Ctrl Pts',(7.44952727736881,2.66287588808511,125.743790149399));
#230439=CARTESIAN_POINT('Ctrl Pts',(7.52666926068978,2.44273708639808,125.734686542393));
#230440=CARTESIAN_POINT('Ctrl Pts',(7.58139981358505,2.26717819798533,125.727728087577));
#230441=CARTESIAN_POINT('Ctrl Pts',(7.68390267132705,1.89294645775595,125.713428158753));
#230442=CARTESIAN_POINT('Ctrl Pts',(7.73019685524648,1.69400959082773,125.706135425957));
#230443=CARTESIAN_POINT('Ctrl Pts',(7.8906155727032,0.859557701313235,125.676411561693));
#230444=CARTESIAN_POINT('Ctrl Pts',(7.93442306835519,0.213160889392909,
125.655658793264));
#230445=CARTESIAN_POINT('Ctrl Pts',(7.88902818395549,-0.618216988985789,
125.625194202305));
#230446=CARTESIAN_POINT('Ctrl Pts',(7.87219328848059,-0.804687226644158,
125.618097166479));
#230447=CARTESIAN_POINT('Ctrl Pts',(7.84712950857229,-1.00331938405422,
125.610084652234));
#230448=CARTESIAN_POINT('Ctrl Pts',(7.84546374974153,-1.01626269274336,
125.609560462585));
#230449=CARTESIAN_POINT('Ctrl Pts',(7.84310285809497,-1.03425554626636,
125.608828850098));
#230450=CARTESIAN_POINT('Ctrl Pts',(7.84243489118831,-1.039308402198,125.608623076003));
#230451=CARTESIAN_POINT('Ctrl Pts',(7.84127352707207,-1.04802870538149,
125.608267401965));
#230452=CARTESIAN_POINT('Ctrl Pts',(7.84078243810846,-1.05169646372878,
125.608117638843));
#230453=CARTESIAN_POINT('Ctrl Pts',(7.83976133595189,-1.05928222254363,
125.607807551754));
#230454=CARTESIAN_POINT('Ctrl Pts',(7.83923095876655,-1.06320017244497,
125.60764720639));
#230455=CARTESIAN_POINT('Ctrl Pts',(7.83800044054134,-1.07223915677601,
125.607276844314));
#230456=CARTESIAN_POINT('Ctrl Pts',(7.83729821802299,-1.07735990123007,
125.607066706063));
#230457=CARTESIAN_POINT('Ctrl Pts',(7.83506463134977,-1.09352990539793,
125.606402135226));
#230458=CARTESIAN_POINT('Ctrl Pts',(7.83351492122607,-1.10457657404098,
125.605946641682));
#230459=CARTESIAN_POINT('Ctrl Pts',(7.82985426549375,-1.13027532998632,
125.604883588209));
#230460=CARTESIAN_POINT('Ctrl Pts',(7.82772555260544,-1.1449248044948,125.604275023228));
#230461=CARTESIAN_POINT('Ctrl Pts',(7.80588674127882,-1.29230798273358,
125.598127122476));
#230462=CARTESIAN_POINT('Ctrl Pts',(7.78284450949898,-1.42451936879187,
125.592405240124));
#230463=CARTESIAN_POINT('Ctrl Pts',(7.71766242252076,-1.74942798209611,
125.577936324642));
#230464=CARTESIAN_POINT('Ctrl Pts',(7.6716576810272,-1.94125538724996,125.569036602514));
#230465=CARTESIAN_POINT('Ctrl Pts',(7.61139715877473,-2.15667724440141,
125.558775271194));
#230466=CARTESIAN_POINT('Ctrl Pts',(7.60412911015608,-2.18216495924209,
125.557556878738));
#230467=CARTESIAN_POINT('Ctrl Pts',(7.33933782944703,-3.09335109922466,
125.513854436762));
#230468=CARTESIAN_POINT('Ctrl Pts',(6.92890690384614,-3.92756140772201,
125.470039969002));
#230469=CARTESIAN_POINT('Ctrl Pts',(6.34918129601219,-4.71966878076143,
125.429720159627));
#230470=CARTESIAN_POINT('Ctrl Pts',(6.31393553024771,-4.76671740775451,
125.427326073275));
#230471=CARTESIAN_POINT('Ctrl Pts',(6.26993631507333,-4.82410640934887,
125.424406056187));
#230472=CARTESIAN_POINT('Ctrl Pts',(6.26167694933377,-4.83482221269164,
125.423860833575));
#230473=CARTESIAN_POINT('Ctrl Pts',(6.24795055717997,-4.8525368318491,125.422959510497));
#230474=CARTESIAN_POINT('Ctrl Pts',(6.24249917792306,-4.85954770361516,
125.422602796284));
#230475=CARTESIAN_POINT('Ctrl Pts',(6.23261263798222,-4.87221842786834,
125.421958103453));
#230476=CARTESIAN_POINT('Ctrl Pts',(6.22818154835895,-4.87788143613881,
125.421669965117));
#230477=CARTESIAN_POINT('Ctrl Pts',(6.21866957763577,-4.89000380598412,
125.421053162674));
#230478=CARTESIAN_POINT('Ctrl Pts',(6.21358633757495,-4.89646131041344,
125.420724592106));
#230479=CARTESIAN_POINT('Ctrl Pts',(6.1997614458816,-4.91396759303291,125.419833820536));
#230480=CARTESIAN_POINT('Ctrl Pts',(6.19100030819866,-4.92500098250914,
125.419272390178));
#230481=CARTESIAN_POINT('Ctrl Pts',(6.14695158364825,-4.98017072500174,
125.416464940225));
#230482=CARTESIAN_POINT('Ctrl Pts',(6.11122088074866,-5.02395200349827,
125.414236534867));
#230483=CARTESIAN_POINT('Ctrl Pts',(5.7011711531951,-5.51554290317883,125.389199272512));
#230484=CARTESIAN_POINT('Ctrl Pts',(5.27884737525716,-5.92101422831183,
125.368570731182));
#230485=CARTESIAN_POINT('Ctrl Pts',(4.62759298230258,-6.42071255103389,
125.340091601594));
#230486=CARTESIAN_POINT('Ctrl Pts',(4.43304170897174,-6.55654676419223,
125.331916077587));
#230487=CARTESIAN_POINT('Ctrl Pts',(3.9029302434727,-6.89227159343943,125.309869422917));
#230488=CARTESIAN_POINT('Ctrl Pts',(3.55816876208995,-7.07642026883306,
125.295702547856));
#230489=CARTESIAN_POINT('Ctrl Pts',(3.17654355457447,-7.24528948411616,
125.279114606962));
#230490=CARTESIAN_POINT('Ctrl Pts',(3.15182002323524,-7.25607877455861,
125.278037265548));
#230491=CARTESIAN_POINT('Ctrl Pts',(3.11829418162056,-7.27050569708356,
125.276573105993));
#230492=CARTESIAN_POINT('Ctrl Pts',(3.10953961624805,-7.2742542620215,125.276190472615));
#230493=CARTESIAN_POINT('Ctrl Pts',(3.09472605600223,-7.28056556300747,
125.275542535977));
#230494=CARTESIAN_POINT('Ctrl Pts',(3.08867058271744,-7.28313657088273,
125.275277536421));
#230495=CARTESIAN_POINT('Ctrl Pts',(3.07653209712454,-7.28827241785366,
125.274746066624));
#230496=CARTESIAN_POINT('Ctrl Pts',(3.07044906753319,-7.29083720191749,
125.274479594698));
#230497=CARTESIAN_POINT('Ctrl Pts',(3.05672608281624,-7.29660299523593,
125.273878156989));
#230498=CARTESIAN_POINT('Ctrl Pts',(3.04908430099351,-7.29979962329984,
125.273543036924));
#230499=CARTESIAN_POINT('Ctrl Pts',(3.0330918954078,-7.30645990092626,125.272841302842));
#230500=CARTESIAN_POINT('Ctrl Pts',(3.02474032887015,-7.30992124937225,
125.272474610134));
#230501=CARTESIAN_POINT('Ctrl Pts',(3.00290228599648,-7.31892830274964,
125.271515185256));
#230502=CARTESIAN_POINT('Ctrl Pts',(2.98940640453432,-7.32445103647046,
125.270921684209));
#230503=CARTESIAN_POINT('Ctrl Pts',(2.94924672293705,-7.3407555450251,125.269154013925));
#230504=CARTESIAN_POINT('Ctrl Pts',(2.92253943223886,-7.35142921142041,
125.267976386931));
#230505=CARTESIAN_POINT('Ctrl Pts',(2.60007143107992,-7.47826976341001,
125.25373636806));
#230506=CARTESIAN_POINT('Ctrl Pts',(2.29763746982637,-7.57665751945182,
125.240181771873));
#230507=CARTESIAN_POINT('Ctrl Pts',(1.45057484115349,-7.79682816944643,
125.202597374796));
#230508=CARTESIAN_POINT('Ctrl Pts',(0.897688609357691,-7.87965090294242,
125.178601302641));
#230509=CARTESIAN_POINT('Ctrl Pts',(0.0971795667018823,-7.91415727650146,
125.145046872331));
#230510=CARTESIAN_POINT('Ctrl Pts',(-0.146689868489533,-7.91339462922862,
125.134955670431));
#230511=CARTESIAN_POINT('Ctrl Pts',(-0.64365607723417,-7.88885644262455,
125.114465558586));
#230512=CARTESIAN_POINT('Ctrl Pts',(-0.896429603056834,-7.86414441545999,
125.104070149568));
#230513=CARTESIAN_POINT('Ctrl Pts',(-1.18672555369331,-7.82158352019872,
125.092194347674));
#230514=CARTESIAN_POINT('Ctrl Pts',(-1.22582750031856,-7.81555073313311,
125.090595930217));
#230515=CARTESIAN_POINT('Ctrl Pts',(-1.28971095214331,-7.80520334624525,
125.087986425344));
#230516=CARTESIAN_POINT('Ctrl Pts',(-1.31451996793325,-7.80106344515821,
125.086973507251));
#230517=CARTESIAN_POINT('Ctrl Pts',(-1.35899786597839,-7.79342318211579,
125.085158363482));
#230518=CARTESIAN_POINT('Ctrl Pts',(-1.37867401338701,-7.78996649946024,
125.084355670738));
#230519=CARTESIAN_POINT('Ctrl Pts',(-1.42049180787295,-7.78245659765812,
125.082650299644));
#230520=CARTESIAN_POINT('Ctrl Pts',(-1.44262968623985,-7.77838333221277,
125.081747850522));
#230521=CARTESIAN_POINT('Ctrl Pts',(-1.50213999685694,-7.76717091840272,
125.079322818319));
#230522=CARTESIAN_POINT('Ctrl Pts',(-1.53947888135586,-7.75985653464033,
125.077802227096));
#230523=CARTESIAN_POINT('Ctrl Pts',(-1.72718887287239,-7.72167750091729,
125.070162110732));
#230524=CARTESIAN_POINT('Ctrl Pts',(-1.87669336224166,-7.68670983110924,
125.064091345553));
#230525=CARTESIAN_POINT('Ctrl Pts',(-2.30394429057833,-7.5735708609033,
125.046743009256));
#230526=CARTESIAN_POINT('Ctrl Pts',(-2.57855601481965,-7.48452993172522,
125.035599852609));
#230527=CARTESIAN_POINT('Ctrl Pts',(-3.08357957310658,-7.28967647439913,
125.014780023421));
#230528=CARTESIAN_POINT('Ctrl Pts',(-3.31496465206026,-7.1874093931488,
125.005102184807));
#230529=CARTESIAN_POINT('Ctrl Pts',(-3.73716307085386,-6.97607543468883,
124.98682640429));
#230530=CARTESIAN_POINT('Ctrl Pts',(-3.9291014515391,-6.86980152526605,
124.978262080794));
#230531=CARTESIAN_POINT('Ctrl Pts',(-4.13703042743721,-6.74310651858173,
124.9685227118));
#230532=CARTESIAN_POINT('Ctrl Pts',(-4.15763202068206,-6.73042363120194,
124.96755251749));
#230533=CARTESIAN_POINT('Ctrl Pts',(-4.1885546364534,-6.71119068935444,
124.966088102444));
#230534=CARTESIAN_POINT('Ctrl Pts',(-4.19891916745838,-6.7047108987106,
124.96559588623));
#230535=CARTESIAN_POINT('Ctrl Pts',(-4.21741437817623,-6.69308819004384,
124.964715104109));
#230536=CARTESIAN_POINT('Ctrl Pts',(-4.22555078204119,-6.6879544065977,
124.964326785112));
#230537=CARTESIAN_POINT('Ctrl Pts',(-4.24322686942633,-6.67675628701435,
124.963481350817));
#230538=CARTESIAN_POINT('Ctrl Pts',(-4.25276295636639,-6.67068632283051,
124.963024088149));
#230539=CARTESIAN_POINT('Ctrl Pts',(-4.27808715726214,-6.6544904443003,
124.961806724255));
#230540=CARTESIAN_POINT('Ctrl Pts',(-4.29385229608871,-6.64432880384139,
124.961045714642));
#230541=CARTESIAN_POINT('Ctrl Pts',(-4.36754330930282,-6.59645842799155,
124.957473969921));
#230542=CARTESIAN_POINT('Ctrl Pts',(-4.4250090261526,-6.5580479782329,124.954646380474));
#230543=CARTESIAN_POINT('Ctrl Pts',(-4.58510779903765,-6.44797450463757,
124.94665712134));
#230544=CARTESIAN_POINT('Ctrl Pts',(-4.68655337529715,-6.37462198529496,
124.941463532283));
#230545=CARTESIAN_POINT('Ctrl Pts',(-5.10302764582345,-6.05816404192636,
124.919648133921));
#230546=CARTESIAN_POINT('Ctrl Pts',(-5.4012281631724,-5.79387438274418,
124.902838930953));
#230547=CARTESIAN_POINT('Ctrl Pts',(-5.845150387183,-5.33625109209956,124.876237546936));
#230548=CARTESIAN_POINT('Ctrl Pts',(-6.00412150467398,-5.15673226477471,
124.866320311031));
#230549=CARTESIAN_POINT('Ctrl Pts',(-6.22816821441472,-4.87929461809403,
124.85172904736));
#230550=CARTESIAN_POINT('Ctrl Pts',(-6.29961111500287,-4.78669986413973,
124.84697174565));
#230551=CARTESIAN_POINT('Ctrl Pts',(-6.39291386402894,-4.66006458744514,
124.84060828002));
#230552=CARTESIAN_POINT('Ctrl Pts',(-6.4166030629926,-4.62739179070427,
124.838978869244));
#230553=CARTESIAN_POINT('Ctrl Pts',(-6.45360327963279,-4.57552958646275,
124.836411546804));
#230554=CARTESIAN_POINT('Ctrl Pts',(-6.46708105707976,-4.55646012739608,
124.835471578598));
#230555=CARTESIAN_POINT('Ctrl Pts',(-6.49300110364074,-4.51943964445777,
124.833654425817));
#230556=CARTESIAN_POINT('Ctrl Pts',(-6.50545385162708,-4.50149622006467,
124.83277712069));
#230557=CARTESIAN_POINT('Ctrl Pts',(-6.53495007711042,-4.45861646415103,
124.830688686846));
#230558=CARTESIAN_POINT('Ctrl Pts',(-6.5519253836605,-4.43363361811748,
124.829478377923));
#230559=CARTESIAN_POINT('Ctrl Pts',(-6.60258213841443,-4.35815492018115,
124.825840736919));
#230560=CARTESIAN_POINT('Ctrl Pts',(-6.63582601931868,-4.30736790917346,
124.823418461358));
#230561=CARTESIAN_POINT('Ctrl Pts',(-6.86437293930103,-3.94928794181919,
124.806507319531));
#230562=CARTESIAN_POINT('Ctrl Pts',(-7.03884933118497,-3.62920176066911,
124.79218606703));
#230563=CARTESIAN_POINT('Ctrl Pts',(-7.2831758316515,-3.09653266062842,
124.769528622915));
#230564=CARTESIAN_POINT('Ctrl Pts',(-7.36716716733706,-2.89102336224576,
124.761060749494));
#230565=CARTESIAN_POINT('Ctrl Pts',(-7.65413306094499,-2.09478266867559,
124.7291235553));
#230566=CARTESIAN_POINT('Ctrl Pts',(-7.79554110652291,-1.48435692690218,
124.706647573883));
#230567=CARTESIAN_POINT('Ctrl Pts',(-7.867901392112,-0.825543785212832,
124.681116428796));
#230568=CARTESIAN_POINT('Ctrl Pts',(-7.87181494712228,-0.787352686920916,
124.679630987546));
#230569=CARTESIAN_POINT('Ctrl Pts',(-7.88413564961273,-0.657828510897786,
124.67457114074));
#230570=CARTESIAN_POINT('Ctrl Pts',(-7.89123225152605,-0.566379839892654,
124.670961737013));
#230571=CARTESIAN_POINT('Ctrl Pts',(-7.89757522177108,-0.460892176095586,
124.66673776609));
#230572=CARTESIAN_POINT('Ctrl Pts',(-7.89837642923913,-0.446951631147566,
124.666178337471));
#230573=CARTESIAN_POINT('Ctrl Pts',(-7.89958770502583,-0.424855009915973,
124.665289590344));
#230574=CARTESIAN_POINT('Ctrl Pts',(-7.90002206211765,-0.416700259522344,
124.664961162986));
#230575=CARTESIAN_POINT('Ctrl Pts',(-7.90075589471278,-0.402509399242728,
124.664388857424));
#230576=CARTESIAN_POINT('Ctrl Pts',(-7.90106108202511,-0.396473583194797,
124.664145193218));
#230577=CARTESIAN_POINT('Ctrl Pts',(-7.90163835793126,-0.384791136831793,
124.663673093381));
#230578=CARTESIAN_POINT('Ctrl Pts',(-7.90191131102326,-0.379144551623895,
124.66344469075));
#230579=CARTESIAN_POINT('Ctrl Pts',(-7.90247644215173,-0.367187939756693,
124.662960579307));
#230580=CARTESIAN_POINT('Ctrl Pts',(-7.90276711538835,-0.360877848446002,
124.662704812686));
#230581=CARTESIAN_POINT('Ctrl Pts',(-7.90344019104552,-0.345875481302911,
124.662096050663));
#230582=CARTESIAN_POINT('Ctrl Pts',(-7.90381581133093,-0.337182920321436,
124.661742790166));
#230583=CARTESIAN_POINT('Ctrl Pts',(-7.90477362281569,-0.314135897118142,
124.660804714397));
#230584=CARTESIAN_POINT('Ctrl Pts',(-7.90533105252766,-0.299780479742971,
124.660218910609));
#230585=CARTESIAN_POINT('Ctrl Pts',(-7.90928581584208,-0.190238895561674,
124.655736901715));
#230586=CARTESIAN_POINT('Ctrl Pts',(-7.91100275360645,-0.0950102628663944,
124.6517680464));
#230587=CARTESIAN_POINT('Ctrl Pts',(-7.9109999966855,0.000229002203636593,
124.647722132928));
#230588=CARTESIAN_POINT('',(-7.91099929352038,0.00334333966528006,120.642331508237));
#230589=CARTESIAN_POINT('Ctrl Pts',(-7.9109999968515,0.000223194498397833,
124.647722379649));
#230590=CARTESIAN_POINT('Ctrl Pts',(-7.9109779547213,0.781493759624896,
124.614532803849));
#230591=CARTESIAN_POINT('Ctrl Pts',(-7.79522920292053,1.55848580366607,
124.577023027943));
#230592=CARTESIAN_POINT('Ctrl Pts',(-7.47181302200089,2.61985210386416,
124.527212159827));
#230593=CARTESIAN_POINT('Ctrl Pts',(-7.35671161125456,2.92753127098832,
124.512897498815));
#230594=CARTESIAN_POINT('Ctrl Pts',(-7.21432761035792,3.24620264622964,
124.498308490905));
#230595=CARTESIAN_POINT('Ctrl Pts',(-7.20575912924286,3.26517838250959,
124.497440615841));
#230596=CARTESIAN_POINT('Ctrl Pts',(-7.15602231928925,3.3741760935384,124.492460348662));
#230597=CARTESIAN_POINT('Ctrl Pts',(-7.11324132989328,3.46345469444898,
124.488400335366));
#230598=CARTESIAN_POINT('Ctrl Pts',(-7.06108777803045,3.56724754729824,
124.483701071417));
#230599=CARTESIAN_POINT('Ctrl Pts',(-7.05333057653428,3.58256101908969,
124.483008281119));
#230600=CARTESIAN_POINT('Ctrl Pts',(-7.04138885304668,3.6059460166166,124.48195112539));
#230601=CARTESIAN_POINT('Ctrl Pts',(-7.03724018074677,3.6140357349824,124.481585562906));
#230602=CARTESIAN_POINT('Ctrl Pts',(-7.02966017629616,3.62875385151286,
124.480920734683));
#230603=CARTESIAN_POINT('Ctrl Pts',(-7.02623339412023,3.63538457398943,
124.480621317035));
#230604=CARTESIAN_POINT('Ctrl Pts',(-7.01881700278139,3.64968541504211,
124.479975753209));
#230605=CARTESIAN_POINT('Ctrl Pts',(-7.01482419166842,3.65735386691965,
124.479629715001));
#230606=CARTESIAN_POINT('Ctrl Pts',(-7.00399690581999,3.67806541196798,
124.478695450042));
#230607=CARTESIAN_POINT('Ctrl Pts',(-6.99713855775811,3.69109602121912,
124.478108026931));
#230608=CARTESIAN_POINT('Ctrl Pts',(-6.965027527371,3.75169467706055,124.47537788186));
#230609=CARTESIAN_POINT('Ctrl Pts',(-6.93932564449243,3.79902370942493,
124.473250351369));
#230610=CARTESIAN_POINT('Ctrl Pts',(-6.49044987221057,4.60585462122559,
124.437052605469));
#230611=CARTESIAN_POINT('Ctrl Pts',(-5.94546002243732,5.29068073938031,
124.408192297818));
#230612=CARTESIAN_POINT('Ctrl Pts',(-5.15244489468381,6.00630827580459,
124.370743145328));
#230613=CARTESIAN_POINT('Ctrl Pts',(-4.99992161593218,6.13385737063263,
124.363667144406));
#230614=CARTESIAN_POINT('Ctrl Pts',(-4.72974173976885,6.34301926840573,
124.351086125048));
#230615=CARTESIAN_POINT('Ctrl Pts',(-4.61437451620979,6.42743299954095,
124.345700058648));
#230616=CARTESIAN_POINT('Ctrl Pts',(-4.46187281779876,6.53279519216821,
124.338487462888));
#230617=CARTESIAN_POINT('Ctrl Pts',(-4.42676342051837,6.55663691562303,
124.336820743516));
#230618=CARTESIAN_POINT('Ctrl Pts',(-4.37620780220931,6.59037652112767,
124.334409797168));
#230619=CARTESIAN_POINT('Ctrl Pts',(-4.36091630829756,6.60050500807277,
124.333679174745));
#230620=CARTESIAN_POINT('Ctrl Pts',(-4.33734526110926,6.61599988151902,
124.332551005164));
#230621=CARTESIAN_POINT('Ctrl Pts',(-4.32909058793893,6.62140415821417,
124.332155549122));
#230622=CARTESIAN_POINT('Ctrl Pts',(-4.31370567184137,6.63143548764466,
124.331417855976));
#230623=CARTESIAN_POINT('Ctrl Pts',(-4.3065780317186,6.63606652362331,124.331075833448));
#230624=CARTESIAN_POINT('Ctrl Pts',(-4.29486682013669,6.64364882548795,
124.330513460949));
#230625=CARTESIAN_POINT('Ctrl Pts',(-4.290287624824,6.64660686479829,124.330293466414));
#230626=CARTESIAN_POINT('Ctrl Pts',(-4.28150357158588,6.65226827146771,
124.329871272427));
#230627=CARTESIAN_POINT('Ctrl Pts',(-4.27729920021973,6.65497239218263,
124.329669112033));
#230628=CARTESIAN_POINT('Ctrl Pts',(-4.26754069604263,6.66123569045777,
124.329199703399));
#230629=CARTESIAN_POINT('Ctrl Pts',(-4.2619846737903,6.66479190644462,124.328932304617));
#230630=CARTESIAN_POINT('Ctrl Pts',(-4.24466179740084,6.675849155748,124.328098173599));
#230631=CARTESIAN_POINT('Ctrl Pts',(-4.23287958013209,6.68332598196764,
124.327530233364));
#230632=CARTESIAN_POINT('Ctrl Pts',(-4.14063557463364,6.74152093161513,
124.32307945167));
#230633=CARTESIAN_POINT('Ctrl Pts',(-4.05928678219419,6.79081418519741,
124.319128777842));
#230634=CARTESIAN_POINT('Ctrl Pts',(-3.73132011221571,6.9815464442122,124.303158560153));
#230635=CARTESIAN_POINT('Ctrl Pts',(-3.47805134277313,7.11111020427043,
124.290740059382));
#230636=CARTESIAN_POINT('Ctrl Pts',(-2.98296903435455,7.33159058642938,
124.266910467727));
#230637=CARTESIAN_POINT('Ctrl Pts',(-2.74258321459801,7.42486126728823,
124.255526911098));
#230638=CARTESIAN_POINT('Ctrl Pts',(-2.03509896471989,7.66031191385824,
124.222969203287));
#230639=CARTESIAN_POINT('Ctrl Pts',(-1.55883606936582,7.77123575444322,
124.20228203286));
#230640=CARTESIAN_POINT('Ctrl Pts',(-1.03333637487193,7.84333703034172,
124.180773679725));
#230641=CARTESIAN_POINT('Ctrl Pts',(-0.991271441883657,7.84876428529563,
124.179060209349));
#230642=CARTESIAN_POINT('Ctrl Pts',(-0.9313419451915,7.85600696723329,124.176630097689));
#230643=CARTESIAN_POINT('Ctrl Pts',(-0.913511921898627,7.85810023222889,
124.175908488046));
#230644=CARTESIAN_POINT('Ctrl Pts',(-0.882750407504784,7.86160555670332,
124.174665849921));
#230645=CARTESIAN_POINT('Ctrl Pts',(-0.869822295907359,7.86304644433966,
124.174144316529));
#230646=CARTESIAN_POINT('Ctrl Pts',(-0.84507559853392,7.86574278030027,
124.173147336595));
#230647=CARTESIAN_POINT('Ctrl Pts',(-0.833257626124414,7.86700349449899,
124.172671800173));
#230648=CARTESIAN_POINT('Ctrl Pts',(-0.805567205088771,7.86989434924505,
124.171558909382));
#230649=CARTESIAN_POINT('Ctrl Pts',(-0.789692563204766,7.87150311235881,
124.170921921583));
#230650=CARTESIAN_POINT('Ctrl Pts',(-0.73485975367032,7.87689241808011,
124.168725115327));
#230651=CARTESIAN_POINT('Ctrl Pts',(-0.695878252535864,7.88043187326883,
124.167169290571));
#230652=CARTESIAN_POINT('Ctrl Pts',(-0.311668414623715,7.91244441285793,
124.151889982918));
#230653=CARTESIAN_POINT('Ctrl Pts',(0.0350609493567653,7.91850381125998,
124.138565662273));
#230654=CARTESIAN_POINT('Ctrl Pts',(0.889346997484526,7.87730375127847,
124.106403859199));
#230655=CARTESIAN_POINT('Ctrl Pts',(1.39404755510762,7.80381155641685,124.088030599812));
#230656=CARTESIAN_POINT('Ctrl Pts',(2.10999840140295,7.62784379124977,124.06061675839));
#230657=CARTESIAN_POINT('Ctrl Pts',(2.32933896935196,7.56374687982564,124.052011594808));
#230658=CARTESIAN_POINT('Ctrl Pts',(2.63316213845387,7.46049145608525,124.03951493596));
#230659=CARTESIAN_POINT('Ctrl Pts',(2.72020353117039,7.4291969675305,124.035866151867));
#230660=CARTESIAN_POINT('Ctrl Pts',(2.81980195693749,7.39140278156724,124.031594659746));
#230661=CARTESIAN_POINT('Ctrl Pts',(2.83291644346128,7.38638630027789,124.031030275854));
#230662=CARTESIAN_POINT('Ctrl Pts',(2.85267824203587,7.37876675394805,124.030176814855));
#230663=CARTESIAN_POINT('Ctrl Pts',(2.85933553844508,7.37618954745027,124.029888787257));
#230664=CARTESIAN_POINT('Ctrl Pts',(2.87133338504519,7.37152619648332,124.02936875746));
#230665=CARTESIAN_POINT('Ctrl Pts',(2.87667517788921,7.36944324859127,124.029136887228));
#230666=CARTESIAN_POINT('Ctrl Pts',(2.88798910528333,7.36501738514403,124.028645062199));
#230667=CARTESIAN_POINT('Ctrl Pts',(2.89396066149947,7.36267300951799,124.028385046485));
#230668=CARTESIAN_POINT('Ctrl Pts',(2.90962676414748,7.35650064441232,124.027701771248));
#230669=CARTESIAN_POINT('Ctrl Pts',(2.91931658906666,7.35266076256004,124.027278007647));
#230670=CARTESIAN_POINT('Ctrl Pts',(2.95992905620287,7.3364739242029,124.025497021018));
#230671=CARTESIAN_POINT('Ctrl Pts',(2.99078087645229,7.32395107571189,124.024132168789));
#230672=CARTESIAN_POINT('Ctrl Pts',(3.49425201402917,7.11587889232877,124.001652450288));
#230673=CARTESIAN_POINT('Ctrl Pts',(3.94679577579872,6.87518143711971,123.9781489169));
#230674=CARTESIAN_POINT('Ctrl Pts',(4.76057938958845,6.33539835606597,123.933187011665));
#230675=CARTESIAN_POINT('Ctrl Pts',(5.12488966443246,6.0444985594457,123.911859840813));
#230676=CARTESIAN_POINT('Ctrl Pts',(5.58444055249789,5.60596157415513,123.884324687986));
#230677=CARTESIAN_POINT('Ctrl Pts',(5.70353818750872,5.48474596580471,123.877113003325));
#230678=CARTESIAN_POINT('Ctrl Pts',(5.87833219753157,5.2949875045911,123.8664224604));
#230679=CARTESIAN_POINT('Ctrl Pts',(5.93693356543073,5.22919712920106,123.862818594296));
#230680=CARTESIAN_POINT('Ctrl Pts',(6.00465085098008,5.15056644532237,123.858629551144));
#230681=CARTESIAN_POINT('Ctrl Pts',(6.01484129881088,5.1386623457643,123.857998486431));
#230682=CARTESIAN_POINT('Ctrl Pts',(6.03040433910354,5.12037246166174,123.857033660691));
#230683=CARTESIAN_POINT('Ctrl Pts',(6.03580227994053,5.11400835717489,123.856698821679));
#230684=CARTESIAN_POINT('Ctrl Pts',(6.04519873533077,5.10289445301531,123.856115607461));
#230685=CARTESIAN_POINT('Ctrl Pts',(6.04920174194431,5.09814847113668,123.855867041629));
#230686=CARTESIAN_POINT('Ctrl Pts',(6.05755991692645,5.08821527917915,123.855347812337));
#230687=CARTESIAN_POINT('Ctrl Pts',(6.06191402042494,5.08302717715645,123.855077194077));
#230688=CARTESIAN_POINT('Ctrl Pts',(6.07393722820976,5.06866358640106,123.85432955633));
#230689=CARTESIAN_POINT('Ctrl Pts',(6.08159221362435,5.05947627261939,123.853853134371));
#230690=CARTESIAN_POINT('Ctrl Pts',(6.11153404319872,5.02337473353192,123.85198800684));
#230691=CARTESIAN_POINT('Ctrl Pts',(6.13366345153975,4.99633013108507,123.850605943454));
#230692=CARTESIAN_POINT('Ctrl Pts',(6.48879128108573,4.55640899259165,123.828366083917));
#230693=CARTESIAN_POINT('Ctrl Pts',(6.77962536888392,4.11120925782116,123.809411418267));
#230694=CARTESIAN_POINT('Ctrl Pts',(7.15889177034146,3.37941764166433,123.781259172598));
#230695=CARTESIAN_POINT('Ctrl Pts',(7.27941941898504,3.11130978001857,123.771475590845));
#230696=CARTESIAN_POINT('Ctrl Pts',(7.49529320832895,2.54941108509627,123.751162180277));
#230697=CARTESIAN_POINT('Ctrl Pts',(7.58891455534187,2.25549864566818,123.740634500011));
#230698=CARTESIAN_POINT('Ctrl Pts',(7.71082118838906,1.77799031810052,123.72271601438));
#230699=CARTESIAN_POINT('Ctrl Pts',(7.75021433846112,1.59755505973086,123.715762995025));
#230700=CARTESIAN_POINT('Ctrl Pts',(7.78799888847079,1.38985472168838,123.707391889824));
#230701=CARTESIAN_POINT('Ctrl Pts',(7.79260947140494,1.3637669990782,123.706333879372));
#230702=CARTESIAN_POINT('Ctrl Pts',(7.79827583549108,1.33073824266183,123.704985528162));
#230703=CARTESIAN_POINT('Ctrl Pts',(7.79945357933817,1.32381801619597,123.704702529612));
#230704=CARTESIAN_POINT('Ctrl Pts',(7.80121165741433,1.31340405786741,123.704275907768));
#230705=CARTESIAN_POINT('Ctrl Pts',(7.80179886163868,1.30991147237225,123.704132702567));
#230706=CARTESIAN_POINT('Ctrl Pts',(7.80293527413752,1.30312442336521,123.70385416754));
#230707=CARTESIAN_POINT('Ctrl Pts',(7.80348474189081,1.2998300035608,123.703718853636));
#230708=CARTESIAN_POINT('Ctrl Pts',(7.80463071578757,1.2929322218325,123.703435296959));
#230709=CARTESIAN_POINT('Ctrl Pts',(7.80522681294202,1.28932879379447,123.703287029064));
#230710=CARTESIAN_POINT('Ctrl Pts',(7.80669366051943,1.28042335202764,123.702920262012));
#230711=CARTESIAN_POINT('Ctrl Pts',(7.80756150178545,1.27512088247368,123.702701583056));
#230712=CARTESIAN_POINT('Ctrl Pts',(7.81100622341778,1.25393843247833,123.701826816964));
#230713=CARTESIAN_POINT('Ctrl Pts',(7.81354004740365,1.23805158810275,123.701168091365));
#230714=CARTESIAN_POINT('Ctrl Pts',(7.85521455938794,0.971531837579941,
123.690074249616));
#230715=CARTESIAN_POINT('Ctrl Pts',(7.88232314874255,0.71918660285763,123.678936860042));
#230716=CARTESIAN_POINT('Ctrl Pts',(7.9375050194115,-0.21597568715271,123.63651840214));
#230717=CARTESIAN_POINT('Ctrl Pts',(7.8892490030556,-0.900315089013139,
123.603552535456));
#230718=CARTESIAN_POINT('Ctrl Pts',(7.7043471289416,-1.81346362295349,123.562112929261));
#230719=CARTESIAN_POINT('Ctrl Pts',(7.64361287548753,-2.0544616709585,123.551387302088));
#230720=CARTESIAN_POINT('Ctrl Pts',(7.54183995843612,-2.39063690095441,
123.536772056054));
#230721=CARTESIAN_POINT('Ctrl Pts',(7.51012847813366,-2.48846662142211,
123.532560418863));
#230722=CARTESIAN_POINT('Ctrl Pts',(7.47134590554917,-2.6006079590647,123.52777847616));
#230723=CARTESIAN_POINT('Ctrl Pts',(7.46612908571469,-2.61554733786892,
123.527142371222));
#230724=CARTESIAN_POINT('Ctrl Pts',(7.45815127397746,-2.63817499481411,
123.526180316297));
#230725=CARTESIAN_POINT('Ctrl Pts',(7.45542315605889,-2.64587476904186,
123.525853194773));
#230726=CARTESIAN_POINT('Ctrl Pts',(7.45048961413376,-2.65973086484823,
123.525264968006));
#230727=CARTESIAN_POINT('Ctrl Pts',(7.44828847559589,-2.66588869766385,
123.525003710119));
#230728=CARTESIAN_POINT('Ctrl Pts',(7.44354431968846,-2.67910905091557,
123.524443148316));
#230729=CARTESIAN_POINT('Ctrl Pts',(7.44099887945694,-2.68617069863672,
123.52414393127));
#230730=CARTESIAN_POINT('Ctrl Pts',(7.43409569635163,-2.7052366384214,123.523336621567));
#230731=CARTESIAN_POINT('Ctrl Pts',(7.42971892115776,-2.71723404348389,
123.522829209811));
#230732=CARTESIAN_POINT('Ctrl Pts',(7.41015062029799,-2.77047296015645,
123.520580158316));
#230733=CARTESIAN_POINT('Ctrl Pts',(7.39464447526628,-2.81159844346842,
123.51884979564));
#230734=CARTESIAN_POINT('Ctrl Pts',(7.1417046519609,-3.4658773384298,123.491426009096));
#230735=CARTESIAN_POINT('Ctrl Pts',(6.82906537484602,-4.04724494525259,
123.468859418155));
#230736=CARTESIAN_POINT('Ctrl Pts',(6.21542807790977,-4.91056682792052,
123.43287648409));
#230737=CARTESIAN_POINT('Ctrl Pts',(5.95818056363805,-5.21969881286509,
123.419283873117));
#230738=CARTESIAN_POINT('Ctrl Pts',(5.57157553089353,-5.61828229777972,
123.398802386977));
#230739=CARTESIAN_POINT('Ctrl Pts',(5.46136432201779,-5.72547329681315,
123.392954751863));
#230740=CARTESIAN_POINT('Ctrl Pts',(5.33654046893791,-5.83999171455548,
123.386225414379));
#230741=CARTESIAN_POINT('Ctrl Pts',(5.32494217755777,-5.85056904937764,
123.385599160833));
#230742=CARTESIAN_POINT('Ctrl Pts',(5.30734593751664,-5.86652068581035,
123.384647420858));
#230743=CARTESIAN_POINT('Ctrl Pts',(5.30137108343511,-5.87192051148682,
123.384323971569));
#230744=CARTESIAN_POINT('Ctrl Pts',(5.29027343966927,-5.88191935738502,
123.383722659039));
#230745=CARTESIAN_POINT('Ctrl Pts',(5.28515291475787,-5.88652079417768,
123.383444999238));
#230746=CARTESIAN_POINT('Ctrl Pts',(5.2769033003488,-5.89391467089273,123.382997336465));
#230747=CARTESIAN_POINT('Ctrl Pts',(5.27377797509923,-5.89671132566469,
123.382827665984));
#230748=CARTESIAN_POINT('Ctrl Pts',(5.26772999789093,-5.90211462154354,
123.382499184284));
#230749=CARTESIAN_POINT('Ctrl Pts',(5.26480763057314,-5.90472158102898,
123.38234039803));
#230750=CARTESIAN_POINT('Ctrl Pts',(5.2581390967781,-5.91066150116706,123.381977919533));
#230751=CARTESIAN_POINT('Ctrl Pts',(5.25439169807175,-5.91399306944942,
123.381774119674));
#230752=CARTESIAN_POINT('Ctrl Pts',(5.24466723866885,-5.92262191450342,
123.381244997225));
#230753=CARTESIAN_POINT('Ctrl Pts',(5.23868533309739,-5.92791369424147,
123.380919254649));
#230754=CARTESIAN_POINT('Ctrl Pts',(5.20241893046063,-5.95989831560864,
123.378942875465));
#230755=CARTESIAN_POINT('Ctrl Pts',(5.17193898792222,-5.98636765107903,
123.377275494925));
#230756=CARTESIAN_POINT('Ctrl Pts',(4.62835579432831,-6.45117499725341,
123.347448589511));
#230757=CARTESIAN_POINT('Ctrl Pts',(4.06147261782022,-6.82229419530351,
123.315129351093));
#230758=CARTESIAN_POINT('Ctrl Pts',(3.13391786840199,-7.27250982956716,
123.267321414984));
#230759=CARTESIAN_POINT('Ctrl Pts',(2.80325758701635,-7.40625558932694,
123.251100110583));
#230760=CARTESIAN_POINT('Ctrl Pts',(2.28864457235289,-7.57498176602784,
123.227465605274));
#230761=CARTESIAN_POINT('Ctrl Pts',(2.11062401390143,-7.62650084401321,
123.219564390662));
#230762=CARTESIAN_POINT('Ctrl Pts',(1.83675877070318,-7.69543191045217,
123.207827347008));
#230763=CARTESIAN_POINT('Ctrl Pts',(1.74213673484754,-7.71740342048326,
123.203846425385));
#230764=CARTESIAN_POINT('Ctrl Pts',(1.63088699677973,-7.74108548292331,
123.199249923026));
#230765=CARTESIAN_POINT('Ctrl Pts',(1.61463133211905,-7.74449239885322,
123.198580372193));
#230766=CARTESIAN_POINT('Ctrl Pts',(1.58977803918717,-7.74961958163247,
123.197559852473));
#230767=CARTESIAN_POINT('Ctrl Pts',(1.5811881275716,-7.7513767796288,123.197207711041));
#230768=CARTESIAN_POINT('Ctrl Pts',(1.5655553574462,-7.75454763493599,123.196567890951));
#230769=CARTESIAN_POINT('Ctrl Pts',(1.5585134669104,-7.7559659858414,123.196280063718));
#230770=CARTESIAN_POINT('Ctrl Pts',(1.54332698516611,-7.7590032718011,123.195660162825));
#230771=CARTESIAN_POINT('Ctrl Pts',(1.53518175316004,-7.7606189791965,123.195328191658));
#230772=CARTESIAN_POINT('Ctrl Pts',(1.51319640903882,-7.76494407683624,
123.194433518295));
#230773=CARTESIAN_POINT('Ctrl Pts',(1.4993515421814,-7.76762929369715,123.193871580708));
#230774=CARTESIAN_POINT('Ctrl Pts',(1.43523658337371,-7.77988660895136,
123.191276000259));
#230775=CARTESIAN_POINT('Ctrl Pts',(1.38488102837438,-7.78900791874657,
123.189256582271));
#230776=CARTESIAN_POINT('Ctrl Pts',(0.47310283919901,-7.94504399997736,
123.153024448447));
#230777=CARTESIAN_POINT('Ctrl Pts',(-0.406594615782335,-7.94871893386163,
123.12424842017));
#230778=CARTESIAN_POINT('Ctrl Pts',(-1.60915479404307,-7.75327332410205,
123.081082630441));
#230779=CARTESIAN_POINT('Ctrl Pts',(-1.94525298587466,-7.67584699683704,
123.06842094574));
#230780=CARTESIAN_POINT('Ctrl Pts',(-2.30099187303705,-7.56902107345386,
123.053652347881));
#230781=CARTESIAN_POINT('Ctrl Pts',(-2.32669775838299,-7.5611587161149,
123.052578450725));
#230782=CARTESIAN_POINT('Ctrl Pts',(-2.36213750553983,-7.55012133779748,
123.051089016778));
#230783=CARTESIAN_POINT('Ctrl Pts',(-2.37190618617987,-7.5470581588716,
123.050677530728));
#230784=CARTESIAN_POINT('Ctrl Pts',(-2.38837376874113,-7.54185926527456,
123.049982313534));
#230785=CARTESIAN_POINT('Ctrl Pts',(-2.39507583352584,-7.53973356211778,
123.049698935686));
#230786=CARTESIAN_POINT('Ctrl Pts',(-2.40832298395694,-7.5355124997351,
123.049137967277));
#230787=CARTESIAN_POINT('Ctrl Pts',(-2.4148681917356,-7.53341754086006,
123.048860390748));
#230788=CARTESIAN_POINT('Ctrl Pts',(-2.42928176201579,-7.52878339968553,
123.048248228249));
#230789=CARTESIAN_POINT('Ctrl Pts',(-2.43714888598366,-7.52624040711141,
123.047913512924));
#230790=CARTESIAN_POINT('Ctrl Pts',(-2.463816484596,-7.51757409563833,123.046776940226));
#230791=CARTESIAN_POINT('Ctrl Pts',(-2.48259791271204,-7.51139265048349,
123.045973151054));
#230792=CARTESIAN_POINT('Ctrl Pts',(-2.67867321445553,-7.4460435629207,
123.037548020464));
#230793=CARTESIAN_POINT('Ctrl Pts',(-2.85383543268809,-7.3806824797968,
123.029734754841));
#230794=CARTESIAN_POINT('Ctrl Pts',(-3.47074672944409,-7.12523809573485,
123.001461008212));
#230795=CARTESIAN_POINT('Ctrl Pts',(-3.89728795680806,-6.90117791265394,
122.980568108106));
#230796=CARTESIAN_POINT('Ctrl Pts',(-4.59883555721635,-6.44675787271908,
122.944895026799));
#230797=CARTESIAN_POINT('Ctrl Pts',(-4.88349938083753,-6.2338930023871,
122.929964564455));
#230798=CARTESIAN_POINT('Ctrl Pts',(-5.43705503987908,-5.75869711831123,
122.899695845164));
#230799=CARTESIAN_POINT('Ctrl Pts',(-5.7035349141928,-5.49489421934162,
122.88431788687));
#230800=CARTESIAN_POINT('Ctrl Pts',(-5.98158904736257,-5.17752491559607,
122.867229592199));
#230801=CARTESIAN_POINT('Ctrl Pts',(-6.01253124463689,-5.1415600598388,
122.865312504795));
#230802=CARTESIAN_POINT('Ctrl Pts',(-6.05896052812327,-5.0866018791294,
122.862412079936));
#230803=CARTESIAN_POINT('Ctrl Pts',(-6.07468587693151,-5.06781144672001,
122.861425489038));
#230804=CARTESIAN_POINT('Ctrl Pts',(-6.10304025392766,-5.03360881148736,
122.859638820471));
#230805=CARTESIAN_POINT('Ctrl Pts',(-6.11569882533755,-5.01822138695761,
122.858838336318));
#230806=CARTESIAN_POINT('Ctrl Pts',(-6.14281807100243,-4.98500092921588,
122.857117241277));
#230807=CARTESIAN_POINT('Ctrl Pts',(-6.15725952746218,-4.96715242701767,
122.856196906606));
#230808=CARTESIAN_POINT('Ctrl Pts',(-6.19605855126245,-4.91877067747951,
122.853713855975));
#230809=CARTESIAN_POINT('Ctrl Pts',(-6.22026807789476,-4.8881194346548,
122.852153255539));
#230810=CARTESIAN_POINT('Ctrl Pts',(-6.33669188766635,-4.73845175375869,
122.844592532332));
#230811=CARTESIAN_POINT('Ctrl Pts',(-6.42572371753769,-4.61699739160262,
122.838638996535));
#230812=CARTESIAN_POINT('Ctrl Pts',(-6.5157098365615,-4.48659206573222,
122.832419858857));
#230813=CARTESIAN_POINT('Ctrl Pts',(-6.52017360701209,-4.48010258510469,
122.832110809568));
#230814=CARTESIAN_POINT('Ctrl Pts',(-6.91668414056494,-3.90180325662953,
122.804609239786));
#230815=CARTESIAN_POINT('Ctrl Pts',(-7.23185592982941,-3.28097163589568,
122.778748434194));
#230816=CARTESIAN_POINT('Ctrl Pts',(-7.48606138635359,-2.55891115136077,
122.74848965973));
#230817=CARTESIAN_POINT('Ctrl Pts',(-7.50911960040304,-2.49043448998333,
122.745615501153));
#230818=CARTESIAN_POINT('Ctrl Pts',(-7.53666802528933,-2.4047600570583,
122.742006557392));
#230819=CARTESIAN_POINT('Ctrl Pts',(-7.54204283422624,-2.38784960533014,
122.741293578467));
#230820=CARTESIAN_POINT('Ctrl Pts',(-7.55066845398457,-2.36039164347064,
122.740134834693));
#230821=CARTESIAN_POINT('Ctrl Pts',(-7.55395415199241,-2.34985520430915,
122.739689943871));
#230822=CARTESIAN_POINT('Ctrl Pts',(-7.56023399076726,-2.32956799576375,
122.73883288756));
#230823=CARTESIAN_POINT('Ctrl Pts',(-7.56323134486293,-2.31981823973345,
122.738420798884));
#230824=CARTESIAN_POINT('Ctrl Pts',(-7.57005098372382,-2.29748169541128,
122.737476277375));
#230825=CARTESIAN_POINT('Ctrl Pts',(-7.5738607445911,-2.28489112584598,
122.736943559449));
#230826=CARTESIAN_POINT('Ctrl Pts',(-7.58389567627036,-2.25142662428004,
122.73552687063));
#230827=CARTESIAN_POINT('Ctrl Pts',(-7.59006605464234,-2.23053642713359,
122.734641702204));
#230828=CARTESIAN_POINT('Ctrl Pts',(-7.63305346135819,-2.08275598001856,
122.728374903688));
#230829=CARTESIAN_POINT('Ctrl Pts',(-7.66677230964546,-1.95498820016653,
122.72293111468));
#230830=CARTESIAN_POINT('Ctrl Pts',(-7.75481273958398,-1.58395380557029,
122.707105036482));
#230831=CARTESIAN_POINT('Ctrl Pts',(-7.80085936015728,-1.3388880784233,
122.696633733668));
#230832=CARTESIAN_POINT('Ctrl Pts',(-7.88568895207708,-0.730257288688616,
122.670817739835));
#230833=CARTESIAN_POINT('Ctrl Pts',(-7.91099667283217,-0.365387611985288,
122.655518059375));
#230834=CARTESIAN_POINT('Ctrl Pts',(-7.91100007201382,0.00786949525208386,
122.640138565923));
#230835=CARTESIAN_POINT('Ctrl Pts',(-7.91098818603604,0.0158110199212082,
122.639811462769));
#230836=CARTESIAN_POINT('Ctrl Pts',(-7.91044581199246,0.196452996655032,
122.632373620344));
#230837=CARTESIAN_POINT('Ctrl Pts',(-7.90427221289167,0.369092327641354,
122.625320690788));
#230838=CARTESIAN_POINT('Ctrl Pts',(-7.88927449177412,0.587729650601402,
122.616444553963));
#230839=CARTESIAN_POINT('Ctrl Pts',(-7.8856879896008,0.634037152709973,
122.614567707779));
#230840=CARTESIAN_POINT('Ctrl Pts',(-7.8793478000732,0.707491008283121,
122.611594981302));
#230841=CARTESIAN_POINT('Ctrl Pts',(-7.87686112252303,0.734659202661326,
122.610496414201));
#230842=CARTESIAN_POINT('Ctrl Pts',(-7.87193000201876,0.78562806661664,
122.608437065062));
#230843=CARTESIAN_POINT('Ctrl Pts',(-7.86951802707497,0.809431554486408,
122.607475970054));
#230844=CARTESIAN_POINT('Ctrl Pts',(-7.86380648047646,0.863357915580631,
122.605299985629));
#230845=CARTESIAN_POINT('Ctrl Pts',(-7.86044173736246,0.893473533137972,
122.604085751629));
#230846=CARTESIAN_POINT('Ctrl Pts',(-7.84975865666005,0.984355673137799,
122.600423954416));
#230847=CARTESIAN_POINT('Ctrl Pts',(-7.84190805761375,1.0450574803776,122.597981548252));
#230848=CARTESIAN_POINT('Ctrl Pts',(-7.78152407357358,1.47286360546611,
122.580783040251));
#230849=CARTESIAN_POINT('Ctrl Pts',(-7.7039359498709,1.83598210164303,122.566200270977));
#230850=CARTESIAN_POINT('Ctrl Pts',(-7.51235336307921,2.50023321942439,
122.539493705509));
#230851=CARTESIAN_POINT('Ctrl Pts',(-7.40491614676532,2.80247125685759,
122.527362143228));
#230852=CARTESIAN_POINT('Ctrl Pts',(-7.11527040245073,3.48319761801135,
122.499707862931));
#230853=CARTESIAN_POINT('Ctrl Pts',(-6.92069050588661,3.8553555720628,122.484356951973));
#230854=CARTESIAN_POINT('Ctrl Pts',(-6.68252037080982,4.23422235476954,
122.467445318905));
#230855=CARTESIAN_POINT('Ctrl Pts',(-6.66737282621719,4.2580344105564,122.466376461572));
#230856=CARTESIAN_POINT('Ctrl Pts',(-6.64245729175586,4.29674288475144,
122.464628568916));
#230857=CARTESIAN_POINT('Ctrl Pts',(-6.63276580421925,4.31168830896625,
122.463951160691));
#230858=CARTESIAN_POINT('Ctrl Pts',(-6.61914728454546,4.33253510886889,
122.463002565876));
#230859=CARTESIAN_POINT('Ctrl Pts',(-6.61526265261768,4.33846416151682,
122.462732354847));
#230860=CARTESIAN_POINT('Ctrl Pts',(-6.60473339329572,4.35448778329756,
122.462000937356));
#230861=CARTESIAN_POINT('Ctrl Pts',(-6.59807360247052,4.36457234866685,
122.461539371968));
#230862=CARTESIAN_POINT('Ctrl Pts',(-6.58548624673853,4.38353805779245,
122.460668915294));
#230863=CARTESIAN_POINT('Ctrl Pts',(-6.57956375607474,4.39242254218495,
122.460260151324));
#230864=CARTESIAN_POINT('Ctrl Pts',(-6.51961042651408,4.48196677973715,
122.456130014865));
#230865=CARTESIAN_POINT('Ctrl Pts',(-6.46411805795101,4.56163603970415,
122.452370827905));
#230866=CARTESIAN_POINT('Ctrl Pts',(-6.39996873261838,4.65021205389714,
122.448075082794));
#230867=CARTESIAN_POINT('Ctrl Pts',(-6.39273963457286,4.66014505005677,
122.447591677118));
#230868=CARTESIAN_POINT('Ctrl Pts',(-6.36899470625122,4.69261206435841,
122.446005994529));
#230869=CARTESIAN_POINT('Ctrl Pts',(-6.35238272888113,4.7150753121587,122.444899999383));
#230870=CARTESIAN_POINT('Ctrl Pts',(-6.3201710065246,4.75815381920606,122.442760948201));
#230871=CARTESIAN_POINT('Ctrl Pts',(-6.30458850050066,4.77878155390664,
122.441728625597));
#230872=CARTESIAN_POINT('Ctrl Pts',(-6.28296776955826,4.80711272951643,
122.440299137008));
#230873=CARTESIAN_POINT('Ctrl Pts',(-6.27701584665144,4.81488201801712,
122.439905911582));
#230874=CARTESIAN_POINT('Ctrl Pts',(-6.2675037806945,4.82725089359206,122.439277916591));
#230875=CARTESIAN_POINT('Ctrl Pts',(-6.2639529451683,4.83185764806973,122.439043584145));
#230876=CARTESIAN_POINT('Ctrl Pts',(-6.25665572952526,4.84130328862421,
122.438562204498));
#230877=CARTESIAN_POINT('Ctrl Pts',(-6.25290880962877,4.84614175075723,
122.438315131578));
#230878=CARTESIAN_POINT('Ctrl Pts',(-6.24424224347191,4.85730625209324,
122.437743880566));
#230879=CARTESIAN_POINT('Ctrl Pts',(-6.23931859640703,4.86362916695968,
122.43741950822));
#230880=CARTESIAN_POINT('Ctrl Pts',(-6.22386241231381,4.88341580033775,
122.436401733714));
#230881=CARTESIAN_POINT('Ctrl Pts',(-6.21329588228058,4.89685281374519,
122.435706643586));
#230882=CARTESIAN_POINT('Ctrl Pts',(-6.00455084528704,5.16054172602848,
122.421986641349));
#230883=CARTESIAN_POINT('Ctrl Pts',(-5.79149153027634,5.39855247604332,
122.408047337165));
#230884=CARTESIAN_POINT('Ctrl Pts',(-5.45536921920309,5.73118839155223,
122.386726740543));
#230885=CARTESIAN_POINT('Ctrl Pts',(-5.34292530557486,5.83615636523896,
122.379699543903));
#230886=CARTESIAN_POINT('Ctrl Pts',(-5.11254968953585,6.03897424631014,
122.365602196726));
#230887=CARTESIAN_POINT('Ctrl Pts',(-4.99468956531507,6.13681108108331,
122.358535302134));
#230888=CARTESIAN_POINT('Ctrl Pts',(-4.52643316128406,6.50308478059612,
122.331164786358));
#230889=CARTESIAN_POINT('Ctrl Pts',(-4.15663155711402,6.7454562686423,122.311074659838));
#230890=CARTESIAN_POINT('Ctrl Pts',(-3.54761463452131,7.07541341267905,
122.281089942063));
#230891=CARTESIAN_POINT('Ctrl Pts',(-3.32112236743532,7.18451148461951,
122.270536729567));
#230892=CARTESIAN_POINT('Ctrl Pts',(-3.06806777786713,7.29187484766734,
122.259382560491));
#230893=CARTESIAN_POINT('Ctrl Pts',(-3.04628684506019,7.30100096927076,
122.258427475878));
#230894=CARTESIAN_POINT('Ctrl Pts',(-3.01562164643922,7.31368844585405,
122.25708975166));
#230895=CARTESIAN_POINT('Ctrl Pts',(-3.00677138638473,7.31733137340926,
122.256704480644));
#230896=CARTESIAN_POINT('Ctrl Pts',(-2.99139556123321,7.32362773625407,
122.256036535657));
#230897=CARTESIAN_POINT('Ctrl Pts',(-2.98487303083925,7.32628852920094,
122.255753624758));
#230898=CARTESIAN_POINT('Ctrl Pts',(-2.9712886529523,7.3318089710388,122.255165315012));
#230899=CARTESIAN_POINT('Ctrl Pts',(-2.96422620885145,7.3346671383326,122.254859964059));
#230900=CARTESIAN_POINT('Ctrl Pts',(-2.94757725135526,7.34137698824372,
122.254141324682));
#230901=CARTESIAN_POINT('Ctrl Pts',(-2.93798729005412,7.34522010702862,
122.253728311872));
#230902=CARTESIAN_POINT('Ctrl Pts',(-2.90657488088151,7.3577370783932,122.252378497575));
#230903=CARTESIAN_POINT('Ctrl Pts',(-2.88472124707806,7.36633258760392,
122.251444210902));
#230904=CARTESIAN_POINT('Ctrl Pts',(-2.48294963364251,7.5222959841929,122.234354330079));
#230905=CARTESIAN_POINT('Ctrl Pts',(-2.0922287848583,7.64019631154346,122.219195962468));
#230906=CARTESIAN_POINT('Ctrl Pts',(-1.1405021448231,7.84884777212554,122.184404599306));
#230907=CARTESIAN_POINT('Ctrl Pts',(-0.575458860413354,7.91037125879405,
122.165480450824));
#230908=CARTESIAN_POINT('Ctrl Pts',(0.120836509500774,7.9111378257672,122.140761480949));
#230909=CARTESIAN_POINT('Ctrl Pts',(0.250363447632309,7.90809836448072,
122.136098413506));
#230910=CARTESIAN_POINT('Ctrl Pts',(0.583797563593487,7.89207395525814,
122.123819557991));
#230911=CARTESIAN_POINT('Ctrl Pts',(0.787381334560894,7.8743685428624,122.116054207754));
#230912=CARTESIAN_POINT('Ctrl Pts',(1.005581907044,7.8468446584285,122.107268112165));
#230913=CARTESIAN_POINT('Ctrl Pts',(1.02110745928984,7.84483942579828,122.106640565912));
#230914=CARTESIAN_POINT('Ctrl Pts',(1.04302689041769,7.84194220723988,122.105751296554));
#230915=CARTESIAN_POINT('Ctrl Pts',(1.04942585670393,7.84108844783441,122.105491295826));
#230916=CARTESIAN_POINT('Ctrl Pts',(1.06057388418235,7.83958717083396,122.105037652468));
#230917=CARTESIAN_POINT('Ctrl Pts',(1.06532342094417,7.83894316738814,122.104844165728));
#230918=CARTESIAN_POINT('Ctrl Pts',(1.07524832612742,7.83758823408588,122.104439398932));
#230919=CARTESIAN_POINT('Ctrl Pts',(1.08042358097314,7.83687649356574,122.104228083419));
#230920=CARTESIAN_POINT('Ctrl Pts',(1.09268381698111,7.8351779971384,122.103726880192));
#230921=CARTESIAN_POINT('Ctrl Pts',(1.09976816505213,7.83418675762804,122.103436798779));
#230922=CARTESIAN_POINT('Ctrl Pts',(1.12325330600757,7.83086824133311,122.102473618676));
#230923=CARTESIAN_POINT('Ctrl Pts',(1.13964806417693,7.82849906984852,122.101798742745));
#230924=CARTESIAN_POINT('Ctrl Pts',(1.6030606347084,7.7600457269014,122.082654632283));
#230925=CARTESIAN_POINT('Ctrl Pts',(2.04358792758315,7.65583608302759,122.062722469412));
#230926=CARTESIAN_POINT('Ctrl Pts',(2.82399970385248,7.39903071538375,122.026536444565));
#230927=CARTESIAN_POINT('Ctrl Pts',(3.16669395516515,7.25897376123151,122.010306476261));
#230928=CARTESIAN_POINT('Ctrl Pts',(3.77536257405946,6.95887577122387,121.981352237365));
#230929=CARTESIAN_POINT('Ctrl Pts',(4.04415426640064,6.80618455789069,121.968508741788));
#230930=CARTESIAN_POINT('Ctrl Pts',(4.33058821635751,6.62049703507536,121.954689112334));
#230931=CARTESIAN_POINT('Ctrl Pts',(4.35772494816115,6.60266677837436,121.953378273905));
#230932=CARTESIAN_POINT('Ctrl Pts',(4.39839518690331,6.57558434539542,121.951411026019));
#230933=CARTESIAN_POINT('Ctrl Pts',(4.41201087066399,6.56645640989891,121.950751970742));
#230934=CARTESIAN_POINT('Ctrl Pts',(4.4355396067671,6.55057655854401,121.94961224369));
#230935=CARTESIAN_POINT('Ctrl Pts',(4.44546584197748,6.54384430600786,121.949131158936));
#230936=CARTESIAN_POINT('Ctrl Pts',(4.46605167600794,6.52981395713853,121.948132881055));
#230937=CARTESIAN_POINT('Ctrl Pts',(4.47670878808498,6.5225122702391,121.947615764887));
#230938=CARTESIAN_POINT('Ctrl Pts',(4.50171548402078,6.50528885214098,121.946401582238));
#230939=CARTESIAN_POINT('Ctrl Pts',(4.51605024174706,6.49534568484078,121.945704961867));
#230940=CARTESIAN_POINT('Ctrl Pts',(4.5461665180098,6.47430792672925,121.944240051328));
#230941=CARTESIAN_POINT('Ctrl Pts',(4.56194058858483,6.46320285998722,121.943471979079));
#230942=CARTESIAN_POINT('Ctrl Pts',(4.60451906794802,6.432993749524,121.941396442249));
#230943=CARTESIAN_POINT('Ctrl Pts',(4.63124523176377,6.41377985677793,121.940091143748));
#230944=CARTESIAN_POINT('Ctrl Pts',(5.10264219299502,6.07040177178243,121.917022707642));
#230945=CARTESIAN_POINT('Ctrl Pts',(5.51242335048445,5.70087479389796,121.896383173171));
#230946=CARTESIAN_POINT('Ctrl Pts',(6.13444507014976,5.00964810986327,121.862115279552));
#230947=CARTESIAN_POINT('Ctrl Pts',(6.36770087344635,4.70960326530832,121.848305379942));
#230948=CARTESIAN_POINT('Ctrl Pts',(6.65766201550409,4.27548413925649,121.828635140419));
#230949=CARTESIAN_POINT('Ctrl Pts',(6.73359393454971,4.15486929477825,121.823197269));
#230950=CARTESIAN_POINT('Ctrl Pts',(6.8520463974024,3.95492893328371,121.814144550234));
#230951=CARTESIAN_POINT('Ctrl Pts',(6.89654526902927,3.87681123296082,121.810598276778));
#230952=CARTESIAN_POINT('Ctrl Pts',(6.94684523472325,3.78490206751853,121.806399573757));
#230953=CARTESIAN_POINT('Ctrl Pts',(6.95395141588179,3.77183007010281,121.805801788944));
#230954=CARTESIAN_POINT('Ctrl Pts',(6.96459014680506,3.752127600154,121.804899775356));
#230955=CARTESIAN_POINT('Ctrl Pts',(6.96815021998524,3.74551197462206,121.804596728551));
#230956=CARTESIAN_POINT('Ctrl Pts',(6.97447576682979,3.73371708229041,121.804056111107));
#230957=CARTESIAN_POINT('Ctrl Pts',(6.97724491150819,3.72853978351801,121.803818700568));
#230958=CARTESIAN_POINT('Ctrl Pts',(6.98306334205063,3.71763224308012,121.803318284873));
#230959=CARTESIAN_POINT('Ctrl Pts',(6.98611134303106,3.71190132362431,121.803055223426));
#230960=CARTESIAN_POINT('Ctrl Pts',(6.99412617491511,3.69678681703955,121.802361056737));
#230961=CARTESIAN_POINT('Ctrl Pts',(6.9990811648969,3.68739699069471,121.801929424484));
#230962=CARTESIAN_POINT('Ctrl Pts',(7.02123286621443,3.64521346335347,121.799988505945));
#230963=CARTESIAN_POINT('Ctrl Pts',(7.03821791531186,3.61230960265677,121.798469621436));
#230964=CARTESIAN_POINT('Ctrl Pts',(7.15661591513859,3.37894071928148,121.787655443127));
#230965=CARTESIAN_POINT('Ctrl Pts',(7.24966354982402,3.17438824039553,121.777909970264));
#230966=CARTESIAN_POINT('Ctrl Pts',(7.52384049416456,2.49648673551076,121.745288336194));
#230967=CARTESIAN_POINT('Ctrl Pts',(7.66824717562286,2.00963183637676,121.721500248117));
#230968=CARTESIAN_POINT('Ctrl Pts',(7.85627549181512,1.0441796902873,121.67688117192));
#230969=CARTESIAN_POINT('Ctrl Pts',(7.90493716167581,0.568724338412397,
121.656054115293));
#230970=CARTESIAN_POINT('Ctrl Pts',(7.91082541849235,0.0609205216541271,
121.635412214022));
#230971=CARTESIAN_POINT('Ctrl Pts',(7.91100267697548,0.0301128819094594,
121.634165787443));
#230972=CARTESIAN_POINT('Ctrl Pts',(7.9109989717153,-0.0120481679108156,
121.632467999411));
#230973=CARTESIAN_POINT('Ctrl Pts',(7.91097353544595,-0.0234011056981993,
121.632011618229));
#230974=CARTESIAN_POINT('Ctrl Pts',(7.91089443484175,-0.0414064914464311,
121.631289062771));
#230975=CARTESIAN_POINT('Ctrl Pts',(7.91085681782842,-0.0480589725781283,
121.631022369591));
#230976=CARTESIAN_POINT('Ctrl Pts',(7.91076765403138,-0.0609513096375462,
121.630506048172));
#230977=CARTESIAN_POINT('Ctrl Pts',(7.91071711576061,-0.0671911666543467,
121.630256387449));
#230978=CARTESIAN_POINT('Ctrl Pts',(7.91057931389433,-0.0820364512229167,
121.629662981486));
#230979=CARTESIAN_POINT('Ctrl Pts',(7.91048539106875,-0.090641817347533,
121.629319452342));
#230980=CARTESIAN_POINT('Ctrl Pts',(7.91016526583808,-0.116157053060414,
121.628302206005));
#230981=CARTESIAN_POINT('Ctrl Pts',(7.90989888219174,-0.133066419785025,
121.627629793095));
#230982=CARTESIAN_POINT('Ctrl Pts',(7.90733248462793,-0.268416575690285,
121.62226125425));
#230983=CARTESIAN_POINT('Ctrl Pts',(7.90242652814297,-0.386795831909862,
121.617650510753));
#230984=CARTESIAN_POINT('Ctrl Pts',(7.87550275685157,-0.807685907948852,
121.601532546116));
#230985=CARTESIAN_POINT('Ctrl Pts',(7.838752817635,-1.10899703523779,121.590513181226));
#230986=CARTESIAN_POINT('Ctrl Pts',(7.72652858173331,-1.72971435303638,
121.568389622819));
#230987=CARTESIAN_POINT('Ctrl Pts',(7.64831463857171,-2.04803485573906,
121.557371101431));
#230988=CARTESIAN_POINT('Ctrl Pts',(7.37710215899867,-2.91553484378619,
121.526828009285));
#230989=CARTESIAN_POINT('Ctrl Pts',(7.14297834487907,-3.44958953269405,
121.507473592931));
#230990=CARTESIAN_POINT('Ctrl Pts',(6.83406459812971,-3.9850778406863,121.483125923467));
#230991=CARTESIAN_POINT('Ctrl Pts',(6.81539079688638,-4.01693073461318,
121.481657456047));
#230992=CARTESIAN_POINT('Ctrl Pts',(6.79266004772222,-4.05508897899298,
121.479872573196));
#230993=CARTESIAN_POINT('Ctrl Pts',(6.78881596659692,-4.06152125716694,
121.479570813516));
#230994=CARTESIAN_POINT('Ctrl Pts',(6.78252669647948,-4.07201118061901,
121.479077235551));
#230995=CARTESIAN_POINT('Ctrl Pts',(6.78008698448998,-4.07607211983111,
121.478885799908));
#230996=CARTESIAN_POINT('Ctrl Pts',(6.7757246782787,-4.08331849450716,121.478543556785));
#230997=CARTESIAN_POINT('Ctrl Pts',(6.77380347979196,-4.08650477308932,
121.478392847718));
#230998=CARTESIAN_POINT('Ctrl Pts',(6.76974430110557,-4.09322613172561,
121.478074459256));
#230999=CARTESIAN_POINT('Ctrl Pts',(6.76760579893498,-4.09676089342325,
121.477906742798));
#231000=CARTESIAN_POINT('Ctrl Pts',(6.76190013653118,-4.10617520783546,
121.477459314837));
#231001=CARTESIAN_POINT('Ctrl Pts',(6.7583280884598,-4.11205176788634,121.477179253055));
#231002=CARTESIAN_POINT('Ctrl Pts',(6.74131377542368,-4.13996083416053,
121.475845546104));
#231003=CARTESIAN_POINT('Ctrl Pts',(6.72777154754702,-4.16193189512592,
121.474784829611));
#231004=CARTESIAN_POINT('Ctrl Pts',(6.61968634619532,-4.33538449827017,
121.4663281675));
#231005=CARTESIAN_POINT('Ctrl Pts',(6.52015239408849,-4.48368268114007,
121.458597008266));
#231006=CARTESIAN_POINT('Ctrl Pts',(6.2030659638144,-4.92320738865209,121.434473295189));
#231007=CARTESIAN_POINT('Ctrl Pts',(5.97038900287542,-5.20292551545113,
121.417448469429));
#231008=CARTESIAN_POINT('Ctrl Pts',(5.51399504814044,-5.68050181870736,
121.386586269516));
#231009=CARTESIAN_POINT('Ctrl Pts',(5.29671763167392,-5.88362461205754,
121.372753714829));
#231010=CARTESIAN_POINT('Ctrl Pts',(4.74755264420394,-6.34187810277763,
121.340373559345));
#231011=CARTESIAN_POINT('Ctrl Pts',(4.40583709701723,-6.58387036294046,
121.322275461513));
#231012=CARTESIAN_POINT('Ctrl Pts',(4.02229809609323,-6.81218288859636,
121.304180485345));
#231013=CARTESIAN_POINT('Ctrl Pts',(3.99796724913797,-6.82649072214591,
121.303041327586));
#231014=CARTESIAN_POINT('Ctrl Pts',(3.96432550431203,-6.84603230705104,
121.30147816504));
#231015=CARTESIAN_POINT('Ctrl Pts',(3.95507996229367,-6.85137778453623,
121.301049805927));
#231016=CARTESIAN_POINT('Ctrl Pts',(3.94033139021809,-6.85986513635622,
121.300368442024));
#231017=CARTESIAN_POINT('Ctrl Pts',(3.93483537760024,-6.86301913921076,
121.300114965952));
#231018=CARTESIAN_POINT('Ctrl Pts',(3.92413198207343,-6.86914442506605,
121.299622164204));
#231019=CARTESIAN_POINT('Ctrl Pts',(3.9189249996244,-6.87211639836691,121.29938281182));
#231020=CARTESIAN_POINT('Ctrl Pts',(3.90645763308859,-6.87921358086701,
121.298810637208));
#231021=CARTESIAN_POINT('Ctrl Pts',(3.89919407915302,-6.88333322337214,
121.298478030675));
#231022=CARTESIAN_POINT('Ctrl Pts',(3.87819984434484,-6.89519654996592,
121.297518824582));
#231023=CARTESIAN_POINT('Ctrl Pts',(3.86445248517939,-6.90291072585189,
121.296893364907));
#231024=CARTESIAN_POINT('Ctrl Pts',(3.75553865260428,-6.96359916532429,
121.291958890076));
#231025=CARTESIAN_POINT('Ctrl Pts',(3.65930826977888,-7.01464526115448,
121.287724321613));
#231026=CARTESIAN_POINT('Ctrl Pts',(3.2855917547353,-7.20310167547326,121.27172759516));
#231027=CARTESIAN_POINT('Ctrl Pts',(3.00117445277655,-7.32616947697695,
121.260500695372));
#231028=CARTESIAN_POINT('Ctrl Pts',(2.50274438743094,-7.5079278073775,121.241891596508));
#231029=CARTESIAN_POINT('Ctrl Pts',(2.29214902980414,-7.57487724898308,
121.234333891815));
#231030=CARTESIAN_POINT('Ctrl Pts',(1.5032710671529,-7.7897485842773,121.20651751995));
#231031=CARTESIAN_POINT('Ctrl Pts',(0.911699572768521,-7.88090210862725,
121.186730995063));
#231032=CARTESIAN_POINT('Ctrl Pts',(0.279910596700759,-7.90612719985605,
121.161811108329));
#231033=CARTESIAN_POINT('Ctrl Pts',(0.244205810922867,-7.90731058482555,
121.160389670526));
#231034=CARTESIAN_POINT('Ctrl Pts',(0.201021844090053,-7.90844909587385,
121.158653266416));
#231035=CARTESIAN_POINT('Ctrl Pts',(0.19354865470272,-7.90863552080794,
121.15835214945));
#231036=CARTESIAN_POINT('Ctrl Pts',(0.181217921522819,-7.90892563320714,
121.157854290361));
#231037=CARTESIAN_POINT('Ctrl Pts',(0.176360501279567,-7.9090354392975,
121.157657909331));
#231038=CARTESIAN_POINT('Ctrl Pts',(0.167604170880889,-7.90922531287796,
121.157303433255));
#231039=CARTESIAN_POINT('Ctrl Pts',(0.1637052929805,-7.90930697247932,121.157145431423));
#231040=CARTESIAN_POINT('Ctrl Pts',(0.155387770111011,-7.90947502510971,
121.156808011483));
#231041=CARTESIAN_POINT('Ctrl Pts',(0.150969111767284,-7.90956059835645,
121.156628545817));
#231042=CARTESIAN_POINT('Ctrl Pts',(0.139068748611965,-7.90978108909305,
121.156144639855));
#231043=CARTESIAN_POINT('Ctrl Pts',(0.131586936268826,-7.90990909376826,
121.155839801669));
#231044=CARTESIAN_POINT('Ctrl Pts',(0.0952926185785408,-7.91047853630061,
121.154358135146));
#231045=CARTESIAN_POINT('Ctrl Pts',(0.0664783595287169,-7.91077315709305,
121.153172983271));
#231046=CARTESIAN_POINT('Ctrl Pts',(-0.168834078612055,-7.91189346920868,
121.143425676321));
#231047=CARTESIAN_POINT('Ctrl Pts',(-0.375277098152051,-7.90479084434174,
121.134442993002));
#231048=CARTESIAN_POINT('Ctrl Pts',(-0.968561250397912,-7.86108649676241,
121.107825735296));
#231049=CARTESIAN_POINT('Ctrl Pts',(-1.35329239147617,-7.80406132204472,
121.08959886076));
#231050=CARTESIAN_POINT('Ctrl Pts',(-1.89414786949916,-7.6826851470739,
121.063753164238));
#231051=CARTESIAN_POINT('Ctrl Pts',(-2.05485124326905,-7.64127183462109,
121.056040772332));
#231052=CARTESIAN_POINT('Ctrl Pts',(-2.7316186001039,-7.44397265820379,
121.023603861077));
#231053=CARTESIAN_POINT('Ctrl Pts',(-3.23238283406999,-7.24060217193323,
120.999836659265));
#231054=CARTESIAN_POINT('Ctrl Pts',(-3.73967447955794,-6.9713693769398,
120.976442565805));
#231055=CARTESIAN_POINT('Ctrl Pts',(-3.77060883421412,-6.95468656833446,
120.975018271509));
#231056=CARTESIAN_POINT('Ctrl Pts',(-3.81221651153987,-6.93188845221738,
120.973105428234));
#231057=CARTESIAN_POINT('Ctrl Pts',(-3.82298800621975,-6.92595372139532,
120.972610488452));
#231058=CARTESIAN_POINT('Ctrl Pts',(-3.83990025473975,-6.9165841669824,
120.97183378794));
#231059=CARTESIAN_POINT('Ctrl Pts',(-3.84605031808688,-6.91316623960174,
120.971551427864));
#231060=CARTESIAN_POINT('Ctrl Pts',(-3.85786739276228,-6.9065781935953,
120.971009043686));
#231061=CARTESIAN_POINT('Ctrl Pts',(-3.86353507539164,-6.90340929438943,
120.97074897656));
#231062=CARTESIAN_POINT('Ctrl Pts',(-3.8768687802879,-6.8959326261873,120.970137309157));
#231063=CARTESIAN_POINT('Ctrl Pts',(-3.88453154161697,-6.8916190425264,
120.969785916111));
#231064=CARTESIAN_POINT('Ctrl Pts',(-3.90675208817579,-6.87906163733155,
120.968767303249));
#231065=CARTESIAN_POINT('Ctrl Pts',(-3.92129097492854,-6.87078437902002,
120.968101275036));
#231066=CARTESIAN_POINT('Ctrl Pts',(-4.02074624998288,-6.81374413891597,
120.963548158711));
#231067=CARTESIAN_POINT('Ctrl Pts',(-4.10477880738604,-6.76345336197736,
120.959715985035));
#231068=CARTESIAN_POINT('Ctrl Pts',(-4.36497496643559,-6.60109829921007,
120.94788078816));
#231069=CARTESIAN_POINT('Ctrl Pts',(-4.53765361511666,-6.48361099897565,
120.940073704662));
#231070=CARTESIAN_POINT('Ctrl Pts',(-4.7862127345976,-6.29969622197205,
120.928792257694));
#231071=CARTESIAN_POINT('Ctrl Pts',(-4.86579257352607,-6.23843474185694,
120.925172774717));
#231072=CARTESIAN_POINT('Ctrl Pts',(-4.99528101553143,-6.13476752973713,
120.919251507299));
#231073=CARTESIAN_POINT('Ctrl Pts',(-5.04586705509031,-6.09322827852271,
120.916929955196));
#231074=CARTESIAN_POINT('Ctrl Pts',(-5.24247012639813,-5.92765812084226,
120.907859911089));
#231075=CARTESIAN_POINT('Ctrl Pts',(-5.38447832765632,-5.79896701108558,
120.901205784861));
#231076=CARTESIAN_POINT('Ctrl Pts',(-5.66188234169319,-5.52859308021142,
120.887780004742));
#231077=CARTESIAN_POINT('Ctrl Pts',(-5.79696653936588,-5.38678296949157,
120.881013477701));
#231078=CARTESIAN_POINT('Ctrl Pts',(-6.19111456957088,-4.94099509235523,
120.860145242084));
#231079=CARTESIAN_POINT('Ctrl Pts',(-6.43256020973177,-4.62228501768219,
120.845708533327));
#231080=CARTESIAN_POINT('Ctrl Pts',(-6.6648584408398,-4.26197703409882,
120.828688052114));
#231081=CARTESIAN_POINT('Ctrl Pts',(-6.68065958892634,-4.23716576319373,
120.827514060391));
#231082=CARTESIAN_POINT('Ctrl Pts',(-6.70216550551455,-4.20297739517431,
120.825894226977));
#231083=CARTESIAN_POINT('Ctrl Pts',(-6.70798979449527,-4.19367551954443,
120.825453290249));
#231084=CARTESIAN_POINT('Ctrl Pts',(-6.71721563633876,-4.17887268599546,
120.824751277155));
#231085=CARTESIAN_POINT('Ctrl Pts',(-6.72062984310777,-4.17337960680574,
120.824490703421));
#231086=CARTESIAN_POINT('Ctrl Pts',(-6.72724740495691,-4.1627035058646,
120.823984138275));
#231087=CARTESIAN_POINT('Ctrl Pts',(-6.73045151642247,-4.15752095726362,
120.823738176592));
#231088=CARTESIAN_POINT('Ctrl Pts',(-6.73808350622551,-4.14514451153135,
120.823150666014));
#231089=CARTESIAN_POINT('Ctrl Pts',(-6.7425058516263,-4.13794722036546,
120.822808906037));
#231090=CARTESIAN_POINT('Ctrl Pts',(-6.75566779606539,-4.11644926109138,
120.821787800096));
#231091=CARTESIAN_POINT('Ctrl Pts',(-6.76437346158028,-4.10212793044029,
120.821107192135));
#231092=CARTESIAN_POINT('Ctrl Pts',(-6.83844620973009,-3.97939693315188,
120.815271857149));
#231093=CARTESIAN_POINT('Ctrl Pts',(-6.90124648880263,-3.8694627342908,
120.810027589514));
#231094=CARTESIAN_POINT('Ctrl Pts',(-7.1790169352521,-3.35492611327057,
120.785521548263));
#231095=CARTESIAN_POINT('Ctrl Pts',(-7.36122042076578,-2.9336400575739,
120.765632169292));
#231096=CARTESIAN_POINT('Ctrl Pts',(-7.72075526074726,-1.8537327561986,
120.716815077764));
#231097=CARTESIAN_POINT('Ctrl Pts',(-7.85148547063976,-1.1834784090553,
120.688520336153));
#231098=CARTESIAN_POINT('Ctrl Pts',(-7.90226451682542,-0.389270818588789,
120.655930261483));
#231099=CARTESIAN_POINT('Ctrl Pts',(-7.90711381548192,-0.273619773638637,
120.651209371742));
#231100=CARTESIAN_POINT('Ctrl Pts',(-7.91047403648233,-0.105305139888183,
120.644377508997));
#231101=CARTESIAN_POINT('Ctrl Pts',(-7.91099940645487,-0.0526978673707179,
120.642247651637));
#231102=CARTESIAN_POINT('Ctrl Pts',(-7.91099999949736,-8.91784084347633E-5,
120.64012317337));
#231103=CARTESIAN_POINT('',(-7.91099999889219,0.000132392670232489,118.642430830134));
#231104=CARTESIAN_POINT('Ctrl Pts',(-7.91099929352038,0.00334333966528006,
120.642331508237));
#231105=CARTESIAN_POINT('Ctrl Pts',(-7.91091098853137,0.212290313526421,
120.633939442701));
#231106=CARTESIAN_POINT('Ctrl Pts',(-7.90254028181684,0.421122619949147,
120.625547377165));
#231107=CARTESIAN_POINT('Ctrl Pts',(-7.88593972319406,0.62918652413254,
120.617155311629));
#231108=CARTESIAN_POINT('Ctrl Pts',(-7.86910331169471,0.840206501748585,
120.6086440156));
#231109=CARTESIAN_POINT('Ctrl Pts',(-7.84380147092849,1.05043578307963,
120.60013271957));
#231110=CARTESIAN_POINT('Ctrl Pts',(-7.81014299452937,1.25920109792034,
120.591621423541));
#231111=CARTESIAN_POINT('Ctrl Pts',(-7.77687976097489,1.46551493528119,
120.583210073475));
#231112=CARTESIAN_POINT('Ctrl Pts',(-7.73545518240527,1.67039873955153,
120.574798723409));
#231113=CARTESIAN_POINT('Ctrl Pts',(-7.68602535642838,1.87321520929656,
120.566387373343));
#231114=CARTESIAN_POINT('Ctrl Pts',(-7.63571452237108,2.07964656024245,
120.557826104332));
#231115=CARTESIAN_POINT('Ctrl Pts',(-7.57711049069753,2.28393590058186,
120.549264835321));
#231116=CARTESIAN_POINT('Ctrl Pts',(-7.51043042045454,2.48542871543543,
120.54070356631));
#231117=CARTESIAN_POINT('Ctrl Pts',(-7.44375035021156,2.686921530289,120.532142297299));
#231118=CARTESIAN_POINT('Ctrl Pts',(-7.36899437388891,2.88561754922279,
120.523581028288));
#231119=CARTESIAN_POINT('Ctrl Pts',(-7.28643086389093,3.08088400718651,
120.515019759277));
#231120=CARTESIAN_POINT('Ctrl Pts',(-7.20254663432856,3.27927402701565,
120.506321540716));
#231121=CARTESIAN_POINT('Ctrl Pts',(-7.110535319717,3.4742852672912,120.497623322156));
#231122=CARTESIAN_POINT('Ctrl Pts',(-7.01068098269354,3.66527941075426,
120.488925103595));
#231123=CARTESIAN_POINT('Ctrl Pts',(-6.91091438109058,3.85610574025963,
120.480234527586));
#231124=CARTESIAN_POINT('Ctrl Pts',(-6.80331862294041,4.04292181806838,
120.471543951577));
#231125=CARTESIAN_POINT('Ctrl Pts',(-6.68822440143792,4.22511246667001,
120.462853375567));
#231126=CARTESIAN_POINT('Ctrl Pts',(-6.57036992268928,4.41167251845644,
120.453954377058));
#231127=CARTESIAN_POINT('Ctrl Pts',(-6.44465290972965,4.59338228731657,
120.445055378548));
#231128=CARTESIAN_POINT('Ctrl Pts',(-6.31147843001338,4.76960805805632,
120.436156380038));
#231129=CARTESIAN_POINT('Ctrl Pts',(-6.18180622154059,4.94119937893348,
120.427491410651));
#231130=CARTESIAN_POINT('Ctrl Pts',(-6.04506393641537,5.10759126157416,
120.418826441263));
#231131=CARTESIAN_POINT('Ctrl Pts',(-5.90167009850677,5.26822655628923,
120.410161471876));
#231132=CARTESIAN_POINT('Ctrl Pts',(-5.75246694971074,5.43536966459033,
120.401145458805));
#231133=CARTESIAN_POINT('Ctrl Pts',(-5.59606220092296,5.59627984384596,
120.392129445734));
#231134=CARTESIAN_POINT('Ctrl Pts',(-5.43297594668917,5.75036462867329,
120.383113432664));
#231135=CARTESIAN_POINT('Ctrl Pts',(-5.26988969245527,5.90444941350073,
120.374097419593));
#231136=CARTESIAN_POINT('Ctrl Pts',(-5.10012208988998,6.05170856300526,
120.365081406522));
#231137=CARTESIAN_POINT('Ctrl Pts',(-4.92424059686758,6.1915890968443,120.356065393452));
#231138=CARTESIAN_POINT('Ctrl Pts',(-4.77187701342577,6.31276557211311,
120.348254952249));
#231139=CARTESIAN_POINT('Ctrl Pts',(-4.61499064308439,6.42835209568637,
120.340444511047));
#231140=CARTESIAN_POINT('Ctrl Pts',(-4.45403904311079,6.53800100966991,
120.332634069845));
#231141=CARTESIAN_POINT('Ctrl Pts',(-4.29309904742363,6.64764201818742,
120.32482419176));
#231142=CARTESIAN_POINT('Ctrl Pts',(-4.12809469697285,6.75134607155191,
120.317014313675));
#231143=CARTESIAN_POINT('Ctrl Pts',(-3.95951323902655,6.84880835693141,
120.30920443559));
#231144=CARTESIAN_POINT('Ctrl Pts',(-3.79091417992887,6.94628081809453,
120.301393742096));
#231145=CARTESIAN_POINT('Ctrl Pts',(-3.61873757474325,7.03751003765976,
120.293583048601));
#231146=CARTESIAN_POINT('Ctrl Pts',(-3.44349613871934,7.12223668117151,
120.285772355107));
#231147=CARTESIAN_POINT('Ctrl Pts',(-3.26813034162216,7.20702345142362,
120.27795611871));
#231148=CARTESIAN_POINT('Ctrl Pts',(-3.08969568584033,7.28529827283452,
120.270139882314));
#231149=CARTESIAN_POINT('Ctrl Pts',(-2.90872658560965,7.35684923388862,
120.262323645917));
#231150=CARTESIAN_POINT('Ctrl Pts',(-2.7276905784827,7.42842664836888,120.254504519744));
#231151=CARTESIAN_POINT('Ctrl Pts',(-2.54411859056901,7.49327512860597,
120.246685393572));
#231152=CARTESIAN_POINT('Ctrl Pts',(-2.35856127198287,7.5512323316332,120.238866267399));
#231153=CARTESIAN_POINT('Ctrl Pts',(-2.17279761910007,7.60925398137056,
120.231038446587));
#231154=CARTESIAN_POINT('Ctrl Pts',(-1.9850445641325,7.66036894975479,120.223210625776));
#231155=CARTESIAN_POINT('Ctrl Pts',(-1.79586513157526,7.70446555117175,
120.215382804964));
#231156=CARTESIAN_POINT('Ctrl Pts',(-1.64867029273373,7.73877579331218,
120.209292212518));
#231157=CARTESIAN_POINT('Ctrl Pts',(-1.50061219689754,7.76883818722276,
120.203201620073));
#231158=CARTESIAN_POINT('Ctrl Pts',(-1.3519584093979,7.79462182913695,120.197111027627));
#231159=CARTESIAN_POINT('Ctrl Pts',(-1.15384637310099,7.82898388535286,
120.188994048625));
#231160=CARTESIAN_POINT('Ctrl Pts',(-0.954282375878709,7.85581318678384,
120.180877069623));
#231161=CARTESIAN_POINT('Ctrl Pts',(-0.753866334332839,7.87499882856878,
120.172760090621));
#231162=CARTESIAN_POINT('Ctrl Pts',(-0.553596890164613,7.89417043672271,
120.164649048907));
#231163=CARTESIAN_POINT('Ctrl Pts',(-0.352476962419628,7.90570950263969,
120.156538007194));
#231164=CARTESIAN_POINT('Ctrl Pts',(-0.151114232342218,7.90955659242562,
120.14842696548));
#231165=CARTESIAN_POINT('Ctrl Pts',(0.0501298381038666,7.91340141518699,
120.140320703465));
#231166=CARTESIAN_POINT('Ctrl Pts',(0.251616105748743,7.90956329425575,
120.132214441451));
#231167=CARTESIAN_POINT('Ctrl Pts',(0.452733642698382,7.89803477130666,
120.124108179436));
#231168=CARTESIAN_POINT('Ctrl Pts',(0.653761229303729,7.8865114045196,120.116005542968));
#231169=CARTESIAN_POINT('Ctrl Pts',(0.854420094469794,7.86730451340781,
120.1079029065));
#231170=CARTESIAN_POINT('Ctrl Pts',(1.05410060874855,7.84045871787078,120.099800270033));
#231171=CARTESIAN_POINT('Ctrl Pts',(1.25372015268909,7.81362111941417,120.091700107619));
#231172=CARTESIAN_POINT('Ctrl Pts',(1.45236162407149,7.77914931137497,120.083599945206));
#231173=CARTESIAN_POINT('Ctrl Pts',(1.64942122828133,7.73713969188194,120.075499782793));
#231174=CARTESIAN_POINT('Ctrl Pts',(1.84840028926463,7.69472087818084,120.067320720842));
#231175=CARTESIAN_POINT('Ctrl Pts',(2.04576617395715,7.64461667052208,120.059141658892));
#231176=CARTESIAN_POINT('Ctrl Pts',(2.24090766890899,7.58697922887791,120.050962596941));
#231177=CARTESIAN_POINT('Ctrl Pts',(2.43416566604806,7.52989810148817,120.042862478965));
#231178=CARTESIAN_POINT('Ctrl Pts',(2.625241717471,7.46542863287169,120.03476236099));
#231179=CARTESIAN_POINT('Ctrl Pts',(2.81355695240561,7.39376888167125,120.026662243014));
#231180=CARTESIAN_POINT('Ctrl Pts',(3.00189753125902,7.32209948632854,120.018561034905));
#231181=CARTESIAN_POINT('Ctrl Pts',(3.18747625277086,7.24323799259667,120.010459826796));
#231182=CARTESIAN_POINT('Ctrl Pts',(3.36973331737352,7.15743098952291,120.002358618687));
#231183=CARTESIAN_POINT('Ctrl Pts',(3.55203844894086,7.07160135642272,119.994255274032));
#231184=CARTESIAN_POINT('Ctrl Pts',(3.73101988639512,6.97882269759998,119.986151929378));
#231185=CARTESIAN_POINT('Ctrl Pts',(3.90614107532493,6.8793882649302,119.978048584723));
#231186=CARTESIAN_POINT('Ctrl Pts',(4.08415480859021,6.77831143531962,119.969811393995));
#231187=CARTESIAN_POINT('Ctrl Pts',(4.25817935482203,6.67035720521288,119.961574203266));
#231188=CARTESIAN_POINT('Ctrl Pts',(4.42768062329741,6.55588020772776,119.953337012537));
#231189=CARTESIAN_POINT('Ctrl Pts',(4.59464480656754,6.44311669533496,119.945223115604));
#231190=CARTESIAN_POINT('Ctrl Pts',(4.75721993336558,6.32402453276771,119.93710921867));
#231191=CARTESIAN_POINT('Ctrl Pts',(4.91492768655627,6.19898433906093,119.928995321737));
#231192=CARTESIAN_POINT('Ctrl Pts',(5.07623008501358,6.07109409434934,119.92069648411));
#231193=CARTESIAN_POINT('Ctrl Pts',(5.23244030786489,5.93698167287731,119.912397646484));
#231194=CARTESIAN_POINT('Ctrl Pts',(5.38308501857763,5.79709553852316,119.904098808857));
#231195=CARTESIAN_POINT('Ctrl Pts',(5.53372972929025,5.65720940416911,119.895799971231));
#231196=CARTESIAN_POINT('Ctrl Pts',(5.67880870147179,5.51154983408021,119.887501133604));
#231197=CARTESIAN_POINT('Ctrl Pts',(5.81789105147127,5.36060301768472,119.879202295978));
#231198=CARTESIAN_POINT('Ctrl Pts',(5.95069117764302,5.21647433232227,119.871278309333));
#231199=CARTESIAN_POINT('Ctrl Pts',(6.0783092372046,5.06721585926902,119.863354322688));
#231200=CARTESIAN_POINT('Ctrl Pts',(6.20032688890408,4.9132339116648,119.855430336044));
#231201=CARTESIAN_POINT('Ctrl Pts',(6.32221389513008,4.75941683401319,119.847514833688));
#231202=CARTESIAN_POINT('Ctrl Pts',(6.43851222620911,4.60088662091117,119.839599331332));
#231203=CARTESIAN_POINT('Ctrl Pts',(6.54884061410087,4.43808603016018,119.831683828976));
#231204=CARTESIAN_POINT('Ctrl Pts',(6.65906907508675,4.27543289157104,119.823775495869));
#231205=CARTESIAN_POINT('Ctrl Pts',(6.76333817336143,4.10851736181211,119.815867162762));
#231206=CARTESIAN_POINT('Ctrl Pts',(6.86130698010753,3.93781506989952,119.807958829655));
#231207=CARTESIAN_POINT('Ctrl Pts',(6.95918939571486,3.76726330717961,119.800057470298));
#231208=CARTESIAN_POINT('Ctrl Pts',(7.05078242589187,3.59293173501396,119.79215611094));
#231209=CARTESIAN_POINT('Ctrl Pts',(7.13578851470322,3.41532476836824,119.784254751582));
#231210=CARTESIAN_POINT('Ctrl Pts',(7.22075083607071,3.23780924697133,119.776357460431));
#231211=CARTESIAN_POINT('Ctrl Pts',(7.29913282465987,3.05702199843288,119.768460169279));
#231212=CARTESIAN_POINT('Ctrl Pts',(7.37068263227046,2.87349239329888,119.760562878128));
#231213=CARTESIAN_POINT('Ctrl Pts',(7.44220811533019,2.69002518211625,119.752668271792));
#231214=CARTESIAN_POINT('Ctrl Pts',(7.50690592054313,2.50381779018915,119.744773665457));
#231215=CARTESIAN_POINT('Ctrl Pts',(7.5645720438335,2.31542021966913,119.736879059121));
#231216=CARTESIAN_POINT('Ctrl Pts',(7.60506605087208,2.18312465146743,119.731335349465));
#231217=CARTESIAN_POINT('Ctrl Pts',(7.64209368900089,2.04974954280903,119.725791639809));
#231218=CARTESIAN_POINT('Ctrl Pts',(7.67559886220684,1.9154903044623,119.720247930153));
#231219=CARTESIAN_POINT('Ctrl Pts',(7.72709100046858,1.70915514477309,119.711728127484));
#231220=CARTESIAN_POINT('Ctrl Pts',(7.77021027758681,1.50093760967826,119.703208324815));
#231221=CARTESIAN_POINT('Ctrl Pts',(7.80486517080185,1.29151100096133,119.694688522146));
#231222=CARTESIAN_POINT('Ctrl Pts',(7.83958274037241,1.08170562620691,119.686153310681));
#231223=CARTESIAN_POINT('Ctrl Pts',(7.86580528925962,0.870687053414497,
119.677618099217));
#231224=CARTESIAN_POINT('Ctrl Pts',(7.88349314166519,0.659133435138885,
119.669082887752));
#231225=CARTESIAN_POINT('Ctrl Pts',(7.90210781074785,0.436494727671951,
119.660100444133));
#231226=CARTESIAN_POINT('Ctrl Pts',(7.91126947324658,0.213263758363993,
119.651118000514));
#231227=CARTESIAN_POINT('Ctrl Pts',(7.91099396437362,-0.00977218728067248,
119.642135556896));
#231228=CARTESIAN_POINT('Ctrl Pts',(7.91073107405129,-0.222592888874181,
119.633564517159));
#231229=CARTESIAN_POINT('Ctrl Pts',(7.90187616522459,-0.435235809622482,
119.624993477421));
#231230=CARTESIAN_POINT('Ctrl Pts',(7.88449626961741,-0.647023627380878,
119.616422437684));
#231231=CARTESIAN_POINT('Ctrl Pts',(7.86709456537519,-0.85907720066102,
119.607840642838));
#231232=CARTESIAN_POINT('Ctrl Pts',(7.84114652881282,-1.07027327980192,
119.599258847991));
#231233=CARTESIAN_POINT('Ctrl Pts',(7.80677070269115,-1.27994226260526,
119.590677053144));
#231234=CARTESIAN_POINT('Ctrl Pts',(7.77233737656482,-1.48996195603431,
119.582080903639));
#231235=CARTESIAN_POINT('Ctrl Pts',(7.72944811778225,-1.69844920048983,
119.573484754134));
#231236=CARTESIAN_POINT('Ctrl Pts',(7.67827243744755,-1.90474496359311,
119.564888604629));
#231237=CARTESIAN_POINT('Ctrl Pts',(7.67113828848329,-1.93350363753839,
119.563690257862));
#231238=CARTESIAN_POINT('Ctrl Pts',(7.66384318186019,-1.96221974818347,
119.562491911095));
#231239=CARTESIAN_POINT('Ctrl Pts',(7.6563876530204,-1.99089153563845,119.561293564328));
#231240=CARTESIAN_POINT('Ctrl Pts',(7.60718904108358,-2.18009503479242,
119.553385741981));
#231241=CARTESIAN_POINT('Ctrl Pts',(7.55090996100169,-2.36771584605605,
119.545477919635));
#231242=CARTESIAN_POINT('Ctrl Pts',(7.48766754116734,-2.55318542079281,
119.537570097288));
#231243=CARTESIAN_POINT('Ctrl Pts',(7.42448973161107,-2.73846551446876,
119.529670353801));
#231244=CARTESIAN_POINT('Ctrl Pts',(7.35436286295951,-2.92159842557687,
119.521770610313));
#231245=CARTESIAN_POINT('Ctrl Pts',(7.27745470569158,-3.10202740262033,
119.513870866826));
#231246=CARTESIAN_POINT('Ctrl Pts',(7.20061083917921,-3.28230555151149,
119.505977727065));
#231247=CARTESIAN_POINT('Ctrl Pts',(7.11699711146433,-3.45988395372397,
119.498084587305));
#231248=CARTESIAN_POINT('Ctrl Pts',(7.02683065685552,-3.63422232669872,
119.490191447545));
#231249=CARTESIAN_POINT('Ctrl Pts',(6.93672283806905,-3.80844732631406,
119.482303440744));
#231250=CARTESIAN_POINT('Ctrl Pts',(6.84007094039396,-3.97943618941263,
119.474415433942));
#231251=CARTESIAN_POINT('Ctrl Pts',(6.73713974614513,-4.14666963247755,
119.466527427141));
#231252=CARTESIAN_POINT('Ctrl Pts',(6.63425638482468,-4.3138253608578,119.458643085959));
#231253=CARTESIAN_POINT('Ctrl Pts',(6.52509972209648,-4.47722885365726,
119.450758744776));
#231254=CARTESIAN_POINT('Ctrl Pts',(6.409980050507,-4.63638617374592,119.442874403593));
#231255=CARTESIAN_POINT('Ctrl Pts',(6.29489251298313,-4.79549906726788,
119.434992263215));
#231256=CARTESIAN_POINT('Ctrl Pts',(6.17384548609188,-4.9503678712725,119.427110122837));
#231257=CARTESIAN_POINT('Ctrl Pts',(6.04719223231534,-5.10052812024647,
119.419227982459));
#231258=CARTESIAN_POINT('Ctrl Pts',(5.92052512982028,-5.25070478827767,
119.41134498022));
#231259=CARTESIAN_POINT('Ctrl Pts',(5.78825079264541,-5.3961716043426,119.40346197798));
#231260=CARTESIAN_POINT('Ctrl Pts',(5.6507627768379,-5.53649718142286,119.395578975741));
#231261=CARTESIAN_POINT('Ctrl Pts',(5.51325817950287,-5.67683968225028,
119.387695022785));
#231262=CARTESIAN_POINT('Ctrl Pts',(5.37053889165724,-5.81203946155636,
119.379811069828));
#231263=CARTESIAN_POINT('Ctrl Pts',(5.22303531336471,-5.94170203858669,
119.371927116872));
#231264=CARTESIAN_POINT('Ctrl Pts',(5.075489139727,-6.07140205892714,119.364040887227));
#231265=CARTESIAN_POINT('Ctrl Pts',(4.92315618160286,-6.19556146279644,
119.356154657582));
#231266=CARTESIAN_POINT('Ctrl Pts',(4.76650006525322,-6.31382595008296,
119.348268427937));
#231267=CARTESIAN_POINT('Ctrl Pts',(4.60977236485902,-6.43214447835125,
119.340378594678));
#231268=CARTESIAN_POINT('Ctrl Pts',(4.44871784478241,-6.54456251468769,
119.332488761419));
#231269=CARTESIAN_POINT('Ctrl Pts',(4.28382944230653,-6.65076885098465,
119.324598928159));
#231270=CARTESIAN_POINT('Ctrl Pts',(4.11875088070683,-6.75709767075257,
119.316699995875));
#231271=CARTESIAN_POINT('Ctrl Pts',(3.9498298952369,-6.85720029470447,119.30880106359));
#231272=CARTESIAN_POINT('Ctrl Pts',(3.77758538487601,-6.95081071961905,
119.300902131305));
#231273=CARTESIAN_POINT('Ctrl Pts',(3.60522710958061,-7.04448297282552,
119.292997981893));
#231274=CARTESIAN_POINT('Ctrl Pts',(3.4295412413218,-7.131654325894,119.285093832481));
#231275=CARTESIAN_POINT('Ctrl Pts',(3.25106724203831,-7.21210668166698,
119.27718968307));
#231276=CARTESIAN_POINT('Ctrl Pts',(3.07234865058636,-7.29266929448711,
119.269274701306));
#231277=CARTESIAN_POINT('Ctrl Pts',(2.89083461439281,-7.36649438833812,
119.261359719543));
#231278=CARTESIAN_POINT('Ctrl Pts',(2.70708146099895,-7.43341314360475,
119.25344473778));
#231279=CARTESIAN_POINT('Ctrl Pts',(2.62923165916585,-7.46176428610328,
119.25009143608));
#231280=CARTESIAN_POINT('Ctrl Pts',(2.55098010368526,-7.4888764183176,119.246738134379));
#231281=CARTESIAN_POINT('Ctrl Pts',(2.47236966538131,-7.5147394657235,119.243384832678));
#231282=CARTESIAN_POINT('Ctrl Pts',(2.29044769764415,-7.57459228651009,
119.235624549732));
#231283=CARTESIAN_POINT('Ctrl Pts',(2.10603030035115,-7.62794040411432,
119.227864266785));
#231284=CARTESIAN_POINT('Ctrl Pts',(1.91963366571711,-7.67456367420621,
119.220103983839));
#231285=CARTESIAN_POINT('Ctrl Pts',(1.73346136875679,-7.72113083086035,
119.212353040781));
#231286=CARTESIAN_POINT('Ctrl Pts',(1.54531491949674,-7.76098916388495,
119.204602097723));
#231287=CARTESIAN_POINT('Ctrl Pts',(1.35572989318228,-7.79396673438705,
119.196851154665));
#231288=CARTESIAN_POINT('Ctrl Pts',(1.16633456184877,-7.82691130819247,
119.189107967046));
#231289=CARTESIAN_POINT('Ctrl Pts',(0.975503869296235,-7.85298876381619,
119.181364779426));
#231290=CARTESIAN_POINT('Ctrl Pts',(0.783788036869903,-7.87207706474344,
119.173621591807));
#231291=CARTESIAN_POINT('Ctrl Pts',(0.592225175821566,-7.89115013498442,
119.16588458253));
#231292=CARTESIAN_POINT('Ctrl Pts',(0.399778936163565,-7.90324511807019,
119.158147573253));
#231293=CARTESIAN_POINT('Ctrl Pts',(0.207009301237229,-7.90829110169835,
119.150410563976));
#231294=CARTESIAN_POINT('Ctrl Pts',(0.0143544498453649,-7.91333408072552,
119.142678161655));
#231295=CARTESIAN_POINT('Ctrl Pts',(-0.178623055673287,-7.91133640881234,
119.134945759334));
#231296=CARTESIAN_POINT('Ctrl Pts',(-0.371358452897033,-7.9022790319921,
119.127213357014));
#231297=CARTESIAN_POINT('Ctrl Pts',(-0.564018081155927,-7.89322521584662,
119.119483994488));
#231298=CARTESIAN_POINT('Ctrl Pts',(-0.75643543260841,-7.87711723920018,
119.111754631962));
#231299=CARTESIAN_POINT('Ctrl Pts',(-0.948045998137102,-7.85398814523018,
119.104025269437));
#231300=CARTESIAN_POINT('Ctrl Pts',(-1.13965648890694,-7.83085906028424,
119.096295909927));
#231301=CARTESIAN_POINT('Ctrl Pts',(-1.3304598366005,-7.80070889512617,
119.088566550417));
#231302=CARTESIAN_POINT('Ctrl Pts',(-1.5198964984915,-7.76362258445587,
119.080837190907));
#231303=CARTESIAN_POINT('Ctrl Pts',(-1.709342655628,-7.72653441488656,119.073107443974));
#231304=CARTESIAN_POINT('Ctrl Pts',(-1.89742163769417,-7.6825094755358,
119.065377697041));
#231305=CARTESIAN_POINT('Ctrl Pts',(-2.08358411429127,-7.63168384032469,
119.057647950107));
#231306=CARTESIAN_POINT('Ctrl Pts',(-2.26979003381238,-7.58084634443012,
119.049916399359));
#231307=CARTESIAN_POINT('Ctrl Pts',(-2.45407821065823,-7.52320508683362,
119.04218484861));
#231308=CARTESIAN_POINT('Ctrl Pts',(-2.63591444857387,-7.45894603947498,
119.034453297861));
#231309=CARTESIAN_POINT('Ctrl Pts',(-2.81782644964922,-7.39466021819865,
119.026718525715));
#231310=CARTESIAN_POINT('Ctrl Pts',(-2.9972841391664,-7.32375123608725,
119.018983753569));
#231311=CARTESIAN_POINT('Ctrl Pts',(-3.17377322716147,-7.24645323607026,
119.011248981423));
#231312=CARTESIAN_POINT('Ctrl Pts',(-3.35047277848421,-7.16906305814872,
119.003504985557));
#231313=CARTESIAN_POINT('Ctrl Pts',(-3.52419632934436,-7.08526879055976,
118.995760989692));
#231314=CARTESIAN_POINT('Ctrl Pts',(-3.694453207486,-6.99535106322023,118.988016993826));
#231315=CARTESIAN_POINT('Ctrl Pts',(-3.86482059088245,-6.90537497476495,
118.980267971719));
#231316=CARTESIAN_POINT('Ctrl Pts',(-4.0317165097013,-6.80926768825269,
118.972518949611));
#231317=CARTESIAN_POINT('Ctrl Pts',(-4.19467935553122,-6.7073531369893,
118.964769927504));
#231318=CARTESIAN_POINT('Ctrl Pts',(-4.35789124697762,-6.60528283628425,
118.957009063065));
#231319=CARTESIAN_POINT('Ctrl Pts',(-4.51715776492919,-6.49738774640278,
118.949248198626));
#231320=CARTESIAN_POINT('Ctrl Pts',(-4.6720495024841,-6.38403277296867,
118.941487334188));
#231321=CARTESIAN_POINT('Ctrl Pts',(-4.77856717819169,-6.30607956196659,
118.936150256468));
#231322=CARTESIAN_POINT('Ctrl Pts',(-4.88301665375129,-6.22554509245663,
118.930813178748));
#231323=CARTESIAN_POINT('Ctrl Pts',(-4.98526863013717,-6.14255791062406,
118.925476101028));
#231324=CARTESIAN_POINT('Ctrl Pts',(-5.13739362236662,-6.01909404383501,
118.917535883779));
#231325=CARTESIAN_POINT('Ctrl Pts',(-5.28513570249431,-5.8898081660217,
118.90959566653));
#231326=CARTESIAN_POINT('Ctrl Pts',(-5.42802194939112,-5.75504115684052,
118.901655449281));
#231327=CARTESIAN_POINT('Ctrl Pts',(-5.57074417390803,-5.62042884978118,
118.893724346788));
#231328=CARTESIAN_POINT('Ctrl Pts',(-5.7086214224054,-5.48034817828785,
118.885793244296));
#231329=CARTESIAN_POINT('Ctrl Pts',(-5.84121220755203,-5.33518143518523,
118.877862141803));
#231330=CARTESIAN_POINT('Ctrl Pts',(-5.97367496823488,-5.19015485939834,
118.869938697272));
#231331=CARTESIAN_POINT('Ctrl Pts',(-6.10086120575228,-5.04005224749073,
118.862015252741));
#231332=CARTESIAN_POINT('Ctrl Pts',(-6.22236458861824,-4.88529425176311,
118.85409180821));
#231333=CARTESIAN_POINT('Ctrl Pts',(-6.34377280199706,-4.7306574727353,
118.846174569845));
#231334=CARTESIAN_POINT('Ctrl Pts',(-6.45950681961976,-4.57137284403264,
118.83825733148));
#231335=CARTESIAN_POINT('Ctrl Pts',(-6.56919888362942,-4.40789598644547,
118.830340093115));
#231336=CARTESIAN_POINT('Ctrl Pts',(-6.67882041729674,-4.24452424201149,
118.822427945414));
#231337=CARTESIAN_POINT('Ctrl Pts',(-6.7824075511453,-4.07696592563811,
118.814515797714));
#231338=CARTESIAN_POINT('Ctrl Pts',(-6.87963422419451,-3.90570786686506,
118.806603650014));
#231339=CARTESIAN_POINT('Ctrl Pts',(-6.97682642627412,-3.73451052632038,
118.798694307504));
#231340=CARTESIAN_POINT('Ctrl Pts',(-7.06766249101362,-3.55961635387914,
118.790784964995));
#231341=CARTESIAN_POINT('Ctrl Pts',(-7.15186067466932,-3.38153957393944,
118.782875622486));
#231342=CARTESIAN_POINT('Ctrl Pts',(-7.23604290927774,-3.20349652578421,
118.774967778186));
#231343=CARTESIAN_POINT('Ctrl Pts',(-7.31358962186788,-3.02227238087351,
118.767059933886));
#231344=CARTESIAN_POINT('Ctrl Pts',(-7.38426575303584,-2.83840453222265,
118.759152089586));
#231345=CARTESIAN_POINT('Ctrl Pts',(-7.45494016611141,-2.65454115328379,
118.75124443752));
#231346=CARTESIAN_POINT('Ctrl Pts',(-7.51874420845123,-2.46803451864746,
118.743336785455));
#231347=CARTESIAN_POINT('Ctrl Pts',(-7.57549145837475,-2.27944075687244,
118.735429133389));
#231348=CARTESIAN_POINT('Ctrl Pts',(-7.63226697869891,-2.09075304127216,
118.727517541882));
#231349=CARTESIAN_POINT('Ctrl Pts',(-7.68197858067864,-1.89997644855941,
118.719605950375));
#231350=CARTESIAN_POINT('Ctrl Pts',(-7.72448986496527,-1.70768185738702,
118.711694358868));
#231351=CARTESIAN_POINT('Ctrl Pts',(-7.76701132841194,-1.5153412220301,
118.703780872961));
#231352=CARTESIAN_POINT('Ctrl Pts',(-7.80232897046963,-1.32148219976192,
118.695867387054));
#231353=CARTESIAN_POINT('Ctrl Pts',(-7.83035771582106,-1.12668497916744,
118.687953901147));
#231354=CARTESIAN_POINT('Ctrl Pts',(-7.85841247724998,-0.931706949210253,
118.680033070001));
#231355=CARTESIAN_POINT('Ctrl Pts',(-7.87916478002963,-0.735789321072113,
118.672112238854));
#231356=CARTESIAN_POINT('Ctrl Pts',(-7.89258143142248,-0.539517699770027,
118.664191407707));
#231357=CARTESIAN_POINT('Ctrl Pts',(-7.90486777183239,-0.359781349654463,
118.656937881849));
#231358=CARTESIAN_POINT('Ctrl Pts',(-7.9110030092443,-0.179748378292146,
118.649684355992));
#231359=CARTESIAN_POINT('Ctrl Pts',(-7.91099999889219,0.000132392670232489,
118.642430830134));
#231360=CARTESIAN_POINT('',(-7.91099996199236,-0.000775472076273572,114.634517289408));
#231361=CARTESIAN_POINT('Ctrl Pts',(-7.91099999750142,0.000198827776959343,
118.644324710193));
#231362=CARTESIAN_POINT('Ctrl Pts',(-7.91099106136341,0.355751702830156,
118.631767639541));
#231363=CARTESIAN_POINT('Ctrl Pts',(-7.88701277954247,0.710905018268822,
118.618770631039));
#231364=CARTESIAN_POINT('Ctrl Pts',(-7.83644873986753,1.08370568293652,
118.60384143357));
#231365=CARTESIAN_POINT('Ctrl Pts',(-7.83359517610902,1.10414377095752,
118.603019502035));
#231366=CARTESIAN_POINT('Ctrl Pts',(-7.82901350979031,1.1360470478016,118.601731273111));
#231367=CARTESIAN_POINT('Ctrl Pts',(-7.82734010322373,1.14752008178653,
118.601266946033));
#231368=CARTESIAN_POINT('Ctrl Pts',(-7.82449765892094,1.16671262214085,
118.60048847286));
#231369=CARTESIAN_POINT('Ctrl Pts',(-7.82334240166554,1.17443417138983,
118.600174808686));
#231370=CARTESIAN_POINT('Ctrl Pts',(-7.82122460117877,1.18844741145488,
118.599604725457));
#231371=CARTESIAN_POINT('Ctrl Pts',(-7.82026589108492,1.19473968057792,
118.599348437834));
#231372=CARTESIAN_POINT('Ctrl Pts',(-7.81829152397392,1.20759377912051,
118.598824263193));
#231373=CARTESIAN_POINT('Ctrl Pts',(-7.81727519732579,1.21415550000509,
118.598556353796));
#231374=CARTESIAN_POINT('Ctrl Pts',(-7.81503628937616,1.22849123963937,
118.597970324945));
#231375=CARTESIAN_POINT('Ctrl Pts',(-7.81381036744397,1.23626472540433,
118.597652095217));
#231376=CARTESIAN_POINT('Ctrl Pts',(-7.81042331473759,1.25753548323976,
118.596780079973));
#231377=CARTESIAN_POINT('Ctrl Pts',(-7.8082388020532,1.27102897474806,118.596225538105));
#231378=CARTESIAN_POINT('Ctrl Pts',(-7.79738594568447,1.33698187922346,
118.593508576135));
#231379=CARTESIAN_POINT('Ctrl Pts',(-7.78822393567046,1.38935809875853,
118.591330811541));
#231380=CARTESIAN_POINT('Ctrl Pts',(-7.70012354868957,1.86471476825476,
118.571400921319));
#231381=CARTESIAN_POINT('Ctrl Pts',(-7.58732784647485,2.28068047838237,
118.552822236139));
#231382=CARTESIAN_POINT('Ctrl Pts',(-7.41540952306428,2.75706883980788,
118.531032738851));
#231383=CARTESIAN_POINT('Ctrl Pts',(-7.38851018548077,2.8283642379192,118.527756104055));
#231384=CARTESIAN_POINT('Ctrl Pts',(-7.13734293989879,3.46602276743735,
118.498325232205));
#231385=CARTESIAN_POINT('Ctrl Pts',(-6.84938009783869,4.00512489118188,
118.472784453132));
#231386=CARTESIAN_POINT('Ctrl Pts',(-6.36931748935878,4.69790541579123,
118.438088876225));
#231387=CARTESIAN_POINT('Ctrl Pts',(-6.22778336131068,4.88397770089324,
118.428519820094));
#231388=CARTESIAN_POINT('Ctrl Pts',(-6.05541147508588,5.09089212345301,
118.417608050055));
#231389=CARTESIAN_POINT('Ctrl Pts',(-6.03241913001597,5.11811588370871,
118.416166635528));
#231390=CARTESIAN_POINT('Ctrl Pts',(-5.99391169001065,5.16309009869847,
118.413775754193));
#231391=CARTESIAN_POINT('Ctrl Pts',(-5.97849981594452,5.18092816683152,
118.412824908859));
#231392=CARTESIAN_POINT('Ctrl Pts',(-5.94816135999849,5.21572697584266,
118.410964943565));
#231393=CARTESIAN_POINT('Ctrl Pts',(-5.93324139611308,5.23269318710021,
118.410055741633));
#231394=CARTESIAN_POINT('Ctrl Pts',(-5.90500037625875,5.26453133395445,
118.408345054883));
#231395=CARTESIAN_POINT('Ctrl Pts',(-5.89169530800487,5.27941720363808,
118.407543348253));
#231396=CARTESIAN_POINT('Ctrl Pts',(-5.86159034698265,5.31284345481193,
118.405738840661));
#231397=CARTESIAN_POINT('Ctrl Pts',(-5.84475855154929,5.33135484192352,
118.404736519601));
#231398=CARTESIAN_POINT('Ctrl Pts',(-5.79517202648474,5.3853723835909,118.401802790383));
#231399=CARTESIAN_POINT('Ctrl Pts',(-5.76217947365969,5.42065884166639,
118.399875013768));
#231400=CARTESIAN_POINT('Ctrl Pts',(-5.4453582577686,5.753346819243,118.381587992475));
#231401=CARTESIAN_POINT('Ctrl Pts',(-5.13907273323627,6.02850500968855,
118.365645121367));
#231402=CARTESIAN_POINT('Ctrl Pts',(-4.59084093686234,6.4487442649206,118.339066656222));
#231403=CARTESIAN_POINT('Ctrl Pts',(-4.36003503901393,6.60698230071374,
118.328372571815));
#231404=CARTESIAN_POINT('Ctrl Pts',(-3.96026396694388,6.85097363783537,
118.310219311058));
#231405=CARTESIAN_POINT('Ctrl Pts',(-3.79572699290668,6.94348499568284,
118.302842968806));
#231406=CARTESIAN_POINT('Ctrl Pts',(-3.59628254169681,7.046414007054,118.293895506484));
#231407=CARTESIAN_POINT('Ctrl Pts',(-3.564410431711,7.06258994430526,118.292465440846));
#231408=CARTESIAN_POINT('Ctrl Pts',(-3.51985132493643,7.0848264111623,118.290464814799));
#231409=CARTESIAN_POINT('Ctrl Pts',(-3.50725597643418,7.09107002782422,
118.28989915939));
#231410=CARTESIAN_POINT('Ctrl Pts',(-3.48560266717887,7.10173194463671,
118.288926507233));
#231411=CARTESIAN_POINT('Ctrl Pts',(-3.47655276299725,7.10616657926794,
118.288519930332));
#231412=CARTESIAN_POINT('Ctrl Pts',(-3.46144228021639,7.11353524484304,
118.287840989445));
#231413=CARTESIAN_POINT('Ctrl Pts',(-3.45538637631346,7.11647885748803,
118.287568863956));
#231414=CARTESIAN_POINT('Ctrl Pts',(-3.437701886152,7.1250469191751,118.286774142821));
#231415=CARTESIAN_POINT('Ctrl Pts',(-3.42606329110939,7.13065061424208,
118.286251043711));
#231416=CARTESIAN_POINT('Ctrl Pts',(-3.39079549424877,7.14752490594762,
118.284665763407));
#231417=CARTESIAN_POINT('Ctrl Pts',(-3.36712409314705,7.15870670548321,
118.283601519787));
#231418=CARTESIAN_POINT('Ctrl Pts',(-3.15742247371022,7.25649447877688,
118.274173061075));
#231419=CARTESIAN_POINT('Ctrl Pts',(-2.96814693131328,7.33594773395008,
118.265661294186));
#231420=CARTESIAN_POINT('Ctrl Pts',(-2.67972256895294,7.4440297723605,118.252791580943));
#231421=CARTESIAN_POINT('Ctrl Pts',(-2.58274988674574,7.47822807565744,
118.248480890511));
#231422=CARTESIAN_POINT('Ctrl Pts',(-2.14481439325722,7.62313541998329,
118.229115938397));
#231423=CARTESIAN_POINT('Ctrl Pts',(-1.79722396849072,7.71248440121074,
118.21403978491));
#231424=CARTESIAN_POINT('Ctrl Pts',(-1.26691953518036,7.81098961437478,
118.191673498208));
#231425=CARTESIAN_POINT('Ctrl Pts',(-1.08798416761233,7.8379165674423,118.184228848384));
#231426=CARTESIAN_POINT('Ctrl Pts',(-0.813143558300402,7.86968173154199,
118.172940058753));
#231427=CARTESIAN_POINT('Ctrl Pts',(-0.717813786335819,7.87894895602759,
118.169050867178));
#231428=CARTESIAN_POINT('Ctrl Pts',(-0.594684962985234,7.88866530395628,
118.164058056211));
#231429=CARTESIAN_POINT('Ctrl Pts',(-0.567020027395226,7.89070204596984,
118.162938230848));
#231430=CARTESIAN_POINT('Ctrl Pts',(-0.512440120997703,7.8944317952196,
118.160732663178));
#231431=CARTESIAN_POINT('Ctrl Pts',(-0.485526069874737,7.89613276791149,
118.15964685432));
#231432=CARTESIAN_POINT('Ctrl Pts',(-0.434433687490773,7.89909960280163,
118.157588831313));
#231433=CARTESIAN_POINT('Ctrl Pts',(-0.410257223797544,7.90039215345614,
118.156616362609));
#231434=CARTESIAN_POINT('Ctrl Pts',(-0.355166678512057,7.90308390729053,
118.154403381692));
#231435=CARTESIAN_POINT('Ctrl Pts',(-0.324249529550282,7.90441274646032,
118.153163572298));
#231436=CARTESIAN_POINT('Ctrl Pts',(-0.24342019827765,7.90741181145971,
118.149927406893));
#231437=CARTESIAN_POINT('Ctrl Pts',(-0.193498505245793,7.90879088808833,
118.147933849117));
#231438=CARTESIAN_POINT('Ctrl Pts',(0.100507788589648,7.91412732279716,
118.136219368982));
#231439=CARTESIAN_POINT('Ctrl Pts',(0.344661485737856,7.90725769782168,
118.126584499178));
#231440=CARTESIAN_POINT('Ctrl Pts',(0.899194143444628,7.86591915778065,
118.104810475318));
#231441=CARTESIAN_POINT('Ctrl Pts',(1.20864364230712,7.82434818916022,118.092788265135));
#231442=CARTESIAN_POINT('Ctrl Pts',(1.93502465328261,7.68263484486815,118.064750749951));
#231443=CARTESIAN_POINT('Ctrl Pts',(2.34785991602701,7.56668706509408,118.04898910486));
#231444=CARTESIAN_POINT('Ctrl Pts',(2.97075612076491,7.3358241341791,118.024252212511));
#231445=CARTESIAN_POINT('Ctrl Pts',(3.1884335535939,7.24386588900238,118.015401345471));
#231446=CARTESIAN_POINT('Ctrl Pts',(3.47991695237149,7.10504127987971,118.002959158468));
#231447=CARTESIAN_POINT('Ctrl Pts',(3.5575510323201,7.06648878177986,117.99958536408));
#231448=CARTESIAN_POINT('Ctrl Pts',(3.67666333569253,7.00487811512001,117.994295836328));
#231449=CARTESIAN_POINT('Ctrl Pts',(3.71859486811153,6.98270884330381,117.992411636314));
#231450=CARTESIAN_POINT('Ctrl Pts',(3.77084777518922,6.95447849467578,117.990033082974));
#231451=CARTESIAN_POINT('Ctrl Pts',(3.78135862597255,6.9487690288601,117.989553068733));
#231452=CARTESIAN_POINT('Ctrl Pts',(3.79698649552106,6.94023405367322,117.98883698945));
#231453=CARTESIAN_POINT('Ctrl Pts',(3.8021134238384,6.93742666116076,117.988601688154));
#231454=CARTESIAN_POINT('Ctrl Pts',(3.81204023105679,6.93197665165687,117.988145346754));
#231455=CARTESIAN_POINT('Ctrl Pts',(3.81684048634643,6.92933472448194,117.987924336257));
#231456=CARTESIAN_POINT('Ctrl Pts',(3.82679765568827,6.92384108919891,117.987465181269));
#231457=CARTESIAN_POINT('Ctrl Pts',(3.83195413425719,6.92098860270391,117.987227003008));
#231458=CARTESIAN_POINT('Ctrl Pts',(3.84448670292844,6.91403747434703,117.986647144444));
#231459=CARTESIAN_POINT('Ctrl Pts',(3.85185942211341,6.90993279252586,117.986305197405));
#231460=CARTESIAN_POINT('Ctrl Pts',(3.87958544538451,6.89443846542512,117.985016106696));
#231461=CARTESIAN_POINT('Ctrl Pts',(3.89989478618646,6.88297069747746,117.984065434212));
#231462=CARTESIAN_POINT('Ctrl Pts',(4.12761216870934,6.75305754506152,117.973330748972));
#231463=CARTESIAN_POINT('Ctrl Pts',(4.32956761866814,6.62538888642573,117.963042008483));
#231464=CARTESIAN_POINT('Ctrl Pts',(4.59286943636232,6.44175709700302,117.948780094229));
#231465=CARTESIAN_POINT('Ctrl Pts',(4.65958468824241,6.39366516472849,117.945091026266));
#231466=CARTESIAN_POINT('Ctrl Pts',(5.14334612085052,6.03335038877545,117.917840476475));
#231467=CARTESIAN_POINT('Ctrl Pts',(5.52939826495414,5.68164675462671,117.89340905128));
#231468=CARTESIAN_POINT('Ctrl Pts',(5.94470320214601,5.2205684201839,117.865422654086));
#231469=CARTESIAN_POINT('Ctrl Pts',(6.00992587536757,5.1453495925788,117.860966317115));
#231470=CARTESIAN_POINT('Ctrl Pts',(6.22010001454147,4.89351336443058,117.846417871602));
#231471=CARTESIAN_POINT('Ctrl Pts',(6.35882649361934,4.71184179482672,117.836510816682));
#231472=CARTESIAN_POINT('Ctrl Pts',(6.57359713123326,4.40378964132639,117.820690995779));
#231473=CARTESIAN_POINT('Ctrl Pts',(6.65431589229357,4.28084400348727,117.814615313237));
#231474=CARTESIAN_POINT('Ctrl Pts',(6.7415008771862,4.13961891592254,117.807895559324));
#231475=CARTESIAN_POINT('Ctrl Pts',(6.75138031963018,4.12348670812215,117.807131681476));
#231476=CARTESIAN_POINT('Ctrl Pts',(6.76611132695088,4.09923748124737,117.805988996535));
#231477=CARTESIAN_POINT('Ctrl Pts',(6.77100632422291,4.09114699986086,117.805608673903));
#231478=CARTESIAN_POINT('Ctrl Pts',(6.77939101909424,4.07723245685653,117.80495614661));
#231479=CARTESIAN_POINT('Ctrl Pts',(6.78288774104903,4.07141265282832,117.804683697482));
#231480=CARTESIAN_POINT('Ctrl Pts',(6.79006506406966,4.05943209416671,117.804123807184));
#231481=CARTESIAN_POINT('Ctrl Pts',(6.793744783667,4.0532708170304,117.803836396795));
#231482=CARTESIAN_POINT('Ctrl Pts',(6.80360455741841,4.03671058624747,117.803065305712));
#231483=CARTESIAN_POINT('Ctrl Pts',(6.80976916296643,4.02630243269858,117.80258216138));
#231484=CARTESIAN_POINT('Ctrl Pts',(6.83214921944812,3.98831811979547,117.80082433255));
#231485=CARTESIAN_POINT('Ctrl Pts',(6.84822133197127,3.96065764729153,117.799554608042));
#231486=CARTESIAN_POINT('Ctrl Pts',(7.10145378703417,3.51868881962593,117.779428478398));
#231487=CARTESIAN_POINT('Ctrl Pts',(7.30081185460424,3.08383307414289,117.761961722015));
#231488=CARTESIAN_POINT('Ctrl Pts',(7.54591783043798,2.38956664829265,117.736053227547));
#231489=CARTESIAN_POINT('Ctrl Pts',(7.62005041465412,2.14143377204158,117.72714044994));
#231490=CARTESIAN_POINT('Ctrl Pts',(7.7746470775141,1.51311465575999,117.704784800351));
#231491=CARTESIAN_POINT('Ctrl Pts',(7.83952366448432,1.12981844899826,117.691341788531));
#231492=CARTESIAN_POINT('Ctrl Pts',(7.89065725190166,0.588032903391812,
117.671094480529));
#231493=CARTESIAN_POINT('Ctrl Pts',(7.90071746309055,0.432336532810252,
117.665131225176));
#231494=CARTESIAN_POINT('Ctrl Pts',(7.90710741650846,0.249590867320354,
117.657874724475));
#231495=CARTESIAN_POINT('Ctrl Pts',(7.90790969886776,0.222727332230216,
117.656801624431));
#231496=CARTESIAN_POINT('Ctrl Pts',(7.90879013129322,0.187176691278592,
117.655373513505));
#231497=CARTESIAN_POINT('Ctrl Pts',(7.90899088733893,0.178492570427434,
117.655024031185));
#231498=CARTESIAN_POINT('Ctrl Pts',(7.90929714994126,0.164227736506731,
117.654448942656));
#231499=CARTESIAN_POINT('Ctrl Pts',(7.90941105408813,0.15864719582357,117.654223706849));
#231500=CARTESIAN_POINT('Ctrl Pts',(7.90961887598819,0.147908263766134,
117.653789787719));
#231501=CARTESIAN_POINT('Ctrl Pts',(7.90971365389144,0.142749890159383,
117.653581141884));
#231502=CARTESIAN_POINT('Ctrl Pts',(7.90991898797164,0.130945723813463,
117.653103199151));
#231503=CARTESIAN_POINT('Ctrl Pts',(7.91002621472679,0.124299882584173,
117.652833759609));
#231504=CARTESIAN_POINT('Ctrl Pts',(7.91028800089844,0.106699438788301,
117.6521192689));
#231505=CARTESIAN_POINT('Ctrl Pts',(7.91042817966825,0.0957446605316113,
117.65167361203));
#231506=CARTESIAN_POINT('Ctrl Pts',(7.91119881181689,0.0238476818519216,
117.648742671783));
#231507=CARTESIAN_POINT('Ctrl Pts',(7.91114775289066,-0.0370987612768795,
117.64622956681));
#231508=CARTESIAN_POINT('Ctrl Pts',(7.90253949227138,-0.731677882831249,
117.617307792944));
#231509=CARTESIAN_POINT('Ctrl Pts',(7.81858423180687,-1.36207962219676,
117.588648613337));
#231510=CARTESIAN_POINT('Ctrl Pts',(7.56087480386716,-2.36127938693626,
117.543835652452));
#231511=CARTESIAN_POINT('Ctrl Pts',(7.43246074688659,-2.73880128897324,
117.526996031401));
#231512=CARTESIAN_POINT('Ctrl Pts',(7.24899631664689,-3.16871611595521,
117.507924261073));
#231513=CARTESIAN_POINT('Ctrl Pts',(7.22100175680082,-3.23200297625685,
117.50511813878));
#231514=CARTESIAN_POINT('Ctrl Pts',(7.18350805555592,-3.3138446784607,117.501488821225));
#231515=CARTESIAN_POINT('Ctrl Pts',(7.17476119706971,-3.33274005993869,
117.500650857603));
#231516=CARTESIAN_POINT('Ctrl Pts',(7.15998080358407,-3.36434150006342,
117.49924925356));
#231517=CARTESIAN_POINT('Ctrl Pts',(7.15398781086243,-3.37706636598281,
117.49868483027));
#231518=CARTESIAN_POINT('Ctrl Pts',(7.14249132531801,-3.40130880809513,
117.497609415941));
#231519=CARTESIAN_POINT('Ctrl Pts',(7.13699383239629,-3.41282917499417,
117.497098312037));
#231520=CARTESIAN_POINT('Ctrl Pts',(7.12436207501018,-3.43913587332755,
117.495931058534));
#231521=CARTESIAN_POINT('Ctrl Pts',(7.11720961159171,-3.45391341495088,
117.495275255922));
#231522=CARTESIAN_POINT('Ctrl Pts',(7.09843807119191,-3.49239096266952,
117.493567317545));
#231523=CARTESIAN_POINT('Ctrl Pts',(7.08674627335765,-3.51605531130416,
117.492516540184));
#231524=CARTESIAN_POINT('Ctrl Pts',(7.01899887444197,-3.65146617617828,
117.48650091363));
#231525=CARTESIAN_POINT('Ctrl Pts',(6.96041832273227,-3.76193143988808,
117.48158249291));
#231526=CARTESIAN_POINT('Ctrl Pts',(6.50594743903832,-4.57193782554782,
117.445400334699));
#231527=CARTESIAN_POINT('Ctrl Pts',(6.00815002531249,-5.20884137922286,
117.416855312353));
#231528=CARTESIAN_POINT('Ctrl Pts',(5.25144028937711,-5.92130102609426,
117.377900198792));
#231529=CARTESIAN_POINT('Ctrl Pts',(5.07277967403856,-6.07505782159162,
117.368908928476));
#231530=CARTESIAN_POINT('Ctrl Pts',(4.869018078646,-6.23515344034737,117.358619864292));
#231531=CARTESIAN_POINT('Ctrl Pts',(4.85043754468806,-6.24961847523805,
117.357681303783));
#231532=CARTESIAN_POINT('Ctrl Pts',(4.81797107495771,-6.27466177812577,
117.356040334179));
#231533=CARTESIAN_POINT('Ctrl Pts',(4.80411414303069,-6.28527748025144,
117.355339645518));
#231534=CARTESIAN_POINT('Ctrl Pts',(4.78394628551389,-6.30062228091296,
117.354319244729));
#231535=CARTESIAN_POINT('Ctrl Pts',(4.77766319066552,-6.30538798373337,
117.354001265694));
#231536=CARTESIAN_POINT('Ctrl Pts',(4.76662596985367,-6.31373370374274,
117.353442524444));
#231537=CARTESIAN_POINT('Ctrl Pts',(4.76187490398588,-6.31731777076396,
117.353201956901));
#231538=CARTESIAN_POINT('Ctrl Pts',(4.75271520623512,-6.32421137831187,
117.352738051876));
#231539=CARTESIAN_POINT('Ctrl Pts',(4.74830714863814,-6.32752168002281,
117.352514751499));
#231540=CARTESIAN_POINT('Ctrl Pts',(4.73788966803902,-6.33532783835822,
117.351986908061));
#231541=CARTESIAN_POINT('Ctrl Pts',(4.73187730740598,-6.33981975083672,
117.351682172163));
#231542=CARTESIAN_POINT('Ctrl Pts',(4.71404106577142,-6.35310593126007,
117.350777837566));
#231543=CARTESIAN_POINT('Ctrl Pts',(4.70219903592498,-6.36187569558878,
117.350177023742));
#231544=CARTESIAN_POINT('Ctrl Pts',(4.58750552195451,-6.44631824317775,
117.344353539543));
#231545=CARTESIAN_POINT('Ctrl Pts',(4.4828751043067,-6.51951333781007,117.338997906481));
#231546=CARTESIAN_POINT('Ctrl Pts',(3.77788377971231,-6.98769751229932,
117.302592190623));
#231547=CARTESIAN_POINT('Ctrl Pts',(3.12788074321745,-7.30183359653573,
117.268182605252));
#231548=CARTESIAN_POINT('Ctrl Pts',(2.06047679600729,-7.6486135496008,117.217945719112));
#231549=CARTESIAN_POINT('Ctrl Pts',(1.6675675797021,-7.74378044474482,117.200585561463));
#231550=CARTESIAN_POINT('Ctrl Pts',(1.24807344246182,-7.81195789220473,
117.183383375346));
#231551=CARTESIAN_POINT('Ctrl Pts',(1.2270647875249,-7.81528537189074,117.182525210302));
#231552=CARTESIAN_POINT('Ctrl Pts',(1.1967009664676,-7.81996912681385,117.181289691594));
#231553=CARTESIAN_POINT('Ctrl Pts',(1.18735647995318,-7.82139341407987,
117.180910113993));
#231554=CARTESIAN_POINT('Ctrl Pts',(1.17107986425141,-7.82384445522013,
117.180250085218));
#231555=CARTESIAN_POINT('Ctrl Pts',(1.16414889214334,-7.82487875082973,
117.179969387414));
#231556=CARTESIAN_POINT('Ctrl Pts',(1.15078112595938,-7.82685544265866,
117.179428694516));
#231557=CARTESIAN_POINT('Ctrl Pts',(1.14434452809189,-7.82779911095196,
117.17916865798));
#231558=CARTESIAN_POINT('Ctrl Pts',(1.12912078655872,-7.83001188208366,
117.178554349693));
#231559=CARTESIAN_POINT('Ctrl Pts',(1.12033264672264,-7.83127413551633,
117.178200302552));
#231560=CARTESIAN_POINT('Ctrl Pts',(1.08965398358835,-7.83562785913713,
117.17696634175));
#231561=CARTESIAN_POINT('Ctrl Pts',(1.06775254546759,-7.83864237371611,
117.176088951324));
#231562=CARTESIAN_POINT('Ctrl Pts',(0.805858833662692,-7.87357144223106,
117.165639040871));
#231563=CARTESIAN_POINT('Ctrl Pts',(0.564526587492866,-7.89454608600728,
117.156434420372));
#231564=CARTESIAN_POINT('Ctrl Pts',(0.145341007530778,-7.9116540109927,
117.141033286342));
#231565=CARTESIAN_POINT('Ctrl Pts',(-0.0321131525079635,-7.91292396362523,
117.134693378899));
#231566=CARTESIAN_POINT('Ctrl Pts',(-0.643731356682046,-7.89672401144403,
117.113266199803));
#231567=CARTESIAN_POINT('Ctrl Pts',(-1.07631913203097,-7.84947012280132,
117.098889930226));
#231568=CARTESIAN_POINT('Ctrl Pts',(-1.79285545265694,-7.71082703231405,
117.074231231002));
#231569=CARTESIAN_POINT('Ctrl Pts',(-2.07949576055718,-7.6385119413124,
117.064115062868));
#231570=CARTESIAN_POINT('Ctrl Pts',(-2.50146469555151,-7.50653921648612,
117.048041704247));
#231571=CARTESIAN_POINT('Ctrl Pts',(-2.64027226680974,-7.45884809696728,
117.042554986074));
#231572=CARTESIAN_POINT('Ctrl Pts',(-2.83502650192841,-7.38581739387184,
117.034471799829));
#231573=CARTESIAN_POINT('Ctrl Pts',(-2.89213340522334,-7.3636429723869,
117.032053752685));
#231574=CARTESIAN_POINT('Ctrl Pts',(-2.95735547313544,-7.3374417313818,
117.02923101093));
#231575=CARTESIAN_POINT('Ctrl Pts',(-2.96572959458317,-7.33406098463771,
117.028867425563));
#231576=CARTESIAN_POINT('Ctrl Pts',(-2.97837683812393,-7.32892991734553,
117.028316528112));
#231577=CARTESIAN_POINT('Ctrl Pts',(-2.98265427175697,-7.32719017210704,
117.028129900035));
#231578=CARTESIAN_POINT('Ctrl Pts',(-2.99003802969178,-7.32417946568983,
117.027807203405));
#231579=CARTESIAN_POINT('Ctrl Pts',(-2.99314507737281,-7.32291026917352,
117.027671249974));
#231580=CARTESIAN_POINT('Ctrl Pts',(-2.99956967780685,-7.32028111507021,
117.027389790423));
#231581=CARTESIAN_POINT('Ctrl Pts',(-3.00288711481493,-7.3189208788771,
117.027244266028));
#231582=CARTESIAN_POINT('Ctrl Pts',(-3.01192748369076,-7.31520690924474,
117.026847179475));
#231583=CARTESIAN_POINT('Ctrl Pts',(-3.01764854630388,-7.31284872961152,
117.026595322878));
#231584=CARTESIAN_POINT('Ctrl Pts',(-3.03959018839673,-7.30377441472172,
117.025627235336));
#231585=CARTESIAN_POINT('Ctrl Pts',(-3.05579105679746,-7.29701104711736,
117.024907910446));
#231586=CARTESIAN_POINT('Ctrl Pts',(-3.32972063923137,-7.18158157554029,
117.012670490454));
#231587=CARTESIAN_POINT('Ctrl Pts',(-3.58150902964062,-7.05938510572658,
117.000303881305));
#231588=CARTESIAN_POINT('Ctrl Pts',(-4.39139741732715,-6.61184077083736,
116.958142560529));
#231589=CARTESIAN_POINT('Ctrl Pts',(-4.91618635689275,-6.23153857999667,
116.927118721136));
#231590=CARTESIAN_POINT('Ctrl Pts',(-5.64869545453544,-5.54995726483783,
116.882521687796));
#231591=CARTESIAN_POINT('Ctrl Pts',(-5.89189262578322,-5.29107112524182,
116.867376604445));
#231592=CARTESIAN_POINT('Ctrl Pts',(-6.12934645588315,-5.00154151460192,
116.852257870871));
#231593=CARTESIAN_POINT('Ctrl Pts',(-6.1417247765091,-4.98633355040616,
116.851468613838));
#231594=CARTESIAN_POINT('Ctrl Pts',(-6.15964961833961,-4.96414313748657,
116.850324022488));
#231595=CARTESIAN_POINT('Ctrl Pts',(-6.16524102892711,-4.95719714820035,
116.849966742657));
#231596=CARTESIAN_POINT('Ctrl Pts',(-6.17500898340934,-4.94502071333443,
116.849342164551));
#231597=CARTESIAN_POINT('Ctrl Pts',(-6.17919064944181,-4.93979440044247,
116.849074645101));
#231598=CARTESIAN_POINT('Ctrl Pts',(-6.18727890687082,-4.92965922622586,
116.848556935472));
#231599=CARTESIAN_POINT('Ctrl Pts',(-6.19118630045289,-4.92475101415718,
116.848306710809));
#231600=CARTESIAN_POINT('Ctrl Pts',(-6.20047101662896,-4.91305964735328,
116.847711836219));
#231601=CARTESIAN_POINT('Ctrl Pts',(-6.20584305880946,-4.90627229743856,
116.847367413248));
#231602=CARTESIAN_POINT('Ctrl Pts',(-6.22485761261875,-4.88216701172168,
116.846147471742));
#231603=CARTESIAN_POINT('Ctrl Pts',(-6.23843892300201,-4.86480080193035,
116.845274573557));
#231604=CARTESIAN_POINT('Ctrl Pts',(-6.41907148236379,-4.63182839979569,
116.833643578032));
#231605=CARTESIAN_POINT('Ctrl Pts',(-6.57494330844314,-4.40777163193627,
116.82337100424));
#231606=CARTESIAN_POINT('Ctrl Pts',(-7.03711628433842,-3.66417917277177,
116.791608251754));
#231607=CARTESIAN_POINT('Ctrl Pts',(-7.29572840442103,-3.11761675966364,
116.771846710286));
#231608=CARTESIAN_POINT('Ctrl Pts',(-7.54888038781228,-2.37318918425704,
116.744651907063));
#231609=CARTESIAN_POINT('Ctrl Pts',(-7.60191489861735,-2.19738645611294,
116.738193583418));
#231610=CARTESIAN_POINT('Ctrl Pts',(-7.69456579927984,-1.84654485218379,
116.724958823021));
#231611=CARTESIAN_POINT('Ctrl Pts',(-7.73443734509595,-1.67168832178477,
116.718196782917));
#231612=CARTESIAN_POINT('Ctrl Pts',(-7.7732525378035,-1.47008277402918,
116.710052860398));
#231613=CARTESIAN_POINT('Ctrl Pts',(-7.77804688671567,-1.44450164271278,
116.709013138756));
#231614=CARTESIAN_POINT('Ctrl Pts',(-7.78399089626607,-1.41189848776171,
116.707679380905));
#231615=CARTESIAN_POINT('Ctrl Pts',(-7.785257449136,-1.4048978834481,116.707392491511));
#231616=CARTESIAN_POINT('Ctrl Pts',(-7.78728089775761,-1.3936269329508,
116.706929802121));
#231617=CARTESIAN_POINT('Ctrl Pts',(-7.78804373070418,-1.38935764197675,
116.706754357048));
#231618=CARTESIAN_POINT('Ctrl Pts',(-7.78948829260269,-1.38123439617448,
116.706420187271));
#231619=CARTESIAN_POINT('Ctrl Pts',(-7.79017067329978,-1.37738055689878,
116.706261501239));
#231620=CARTESIAN_POINT('Ctrl Pts',(-7.79171732410764,-1.3686077176383,
116.705899933774));
#231621=CARTESIAN_POINT('Ctrl Pts',(-7.7925797957553,-1.36368840655859,
116.705696946694));
#231622=CARTESIAN_POINT('Ctrl Pts',(-7.79479823308611,-1.3509641966725,
116.705171287491));
#231623=CARTESIAN_POINT('Ctrl Pts',(-7.79614713170791,-1.34315809012247,
116.704848204382));
#231624=CARTESIAN_POINT('Ctrl Pts',(-7.80414132568621,-1.29647774260131,
116.702912646225));
#231625=CARTESIAN_POINT('Ctrl Pts',(-7.81050746845904,-1.25755689700789,
116.701284206284));
#231626=CARTESIAN_POINT('Ctrl Pts',(-7.83736072539268,-1.08530818055408,
116.694017681966));
#231627=CARTESIAN_POINT('Ctrl Pts',(-7.85472588874391,-0.951522278462937,
116.688216164074));
#231628=CARTESIAN_POINT('Ctrl Pts',(-7.89686769496231,-0.545828745646157,
116.670279010351));
#231629=CARTESIAN_POINT('Ctrl Pts',(-7.91099797524739,-0.273027730968651,
116.657756563083));
#231630=CARTESIAN_POINT('Ctrl Pts',(-7.91100408729714,0.551041996280015,
116.619499028887));
#231631=CARTESIAN_POINT('Ctrl Pts',(-7.85342008312486,1.10069144869308,
116.593514735652));
#231632=CARTESIAN_POINT('Ctrl Pts',(-7.66828776789497,1.97438093723589,
116.55388855431));
#231633=CARTESIAN_POINT('Ctrl Pts',(-7.57580094590423,2.30393055830503,
116.539315625526));
#231634=CARTESIAN_POINT('Ctrl Pts',(-7.45403472262007,2.64988726639005,
116.524436848088));
#231635=CARTESIAN_POINT('Ctrl Pts',(-7.44569009647523,2.67324431589141,
116.52343429898));
#231636=CARTESIAN_POINT('Ctrl Pts',(-7.43397644084802,2.70555109095403,
116.522050281538));
#231637=CARTESIAN_POINT('Ctrl Pts',(-7.430700866726,2.71453440922827,116.521665725253));
#231638=CARTESIAN_POINT('Ctrl Pts',(-7.42504364712464,2.72996246208796,
116.521005773071));
#231639=CARTESIAN_POINT('Ctrl Pts',(-7.42266988142133,2.73641006391288,
116.520730116758));
#231640=CARTESIAN_POINT('Ctrl Pts',(-7.41776515605248,2.7496788947595,116.520163130622));
#231641=CARTESIAN_POINT('Ctrl Pts',(-7.41523317934636,2.75649974259466,
116.519871834794));
#231642=CARTESIAN_POINT('Ctrl Pts',(-7.40933846995057,2.77231250037182,
116.519196900343));
#231643=CARTESIAN_POINT('Ctrl Pts',(-7.40596876883543,2.78130180992139,
116.518813492929));
#231644=CARTESIAN_POINT('Ctrl Pts',(-7.39526430162284,2.80970059510629,
116.517603124158));
#231645=CARTESIAN_POINT('Ctrl Pts',(-7.38786950617857,2.82908743113183,
116.516778152512));
#231646=CARTESIAN_POINT('Ctrl Pts',(-7.27096223413252,3.13199734876724,
116.503908168259));
#231647=CARTESIAN_POINT('Ctrl Pts',(-7.14527194433361,3.40901883395341,
116.492423735195));
#231648=CARTESIAN_POINT('Ctrl Pts',(-6.65157175957509,4.34912683230948,
116.453714151767));
#231649=CARTESIAN_POINT('Ctrl Pts',(-6.20465549154878,4.96592284120455,
116.429108283361));
#231650=CARTESIAN_POINT('Ctrl Pts',(-5.53303647572045,5.65792324817929,
116.393563996317));
#231651=CARTESIAN_POINT('Ctrl Pts',(-5.38345208318239,5.80043333589012,
116.385663185485));
#231652=CARTESIAN_POINT('Ctrl Pts',(-5.21366624438295,5.94995740033911,
116.376635657692));
#231653=CARTESIAN_POINT('Ctrl Pts',(-5.19883960965301,5.9629166922425,116.375847253632));
#231654=CARTESIAN_POINT('Ctrl Pts',(-5.17722312525201,5.98166877761607,
116.374697857564));
#231655=CARTESIAN_POINT('Ctrl Pts',(-5.17047155105633,5.98750570711496,
116.374338869533));
#231656=CARTESIAN_POINT('Ctrl Pts',(-5.15854834532258,5.99777845466058,
116.37370493254));
#231657=CARTESIAN_POINT('Ctrl Pts',(-5.15338082673286,6.0022190460331,116.373430194714));
#231658=CARTESIAN_POINT('Ctrl Pts',(-5.14269500475926,6.01137769565537,
116.372862100054));
#231659=CARTESIAN_POINT('Ctrl Pts',(-5.13717593098592,6.01609484346085,
116.37256870429));
#231660=CARTESIAN_POINT('Ctrl Pts',(-5.12304901319749,6.02813549426118,
116.37181776975));
#231661=CARTESIAN_POINT('Ctrl Pts',(-5.11443196842435,6.03544814970255,
116.371359773613));
#231662=CARTESIAN_POINT('Ctrl Pts',(-5.07932765454066,6.06510944796254,
116.369494278859));
#231663=CARTESIAN_POINT('Ctrl Pts',(-5.05270951696767,6.08730223801123,
116.368080446881));
#231664=CARTESIAN_POINT('Ctrl Pts',(-4.68633612855896,6.38870621274969,
116.348637543071));
#231665=CARTESIAN_POINT('Ctrl Pts',(-4.32402926779007,6.63928189438814,
116.329666587344));
#231666=CARTESIAN_POINT('Ctrl Pts',(-3.30519487839172,7.22499118250048,
116.279100202995));
#231667=CARTESIAN_POINT('Ctrl Pts',(-2.61955682074068,7.50085520269922,
116.248171834691));
#231668=CARTESIAN_POINT('Ctrl Pts',(-1.89627838422932,7.68037391716766,
116.217541625687));
#231669=CARTESIAN_POINT('Ctrl Pts',(-1.88685333038075,7.68269482198705,
116.217142757027));
#231670=CARTESIAN_POINT('Ctrl Pts',(-1.87487060133419,7.6856221698276,116.216635999221));
#231671=CARTESIAN_POINT('Ctrl Pts',(-1.87231686649916,7.68624469168908,
116.216528020317));
#231672=CARTESIAN_POINT('Ctrl Pts',(-1.84801861994013,7.69215502737025,
116.215500817408));
#231673=CARTESIAN_POINT('Ctrl Pts',(-1.82625205199896,7.69735183224469,
116.214582115104));
#231674=CARTESIAN_POINT('Ctrl Pts',(-1.62966687413072,7.74340607890182,
116.206298408681));
#231675=CARTESIAN_POINT('Ctrl Pts',(-1.45352483222994,7.77839436669596,
116.198974218713));
#231676=CARTESIAN_POINT('Ctrl Pts',(-1.23645257876753,7.81388122531212,
116.190075664475));
#231677=CARTESIAN_POINT('Ctrl Pts',(-1.19651251468582,7.82009671333895,
116.188443559855));
#231678=CARTESIAN_POINT('Ctrl Pts',(-1.13351802968146,7.82940603269124,
116.185877446158));
#231679=CARTESIAN_POINT('Ctrl Pts',(-1.11049468977524,7.83270473696248,
116.184941274263));
#231680=CARTESIAN_POINT('Ctrl Pts',(-1.06773950438045,7.83863825048239,
116.183205887279));
#231681=CARTESIAN_POINT('Ctrl Pts',(-1.04801162450513,7.84130020523693,
116.182406383934));
#231682=CARTESIAN_POINT('Ctrl Pts',(-1.00434710887154,7.84702429035397,
116.180639504024));
#231683=CARTESIAN_POINT('Ctrl Pts',(-0.980406068816571,7.8500514185209,
116.179672520702));
#231684=CARTESIAN_POINT('Ctrl Pts',(-0.911203864228038,7.85847989353954,
116.176882516298));
#231685=CARTESIAN_POINT('Ctrl Pts',(-0.865909271209853,7.86359967732496,
116.175062670449));
#231686=CARTESIAN_POINT('Ctrl Pts',(-0.51051986847832,7.90066255561776,
116.16083119563));
#231687=CARTESIAN_POINT('Ctrl Pts',(-0.198821857089528,7.9146432303336,
116.148644461999));
#231688=CARTESIAN_POINT('Ctrl Pts',(0.605481302614832,7.90316424123078,
116.117528490128));
#231689=CARTESIAN_POINT('Ctrl Pts',(1.0963210825232,7.8501381644512,116.098896770273));
#231690=CARTESIAN_POINT('Ctrl Pts',(1.67993384796268,7.73125791559428,116.075496097349));
#231691=CARTESIAN_POINT('Ctrl Pts',(1.78043303949063,7.70873428241009,116.071417821523));
#231692=CARTESIAN_POINT('Ctrl Pts',(1.90038524812652,7.67938002748687,116.066471526625));
#231693=CARTESIAN_POINT('Ctrl Pts',(1.92028907071842,7.67442711736106,116.065648149467));
#231694=CARTESIAN_POINT('Ctrl Pts',(1.95151933237095,7.66652660995701,116.064351957554));
#231695=CARTESIAN_POINT('Ctrl Pts',(1.96285874595188,7.66363122208441,116.063880448144));
#231696=CARTESIAN_POINT('Ctrl Pts',(1.98297704826265,7.65844666592033,116.063042373965));
#231697=CARTESIAN_POINT('Ctrl Pts',(1.99175851255851,7.65616753577282,116.06267604507));
#231698=CARTESIAN_POINT('Ctrl Pts',(2.01199766409598,7.65087751461665,116.061830569766));
#231699=CARTESIAN_POINT('Ctrl Pts',(2.02345253884151,7.64785598491124,116.061351181139));
#231700=CARTESIAN_POINT('Ctrl Pts',(2.05539752532561,7.63935284597185,116.060011892445));
#231701=CARTESIAN_POINT('Ctrl Pts',(2.07587239655663,7.63381455627029,116.059150745043));
#231702=CARTESIAN_POINT('Ctrl Pts',(2.19427285377355,7.6012766056243,116.054155593316));
#231703=CARTESIAN_POINT('Ctrl Pts',(2.29169226216281,7.57247551490085,116.049984701333));
#231704=CARTESIAN_POINT('Ctrl Pts',(3.07537074969939,7.32428054813343,116.016010232481));
#231705=CARTESIAN_POINT('Ctrl Pts',(3.72929909166269,7.01394285862001,115.985323118855));
#231706=CARTESIAN_POINT('Ctrl Pts',(4.4340344111253,6.5527153421695,115.950840748322));
#231707=CARTESIAN_POINT('Ctrl Pts',(4.53433946016617,6.48371080111128,115.94588661242));
#231708=CARTESIAN_POINT('Ctrl Pts',(4.66554275193139,6.38891558801009,115.939337404855));
#231709=CARTESIAN_POINT('Ctrl Pts',(4.69789316259605,6.36516546634541,115.937716828595));
#231710=CARTESIAN_POINT('Ctrl Pts',(4.74901718379636,6.32703058558189,115.935146199785));
#231711=CARTESIAN_POINT('Ctrl Pts',(4.76790935285062,6.31280608366394,115.934194150021));
#231712=CARTESIAN_POINT('Ctrl Pts',(4.8040634292249,6.28532967600904,115.932368031252));
#231713=CARTESIAN_POINT('Ctrl Pts',(4.82133499118411,6.27209083751342,115.931493808739));
#231714=CARTESIAN_POINT('Ctrl Pts',(4.8619262619239,6.24071045094472,115.929434747549));
#231715=CARTESIAN_POINT('Ctrl Pts',(4.88519942403692,6.22250918069546,115.928250662501));
#231716=CARTESIAN_POINT('Ctrl Pts',(4.95335885297179,6.16858556519661,115.924772106377));
#231717=CARTESIAN_POINT('Ctrl Pts',(4.99795928003246,6.1325047809436,115.922482054546));
#231718=CARTESIAN_POINT('Ctrl Pts',(5.29105529554038,5.89007497406277,115.9073332087));
#231719=CARTESIAN_POINT('Ctrl Pts',(5.52711392368034,5.66915070942462,115.894610970461));
#231720=CARTESIAN_POINT('Ctrl Pts',(6.04561773586974,5.1206313754462,115.865284889384));
#231721=CARTESIAN_POINT('Ctrl Pts',(6.31604723636686,4.78308756775227,115.848975329558));
#231722=CARTESIAN_POINT('Ctrl Pts',(6.80110145347412,4.0642909548411,115.816679950595));
#231723=CARTESIAN_POINT('Ctrl Pts',(7.01440397740474,3.68395865398956,115.800747199353));
#231724=CARTESIAN_POINT('Ctrl Pts',(7.24604930290235,3.17703979059333,115.779398427923));
#231725=CARTESIAN_POINT('Ctrl Pts',(7.29419230869431,3.06489305539442,115.774664457431));
#231726=CARTESIAN_POINT('Ctrl Pts',(7.35465435202675,2.91454667321587,115.76825671222));
#231727=CARTESIAN_POINT('Ctrl Pts',(7.36930569792999,2.87730019509821,115.766664326652));
#231728=CARTESIAN_POINT('Ctrl Pts',(7.38786235728985,2.82905407115898,115.764593601695));
#231729=CARTESIAN_POINT('Ctrl Pts',(7.39202698827084,2.81815438731001,115.764125256874));
#231730=CARTESIAN_POINT('Ctrl Pts',(7.39860856941201,2.80081408869812,115.763379272603));
#231731=CARTESIAN_POINT('Ctrl Pts',(7.40104126787672,2.79437944339012,115.763102256927));
#231732=CARTESIAN_POINT('Ctrl Pts',(7.40538965800088,2.78283215846149,115.762604775946));
#231733=CARTESIAN_POINT('Ctrl Pts',(7.40730845767646,2.77772068819915,115.762384435846));
#231734=CARTESIAN_POINT('Ctrl Pts',(7.41177149021943,2.76579415269531,115.761870013816));
#231735=CARTESIAN_POINT('Ctrl Pts',(7.41431161497342,2.75897756314154,115.76157576481));
#231736=CARTESIAN_POINT('Ctrl Pts',(7.42152727769009,2.73953193447622,115.76073567853));
#231737=CARTESIAN_POINT('Ctrl Pts',(7.42617996176327,2.72689448384872,115.760188895453));
#231738=CARTESIAN_POINT('Ctrl Pts',(7.45540179618182,2.64689374860291,115.756721986674));
#231739=CARTESIAN_POINT('Ctrl Pts',(7.47908620445817,2.57921149367012,115.753763979841));
#231740=CARTESIAN_POINT('Ctrl Pts',(7.54245218844816,2.38991601454081,115.745401233506));
#231741=CARTESIAN_POINT('Ctrl Pts',(7.5801074716033,2.26765333164216,115.739902186985));
#231742=CARTESIAN_POINT('Ctrl Pts',(7.73439086533888,1.71982677533538,115.714975137089));
#231743=CARTESIAN_POINT('Ctrl Pts',(7.81825523334347,1.28587061474553,115.694500122485));
#231744=CARTESIAN_POINT('Ctrl Pts',(7.93617808370223,0.191071703140395,
115.643818837889));
#231745=CARTESIAN_POINT('Ctrl Pts',(7.92448362114155,-0.471424432176066,
115.614208221002));
#231746=CARTESIAN_POINT('Ctrl Pts',(7.82468018388264,-1.16621094109064,
115.585532600301));
#231747=CARTESIAN_POINT('Ctrl Pts',(7.81840945810377,-1.20753532105886,
115.583834959094));
#231748=CARTESIAN_POINT('Ctrl Pts',(7.80968069518058,-1.26213732931399,
115.581602119156));
#231749=CARTESIAN_POINT('Ctrl Pts',(7.80751580608146,-1.27546075547408,
115.581058093484));
#231750=CARTESIAN_POINT('Ctrl Pts',(7.80410213840577,-1.2961351811532,115.580215155254));
#231751=CARTESIAN_POINT('Ctrl Pts',(7.80287705393131,-1.30349003682376,
115.579915527765));
#231752=CARTESIAN_POINT('Ctrl Pts',(7.80040367636901,-1.3182106424387,115.579316316699));
#231753=CARTESIAN_POINT('Ctrl Pts',(7.79915534389789,-1.32557637813875,
115.579016734656));
#231754=CARTESIAN_POINT('Ctrl Pts',(7.79637675627202,-1.34183152337952,
115.578356136219));
#231755=CARTESIAN_POINT('Ctrl Pts',(7.79484172660835,-1.35072011188928,
115.577995264611));
#231756=CARTESIAN_POINT('Ctrl Pts',(7.79036153311696,-1.37640067812506,
115.576953666647));
#231757=CARTESIAN_POINT('Ctrl Pts',(7.78737727918901,-1.39318583090562,
115.576274123805));
#231758=CARTESIAN_POINT('Ctrl Pts',(7.7805302828666,-1.43098781887351,115.574746517097));
#231759=CARTESIAN_POINT('Ctrl Pts',(7.77663659196238,-1.45199894821325,
115.573899393291));
#231760=CARTESIAN_POINT('Ctrl Pts',(7.69822988312715,-1.8657334624993,115.557256207842));
#231761=CARTESIAN_POINT('Ctrl Pts',(7.59414053067719,-2.25228252782829,
115.542415552671));
#231762=CARTESIAN_POINT('Ctrl Pts',(7.31079790781519,-3.05632339119236,
115.511997211471));
#231763=CARTESIAN_POINT('Ctrl Pts',(7.12395142877413,-3.46961022634724,
115.496641631285));
#231764=CARTESIAN_POINT('Ctrl Pts',(6.69339881047408,-4.23863840243437,
115.465933509126));
#231765=CARTESIAN_POINT('Ctrl Pts',(6.45397361302279,-4.5949765053536,115.450649427798));
#231766=CARTESIAN_POINT('Ctrl Pts',(6.17009874320876,-4.95121489076884,
115.432577596861));
#231767=CARTESIAN_POINT('Ctrl Pts',(6.15319497420201,-4.97220665071132,
115.431501705299));
#231768=CARTESIAN_POINT('Ctrl Pts',(6.13049376049492,-5.00010485333914,
115.430057593258));
#231769=CARTESIAN_POINT('Ctrl Pts',(6.12479115658163,-5.00708853318127,
115.429694893127));
#231770=CARTESIAN_POINT('Ctrl Pts',(6.11587393287609,-5.01797096157041,
115.429127856254));
#231771=CARTESIAN_POINT('Ctrl Pts',(6.11266748315087,-5.0218764196521,115.428923985847));
#231772=CARTESIAN_POINT('Ctrl Pts',(6.10624008707155,-5.02968971655229,
115.428515376684));
#231773=CARTESIAN_POINT('Ctrl Pts',(6.10301912585457,-5.03359754003327,
115.4283106371));
#231774=CARTESIAN_POINT('Ctrl Pts',(6.09575118258457,-5.04239812363682,
115.427848717581));
#231775=CARTESIAN_POINT('Ctrl Pts',(6.09170206060011,-5.04728910622151,
115.427591418237));
#231776=CARTESIAN_POINT('Ctrl Pts',(6.0797430800045,-5.06169914748906,115.426831638858));
#231777=CARTESIAN_POINT('Ctrl Pts',(6.07181678906869,-5.0712044975632,115.426328254952));
#231778=CARTESIAN_POINT('Ctrl Pts',(6.01035696262352,-5.14455756669678,
115.422426782989));
#231779=CARTESIAN_POINT('Ctrl Pts',(5.95584122856075,-5.20757313703596,
115.418976270473));
#231780=CARTESIAN_POINT('Ctrl Pts',(5.75987758249643,-5.42698777974775,
115.406643068526));
#231781=CARTESIAN_POINT('Ctrl Pts',(5.61318586084218,-5.57857727366622,
115.397538209988));
#231782=CARTESIAN_POINT('Ctrl Pts',(5.02384194107628,-6.14079180232958,
115.361963182065));
#231783=CARTESIAN_POINT('Ctrl Pts',(4.54075735063141,-6.50614616445817,
115.335064517024));
#231784=CARTESIAN_POINT('Ctrl Pts',(3.81219784840903,-6.93611923707059,
115.299364313218));
#231785=CARTESIAN_POINT('Ctrl Pts',(3.59802625861965,-7.04959700554827,
115.289356587062));
#231786=CARTESIAN_POINT('Ctrl Pts',(3.34874178334811,-7.16735429477087,
115.278200890594));
#231787=CARTESIAN_POINT('Ctrl Pts',(3.3184167396995,-7.18144480453668,115.276851763404));
#231788=CARTESIAN_POINT('Ctrl Pts',(3.27313711282507,-7.20213590449756,
115.274848782527));
#231789=CARTESIAN_POINT('Ctrl Pts',(3.25825004737886,-7.20888304644383,
115.274192074306));
#231790=CARTESIAN_POINT('Ctrl Pts',(3.23187625813565,-7.22073783491047,
115.273031843864));
#231791=CARTESIAN_POINT('Ctrl Pts',(3.22039808343036,-7.22586432295078,
115.272527962703));
#231792=CARTESIAN_POINT('Ctrl Pts',(3.19631413314722,-7.23655213441936,
115.271472899743));
#231793=CARTESIAN_POINT('Ctrl Pts',(3.18370594656166,-7.24210793064462,
115.270921823337));
#231794=CARTESIAN_POINT('Ctrl Pts',(3.15124059877901,-7.25631261698167,
115.269506021122));
#231795=CARTESIAN_POINT('Ctrl Pts',(3.13136228680717,-7.26491296166915,
115.268642194305));
#231796=CARTESIAN_POINT('Ctrl Pts',(3.05112354510443,-7.299237714403,115.265167355863));
#231797=CARTESIAN_POINT('Ctrl Pts',(2.99047875962188,-7.32429266539306,
115.26256811104));
#231798=CARTESIAN_POINT('Ctrl Pts',(2.61111738579847,-7.47552576778342,
115.246472167339));
#231799=CARTESIAN_POINT('Ctrl Pts',(2.28478438932175,-7.5816354859581,115.233361119966));
#231800=CARTESIAN_POINT('Ctrl Pts',(1.25156839153174,-7.84479454699652,
115.193426027796));
#231801=CARTESIAN_POINT('Ctrl Pts',(0.529441153454571,-7.92633254788837,
115.16797477931));
#231802=CARTESIAN_POINT('Ctrl Pts',(-0.268644741614546,-7.90679345215649,
115.136730508297));
#231803=CARTESIAN_POINT('Ctrl Pts',(-0.343635540229735,-7.90388935155108,
115.133761118866));
#231804=CARTESIAN_POINT('Ctrl Pts',(-0.431377775716765,-7.89924038487294,
115.130238355869));
#231805=CARTESIAN_POINT('Ctrl Pts',(-0.444181646725833,-7.89853075614155,
115.129723083334));
#231806=CARTESIAN_POINT('Ctrl Pts',(-0.464659020671794,-7.89734588975695,
115.128897003468));
#231807=CARTESIAN_POINT('Ctrl Pts',(-0.472333683808938,-7.89689059051496,
115.128586949863));
#231808=CARTESIAN_POINT('Ctrl Pts',(-0.485910869848464,-7.89606526083035,
115.128037626513));
#231809=CARTESIAN_POINT('Ctrl Pts',(-0.491813671303911,-7.89569979730756,
115.127798532412));
#231810=CARTESIAN_POINT('Ctrl Pts',(-0.504049436572287,-7.89492846305252,
115.127302350654));
#231811=CARTESIAN_POINT('Ctrl Pts',(-0.510382331353193,-7.89452159074639,
115.127045224189));
#231812=CARTESIAN_POINT('Ctrl Pts',(-0.526660673205268,-7.89345607963703,
115.126383469426));
#231813=CARTESIAN_POINT('Ctrl Pts',(-0.53660535924529,-7.89278626551327,
115.125978400691));
#231814=CARTESIAN_POINT('Ctrl Pts',(-0.577681147846379,-7.88994165806629,
115.124301941963));
#231815=CARTESIAN_POINT('Ctrl Pts',(-0.608800231849868,-7.8876014804734,
115.123023898075));
#231816=CARTESIAN_POINT('Ctrl Pts',(-0.806611886662481,-7.87154830411064,
115.114845593408));
#231817=CARTESIAN_POINT('Ctrl Pts',(-0.972822283090363,-7.85273838432535,
115.10770321241));
#231818=CARTESIAN_POINT('Ctrl Pts',(-1.53342911841054,-7.77122529965061,
115.082855369394));
#231819=CARTESIAN_POINT('Ctrl Pts',(-1.9236259172581,-7.68394359205734,
115.064367310476));
#231820=CARTESIAN_POINT('Ctrl Pts',(-2.48644572906544,-7.51247424939248,
115.037296477165));
#231821=CARTESIAN_POINT('Ctrl Pts',(-2.66531074734442,-7.45089276487872,
115.028625332138));
#231822=CARTESIAN_POINT('Ctrl Pts',(-3.10707470391562,-7.28085190283259,
115.007202796167));
#231823=CARTESIAN_POINT('Ctrl Pts',(-3.36666689719746,-7.16451609057546,
114.994615008494));
#231824=CARTESIAN_POINT('Ctrl Pts',(-3.78775697637102,-6.9478518277163,
114.974392549006));
#231825=CARTESIAN_POINT('Ctrl Pts',(-3.95290901590641,-6.85523631441762,
114.966512262409));
#231826=CARTESIAN_POINT('Ctrl Pts',(-4.13260102551079,-6.74581163034636,
114.957997317052));
#231827=CARTESIAN_POINT('Ctrl Pts',(-4.1505701404222,-6.73477047172949,
114.957146473416));
#231828=CARTESIAN_POINT('Ctrl Pts',(-4.17570032534715,-6.71919040250287,
114.955957432969));
#231829=CARTESIAN_POINT('Ctrl Pts',(-4.18289849710914,-6.71471168671104,
114.955616951716));
#231830=CARTESIAN_POINT('Ctrl Pts',(-4.19606622369326,-6.7064893123318,
114.954994288249));
#231831=CARTESIAN_POINT('Ctrl Pts',(-4.20203799873123,-6.70274923502462,
114.954711969922));
#231832=CARTESIAN_POINT('Ctrl Pts',(-4.21348485984275,-6.69555884275751,
114.954170946286));
#231833=CARTESIAN_POINT('Ctrl Pts',(-4.21896072303947,-6.69210977933483,
114.953912193484));
#231834=CARTESIAN_POINT('Ctrl Pts',(-4.23266503850478,-6.68345438264078,
114.953264762467));
#231835=CARTESIAN_POINT('Ctrl Pts',(-4.24088813305018,-6.67823956270512,
114.952876409895));
#231836=CARTESIAN_POINT('Ctrl Pts',(-4.26845541248025,-6.66068583825584,
114.951574916135));
#231837=CARTESIAN_POINT('Ctrl Pts',(-4.28775562699343,-6.64827790779195,
114.950664432149));
#231838=CARTESIAN_POINT('Ctrl Pts',(-4.33333962483289,-6.61869130680911,
114.948515608679));
#231839=CARTESIAN_POINT('Ctrl Pts',(-4.35957573720787,-6.60143971724083,
114.947280105852));
#231840=CARTESIAN_POINT('Ctrl Pts',(-4.4514990035468,-6.54020844609792,
114.942955340218));
#231841=CARTESIAN_POINT('Ctrl Pts',(-4.51662993087941,-6.49540025134938,
114.939898483332));
#231842=CARTESIAN_POINT('Ctrl Pts',(-4.75263610153431,-6.32776826274899,
114.928840264551));
#231843=CARTESIAN_POINT('Ctrl Pts',(-4.91926806430558,-6.19911366247368,
114.9210716483));
#231844=CARTESIAN_POINT('Ctrl Pts',(-5.62990843038554,-5.60371659717378,
114.887794713049));
#231845=CARTESIAN_POINT('Ctrl Pts',(-6.11409611074967,-5.07101836013405,
114.865051970489));
#231846=CARTESIAN_POINT('Ctrl Pts',(-6.56508929603143,-4.41473451404926,
114.837176956544));
#231847=CARTESIAN_POINT('Ctrl Pts',(-6.60924966540691,-4.34834413795392,
114.834354473511));
#231848=CARTESIAN_POINT('Ctrl Pts',(-6.66676497367065,-4.25897529064251,
114.830537115142));
#231849=CARTESIAN_POINT('Ctrl Pts',(-6.68101918163342,-4.23657980178738,
114.829579016298));
#231850=CARTESIAN_POINT('Ctrl Pts',(-6.80519630601589,-4.03929374743746,
114.821122362088));
#231851=CARTESIAN_POINT('Ctrl Pts',(-6.90833533183499,-3.86024372311409,
114.813333872112));
#231852=CARTESIAN_POINT('Ctrl Pts',(-7.01059455247853,-3.66546939655364,
114.804533461345));
#231853=CARTESIAN_POINT('Ctrl Pts',(-7.01681583177302,-3.65354587420396,
114.803993446183));
#231854=CARTESIAN_POINT('Ctrl Pts',(-7.02532525838795,-3.63713505176211,
114.803248370268));
#231855=CARTESIAN_POINT('Ctrl Pts',(-7.02763960207304,-3.63266128259242,
114.803045067803));
#231856=CARTESIAN_POINT('Ctrl Pts',(-7.03158701590246,-3.62501279771316,
114.802697172362));
#231857=CARTESIAN_POINT('Ctrl Pts',(-7.03322221503302,-3.62183917639508,
114.802552723377));
#231858=CARTESIAN_POINT('Ctrl Pts',(-7.03639337664261,-3.61567428787935,
114.802271938727));
#231859=CARTESIAN_POINT('Ctrl Pts',(-7.03792958139306,-3.612683146107,114.80213561962));
#231860=CARTESIAN_POINT('Ctrl Pts',(-7.04159169017628,-3.60554145938853,
114.801809937061));
#231861=CARTESIAN_POINT('Ctrl Pts',(-7.04371581839078,-3.60139003944941,
114.801620453943));
#231862=CARTESIAN_POINT('Ctrl Pts',(-7.05013163271111,-3.58882351104592,
114.801046375671));
#231863=CARTESIAN_POINT('Ctrl Pts',(-7.05441188517672,-3.58040265678223,
114.800661003337));
#231864=CARTESIAN_POINT('Ctrl Pts',(-7.09488796807132,-3.50041674956804,
114.796994230623));
#231865=CARTESIAN_POINT('Ctrl Pts',(-7.13000746507062,-3.42831523567537,
114.793641160497));
#231866=CARTESIAN_POINT('Ctrl Pts',(-7.2732033674255,-3.12260841572409,
114.779269377551));
#231867=CARTESIAN_POINT('Ctrl Pts',(-7.37093551387112,-2.88434765136892,
114.767696025035));
#231868=CARTESIAN_POINT('Ctrl Pts',(-7.75725811981538,-1.79388099260181,
114.714525136329));
#231869=CARTESIAN_POINT('Ctrl Pts',(-7.91091024119016,-0.900670596073987,
114.671494346077));
#231870=CARTESIAN_POINT('Ctrl Pts',(-7.91099996068087,-0.00078873785590905,
114.634517834504));
#231871=CARTESIAN_POINT('',(-7.9109991388093,-0.00369130851947151,110.642331508237));
#231872=CARTESIAN_POINT('Ctrl Pts',(-7.91099996199236,-0.000775472076273572,
114.634517289408));
#231873=CARTESIAN_POINT('Ctrl Pts',(-7.91100579301261,0.0587098433008668,
114.632073016955));
#231874=CARTESIAN_POINT('Ctrl Pts',(-7.91034069134381,0.118194551747119,
114.629651328104));
#231875=CARTESIAN_POINT('Ctrl Pts',(-7.90873371509585,0.189730367056336,
114.626765571885));
#231876=CARTESIAN_POINT('Ctrl Pts',(-7.90843513499218,0.201792730061897,
114.626279883153));
#231877=CARTESIAN_POINT('Ctrl Pts',(-7.90789406828848,0.221800803016074,
114.625475757813));
#231878=CARTESIAN_POINT('Ctrl Pts',(-7.90766720070255,0.229746893208682,
114.625156795512));
#231879=CARTESIAN_POINT('Ctrl Pts',(-7.90723782622641,0.244031087484476,
114.624584117389));
#231880=CARTESIAN_POINT('Ctrl Pts',(-7.90703967495095,0.250369309574613,
114.624330255095));
#231881=CARTESIAN_POINT('Ctrl Pts',(-7.90662188692477,0.26323758628399,
114.623815348885));
#231882=CARTESIAN_POINT('Ctrl Pts',(-7.90640178086051,0.269767621334624,
114.623554320976));
#231883=CARTESIAN_POINT('Ctrl Pts',(-7.90591094537004,0.2838127436196,114.622993451409));
#231884=CARTESIAN_POINT('Ctrl Pts',(-7.90563758973299,0.291327736056126,
114.622693698393));
#231885=CARTESIAN_POINT('Ctrl Pts',(-7.90486880189324,0.311664679003659,
114.621883444601));
#231886=CARTESIAN_POINT('Ctrl Pts',(-7.90435288791472,0.324485859066189,
114.62137363334));
#231887=CARTESIAN_POINT('Ctrl Pts',(-7.90190864088364,0.381759868535767,
114.619100680168));
#231888=CARTESIAN_POINT('Ctrl Pts',(-7.89963647416791,0.42619764157554,
114.617349112525));
#231889=CARTESIAN_POINT('Ctrl Pts',(-7.89468230275719,0.509329481031571,
114.614094014422));
#231890=CARTESIAN_POINT('Ctrl Pts',(-7.89209041820312,0.54802743451356,
114.612587550955));
#231891=CARTESIAN_POINT('Ctrl Pts',(-7.81733217323739,1.55327480754709,
114.573674500102));
#231892=CARTESIAN_POINT('Ctrl Pts',(-7.56849444604616,2.49814016768892,
114.543782118253));
#231893=CARTESIAN_POINT('Ctrl Pts',(-7.10941212781202,3.47155414636616,
114.504878466237));
#231894=CARTESIAN_POINT('Ctrl Pts',(-7.06168512508699,3.56763658370474,
114.500926450934));
#231895=CARTESIAN_POINT('Ctrl Pts',(-6.98097845923512,3.72214401841444,
114.494340019431));
#231896=CARTESIAN_POINT('Ctrl Pts',(-6.94918270954362,3.7811738352896,114.491767443643));
#231897=CARTESIAN_POINT('Ctrl Pts',(-6.89136646568287,3.88531862618823,
114.487115164482));
#231898=CARTESIAN_POINT('Ctrl Pts',(-6.86564328632307,3.93059468982792,
114.485053796574));
#231899=CARTESIAN_POINT('Ctrl Pts',(-6.83508019006939,3.98317414802832,
114.482610273899));
#231900=CARTESIAN_POINT('Ctrl Pts',(-6.83067229322775,3.9907284445824,114.482257994627));
#231901=CARTESIAN_POINT('Ctrl Pts',(-6.82387818863219,4.00232801319199,
114.481715229317));
#231902=CARTESIAN_POINT('Ctrl Pts',(-6.8215008676627,4.00637853563081,114.481525351874));
#231903=CARTESIAN_POINT('Ctrl Pts',(-6.81733971998819,4.01345393323815,
114.481193074807));
#231904=CARTESIAN_POINT('Ctrl Pts',(-6.81555748141575,4.01647974592083,
114.481050783049));
#231905=CARTESIAN_POINT('Ctrl Pts',(-6.81181828103429,4.02281835415367,
114.480752301782));
#231906=CARTESIAN_POINT('Ctrl Pts',(-6.80986091639393,4.02613090989576,
114.480596085081));
#231907=CARTESIAN_POINT('Ctrl Pts',(-6.80503103664114,4.0342911821173,114.480210689479));
#231908=CARTESIAN_POINT('Ctrl Pts',(-6.80215576108304,4.0391372535984,114.479981325427));
#231909=CARTESIAN_POINT('Ctrl Pts',(-6.79090572551468,4.05805230379196,
114.479084166217));
#231910=CARTESIAN_POINT('Ctrl Pts',(-6.78249252699713,4.07209825359602,
114.478413817637));
#231911=CARTESIAN_POINT('Ctrl Pts',(-6.63298928719216,4.31994727149369,
114.466513280177));
#231912=CARTESIAN_POINT('Ctrl Pts',(-6.4799417815432,4.5462973459964,114.454515669699));
#231913=CARTESIAN_POINT('Ctrl Pts',(-5.87335454313425,5.35039084591772,
114.408882386469));
#231914=CARTESIAN_POINT('Ctrl Pts',(-5.3517385198692,5.87214573423439,114.373516066576));
#231915=CARTESIAN_POINT('Ctrl Pts',(-4.59652138720038,6.44210921363292,
114.331716605015));
#231916=CARTESIAN_POINT('Ctrl Pts',(-4.42240137194119,6.5628618071467,114.322586989178));
#231917=CARTESIAN_POINT('Ctrl Pts',(-4.17581324947497,6.71959543969107,
114.310353468899));
#231918=CARTESIAN_POINT('Ctrl Pts',(-4.10733697760519,6.76166862729888,
114.307026582574));
#231919=CARTESIAN_POINT('Ctrl Pts',(-4.01060801158991,6.81908910515552,
114.302423249038));
#231920=CARTESIAN_POINT('Ctrl Pts',(-3.98288606977512,6.83531794679929,
114.30111483139));
#231921=CARTESIAN_POINT('Ctrl Pts',(-3.93491757888023,6.86300851502499,
114.298869329601));
#231922=CARTESIAN_POINT('Ctrl Pts',(-3.91471800823017,6.87455054225053,
114.297929357534));
#231923=CARTESIAN_POINT('Ctrl Pts',(-3.88557154431861,6.89103469951997,
114.296581040933));
#231924=CARTESIAN_POINT('Ctrl Pts',(-3.87666562177488,6.89604880449441,
114.296170121529));
#231925=CARTESIAN_POINT('Ctrl Pts',(-3.86185654992293,6.90434867531953,
114.295488597606));
#231926=CARTESIAN_POINT('Ctrl Pts',(-3.85595887604933,6.90764415622845,
114.295217646786));
#231927=CARTESIAN_POINT('Ctrl Pts',(-3.84363773274675,6.91450822364827,
114.294652555092));
#231928=CARTESIAN_POINT('Ctrl Pts',(-3.83721349720302,6.91807542404162,
114.294358463703));
#231929=CARTESIAN_POINT('Ctrl Pts',(-3.82307638848506,6.92589961938682,
114.293712487471));
#231930=CARTESIAN_POINT('Ctrl Pts',(-3.81536135049653,6.93015269498555,
114.293360741866));
#231931=CARTESIAN_POINT('Ctrl Pts',(-3.78929796087774,6.94446396720245,
114.292175083953));
#231932=CARTESIAN_POINT('Ctrl Pts',(-3.77091674154496,6.9544622915754,114.29134328938));
#231933=CARTESIAN_POINT('Ctrl Pts',(-3.601009096742,7.04601057820812,114.283694589688));
#231934=CARTESIAN_POINT('Ctrl Pts',(-3.44689474323059,7.12267172868053,
114.277051155367));
#231935=CARTESIAN_POINT('Ctrl Pts',(-2.96804520552956,7.34168068513377,
114.257193781941));
#231936=CARTESIAN_POINT('Ctrl Pts',(-2.63613776309559,7.46728644781195,
114.244518838581));
#231937=CARTESIAN_POINT('Ctrl Pts',(-2.09530135947347,7.63138400505904,
114.224743324583));
#231938=CARTESIAN_POINT('Ctrl Pts',(-1.89132700684193,7.68447736819271,
114.21746962895));
#231939=CARTESIAN_POINT('Ctrl Pts',(-1.62476059199439,7.74260523093262,
114.208006019346));
#231940=CARTESIAN_POINT('Ctrl Pts',(-1.56389071776369,7.75512917519444,
114.205847639701));
#231941=CARTESIAN_POINT('Ctrl Pts',(-1.31352031196943,7.80357513776435,
114.196962878063));
#231942=CARTESIAN_POINT('Ctrl Pts',(-1.12288841265363,7.83327764592251,
114.190182831868));
#231943=CARTESIAN_POINT('Ctrl Pts',(-0.687675239913562,7.88487438375678,
114.174356538105));
#231944=CARTESIAN_POINT('Ctrl Pts',(-0.442777007086627,7.90241052361514,
114.165183665185));
#231945=CARTESIAN_POINT('Ctrl Pts',(-0.155869012230444,7.90957368998094,
114.153849163629));
#231946=CARTESIAN_POINT('Ctrl Pts',(-0.114280351862891,7.91028387781438,
114.152193782938));
#231947=CARTESIAN_POINT('Ctrl Pts',(-0.0605925824389661,7.91077719715592,
114.150042179127));
#231948=CARTESIAN_POINT('Ctrl Pts',(-0.0484964426018806,7.91086059903049,
114.149556452277));
#231949=CARTESIAN_POINT('Ctrl Pts',(-0.028962908378574,7.91095047793766,
114.148770564981));
#231950=CARTESIAN_POINT('Ctrl Pts',(-0.0215255885499998,7.91097421074427,
114.148470988327));
#231951=CARTESIAN_POINT('Ctrl Pts',(-0.00733222728977448,7.91099948695315,
114.147898614442));
#231952=CARTESIAN_POINT('Ctrl Pts',(-0.00057619281659804,7.91100286384868,
114.147625878188));
#231953=CARTESIAN_POINT('Ctrl Pts',(0.0148661919916847,7.91099080073623,
114.147001835228));
#231954=CARTESIAN_POINT('Ctrl Pts',(0.0235525222599233,7.91096970864169,
114.146650345047));
#231955=CARTESIAN_POINT('Ctrl Pts',(0.0495855861933373,7.91086361823253,
114.145595552935));
#231956=CARTESIAN_POINT('Ctrl Pts',(0.0669320404917187,7.91073587055013,
114.144890895756));
#231957=CARTESIAN_POINT('Ctrl Pts',(0.194657404993967,7.90937510308107,
114.139689462875));
#231958=CARTESIAN_POINT('Ctrl Pts',(0.304997985822899,7.90588901972775,
114.13512522899));
#231959=CARTESIAN_POINT('Ctrl Pts',(1.09639089180065,7.86429362762633,114.102004080089));
#231960=CARTESIAN_POINT('Ctrl Pts',(1.77007917957722,7.74054731432652,114.072103532186));
#231961=CARTESIAN_POINT('Ctrl Pts',(2.83006584447053,7.40003837323588,114.025016898902));
#231962=CARTESIAN_POINT('Ctrl Pts',(3.22912425618619,7.23481935467894,114.007178696705));
#231963=CARTESIAN_POINT('Ctrl Pts',(3.78239419646353,6.95081176089013,113.981649947119));
#231964=CARTESIAN_POINT('Ctrl Pts',(3.94885073586882,6.85761399384283,113.973866711315));
#231965=CARTESIAN_POINT('Ctrl Pts',(4.14594900292095,6.73770195786656,113.964534479781));
#231966=CARTESIAN_POINT('Ctrl Pts',(4.17996152825557,6.71665411127056,113.962919657506));
#231967=CARTESIAN_POINT('Ctrl Pts',(4.23321824147934,6.68313624250312,113.960384163536));
#231968=CARTESIAN_POINT('Ctrl Pts',(4.2525702571977,6.67083899726109,113.959461363264));
#231969=CARTESIAN_POINT('Ctrl Pts',(4.28864117034431,6.64769697164591,113.957738537487));
#231970=CARTESIAN_POINT('Ctrl Pts',(4.30537307481393,6.63687281813398,113.956938256227));
#231971=CARTESIAN_POINT('Ctrl Pts',(4.34202380469651,6.61296591453171,113.955182752732));
#231972=CARTESIAN_POINT('Ctrl Pts',(4.36192478765904,6.59985613923829,113.954227892123));
#231973=CARTESIAN_POINT('Ctrl Pts',(4.41196168130757,6.56656914924889,113.951822881017));
#231974=CARTESIAN_POINT('Ctrl Pts',(4.44201869468206,6.54627422289323,113.950374319441));
#231975=CARTESIAN_POINT('Ctrl Pts',(4.57838253454433,6.45282778709755,113.943784143384));
#231976=CARTESIAN_POINT('Ctrl Pts',(4.68303016132383,6.37728800460461,113.938676077267));
#231977=CARTESIAN_POINT('Ctrl Pts',(4.80702283426289,6.28308554109769,113.932551686855));
#231978=CARTESIAN_POINT('Ctrl Pts',(4.82817976111648,6.26684231858872,113.93150406539));
#231979=CARTESIAN_POINT('Ctrl Pts',(4.96923849630088,6.15740619421311,113.92450108791));
#231980=CARTESIAN_POINT('Ctrl Pts',(5.08651863851926,6.06088370682491,113.918590781271));
#231981=CARTESIAN_POINT('Ctrl Pts',(5.46944203580366,5.72678704840285,113.898915528615));
#231982=CARTESIAN_POINT('Ctrl Pts',(5.72179992401643,5.47465892143718,113.885327865333));
#231983=CARTESIAN_POINT('Ctrl Pts',(6.07000405933151,5.07629995589437,113.864890759587));
#231984=CARTESIAN_POINT('Ctrl Pts',(6.17941382012483,4.94253107216828,113.858177721761));
#231985=CARTESIAN_POINT('Ctrl Pts',(6.3348634033076,4.739234244161,113.848083508332));
#231986=CARTESIAN_POINT('Ctrl Pts',(6.38432734639594,4.67238692080265,113.844780672652));
#231987=CARTESIAN_POINT('Ctrl Pts',(6.44349862771441,4.58972644649087,113.840705371846));
#231988=CARTESIAN_POINT('Ctrl Pts',(6.45421670093369,4.5746420835081,113.839962020496));
#231989=CARTESIAN_POINT('Ctrl Pts',(6.47133139950275,4.55037538488,113.838766659207));
#231990=CARTESIAN_POINT('Ctrl Pts',(6.47776159667329,4.5412168987171,113.838315637896));
#231991=CARTESIAN_POINT('Ctrl Pts',(6.48999081757093,4.52372007798592,113.83745423802));
#231992=CARTESIAN_POINT('Ctrl Pts',(6.49579326097076,4.51538415487991,113.837043954804));
#231993=CARTESIAN_POINT('Ctrl Pts',(6.50901879890834,4.49630579227316,113.836105214814));
#231994=CARTESIAN_POINT('Ctrl Pts',(6.51643137622854,4.48555611040658,113.83557647929));
#231995=CARTESIAN_POINT('Ctrl Pts',(6.53911203131193,4.45248986350638,113.833950744053));
#231996=CARTESIAN_POINT('Ctrl Pts',(6.5542922866093,4.43011340171523,113.832851512073));
#231997=CARTESIAN_POINT('Ctrl Pts',(6.75070031431382,4.13737878876414,113.818485516664));
#231998=CARTESIAN_POINT('Ctrl Pts',(6.91518644639465,3.8561697374287,113.804855829073));
#231999=CARTESIAN_POINT('Ctrl Pts',(7.21748503516139,3.25745604314694,113.776689335002));
#232000=CARTESIAN_POINT('Ctrl Pts',(7.35275217020087,2.93941361845353,113.762181398554));
#232001=CARTESIAN_POINT('Ctrl Pts',(7.52026980655846,2.46082240106188,113.741162802782));
#232002=CARTESIAN_POINT('Ctrl Pts',(7.56903033656544,2.30648778501472,113.734500536522));
#232003=CARTESIAN_POINT('Ctrl Pts',(7.64225117447324,2.04730926579286,113.723496288921));
#232004=CARTESIAN_POINT('Ctrl Pts',(7.6693668485218,1.94326806808357,113.719127008371));
#232005=CARTESIAN_POINT('Ctrl Pts',(7.70314522095087,1.80191714298028,113.713250661925));
#232006=CARTESIAN_POINT('Ctrl Pts',(7.7116725865063,1.7650658969837,113.711724083907));
#232007=CARTESIAN_POINT('Ctrl Pts',(7.72548792944276,1.70335061883701,113.709176208486));
#232008=CARTESIAN_POINT('Ctrl Pts',(7.73092093279273,1.67851976889971,113.708153429652));
#232009=CARTESIAN_POINT('Ctrl Pts',(7.74137010793287,1.6296360119952,113.706144383823));
#232010=CARTESIAN_POINT('Ctrl Pts',(7.74639408238674,1.60558506606705,113.705158048417));
#232011=CARTESIAN_POINT('Ctrl Pts',(7.75803435389844,1.54853373846273,113.702823213518));
#232012=CARTESIAN_POINT('Ctrl Pts',(7.76455226704611,1.51551373425353,113.70147570528));
#232013=CARTESIAN_POINT('Ctrl Pts',(7.78552595448471,1.40557192378669,113.697001212718));
#232014=CARTESIAN_POINT('Ctrl Pts',(7.79905095799791,1.32847698549921,113.693883241214));
#232015=CARTESIAN_POINT('Ctrl Pts',(7.82919408090104,1.14028798327482,113.686313235545));
#232016=CARTESIAN_POINT('Ctrl Pts',(7.84459450253147,1.02901602708435,113.681871853586));
#232017=CARTESIAN_POINT('Ctrl Pts',(7.8869454455207,0.666297187546621,113.667474118777));
#232018=CARTESIAN_POINT('Ctrl Pts',(7.90421231435547,0.413875400263871,
113.657590547339));
#232019=CARTESIAN_POINT('Ctrl Pts',(7.91979847995507,-0.35155158898817,
113.628087938584));
#232020=CARTESIAN_POINT('Ctrl Pts',(7.88037992427006,-0.863957579144894,
113.609069262493));
#232021=CARTESIAN_POINT('Ctrl Pts',(7.72354327689219,-1.75662499191642,
113.575415831525));
#232022=CARTESIAN_POINT('Ctrl Pts',(7.6265963301856,-2.13865495738272,113.560798380348));
#232023=CARTESIAN_POINT('Ctrl Pts',(7.48686749932487,-2.55595355440418,
113.543432472595));
#232024=CARTESIAN_POINT('Ctrl Pts',(7.47171377836206,-2.59991858269763,
113.541584504388));
#232025=CARTESIAN_POINT('Ctrl Pts',(7.45224156219398,-2.65483617775734,
113.539250503246));
#232026=CARTESIAN_POINT('Ctrl Pts',(7.44828490189104,-2.66591662481712,
113.538778267818));
#232027=CARTESIAN_POINT('Ctrl Pts',(7.44196836605903,-2.68348196585731,
113.538027510647));
#232028=CARTESIAN_POINT('Ctrl Pts',(7.43962469023442,-2.68997269327859,
113.537749626476));
#232029=CARTESIAN_POINT('Ctrl Pts',(7.43520624940313,-2.70215946577246,
113.537226993314));
#232030=CARTESIAN_POINT('Ctrl Pts',(7.43313342314835,-2.70785621166325,
113.536982322144));
#232031=CARTESIAN_POINT('Ctrl Pts',(7.42847473227035,-2.72061402950442,
113.536433555154));
#232032=CARTESIAN_POINT('Ctrl Pts',(7.42588534587853,-2.72767380287272,
113.536129316073));
#232033=CARTESIAN_POINT('Ctrl Pts',(7.41930857286423,-2.74552612063222,
113.5353585125));
#232034=CARTESIAN_POINT('Ctrl Pts',(7.41530770804152,-2.75631365625485,
113.534891388578));
#232035=CARTESIAN_POINT('Ctrl Pts',(7.39350705716242,-2.81470375604336,
113.532355451843));
#232036=CARTESIAN_POINT('Ctrl Pts',(7.37527268616106,-2.8621419372535,113.530268074772));
#232037=CARTESIAN_POINT('Ctrl Pts',(7.06207546961965,-3.65407877049914,
113.494917796717));
#232038=CARTESIAN_POINT('Ctrl Pts',(6.65623160066468,-4.34967469766674,
113.45644601264));
#232039=CARTESIAN_POINT('Ctrl Pts',(5.97030351323842,-5.19844402966377,
113.407170975701));
#232040=CARTESIAN_POINT('Ctrl Pts',(5.77535354513684,-5.41420866481935,
113.394344478153));
#232041=CARTESIAN_POINT('Ctrl Pts',(5.44712486492886,-5.73952770551166,
113.374651660728));
#232042=CARTESIAN_POINT('Ctrl Pts',(5.32138803970804,-5.85629418175103,
113.367499111816));
#232043=CARTESIAN_POINT('Ctrl Pts',(5.17489428439722,-5.98371966829777,
113.359591597057));
#232044=CARTESIAN_POINT('Ctrl Pts',(5.15777616691329,-5.99848121994882,
113.358673907399));
#232045=CARTESIAN_POINT('Ctrl Pts',(5.12703394914865,-6.02476241733021,
113.35703705698));
#232046=CARTESIAN_POINT('Ctrl Pts',(5.11343373696757,-6.03630969416128,
113.356316813134));
#232047=CARTESIAN_POINT('Ctrl Pts',(5.0927654891225,-6.05373811887285,113.355228113205));
#232048=CARTESIAN_POINT('Ctrl Pts',(5.08572611306931,-6.05965307939724,
113.354858337285));
#232049=CARTESIAN_POINT('Ctrl Pts',(5.07347880131543,-6.06990772643741,
113.354216761166));
#232050=CARTESIAN_POINT('Ctrl Pts',(5.068275577176,-6.07425300995367,113.35394474324));
#232051=CARTESIAN_POINT('Ctrl Pts',(5.05753096490723,-6.08320256485267,
113.353384166553));
#232052=CARTESIAN_POINT('Ctrl Pts',(5.05198885911748,-6.08780596550942,
113.35309564171));
#232053=CARTESIAN_POINT('Ctrl Pts',(5.03860339487771,-6.09889337415696,
113.35240028448));
#232054=CARTESIAN_POINT('Ctrl Pts',(5.03075378928449,-6.10536983914922,
113.351993744307));
#232055=CARTESIAN_POINT('Ctrl Pts',(5.00653612553713,-6.12527266351154,
113.350743274616));
#232056=CARTESIAN_POINT('Ctrl Pts',(4.99012659490277,-6.13864852830099,
113.349901293058));
#232057=CARTESIAN_POINT('Ctrl Pts',(4.79600797862402,-6.29558727980826,
113.340003036966));
#232058=CARTESIAN_POINT('Ctrl Pts',(4.6122078953207,-6.43145859270225,113.331246159529));
#232059=CARTESIAN_POINT('Ctrl Pts',(4.00092727158216,-6.84363698581708,
113.303803107243));
#232060=CARTESIAN_POINT('Ctrl Pts',(3.55260747045815,-7.08673381874128,
113.286252489727));
#232061=CARTESIAN_POINT('Ctrl Pts',(2.76546831356759,-7.41995871267594,
113.256727579886));
#232062=CARTESIAN_POINT('Ctrl Pts',(2.43839833890373,-7.53377705021515,
113.244770397935));
#232063=CARTESIAN_POINT('Ctrl Pts',(1.99246000084619,-7.65686890110851,
113.227864562993));
#232064=CARTESIAN_POINT('Ctrl Pts',(1.87930374257606,-7.68542478218803,
113.223523303817));
#232065=CARTESIAN_POINT('Ctrl Pts',(1.65573706542054,-7.7366109670845,113.214783950523));
#232066=CARTESIAN_POINT('Ctrl Pts',(1.54539125460966,-7.75940593302801,
113.210391989784));
#232067=CARTESIAN_POINT('Ctrl Pts',(1.4219204773644,-7.78217381090321,113.205365827969));
#232068=CARTESIAN_POINT('Ctrl Pts',(1.40924180057216,-7.78447972645805,
113.204848499986));
#232069=CARTESIAN_POINT('Ctrl Pts',(1.39020422224186,-7.78789412385165,
113.204069947982));
#232070=CARTESIAN_POINT('Ctrl Pts',(1.38384946323937,-7.78902582654478,
113.203809772315));
#232071=CARTESIAN_POINT('Ctrl Pts',(1.37292371749809,-7.79095777169169,
113.203361954382));
#232072=CARTESIAN_POINT('Ctrl Pts',(1.3683533913763,-7.79176177321571,113.203174479009));
#232073=CARTESIAN_POINT('Ctrl Pts',(1.35894567521188,-7.79340822502756,
113.202788269167));
#232074=CARTESIAN_POINT('Ctrl Pts',(1.35410820455498,-7.79425019359295,
113.202589513716));
#232075=CARTESIAN_POINT('Ctrl Pts',(1.34246884811117,-7.79626487703156,
113.202110898841));
#232076=CARTESIAN_POINT('Ctrl Pts',(1.33566621359169,-7.79743319345547,
113.20183084932));
#232077=CARTESIAN_POINT('Ctrl Pts',(1.31083141469081,-7.80166498553403,
113.200807299654));
#232078=CARTESIAN_POINT('Ctrl Pts',(1.29279025653177,-7.80467480995383,
113.20006152277));
#232079=CARTESIAN_POINT('Ctrl Pts',(1.26045590306844,-7.80995399213806,
113.198721115593));
#232080=CARTESIAN_POINT('Ctrl Pts',(1.2461665678263,-7.81224675265937,113.198127434967));
#232081=CARTESIAN_POINT('Ctrl Pts',(1.21194253084613,-7.81764180033606,
113.196702487885));
#232082=CARTESIAN_POINT('Ctrl Pts',(1.19200214780665,-7.82070705796359,
113.19586978872));
#232083=CARTESIAN_POINT('Ctrl Pts',(1.14785007464116,-7.82732138117898,
113.194020886138));
#232084=CARTESIAN_POINT('Ctrl Pts',(1.12363324185207,-7.8308344459447,113.193003374296));
#232085=CARTESIAN_POINT('Ctrl Pts',(1.09246134556991,-7.83520888751034,
113.191689564798));
#232086=CARTESIAN_POINT('Ctrl Pts',(1.08552074697029,-7.836173480087,113.19139677846));
#232087=CARTESIAN_POINT('Ctrl Pts',(0.623368918795017,-7.8997767734597,
113.171884217319));
#232088=CARTESIAN_POINT('Ctrl Pts',(0.163577765085867,-7.92264390551656,
113.151450610919));
#232089=CARTESIAN_POINT('Ctrl Pts',(-0.898434728084774,-7.88293565769442,
113.104720070733));
#232090=CARTESIAN_POINT('Ctrl Pts',(-1.4967817999997,-7.79151050136518,
113.078861926769));
#232091=CARTESIAN_POINT('Ctrl Pts',(-2.11315342300981,-7.62363166501894,
113.053003877987));
#232092=CARTESIAN_POINT('Ctrl Pts',(-2.14728713903963,-7.61408793751334,
113.05157365325));
#232093=CARTESIAN_POINT('Ctrl Pts',(-2.19739786157058,-7.59971329487891,
113.049476175118));
#232094=CARTESIAN_POINT('Ctrl Pts',(-2.21342541982846,-7.59506072653445,
113.048805642436));
#232095=CARTESIAN_POINT('Ctrl Pts',(-2.24172040840283,-7.58674992854055,
113.047622417813));
#232096=CARTESIAN_POINT('Ctrl Pts',(-2.25399389143973,-7.58311258034037,
113.047109348872));
#232097=CARTESIAN_POINT('Ctrl Pts',(-2.27796830204144,-7.57594421789799,
113.046107463507));
#232098=CARTESIAN_POINT('Ctrl Pts',(-2.28966998029559,-7.57241584701241,
113.045618601314));
#232099=CARTESIAN_POINT('Ctrl Pts',(-2.32120563157643,-7.56282721783734,
113.044301498395));
#232100=CARTESIAN_POINT('Ctrl Pts',(-2.34102405948631,-7.55671605052908,
113.043474161789));
#232101=CARTESIAN_POINT('Ctrl Pts',(-2.41274696555027,-7.53429049698047,
113.04048120297));
#232102=CARTESIAN_POINT('Ctrl Pts',(-2.46450733505366,-7.51751853335709,
113.038323353573));
#232103=CARTESIAN_POINT('Ctrl Pts',(-2.63161917342696,-7.46145765772914,
113.031361970042));
#232104=CARTESIAN_POINT('Ctrl Pts',(-2.74623821627457,-7.42003681844865,
113.026596196436));
#232105=CARTESIAN_POINT('Ctrl Pts',(-3.50596448740633,-7.12547164732345,
112.995030906438));
#232106=CARTESIAN_POINT('Ctrl Pts',(-4.11633637035354,-6.79116331465217,
112.97009834102));
#232107=CARTESIAN_POINT('Ctrl Pts',(-4.87228790323076,-6.23733444900761,
112.935328497478));
#232108=CARTESIAN_POINT('Ctrl Pts',(-5.06244668973513,-6.08400816683078,
112.926157016051));
#232109=CARTESIAN_POINT('Ctrl Pts',(-5.31653554654547,-5.85896326461784,
112.912949759176));
#232110=CARTESIAN_POINT('Ctrl Pts',(-5.38671863427287,-5.7945027620374,
112.909192719125));
#232111=CARTESIAN_POINT('Ctrl Pts',(-5.46596082754466,-5.71903779309484,
112.90480524425));
#232112=CARTESIAN_POINT('Ctrl Pts',(-5.47617691671409,-5.70925629313809,
112.904236760569));
#232113=CARTESIAN_POINT('Ctrl Pts',(-5.49159668429594,-5.69441301241333,
112.903374324352));
#232114=CARTESIAN_POINT('Ctrl Pts',(-5.49681974719299,-5.689371350627,112.903081429476));
#232115=CARTESIAN_POINT('Ctrl Pts',(-5.50619738609891,-5.68029443683308,
112.902554165535));
#232116=CARTESIAN_POINT('Ctrl Pts',(-5.51035448844059,-5.67626179411214,
112.902319936223));
#232117=CARTESIAN_POINT('Ctrl Pts',(-5.51865199128004,-5.66819500515379,
112.901851424256));
#232118=CARTESIAN_POINT('Ctrl Pts',(-5.52279240573574,-5.66416087873738,
112.901617142688));
#232119=CARTESIAN_POINT('Ctrl Pts',(-5.53431224342692,-5.65291212554321,
112.900963909187));
#232120=CARTESIAN_POINT('Ctrl Pts',(-5.54168196012169,-5.64568760722472,
112.900544411812));
#232121=CARTESIAN_POINT('Ctrl Pts',(-5.57105765272962,-5.6167777371395,
112.898865822621));
#232122=CARTESIAN_POINT('Ctrl Pts',(-5.59295045321362,-5.59497816870379,
112.897600269055));
#232123=CARTESIAN_POINT('Ctrl Pts',(-5.95483986629369,-5.23038330241046,
112.876427902634));
#232124=CARTESIAN_POINT('Ctrl Pts',(-6.26280943483639,-4.85737050485626,
112.854380724581));
#232125=CARTESIAN_POINT('Ctrl Pts',(-6.76209061921953,-4.12561112994304,
112.813612699308));
#232126=CARTESIAN_POINT('Ctrl Pts',(-6.96358060813342,-3.77559485417696,
112.795024123401));
#232127=CARTESIAN_POINT('Ctrl Pts',(-7.24248234946587,-3.19211813449322,
112.766406024907));
#232128=CARTESIAN_POINT('Ctrl Pts',(-7.33726930677978,-2.96777042969169,
112.755910608214));
#232129=CARTESIAN_POINT('Ctrl Pts',(-7.45853864341839,-2.63922769003488,
112.741315591248));
#232130=CARTESIAN_POINT('Ctrl Pts',(-7.49348088077412,-2.538319718117,112.736933747415));
#232131=CARTESIAN_POINT('Ctrl Pts',(-7.53144841134671,-2.42104886094696,
112.731955751157));
#232132=CARTESIAN_POINT('Ctrl Pts',(-7.536477120866,-2.40534932410206,112.73129166691));
#232133=CARTESIAN_POINT('Ctrl Pts',(-7.54402950109423,-2.38151473439015,
112.730287005249));
#232134=CARTESIAN_POINT('Ctrl Pts',(-7.54658915234622,-2.37339118347494,
112.729945207109));
#232135=CARTESIAN_POINT('Ctrl Pts',(-7.55117534686139,-2.35875357345477,
112.729330445335));
#232136=CARTESIAN_POINT('Ctrl Pts',(-7.55320659083397,-2.352241002922,112.72905732236));
#232137=CARTESIAN_POINT('Ctrl Pts',(-7.55755256641395,-2.33824327032506,
112.728471139));
#232138=CARTESIAN_POINT('Ctrl Pts',(-7.55986460862298,-2.33075727717245,
112.728158170108));
#232139=CARTESIAN_POINT('Ctrl Pts',(-7.5660831471851,-2.31051612502935,
112.72731335008));
#232140=CARTESIAN_POINT('Ctrl Pts',(-7.5699685163275,-2.29775447301757,
112.72678221624));
#232141=CARTESIAN_POINT('Ctrl Pts',(-7.5871089106869,-2.24094079504664,
112.724424333573));
#232142=CARTESIAN_POINT('Ctrl Pts',(-7.60001194797521,-2.1967830467125,
112.722609536252));
#232143=CARTESIAN_POINT('Ctrl Pts',(-7.79914576292799,-1.49253143542186,
112.693943712674));
#232144=CARTESIAN_POINT('Ctrl Pts',(-7.89914780911132,-0.811104103549981,
112.670432777604));
#232145=CARTESIAN_POINT('Ctrl Pts',(-7.91070713680184,-0.0811266043454294,
112.645890246744));
#232146=CARTESIAN_POINT('Ctrl Pts',(-7.91103662902964,-0.0369916938798452,
112.644407443864));
#232147=CARTESIAN_POINT('Ctrl Pts',(-7.91052058691599,0.534480418306826,
112.625201902882));
#232148=CARTESIAN_POINT('Ctrl Pts',(-7.85731819019845,1.06039377385093,
112.607529184521));
#232149=CARTESIAN_POINT('Ctrl Pts',(-7.73864859412972,1.64373732978102,
112.584496245443));
#232150=CARTESIAN_POINT('Ctrl Pts',(-7.72421915107394,1.7102609329705,112.581817198238));
#232151=CARTESIAN_POINT('Ctrl Pts',(-7.70665313769354,1.78648300389155,
112.578679037429));
#232152=CARTESIAN_POINT('Ctrl Pts',(-7.70435375008926,1.79637340202614,
112.578270505813));
#232153=CARTESIAN_POINT('Ctrl Pts',(-7.70094117000557,1.81092491873939,
112.577667447668));
#232154=CARTESIAN_POINT('Ctrl Pts',(-7.6998427657516,1.81558953172193,112.577473830222));
#232155=CARTESIAN_POINT('Ctrl Pts',(-7.69787999262547,1.82389105855173,
112.577128710674));
#232156=CARTESIAN_POINT('Ctrl Pts',(-7.69701728212897,1.82752836717775,
112.576977311413));
#232157=CARTESIAN_POINT('Ctrl Pts',(-7.69521172663924,1.83511688544628,
112.576661057798));
#232158=CARTESIAN_POINT('Ctrl Pts',(-7.69426841608465,1.83906798193346,
112.576496174422));
#232159=CARTESIAN_POINT('Ctrl Pts',(-7.69179523779342,1.84939178429493,
112.57606477155));
#232160=CARTESIAN_POINT('Ctrl Pts',(-7.69026050025146,1.85576329022109,
112.575797945626));
#232161=CARTESIAN_POINT('Ctrl Pts',(-7.68341105032408,1.88404456345179,
112.574611038228));
#232162=CARTESIAN_POINT('Ctrl Pts',(-7.67801065730547,1.90593326498587,
112.573685631838));
#232163=CARTESIAN_POINT('Ctrl Pts',(-7.63785730026498,2.06574111364481,
112.566881422263));
#232164=CARTESIAN_POINT('Ctrl Pts',(-7.59948583546931,2.20271673573322,
112.560788600797));
#232165=CARTESIAN_POINT('Ctrl Pts',(-7.50078270262243,2.52169021405716,
112.546119576812));
#232166=CARTESIAN_POINT('Ctrl Pts',(-7.43748560225496,2.70267715976454,
112.537422201172));
#232167=CARTESIAN_POINT('Ctrl Pts',(-7.16885069260496,3.38962428088298,
112.50344593749));
#232168=CARTESIAN_POINT('Ctrl Pts',(-6.91789734176502,3.87617714141812,
112.477449769005));
#232169=CARTESIAN_POINT('Ctrl Pts',(-6.40795510046922,4.65513353462324,
112.435601828651));
#232170=CARTESIAN_POINT('Ctrl Pts',(-6.17382596418324,4.96146035562347,
112.419040055832));
#232171=CARTESIAN_POINT('Ctrl Pts',(-5.9013024602782,5.26870055621896,112.40240956427));
#232172=CARTESIAN_POINT('Ctrl Pts',(-5.88422300577274,5.28776851937222,
112.40137717493));
#232173=CARTESIAN_POINT('Ctrl Pts',(-5.86086320639216,5.31359469386752,
112.399978445572));
#232174=CARTESIAN_POINT('Ctrl Pts',(-5.85466325138469,5.32042519996339,
112.399608468074));
#232175=CARTESIAN_POINT('Ctrl Pts',(-5.84412313802294,5.3319965359537,112.398981626152));
#232176=CARTESIAN_POINT('Ctrl Pts',(-5.83978913068446,5.33674294127286,
112.398724482531));
#232177=CARTESIAN_POINT('Ctrl Pts',(-5.83142113724213,5.34588478297197,
112.398229166124));
#232178=CARTESIAN_POINT('Ctrl Pts',(-5.82738795495744,5.35028094732624,
112.397990957017));
#232179=CARTESIAN_POINT('Ctrl Pts',(-5.81784620955809,5.36065785097451,
112.39742862973));
#232180=CARTESIAN_POINT('Ctrl Pts',(-5.81233338603798,5.3666346739256,112.397104706412));
#232181=CARTESIAN_POINT('Ctrl Pts',(-5.79618724268989,5.38408573226781,
112.396158802609));
#232182=CARTESIAN_POINT('Ctrl Pts',(-5.78552906125236,5.39553697142363,
112.395537961112));
#232183=CARTESIAN_POINT('Ctrl Pts',(-5.70765179494423,5.47871287801388,
112.391027296917));
#232184=CARTESIAN_POINT('Ctrl Pts',(-5.63913361408311,5.54921226987187,
112.387197779424));
#232185=CARTESIAN_POINT('Ctrl Pts',(-5.41503067902359,5.77135672064771,
112.37509383494));
#232186=CARTESIAN_POINT('Ctrl Pts',(-5.25450415597635,5.91788052226589,
112.367055924889));
#232187=CARTESIAN_POINT('Ctrl Pts',(-4.9208061765846,6.19817268219947,112.351383868402));
#232188=CARTESIAN_POINT('Ctrl Pts',(-4.74771440858341,6.33173679699968,
112.343759134459));
#232189=CARTESIAN_POINT('Ctrl Pts',(-4.41354777934905,6.5681751577929,112.329690138851));
#232190=CARTESIAN_POINT('Ctrl Pts',(-4.25384838785275,6.67271335445584,
112.323222706623));
#232191=CARTESIAN_POINT('Ctrl Pts',(-3.69173636729675,7.0122800344171,112.300903630733));
#232192=CARTESIAN_POINT('Ctrl Pts',(-3.27248271782822,7.21746215752754,
112.285047760965));
#232193=CARTESIAN_POINT('Ctrl Pts',(-2.76508760558085,7.4124393604572,112.264126196738));
#232194=CARTESIAN_POINT('Ctrl Pts',(-2.69210259560071,7.43925732745265,
112.261075767721));
#232195=CARTESIAN_POINT('Ctrl Pts',(-2.60975324957411,7.46814566053639,
112.257575271975));
#232196=CARTESIAN_POINT('Ctrl Pts',(-2.60076441714839,7.47128075198408,
112.257192390781));
#232197=CARTESIAN_POINT('Ctrl Pts',(-2.58712288988608,7.47601099142808,
112.256610138986));
#232198=CARTESIAN_POINT('Ctrl Pts',(-2.58247437606134,7.47761802234531,
112.256411521769));
#232199=CARTESIAN_POINT('Ctrl Pts',(-2.57436915886316,7.4804116056973,112.256064851282));
#232200=CARTESIAN_POINT('Ctrl Pts',(-2.57091312191444,7.48160010133083,
112.255916918622));
#232201=CARTESIAN_POINT('Ctrl Pts',(-2.5636862234181,7.48407975868727,112.255607342027));
#232202=CARTESIAN_POINT('Ctrl Pts',(-2.5599152079401,7.48537046608772,112.25544567017));
#232203=CARTESIAN_POINT('Ctrl Pts',(-2.55097397450865,7.48842323973973,
112.255062024824));
#232204=CARTESIAN_POINT('Ctrl Pts',(-2.5458029095474,7.49018280027567,112.254839898448));
#232205=CARTESIAN_POINT('Ctrl Pts',(-2.52863953070263,7.49600316366971,
112.254101817632));
#232206=CARTESIAN_POINT('Ctrl Pts',(-2.51663934455676,7.50004051401404,
112.253584448281));
#232207=CARTESIAN_POINT('Ctrl Pts',(-2.30543729789122,7.57053350963195,
112.244456206782));
#232208=CARTESIAN_POINT('Ctrl Pts',(-2.10369098035574,7.62905563255482,
112.235384477075));
#232209=CARTESIAN_POINT('Ctrl Pts',(-1.41324078680129,7.79987023753732,
112.20370808742));
#232210=CARTESIAN_POINT('Ctrl Pts',(-0.916279749184769,7.87373114606134,
112.179928462444));
#232211=CARTESIAN_POINT('Ctrl Pts',(0.1846609846624,7.93166019708067,112.128819944313));
#232212=CARTESIAN_POINT('Ctrl Pts',(0.786726088605145,7.89471988969007,
112.101987522156));
#232213=CARTESIAN_POINT('Ctrl Pts',(1.41984442582819,7.7826534291933,112.075734421887));
#232214=CARTESIAN_POINT('Ctrl Pts',(1.46076240340292,7.77507722550135,112.074045601871));
#232215=CARTESIAN_POINT('Ctrl Pts',(1.51454879200776,7.76467876872756,112.071835775343));
#232216=CARTESIAN_POINT('Ctrl Pts',(1.52747224572763,7.76214680134332,112.071305582399));
#232217=CARTESIAN_POINT('Ctrl Pts',(1.54746249932182,7.75817844690892,112.070486648974));
#232218=CARTESIAN_POINT('Ctrl Pts',(1.55453372987065,7.75676465312302,112.070197193081));
#232219=CARTESIAN_POINT('Ctrl Pts',(1.56794197680835,7.75406479008347,112.069648766825));
#232220=CARTESIAN_POINT('Ctrl Pts',(1.57427936616429,7.7527806165897,112.069389736666));
#232221=CARTESIAN_POINT('Ctrl Pts',(1.58892828366458,7.74979353857117,112.06879140686));
#232222=CARTESIAN_POINT('Ctrl Pts',(1.59723866800853,7.74808502916086,112.068452285077));
#232223=CARTESIAN_POINT('Ctrl Pts',(1.62052090852031,7.74325944656354,112.067503076921));
#232224=CARTESIAN_POINT('Ctrl Pts',(1.63548653414615,7.74011231647928,112.066893943067));
#232225=CARTESIAN_POINT('Ctrl Pts',(1.721757171729,7.72170903245117,112.063388271127));
#232226=CARTESIAN_POINT('Ctrl Pts',(1.79285871039398,7.70551076413261,112.060521660518));
#232227=CARTESIAN_POINT('Ctrl Pts',(1.99695951658718,7.656034716535,112.052352417551));
#232228=CARTESIAN_POINT('Ctrl Pts',(2.12933290619281,7.62027941527067,112.047127790685));
#232229=CARTESIAN_POINT('Ctrl Pts',(2.58701521984609,7.48379674542077,112.029255871272));
#232230=CARTESIAN_POINT('Ctrl Pts',(2.90670469264634,7.36552424538543,112.017131959862));
#232231=CARTESIAN_POINT('Ctrl Pts',(3.52866640681707,7.08859914083725,111.993349623488));
#232232=CARTESIAN_POINT('Ctrl Pts',(3.8302831698902,6.93027054635327,111.981712036828));
#232233=CARTESIAN_POINT('Ctrl Pts',(4.43647602569573,6.56036509885454,111.956694794425));
#232234=CARTESIAN_POINT('Ctrl Pts',(4.7382920730877,6.34581052912333,111.943224246407));
#232235=CARTESIAN_POINT('Ctrl Pts',(5.04737757370442,6.09170063017525,111.927344412878));
#232236=CARTESIAN_POINT('Ctrl Pts',(5.07064496526052,6.0723468729355,111.926136824991));
#232237=CARTESIAN_POINT('Ctrl Pts',(5.1022974516512,6.04570963937785,111.924477864752));
#232238=CARTESIAN_POINT('Ctrl Pts',(5.1107792804007,6.03854117104392,111.924031715948));
#232239=CARTESIAN_POINT('Ctrl Pts',(5.12419651889446,6.02715299288839,111.92332344986));
#232240=CARTESIAN_POINT('Ctrl Pts',(5.12914189238221,6.02294501149395,111.923061851703));
#232241=CARTESIAN_POINT('Ctrl Pts',(5.13912362365291,6.01443042129828,111.922532752217));
#232242=CARTESIAN_POINT('Ctrl Pts',(5.14415976185402,6.01012356412406,111.922265240131));
#232243=CARTESIAN_POINT('Ctrl Pts',(5.15563377340891,6.0002861122001,111.921654482681));
#232244=CARTESIAN_POINT('Ctrl Pts',(5.16206816534394,5.99475147854484,111.921311064176));
#232245=CARTESIAN_POINT('Ctrl Pts',(5.17555368921598,5.98311390284775,111.920589398495));
#232246=CARTESIAN_POINT('Ctrl Pts',(5.18260295955651,5.97700882776834,111.92021106186));
#232247=CARTESIAN_POINT('Ctrl Pts',(5.20116649400566,5.96087420366462,111.919211871433));
#232248=CARTESIAN_POINT('Ctrl Pts',(5.21266251780874,5.95082377846834,111.918590161127));
#232249=CARTESIAN_POINT('Ctrl Pts',(5.2471467513808,5.92049925814134,111.916716544574));
#232250=CARTESIAN_POINT('Ctrl Pts',(5.27004619179904,5.90012488064244,111.915460683213));
#232251=CARTESIAN_POINT('Ctrl Pts',(5.56022372823688,5.63890734391712,111.899402005965));
#232252=CARTESIAN_POINT('Ctrl Pts',(5.81088135188796,5.38024221944273,111.88398235848));
#232253=CARTESIAN_POINT('Ctrl Pts',(6.38462290335778,4.70113133761827,111.8457484389));
#232254=CARTESIAN_POINT('Ctrl Pts',(6.68477048956573,4.26355829717568,111.823047272943));
#232255=CARTESIAN_POINT('Ctrl Pts',(6.95537383710379,3.76933179892526,111.799485201527));
#232256=CARTESIAN_POINT('Ctrl Pts',(6.97158180182717,3.73926926230999,111.798059076561));
#232257=CARTESIAN_POINT('Ctrl Pts',(7.18577932424425,3.33574161648553,111.779008338274));
#232258=CARTESIAN_POINT('Ctrl Pts',(7.35372820958812,2.94708229346627,111.761636113289));
#232259=CARTESIAN_POINT('Ctrl Pts',(7.50849735888368,2.49193793688402,111.742135234959));
#232260=CARTESIAN_POINT('Ctrl Pts',(7.52657140659689,2.43680327303146,111.739787948531));
#232261=CARTESIAN_POINT('Ctrl Pts',(7.55206797975294,2.35603520327152,111.736371061823));
#232262=CARTESIAN_POINT('Ctrl Pts',(7.55996986438192,2.33055536420826,111.735296269418));
#232263=CARTESIAN_POINT('Ctrl Pts',(7.57364094954481,2.28567135550215,111.733408432078));
#232264=CARTESIAN_POINT('Ctrl Pts',(7.57946482655216,2.26628412247278,111.732594783776));
#232265=CARTESIAN_POINT('Ctrl Pts',(7.59133159270417,2.22622316008193,111.730917152477));
#232266=CARTESIAN_POINT('Ctrl Pts',(7.59736459568749,2.20554666973773,111.730053287685));
#232267=CARTESIAN_POINT('Ctrl Pts',(7.61260208808465,2.15251984859686,111.727842906393));
#232268=CARTESIAN_POINT('Ctrl Pts',(7.62168486080764,2.1201349356626,111.726497799911));
#232269=CARTESIAN_POINT('Ctrl Pts',(7.64094068252225,2.04975451102119,111.723584834628));
#232270=CARTESIAN_POINT('Ctrl Pts',(7.65103745866591,2.01173902279244,111.722017889209));
#232271=CARTESIAN_POINT('Ctrl Pts',(7.7771514331278,1.52221938418228,111.701921376334));
#232272=CARTESIAN_POINT('Ctrl Pts',(7.85332464510056,1.06138845881248,111.683947989645));
#232273=CARTESIAN_POINT('Ctrl Pts',(7.91810388045191,0.204746528739609,
111.650939998041));
#232274=CARTESIAN_POINT('Ctrl Pts',(7.91850164150383,-0.188683439909868,
111.635914772417));
#232275=CARTESIAN_POINT('Ctrl Pts',(7.88661785189892,-0.622023875752945,
111.618622994193));
#232276=CARTESIAN_POINT('Ctrl Pts',(7.88323461667545,-0.663526015734557,
111.616959081432));
#232277=CARTESIAN_POINT('Ctrl Pts',(7.87819218186543,-0.719883505418238,
111.61468739305));
#232278=CARTESIAN_POINT('Ctrl Pts',(7.87681828539855,-0.734763914900181,
111.614086417659));
#232279=CARTESIAN_POINT('Ctrl Pts',(7.87442117027659,-0.759946987317319,
111.613067409755));
#232280=CARTESIAN_POINT('Ctrl Pts',(7.87341987113188,-0.770251726726619,
111.612649890272));
#232281=CARTESIAN_POINT('Ctrl Pts',(7.87139186024123,-0.790705533046299,
111.611820090674));
#232282=CARTESIAN_POINT('Ctrl Pts',(7.87036574130037,-0.800854640311396,
111.611407824644));
#232283=CARTESIAN_POINT('Ctrl Pts',(7.86783801239251,-0.825381724815755,
111.610410273401));
#232284=CARTESIAN_POINT('Ctrl Pts',(7.86631661806772,-0.839757609815118,
111.609824556499));
#232285=CARTESIAN_POINT('Ctrl Pts',(7.86100591509645,-0.888658152848299,
111.607828793702));
#232286=CARTESIAN_POINT('Ctrl Pts',(7.85702866795913,-0.923161846681067,
111.606414824047));
#232287=CARTESIAN_POINT('Ctrl Pts',(7.84687561329931,-1.00641893485256,
111.602989880116));
#232288=CARTESIAN_POINT('Ctrl Pts',(7.84047250443339,-1.05514302689035,
111.600974695536));
#232289=CARTESIAN_POINT('Ctrl Pts',(7.81437345816508,-1.24036604674837,
111.593276721959));
#232290=CARTESIAN_POINT('Ctrl Pts',(7.79156355174329,-1.3763999970876,111.587546066637));
#232291=CARTESIAN_POINT('Ctrl Pts',(7.72064885037628,-1.74065442281843,
111.572047336249));
#232292=CARTESIAN_POINT('Ctrl Pts',(7.66598971947217,-1.96745962859462,
111.562234882232));
#232293=CARTESIAN_POINT('Ctrl Pts',(7.50660473977578,-2.52029470362026,
111.538080029504));
#232294=CARTESIAN_POINT('Ctrl Pts',(7.39058422396799,-2.84258238656474,
111.523798477966));
#232295=CARTESIAN_POINT('Ctrl Pts',(7.19327508315327,-3.29604682436632,
111.503480505372));
#232296=CARTESIAN_POINT('Ctrl Pts',(7.12846730226794,-3.43396070733405,
111.497266942646));
#232297=CARTESIAN_POINT('Ctrl Pts',(7.03958940059646,-3.6097217990437,111.489292499587));
#232298=CARTESIAN_POINT('Ctrl Pts',(7.01912568190696,-3.64935406408052,
111.487490549286));
#232299=CARTESIAN_POINT('Ctrl Pts',(6.98579420650509,-3.71258977160168,
111.48460877309));
#232300=CARTESIAN_POINT('Ctrl Pts',(6.97313945824269,-3.73630427156449,
111.4835265408));
#232301=CARTESIAN_POINT('Ctrl Pts',(6.95000413926029,-3.77913198934423,
111.481569156271));
#232302=CARTESIAN_POINT('Ctrl Pts',(6.93956497578531,-3.79826724686233,
111.480693547084));
#232303=CARTESIAN_POINT('Ctrl Pts',(6.91463924627986,-3.84351097183807,
111.478620616649));
#232304=CARTESIAN_POINT('Ctrl Pts',(6.90008367977602,-3.86958107767362,
111.477424080412));
#232305=CARTESIAN_POINT('Ctrl Pts',(6.85635964697601,-3.94686290188376,
111.473870477624));
#232306=CARTESIAN_POINT('Ctrl Pts',(6.82676604488052,-3.99783188732277,
111.471518125612));
#232307=CARTESIAN_POINT('Ctrl Pts',(6.62569997611054,-4.33538366262448,
111.455873394658));
#232308=CARTESIAN_POINT('Ctrl Pts',(6.43679086253933,-4.61120213876708,
111.442724663278));
#232309=CARTESIAN_POINT('Ctrl Pts',(5.950388605081,-5.2329955114721,111.412095534704));
#232310=CARTESIAN_POINT('Ctrl Pts',(5.63930299689599,-5.56683474593546,
111.394960583603));
#232311=CARTESIAN_POINT('Ctrl Pts',(4.93344773447329,-6.20407109166134,
111.359605980503));
#232312=CARTESIAN_POINT('Ctrl Pts',(4.53533003857126,-6.50077865161586,
111.341503892046));
#232313=CARTESIAN_POINT('Ctrl Pts',(4.10713212375609,-6.76131797390543,
111.321831028263));
#232314=CARTESIAN_POINT('Ctrl Pts',(4.10214553370757,-6.76434453929955,
111.321601888493));
#232315=CARTESIAN_POINT('Ctrl Pts',(4.09341197903241,-6.76963208170764,
111.32120049619));
#232316=CARTESIAN_POINT('Ctrl Pts',(4.0896664743973,-6.77189547171881,111.321028329485));
#232317=CARTESIAN_POINT('Ctrl Pts',(4.06155894517909,-6.78884888918424,
111.319736139082));
#232318=CARTESIAN_POINT('Ctrl Pts',(4.03711987854779,-6.80341042194274,
111.318611510874));
#232319=CARTESIAN_POINT('Ctrl Pts',(3.98759450182436,-6.8325583166099,111.316329332017));
#232320=CARTESIAN_POINT('Ctrl Pts',(3.96250542414426,-6.84713909591076,
111.315171591118));
#232321=CARTESIAN_POINT('Ctrl Pts',(3.92843139823489,-6.86669157390015,
111.313596377551));
#232322=CARTESIAN_POINT('Ctrl Pts',(3.91951599262595,-6.87178439737819,
111.313183962083));
#232323=CARTESIAN_POINT('Ctrl Pts',(3.90545208116505,-6.87978197229042,
111.312532932222));
#232324=CARTESIAN_POINT('Ctrl Pts',(3.90031017346697,-6.88269834404029,
111.31229481438));
#232325=CARTESIAN_POINT('Ctrl Pts',(3.8900333939987,-6.88851188241089,111.311818706654));
#232326=CARTESIAN_POINT('Ctrl Pts',(3.88489854310113,-6.89140907725707,
111.311580718258));
#232327=CARTESIAN_POINT('Ctrl Pts',(3.87322205158826,-6.89798001074148,
111.311039306507));
#232328=CARTESIAN_POINT('Ctrl Pts',(3.86667841954505,-6.90165018592094,
111.31073572721));
#232329=CARTESIAN_POINT('Ctrl Pts',(3.84739268711605,-6.91243107993378,
111.309840486735));
#232330=CARTESIAN_POINT('Ctrl Pts',(3.83463616454897,-6.91951583605683,
111.309247669123));
#232331=CARTESIAN_POINT('Ctrl Pts',(3.80576419757159,-6.93544647657645,
111.307904295135));
#232332=CARTESIAN_POINT('Ctrl Pts',(3.78963740938042,-6.94427154238952,
111.307152784459));
#232333=CARTESIAN_POINT('Ctrl Pts',(3.73853757340752,-6.97200390219291,
111.304767461512));
#232334=CARTESIAN_POINT('Ctrl Pts',(3.70345306045986,-6.99070360849325,
111.303123732742));
#232335=CARTESIAN_POINT('Ctrl Pts',(3.56958117391429,-7.06076540902813,
111.29682383237));
#232336=CARTESIAN_POINT('Ctrl Pts',(3.46985809830789,-7.11030242170683,
111.292072624146));
#232337=CARTESIAN_POINT('Ctrl Pts',(3.13213093139495,-7.26927014301055,
111.2758602999));
#232338=CARTESIAN_POINT('Ctrl Pts',(2.88975138593265,-7.36897930136424,
111.264029474646));
#232339=CARTESIAN_POINT('Ctrl Pts',(2.10174187432691,-7.64828276653502,
111.225770356771));
#232340=CARTESIAN_POINT('Ctrl Pts',(1.5412703510745,-7.78062527016558,111.198985420755));
#232341=CARTESIAN_POINT('Ctrl Pts',(0.867232250670853,-7.86402227863397,
111.169160921739));
#232342=CARTESIAN_POINT('Ctrl Pts',(0.762815493206369,-7.8748366125221,
111.16460217229));
#232343=CARTESIAN_POINT('Ctrl Pts',(0.445424056729578,-7.90133613885045,
111.150940046646));
#232344=CARTESIAN_POINT('Ctrl Pts',(0.231995195635322,-7.91048054978834,
111.142020878728));
#232345=CARTESIAN_POINT('Ctrl Pts',(-0.00235140532270151,-7.91102698930574,
111.132515582081));
#232346=CARTESIAN_POINT('Ctrl Pts',(-0.0231495041654061,-7.91099346879504,
111.131674450472));
#232347=CARTESIAN_POINT('Ctrl Pts',(-0.0540324159673709,-7.91082190484312,
111.130429073522));
#232348=CARTESIAN_POINT('Ctrl Pts',(-0.0641174088612166,-7.91074659377375,
111.130022960402));
#232349=CARTESIAN_POINT('Ctrl Pts',(-0.0813818067504496,-7.91058465298454,
111.129328713199));
#232350=CARTESIAN_POINT('Ctrl Pts',(-0.0885612775438487,-7.91050753434852,
111.129040295934));
#232351=CARTESIAN_POINT('Ctrl Pts',(-0.102528298626715,-7.91033849003725,
111.128479764394));
#232352=CARTESIAN_POINT('Ctrl Pts',(-0.109315854686147,-7.91024760188971,
111.128207619409));
#232353=CARTESIAN_POINT('Ctrl Pts',(-0.125549181610145,-7.91000933292641,
111.127557360462));
#232354=CARTESIAN_POINT('Ctrl Pts',(-0.134994831181229,-7.90985376857823,
111.127179490808));
#232355=CARTESIAN_POINT('Ctrl Pts',(-0.16330912476675,-7.90933671585864,
111.126048263469));
#232356=CARTESIAN_POINT('Ctrl Pts',(-0.182176835170889,-7.90892462739567,
111.125296415184));
#232357=CARTESIAN_POINT('Ctrl Pts',(-0.346466217203392,-7.90474817736555,
111.118766631609));
#232358=CARTESIAN_POINT('Ctrl Pts',(-0.491763757892237,-7.89704081335171,
111.113107615084));
#232359=CARTESIAN_POINT('Ctrl Pts',(-1.02375288340134,-7.85408063664059,
111.092753650817));
#232360=CARTESIAN_POINT('Ctrl Pts',(-1.40792547580746,-7.7943844299036,
111.078795147707));
#232361=CARTESIAN_POINT('Ctrl Pts',(-1.85159402073955,-7.69155572615592,
111.062854385325));
#232362=CARTESIAN_POINT('Ctrl Pts',(-1.91681306457954,-7.67556236793706,
111.060514799688));
#232363=CARTESIAN_POINT('Ctrl Pts',(-2.03647610356062,-7.64459765425372,
111.056221222414));
#232364=CARTESIAN_POINT('Ctrl Pts',(-2.09097850024661,-7.6298700616622,
111.054265278994));
#232365=CARTESIAN_POINT('Ctrl Pts',(-2.19196070026748,-7.60141943631396,
111.050635652101));
#232366=CARTESIAN_POINT('Ctrl Pts',(-2.23848101643335,-7.58785028227303,
111.048961312495));
#232367=CARTESIAN_POINT('Ctrl Pts',(-2.32524980233874,-7.56167395148363,
111.045830831975));
#232368=CARTESIAN_POINT('Ctrl Pts',(-2.36552779220756,-7.54917067337047,
111.044374604609));
#232369=CARTESIAN_POINT('Ctrl Pts',(-2.44102271524304,-7.52507166964829,
111.041637080661));
#232370=CARTESIAN_POINT('Ctrl Pts',(-2.47626184338731,-7.51354928169662,
111.040355954133));
#232371=CARTESIAN_POINT('Ctrl Pts',(-2.81608528283476,-7.39978441996949,
111.027961215968));
#232372=CARTESIAN_POINT('Ctrl Pts',(-3.11424351042991,-7.2793279900415,
111.016779634582));
#232373=CARTESIAN_POINT('Ctrl Pts',(-3.59223945019578,-7.05146181911222,
110.997327884815));
#232374=CARTESIAN_POINT('Ctrl Pts',(-3.77662592146045,-6.95445130273584,
110.989419127928));
#232375=CARTESIAN_POINT('Ctrl Pts',(-3.970578985214,-6.8424170131216,110.980471380863));
#232376=CARTESIAN_POINT('Ctrl Pts',(-3.98416605645883,-6.8345145320256,
110.979841303779));
#232377=CARTESIAN_POINT('Ctrl Pts',(-4.00330987262827,-6.82330366355085,
110.978949037186));
#232378=CARTESIAN_POINT('Ctrl Pts',(-4.00888631224433,-6.82002883838947,
110.978688585846));
#232379=CARTESIAN_POINT('Ctrl Pts',(-4.01859119105505,-6.81431352663,110.978234378188));
#232380=CARTESIAN_POINT('Ctrl Pts',(-4.0227214431666,-6.81187611385912,
110.978040778753));
#232381=CARTESIAN_POINT('Ctrl Pts',(-4.03104700064761,-6.80695268526882,
110.977649938508));
#232382=CARTESIAN_POINT('Ctrl Pts',(-4.03524222936281,-6.80446654272952,
110.977452691322));
#232383=CARTESIAN_POINT('Ctrl Pts',(-4.04382060397708,-6.79937217232032,
110.977048744196));
#232384=CARTESIAN_POINT('Ctrl Pts',(-4.04820353142919,-6.79676358150146,
110.976842026174));
#232385=CARTESIAN_POINT('Ctrl Pts',(-4.06274919730392,-6.78808736370599,
110.976154899337));
#232386=CARTESIAN_POINT('Ctrl Pts',(-4.07290080979013,-6.7820011861529,
110.97567357628));
#232387=CARTESIAN_POINT('Ctrl Pts',(-4.14367277157242,-6.73935519264396,
110.972305878843));
#232388=CARTESIAN_POINT('Ctrl Pts',(-4.2038125001105,-6.70200660272594,
110.969381783264));
#232389=CARTESIAN_POINT('Ctrl Pts',(-4.39431525120925,-6.5801256287458,
110.959937956363));
#232390=CARTESIAN_POINT('Ctrl Pts',(-4.5226901008181,-6.49255966865117,
110.953299013851));
#232391=CARTESIAN_POINT('Ctrl Pts',(-4.78121643000406,-6.3048261755347,
110.939471899504));
#232392=CARTESIAN_POINT('Ctrl Pts',(-4.91099821715921,-6.20426938742024,
110.932277328013));
#232393=CARTESIAN_POINT('Ctrl Pts',(-5.38933714422978,-5.80922712670214,
110.904990526582));
#232394=CARTESIAN_POINT('Ctrl Pts',(-5.71534656372106,-5.48880020943202,
110.884849278843));
#232395=CARTESIAN_POINT('Ctrl Pts',(-6.20145865784987,-4.92045328379064,
110.853027434505));
#232396=CARTESIAN_POINT('Ctrl Pts',(-6.37860261586297,-4.68853850562576,
110.84092226146));
#232397=CARTESIAN_POINT('Ctrl Pts',(-6.56259133278112,-4.41787137633144,
110.827674004635));
#232398=CARTESIAN_POINT('Ctrl Pts',(-6.58243787344046,-4.38824613782523,
110.826235016445));
#232399=CARTESIAN_POINT('Ctrl Pts',(-6.61120130874972,-4.34467629869567,
110.824134432034));
#232400=CARTESIAN_POINT('Ctrl Pts',(-6.62027573997042,-4.33083641049326,
110.823469488958));
#232401=CARTESIAN_POINT('Ctrl Pts',(-6.63630348094039,-4.30622357861167,
110.822290983533));
#232402=CARTESIAN_POINT('Ctrl Pts',(-6.64327414588325,-4.2954620268234,
110.82177706116));
#232403=CARTESIAN_POINT('Ctrl Pts',(-6.65772833241956,-4.27302781452356,
110.820708501143));
#232404=CARTESIAN_POINT('Ctrl Pts',(-6.66520739301084,-4.26135232778572,
110.820153956034));
#232405=CARTESIAN_POINT('Ctrl Pts',(-6.68450323710811,-4.23105470184876,
110.818718929504));
#232406=CARTESIAN_POINT('Ctrl Pts',(-6.69627292924543,-4.21240267298676,
110.817839394459));
#232407=CARTESIAN_POINT('Ctrl Pts',(-6.74432992799329,-4.13553391334734,
110.814230331489));
#232408=CARTESIAN_POINT('Ctrl Pts',(-6.77993768657995,-4.07689490615675,
110.811513743266));
#232409=CARTESIAN_POINT('Ctrl Pts',(-7.00209447447337,-3.70008437201776,
110.794283977837));
#232410=CARTESIAN_POINT('Ctrl Pts',(-7.16696771580084,-3.36965062731502,
110.780223435643));
#232411=CARTESIAN_POINT('Ctrl Pts',(-7.49821346624278,-2.57041591087699,
110.747930290955));
#232412=CARTESIAN_POINT('Ctrl Pts',(-7.64466414307928,-2.09507407916465,
110.730037128669));
#232413=CARTESIAN_POINT('Ctrl Pts',(-7.7538733298244,-1.56940062958409,
110.709936685136));
#232414=CARTESIAN_POINT('Ctrl Pts',(-7.76182688411091,-1.52957946506288,
110.708411634109));
#232415=CARTESIAN_POINT('Ctrl Pts',(-7.79560845134439,-1.35339287706458,
110.701648713176));
#232416=CARTESIAN_POINT('Ctrl Pts',(-7.81815132214717,-1.21642568737082,
110.696350802941));
#232417=CARTESIAN_POINT('Ctrl Pts',(-7.84945358411972,-0.989055971269558,
110.68741255796));
#232418=CARTESIAN_POINT('Ctrl Pts',(-7.86028052091558,-0.898967564056434,
110.683834002599));
#232419=CARTESIAN_POINT('Ctrl Pts',(-7.87108054967468,-0.793873155461385,
110.679600336813));
#232420=CARTESIAN_POINT('Ctrl Pts',(-7.87256377471032,-0.779027095671503,
110.679000902662));
#232421=CARTESIAN_POINT('Ctrl Pts',(-7.87473154053604,-0.756690648616988,
110.678096878959));
#232422=CARTESIAN_POINT('Ctrl Pts',(-7.87544741611877,-0.749203289281413,
110.677793479182));
#232423=CARTESIAN_POINT('Ctrl Pts',(-7.87670319390409,-0.735868385275503,
110.677252465814));
#232424=CARTESIAN_POINT('Ctrl Pts',(-7.87724726570195,-0.730021232607731,
110.67701501319));
#232425=CARTESIAN_POINT('Ctrl Pts',(-7.87828431509094,-0.71873988627927,
110.676556433943));
#232426=CARTESIAN_POINT('Ctrl Pts',(-7.87877818209959,-0.713305776377036,
110.676335342184));
#232427=CARTESIAN_POINT('Ctrl Pts',(-7.87983326485453,-0.701561721111284,
110.675857088325));
#232428=CARTESIAN_POINT('Ctrl Pts',(-7.88039252403279,-0.695251607182838,
110.675599849153));
#232429=CARTESIAN_POINT('Ctrl Pts',(-7.88172741698934,-0.679981476153497,
110.674976674643));
#232430=CARTESIAN_POINT('Ctrl Pts',(-7.88249535100039,-0.671020807569307,
110.674610431649));
#232431=CARTESIAN_POINT('Ctrl Pts',(-7.88452897022534,-0.646806156399707,
110.673619179338));
#232432=CARTESIAN_POINT('Ctrl Pts',(-7.88576566332396,-0.631549827668696,
110.672992990196));
#232433=CARTESIAN_POINT('Ctrl Pts',(-7.90289099036284,-0.412388850801295,
110.663972883019));
#232434=CARTESIAN_POINT('Ctrl Pts',(-7.91090819443579,-0.207985776564891,
110.655206635585));
#232435=CARTESIAN_POINT('Ctrl Pts',(-7.91099921610637,-0.0035217558676004,
110.646171848042));
#232436=CARTESIAN_POINT('',(-7.91099910237999,-0.00376857307924841,108.642331508237));
#232437=CARTESIAN_POINT('Ctrl Pts',(-7.9109991388093,-0.00369130851947151,
110.642331508237));
#232438=CARTESIAN_POINT('Ctrl Pts',(-7.91108984706874,0.190709392081641,
110.634473652374));
#232439=CARTESIAN_POINT('Ctrl Pts',(-7.90401071543908,0.385365611992972,
110.626615796511));
#232440=CARTESIAN_POINT('Ctrl Pts',(-7.88973162020115,0.579703338957264,
110.618757940648));
#232441=CARTESIAN_POINT('Ctrl Pts',(-7.87546640843135,0.773852112658492,
110.610907724926));
#232442=CARTESIAN_POINT('Ctrl Pts',(-7.85401520049234,0.967682664111825,
110.603057509203));
#232443=CARTESIAN_POINT('Ctrl Pts',(-7.82539986755185,1.16061962456248,
110.595207293481));
#232444=CARTESIAN_POINT('Ctrl Pts',(-7.79680686265294,1.35340603969237,
110.587363203143));
#232445=CARTESIAN_POINT('Ctrl Pts',(-7.76106091824334,1.54529990849815,
110.579519112806));
#232446=CARTESIAN_POINT('Ctrl Pts',(-7.71823583503914,1.73572941287452,
110.571675022469));
#232447=CARTESIAN_POINT('Ctrl Pts',(-7.67543594727013,1.92604688117582,
110.563835547074));
#232448=CARTESIAN_POINT('Ctrl Pts',(-7.62556529419268,2.11490136119825,
110.555996071679));
#232449=CARTESIAN_POINT('Ctrl Pts',(-7.56874906919273,2.30172946446671,
110.548156596284));
#232450=CARTESIAN_POINT('Ctrl Pts',(-7.51195536767827,2.4884835040311,110.540320228668));
#232451=CARTESIAN_POINT('Ctrl Pts',(-7.44822168199577,2.67321243338912,
110.532483861052));
#232452=CARTESIAN_POINT('Ctrl Pts',(-7.3777235947799,2.85536609894912,110.524647493437));
#232453=CARTESIAN_POINT('Ctrl Pts',(-7.30722777829498,3.0375138973717,110.516811378229));
#232454=CARTESIAN_POINT('Ctrl Pts',(-7.2299681116985,3.21708626780124,110.508975263022));
#232455=CARTESIAN_POINT('Ctrl Pts',(-7.14616922654664,3.39355070472768,
110.501139147814));
#232456=CARTESIAN_POINT('Ctrl Pts',(-7.06236815198715,3.57001975212819,
110.493302827873));
#232457=CARTESIAN_POINT('Ctrl Pts',(-6.97202766773697,3.74338038774425,
110.485466507932));
#232458=CARTESIAN_POINT('Ctrl Pts',(-6.87541949451138,3.91312250951754,
110.477630187991));
#232459=CARTESIAN_POINT('Ctrl Pts',(-6.77879200126569,4.08289857687842,
110.469792300917));
#232460=CARTESIAN_POINT('Ctrl Pts',(-6.67589449477884,4.24905438453467,
110.461954413843));
#232461=CARTESIAN_POINT('Ctrl Pts',(-6.56704344752397,4.41110659113249,
110.454116526768));
#232462=CARTESIAN_POINT('Ctrl Pts',(-6.45815170657815,4.57321938054122,
110.44627570952));
#232463=CARTESIAN_POINT('Ctrl Pts',(-6.34330218571348,4.73122522240785,
110.438434892271));
#232464=CARTESIAN_POINT('Ctrl Pts',(-6.22285335870696,4.88467164464814,
110.430594075023));
#232465=CARTESIAN_POINT('Ctrl Pts',(-6.10227040815279,5.03828893429358,
110.422744526778));
#232466=CARTESIAN_POINT('Ctrl Pts',(-5.97607591239378,5.18733638688799,
110.414894978533));
#232467=CARTESIAN_POINT('Ctrl Pts',(-5.84466789434017,5.33139552133109,
110.407045430289));
#232468=CARTESIAN_POINT('Ctrl Pts',(-5.71318149038901,5.47554058816038,
110.399191199728));
#232469=CARTESIAN_POINT('Ctrl Pts',(-5.57647561008188,5.61469115706509,
110.391336969167));
#232470=CARTESIAN_POINT('Ctrl Pts',(-5.43498356081272,5.74846716035636,
110.383482738607));
#232471=CARTESIAN_POINT('Ctrl Pts',(-5.29328537013972,5.8824380634548,110.375617065127));
#232472=CARTESIAN_POINT('Ctrl Pts',(-5.14678734116829,6.01101852628486,
110.367751391646));
#232473=CARTESIAN_POINT('Ctrl Pts',(-4.99595517980301,6.13386932053491,
110.359885718166));
#232474=CARTESIAN_POINT('Ctrl Pts',(-4.88124835895589,6.22729650422978,
110.353903927608));
#232475=CARTESIAN_POINT('Ctrl Pts',(-4.76403555096897,6.31741078624118,
110.34792213705));
#232476=CARTESIAN_POINT('Ctrl Pts',(-4.64453177222975,6.40408038806106,
110.341940346492));
#232477=CARTESIAN_POINT('Ctrl Pts',(-4.4894974013035,6.5165183991293,110.334180063545));
#232478=CARTESIAN_POINT('Ctrl Pts',(-4.33010429121461,6.62352136419305,
110.326419780599));
#232479=CARTESIAN_POINT('Ctrl Pts',(-4.16677701121442,6.7247223242908,110.318659497652));
#232480=CARTESIAN_POINT('Ctrl Pts',(-4.0036463037658,6.82580148397071,110.310908554594));
#232481=CARTESIAN_POINT('Ctrl Pts',(-3.83659115209274,6.92109235121469,
110.303157611536));
#232482=CARTESIAN_POINT('Ctrl Pts',(-3.6660692748929,7.01026797431356,110.295406668478));
#232483=CARTESIAN_POINT('Ctrl Pts',(-3.49571801846821,7.09935437006993,
110.287663480859));
#232484=CARTESIAN_POINT('Ctrl Pts',(-3.32190725683863,7.18233753736193,
110.27992029324));
#232485=CARTESIAN_POINT('Ctrl Pts',(-3.1451238635176,7.25893359131575,110.27217710562));
#232486=CARTESIAN_POINT('Ctrl Pts',(-2.96848152687951,7.33546852875237,
110.264440096343));
#232487=CARTESIAN_POINT('Ctrl Pts',(-2.78887160832139,7.40562635746628,
110.256703087066));
#232488=CARTESIAN_POINT('Ctrl Pts',(-2.60680585660291,7.46916891133015,
110.248966077789));
#232489=CARTESIAN_POINT('Ctrl Pts',(-2.42484851485477,7.53267362915778,
110.241233675469));
#232490=CARTESIAN_POINT('Ctrl Pts',(-2.24043858962186,7.58957079784827,
110.233501273148));
#232491=CARTESIAN_POINT('Ctrl Pts',(-2.05410818262262,7.63967018752006,
110.225768870827));
#232492=CARTESIAN_POINT('Ctrl Pts',(-1.86785102663061,7.68974988190532,
110.218039508302));
#232493=CARTESIAN_POINT('Ctrl Pts',(-1.67967523874005,7.733037026691,110.210310145776));
#232494=CARTESIAN_POINT('Ctrl Pts',(-1.49012855330268,7.76939108905145,
110.20258078325));
#232495=CARTESIAN_POINT('Ctrl Pts',(-1.30058194181951,7.80574513722787,
110.19485142374));
#232496=CARTESIAN_POINT('Ctrl Pts',(-1.10966478426686,7.83516602950222,
110.18712206423));
#232497=CARTESIAN_POINT('Ctrl Pts',(-0.917935896002376,7.85756417032851,
110.179392704721));
#232498=CARTESIAN_POINT('Ctrl Pts',(-0.726197397598077,7.87996343382998,
110.171662957787));
#232499=CARTESIAN_POINT('Ctrl Pts',(-0.533647444270986,7.8953392022199,
110.163933210854));
#232500=CARTESIAN_POINT('Ctrl Pts',(-0.340850706672871,7.90365369912932,
110.156203463921));
#232501=CARTESIAN_POINT('Ctrl Pts',(-0.148008977977571,7.91197013631192,
110.148471913172));
#232502=CARTESIAN_POINT('Ctrl Pts',(0.0450792907685641,7.91322200498196,
110.140740362423));
#232503=CARTESIAN_POINT('Ctrl Pts',(0.237848639590673,7.90742366543268,
110.133008811675));
#232504=CARTESIAN_POINT('Ctrl Pts',(0.430698306918309,7.90162290997046,
110.125274039529));
#232505=CARTESIAN_POINT('Ctrl Pts',(0.623228431069579,7.88876610768087,
110.117539267383));
#232506=CARTESIAN_POINT('Ctrl Pts',(0.814877834195721,7.86891956467573,
110.109804495237));
#232507=CARTESIAN_POINT('Ctrl Pts',(1.00675577933338,7.84904935465788,110.102060499371));
#232508=CARTESIAN_POINT('Ctrl Pts',(1.19775054866705,7.82217279439749,110.094316503505));
#232509=CARTESIAN_POINT('Ctrl Pts',(1.38730929452159,7.7884076627597,110.08657250764));
#232510=CARTESIAN_POINT('Ctrl Pts',(1.5769910735121,7.75462061585753,110.078823485532));
#232511=CARTESIAN_POINT('Ctrl Pts',(1.76523462286795,7.71393616716581,110.071074463425));
#232512=CARTESIAN_POINT('Ctrl Pts',(1.95150158229113,7.66652219551442,110.063325441317));
#232513=CARTESIAN_POINT('Ctrl Pts',(2.13805320150523,7.61903576414554,110.055564576879));
#232514=CARTESIAN_POINT('Ctrl Pts',(2.32262185483804,7.56479937075622,110.04780371244));
#232515=CARTESIAN_POINT('Ctrl Pts',(2.50468736810706,7.50402972995476,110.040042848002));
#232516=CARTESIAN_POINT('Ctrl Pts',(2.62989220863503,7.46223898634344,110.034705770282));
#232517=CARTESIAN_POINT('Ctrl Pts',(2.75391369809306,7.41735954922493,110.029368692562));
#232518=CARTESIAN_POINT('Ctrl Pts',(2.87658951799054,7.36947445514176,110.024031614842));
#232519=CARTESIAN_POINT('Ctrl Pts',(3.06079135591703,7.29757338819333,110.016017814519));
#232520=CARTESIAN_POINT('Ctrl Pts',(3.2425232983405,7.21867327368883,110.008004014196));
#232521=CARTESIAN_POINT('Ctrl Pts',(3.42122357856288,7.13296223356646,109.999990213873));
#232522=CARTESIAN_POINT('Ctrl Pts',(3.59972016156027,7.04734889391217,109.991985548336));
#232523=CARTESIAN_POINT('Ctrl Pts',(3.77519166916802,6.95494024196256,109.9839808828));
#232524=CARTESIAN_POINT('Ctrl Pts',(3.9470940922213,6.85597325163625,109.975976217263));
#232525=CARTESIAN_POINT('Ctrl Pts',(4.11882975007928,6.7571022707156,109.967979317176));
#232526=CARTESIAN_POINT('Ctrl Pts',(4.28700293523296,6.65168579631498,109.959982417089));
#232527=CARTESIAN_POINT('Ctrl Pts',(4.4510917630098,6.5400078835783,109.951985517002));
#232528=CARTESIAN_POINT('Ctrl Pts',(4.61504924455739,6.42841936433006,109.943995018098));
#232529=CARTESIAN_POINT('Ctrl Pts',(4.77492860934756,6.31057958338252,109.936004519195));
#232530=CARTESIAN_POINT('Ctrl Pts',(4.93023428250269,6.18681751142178,109.928014020291));
#232531=CARTESIAN_POINT('Ctrl Pts',(5.08544197471628,6.06313351983049,109.920028562521));
#232532=CARTESIAN_POINT('Ctrl Pts',(5.2360814660925,5.93353489277946,109.91204310475));
#232533=CARTESIAN_POINT('Ctrl Pts',(5.38168745955893,5.79839297457719,109.90405764698));
#232534=CARTESIAN_POINT('Ctrl Pts',(5.53206752517141,5.65882007622024,109.895810365155));
#232535=CARTESIAN_POINT('Ctrl Pts',(5.6770781182688,5.51333442269674,109.887563083331));
#232536=CARTESIAN_POINT('Ctrl Pts',(5.8162441027465,5.36238990910457,109.879315801506));
#232537=CARTESIAN_POINT('Ctrl Pts',(5.95090076998973,5.21633636581053,109.871335751723));
#232538=CARTESIAN_POINT('Ctrl Pts',(6.08008541267052,5.06517244672517,109.863355701939));
#232539=CARTESIAN_POINT('Ctrl Pts',(6.2034053625291,4.90934648483332,109.855375652156));
#232540=CARTESIAN_POINT('Ctrl Pts',(6.32671551924724,4.75353289746425,109.847396236088));
#232541=CARTESIAN_POINT('Ctrl Pts',(6.44416170370999,4.59305826745981,109.83941682002));
#232542=CARTESIAN_POINT('Ctrl Pts',(6.5553918727083,4.42840359443783,109.831437403952));
#232543=CARTESIAN_POINT('Ctrl Pts',(6.66663030299142,4.26373669218741,109.823457395237));
#232544=CARTESIAN_POINT('Ctrl Pts',(6.77165161057924,4.09488940555458,109.815477386521));
#232545=CARTESIAN_POINT('Ctrl Pts',(6.87014717706925,3.92237157411271,109.807497377806));
#232546=CARTESIAN_POINT('Ctrl Pts',(6.96866519646812,3.74981441575203,109.79951554998));
#232547=CARTESIAN_POINT('Ctrl Pts',(7.06065434426004,3.57358533551647,109.791533722153));
#232548=CARTESIAN_POINT('Ctrl Pts',(7.14585185770023,3.39421894223136,109.783551894327));
#232549=CARTESIAN_POINT('Ctrl Pts',(7.23111271932207,3.2147191819687,109.775564131652));
#232550=CARTESIAN_POINT('Ctrl Pts',(7.30957171547397,3.03207775126201,109.767576368978));
#232551=CARTESIAN_POINT('Ctrl Pts',(7.38101375529517,2.84685035506672,109.759588606303));
#232552=CARTESIAN_POINT('Ctrl Pts',(7.45248726073062,2.66154137814094,109.751597325534));
#232553=CARTESIAN_POINT('Ctrl Pts',(7.51693753527625,2.47364447953964,109.743606044765));
#232554=CARTESIAN_POINT('Ctrl Pts',(7.57419913373819,2.28373126319181,109.735614763996));
#232555=CARTESIAN_POINT('Ctrl Pts',(7.6315146077514,2.09363936375619,109.727615964495));
#232556=CARTESIAN_POINT('Ctrl Pts',(7.68162780970203,1.90152768005897,109.719617164993));
#232557=CARTESIAN_POINT('Ctrl Pts',(7.72442400785416,1.70797972671993,109.711618365491));
#232558=CARTESIAN_POINT('Ctrl Pts',(7.73422488482039,1.66365476890481,109.709786538058));
#232559=CARTESIAN_POINT('Ctrl Pts',(7.74364222166496,1.61925451409568,109.707954710625));
#232560=CARTESIAN_POINT('Ctrl Pts',(7.75267502192603,1.57478601860831,109.706122883193));
#232561=CARTESIAN_POINT('Ctrl Pts',(7.79274781062006,1.37750759201822,109.697996230159));
#232562=CARTESIAN_POINT('Ctrl Pts',(7.82531900144262,1.17853770587763,109.689869577126));
#232563=CARTESIAN_POINT('Ctrl Pts',(7.850255474966,0.978473289245222,109.681742924093));
#232564=CARTESIAN_POINT('Ctrl Pts',(7.87517072144489,0.778579176415713,
109.673623188832));
#232565=CARTESIAN_POINT('Ctrl Pts',(7.89246416802303,0.577592705525485,
109.66550345357));
#232566=CARTESIAN_POINT('Ctrl Pts',(7.90205380306755,0.376120583624052,
109.657383718309));
#232567=CARTESIAN_POINT('Ctrl Pts',(7.91163648259541,0.174794592695505,
109.649269872422));
#232568=CARTESIAN_POINT('Ctrl Pts',(7.913526476612,-0.0270160294569833,
109.641156026535));
#232569=CARTESIAN_POINT('Ctrl Pts',(7.90769357227617,-0.228699293794433,
109.633042180648));
#232570=CARTESIAN_POINT('Ctrl Pts',(7.90186481243599,-0.430239254665368,
109.624934099951));
#232571=CARTESIAN_POINT('Ctrl Pts',(7.88832411098061,-0.631651720315048,
109.616826019253));
#232572=CARTESIAN_POINT('Ctrl Pts',(7.86709333146714,-0.832324164004231,
109.608717938556));
#232573=CARTESIAN_POINT('Ctrl Pts',(7.84587167068052,-1.03291041786692,
109.60061334032));
#232574=CARTESIAN_POINT('Ctrl Pts',(7.81696655103517,-1.23275696702579,
109.592508742084));
#232575=CARTESIAN_POINT('Ctrl Pts',(7.7804517929624,-1.43125500781244,109.584404143848));
#232576=CARTESIAN_POINT('Ctrl Pts',(7.74394844833724,-1.62969100390513,
109.576302078873));
#232577=CARTESIAN_POINT('Ctrl Pts',(7.69984026663045,-1.82677901903057,
109.568200013898));
#232578=CARTESIAN_POINT('Ctrl Pts',(7.64825251602038,-2.02191850755365,
109.560097948923));
#232579=CARTESIAN_POINT('Ctrl Pts',(7.62081094021264,-2.12572096073413,
109.555788138405));
#232580=CARTESIAN_POINT('Ctrl Pts',(7.59125381393921,-2.22897221777876,
109.551478327886));
#232581=CARTESIAN_POINT('Ctrl Pts',(7.55960584956201,-2.33158323876029,
109.547168517368));
#232582=CARTESIAN_POINT('Ctrl Pts',(7.49873986594993,-2.52892675972239,
109.538879805548));
#232583=CARTESIAN_POINT('Ctrl Pts',(7.43016362405021,-2.7238163790082,109.530591093729));
#232584=CARTESIAN_POINT('Ctrl Pts',(7.35410670943434,-2.91565352987162,
109.522302381909));
#232585=CARTESIAN_POINT('Ctrl Pts',(7.27800594875135,-3.10760127297554,
109.514008891728));
#232586=CARTESIAN_POINT('Ctrl Pts',(7.19441601513077,-3.29649276321163,
109.505715401548));
#232587=CARTESIAN_POINT('Ctrl Pts',(7.10361425212357,-3.48175035822888,
109.497421911367));
#232588=CARTESIAN_POINT('Ctrl Pts',(7.01275466831162,-3.66712592169601,
109.489123140052));
#232589=CARTESIAN_POINT('Ctrl Pts',(6.91467421693953,-3.84886270843043,
109.480824368738));
#232590=CARTESIAN_POINT('Ctrl Pts',(6.80969610124708,-4.02640782940083,
109.472525597423));
#232591=CARTESIAN_POINT('Ctrl Pts',(6.70459578496858,-4.20415962314003,
109.464217165859));
#232592=CARTESIAN_POINT('Ctrl Pts',(6.59258190387364,-4.37770974581563,
109.455908734296));
#232593=CARTESIAN_POINT('Ctrl Pts',(6.47402183737178,-4.54653299220772,
109.447600302732));
#232594=CARTESIAN_POINT('Ctrl Pts',(6.35538863498052,-4.71546038022727,
109.439286745965));
#232595=CARTESIAN_POINT('Ctrl Pts',(6.23020135995381,-4.87965483613162,
109.430973189197));
#232596=CARTESIAN_POINT('Ctrl Pts',(6.09886844428007,-5.03862329405213,
109.422659632429));
#232597=CARTESIAN_POINT('Ctrl Pts',(5.96739194339273,-5.19776555090089,
109.414336986518));
#232598=CARTESIAN_POINT('Ctrl Pts',(5.82975656395019,-5.35167016876399,
109.406014340606));
#232599=CARTESIAN_POINT('Ctrl Pts',(5.68640953515548,-5.49987887125642,
109.397691694694));
#232600=CARTESIAN_POINT('Ctrl Pts',(5.63199664509901,-5.55613719695694,
109.394532513643));
#232601=CARTESIAN_POINT('Ctrl Pts',(5.57676114622288,-5.6115752026096,109.391373332593));
#232602=CARTESIAN_POINT('Ctrl Pts',(5.52072881163614,-5.66616928694957,
109.388214151543));
#232603=CARTESIAN_POINT('Ctrl Pts',(5.36645418003875,-5.81648396348526,
109.379515932983));
#232604=CARTESIAN_POINT('Ctrl Pts',(5.20599955280938,-5.96053179738248,
109.370817714422));
#232605=CARTESIAN_POINT('Ctrl Pts',(5.03987436346788,-6.09783464850099,
109.362119495862));
#232606=CARTESIAN_POINT('Ctrl Pts',(4.87389513737398,-6.23501686065962,
109.353428919853));
#232607=CARTESIAN_POINT('Ctrl Pts',(4.70225547390781,-6.36546577795881,
109.344738343843));
#232608=CARTESIAN_POINT('Ctrl Pts',(4.5254988093669,-6.48874267685341,109.336047767834));
#232609=CARTESIAN_POINT('Ctrl Pts',(4.34450306263844,-6.61497607477224,
109.327148769324));
#232610=CARTESIAN_POINT('Ctrl Pts',(4.15814197773161,-6.73368897836446,
109.318249770815));
#232611=CARTESIAN_POINT('Ctrl Pts',(3.96703473234633,-6.8444544291242,109.309350772305));
#232612=CARTESIAN_POINT('Ctrl Pts',(3.78095329529558,-6.95230692949065,
109.300685802918));
#232613=CARTESIAN_POINT('Ctrl Pts',(3.5903723669843,-7.05262452970903,109.29202083353));
#232614=CARTESIAN_POINT('Ctrl Pts',(3.39589382667509,-7.14505606121814,
109.283355864143));
#232615=CARTESIAN_POINT('Ctrl Pts',(3.19353638223454,-7.24123226900009,
109.274339851072));
#232616=CARTESIAN_POINT('Ctrl Pts',(2.98695913189684,-7.3288699941815,109.265323838002));
#232617=CARTESIAN_POINT('Ctrl Pts',(2.77687127159029,-7.40762491902881,
109.256307824931));
#232618=CARTESIAN_POINT('Ctrl Pts',(2.56678341128373,-7.48637984387611,
109.24729181186));
#232619=CARTESIAN_POINT('Ctrl Pts',(2.35318517926726,-7.55625180730581,
109.23827579879));
#232620=CARTESIAN_POINT('Ctrl Pts',(2.13681410900544,-7.61695125779044,
109.229259785719));
#232621=CARTESIAN_POINT('Ctrl Pts',(1.94937499274639,-7.66953431033291,
109.221449344517));
#232622=CARTESIAN_POINT('Ctrl Pts',(1.7599356938672,-7.71521066824004,109.213638903314));
#232623=CARTESIAN_POINT('Ctrl Pts',(1.56905280285073,-7.75383739201863,
109.205828462112));
#232624=CARTESIAN_POINT('Ctrl Pts',(1.37818367410655,-7.79246133088818,
109.198018584027));
#232625=CARTESIAN_POINT('Ctrl Pts',(1.18587150571842,-7.82403657819675,
109.190208705942));
#232626=CARTESIAN_POINT('Ctrl Pts',(0.992683632893948,-7.84847120176818,
109.182398827856));
#232627=CARTESIAN_POINT('Ctrl Pts',(0.799475589824402,-7.87290837649533,
109.174588134362));
#232628=CARTESIAN_POINT('Ctrl Pts',(0.605392009711438,-7.89020339912728,
109.166777440868));
#232629=CARTESIAN_POINT('Ctrl Pts',(0.411006059568197,-7.90031613411756,
109.158966747373));
#232630=CARTESIAN_POINT('Ctrl Pts',(0.216482162341099,-7.91043604566716,
109.151150510976));
#232631=CARTESIAN_POINT('Ctrl Pts',(0.0216558185147771,-7.91336346825997,
109.14333427458));
#232632=CARTESIAN_POINT('Ctrl Pts',(-0.172898201283247,-7.90911039321067,
109.135518038183));
#232633=CARTESIAN_POINT('Ctrl Pts',(-0.367524150519129,-7.90485574573795,
109.12769891201));
#232634=CARTESIAN_POINT('Ctrl Pts',(-0.561877223508443,-7.89341532807992,
109.119879785837));
#232635=CARTESIAN_POINT('Ctrl Pts',(-0.755386913642639,-7.8748531167697,
109.112060659664));
#232636=CARTESIAN_POINT('Ctrl Pts',(-0.949111780877585,-7.85627026482484,
109.104232838853));
#232637=CARTESIAN_POINT('Ctrl Pts',(-1.14199104230984,-7.83054984194879,
109.096405018041));
#232638=CARTESIAN_POINT('Ctrl Pts',(-1.33346243683517,-7.79780731549258,
109.088577197229));
#232639=CARTESIAN_POINT('Ctrl Pts',(-1.48244058248134,-7.77233133832476,
109.082486604784));
#232640=CARTESIAN_POINT('Ctrl Pts',(-1.63056657031458,-7.74260527241938,
109.076396012339));
#232641=CARTESIAN_POINT('Ctrl Pts',(-1.777581798872,-7.70870442735477,109.070305419894));
#232642=CARTESIAN_POINT('Ctrl Pts',(-1.973510115189,-7.66352451259077,109.062188440892));
#232643=CARTESIAN_POINT('Ctrl Pts',(-2.16785460434176,-7.61083846189063,
109.05407146189));
#232644=CARTESIAN_POINT('Ctrl Pts',(-2.36001930486389,-7.55077677333066,
109.045954482888));
#232645=CARTESIAN_POINT('Ctrl Pts',(-2.55204344357749,-7.49075901781118,
109.037843441174));
#232646=CARTESIAN_POINT('Ctrl Pts',(-2.74189066777205,-7.42337647672191,
109.029732399461));
#232647=CARTESIAN_POINT('Ctrl Pts',(-2.92897782586889,-7.3488101006604,
109.021621357747));
#232648=CARTESIAN_POINT('Ctrl Pts',(-3.11595473668627,-7.27428766529575,
109.013515095732));
#232649=CARTESIAN_POINT('Ctrl Pts',(-3.30017452750284,-7.19258995484459,
109.005408833718));
#232650=CARTESIAN_POINT('Ctrl Pts',(-3.48107121657821,-7.10394708490363,
108.997302571703));
#232651=CARTESIAN_POINT('Ctrl Pts',(-3.66188699913664,-7.0153438607179,
108.989199935235));
#232652=CARTESIAN_POINT('Ctrl Pts',(-3.83938235646557,-6.91980181257971,
108.981097298767));
#232653=CARTESIAN_POINT('Ctrl Pts',(-4.01301270567199,-6.81759855257811,
108.9729946623));
#232654=CARTESIAN_POINT('Ctrl Pts',(-4.18659003868377,-6.71542649926331,
108.964894499886));
#232655=CARTESIAN_POINT('Ctrl Pts',(-4.35630444132098,-6.6065974533241,
108.956794337473));
#232656=CARTESIAN_POINT('Ctrl Pts',(-4.52163679432532,-6.4914344870917,
108.94869417506));
#232657=CARTESIAN_POINT('Ctrl Pts',(-4.68857956518314,-6.37514977733172,
108.940515113109));
#232658=CARTESIAN_POINT('Ctrl Pts',(-4.85105417908357,-6.25240726675152,
108.932336051159));
#232659=CARTESIAN_POINT('Ctrl Pts',(-5.00855630989213,-6.12358430093354,
108.924156989208));
#232660=CARTESIAN_POINT('Ctrl Pts',(-5.16453823650683,-5.99600472916932,
108.916056871232));
#232661=CARTESIAN_POINT('Ctrl Pts',(-5.31564300692924,-5.86246178414278,
108.907956753257));
#232662=CARTESIAN_POINT('Ctrl Pts',(-5.46141390999176,-5.7233625696568,
108.899856635281));
#232663=CARTESIAN_POINT('Ctrl Pts',(-5.60720443125477,-5.58424463486231,
108.891755427172));
#232664=CARTESIAN_POINT('Ctrl Pts',(-5.74765942142636,-5.43956916075739,
108.883654219063));
#232665=CARTESIAN_POINT('Ctrl Pts',(-5.8823585729667,-5.28978058326101,
108.875553010954));
#232666=CARTESIAN_POINT('Ctrl Pts',(-6.01709324894237,-5.13995250176944,
108.867449666299));
#232667=CARTESIAN_POINT('Ctrl Pts',(-6.14606884454124,-4.98500886612771,
108.859346321645));
#232668=CARTESIAN_POINT('Ctrl Pts',(-6.26890457849071,-4.82542810388656,
108.851242976991));
#232669=CARTESIAN_POINT('Ctrl Pts',(-6.39376923771602,-4.66321148454064,
108.843005786262));
#232670=CARTESIAN_POINT('Ctrl Pts',(-6.51228922049973,-4.49620348422213,
108.834768595533));
#232671=CARTESIAN_POINT('Ctrl Pts',(-6.62410982722081,-4.32493814949031,
108.826531404804));
#232672=CARTESIAN_POINT('Ctrl Pts',(-6.73425670955243,-4.1562363044069,
108.818417507871));
#232673=CARTESIAN_POINT('Ctrl Pts',(-6.83790322830827,-3.9834039747118,
108.810303610938));
#232674=CARTESIAN_POINT('Ctrl Pts',(-6.93475617044715,-3.80697752245075,
108.802189714004));
#232675=CARTESIAN_POINT('Ctrl Pts',(-7.03381668934199,-3.6265297681358,
108.793890876378));
#232676=CARTESIAN_POINT('Ctrl Pts',(-7.12577008698123,-3.44232241763237,
108.785592038751));
#232677=CARTESIAN_POINT('Ctrl Pts',(-7.21035405914674,-3.25495243310038,
108.777293201124));
#232678=CARTESIAN_POINT('Ctrl Pts',(-7.2949380313122,-3.06758244856853,
108.768994363498));
#232679=CARTESIAN_POINT('Ctrl Pts',(-7.37215247684972,-2.87705017327477,
108.760695525871));
#232680=CARTESIAN_POINT('Ctrl Pts',(-7.44178885452139,-2.68397087255454,
108.752396688245));
#232681=CARTESIAN_POINT('Ctrl Pts',(-7.51210891726181,-2.48899593281056,
108.744016373213));
#232682=CARTESIAN_POINT('Ctrl Pts',(-7.57483708588991,-2.29104890570404,
108.735636058181));
#232683=CARTESIAN_POINT('Ctrl Pts',(-7.62972938591883,-2.09072965675782,
108.727255743149));
#232684=CARTESIAN_POINT('Ctrl Pts',(-7.6844870541156,-1.89090172166594,
108.718895982132));
#232685=CARTESIAN_POINT('Ctrl Pts',(-7.73144712293042,-1.68871344245385,
108.710536221115));
#232686=CARTESIAN_POINT('Ctrl Pts',(-7.77041471610678,-1.48478151244931,
108.702176460098));
#232687=CARTESIAN_POINT('Ctrl Pts',(-7.80932420579393,-1.28115365964657,
108.693829164087));
#232688=CARTESIAN_POINT('Ctrl Pts',(-7.84026492959831,-1.07578761402196,
108.685481868076));
#232689=CARTESIAN_POINT('Ctrl Pts',(-7.86309182568463,-0.86931463858117,
108.677134572065));
#232690=CARTESIAN_POINT('Ctrl Pts',(-7.88587227225744,-0.663261806519804,
108.668804261624));
#232691=CARTESIAN_POINT('Ctrl Pts',(-7.90057179809203,-0.456106816128255,
108.660473951183));
#232692=CARTESIAN_POINT('Ctrl Pts',(-7.90709640401639,-0.248490357139009,
108.652143640742));
#232693=CARTESIAN_POINT('Ctrl Pts',(-7.90965814519557,-0.166974379218875,
108.648872929907));
#232694=CARTESIAN_POINT('Ctrl Pts',(-7.91096022151875,-0.0853873852617121,
108.645602219072));
#232695=CARTESIAN_POINT('Ctrl Pts',(-7.91099910237999,-0.00376857307924841,
108.642331508237));
#232696=CARTESIAN_POINT('',(-7.9109999968991,0.000221500451111772,104.648002515785));
#232697=CARTESIAN_POINT('Ctrl Pts',(-7.91099992240033,-0.00110805323541054,
108.640263793438));
#232698=CARTESIAN_POINT('Ctrl Pts',(-7.91103873502507,0.275996567276769,
108.628470434012));
#232699=CARTESIAN_POINT('Ctrl Pts',(-7.89651817900392,0.552923481285257,
108.616947714325));
#232700=CARTESIAN_POINT('Ctrl Pts',(-7.86419060080753,0.859896389659774,
108.604418225675));
#232701=CARTESIAN_POINT('Ctrl Pts',(-7.86070010247159,0.891240440873543,
108.603141580458));
#232702=CARTESIAN_POINT('Ctrl Pts',(-7.85483141328906,0.941221228490136,
108.601109894987));
#232703=CARTESIAN_POINT('Ctrl Pts',(-7.8525741142427,0.959871718574376,
108.600352662609));
#232704=CARTESIAN_POINT('Ctrl Pts',(-7.84858713101809,0.991857786608685,
108.599055460503));
#232705=CARTESIAN_POINT('Ctrl Pts',(-7.8468898438213,1.00519729520292,108.598514913088));
#232706=CARTESIAN_POINT('Ctrl Pts',(-7.84363450499322,1.03027126275294,
108.597499655182));
#232707=CARTESIAN_POINT('Ctrl Pts',(-7.84208411189063,1.042006672573,108.597024810785));
#232708=CARTESIAN_POINT('Ctrl Pts',(-7.83879483978766,1.06648101827162,
108.596035178665));
#232709=CARTESIAN_POINT('Ctrl Pts',(-7.83705123336003,1.07921928699073,
108.595520474955));
#232710=CARTESIAN_POINT('Ctrl Pts',(-7.8329608358385,1.10856980663129,108.594335363788));
#232711=CARTESIAN_POINT('Ctrl Pts',(-7.83059223562941,1.12517896961357,
108.593665333842));
#232712=CARTESIAN_POINT('Ctrl Pts',(-7.82287099903963,1.17811660385707,
108.591531620703));
#232713=CARTESIAN_POINT('Ctrl Pts',(-7.81731822947769,1.21441554684441,
108.590071294421));
#232714=CARTESIAN_POINT('Ctrl Pts',(-7.77186678921918,1.49829794897225,
108.578669750233));
#232715=CARTESIAN_POINT('Ctrl Pts',(-7.72046783173518,1.74390193891802,
108.56892819052));
#232716=CARTESIAN_POINT('Ctrl Pts',(-7.63974451673771,2.05504663766676,
108.556670802049));
#232717=CARTESIAN_POINT('Ctrl Pts',(-7.6210859948363,2.12319602660876,108.553990904865));
#232718=CARTESIAN_POINT('Ctrl Pts',(-7.427318355995,2.79543227659978,108.527580834253));
#232719=CARTESIAN_POINT('Ctrl Pts',(-7.18168134098618,3.37681864169952,
108.505142366302));
#232720=CARTESIAN_POINT('Ctrl Pts',(-6.79114594000115,4.06071716895559,
108.475448713363));
#232721=CARTESIAN_POINT('Ctrl Pts',(-6.70835558352547,4.19607549754085,
108.469381483872));
#232722=CARTESIAN_POINT('Ctrl Pts',(-6.58149380023279,4.39012759383339,
108.460298291023));
#232723=CARTESIAN_POINT('Ctrl Pts',(-6.54058491359736,4.450845933314,108.45739888142));
#232724=CARTESIAN_POINT('Ctrl Pts',(-6.49130915152878,4.52183601243383,
108.453932159361));
#232725=CARTESIAN_POINT('Ctrl Pts',(-6.48375118393902,4.53266654478494,
108.4534011235));
#232726=CARTESIAN_POINT('Ctrl Pts',(-6.47211043316828,4.54925899559632,
108.452584218525));
#232727=CARTESIAN_POINT('Ctrl Pts',(-6.46804697642293,4.55503448708368,
108.452299244677));
#232728=CARTESIAN_POINT('Ctrl Pts',(-6.46094003579209,4.56510707231958,
108.451801138602));
#232729=CARTESIAN_POINT('Ctrl Pts',(-6.45789998108347,4.56940658751058,
108.451588168021));
#232730=CARTESIAN_POINT('Ctrl Pts',(-6.45104300225777,4.57908382450968,
108.451108018865));
#232731=CARTESIAN_POINT('Ctrl Pts',(-6.44722364479174,4.5844598114236,108.450840724202));
#232732=CARTESIAN_POINT('Ctrl Pts',(-6.43696948745215,4.59885502825793,
108.450123481599));
#232733=CARTESIAN_POINT('Ctrl Pts',(-6.43052246923753,4.60786550631417,
108.449672941324));
#232734=CARTESIAN_POINT('Ctrl Pts',(-6.40251233371481,4.64683974470204,
108.447717137723));
#232735=CARTESIAN_POINT('Ctrl Pts',(-6.38075879291021,4.6766655810871,108.446202399004));
#232736=CARTESIAN_POINT('Ctrl Pts',(-6.04550344391281,5.12963369117308,
108.422906836292));
#232737=CARTESIAN_POINT('Ctrl Pts',(-5.69078527475396,5.52050764703951,
108.398612357703));
#232738=CARTESIAN_POINT('Ctrl Pts',(-5.20377896721509,5.95998249015012,
108.368410768895));
#232739=CARTESIAN_POINT('Ctrl Pts',(-5.10547413383884,6.04440577611858,
108.362450626835));
#232740=CARTESIAN_POINT('Ctrl Pts',(-4.90816870987172,6.20560074887935,
108.350797086165));
#232741=CARTESIAN_POINT('Ctrl Pts',(-4.80932894074798,6.28251199023904,
108.345103034362));
#232742=CARTESIAN_POINT('Ctrl Pts',(-4.35446348790882,6.61943367019816,
108.319612266744));
#232743=CARTESIAN_POINT('Ctrl Pts',(-3.97888238939687,6.85177580012234,
108.30054629876));
#232744=CARTESIAN_POINT('Ctrl Pts',(-3.56737078471907,7.06103509720357,
108.28186461619));
#232745=CARTESIAN_POINT('Ctrl Pts',(-3.54885081543075,7.07036129615967,
108.281028164409));
#232746=CARTESIAN_POINT('Ctrl Pts',(-3.52192312336513,7.08378895893593,
108.279818197952));
#232747=CARTESIAN_POINT('Ctrl Pts',(-3.5135445339305,7.08794845569086,108.279442585562));
#232748=CARTESIAN_POINT('Ctrl Pts',(-3.49889094563807,7.09519076764042,
108.278787181001));
#232749=CARTESIAN_POINT('Ctrl Pts',(-3.49261920997549,7.09828013909828,
108.278507152115));
#232750=CARTESIAN_POINT('Ctrl Pts',(-3.48048088232119,7.10423933157402,
108.277966118088));
#232751=CARTESIAN_POINT('Ctrl Pts',(-3.47461481772515,7.10711020888153,
108.277705074956));
#232752=CARTESIAN_POINT('Ctrl Pts',(-3.4606775910403,7.11390976810636,108.277085858546));
#232753=CARTESIAN_POINT('Ctrl Pts',(-3.4526032752741,7.11783198749361,108.276727918619));
#232754=CARTESIAN_POINT('Ctrl Pts',(-3.42410351819002,7.13161626520489,
108.275467293829));
#232755=CARTESIAN_POINT('Ctrl Pts',(-3.40364226453461,7.14140425993823,
108.274567279731));
#232756=CARTESIAN_POINT('Ctrl Pts',(-3.14118878751259,7.2655692271866,108.263086904772));
#232757=CARTESIAN_POINT('Ctrl Pts',(-2.89357510000623,7.36768639682128,
108.252958957398));
#232758=CARTESIAN_POINT('Ctrl Pts',(-2.57932830896192,7.47899063788279,
108.240813946756));
#232759=CARTESIAN_POINT('Ctrl Pts',(-2.51714118479853,7.50014906161037,
108.238443646858));
#232760=CARTESIAN_POINT('Ctrl Pts',(-2.19799388570766,7.60431855984757,
108.226433759326));
#232761=CARTESIAN_POINT('Ctrl Pts',(-1.93716269534709,7.67491023532557,
108.21713528707));
#232762=CARTESIAN_POINT('Ctrl Pts',(-1.38764946739131,7.79382591865973,
108.198080457563));
#232763=CARTESIAN_POINT('Ctrl Pts',(-1.09887246608668,7.83975578017106,
108.188363963765));
#232764=CARTESIAN_POINT('Ctrl Pts',(-0.700385917824278,7.88068088575683,
108.174758441005));
#232765=CARTESIAN_POINT('Ctrl Pts',(-0.592337749857318,7.88953782200925,
108.171048541025));
#232766=CARTESIAN_POINT('Ctrl Pts',(-0.314452245628844,7.90657600209386,
108.161387492466));
#232767=CARTESIAN_POINT('Ctrl Pts',(-0.144475853018282,7.91150723820138,
108.155363818877));
#232768=CARTESIAN_POINT('Ctrl Pts',(0.187106768751399,7.91043756433375,
108.143183952302));
#232769=CARTESIAN_POINT('Ctrl Pts',(0.348630174924865,7.90496568590167,
108.137051732549));
#232770=CARTESIAN_POINT('Ctrl Pts',(0.534418261830269,7.89296671673951,
108.129659991877));
#232771=CARTESIAN_POINT('Ctrl Pts',(0.558965607863358,7.8912663047917,108.12867653007));
#232772=CARTESIAN_POINT('Ctrl Pts',(0.590338561631365,7.88894595903172,
108.127410452302));
#232773=CARTESIAN_POINT('Ctrl Pts',(0.597172087466627,7.88843162227037,
108.127134124868));
#232774=CARTESIAN_POINT('Ctrl Pts',(0.608136860096736,7.88759201103033,
108.126689838761));
#232775=CARTESIAN_POINT('Ctrl Pts',(0.612268548044961,7.88727236742977,
108.126522219328));
#232776=CARTESIAN_POINT('Ctrl Pts',(0.620106816447516,7.88665977209606,
108.126203833095));
#232777=CARTESIAN_POINT('Ctrl Pts',(0.62381344674858,7.88636745328055,108.126053104729));
#232778=CARTESIAN_POINT('Ctrl Pts',(0.632225982206083,7.8856980410878,108.125710631178));
#232779=CARTESIAN_POINT('Ctrl Pts',(0.636931727599009,7.88531935067549,
108.125518789118));
#232780=CARTESIAN_POINT('Ctrl Pts',(0.649162501104753,7.88432407076801,
108.12501946115));
#232781=CARTESIAN_POINT('Ctrl Pts',(0.656686931967718,7.88370092521737,
108.124711576769));
#232782=CARTESIAN_POINT('Ctrl Pts',(0.703284094136714,7.87977474760893,
108.12280066378));
#232783=CARTESIAN_POINT('Ctrl Pts',(0.742332056170847,7.87619207484784,
108.121180818793));
#232784=CARTESIAN_POINT('Ctrl Pts',(1.41346791099696,7.80957984843392,108.093042480294));
#232785=CARTESIAN_POINT('Ctrl Pts',(2.03569442888879,7.67093968598267,108.062612667835));
#232786=CARTESIAN_POINT('Ctrl Pts',(2.96431042009534,7.34295900447116,108.016850928095));
#232787=CARTESIAN_POINT('Ctrl Pts',(3.28594820497965,7.20477357306866,108.000888183592));
#232788=CARTESIAN_POINT('Ctrl Pts',(3.76235179774446,6.96153204860795,107.977525606507));
#232789=CARTESIAN_POINT('Ctrl Pts',(3.92429314252192,6.871546360986,107.969631878361));
#232790=CARTESIAN_POINT('Ctrl Pts',(4.1608200758466,6.7290241366952,107.958185208574));
#232791=CARTESIAN_POINT('Ctrl Pts',(4.2378917494425,6.68075323887232,107.954468582145));
#232792=CARTESIAN_POINT('Ctrl Pts',(4.32703034228173,6.6227612661145,107.95018390057));
#232793=CARTESIAN_POINT('Ctrl Pts',(4.33992015838255,6.61432168809432,107.949564657672));
#232794=CARTESIAN_POINT('Ctrl Pts',(4.35953318542118,6.60139808750223,107.948622924706));
#232795=CARTESIAN_POINT('Ctrl Pts',(4.36627427855076,6.59694135410258,107.948299337124));
#232796=CARTESIAN_POINT('Ctrl Pts',(4.37797530973959,6.5891796690172,107.947737815821));
#232797=CARTESIAN_POINT('Ctrl Pts',(4.38293835716385,6.58587943108554,107.94749969231));
#232798=CARTESIAN_POINT('Ctrl Pts',(4.3932653591498,6.57899552352798,107.947004309274));
#232799=CARTESIAN_POINT('Ctrl Pts',(4.39862867085935,6.57541089443683,107.946747088763));
#232800=CARTESIAN_POINT('Ctrl Pts',(4.41333821012827,6.56555355940951,107.946041780672));
#232801=CARTESIAN_POINT('Ctrl Pts',(4.42267546161771,6.55926744851141,107.94559423582));
#232802=CARTESIAN_POINT('Ctrl Pts',(4.45853858813226,6.53501194915719,107.943875898615));
#232803=CARTESIAN_POINT('Ctrl Pts',(4.48496880332076,6.51690128693292,107.942610842156));
#232804=CARTESIAN_POINT('Ctrl Pts',(4.89793005599667,6.23022744570043,107.922863249005));
#232805=CARTESIAN_POINT('Ctrl Pts',(5.25986804256149,5.92784147446614,107.905896997823));
#232806=CARTESIAN_POINT('Ctrl Pts',(5.88870573742271,5.29925640496127,107.875153710368));
#232807=CARTESIAN_POINT('Ctrl Pts',(6.16067256109226,4.98046914351487,107.861257713819));
#232808=CARTESIAN_POINT('Ctrl Pts',(6.5041830885523,4.50637771722822,107.840893692222));
#232809=CARTESIAN_POINT('Ctrl Pts',(6.59790289879245,4.36801000032904,107.834976730553));
#232810=CARTESIAN_POINT('Ctrl Pts',(6.77360042566366,4.09004006785996,107.822931937608));
#232811=CARTESIAN_POINT('Ctrl Pts',(6.85581345453315,3.95068431762628,107.816819418618));
#232812=CARTESIAN_POINT('Ctrl Pts',(6.94897101629516,3.78110166830769,107.809172012608));
#232813=CARTESIAN_POINT('Ctrl Pts',(6.96408210029957,3.75319710018941,107.807907019386));
#232814=CARTESIAN_POINT('Ctrl Pts',(6.98259895475755,3.7185064811697,107.806325246385));
#232815=CARTESIAN_POINT('Ctrl Pts',(6.98616351772885,3.71180520990043,107.806019272557));
#232816=CARTESIAN_POINT('Ctrl Pts',(6.99179952197368,3.7011728126672,107.805533156125));
#232817=CARTESIAN_POINT('Ctrl Pts',(6.99387731307706,3.69724503842611,107.805353436468));
#232818=CARTESIAN_POINT('Ctrl Pts',(6.99777107736904,3.68986939258878,107.805015694776));
#232819=CARTESIAN_POINT('Ctrl Pts',(6.99958781534629,3.6864219238682,107.804857723265));
#232820=CARTESIAN_POINT('Ctrl Pts',(7.00364775616464,3.67870389909681,107.804503827751));
#232821=CARTESIAN_POINT('Ctrl Pts',(7.0058896000552,3.67443263393524,107.804307814972));
#232822=CARTESIAN_POINT('Ctrl Pts',(7.01154737807487,3.6636291711,107.803811628789));
#232823=CARTESIAN_POINT('Ctrl Pts',(7.0149580844537,3.65709425787,107.803511117356));
#232824=CARTESIAN_POINT('Ctrl Pts',(7.03325238932924,3.62192261280943,107.801891764651));
#232825=CARTESIAN_POINT('Ctrl Pts',(7.04796958381711,3.59320014377403,107.800562339287));
#232826=CARTESIAN_POINT('Ctrl Pts',(7.12749364942584,3.43563048217298,107.793234334793));
#232827=CARTESIAN_POINT('Ctrl Pts',(7.18894028813037,3.30512567014109,107.787038317953));
#232828=CARTESIAN_POINT('Ctrl Pts',(7.4183074295358,2.78127997775518,107.76188067631));
#232829=CARTESIAN_POINT('Ctrl Pts',(7.55777777231555,2.37629257217556,107.741836642829));
#232830=CARTESIAN_POINT('Ctrl Pts',(7.77977682550361,1.50915383640564,107.70008038683));
#232831=CARTESIAN_POINT('Ctrl Pts',(7.85535940108023,1.0468406587608,107.678493895438));
#232832=CARTESIAN_POINT('Ctrl Pts',(7.90997527459674,0.304581900445095,
107.646009680833));
#232833=CARTESIAN_POINT('Ctrl Pts',(7.91578989370547,0.0277468338463155,
107.634351180613));
#232834=CARTESIAN_POINT('Ctrl Pts',(7.9064400872044,-0.269345212587889,
107.622317401591));
#232835=CARTESIAN_POINT('Ctrl Pts',(7.90571517811777,-0.289843452246066,
107.621489507664));
#232836=CARTESIAN_POINT('Ctrl Pts',(7.90453573154146,-0.319886171443628,
107.620279588133));
#232837=CARTESIAN_POINT('Ctrl Pts',(7.90414361179751,-0.329432935214876,
107.619895620958));
#232838=CARTESIAN_POINT('Ctrl Pts',(7.90342273555931,-0.346241098539175,
107.619220499723));
#232839=CARTESIAN_POINT('Ctrl Pts',(7.90310126553972,-0.353502789597305,
107.618929119408));
#232840=CARTESIAN_POINT('Ctrl Pts',(7.90245581468323,-0.367641808360402,
107.618362352575));
#232841=CARTESIAN_POINT('Ctrl Pts',(7.90213286333426,-0.374519175480841,
107.618086934321));
#232842=CARTESIAN_POINT('Ctrl Pts',(7.90124490809039,-0.392915916150992,
107.617350899372));
#232843=CARTESIAN_POINT('Ctrl Pts',(7.90066369005516,-0.40443450998918,
107.616890786659));
#232844=CARTESIAN_POINT('Ctrl Pts',(7.89847412950154,-0.446020224598346,
107.615232264973));
#232845=CARTESIAN_POINT('Ctrl Pts',(7.89671931283085,-0.47607954669343,
107.614038402662));
#232846=CARTESIAN_POINT('Ctrl Pts',(7.86571194561248,-0.959744910370648,
107.594906568759));
#232847=CARTESIAN_POINT('Ctrl Pts',(7.7975888032411,-1.41003513985752,107.578264325206));
#232848=CARTESIAN_POINT('Ctrl Pts',(7.58725278814174,-2.28353343489317,
107.546570453044));
#232849=CARTESIAN_POINT('Ctrl Pts',(7.44721451720778,-2.70553365907301,
107.531531091355));
#232850=CARTESIAN_POINT('Ctrl Pts',(7.20643314004819,-3.26794230015215,
107.509857433568));
#232851=CARTESIAN_POINT('Ctrl Pts',(7.13543824782143,-3.42018172434063,
107.503809955386));
#232852=CARTESIAN_POINT('Ctrl Pts',(7.00605114640692,-3.67604102710862,
107.493171890933));
#232853=CARTESIAN_POINT('Ctrl Pts',(6.95006750951079,-3.78081892361137,
107.488673223691));
#232854=CARTESIAN_POINT('Ctrl Pts',(6.85431285779781,-3.95071240251598,
107.481089960115));
#232855=CARTESIAN_POINT('Ctrl Pts',(6.81592269819971,-4.01658194226487,
107.478078882162));
#232856=CARTESIAN_POINT('Ctrl Pts',(6.76897605576573,-4.09452094408914,
107.474438564009));
#232857=CARTESIAN_POINT('Ctrl Pts',(6.76132936770407,-4.10713571521006,
107.473846908367));
#232858=CARTESIAN_POINT('Ctrl Pts',(6.74946852356746,-4.12657970302851,
107.472931225491));
#232859=CARTESIAN_POINT('Ctrl Pts',(6.74527916281771,-4.13342405412287,
107.47260818683));
#232860=CARTESIAN_POINT('Ctrl Pts',(6.73760441535231,-4.14591990148936,
107.472017115026));
#232861=CARTESIAN_POINT('Ctrl Pts',(6.7341223107259,-4.15157341151867,107.471749210262));
#232862=CARTESIAN_POINT('Ctrl Pts',(6.72649503477134,-4.16392213611211,
107.471162984036));
#232863=CARTESIAN_POINT('Ctrl Pts',(6.722346978254,-4.17061555551253,107.47084455181));
#232864=CARTESIAN_POINT('Ctrl Pts',(6.71095974935212,-4.18892918029538,
107.469971460658));
#232865=CARTESIAN_POINT('Ctrl Pts',(6.70370041068931,-4.20053677953207,
107.469416042334));
#232866=CARTESIAN_POINT('Ctrl Pts',(6.66797846229726,-4.25732731242629,
107.466688836095));
#232867=CARTESIAN_POINT('Ctrl Pts',(6.63908929562512,-4.30223962712991,
107.464501566807));
#232868=CARTESIAN_POINT('Ctrl Pts',(6.58888862297852,-4.37857384122342,
107.460735000138));
#232869=CARTESIAN_POINT('Ctrl Pts',(6.56780135620763,-4.41014143448753,
107.45916277701));
#232870=CARTESIAN_POINT('Ctrl Pts',(6.20055389179387,-4.95143398638683,
107.431963150861));
#232871=CARTESIAN_POINT('Ctrl Pts',(5.79623539046615,-5.41915562713048,
107.404994415516));
#232872=CARTESIAN_POINT('Ctrl Pts',(4.83576913553289,-6.29839676295077,
107.349534007919));
#232873=CARTESIAN_POINT('Ctrl Pts',(4.27168591407825,-6.69381927325144,
107.321238455584));
#232874=CARTESIAN_POINT('Ctrl Pts',(3.61329227770282,-7.03784573737825,
107.291112721341));
#232875=CARTESIAN_POINT('Ctrl Pts',(3.56261742480398,-7.06363297806015,
107.288812973398));
#232876=CARTESIAN_POINT('Ctrl Pts',(3.48806994162967,-7.10056213624238,
107.285457312797));
#232877=CARTESIAN_POINT('Ctrl Pts',(3.46441283942842,-7.11213457776606,
107.284396424292));
#232878=CARTESIAN_POINT('Ctrl Pts',(3.42258077192787,-7.13233949573637,
107.282527506461));
#232879=CARTESIAN_POINT('Ctrl Pts',(3.40442985449154,-7.14102115886371,
107.28171889948));
#232880=CARTESIAN_POINT('Ctrl Pts',(3.36647713574723,-7.1589965196296,107.280032940486));
#232881=CARTESIAN_POINT('Ctrl Pts',(3.34666950340663,-7.16827752755352,
107.279155747152));
#232882=CARTESIAN_POINT('Ctrl Pts',(3.29491923141385,-7.19226423531588,
107.276870967726));
#232883=CARTESIAN_POINT('Ctrl Pts',(3.26291652864971,-7.20683934286083,
107.275464984431));
#232884=CARTESIAN_POINT('Ctrl Pts',(3.13137239188303,-7.26569314518026,
107.269713769935));
#232885=CARTESIAN_POINT('Ctrl Pts',(3.03101787363149,-7.30812705245861,
107.265391631183));
#232886=CARTESIAN_POINT('Ctrl Pts',(2.54191271345103,-7.50313201839154,
107.244618304176));
#232887=CARTESIAN_POINT('Ctrl Pts',(2.14236799683754,-7.62683289746065,
107.228566496144));
#232888=CARTESIAN_POINT('Ctrl Pts',(1.38380201505628,-7.79734104755768,
107.19869571647));
#232889=CARTESIAN_POINT('Ctrl Pts',(1.02771569940745,-7.85221115989053,
107.184898193211));
#232890=CARTESIAN_POINT('Ctrl Pts',(0.636243390613084,-7.885442646872,107.169290064976));
#232891=CARTESIAN_POINT('Ctrl Pts',(0.603323693710573,-7.88802965806492,
107.167974041639));
#232892=CARTESIAN_POINT('Ctrl Pts',(0.545574648575651,-7.89220427193122,
107.165658296055));
#232893=CARTESIAN_POINT('Ctrl Pts',(0.520752102115117,-7.89388099804546,
107.164660592043));
#232894=CARTESIAN_POINT('Ctrl Pts',(0.483553537086185,-7.89621748438922,
107.163161668438));
#232895=CARTESIAN_POINT('Ctrl Pts',(0.471183228782001,-7.8969652998838,
107.162662589451));
#232896=CARTESIAN_POINT('Ctrl Pts',(0.449699379641437,-7.89821339127977,
107.161794789531));
#232897=CARTESIAN_POINT('Ctrl Pts',(0.440586622502075,-7.89872696918875,
107.161426373192));
#232898=CARTESIAN_POINT('Ctrl Pts',(0.421614874633604,-7.89976324773733,
107.160658712896));
#232899=CARTESIAN_POINT('Ctrl Pts',(0.411755754750705,-7.90028326521258,
107.160259409931));
#232900=CARTESIAN_POINT('Ctrl Pts',(0.387650715497898,-7.90150943602075,
107.159282252419));
#232901=CARTESIAN_POINT('Ctrl Pts',(0.373403826394887,-7.90219551930367,
107.15870396621));
#232902=CARTESIAN_POINT('Ctrl Pts',(0.318793541002406,-7.90467735621073,
107.156484532693));
#232903=CARTESIAN_POINT('Ctrl Pts',(0.278418668647009,-7.90620240274193,
107.154837821285));
#232904=CARTESIAN_POINT('Ctrl Pts',(-0.204184554541389,-7.92073003251255,
107.135092149863));
#232905=CARTESIAN_POINT('Ctrl Pts',(-0.64673452237051,-7.89692217675445,
107.11639802416));
#232906=CARTESIAN_POINT('Ctrl Pts',(-1.52627019509153,-7.77514674138457,
107.079150398024));
#232907=CARTESIAN_POINT('Ctrl Pts',(-1.96164221014638,-7.67687388076254,
107.06067053362));
#232908=CARTESIAN_POINT('Ctrl Pts',(-2.43873907987548,-7.52592070714098,
107.040373534423));
#232909=CARTESIAN_POINT('Ctrl Pts',(-2.49087158751566,-7.50882744353128,
107.038154318542));
#232910=CARTESIAN_POINT('Ctrl Pts',(-2.57035493869958,-7.48184749096272,
107.034767813482));
#232911=CARTESIAN_POINT('Ctrl Pts',(-2.59783590945898,-7.47235003088363,
107.033596391875));
#232912=CARTESIAN_POINT('Ctrl Pts',(-2.64576447948011,-7.45548949433536,
107.031552206265));
#232913=CARTESIAN_POINT('Ctrl Pts',(-2.66623523094143,-7.44819326933813,
107.030678745979));
#232914=CARTESIAN_POINT('Ctrl Pts',(-2.71246395269402,-7.4315013316775,
107.028705285011));
#232915=CARTESIAN_POINT('Ctrl Pts',(-2.73820368409924,-7.42205586935601,
107.027605816433));
#232916=CARTESIAN_POINT('Ctrl Pts',(-2.80809453530494,-7.39599563343376,
107.024618356802));
#232917=CARTESIAN_POINT('Ctrl Pts',(-2.8521470691761,-7.37911942267261,
107.022733079687));
#232918=CARTESIAN_POINT('Ctrl Pts',(-3.07346578284434,-7.29205581791694,
107.013247174728));
#232919=CARTESIAN_POINT('Ctrl Pts',(-3.24830584242651,-7.21587002555126,
107.005706037657));
#232920=CARTESIAN_POINT('Ctrl Pts',(-3.77951932133691,-6.96117266607116,
106.982517896535));
#232921=CARTESIAN_POINT('Ctrl Pts',(-4.12529559172205,-6.76200026881434,
106.967113041625));
#232922=CARTESIAN_POINT('Ctrl Pts',(-4.86171080274688,-6.26022164824975,
106.933419392483));
#232923=CARTESIAN_POINT('Ctrl Pts',(-5.24200821832247,-5.94541369153949,
106.915415277217));
#232924=CARTESIAN_POINT('Ctrl Pts',(-5.76934720705291,-5.41870947773786,
106.887452742756));
#232925=CARTESIAN_POINT('Ctrl Pts',(-5.93947616884499,-5.2316719454731,
106.877841336039));
#232926=CARTESIAN_POINT('Ctrl Pts',(-6.11595503219677,-5.01792939687397,
106.866864840891));
#232927=CARTESIAN_POINT('Ctrl Pts',(-6.1314676699316,-4.99896245089779,
106.865890824048));
#232928=CARTESIAN_POINT('Ctrl Pts',(-6.15837983118452,-4.96574384173874,
106.864184421783));
#232929=CARTESIAN_POINT('Ctrl Pts',(-6.1698186627513,-4.9515241803991,106.863453810908));
#232930=CARTESIAN_POINT('Ctrl Pts',(-6.18634520589159,-4.93083377791806,
106.862390311236));
#232931=CARTESIAN_POINT('Ctrl Pts',(-6.19147222782832,-4.92439441995835,
106.862059265456));
#232932=CARTESIAN_POINT('Ctrl Pts',(-6.20041443411364,-4.91312728395238,
106.861479901779));
#232933=CARTESIAN_POINT('Ctrl Pts',(-6.20423405847917,-4.90830302756795,
106.861231795986));
#232934=CARTESIAN_POINT('Ctrl Pts',(-6.21161085229062,-4.89896363118827,
106.860751396426));
#232935=CARTESIAN_POINT('Ctrl Pts',(-6.2151687374642,-4.89444906037574,
106.860519137558));
#232936=CARTESIAN_POINT('Ctrl Pts',(-6.22360565992347,-4.88371948632657,
106.859967037557));
#232937=CARTESIAN_POINT('Ctrl Pts',(-6.22848030713842,-4.87750105016458,
106.859646981988));
#232938=CARTESIAN_POINT('Ctrl Pts',(-6.24564908641879,-4.85553166274263,
106.858515923529));
#232939=CARTESIAN_POINT('Ctrl Pts',(-6.25789278847942,-4.83974152993287,
106.857702414895));
#232940=CARTESIAN_POINT('Ctrl Pts',(-6.39663409473134,-4.65940660462988,
106.848403022673));
#232941=CARTESIAN_POINT('Ctrl Pts',(-6.51664717035395,-4.49002052532004,
106.839541008427));
#232942=CARTESIAN_POINT('Ctrl Pts',(-7.01202511022542,-3.72908808634762,
106.799567769173));
#232943=CARTESIAN_POINT('Ctrl Pts',(-7.31454443108464,-3.09388440706398,
106.766224853787));
#232944=CARTESIAN_POINT('Ctrl Pts',(-7.65456465755592,-2.03906803536624,
106.716724569656));
#232945=CARTESIAN_POINT('Ctrl Pts',(-7.74947821176049,-1.64189127308883,
106.699223689447));
#232946=CARTESIAN_POINT('Ctrl Pts',(-7.8170113916222,-1.21605898354082,
106.681733974598));
#232947=CARTESIAN_POINT('Ctrl Pts',(-7.82056771317408,-1.19297410010201,
106.680789590397));
#232948=CARTESIAN_POINT('Ctrl Pts',(-7.82554619124114,-1.15967843630591,
106.679432848613));
#232949=CARTESIAN_POINT('Ctrl Pts',(-7.82705069238963,-1.1494801984557,
106.679018011163));
#232950=CARTESIAN_POINT('Ctrl Pts',(-7.82963189998488,-1.13174347704899,
106.678297779692));
#232951=CARTESIAN_POINT('Ctrl Pts',(-7.83071766183087,-1.1242063370153,
106.677992113259));
#232952=CARTESIAN_POINT('Ctrl Pts',(-7.83278765151611,-1.10968838254856,
106.677404095344));
#232953=CARTESIAN_POINT('Ctrl Pts',(-7.83377343359339,-1.10270779970503,
106.677121697347));
#232954=CARTESIAN_POINT('Ctrl Pts',(-7.83607844635828,-1.08622630689846,
106.676455730402));
#232955=CARTESIAN_POINT('Ctrl Pts',(-7.83738973243673,-1.07672428689971,
106.676072400833));
#232956=CARTESIAN_POINT('Ctrl Pts',(-7.84188612439639,-1.04369848310175,
106.674742213561));
#232957=CARTESIAN_POINT('Ctrl Pts',(-7.84498264260371,-1.0201626639204,
106.673798021626));
#232958=CARTESIAN_POINT('Ctrl Pts',(-7.88029792735005,-0.742067385307632,
106.662685436911));
#232959=CARTESIAN_POINT('Ctrl Pts',(-7.90022083930181,-0.48608988570781,
106.6528967295));
#232960=CARTESIAN_POINT('Ctrl Pts',(-7.90988634133631,-0.153173819004711,
106.64059170563));
#232961=CARTESIAN_POINT('Ctrl Pts',(-7.91099715275511,-0.0767364826541508,
106.637794989213));
#232962=CARTESIAN_POINT('Ctrl Pts',(-7.91102938135051,0.790196293314509,
106.606350262785));
#232963=CARTESIAN_POINT('Ctrl Pts',(-7.79258590487049,1.57613321728681,
106.58086546829));
#232964=CARTESIAN_POINT('Ctrl Pts',(-7.50519677351402,2.5080075256058,106.544753891518));
#232965=CARTESIAN_POINT('Ctrl Pts',(-7.44455740994452,2.68265623579281,
106.537691872609));
#232966=CARTESIAN_POINT('Ctrl Pts',(-7.3727793296357,2.86814294067703,106.529744565052));
#232967=CARTESIAN_POINT('Ctrl Pts',(-7.3676665108513,2.88125131716837,106.529180605833));
#232968=CARTESIAN_POINT('Ctrl Pts',(-7.3600084237171,2.90073164601198,106.528339125464));
#232969=CARTESIAN_POINT('Ctrl Pts',(-7.35748977246574,2.90711408909429,
106.528062885616));
#232970=CARTESIAN_POINT('Ctrl Pts',(-7.35315863246845,2.91804782778047,
106.527588742163));
#232971=CARTESIAN_POINT('Ctrl Pts',(-7.35135021106269,2.92260073797181,
106.52739103125));
#232972=CARTESIAN_POINT('Ctrl Pts',(-7.34781997390163,2.93146451102109,
106.527005592267));
#232973=CARTESIAN_POINT('Ctrl Pts',(-7.34609858995707,2.93577554569997,
106.526817884429));
#232974=CARTESIAN_POINT('Ctrl Pts',(-7.34196621085253,2.94609828625504,
106.526367840101));
#232975=CARTESIAN_POINT('Ctrl Pts',(-7.33955162717348,2.95210854564664,
106.526105337571));
#232976=CARTESIAN_POINT('Ctrl Pts',(-7.33226968124424,2.97017023923109,
106.525315077434));
#232977=CARTESIAN_POINT('Ctrl Pts',(-7.32738001305489,2.98221261314124,
106.524786303965));
#232978=CARTESIAN_POINT('Ctrl Pts',(-7.28341895743385,3.08971995996512,
106.520049261661));
#232979=CARTESIAN_POINT('Ctrl Pts',(-7.24251460184595,3.18442179584331,
106.515760472332));
#232980=CARTESIAN_POINT('Ctrl Pts',(-7.11836742029221,3.45707317657846,
106.503127241869));
#232981=CARTESIAN_POINT('Ctrl Pts',(-7.03033483765897,3.63275336009474,
106.494629001122));
#232982=CARTESIAN_POINT('Ctrl Pts',(-6.69432060971354,4.24525435998921,
106.464094987481));
#232983=CARTESIAN_POINT('Ctrl Pts',(-6.41138994498458,4.66157014886894,
106.441741829819));
#232984=CARTESIAN_POINT('Ctrl Pts',(-5.87827101674219,5.30479762552317,
106.405964457483));
#232985=CARTESIAN_POINT('Ctrl Pts',(-5.64963788844624,5.5476627118158,106.392075004085));
#232986=CARTESIAN_POINT('Ctrl Pts',(-5.37958556859561,5.80045902386594,
106.377097101586));
#232987=CARTESIAN_POINT('Ctrl Pts',(-5.35263982014906,5.8253337037841,106.375616971292));
#232988=CARTESIAN_POINT('Ctrl Pts',(-5.31314392962237,5.86128849073682,
106.373467815168));
#232989=CARTESIAN_POINT('Ctrl Pts',(-5.30073015043904,5.87251743831149,
106.372795215984));
#232990=CARTESIAN_POINT('Ctrl Pts',(-5.2787226818941,5.89229776978474,106.371607859246));
#232991=CARTESIAN_POINT('Ctrl Pts',(-5.26914363052744,5.90086532316607,
106.371092723231));
#232992=CARTESIAN_POINT('Ctrl Pts',(-5.24924849801795,5.91857256095623,
106.37002625383));
#232993=CARTESIAN_POINT('Ctrl Pts',(-5.23892932179173,5.92770870706984,
106.369475003028));
#232994=CARTESIAN_POINT('Ctrl Pts',(-5.21231740947151,5.95114595639587,
106.368058232583));
#232995=CARTESIAN_POINT('Ctrl Pts',(-5.19598964395698,5.96540716099233,
106.367193614298));
#232996=CARTESIAN_POINT('Ctrl Pts',(-5.12989719699649,6.02265724473699,
106.363712111768));
#232997=CARTESIAN_POINT('Ctrl Pts',(-5.07965541254064,6.06509246355605,
106.361107051081));
#232998=CARTESIAN_POINT('Ctrl Pts',(-4.76329969222687,6.32560418624132,
106.344955672411));
#232999=CARTESIAN_POINT('Ctrl Pts',(-4.48371817320108,6.52675881440461,
106.331798129946));
#233000=CARTESIAN_POINT('Ctrl Pts',(-3.58102953646378,7.09077010431463,
106.291937392995));
#233001=CARTESIAN_POINT('Ctrl Pts',(-2.92093090641103,7.38720445521934,
106.266584319917));
#233002=CARTESIAN_POINT('Ctrl Pts',(-2.15652665017984,7.61177809132325,
106.235417926028));
#233003=CARTESIAN_POINT('Ctrl Pts',(-2.08282331128198,7.63227485800151,
106.23239195626));
#233004=CARTESIAN_POINT('Ctrl Pts',(-1.99635611025489,7.6549754903757,106.228807945466));
#233005=CARTESIAN_POINT('Ctrl Pts',(-1.98386846629955,7.65822129369446,
106.228289515305));
#233006=CARTESIAN_POINT('Ctrl Pts',(-1.96390478998727,7.66335817005293,
106.227459332426));
#233007=CARTESIAN_POINT('Ctrl Pts',(-1.95643380733656,7.66526889441129,
106.227148345312));
#233008=CARTESIAN_POINT('Ctrl Pts',(-1.94322459476225,7.66862661729123,
106.226597937897));
#233009=CARTESIAN_POINT('Ctrl Pts',(-1.93748750576447,7.67007810819928,
106.22635869551));
#233010=CARTESIAN_POINT('Ctrl Pts',(-1.92560447395457,7.6730703474208,106.22586276639));
#233011=CARTESIAN_POINT('Ctrl Pts',(-1.9194582994686,7.67461015184991,106.225606042095));
#233012=CARTESIAN_POINT('Ctrl Pts',(-1.90368193109016,7.67854247693966,
106.224946494069));
#233013=CARTESIAN_POINT('Ctrl Pts',(-1.8940490910787,7.68092426107118,106.224543235584));
#233014=CARTESIAN_POINT('Ctrl Pts',(-1.85445816777126,7.69063437540362,
106.222883522267));
#233015=CARTESIAN_POINT('Ctrl Pts',(-1.82446210215475,7.69780554392879,
106.221620580557));
#233016=CARTESIAN_POINT('Ctrl Pts',(-1.63459563038937,7.74202487858123,
106.213588539659));
#233017=CARTESIAN_POINT('Ctrl Pts',(-1.47367156421402,7.77426092177394,
106.206586974652));
#233018=CARTESIAN_POINT('Ctrl Pts',(-1.20709355409295,7.81908785293875,
106.194742855578));
#233019=CARTESIAN_POINT('Ctrl Pts',(-1.10197456548786,7.83459383796254,
106.190014529623));
#233020=CARTESIAN_POINT('Ctrl Pts',(-0.702892945268238,7.88527135087547,
106.171921255509));
#233021=CARTESIAN_POINT('Ctrl Pts',(-0.40735150003555,7.90604966999354,
106.158239887809));
#233022=CARTESIAN_POINT('Ctrl Pts',(0.525300154104513,7.9191780831024,106.11532311649));
#233023=CARTESIAN_POINT('Ctrl Pts',(1.1607973920164,7.85124920709851,106.08668483371));
#233024=CARTESIAN_POINT('Ctrl Pts',(1.8142596067873,7.7002288587693,106.059319162972));
#233025=CARTESIAN_POINT('Ctrl Pts',(1.84712776248553,7.69241064072372,106.057947622848));
#233026=CARTESIAN_POINT('Ctrl Pts',(1.89455480527723,7.68080785516156,106.05597558122));
#233027=CARTESIAN_POINT('Ctrl Pts',(1.90915433449321,7.67719199633291,106.055369488809));
#233028=CARTESIAN_POINT('Ctrl Pts',(1.93251613700216,7.67133522771092,106.054401167716));
#233029=CARTESIAN_POINT('Ctrl Pts',(1.94128499780341,7.6691208983641,106.054038054395));
#233030=CARTESIAN_POINT('Ctrl Pts',(1.95680196831877,7.66517420508086,106.053396116162));
#233031=CARTESIAN_POINT('Ctrl Pts',(1.96355161491631,7.66344795724127,106.053117087429));
#233032=CARTESIAN_POINT('Ctrl Pts',(1.97754727053993,7.65984881083601,106.05253893333));
#233033=CARTESIAN_POINT('Ctrl Pts',(1.98479292159966,7.65797454101705,106.052239854154));
#233034=CARTESIAN_POINT('Ctrl Pts',(2.0034281351389,7.65312585001196,106.051471250138));
#233035=CARTESIAN_POINT('Ctrl Pts',(2.01481375722863,7.6501362794441,106.051002233295));
#233036=CARTESIAN_POINT('Ctrl Pts',(2.06193104225221,7.6376520131301,106.049063677032));
#233037=CARTESIAN_POINT('Ctrl Pts',(2.09760287671754,7.62793223077538,106.047601706348));
#233038=CARTESIAN_POINT('Ctrl Pts',(2.6927296947057,7.46128296862159,106.023303392563));
#233039=CARTESIAN_POINT('Ctrl Pts',(3.23329596615774,7.24344069571108,106.002787542959));
#233040=CARTESIAN_POINT('Ctrl Pts',(4.28225978382236,6.67966685589333,105.962405803492));
#233041=CARTESIAN_POINT('Ctrl Pts',(4.78411066943029,6.32991630018231,105.942707858317));
#233042=CARTESIAN_POINT('Ctrl Pts',(5.34797797119683,5.83125500655345,105.914651969039));
#233043=CARTESIAN_POINT('Ctrl Pts',(5.45258717427359,5.73355841250004,105.909149629697));
#233044=CARTESIAN_POINT('Ctrl Pts',(5.56320027988232,5.62448873297047,105.902929287309));
#233045=CARTESIAN_POINT('Ctrl Pts',(5.57189712225385,5.61587333520914,105.902437435402));
#233046=CARTESIAN_POINT('Ctrl Pts',(5.58400324881667,5.60382477658801,105.901748820162));
#233047=CARTESIAN_POINT('Ctrl Pts',(5.58742947392514,5.60040858180962,105.901553487847));
#233048=CARTESIAN_POINT('Ctrl Pts',(5.59334089972586,5.59450363746438,105.901215701231));
#233049=CARTESIAN_POINT('Ctrl Pts',(5.59582758202459,5.59201636642067,105.901073372909));
#233050=CARTESIAN_POINT('Ctrl Pts',(5.60097058972605,5.58686527536336,105.900778515686));
#233051=CARTESIAN_POINT('Ctrl Pts',(5.60362667471784,5.58420121792964,105.90062596638));
#233052=CARTESIAN_POINT('Ctrl Pts',(5.60976505086272,5.578035627464,105.900272784378));
#233053=CARTESIAN_POINT('Ctrl Pts',(5.61324593990732,5.57453275216906,105.900072034171));
#233054=CARTESIAN_POINT('Ctrl Pts',(5.62445523817989,5.56323150840667,105.899424049908));
#233055=CARTESIAN_POINT('Ctrl Pts',(5.63217064158063,5.55542036249916,105.898975709172));
#233056=CARTESIAN_POINT('Ctrl Pts',(5.65022540051358,5.53706528775738,105.897921137895));
#233057=CARTESIAN_POINT('Ctrl Pts',(5.66055151266958,5.52650844964806,105.897313809371));
#233058=CARTESIAN_POINT('Ctrl Pts',(5.76846167151175,5.41556743033146,105.890923812287));
#233059=CARTESIAN_POINT('Ctrl Pts',(5.86338912345694,5.31264381674667,105.884930644053));
#233060=CARTESIAN_POINT('Ctrl Pts',(6.09968377031884,5.04239431792184,105.869173144019));
#233061=CARTESIAN_POINT('Ctrl Pts',(6.23692216167477,4.8716193354395,105.8591979773));
#233062=CARTESIAN_POINT('Ctrl Pts',(6.8832363307184,3.99522352431714,105.808859777952));
#233063=CARTESIAN_POINT('Ctrl Pts',(7.28072424632657,3.21442699816221,105.76758485744));
#233064=CARTESIAN_POINT('Ctrl Pts',(7.55984904695948,2.33145893135083,105.729643859279));
#233065=CARTESIAN_POINT('Ctrl Pts',(7.57606398208699,2.27821708350046,105.727383447469));
#233066=CARTESIAN_POINT('Ctrl Pts',(7.59524851848286,2.21275365167149,105.724637086493));
#233067=CARTESIAN_POINT('Ctrl Pts',(7.59875236105398,2.20069110461088,105.72413239445));
#233068=CARTESIAN_POINT('Ctrl Pts',(7.60449470778101,2.18074491863104,105.723300094403));
#233069=CARTESIAN_POINT('Ctrl Pts',(7.60674971108511,2.17286607831082,105.722971908503));
#233070=CARTESIAN_POINT('Ctrl Pts',(7.61079922003587,2.15863378516567,105.722380112604));
#233071=CARTESIAN_POINT('Ctrl Pts',(7.61259802133791,2.15228156893393,105.722116352455));
#233072=CARTESIAN_POINT('Ctrl Pts',(7.61642573634328,2.13869969535905,105.721553192547));
#233073=CARTESIAN_POINT('Ctrl Pts',(7.61845231355171,2.13146938301492,105.721253874663));
#233074=CARTESIAN_POINT('Ctrl Pts',(7.62390082857731,2.11192342197791,105.720446011161));
#233075=CARTESIAN_POINT('Ctrl Pts',(7.62730322434541,2.09960232193685,105.719938148063));
#233076=CARTESIAN_POINT('Ctrl Pts',(7.64389842426363,2.03893340594918,105.717444212544));
#233077=CARTESIAN_POINT('Ctrl Pts',(7.65666161261057,1.99046869587584,105.715473120214));
#233078=CARTESIAN_POINT('Ctrl Pts',(7.75852917657752,1.58816964382418,105.699281176271));
#233079=CARTESIAN_POINT('Ctrl Pts',(7.82352071955822,1.22866433344624,105.685927409384));
#233080=CARTESIAN_POINT('Ctrl Pts',(7.93763427257802,0.192405542143997,
105.649285448962));
#233081=CARTESIAN_POINT('Ctrl Pts',(7.92495832516765,-0.487766230684799,
105.627630277317));
#233082=CARTESIAN_POINT('Ctrl Pts',(7.81662282161649,-1.21994165280978,
105.600446807928));
#233083=CARTESIAN_POINT('Ctrl Pts',(7.80671165764907,-1.28183570373121,
105.598115851771));
#233084=CARTESIAN_POINT('Ctrl Pts',(7.7761730217504,-1.45903165265274,105.591330826772));
#233085=CARTESIAN_POINT('Ctrl Pts',(7.75371964680885,-1.57399789660289,
105.58679236994));
#233086=CARTESIAN_POINT('Ctrl Pts',(7.7264518578499,-1.69881604967526,105.581673062458));
#233087=CARTESIAN_POINT('Ctrl Pts',(7.72415932861255,-1.70920945089628,
105.581245320184));
#233088=CARTESIAN_POINT('Ctrl Pts',(7.72071617951667,-1.7246708910578,105.580606806497));
#233089=CARTESIAN_POINT('Ctrl Pts',(7.71958155801904,-1.72974234380659,
105.580397019714));
#233090=CARTESIAN_POINT('Ctrl Pts',(7.71762464156699,-1.73844895884471,
105.580036263015));
#233091=CARTESIAN_POINT('Ctrl Pts',(7.71680477217257,-1.74208467036115,
105.579885439235));
#233092=CARTESIAN_POINT('Ctrl Pts',(7.71520002201614,-1.74917757490215,
105.579590850105));
#233093=CARTESIAN_POINT('Ctrl Pts',(7.71441538577593,-1.75263482330744,
105.579447099397));
#233094=CARTESIAN_POINT('Ctrl Pts',(7.71254792291515,-1.76083765004398,
105.579105649553));
#233095=CARTESIAN_POINT('Ctrl Pts',(7.71146304075051,-1.76558275479234,
105.578907828254));
#233096=CARTESIAN_POINT('Ctrl Pts',(7.708213801506,-1.77973429361479,105.57831696162));
#233097=CARTESIAN_POINT('Ctrl Pts',(7.70603661477569,-1.78913774085468,
105.577923160743));
#233098=CARTESIAN_POINT('Ctrl Pts',(7.70102677212553,-1.81059686812671,
105.577021828845));
#233099=CARTESIAN_POINT('Ctrl Pts',(7.69818301210616,-1.82264990403977,
105.576513655977));
#233100=CARTESIAN_POINT('Ctrl Pts',(7.57485364604281,-2.33993328393579,
105.554623326156));
#233101=CARTESIAN_POINT('Ctrl Pts',(7.40494280283978,-2.83203348029344,
105.530541066803));
#233102=CARTESIAN_POINT('Ctrl Pts',(7.07044660336402,-3.55977902504154,
105.493182458441));
#233103=CARTESIAN_POINT('Ctrl Pts',(6.93924064256329,-3.80922412902051,
105.480018041427));
#233104=CARTESIAN_POINT('Ctrl Pts',(6.53193628424697,-4.49239820047406,
105.443551223091));
#233105=CARTESIAN_POINT('Ctrl Pts',(6.22648357998664,-4.90702200725167,
105.421002888292));
#233106=CARTESIAN_POINT('Ctrl Pts',(5.86053602123054,-5.31405314187601,
105.398720871085));
#233107=CARTESIAN_POINT('Ctrl Pts',(5.8379803753811,-5.338822756332,105.397363782543));
#233108=CARTESIAN_POINT('Ctrl Pts',(5.80709295227768,-5.37231214995567,
105.395527236734));
#233109=CARTESIAN_POINT('Ctrl Pts',(5.79889773800933,-5.38115707062436,
105.395042020107));
#233110=CARTESIAN_POINT('Ctrl Pts',(5.78592113716253,-5.39509837054032,
105.394276954471));
#233111=CARTESIAN_POINT('Ctrl Pts',(5.78115318128632,-5.40020719307048,
105.393996536657));
#233112=CARTESIAN_POINT('Ctrl Pts',(5.77193337049546,-5.41005993405388,
105.393455616101));
#233113=CARTESIAN_POINT('Ctrl Pts',(5.76748242170962,-5.41480469075562,
105.393195075228));
#233114=CARTESIAN_POINT('Ctrl Pts',(5.75693097140843,-5.42602487438298,
105.39257883588));
#233115=CARTESIAN_POINT('Ctrl Pts',(5.7508253838328,-5.43249551792844,105.392223354427));
#233116=CARTESIAN_POINT('Ctrl Pts',(5.73287003091193,-5.45146023799775,
105.391181181241));
#233117=CARTESIAN_POINT('Ctrl Pts',(5.72099033823889,-5.4639259761035,105.390495768138));
#233118=CARTESIAN_POINT('Ctrl Pts',(5.63178002833542,-5.55692726994508,
105.385379182763));
#233119=CARTESIAN_POINT('Ctrl Pts',(5.55279124185217,-5.63585819828866,
105.381019901706));
#233120=CARTESIAN_POINT('Ctrl Pts',(5.28767653392548,-5.88979229701464,
105.366912647368));
#233121=CARTESIAN_POINT('Ctrl Pts',(5.09474011491395,-6.05745911481499,
105.357468760778));
#233122=CARTESIAN_POINT('Ctrl Pts',(4.57684193019832,-6.46524648868583,
105.333749233714));
#233123=CARTESIAN_POINT('Ctrl Pts',(4.24100692455315,-6.69034838433158,
105.319903515494));
#233124=CARTESIAN_POINT('Ctrl Pts',(3.48134165673463,-7.11925831866761,
105.28959733606));
#233125=CARTESIAN_POINT('Ctrl Pts',(3.05354484548062,-7.31296500264657,
105.273082543309));
#233126=CARTESIAN_POINT('Ctrl Pts',(2.56900603686614,-7.48238727103136,
105.252846144022));
#233127=CARTESIAN_POINT('Ctrl Pts',(2.52677018845004,-7.49675553868532,
105.251072604673));
#233128=CARTESIAN_POINT('Ctrl Pts',(2.4723408612444,-7.51475970462628,105.248776428497));
#233129=CARTESIAN_POINT('Ctrl Pts',(2.46025653384522,-7.51872466166755,
105.248265964616));
#233130=CARTESIAN_POINT('Ctrl Pts',(2.44098501128724,-7.52499635554101,
105.247450880783));
#233131=CARTESIAN_POINT('Ctrl Pts',(2.43380395840812,-7.52732198513062,
105.247146934833));
#233132=CARTESIAN_POINT('Ctrl Pts',(2.42036191966919,-7.53165402839776,
105.24657757588));
#233133=CARTESIAN_POINT('Ctrl Pts',(2.41410173600743,-7.53366292274778,
105.246312249702));
#233134=CARTESIAN_POINT('Ctrl Pts',(2.40025408827323,-7.53808760345943,
105.245724984674));
#233135=CARTESIAN_POINT('Ctrl Pts',(2.39266547079637,-7.54049974140044,
105.245402921272));
#233136=CARTESIAN_POINT('Ctrl Pts',(2.37077548636033,-7.54742137806952,
105.244473238611));
#233137=CARTESIAN_POINT('Ctrl Pts',(2.35646495883801,-7.55190166510348,
105.243864643656));
#233138=CARTESIAN_POINT('Ctrl Pts',(2.26472938666755,-7.58033575969529,
105.239958402624));
#233139=CARTESIAN_POINT('Ctrl Pts',(2.1869540430832,-7.6031388906577,105.236624193573));
#233140=CARTESIAN_POINT('Ctrl Pts',(1.93621839925187,-7.67248709825828,
105.225825885811));
#233141=CARTESIAN_POINT('Ctrl Pts',(1.76202529855718,-7.71435440278824,
105.218250464062));
#233142=CARTESIAN_POINT('Ctrl Pts',(1.20945729845843,-7.82747116259094,
105.19418733778));
#233143=CARTESIAN_POINT('Ctrl Pts',(0.827216387842954,-7.87704313949055,
105.177523376986));
#233144=CARTESIAN_POINT('Ctrl Pts',(0.036421668452692,-7.92138414684184,
105.143655816423));
#233145=CARTESIAN_POINT('Ctrl Pts',(-0.371204159468807,-7.91276686889032,
105.126533007308));
#233146=CARTESIAN_POINT('Ctrl Pts',(-0.858048411075272,-7.86475753657331,
105.106266630712));
#233147=CARTESIAN_POINT('Ctrl Pts',(-0.93960255654408,-7.85543158153127,
105.102876101318));
#233148=CARTESIAN_POINT('Ctrl Pts',(-1.29360066034414,-7.80935911466337,
105.088159693386));
#233149=CARTESIAN_POINT('Ctrl Pts',(-1.56417635887421,-7.7596939649725,
105.076891859814));
#233150=CARTESIAN_POINT('Ctrl Pts',(-1.87102985666812,-7.68666438936108,
105.064122432468));
#233151=CARTESIAN_POINT('Ctrl Pts',(-1.91036781084693,-7.67698228520684,
105.062485534636));
#233152=CARTESIAN_POINT('Ctrl Pts',(-1.974282255296,-7.66072957486322,105.05982611255));
#233153=CARTESIAN_POINT('Ctrl Pts',(-1.99890439893648,-7.65434185622841,
105.058801638611));
#233154=CARTESIAN_POINT('Ctrl Pts',(-2.04283668993195,-7.64271807234374,
105.056973735756));
#233155=CARTESIAN_POINT('Ctrl Pts',(-2.06215857266666,-7.63752730266007,
105.056169813212));
#233156=CARTESIAN_POINT('Ctrl Pts',(-2.10301072108604,-7.62638615963095,
105.054470077423));
#233157=CARTESIAN_POINT('Ctrl Pts',(-2.12453590533921,-7.62041777984972,
105.05357447487));
#233158=CARTESIAN_POINT('Ctrl Pts',(-2.18190424527362,-7.60424905061849,
105.051187474993));
#233159=CARTESIAN_POINT('Ctrl Pts',(-2.21770115747607,-7.59388644587783,
105.049697960601));
#233160=CARTESIAN_POINT('Ctrl Pts',(-2.39130335690778,-7.54229930308727,
105.04247345317));
#233161=CARTESIAN_POINT('Ctrl Pts',(-2.52804145945883,-7.49757413247492,
105.036780862694));
#233162=CARTESIAN_POINT('Ctrl Pts',(-3.34045228452211,-7.20709186589195,
105.00287759895));
#233163=CARTESIAN_POINT('Ctrl Pts',(-3.98122994099946,-6.87390125026642,
104.976111044038));
#233164=CARTESIAN_POINT('Ctrl Pts',(-4.62130200982151,-6.4211936314609,
104.945084104855));
#233165=CARTESIAN_POINT('Ctrl Pts',(-4.67399071621715,-6.38294371955429,
104.942492321192));
#233166=CARTESIAN_POINT('Ctrl Pts',(-4.74030581851302,-6.33354017279517,
104.939176438108));
#233167=CARTESIAN_POINT('Ctrl Pts',(-4.75437573115943,-6.32298519501784,
104.938469776438));
#233168=CARTESIAN_POINT('Ctrl Pts',(-4.77714382200755,-6.30578604948514,
104.937321117851));
#233169=CARTESIAN_POINT('Ctrl Pts',(-4.78586357399881,-6.29917063177192,
104.936879982036));
#233170=CARTESIAN_POINT('Ctrl Pts',(-4.8018291474333,-6.28700573700533,
104.936070057323));
#233171=CARTESIAN_POINT('Ctrl Pts',(-4.80907915385023,-6.2814617717345,
104.9357014255));
#233172=CARTESIAN_POINT('Ctrl Pts',(-4.82620302928776,-6.2683203917819,
104.934828770343));
#233173=CARTESIAN_POINT('Ctrl Pts',(-4.83606856834782,-6.26071218112536,
104.934324448011));
#233174=CARTESIAN_POINT('Ctrl Pts',(-4.86494801153547,-6.23833163554391,
104.932843608189));
#233175=CARTESIAN_POINT('Ctrl Pts',(-4.88391244348126,-6.22349580104308,
104.93186539077));
#233176=CARTESIAN_POINT('Ctrl Pts',(-5.03410132235224,-6.10489410735503,
104.924073269472));
#233177=CARTESIAN_POINT('Ctrl Pts',(-5.1620697590268,-5.99707778083458,
104.917159603426));
#233178=CARTESIAN_POINT('Ctrl Pts',(-5.51401379139163,-5.68094039309349,
104.897458256518));
#233179=CARTESIAN_POINT('Ctrl Pts',(-5.72946565181466,-5.46357519450972,
104.884569955401));
#233180=CARTESIAN_POINT('Ctrl Pts',(-6.2222095992506,-4.90516957865222,
104.853335283329));
#233181=CARTESIAN_POINT('Ctrl Pts',(-6.48474069979273,-4.55244363872441,
104.835134214252));
#233182=CARTESIAN_POINT('Ctrl Pts',(-6.74295310230439,-4.13750896575956,
104.815309969591));
#233183=CARTESIAN_POINT('Ctrl Pts',(-6.76884418641868,-4.09501470091643,
104.813296488418));
#233184=CARTESIAN_POINT('Ctrl Pts',(-6.81020937420422,-4.02565894796312,
104.810036569524));
#233185=CARTESIAN_POINT('Ctrl Pts',(-6.8259294723996,-3.99894592772647,
104.808787237415));
#233186=CARTESIAN_POINT('Ctrl Pts',(-6.85365205280577,-3.95119741858366,
104.806564990027));
#233187=CARTESIAN_POINT('Ctrl Pts',(-6.86571567901906,-3.93019792386195,
104.805591377464));
#233188=CARTESIAN_POINT('Ctrl Pts',(-6.89099281711486,-3.88572574132131,
104.803537182765));
#233189=CARTESIAN_POINT('Ctrl Pts',(-6.90418326365567,-3.86224028381423,
104.80245687244));
#233190=CARTESIAN_POINT('Ctrl Pts',(-6.93906173231599,-3.79938984672886,
104.799577516735));
#233191=CARTESIAN_POINT('Ctrl Pts',(-6.96053471602924,-3.75990657128227,
104.797780860364));
#233192=CARTESIAN_POINT('Ctrl Pts',(-7.07015882352115,-3.55417821031327,
104.78847972497));
#233193=CARTESIAN_POINT('Ctrl Pts',(-7.15269509877856,-3.3850084880439,
104.781034422208));
#233194=CARTESIAN_POINT('Ctrl Pts',(-7.34803107395479,-2.94551802114772,
104.762095799163));
#233195=CARTESIAN_POINT('Ctrl Pts',(-7.45199992584659,-2.67158043128907,
104.750698482321));
#233196=CARTESIAN_POINT('Ctrl Pts',(-7.78611126941897,-1.61854911264299,
104.708410644666));
#233197=CARTESIAN_POINT('Ctrl Pts',(-7.91102272519647,-0.811531069090435,
104.679708267495));
#233198=CARTESIAN_POINT('Ctrl Pts',(-7.9109999968991,0.000221500451111772,
104.648002515785));
#233199=CARTESIAN_POINT('',(-7.91099875017949,0.00164077279768504,100.640436842002));
#233200=CARTESIAN_POINT('Ctrl Pts',(-7.91099999680876,0.00022470367903259,
104.648002390672));
#233201=CARTESIAN_POINT('Ctrl Pts',(-7.91099856279906,0.0507109744170651,
104.646030477437));
#233202=CARTESIAN_POINT('Ctrl Pts',(-7.91051384011523,0.101195664386328,
104.644044926041));
#233203=CARTESIAN_POINT('Ctrl Pts',(-7.90900130355969,0.180073065026429,
104.640917243705));
#233204=CARTESIAN_POINT('Ctrl Pts',(-7.90830372159879,0.208470985230131,
104.639786037387));
#233205=CARTESIAN_POINT('Ctrl Pts',(-7.90716408160562,0.246516605544437,
104.638262975117));
#233206=CARTESIAN_POINT('Ctrl Pts',(-7.90685727935303,0.256168329812173,
104.63787594103));
#233207=CARTESIAN_POINT('Ctrl Pts',(-7.90630759975512,0.272517998349415,
104.637219184298));
#233208=CARTESIAN_POINT('Ctrl Pts',(-7.9060738805796,0.279216252838261,
104.636949796477));
#233209=CARTESIAN_POINT('Ctrl Pts',(-7.9056254789115,0.291615036211121,
104.636450537674));
#233210=CARTESIAN_POINT('Ctrl Pts',(-7.9054131420722,0.297315648930616,
104.636220754024));
#233211=CARTESIAN_POINT('Ctrl Pts',(-7.90497519624272,0.308740942716914,
104.635759730748));
#233212=CARTESIAN_POINT('Ctrl Pts',(-7.90474953415147,0.314465618209801,
104.635528489254));
#233213=CARTESIAN_POINT('Ctrl Pts',(-7.90421395854293,0.327687350318683,
104.63499383911));
#233214=CARTESIAN_POINT('Ctrl Pts',(-7.90389959728831,0.335184214230046,
104.6346902605));
#233215=CARTESIAN_POINT('Ctrl Pts',(-7.90307842516679,0.354123702037099,
104.633922223714));
#233216=CARTESIAN_POINT('Ctrl Pts',(-7.90255742967426,0.365565670643811,
104.633457213143));
#233217=CARTESIAN_POINT('Ctrl Pts',(-7.89961883478154,0.427158283451147,
104.63094840743));
#233218=CARTESIAN_POINT('Ctrl Pts',(-7.89674872372343,0.477285407664686,
104.628886511833));
#233219=CARTESIAN_POINT('Ctrl Pts',(-7.89124278339187,0.559693766779013,
104.625459169533));
#233220=CARTESIAN_POINT('Ctrl Pts',(-7.88888556293277,0.591991795322786,
104.624106200033));
#233221=CARTESIAN_POINT('Ctrl Pts',(-7.81394376102194,1.53871583977549,
104.584164654968));
#233222=CARTESIAN_POINT('Ctrl Pts',(-7.58307770621705,2.43363324719075,
104.539481595288));
#233223=CARTESIAN_POINT('Ctrl Pts',(-7.06830902794243,3.56800813626424,
104.484658793237));
#233224=CARTESIAN_POINT('Ctrl Pts',(-6.91418053371399,3.85821386152608,
104.470723979871));
#233225=CARTESIAN_POINT('Ctrl Pts',(-6.729989376434,4.15833279892066,104.456437009841));
#233226=CARTESIAN_POINT('Ctrl Pts',(-6.71743496433179,4.17858303565186,
104.45547354415));
#233227=CARTESIAN_POINT('Ctrl Pts',(-6.69927320480545,4.2075845252691,104.454094427105));
#233228=CARTESIAN_POINT('Ctrl Pts',(-6.69373985410061,4.21638183476724,
104.453676180859));
#233229=CARTESIAN_POINT('Ctrl Pts',(-6.68411429059146,4.23161852737457,
104.452951949115));
#233230=CARTESIAN_POINT('Ctrl Pts',(-6.6800300747075,4.23806293161227,104.452645682624));
#233231=CARTESIAN_POINT('Ctrl Pts',(-6.67216473705474,4.25043387691242,
104.452057853155));
#233232=CARTESIAN_POINT('Ctrl Pts',(-6.66838502724493,4.2563613038736,104.451776240816));
#233233=CARTESIAN_POINT('Ctrl Pts',(-6.65947143203441,4.27029879087911,
104.451114163599));
#233234=CARTESIAN_POINT('Ctrl Pts',(-6.65433098260269,4.27830465164008,
104.450733931261));
#233235=CARTESIAN_POINT('Ctrl Pts',(-6.63655634382299,4.30587777277385,
104.449424607447));
#233236=CARTESIAN_POINT('Ctrl Pts',(-6.62385013637651,4.32539858058769,
104.448498071353));
#233237=CARTESIAN_POINT('Ctrl Pts',(-6.48042408747497,4.54363282285369,
104.438143967653));
#233238=CARTESIAN_POINT('Ctrl Pts',(-6.34088766361146,4.73641741648619,
104.429041182139));
#233239=CARTESIAN_POINT('Ctrl Pts',(-5.92541193619878,5.25910261397333,
104.404250217426));
#233240=CARTESIAN_POINT('Ctrl Pts',(-5.63096950902634,5.57322839518147,
104.389248594054));
#233241=CARTESIAN_POINT('Ctrl Pts',(-5.0198060940556,6.12710838409801,104.360735954042));
#233242=CARTESIAN_POINT('Ctrl Pts',(-4.70771333084289,6.37003308490911,
104.347227078248));
#233243=CARTESIAN_POINT('Ctrl Pts',(-4.28277127253056,6.65244967306423,
104.328694539707));
#233244=CARTESIAN_POINT('Ctrl Pts',(-4.18535822962497,6.71416349795983,
104.324435906049));
#233245=CARTESIAN_POINT('Ctrl Pts',(-4.00908370712365,6.82051111454271,
104.316657700916));
#233246=CARTESIAN_POINT('Ctrl Pts',(-3.93073784819223,6.86596119122125,
104.313176083664));
#233247=CARTESIAN_POINT('Ctrl Pts',(-3.82464060989635,6.92509927962185,
104.308408775803));
#233248=CARTESIAN_POINT('Ctrl Pts',(-3.79756307748602,6.93998490532024,
104.307187490177));
#233249=CARTESIAN_POINT('Ctrl Pts',(-3.75763579788348,6.96163091256331,
104.305379517897));
#233250=CARTESIAN_POINT('Ctrl Pts',(-3.74485439548694,6.9685147129493,104.304799726108));
#233251=CARTESIAN_POINT('Ctrl Pts',(-3.72470916890797,6.97929308740188,
104.303884366577));
#233252=CARTESIAN_POINT('Ctrl Pts',(-3.71735797276682,6.98321130242447,
104.303550023251));
#233253=CARTESIAN_POINT('Ctrl Pts',(-3.70493776233799,6.98980615156952,
104.302984612616));
#233254=CARTESIAN_POINT('Ctrl Pts',(-3.69987199112979,6.99248890655688,
104.302753855288));
#233255=CARTESIAN_POINT('Ctrl Pts',(-3.68992392858131,6.99774341141572,
104.302300418817));
#233256=CARTESIAN_POINT('Ctrl Pts',(-3.68504185269115,7.00031556391699,
104.302077759935));
#233257=CARTESIAN_POINT('Ctrl Pts',(-3.67570639597185,7.00522153611013,
104.301651747489));
#233258=CARTESIAN_POINT('Ctrl Pts',(-3.67125347194643,7.00755622338647,
104.30144843665));
#233259=CARTESIAN_POINT('Ctrl Pts',(-3.66096760333801,7.01293665358347,
104.30097856469));
#233260=CARTESIAN_POINT('Ctrl Pts',(-3.65513308335295,7.0159793644559,104.30071185706));
#233261=CARTESIAN_POINT('Ctrl Pts',(-3.6373081905813,7.02524680301354,104.299896514485));
#233262=CARTESIAN_POINT('Ctrl Pts',(-3.62530570182206,7.03144807857554,
104.299346766615));
#233263=CARTESIAN_POINT('Ctrl Pts',(-3.53762387447654,7.07646609753964,
104.295325673824));
#233264=CARTESIAN_POINT('Ctrl Pts',(-3.46134046951723,7.11409000268569,
104.291800150482));
#233265=CARTESIAN_POINT('Ctrl Pts',(-3.0728898455068,7.29795167383479,104.273764399361));
#233266=CARTESIAN_POINT('Ctrl Pts',(-2.75201623198666,7.42490008742438,
104.258618476405));
#233267=CARTESIAN_POINT('Ctrl Pts',(-2.1696589011589,7.61234768296996,104.231678047842));
#233268=CARTESIAN_POINT('Ctrl Pts',(-1.91143081212576,7.68125603244696,
104.219909252492));
#233269=CARTESIAN_POINT('Ctrl Pts',(-1.22663432146542,7.82731543238694,
104.189517994866));
#233270=CARTESIAN_POINT('Ctrl Pts',(-0.796335537854923,7.88272771644739,
104.171274756551));
#233271=CARTESIAN_POINT('Ctrl Pts',(-0.324223379771767,7.90445170920404,
104.152124786385));
#233272=CARTESIAN_POINT('Ctrl Pts',(-0.284797795784741,7.90597039412212,
104.150531596297));
#233273=CARTESIAN_POINT('Ctrl Pts',(-0.227937076194581,7.90773479698451,
104.148241983106));
#233274=CARTESIAN_POINT('Ctrl Pts',(-0.210510091046111,7.90821790510105,
104.147541350046));
#233275=CARTESIAN_POINT('Ctrl Pts',(-0.180168731504492,7.90895865901514,
104.146323363445));
#233276=CARTESIAN_POINT('Ctrl Pts',(-0.167255078335444,7.90924228872335,
104.145805558265));
#233277=CARTESIAN_POINT('Ctrl Pts',(-0.142339721462338,7.90972847091561,
104.144807614446));
#233278=CARTESIAN_POINT('Ctrl Pts',(-0.130338140694001,7.9099353379086,
104.144327402964));
#233279=CARTESIAN_POINT('Ctrl Pts',(-0.101912637977869,7.91036058629731,
104.143191168144));
#233280=CARTESIAN_POINT('Ctrl Pts',(-0.0854884000907424,7.91055513391577,
104.14253555087));
#233281=CARTESIAN_POINT('Ctrl Pts',(-0.0365220996372178,7.91098262979195,
104.140583510531));
#233282=CARTESIAN_POINT('Ctrl Pts',(-0.00397896140958066,7.91106593422137,
104.139289557121));
#233283=CARTESIAN_POINT('Ctrl Pts',(0.265172390769217,7.91009411696947,
104.128614061184));
#233284=CARTESIAN_POINT('Ctrl Pts',(0.501628880047005,7.89862519981647,
104.119409741103));
#233285=CARTESIAN_POINT('Ctrl Pts',(0.869731726890195,7.86417193643272,
104.105280080266));
#233286=CARTESIAN_POINT('Ctrl Pts',(1.00190843403903,7.84842748188554,104.100245908461));
#233287=CARTESIAN_POINT('Ctrl Pts',(1.55519146677457,7.768316618034,104.079271341737));
#233288=CARTESIAN_POINT('Ctrl Pts',(1.97113404522159,7.6733301071319,104.063783212418));
#233289=CARTESIAN_POINT('Ctrl Pts',(2.73437620430371,7.43284509590422,104.034220593727));
#233290=CARTESIAN_POINT('Ctrl Pts',(3.08289374782533,7.29518540987065,104.020225438879));
#233291=CARTESIAN_POINT('Ctrl Pts',(3.43990939998329,7.12400278452517,104.004411689016));
#233292=CARTESIAN_POINT('Ctrl Pts',(3.45944719899067,7.11453564331709,104.003541369252));
#233293=CARTESIAN_POINT('Ctrl Pts',(3.48671095917665,7.10118598856891,104.002319750827));
#233294=CARTESIAN_POINT('Ctrl Pts',(3.49446999995576,7.09737100451646,104.001971276511));
#233295=CARTESIAN_POINT('Ctrl Pts',(3.50756641124125,7.09090504702358,104.001381697063));
#233296=CARTESIAN_POINT('Ctrl Pts',(3.5129070788213,7.0882607436867,104.001140876701));
#233297=CARTESIAN_POINT('Ctrl Pts',(3.52356175478686,7.08297033742241,104.000659647086));
#233298=CARTESIAN_POINT('Ctrl Pts',(3.52887578287247,7.08032428278593,104.000419240006));
#233299=CARTESIAN_POINT('Ctrl Pts',(3.54163519371704,7.07395295899538,103.999841048));
#233300=CARTESIAN_POINT('Ctrl Pts',(3.54907767468588,7.07022191800212,103.999503009955));
#233301=CARTESIAN_POINT('Ctrl Pts',(3.57385322992119,7.05775253784545,103.998375057308));
#233302=CARTESIAN_POINT('Ctrl Pts',(3.59115994348341,7.04896219635039,103.997582817923));
#233303=CARTESIAN_POINT('Ctrl Pts',(3.83329365681737,6.92485564972529,103.986436202659));
#233304=CARTESIAN_POINT('Ctrl Pts',(4.05245611547913,6.79892076316857,103.975505902935));
#233305=CARTESIAN_POINT('Ctrl Pts',(4.56722792948259,6.46938632805474,103.94820276911));
#233306=CARTESIAN_POINT('Ctrl Pts',(4.85575974172369,6.25572683493918,103.931573477293));
#233307=CARTESIAN_POINT('Ctrl Pts',(5.15286335876065,6.0027426646834,103.913640516303));
#233308=CARTESIAN_POINT('Ctrl Pts',(5.17680861947608,5.98210438037257,103.912188917948));
#233309=CARTESIAN_POINT('Ctrl Pts',(5.22640822618295,5.93883392210798,103.90916967635));
#233310=CARTESIAN_POINT('Ctrl Pts',(5.25204079594768,5.91617771809421,103.907602331527));
#233311=CARTESIAN_POINT('Ctrl Pts',(5.30532414013013,5.86846225314133,103.904330296113));
#233312=CARTESIAN_POINT('Ctrl Pts',(5.33294623210903,5.84337213905091,103.9026260946));
#233313=CARTESIAN_POINT('Ctrl Pts',(5.43364752316816,5.75059282155087,103.896385459182));
#233314=CARTESIAN_POINT('Ctrl Pts',(5.50562483596642,5.68171971596473,103.891870968999));
#233315=CARTESIAN_POINT('Ctrl Pts',(5.76890783400206,5.42008925136928,103.875182903006));
#233316=CARTESIAN_POINT('Ctrl Pts',(5.95155836003378,5.21887302516532,103.8632588778));
#233317=CARTESIAN_POINT('Ctrl Pts',(6.1926277985352,4.92414461470119,103.847130175559));
#233318=CARTESIAN_POINT('Ctrl Pts',(6.25999151387548,4.83821731243413,103.842574098278));
#233319=CARTESIAN_POINT('Ctrl Pts',(6.36208009351487,4.70229268679639,103.835591715106));
#233320=CARTESIAN_POINT('Ctrl Pts',(6.39804167997069,4.65324429973269,103.833116142368));
#233321=CARTESIAN_POINT('Ctrl Pts',(6.44159415716992,4.59238307454727,103.830097668308));
#233322=CARTESIAN_POINT('Ctrl Pts',(6.44972335417145,4.58095909678863,103.829533367071));
#233323=CARTESIAN_POINT('Ctrl Pts',(6.4624351487452,4.56299427224818,103.828649539093));
#233324=CARTESIAN_POINT('Ctrl Pts',(6.46703826642925,4.55646802264023,103.828329198393));
#233325=CARTESIAN_POINT('Ctrl Pts',(6.47518844514143,4.54487555909633,103.827761484695));
#233326=CARTESIAN_POINT('Ctrl Pts',(6.47873945917347,4.5398121401828,103.82751395516));
#233327=CARTESIAN_POINT('Ctrl Pts',(6.48690492084252,4.52813985185878,103.826944355564));
#233328=CARTESIAN_POINT('Ctrl Pts',(6.49151521651011,4.52152807846796,103.826622449939));
#233329=CARTESIAN_POINT('Ctrl Pts',(6.50409138720802,4.50343330588449,103.825743503475));
#233330=CARTESIAN_POINT('Ctrl Pts',(6.51203696916498,4.49193620041532,103.825187264728));
#233331=CARTESIAN_POINT('Ctrl Pts',(6.5503517340364,4.43618014658881,103.822500473582));
#233332=CARTESIAN_POINT('Ctrl Pts',(6.58030075290248,4.3916334413438,103.820386491526));
#233333=CARTESIAN_POINT('Ctrl Pts',(7.05923587615508,3.66335659088304,103.786343125768));
#233334=CARTESIAN_POINT('Ctrl Pts',(7.39993753790598,2.91443620786812,103.759385090456));
#233335=CARTESIAN_POINT('Ctrl Pts',(7.71172542169029,1.79724950940332,103.72018394223));
#233336=CARTESIAN_POINT('Ctrl Pts',(7.78218057985076,1.46234420252986,103.708445527195));
#233337=CARTESIAN_POINT('Ctrl Pts',(7.85067348193007,0.985145992251968,
103.690557359683));
#233338=CARTESIAN_POINT('Ctrl Pts',(7.86690185332629,0.845835671858197,
103.685196374146));
#233339=CARTESIAN_POINT('Ctrl Pts',(7.88075095986239,0.691308964782714,
103.679028342368));
#233340=CARTESIAN_POINT('Ctrl Pts',(7.88204121753958,0.67643921777803,103.678432544102));
#233341=CARTESIAN_POINT('Ctrl Pts',(7.88421951830941,0.650482359094225,
103.677388430876));
#233342=CARTESIAN_POINT('Ctrl Pts',(7.88512627787465,0.639396818784932,
103.676941218081));
#233343=CARTESIAN_POINT('Ctrl Pts',(7.88640790162829,0.623310959897841,
103.676290355448));
#233344=CARTESIAN_POINT('Ctrl Pts',(7.88680139831528,0.618312095057415,
103.676087822521));
#233345=CARTESIAN_POINT('Ctrl Pts',(7.88748295600495,0.609547278036952,
103.675732230945));
#233346=CARTESIAN_POINT('Ctrl Pts',(7.88777307362143,0.605781482372149,
103.675579296627));
#233347=CARTESIAN_POINT('Ctrl Pts',(7.88832632982372,0.598532302763836,
103.675284597));
#233348=CARTESIAN_POINT('Ctrl Pts',(7.88858985826301,0.595048948634216,
103.67514285544));
#233349=CARTESIAN_POINT('Ctrl Pts',(7.88920743610251,0.586813207691831,
103.674807416396));
#233350=CARTESIAN_POINT('Ctrl Pts',(7.88955949643506,0.582060703364394,
103.674613597783));
#233351=CARTESIAN_POINT('Ctrl Pts',(7.89060365468852,0.567790481269341,
103.674030874639));
#233352=CARTESIAN_POINT('Ctrl Pts',(7.89128282285799,0.558271863926252,
103.673641183815));
#233353=CARTESIAN_POINT('Ctrl Pts',(7.89769805773642,0.466010384051799,
103.669854506698));
#233354=CARTESIAN_POINT('Ctrl Pts',(7.90214955815526,0.383186204922131,
103.666381108505));
#233355=CARTESIAN_POINT('Ctrl Pts',(7.90865809644378,0.211857040404911,
103.659067299869));
#233356=CARTESIAN_POINT('Ctrl Pts',(7.91053339141874,0.123356217289581,
103.655218422766));
#233357=CARTESIAN_POINT('Ctrl Pts',(7.91121929855272,-0.0323641323097026,
103.648345580546));
#233358=CARTESIAN_POINT('Ctrl Pts',(7.91065882071714,-0.0995735600014991,
103.645346260282));
#233359=CARTESIAN_POINT('Ctrl Pts',(7.8961248419811,-0.788878025552247,
103.614305342894));
#233360=CARTESIAN_POINT('Ctrl Pts',(7.80965904895405,-1.40727843097387,
103.584347076154));
#233361=CARTESIAN_POINT('Ctrl Pts',(7.55285147873897,-2.3852765581267,103.538585254946));
#233362=CARTESIAN_POINT('Ctrl Pts',(7.42649934882145,-2.7535935370278,103.521697350389));
#233363=CARTESIAN_POINT('Ctrl Pts',(7.25336652174135,-3.15835874717134,
103.503695342208));
#233364=CARTESIAN_POINT('Ctrl Pts',(7.23272041880199,-3.20535666629566,
103.501613199467));
#233365=CARTESIAN_POINT('Ctrl Pts',(7.20632040626865,-3.26389847753996,
103.499029364916));
#233366=CARTESIAN_POINT('Ctrl Pts',(7.20099403039541,-3.27563307558965,
103.498511931872));
#233367=CARTESIAN_POINT('Ctrl Pts',(7.19250900617055,-3.29420581194,103.497693742401));
#233368=CARTESIAN_POINT('Ctrl Pts',(7.18936923592317,-3.3010525177982,103.497392288688));
#233369=CARTESIAN_POINT('Ctrl Pts',(7.18346023549913,-3.31388949674716,
103.496827397877));
#233370=CARTESIAN_POINT('Ctrl Pts',(7.18069328030043,-3.31988080602141,
103.496563876918));
#233371=CARTESIAN_POINT('Ctrl Pts',(7.1744874467493,-3.33327429027718,103.495975060171));
#233372=CARTESIAN_POINT('Ctrl Pts',(7.1710446009528,-3.34067462490496,103.495649911749));
#233373=CARTESIAN_POINT('Ctrl Pts',(7.16231902368869,-3.35935445233318,
103.494829656243));
#233374=CARTESIAN_POINT('Ctrl Pts',(7.15702108632424,-3.37062684160759,
103.494335113704));
#233375=CARTESIAN_POINT('Ctrl Pts',(7.1284459263344,-3.43105490744321,103.491686348234));
#233376=CARTESIAN_POINT('Ctrl Pts',(7.1046885926265,-3.47998265277427,103.489550005416));
#233377=CARTESIAN_POINT('Ctrl Pts',(6.6913439719332,-4.30937826213792,103.453465180375));
#233378=CARTESIAN_POINT('Ctrl Pts',(6.17591090397008,-5.0202366280083,103.425449145322));
#233379=CARTESIAN_POINT('Ctrl Pts',(5.31291829388461,-5.87131380340866,
103.383204681555));
#233380=CARTESIAN_POINT('Ctrl Pts',(5.05583059861422,-6.09409204115545,
103.370916884798));
#233381=CARTESIAN_POINT('Ctrl Pts',(4.77700366462205,-6.30589122877165,
103.356925986993));
#233382=CARTESIAN_POINT('Ctrl Pts',(4.76874656532475,-6.31213786245352,
103.356511089101));
#233383=CARTESIAN_POINT('Ctrl Pts',(4.75380217986812,-6.32339747957587,
103.355759084553));
#233384=CARTESIAN_POINT('Ctrl Pts',(4.74711917306056,-6.32841610555495,
103.355422401079));
#233385=CARTESIAN_POINT('Ctrl Pts',(4.73677481239256,-6.33615863138277,
103.354900670716));
#233386=CARTESIAN_POINT('Ctrl Pts',(4.73311900186257,-6.33888999268804,
103.354716171604));
#233387=CARTESIAN_POINT('Ctrl Pts',(4.72664529908826,-6.34371795975544,
103.354389262554));
#233388=CARTESIAN_POINT('Ctrl Pts',(4.72382836705896,-6.3458158573037,103.354246946765));
#233389=CARTESIAN_POINT('Ctrl Pts',(4.7179254964359,-6.350205885402,103.353948587294));
#233390=CARTESIAN_POINT('Ctrl Pts',(4.71483928317156,-6.35249764350017,
103.35379251677));
#233391=CARTESIAN_POINT('Ctrl Pts',(4.70627433926906,-6.35884811371101,
103.353359170894));
#233392=CARTESIAN_POINT('Ctrl Pts',(4.70079204118598,-6.36290198531067,
103.353081549041));
#233393=CARTESIAN_POINT('Ctrl Pts',(4.67910162181106,-6.37889757883909,
103.351982214688));
#233394=CARTESIAN_POINT('Ctrl Pts',(4.6628533061964,-6.39078440719886,103.351156634531));
#233395=CARTESIAN_POINT('Ctrl Pts',(4.58430860231699,-6.44778658794271,
103.347156532625));
#233396=CARTESIAN_POINT('Ctrl Pts',(4.52140358945253,-6.49205253341382,
103.343925065604));
#233397=CARTESIAN_POINT('Ctrl Pts',(3.7799890484064,-6.99777975226504,103.305611214986));
#233398=CARTESIAN_POINT('Ctrl Pts',(3.03429820035792,-7.35189984798089,
103.265416322383));
#233399=CARTESIAN_POINT('Ctrl Pts',(1.85212738361698,-7.70217831327837,
103.209768699113));
#233400=CARTESIAN_POINT('Ctrl Pts',(1.44821630912633,-7.78823878177506,
103.191934582948));
#233401=CARTESIAN_POINT('Ctrl Pts',(1.0029135740568,-7.84725681012048,103.173630553383));
#233402=CARTESIAN_POINT('Ctrl Pts',(0.966401122414857,-7.85183698247721,
103.17213913985));
#233403=CARTESIAN_POINT('Ctrl Pts',(0.917869532185374,-7.85758119600065,
103.170169068317));
#233404=CARTESIAN_POINT('Ctrl Pts',(0.905878083954368,-7.85897268277096,
103.169683286687));
#233405=CARTESIAN_POINT('Ctrl Pts',(0.886165495587429,-7.861214413295,103.168886339391));
#233406=CARTESIAN_POINT('Ctrl Pts',(0.878446225545652,-7.86208074027702,
103.168574670828));
#233407=CARTESIAN_POINT('Ctrl Pts',(0.863473223257752,-7.86373882042247,
103.167970918973));
#233408=CARTESIAN_POINT('Ctrl Pts',(0.856219648621964,-7.86453190957875,
103.167678794207));
#233409=CARTESIAN_POINT('Ctrl Pts',(0.839452891192355,-7.86634167687495,
103.167004368767));
#233410=CARTESIAN_POINT('Ctrl Pts',(0.829938931949276,-7.86735113643263,
103.166622293782));
#233411=CARTESIAN_POINT('Ctrl Pts',(0.799407250082365,-7.87053463991475,
103.16539811773));
#233412=CARTESIAN_POINT('Ctrl Pts',(0.778382560432509,-7.87264174645171,
103.164558103741));
#233413=CARTESIAN_POINT('Ctrl Pts',(0.588071873843842,-7.89094496635586,
103.156981022727));
#233414=CARTESIAN_POINT('Ctrl Pts',(0.418308055782274,-7.90176331958711,
103.150413222566));
#233415=CARTESIAN_POINT('Ctrl Pts',(-0.403606746036275,-7.92757536723379,
103.11938390534));
#233416=CARTESIAN_POINT('Ctrl Pts',(-1.05553335628941,-7.86735086313065,
103.097339395148));
#233417=CARTESIAN_POINT('Ctrl Pts',(-2.12828068574673,-7.63237771293475,
103.058986557528));
#233418=CARTESIAN_POINT('Ctrl Pts',(-2.55503929820115,-7.50030469541763,
103.042958264038));
#233419=CARTESIAN_POINT('Ctrl Pts',(-2.98617108620706,-7.3257812154942,
103.024393920752));
#233420=CARTESIAN_POINT('Ctrl Pts',(-3.00390650107437,-7.31852675739403,
103.023626608601));
#233421=CARTESIAN_POINT('Ctrl Pts',(-3.02986154852273,-7.3077999160061,
103.02249849452));
#233422=CARTESIAN_POINT('Ctrl Pts',(-3.03810201411643,-7.30437791784378,
103.022139561492));
#233423=CARTESIAN_POINT('Ctrl Pts',(-3.0526018685897,-7.29832781661137,
103.021506650064));
#233424=CARTESIAN_POINT('Ctrl Pts',(-3.05886370532628,-7.29570558059861,
103.021232884531));
#233425=CARTESIAN_POINT('Ctrl Pts',(-3.07105377248945,-7.29058235845154,
103.020699090741));
#233426=CARTESIAN_POINT('Ctrl Pts',(-3.0769823432685,-7.28808219340441,
103.020439091882));
#233427=CARTESIAN_POINT('Ctrl Pts',(-3.09283884890406,-7.28137247632975,
103.019742663581));
#233428=CARTESIAN_POINT('Ctrl Pts',(-3.1027612219825,-7.27714985983386,
103.019305776717));
#233429=CARTESIAN_POINT('Ctrl Pts',(-3.13865286153165,-7.26178887611833,
103.017721565155));
#233430=CARTESIAN_POINT('Ctrl Pts',(-3.16457089638142,-7.25053173824833,
103.016570200961));
#233431=CARTESIAN_POINT('Ctrl Pts',(-3.19779651205155,-7.23588856398032,
103.015085105061));
#233432=CARTESIAN_POINT('Ctrl Pts',(-3.2051601592962,-7.23262982570161,
103.014755392923));
#233433=CARTESIAN_POINT('Ctrl Pts',(-3.2619736801147,-7.20738353728301,
103.012207127141));
#233434=CARTESIAN_POINT('Ctrl Pts',(-3.31120122605761,-7.18490055991174,
103.009973350813));
#233435=CARTESIAN_POINT('Ctrl Pts',(-3.94319510893822,-6.88838461801055,
102.980987952697));
#233436=CARTESIAN_POINT('Ctrl Pts',(-4.49062304349641,-6.54469026475956,
102.952760980972));
#233437=CARTESIAN_POINT('Ctrl Pts',(-5.50682005398615,-5.71855902207885,
102.897065596));
#233438=CARTESIAN_POINT('Ctrl Pts',(-5.96826747919322,-5.23515192693193,
102.869623944422));
#233439=CARTESIAN_POINT('Ctrl Pts',(-6.39728147384622,-4.65423489949048,
102.840338928498));
#233440=CARTESIAN_POINT('Ctrl Pts',(-6.43035613571116,-4.60843061997615,
102.838053873666));
#233441=CARTESIAN_POINT('Ctrl Pts',(-6.47808662648472,-4.54081542283715,
102.834715548258));
#233442=CARTESIAN_POINT('Ctrl Pts',(-6.4931288398232,-4.51927969037552,
102.833657374142));
#233443=CARTESIAN_POINT('Ctrl Pts',(-6.51949723061543,-4.48112500449891,
102.831791550131));
#233444=CARTESIAN_POINT('Ctrl Pts',(-6.53086780992325,-4.46453705303625,
102.830983328874));
#233445=CARTESIAN_POINT('Ctrl Pts',(-6.55297129153682,-4.43202628305051,
102.82940503384));
#233446=CARTESIAN_POINT('Ctrl Pts',(-6.56370971706843,-4.41610738929351,
102.82863489187));
#233447=CARTESIAN_POINT('Ctrl Pts',(-6.59258900098856,-4.3729580197519,
102.826554531845));
#233448=CARTESIAN_POINT('Ctrl Pts',(-6.61061908642994,-4.34565379250885,
102.825245792869));
#233449=CARTESIAN_POINT('Ctrl Pts',(-6.67781929904982,-4.24250172548014,
102.82033002271));
#233450=CARTESIAN_POINT('Ctrl Pts',(-6.72585796795107,-4.16592442597223,
102.816738317277));
#233451=CARTESIAN_POINT('Ctrl Pts',(-7.07466814903248,-3.58812826170221,
102.790045765497));
#233452=CARTESIAN_POINT('Ctrl Pts',(-7.32036832004342,-3.05578212128145,
102.767863114709));
#233453=CARTESIAN_POINT('Ctrl Pts',(-7.58488708107624,-2.2620704651583,
102.735557422931));
#233454=CARTESIAN_POINT('Ctrl Pts',(-7.65311370151086,-2.01923700958277,
102.725745559407));
#233455=CARTESIAN_POINT('Ctrl Pts',(-7.71488270195008,-1.75072989100462,
102.714720533781));
#233456=CARTESIAN_POINT('Ctrl Pts',(-7.72003533668219,-1.72786708207051,
102.71378035885));
#233457=CARTESIAN_POINT('Ctrl Pts',(-7.72770188568035,-1.6931307839507,
102.712349521941));
#233458=CARTESIAN_POINT('Ctrl Pts',(-7.73029018825794,-1.68127388892119,
102.711860708968));
#233459=CARTESIAN_POINT('Ctrl Pts',(-7.73497830944983,-1.65955812141931,
102.710964733365));
#233460=CARTESIAN_POINT('Ctrl Pts',(-7.73708659056542,-1.64970109274918,
102.710557768769));
#233461=CARTESIAN_POINT('Ctrl Pts',(-7.74162646825939,-1.62827527626141,
102.709672598544));
#233462=CARTESIAN_POINT('Ctrl Pts',(-7.74405098329987,-1.61670501832905,
102.709194234072));
#233463=CARTESIAN_POINT('Ctrl Pts',(-7.75061729057285,-1.58501563038258,
102.707883116761));
#233464=CARTESIAN_POINT('Ctrl Pts',(-7.75470666316061,-1.56488577739826,
102.707049226575));
#233465=CARTESIAN_POINT('Ctrl Pts',(-7.77465135531449,-1.46471021113542,
102.70289464383));
#233466=CARTESIAN_POINT('Ctrl Pts',(-7.78934576149673,-1.38443924166108,
102.699550520324));
#233467=CARTESIAN_POINT('Ctrl Pts',(-7.87480650209391,-0.87304733133862,
102.678180618591));
#233468=CARTESIAN_POINT('Ctrl Pts',(-7.91099794134262,-0.436916952793712,
102.659700643657));
#233469=CARTESIAN_POINT('Ctrl Pts',(-7.91100187939347,0.39883330248103,
102.62470123059));
#233470=CARTESIAN_POINT('Ctrl Pts',(-7.88083747844167,0.797143536104756,
102.60819774669));
#233471=CARTESIAN_POINT('Ctrl Pts',(-7.81323238038289,1.24089423252288,
102.589989098022));
#233472=CARTESIAN_POINT('Ctrl Pts',(-7.80523718402587,1.29022915286847,
102.587966737174));
#233473=CARTESIAN_POINT('Ctrl Pts',(-7.79151592948249,1.37009680287536,
102.584695328422));
#233474=CARTESIAN_POINT('Ctrl Pts',(-7.78607661021762,1.40067724967215,
102.58344335199));
#233475=CARTESIAN_POINT('Ctrl Pts',(-7.77607457087018,1.45505056163304,
102.581218151917));
#233476=CARTESIAN_POINT('Ctrl Pts',(-7.77158239377341,1.47885596653092,
102.580244223992));
#233477=CARTESIAN_POINT('Ctrl Pts',(-7.76187149030842,1.52905054522422,
102.578191150712));
#233478=CARTESIAN_POINT('Ctrl Pts',(-7.75662736691001,1.55543450474728,
102.577112272865));
#233479=CARTESIAN_POINT('Ctrl Pts',(-7.74229560252635,1.62566442327177,
102.574240982736));
#233480=CARTESIAN_POINT('Ctrl Pts',(-7.73297008100907,1.66946092060796,
102.572450935911));
#233481=CARTESIAN_POINT('Ctrl Pts',(-7.68295317455581,1.89494518442984,
102.563235249841));
#233482=CARTESIAN_POINT('Ctrl Pts',(-7.6362284295309,2.07523569441124,102.555867671847));
#233483=CARTESIAN_POINT('Ctrl Pts',(-7.49972722740747,2.53452890355054,
102.53699703844));
#233484=CARTESIAN_POINT('Ctrl Pts',(-7.40073267581886,2.81049976478382,
102.525589659905));
#233485=CARTESIAN_POINT('Ctrl Pts',(-7.02146138931647,3.70767714527854,
102.488296404378));
#233486=CARTESIAN_POINT('Ctrl Pts',(-6.67638465996493,4.29809312752179,
102.463720830186));
#233487=CARTESIAN_POINT('Ctrl Pts',(-6.23457465709597,4.86987961159506,
102.436319917697));
#233488=CARTESIAN_POINT('Ctrl Pts',(-6.20890253554617,4.90256849530669,
102.434738169464));
#233489=CARTESIAN_POINT('Ctrl Pts',(-6.10195314371166,5.03656204672705,
102.428185914335));
#233490=CARTESIAN_POINT('Ctrl Pts',(-6.01844655447808,5.13605770748313,
102.423157561885));
#233491=CARTESIAN_POINT('Ctrl Pts',(-5.90440814510291,5.26532930148985,
102.416347424745));
#233492=CARTESIAN_POINT('Ctrl Pts',(-5.87602907808068,5.29698125276088,
102.414657098464));
#233493=CARTESIAN_POINT('Ctrl Pts',(-5.83945024768144,5.33712291348064,
102.412481937956));
#233494=CARTESIAN_POINT('Ctrl Pts',(-5.83148442588626,5.3458254346334,102.412008462973));
#233495=CARTESIAN_POINT('Ctrl Pts',(-5.81877741454235,5.35964542362705,
102.411253462516));
#233496=CARTESIAN_POINT('Ctrl Pts',(-5.8140488545878,5.36477451372134,102.410972572135));
#233497=CARTESIAN_POINT('Ctrl Pts',(-5.80520351071806,5.37434366795355,
102.410447234914));
#233498=CARTESIAN_POINT('Ctrl Pts',(-5.80108839944702,5.37878527584707,
102.410202873932));
#233499=CARTESIAN_POINT('Ctrl Pts',(-5.7919210052747,5.38865726162878,102.409658582466));
#233500=CARTESIAN_POINT('Ctrl Pts',(-5.78686618005038,5.39408526335588,
102.40935851925));
#233501=CARTESIAN_POINT('Ctrl Pts',(-5.77215563246439,5.4098373519546,102.408485408739));
#233502=CARTESIAN_POINT('Ctrl Pts',(-5.76247989330666,5.42014264533532,
102.407911293879));
#233503=CARTESIAN_POINT('Ctrl Pts',(-5.69327704984363,5.49345343175236,
102.403805859608));
#233504=CARTESIAN_POINT('Ctrl Pts',(-5.63274766968862,5.55550067434415,
102.400217473694));
#233505=CARTESIAN_POINT('Ctrl Pts',(-5.50115260115514,5.6860335944813,102.392401707212));
#233506=CARTESIAN_POINT('Ctrl Pts',(-5.42980399486493,5.75420588246586,
102.388160238178));
#233507=CARTESIAN_POINT('Ctrl Pts',(-5.2009692151596,5.96480698302112,102.374591413487));
#233508=CARTESIAN_POINT('Ctrl Pts',(-5.03901820523858,6.1022365583234,102.365039929599));
#233509=CARTESIAN_POINT('Ctrl Pts',(-4.72998454330482,6.34377959355142,
102.347158727323));
#233510=CARTESIAN_POINT('Ctrl Pts',(-4.58448810909778,6.44971013081252,
102.338869827913));
#233511=CARTESIAN_POINT('Ctrl Pts',(-4.21505235557019,6.69986107379129,
102.318311539271));
#233512=CARTESIAN_POINT('Ctrl Pts',(-3.98719583838662,6.83791494789822,
102.30605718336));
#233513=CARTESIAN_POINT('Ctrl Pts',(-3.34039932236877,7.18645409918913,
102.272862972789));
#233514=CARTESIAN_POINT('Ctrl Pts',(-2.90903097865722,7.37163620290902,
102.252513452378));
#233515=CARTESIAN_POINT('Ctrl Pts',(-2.43382828036063,7.52737624484211,
102.232159260673));
#233516=CARTESIAN_POINT('Ctrl Pts',(-2.40383661911475,7.53700754725137,
102.230882760506));
#233517=CARTESIAN_POINT('Ctrl Pts',(-2.36232313823307,7.55006588313637,
102.229126958453));
#233518=CARTESIAN_POINT('Ctrl Pts',(-2.35085002852569,7.55364611257992,
102.228642872158));
#233519=CARTESIAN_POINT('Ctrl Pts',(-2.33252782886062,7.55931784029084,
102.227871652406));
#233520=CARTESIAN_POINT('Ctrl Pts',(-2.32568400180237,7.56142620191684,
102.227583992884));
#233521=CARTESIAN_POINT('Ctrl Pts',(-2.31161823966552,7.56573850509155,
102.226993623821));
#233522=CARTESIAN_POINT('Ctrl Pts',(-2.30439599164131,7.56794140618736,
102.226690946953));
#233523=CARTESIAN_POINT('Ctrl Pts',(-2.2876884973557,7.57301132498179,102.225991803485));
#233524=CARTESIAN_POINT('Ctrl Pts',(-2.27820098751611,7.57587087077092,
102.225595570017));
#233525=CARTESIAN_POINT('Ctrl Pts',(-2.24838926943168,7.58479508919877,
102.224352965685));
#233526=CARTESIAN_POINT('Ctrl Pts',(-2.22804595622366,7.59079587905936,
102.223508583431));
#233527=CARTESIAN_POINT('Ctrl Pts',(-1.93967888770246,7.67459813288947,
102.21158930663));
#233528=CARTESIAN_POINT('Ctrl Pts',(-1.66773477143276,7.73824839675354,
102.200967327439));
#233529=CARTESIAN_POINT('Ctrl Pts',(-1.04120858234931,7.85031891247838,
102.177558147338));
#233530=CARTESIAN_POINT('Ctrl Pts',(-0.685569232694082,7.88933668721038,
102.165033497741));
#233531=CARTESIAN_POINT('Ctrl Pts',(0.200288488043677,7.92615338159678,
102.134329103512));
#233532=CARTESIAN_POINT('Ctrl Pts',(0.729912487050044,7.89500940809927,
102.1164249202));
#233533=CARTESIAN_POINT('Ctrl Pts',(1.25961206677603,7.81008012785519,102.096281326143));
#233534=CARTESIAN_POINT('Ctrl Pts',(1.2668097509104,7.80891587974101,102.096007175324));
#233535=CARTESIAN_POINT('Ctrl Pts',(1.4124556869612,7.78515052287668,102.090450744091));
#233536=CARTESIAN_POINT('Ctrl Pts',(1.55027814469175,7.75888119596976,102.085026916877));
#233537=CARTESIAN_POINT('Ctrl Pts',(1.70170778145885,7.72582216769708,102.078829765815));
#233538=CARTESIAN_POINT('Ctrl Pts',(1.71607562164115,7.72264345912536,102.078239515518));
#233539=CARTESIAN_POINT('Ctrl Pts',(1.7370121538997,7.71795019533945,102.077376206797));
#233540=CARTESIAN_POINT('Ctrl Pts',(1.74358796998982,7.71646728957164,102.077104593953));
#233541=CARTESIAN_POINT('Ctrl Pts',(1.75520785429415,7.71383128934848,102.07662382984));
#233542=CARTESIAN_POINT('Ctrl Pts',(1.76025270800759,7.71268164622881,102.076414833685));
#233543=CARTESIAN_POINT('Ctrl Pts',(1.77069669266934,7.71029084494988,102.07598161241));
#233544=CARTESIAN_POINT('Ctrl Pts',(1.77609565399494,7.70904896331476,102.075757355286));
#233545=CARTESIAN_POINT('Ctrl Pts',(1.78994617449935,7.70584771199722,102.075181268141));
#233546=CARTESIAN_POINT('Ctrl Pts',(1.79839580930444,7.70388011201673,102.07482907832));
#233547=CARTESIAN_POINT('Ctrl Pts',(1.83308879923478,7.69574124130955,102.073380033605));
#233548=CARTESIAN_POINT('Ctrl Pts',(1.85930356880884,7.68944978614791,102.072278040451));
#233549=CARTESIAN_POINT('Ctrl Pts',(2.28203767147829,7.58570691828012,102.054398901662));
#233550=CARTESIAN_POINT('Ctrl Pts',(2.67044368233444,7.45783788462449,102.036466466933));
#233551=CARTESIAN_POINT('Ctrl Pts',(3.44286892389733,7.13543148933909,101.999609686033));
#233552=CARTESIAN_POINT('Ctrl Pts',(3.82445678386896,6.93839271341209,101.980754192444));
#233553=CARTESIAN_POINT('Ctrl Pts',(4.42631998245801,6.56280349170204,101.950621160848));
#233554=CARTESIAN_POINT('Ctrl Pts',(4.65636340831698,6.4016397219293,101.938981919964));
#233555=CARTESIAN_POINT('Ctrl Pts',(4.90521568994917,6.20677302409815,101.926188403912));
#233556=CARTESIAN_POINT('Ctrl Pts',(4.93292050130342,6.18477709298296,101.924760940064));
#233557=CARTESIAN_POINT('Ctrl Pts',(4.97332711524278,6.15225247519126,101.922673985416));
#233558=CARTESIAN_POINT('Ctrl Pts',(4.98614488966889,6.14186879177211,101.922011209933));
#233559=CARTESIAN_POINT('Ctrl Pts',(5.00886148136085,6.12334809181335,101.920835198596));
#233560=CARTESIAN_POINT('Ctrl Pts',(5.01877317113523,6.11522698276815,101.920321607922));
#233561=CARTESIAN_POINT('Ctrl Pts',(5.03836342062967,6.0990960700042,101.919305537106));
#233562=CARTESIAN_POINT('Ctrl Pts',(5.04804271775977,6.09108722234195,101.91880303773));
#233563=CARTESIAN_POINT('Ctrl Pts',(5.07361051612564,6.06982910104522,101.917474401017));
#233564=CARTESIAN_POINT('Ctrl Pts',(5.08946621847528,6.05654048122313,101.916649133686));
#233565=CARTESIAN_POINT('Ctrl Pts',(5.12366176531408,6.02765217987515,101.914866288702));
#233566=CARTESIAN_POINT('Ctrl Pts',(5.14198291557133,6.01203063773482,101.913909181455));
#233567=CARTESIAN_POINT('Ctrl Pts',(5.19371847814885,5.9675087845616,101.911200850268));
#233568=CARTESIAN_POINT('Ctrl Pts',(5.22696265822815,5.93841175193622,101.909453864303));
#233569=CARTESIAN_POINT('Ctrl Pts',(5.52036923748019,5.67723431109448,101.893974210245));
#233570=CARTESIAN_POINT('Ctrl Pts',(5.76517584834386,5.42846488015547,101.880649165779));
#233571=CARTESIAN_POINT('Ctrl Pts',(6.45725438298539,4.6253671540124,101.840972210185));
#233572=CARTESIAN_POINT('Ctrl Pts',(6.84685192552972,4.02624094089903,101.815902131309));
#233573=CARTESIAN_POINT('Ctrl Pts',(7.18517506317434,3.31112301665101,101.784986786309));
#233574=CARTESIAN_POINT('Ctrl Pts',(7.21817601057139,3.23855073962787,101.781835454439));
#233575=CARTESIAN_POINT('Ctrl Pts',(7.2553048004979,3.1535129856508,101.778115831283));
#233576=CARTESIAN_POINT('Ctrl Pts',(7.26050601423933,3.14151942751638,101.777590602707));
#233577=CARTESIAN_POINT('Ctrl Pts',(7.26874780859433,3.12238475129894,101.776751592231));
#233578=CARTESIAN_POINT('Ctrl Pts',(7.27180766180947,3.11525192708304,101.776438601797));
#233579=CARTESIAN_POINT('Ctrl Pts',(7.27718527533521,3.10266507810156,101.775885861194));
#233580=CARTESIAN_POINT('Ctrl Pts',(7.27950741625484,3.0972129237221,101.775646293822));
#233581=CARTESIAN_POINT('Ctrl Pts',(7.28429171179521,3.08594477357375,101.775150873258));
#233582=CARTESIAN_POINT('Ctrl Pts',(7.28675303170178,3.08012842958827,101.774894985129));
#233583=CARTESIAN_POINT('Ctrl Pts',(7.29302770226996,3.06525114409266,101.77424003234));
#233584=CARTESIAN_POINT('Ctrl Pts',(7.29683112650615,3.05618604677874,101.773840544676));
#233585=CARTESIAN_POINT('Ctrl Pts',(7.31220815353637,3.01934403891531,101.772215231213));
#233586=CARTESIAN_POINT('Ctrl Pts',(7.32364002342858,2.99150852884265,101.770983254459));
#233587=CARTESIAN_POINT('Ctrl Pts',(7.39400863805198,2.81734665774431,101.76324690483));
#233588=CARTESIAN_POINT('Ctrl Pts',(7.44870777131684,2.66937232956217,101.756528986003));
#233589=CARTESIAN_POINT('Ctrl Pts',(7.55034841383505,2.36689721658937,101.742578557181));
#233590=CARTESIAN_POINT('Ctrl Pts',(7.59705694754,2.21239364416783,101.735351855512));
#233591=CARTESIAN_POINT('Ctrl Pts',(7.74818226930986,1.65104929743155,101.708985866782));
#233592=CARTESIAN_POINT('Ctrl Pts',(7.82489407101931,1.23747193192573,101.689394229412));
#233593=CARTESIAN_POINT('Ctrl Pts',(7.91789163871733,0.344833207250371,
101.648678974404));
#233594=CARTESIAN_POINT('Ctrl Pts',(7.92427681924457,-0.133634858413372,
101.627825307441));
#233595=CARTESIAN_POINT('Ctrl Pts',(7.88508760549069,-0.640517685923892,
101.607160831464));
#233596=CARTESIAN_POINT('Ctrl Pts',(7.88253435228384,-0.67120910767514,
101.605914841393));
#233597=CARTESIAN_POINT('Ctrl Pts',(7.87879480672726,-0.713191590711058,
101.604217552401));
#233598=CARTESIAN_POINT('Ctrl Pts',(7.87776335400397,-0.724495956737221,
101.603761237555));
#233599=CARTESIAN_POINT('Ctrl Pts',(7.87608884883206,-0.742421509477063,
101.603038761364));
#233600=CARTESIAN_POINT('Ctrl Pts',(7.87546177138539,-0.749044151009626,
101.602772081318));
#233601=CARTESIAN_POINT('Ctrl Pts',(7.87423027473622,-0.761877627958302,
101.60225576882));
#233602=CARTESIAN_POINT('Ctrl Pts',(7.87362685891368,-0.76808855374721,
101.602006103922));
#233603=CARTESIAN_POINT('Ctrl Pts',(7.87217370794623,-0.782864091843354,
101.601412662297));
#233604=CARTESIAN_POINT('Ctrl Pts',(7.87131734290475,-0.791428052501767,
101.601069101744));
#233605=CARTESIAN_POINT('Ctrl Pts',(7.86873647369019,-0.816819093280207,
101.60005167175));
#233606=CARTESIAN_POINT('Ctrl Pts',(7.86697196910218,-0.833642108832534,
101.599379107306));
#233607=CARTESIAN_POINT('Ctrl Pts',(7.85240618867708,-0.968348243311931,
101.594005944533));
#233608=CARTESIAN_POINT('Ctrl Pts',(7.83700965915583,-1.08593850964951,
101.589390895411));
#233609=CARTESIAN_POINT('Ctrl Pts',(7.77286734457607,-1.50278645074296,
101.573273389498));
#233610=CARTESIAN_POINT('Ctrl Pts',(7.70957128178513,-1.79954562662366,
101.562258176574));
#233611=CARTESIAN_POINT('Ctrl Pts',(7.54094529476901,-2.41452676150146,
101.539892668084));
#233612=CARTESIAN_POINT('Ctrl Pts',(7.43212754990713,-2.73116889940196,
101.52864950722));
#233613=CARTESIAN_POINT('Ctrl Pts',(7.11194622163099,-3.50041007324661,
101.500650247815));
#233614=CARTESIAN_POINT('Ctrl Pts',(6.87720564042173,-3.94164935676828,
101.483978674308));
#233615=CARTESIAN_POINT('Ctrl Pts',(6.54343090002309,-4.44735243440443,
101.461005824069));
#233616=CARTESIAN_POINT('Ctrl Pts',(6.48251811389525,-4.53567950711822,
101.456835107277));
#233617=CARTESIAN_POINT('Ctrl Pts',(6.41374667588285,-4.63118591508616,
101.452118980389));
#233618=CARTESIAN_POINT('Ctrl Pts',(6.40764605564784,-4.63962298317432,
101.45170055808));
#233619=CARTESIAN_POINT('Ctrl Pts',(6.39857649093828,-4.65211405052788,
101.451078377201));
#233620=CARTESIAN_POINT('Ctrl Pts',(6.39562028900442,-4.65617733426838,
101.45087555884));
#233621=CARTESIAN_POINT('Ctrl Pts',(6.39055905157771,-4.66312006394169,
101.450528279605));
#233622=CARTESIAN_POINT('Ctrl Pts',(6.38845593314939,-4.66600091219,101.450383961609));
#233623=CARTESIAN_POINT('Ctrl Pts',(6.38436565832623,-4.6715958146759,101.450103258707));
#233624=CARTESIAN_POINT('Ctrl Pts',(6.3823787178263,-4.67431002577608,101.449966890001));
#233625=CARTESIAN_POINT('Ctrl Pts',(6.37762800742196,-4.6807909401577,101.449640808239));
#233626=CARTESIAN_POINT('Ctrl Pts',(6.37486264897097,-4.68455643932611,
101.449450974682));
#233627=CARTESIAN_POINT('Ctrl Pts',(6.36646991971447,-4.69596335369723,
101.448874764895));
#233628=CARTESIAN_POINT('Ctrl Pts',(6.36083217682909,-4.70359703572875,
101.448487602911));
#233629=CARTESIAN_POINT('Ctrl Pts',(6.30634394596092,-4.77709870130758,
101.444744948415));
#233630=CARTESIAN_POINT('Ctrl Pts',(6.25648745007733,-4.84221125115305,
101.441314497804));
#233631=CARTESIAN_POINT('Ctrl Pts',(6.04709338346306,-5.10704623643425,
101.42692937531));
#233632=CARTESIAN_POINT('Ctrl Pts',(5.87894232339324,-5.29974324115202,
101.415433776848));
#233633=CARTESIAN_POINT('Ctrl Pts',(5.38839993552569,-5.80977022876024,
101.382909401637));
#233634=CARTESIAN_POINT('Ctrl Pts',(5.04767316277967,-6.1081341353459,101.361453787479));
#233635=CARTESIAN_POINT('Ctrl Pts',(4.29437812931619,-6.66146616863703,
101.31862644187));
#233636=CARTESIAN_POINT('Ctrl Pts',(3.88007721994675,-6.91100077140361,
101.297469322006));
#233637=CARTESIAN_POINT('Ctrl Pts',(3.4157194414029,-7.13567658226366,101.276513985717));
#233638=CARTESIAN_POINT('Ctrl Pts',(3.3857926746578,-7.14992500596311,101.275174590178));
#233639=CARTESIAN_POINT('Ctrl Pts',(3.34544088367246,-7.168826722035,101.273383388001));
#233640=CARTESIAN_POINT('Ctrl Pts',(3.33509428821022,-7.17364603022635,
101.272925405188));
#233641=CARTESIAN_POINT('Ctrl Pts',(3.31885505554017,-7.1811673245369,101.272208616958));
#233642=CARTESIAN_POINT('Ctrl Pts',(3.31296948657951,-7.18388447874465,
101.271949248665));
#233643=CARTESIAN_POINT('Ctrl Pts',(3.30167254460052,-7.18908303250905,
101.271452205972));
#233644=CARTESIAN_POINT('Ctrl Pts',(3.29626169898942,-7.19156556335742,
101.271214489748));
#233645=CARTESIAN_POINT('Ctrl Pts',(3.283557158442,-7.19737713806493,101.270657156856));
#233646=CARTESIAN_POINT('Ctrl Pts',(3.27626118810353,-7.20070120947605,
101.27033772433));
#233647=CARTESIAN_POINT('Ctrl Pts',(3.25520317792186,-7.21025668709693,
101.269417579976));
#233648=CARTESIAN_POINT('Ctrl Pts',(3.24142828893996,-7.21645978818696,
101.26881791364));
#233649=CARTESIAN_POINT('Ctrl Pts',(3.15046166060022,-7.25711082546121,
101.264872477449));
#233650=CARTESIAN_POINT('Ctrl Pts',(3.07273840968515,-7.29035976228189,
101.261570940128));
#233651=CARTESIAN_POINT('Ctrl Pts',(2.88724006504119,-7.36621975279476,
101.253847458992));
#233652=CARTESIAN_POINT('Ctrl Pts',(2.77903142017497,-7.40772126812446,
101.249465127804));
#233653=CARTESIAN_POINT('Ctrl Pts',(2.44335492168077,-7.52807291845652,
101.236210422009));
#233654=CARTESIAN_POINT('Ctrl Pts',(2.21316579638061,-7.59893223573594,
101.227598202347));
#233655=CARTESIAN_POINT('Ctrl Pts',(1.77359216019747,-7.71257318030026,
101.211741840146));
#233656=CARTESIAN_POINT('Ctrl Pts',(1.56501277292218,-7.75758672043848,
101.204459063132));
#233657=CARTESIAN_POINT('Ctrl Pts',(0.843337834297487,-7.88303692392558,
101.179553616392));
#233658=CARTESIAN_POINT('Ctrl Pts',(0.324348801329683,-7.92137482742682,
101.162206499269));
#233659=CARTESIAN_POINT('Ctrl Pts',(-0.289570996963616,-7.90626944439895,
101.138779869489));
#233660=CARTESIAN_POINT('Ctrl Pts',(-0.384498837347121,-7.90222166003217,
101.135072887155));
#233661=CARTESIAN_POINT('Ctrl Pts',(-0.490500094864129,-7.89578722828145,
101.13081544588));
#233662=CARTESIAN_POINT('Ctrl Pts',(-0.501671496325903,-7.89508530693915,
101.130365281096));
#233663=CARTESIAN_POINT('Ctrl Pts',(-0.517958829930785,-7.89402723258194,
101.129706811677));
#233664=CARTESIAN_POINT('Ctrl Pts',(-0.523075888615181,-7.89368981609708,
101.129499629186));
#233665=CARTESIAN_POINT('Ctrl Pts',(-0.532128305799828,-7.89308406298051,
101.129132568178));
#233666=CARTESIAN_POINT('Ctrl Pts',(-0.536063803374957,-7.89281775779167,
101.128972808994));
#233667=CARTESIAN_POINT('Ctrl Pts',(-0.544220148336621,-7.8922597100486,
101.128641334026));
#233668=CARTESIAN_POINT('Ctrl Pts',(-0.548440963185407,-7.89196752467198,
101.128469592478));
#233669=CARTESIAN_POINT('Ctrl Pts',(-0.559285397234625,-7.8912080783103,
101.128027812686));
#233670=CARTESIAN_POINT('Ctrl Pts',(-0.565908654739779,-7.8907358645897,
101.127757488203));
#233671=CARTESIAN_POINT('Ctrl Pts',(-0.593197575522974,-7.88875573081618,
101.126641640268));
#233672=CARTESIAN_POINT('Ctrl Pts',(-0.61385770409917,-7.88717497255999,
101.12579196133));
#233673=CARTESIAN_POINT('Ctrl Pts',(-0.753104107237202,-7.87597045092066,
101.120033393248));
#233674=CARTESIAN_POINT('Ctrl Pts',(-0.871461354364118,-7.86375411968934,
101.114982979528));
#233675=CARTESIAN_POINT('Ctrl Pts',(-1.08260098832937,-7.83713615329232,
101.105747771662));
#233676=CARTESIAN_POINT('Ctrl Pts',(-1.17549072621089,-7.82374261657887,
101.101606061657));
#233677=CARTESIAN_POINT('Ctrl Pts',(-1.53075431254588,-7.76604851520293,
101.085516908151));
#233678=CARTESIAN_POINT('Ctrl Pts',(-1.79106248980866,-7.71017525459716,
101.073209770356));
#233679=CARTESIAN_POINT('Ctrl Pts',(-2.28268868290962,-7.57840776136125,
101.049502601147));
#233680=CARTESIAN_POINT('Ctrl Pts',(-2.5143101455397,-7.50474374979458,
101.038128959809));
#233681=CARTESIAN_POINT('Ctrl Pts',(-3.28983456199195,-7.21815750692779,
100.999877728158));
#233682=CARTESIAN_POINT('Ctrl Pts',(-3.81347202669742,-6.95574799272295,
100.973920874342));
#233683=CARTESIAN_POINT('Ctrl Pts',(-4.33557801248443,-6.61726108430481,
100.948545863192));
#233684=CARTESIAN_POINT('Ctrl Pts',(-4.36748846147104,-6.59624329089312,
100.946996316995));
#233685=CARTESIAN_POINT('Ctrl Pts',(-4.40982095516389,-6.56791915650795,
100.944942244192));
#233686=CARTESIAN_POINT('Ctrl Pts',(-4.4203791717025,-6.5608178517136,100.94443006455));
#233687=CARTESIAN_POINT('Ctrl Pts',(-4.43681988137679,-6.5497023639132,
100.943632716053));
#233688=CARTESIAN_POINT('Ctrl Pts',(-4.44271414226381,-6.54570567365332,
100.943346892146));
#233689=CARTESIAN_POINT('Ctrl Pts',(-4.45395900011319,-6.53805874691654,
100.942801678425));
#233690=CARTESIAN_POINT('Ctrl Pts',(-4.45931052480181,-6.53440988892394,
100.942542237217));
#233691=CARTESIAN_POINT('Ctrl Pts',(-4.47178264438394,-6.52588350143272,
100.941937659609));
#233692=CARTESIAN_POINT('Ctrl Pts',(-4.47889975675041,-6.52100087888946,
100.941592715021));
#233693=CARTESIAN_POINT('Ctrl Pts',(-4.49916215136364,-6.50705124798289,
100.940610801492));
#233694=CARTESIAN_POINT('Ctrl Pts',(-4.51228802361258,-6.49795604816645,
100.939974894551));
#233695=CARTESIAN_POINT('Ctrl Pts',(-4.5945843211533,-6.44056156446588,
100.93598886539));
#233696=CARTESIAN_POINT('Ctrl Pts',(-4.66300714312354,-6.39119732710762,
100.932679179627));
#233697=CARTESIAN_POINT('Ctrl Pts',(-4.8633003566092,-6.24176496604875,
100.922994221195));
#233698=CARTESIAN_POINT('Ctrl Pts',(-4.99283644703769,-6.1386405678132,
100.91673605773));
#233699=CARTESIAN_POINT('Ctrl Pts',(-5.2203720428819,-5.94552765317669,
100.905688859674));
#233700=CARTESIAN_POINT('Ctrl Pts',(-5.31951653473187,-5.85698972296726,
100.900854958894));
#233701=CARTESIAN_POINT('Ctrl Pts',(-5.4754042868905,-5.71055389101984,
100.893180731596));
#233702=CARTESIAN_POINT('Ctrl Pts',(-5.53356892741414,-5.65421020308583,
100.890299810085));
#233703=CARTESIAN_POINT('Ctrl Pts',(-5.6301574641391,-5.55772735127853,
100.88547448177));
#233704=CARTESIAN_POINT('Ctrl Pts',(-5.66904172099806,-5.51805875374475,
100.883520213622));
#233705=CARTESIAN_POINT('Ctrl Pts',(-5.82426224927152,-5.35633465765741,
100.87566179634));
#233706=CARTESIAN_POINT('Ctrl Pts',(-5.93710100204922,-5.23098309301972,
100.869817809879));
#233707=CARTESIAN_POINT('Ctrl Pts',(-6.40439639780243,-4.67725316296863,
100.844713339013));
#233708=CARTESIAN_POINT('Ctrl Pts',(-6.71716813747526,-4.21576381357372,
100.825549076382));
#233709=CARTESIAN_POINT('Ctrl Pts',(-6.99909288721042,-3.6876070460383,
100.801926127745));
#233710=CARTESIAN_POINT('Ctrl Pts',(-7.01890916942798,-3.64974806723266,
100.80022659775));
#233711=CARTESIAN_POINT('Ctrl Pts',(-7.04424482897284,-3.60037480095434,
100.798003637669));
#233712=CARTESIAN_POINT('Ctrl Pts',(-7.05004463053605,-3.58900468418872,
100.797491266714));
#233713=CARTESIAN_POINT('Ctrl Pts',(-7.05924784888435,-3.57085401082569,
100.796672678039));
#233714=CARTESIAN_POINT('Ctrl Pts',(-7.06266908545917,-3.56408248325716,
100.796367137267));
#233715=CARTESIAN_POINT('Ctrl Pts',(-7.06880227926466,-3.55189976946472,
100.795817182549));
#233716=CARTESIAN_POINT('Ctrl Pts',(-7.07151777975968,-3.5464903673905,
100.795572900397));
#233717=CARTESIAN_POINT('Ctrl Pts',(-7.0778583946688,-3.53382333454048,
100.795000669654));
#233718=CARTESIAN_POINT('Ctrl Pts',(-7.08147855523264,-3.52656324003484,
100.794672540845));
#233719=CARTESIAN_POINT('Ctrl Pts',(-7.09183220061157,-3.50571917055118,
100.793730043452));
#233720=CARTESIAN_POINT('Ctrl Pts',(-7.09853779442751,-3.49212142431141,
100.793114683854));
#233721=CARTESIAN_POINT('Ctrl Pts',(-7.14228136989907,-3.40277066038664,
100.789068090054));
#233722=CARTESIAN_POINT('Ctrl Pts',(-7.17814465131622,-3.32645008950581,
100.785597243056));
#233723=CARTESIAN_POINT('Ctrl Pts',(-7.29088143511305,-3.07621849122254,
100.774196362235));
#233724=CARTESIAN_POINT('Ctrl Pts',(-7.36270576718467,-2.90010908661768,
100.766141509891));
#233725=CARTESIAN_POINT('Ctrl Pts',(-7.55347100807023,-2.37944768237302,
100.74245318307));
#233726=CARTESIAN_POINT('Ctrl Pts',(-7.65503992796993,-2.02905456234268,
100.726689666936));
#233727=CARTESIAN_POINT('Ctrl Pts',(-7.85114185618216,-1.12268161320065,
100.687022433179));
#233728=CARTESIAN_POINT('Ctrl Pts',(-7.91111634621678,-0.561322702383242,
100.663574107347));
#233729=CARTESIAN_POINT('Ctrl Pts',(-7.91099983056044,0.00163733706294327,
100.640435112007));
#233730=CARTESIAN_POINT('',(-7.91099993049747,-0.00104838700544144,96.6489168813118));
#233731=CARTESIAN_POINT('Ctrl Pts',(-7.91099982986448,0.00164069624814921,
100.640434973936));
#233732=CARTESIAN_POINT('Ctrl Pts',(-7.91096023546984,0.19255430968084,
100.632587971187));
#233733=CARTESIAN_POINT('Ctrl Pts',(-7.90400977593744,0.383408260987037,
100.624780623492));
#233734=CARTESIAN_POINT('Ctrl Pts',(-7.8873653218863,0.612270292793292,
100.615476921052));
#233735=CARTESIAN_POINT('Ctrl Pts',(-7.88428860421902,0.650691828228059,
100.613916925416));
#233736=CARTESIAN_POINT('Ctrl Pts',(-7.87877355984505,0.713765910890866,
100.611359113911));
#233737=CARTESIAN_POINT('Ctrl Pts',(-7.87650001950903,0.738432143384031,
100.610359623253));
#233738=CARTESIAN_POINT('Ctrl Pts',(-7.87223995113123,0.782390741714969,
100.608579777024));
#233739=CARTESIAN_POINT('Ctrl Pts',(-7.87029826045928,0.801687229967151,
100.607798954133));
#233740=CARTESIAN_POINT('Ctrl Pts',(-7.86625559152413,0.840432403845676,
100.606232088795));
#233741=CARTESIAN_POINT('Ctrl Pts',(-7.86415339494466,0.859880828874222,
100.605446065014));
#233742=CARTESIAN_POINT('Ctrl Pts',(-7.85950111331594,0.901476706684397,
100.603765929368));
#233743=CARTESIAN_POINT('Ctrl Pts',(-7.85692949952443,0.923621592483535,
100.602872060322));
#233744=CARTESIAN_POINT('Ctrl Pts',(-7.84983281857965,0.982557772622428,
100.60049468345));
#233745=CARTESIAN_POINT('Ctrl Pts',(-7.84514270547983,1.0193287026047,100.599013031406));
#233746=CARTESIAN_POINT('Ctrl Pts',(-7.82346948154017,1.1802299907184,100.592536243785));
#233747=CARTESIAN_POINT('Ctrl Pts',(-7.80379728290522,1.30398089468504,
100.587572388907));
#233748=CARTESIAN_POINT('Ctrl Pts',(-7.75836584760931,1.55167389131786,
100.577657856124));
#233749=CARTESIAN_POINT('Ctrl Pts',(-7.73255454181628,1.67556955297553,
100.572709248115));
#233750=CARTESIAN_POINT('Ctrl Pts',(-7.59159063495157,2.27928256392769,
100.548590938514));
#233751=CARTESIAN_POINT('Ctrl Pts',(-7.43469521165725,2.74821270809098,
100.529910196967));
#233752=CARTESIAN_POINT('Ctrl Pts',(-7.1695975457342,3.34769501792203,100.504413824522));
#233753=CARTESIAN_POINT('Ctrl Pts',(-7.09950850309346,3.49387574897339,
100.498053363241));
#233754=CARTESIAN_POINT('Ctrl Pts',(-7.01533074305503,3.65643213440784,
100.490744838756));
#233755=CARTESIAN_POINT('Ctrl Pts',(-7.00560672173067,3.67502868588438,
100.489905178286));
#233756=CARTESIAN_POINT('Ctrl Pts',(-6.98979872709786,3.70496969744956,
100.488547308002));
#233757=CARTESIAN_POINT('Ctrl Pts',(-6.9837608580399,3.71633838355598,100.488030315602));
#233758=CARTESIAN_POINT('Ctrl Pts',(-6.97302851061909,3.73642776950073,
100.487114230615));
#233759=CARTESIAN_POINT('Ctrl Pts',(-6.96834537976743,3.74515443662742,
100.486715452006));
#233760=CARTESIAN_POINT('Ctrl Pts',(-6.95880334648676,3.76285544933195,
100.485904891098));
#233761=CARTESIAN_POINT('Ctrl Pts',(-6.95394344125953,3.77182923296794,
100.485493083175));
#233762=CARTESIAN_POINT('Ctrl Pts',(-6.94443918135528,3.7892979812476,100.484689738828));
#233763=CARTESIAN_POINT('Ctrl Pts',(-6.93979656828717,3.79779387597702,
100.484298247024));
#233764=CARTESIAN_POINT('Ctrl Pts',(-6.92731576297593,3.82053421150891,
100.483248282758));
#233765=CARTESIAN_POINT('Ctrl Pts',(-6.91944924769304,3.83476302359058,
100.482589112759));
#233766=CARTESIAN_POINT('Ctrl Pts',(-6.89057304786241,3.88661562627595,
100.480179072825));
#233767=CARTESIAN_POINT('Ctrl Pts',(-6.86930001876524,3.92409163489703,
100.478422022591));
#233768=CARTESIAN_POINT('Ctrl Pts',(-6.64766062351281,4.3072208662608,100.46030956319));
#233769=CARTESIAN_POINT('Ctrl Pts',(-6.42169184364047,4.63739229359507,
100.44346866117));
#233770=CARTESIAN_POINT('Ctrl Pts',(-5.96602809492469,5.20562917588908,
100.412884643212));
#233771=CARTESIAN_POINT('Ctrl Pts',(-5.74449774991016,5.44911187076498,
100.399145479457));
#233772=CARTESIAN_POINT('Ctrl Pts',(-5.42666627675313,5.7574472525951,100.380916287786));
#233773=CARTESIAN_POINT('Ctrl Pts',(-5.34317300155922,5.83501572310704,
100.376250082258));
#233774=CARTESIAN_POINT('Ctrl Pts',(-5.21627036529305,5.94790456427658,
100.369332801011));
#233775=CARTESIAN_POINT('Ctrl Pts',(-5.17411546769705,5.98461146713653,
100.367062654732));
#233776=CARTESIAN_POINT('Ctrl Pts',(-5.1058083335103,6.04282950737379,100.363427290814));
#233777=CARTESIAN_POINT('Ctrl Pts',(-5.07990097745954,6.0646247423254,100.362058244942));
#233778=CARTESIAN_POINT('Ctrl Pts',(-5.0300631220844,6.10600870457515,100.359442930052));
#233779=CARTESIAN_POINT('Ctrl Pts',(-5.00615611258032,6.12562472717346,
100.358196316416));
#233780=CARTESIAN_POINT('Ctrl Pts',(-4.96361053217489,6.16011851997093,
100.355991590398));
#233781=CARTESIAN_POINT('Ctrl Pts',(-4.94501857496561,6.17505311657867,
100.355032754206));
#233782=CARTESIAN_POINT('Ctrl Pts',(-4.9081789387263,6.2043726831379,100.35314177561));
#233783=CARTESIAN_POINT('Ctrl Pts',(-4.88993484882807,6.21876177898432,
100.352209588863));
#233784=CARTESIAN_POINT('Ctrl Pts',(-4.84563703741152,6.25338395230157,
100.349956359648));
#233785=CARTESIAN_POINT('Ctrl Pts',(-4.81951961431992,6.27353487681995,
100.348636335107));
#233786=CARTESIAN_POINT('Ctrl Pts',(-4.71960596046138,6.34963118858123,
100.343617814228));
#233787=CARTESIAN_POINT('Ctrl Pts',(-4.64495512298455,6.4044428923088,100.339932770767));
#233788=CARTESIAN_POINT('Ctrl Pts',(-4.00382955789243,6.85807617367311,
100.308784172112));
#233789=CARTESIAN_POINT('Ctrl Pts',(-3.38815291966685,7.18222672768204,
100.282174738854));
#233790=CARTESIAN_POINT('Ctrl Pts',(-2.59522661509475,7.47475215743371,
100.25068241293));
#233791=CARTESIAN_POINT('Ctrl Pts',(-2.45083247678041,7.52333312808928,
100.245033985847));
#233792=CARTESIAN_POINT('Ctrl Pts',(-2.10295085362331,7.62929786193549,
100.231533932811));
#233793=CARTESIAN_POINT('Ctrl Pts',(-1.8983918469589,7.68275302980015,100.223683795367));
#233794=CARTESIAN_POINT('Ctrl Pts',(-1.53143011979826,7.7630948525063,100.209503204147));
#233795=CARTESIAN_POINT('Ctrl Pts',(-1.36986667422358,7.79322669320617,
100.203225893888));
#233796=CARTESIAN_POINT('Ctrl Pts',(-1.133747753138,7.82969375200893,100.193883556768));
#233797=CARTESIAN_POINT('Ctrl Pts',(-1.05985207079162,7.84003835478334,
100.190935869139));
#233798=CARTESIAN_POINT('Ctrl Pts',(-0.972312000439411,7.8510327847856,
100.187405704028));
#233799=CARTESIAN_POINT('Ctrl Pts',(-0.958797150394343,7.85269472446193,
100.186859625132));
#233800=CARTESIAN_POINT('Ctrl Pts',(-0.938023925078069,7.85519480991179,
100.186018532465));
#233801=CARTESIAN_POINT('Ctrl Pts',(-0.930768530941449,7.85605781082663,
100.185724442232));
#233802=CARTESIAN_POINT('Ctrl Pts',(-0.917560494371384,7.85761030139283,
100.185188461757));
#233803=CARTESIAN_POINT('Ctrl Pts',(-0.911608239238141,7.85830308191866,
100.18494669616));
#233804=CARTESIAN_POINT('Ctrl Pts',(-0.899573157417448,7.85968998225093,
100.184457399832));
#233805=CARTESIAN_POINT('Ctrl Pts',(-0.893490301216162,7.86038380513328,
100.184209857895));
#233806=CARTESIAN_POINT('Ctrl Pts',(-0.876143865552452,7.86234197894077,
100.18350325106));
#233807=CARTESIAN_POINT('Ctrl Pts',(-0.86487839329727,7.86358918242859,
100.183043518891));
#233808=CARTESIAN_POINT('Ctrl Pts',(-0.816829930576569,7.86880414023008,
100.181079026328));
#233809=CARTESIAN_POINT('Ctrl Pts',(-0.780022424271394,7.8725380078429,
100.179564924014));
#233810=CARTESIAN_POINT('Ctrl Pts',(-0.224304485055795,7.92497625101821,
100.15654980273));
#233811=CARTESIAN_POINT('Ctrl Pts',(0.298060922999434,7.9225331701876,100.132655270803));
#233812=CARTESIAN_POINT('Ctrl Pts',(1.06634897471536,7.84283261612408,100.097071085168));
#233813=CARTESIAN_POINT('Ctrl Pts',(1.31503426755326,7.80498641397619,100.085477695556));
#233814=CARTESIAN_POINT('Ctrl Pts',(1.85597674654879,7.69607071133398,100.060416919684));
#233815=CARTESIAN_POINT('Ctrl Pts',(2.14685390951061,7.62005203710519,100.047048990688));
#233816=CARTESIAN_POINT('Ctrl Pts',(2.62390216677596,7.46588418059872,100.025509850565));
#233817=CARTESIAN_POINT('Ctrl Pts',(2.81266930532603,7.39683634955653,100.017088756561));
#233818=CARTESIAN_POINT('Ctrl Pts',(3.0331269876078,7.30653494035904,100.007374046455));
#233819=CARTESIAN_POINT('Ctrl Pts',(3.0675418510025,7.29215326207337,100.005860975287));
#233820=CARTESIAN_POINT('Ctrl Pts',(3.11328449126638,7.27265667194257,100.003854320117));
#233821=CARTESIAN_POINT('Ctrl Pts',(3.12470350337861,7.26775779792038,100.003353757792));
#233822=CARTESIAN_POINT('Ctrl Pts',(3.14349753140918,7.25964248463101,100.002530507865));
#233823=CARTESIAN_POINT('Ctrl Pts',(3.15087924723518,7.25644166960989,100.002207314142));
#233824=CARTESIAN_POINT('Ctrl Pts',(3.16521909690143,7.25019770382553,100.001579767771));
#233825=CARTESIAN_POINT('Ctrl Pts',(3.17217775552793,7.24715578442172,100.001275375576));
#233826=CARTESIAN_POINT('Ctrl Pts',(3.18829898843479,7.24008085437079,100.00057049629));
#233827=CARTESIAN_POINT('Ctrl Pts',(3.19745831785828,7.23604045897654,100.000170250051));
#233828=CARTESIAN_POINT('Ctrl Pts',(3.22702408934927,7.22293120499226,99.9988790214673));
#233829=CARTESIAN_POINT('Ctrl Pts',(3.24739988830144,7.21379329068528,99.9979902922486));
#233830=CARTESIAN_POINT('Ctrl Pts',(3.43888197075628,7.12694381546557,99.9896488369977));
#233831=CARTESIAN_POINT('Ctrl Pts',(3.60721234484717,7.04324228866929,99.9823962327537));
#233832=CARTESIAN_POINT('Ctrl Pts',(4.15179580001342,6.74780032986943,99.9590748360825));
#233833=CARTESIAN_POINT('Ctrl Pts',(4.51371678957193,6.51126794739829,99.9438470014857));
#233834=CARTESIAN_POINT('Ctrl Pts',(5.137337119906,6.02660449699065,99.9164663258873));
#233835=CARTESIAN_POINT('Ctrl Pts',(5.40487010043764,5.7878806761234,99.9042473250419));
#233836=CARTESIAN_POINT('Ctrl Pts',(5.88871201849955,5.29324198779827,99.8796720404773));
#233837=CARTESIAN_POINT('Ctrl Pts',(6.10678053655651,5.04009540122998,99.8673918878904));
#233838=CARTESIAN_POINT('Ctrl Pts',(6.31704554425798,4.76225485964231,99.8534600037516));
#233839=CARTESIAN_POINT('Ctrl Pts',(6.32585640097968,4.75054486835573,99.8528721743785));
#233840=CARTESIAN_POINT('Ctrl Pts',(6.33870991425516,4.73336285403977,99.8520087892971));
#233841=CARTESIAN_POINT('Ctrl Pts',(6.34277816544282,4.72790994294913,99.8517346568589));
#233842=CARTESIAN_POINT('Ctrl Pts',(6.34992304013808,4.71830743690253,99.8512516996337));
#233843=CARTESIAN_POINT('Ctrl Pts',(6.35300264680384,4.71416005820049,99.8510430376621));
#233844=CARTESIAN_POINT('Ctrl Pts',(6.3589876728035,4.70608336710477,99.8506365538977));
#233845=CARTESIAN_POINT('Ctrl Pts',(6.36189351831942,4.70215437245911,99.8504387551703));
#233846=CARTESIAN_POINT('Ctrl Pts',(6.36884313030786,4.69273956530613,99.8499646431162));
#233847=CARTESIAN_POINT('Ctrl Pts',(6.37288344732606,4.68725122141114,99.84968814743));
#233848=CARTESIAN_POINT('Ctrl Pts',(6.38742618768309,4.66744288239805,99.8486898422931));
#233849=CARTESIAN_POINT('Ctrl Pts',(6.39788742897885,4.65309282118608,99.8479658975196));
#233850=CARTESIAN_POINT('Ctrl Pts',(6.59607267379569,4.37930309005527,99.8341415875694));
#233851=CARTESIAN_POINT('Ctrl Pts',(6.76791206266958,4.10874856729093,99.8202918854046));
#233852=CARTESIAN_POINT('Ctrl Pts',(7.28392490375116,3.17568071141,99.773568527802));
#233853=CARTESIAN_POINT('Ctrl Pts',(7.55086697149216,2.47490991569367,99.7405964551002));
#233854=CARTESIAN_POINT('Ctrl Pts',(7.72785658031028,1.69328082791274,99.7077940101454));
#233855=CARTESIAN_POINT('Ctrl Pts',(7.73948218054723,1.63932393455125,99.705545978589));
#233856=CARTESIAN_POINT('Ctrl Pts',(7.75617294865802,1.55772005116019,99.7021695033285));
#233857=CARTESIAN_POINT('Ctrl Pts',(7.7616569364702,1.53016083476523,99.7010332132753));
#233858=CARTESIAN_POINT('Ctrl Pts',(7.77028942712613,1.48553837139456,99.6991996670909));
#233859=CARTESIAN_POINT('Ctrl Pts',(7.77352881588373,1.46849303221902,99.6985007481623));
#233860=CARTESIAN_POINT('Ctrl Pts',(7.77950328594373,1.43648218407326,99.697190901113));
#233861=CARTESIAN_POINT('Ctrl Pts',(7.78225132278862,1.42151918453863,99.6965797419789));
#233862=CARTESIAN_POINT('Ctrl Pts',(7.78719022445499,1.39418337778344,99.6954652019882));
#233863=CARTESIAN_POINT('Ctrl Pts',(7.78939480403437,1.38181310988924,99.6949615797102));
#233864=CARTESIAN_POINT('Ctrl Pts',(7.79367717755843,1.35744806240517,99.6939710521882));
#233865=CARTESIAN_POINT('Ctrl Pts',(7.79575677550779,1.3454536365777,99.6934841167464));
#233866=CARTESIAN_POINT('Ctrl Pts',(7.80068641527391,1.31662596415432,99.6923154106822));
#233867=CARTESIAN_POINT('Ctrl Pts',(7.8035096696653,1.29978818154354,99.6916341021497));
#233868=CARTESIAN_POINT('Ctrl Pts',(7.81196278365642,1.24835374853814,99.6895568025498));
#233869=CARTESIAN_POINT('Ctrl Pts',(7.81741726274164,1.21372854269824,99.6881637263018));
#233870=CARTESIAN_POINT('Ctrl Pts',(7.8699728466667,0.865043447338463,99.6741866319982));
#233871=CARTESIAN_POINT('Ctrl Pts',(7.89835393063116,0.548445323193617,
99.6619342042612));
#233872=CARTESIAN_POINT('Ctrl Pts',(7.91355981181843,0.0278849011738598,
99.6422731571413));
#233873=CARTESIAN_POINT('Ctrl Pts',(7.91166564659692,-0.175372486071327,
99.6347132313587));
#233874=CARTESIAN_POINT('Ctrl Pts',(7.8832111618767,-0.769677659078231,
99.6127308376387));
#233875=CARTESIAN_POINT('Ctrl Pts',(7.83542876299146,-1.15908018817654,
99.5985028876602));
#233876=CARTESIAN_POINT('Ctrl Pts',(7.72328594211843,-1.7228713241323,99.5769567466913));
#233877=CARTESIAN_POINT('Ctrl Pts',(7.68135370557434,-1.90111347503911,
99.569997129403));
#233878=CARTESIAN_POINT('Ctrl Pts',(7.61171910769348,-2.15694033404288,
99.5596387933831));
#233879=CARTESIAN_POINT('Ctrl Pts',(7.58892865381696,-2.2358042651679,99.5563937149455));
#233880=CARTESIAN_POINT('Ctrl Pts',(7.5609307579242,-2.32732305800264,99.5525552474811));
#233881=CARTESIAN_POINT('Ctrl Pts',(7.55691231170079,-2.34033819197734,
99.5520076436016));
#233882=CARTESIAN_POINT('Ctrl Pts',(7.55073336070051,-2.36016902707431,
99.5511705683462));
#233883=CARTESIAN_POINT('Ctrl Pts',(7.5485971855968,-2.36699232147678,99.5508820625613));
#233884=CARTESIAN_POINT('Ctrl Pts',(7.54470016031182,-2.37938113100547,
99.5503573316974));
#233885=CARTESIAN_POINT('Ctrl Pts',(7.54294239308565,-2.38494761576678,
99.5501212310643));
#233886=CARTESIAN_POINT('Ctrl Pts',(7.53940962896568,-2.39609217524037,
99.5496478677686));
#233887=CARTESIAN_POINT('Ctrl Pts',(7.5376345988578,-2.40167023536674,99.5494106038559));
#233888=CARTESIAN_POINT('Ctrl Pts',(7.53260285631892,-2.41742204018513,
99.5487396353783));
#233889=CARTESIAN_POINT('Ctrl Pts',(7.52933173364635,-2.42759114238872,
99.548305334509));
#233890=CARTESIAN_POINT('Ctrl Pts',(7.51566860466237,-2.46977311584975,
99.5464990224979));
#233891=CARTESIAN_POINT('Ctrl Pts',(7.50509305138797,-2.50172581620905,
99.5451192383404));
#233892=CARTESIAN_POINT('Ctrl Pts',(7.47546495840238,-2.58936450532054,
99.5413011268957));
#233893=CARTESIAN_POINT('Ctrl Pts',(7.45599461415861,-2.64490626933408,
99.5388434919309));
#233894=CARTESIAN_POINT('Ctrl Pts',(7.41483006416666,-2.75826555426406,
99.5337437480003));
#233895=CARTESIAN_POINT('Ctrl Pts',(7.39307572047373,-2.81605483236703,
99.5310999296479));
#233896=CARTESIAN_POINT('Ctrl Pts',(7.32034902315607,-3.00259650935262,
99.5224361035409));
#233897=CARTESIAN_POINT('Ctrl Pts',(7.26667347405529,-3.13026348803249,
99.5163048980458));
#233898=CARTESIAN_POINT('Ctrl Pts',(7.17064345063041,-3.34287084919879,
99.5058269500449));
#233899=CARTESIAN_POINT('Ctrl Pts',(7.13005949495648,-3.42858047214099,
99.5015275139111));
#233900=CARTESIAN_POINT('Ctrl Pts',(6.88998130185354,-3.91289596976146,
99.4768753221282));
#233901=CARTESIAN_POINT('Ctrl Pts',(6.6586083678323,-4.29482940987859,99.4560914384027));
#233902=CARTESIAN_POINT('Ctrl Pts',(6.21101513240632,-4.90982206506857,
99.4219182485195));
#233903=CARTESIAN_POINT('Ctrl Pts',(6.01068739264013,-5.15312788475656,
99.4081664314626));
#233904=CARTESIAN_POINT('Ctrl Pts',(5.71651722666356,-5.4698373363519,99.3900952982096));
#233905=CARTESIAN_POINT('Ctrl Pts',(5.63475595446019,-5.55402706363005,
99.385271299003));
#233906=CARTESIAN_POINT('Ctrl Pts',(5.53912969880361,-5.64820748531026,
99.3798499028787));
#233907=CARTESIAN_POINT('Ctrl Pts',(5.52707197193466,-5.66000715892489,
99.3791701996506));
#233908=CARTESIAN_POINT('Ctrl Pts',(5.50881265324479,-5.67776171276216,
99.3781467505668));
#233909=CARTESIAN_POINT('Ctrl Pts',(5.50263898623424,-5.68374516522876,
99.3778017136442));
#233910=CARTESIAN_POINT('Ctrl Pts',(5.49196857140927,-5.6940531374733,99.3772070839257));
#233911=CARTESIAN_POINT('Ctrl Pts',(5.48747644596681,-5.69838241757312,
99.37695727658));
#233912=CARTESIAN_POINT('Ctrl Pts',(5.47818135732832,-5.70731936333021,
99.3764414590151));
#233913=CARTESIAN_POINT('Ctrl Pts',(5.47337768998806,-5.71192629170408,
99.3761754820137));
#233914=CARTESIAN_POINT('Ctrl Pts',(5.46035216943453,-5.72438681984994,
99.3754558735074));
#233915=CARTESIAN_POINT('Ctrl Pts',(5.4521191748671,-5.73222877962892,99.3750027647687));
#233916=CARTESIAN_POINT('Ctrl Pts',(5.42143795171448,-5.76132686785586,
99.3733206128278));
#233917=CARTESIAN_POINT('Ctrl Pts',(5.39888195022409,-5.78246923543712,
99.3720966601603));
#233918=CARTESIAN_POINT('Ctrl Pts',(5.04709138507091,-6.10835949678001,
99.3532022000819));
#233919=CARTESIAN_POINT('Ctrl Pts',(4.69263200080543,-6.3847047074283,99.3368612160111));
#233920=CARTESIAN_POINT('Ctrl Pts',(3.88614493821585,-6.90982399311899,
99.3034611752654));
#233921=CARTESIAN_POINT('Ctrl Pts',(3.42941544221314,-7.1475084261507,99.2867281387099));
#233922=CARTESIAN_POINT('Ctrl Pts',(2.60105305861641,-7.48079302035889,
99.255968514802));
#233923=CARTESIAN_POINT('Ctrl Pts',(2.23953732057409,-7.5968514818461,99.2423844352822));
#233924=CARTESIAN_POINT('Ctrl Pts',(1.85981077478459,-7.6892887085244,99.2267247401516));
#233925=CARTESIAN_POINT('Ctrl Pts',(1.84847536837143,-7.69202156592872,
99.2262560152875));
#233926=CARTESIAN_POINT('Ctrl Pts',(1.83214727308278,-7.69591993558362,
99.2255789765829));
#233927=CARTESIAN_POINT('Ctrl Pts',(1.82715938058704,-7.697105682194,99.2253719052564));
#233928=CARTESIAN_POINT('Ctrl Pts',(1.81849337666459,-7.69915690947033,
99.225011698268));
#233929=CARTESIAN_POINT('Ctrl Pts',(1.81481578590579,-7.70002460650264,
99.224858699838));
#233930=CARTESIAN_POINT('Ctrl Pts',(1.80773920795675,-7.70168891502091,
99.2245640269751));
#233931=CARTESIAN_POINT('Ctrl Pts',(1.80434031152366,-7.70248591221495,
99.2244223766094));
#233932=CARTESIAN_POINT('Ctrl Pts',(1.7963091734363,-7.70436350251064,99.224087393977));
#233933=CARTESIAN_POINT('Ctrl Pts',(1.79167651200185,-7.70544216131351,
99.2238939413955));
#233934=CARTESIAN_POINT('Ctrl Pts',(1.77778162721461,-7.70866420781675,
99.2233130508399));
#233935=CARTESIAN_POINT('Ctrl Pts',(1.76851654688455,-7.71079506955878,
99.2229248334365));
#233936=CARTESIAN_POINT('Ctrl Pts',(1.67944262186945,-7.73111205921468,
99.2191842455526));
#233937=CARTESIAN_POINT('Ctrl Pts',(1.59936259321271,-7.74807457002135,
99.21575745885));
#233938=CARTESIAN_POINT('Ctrl Pts',(1.43020006478053,-7.78117233083112,
99.2084082275603));
#233939=CARTESIAN_POINT('Ctrl Pts',(1.34107442021528,-7.79702721544461,
99.2044722658504));
#233940=CARTESIAN_POINT('Ctrl Pts',(0.700655315249088,-7.89964870131146,
99.1758383943272));
#233941=CARTESIAN_POINT('Ctrl Pts',(0.141825726839241,-7.92939184287613,
99.1491257633281));
#233942=CARTESIAN_POINT('Ctrl Pts',(-0.973481152622563,-7.87073580655182,
99.0975471492314));
#233943=CARTESIAN_POINT('Ctrl Pts',(-1.52686931451837,-7.78235180979279,
99.0728578235253));
#233944=CARTESIAN_POINT('Ctrl Pts',(-2.08598445585518,-7.63105507017697,
99.049463581974));
#233945=CARTESIAN_POINT('Ctrl Pts',(-2.10554850234315,-7.6256801760249,
99.0486467751139));
#233946=CARTESIAN_POINT('Ctrl Pts',(-2.13380177437203,-7.61780104440447,
99.0474697323074));
#233947=CARTESIAN_POINT('Ctrl Pts',(-2.14250763910446,-7.61535710138263,
99.0471073921225));
#233948=CARTESIAN_POINT('Ctrl Pts',(-2.1576703064623,-7.61107252141526,
99.0464769234216));
#233949=CARTESIAN_POINT('Ctrl Pts',(-2.16412898211825,-7.60923858389849,
99.0462085611167));
#233950=CARTESIAN_POINT('Ctrl Pts',(-2.17658598708254,-7.60568428086476,
99.04569133181));
#233951=CARTESIAN_POINT('Ctrl Pts',(-2.18258462879476,-7.60396503659365,
99.0454424258822));
#233952=CARTESIAN_POINT('Ctrl Pts',(-2.19677609137676,-7.59987950731469,
99.0448539569747));
#233953=CARTESIAN_POINT('Ctrl Pts',(-2.20496714134393,-7.59750706663638,
99.0445146095644));
#233954=CARTESIAN_POINT('Ctrl Pts',(-2.23359623278323,-7.58916479068351,
99.0433295954024));
#233955=CARTESIAN_POINT('Ctrl Pts',(-2.25401408461351,-7.58312566606434,
99.0424863548141));
#233956=CARTESIAN_POINT('Ctrl Pts',(-2.50165455647137,-7.50879083467617,
99.0322815345335));
#233957=CARTESIAN_POINT('Ctrl Pts',(-2.7257267695169,-7.430386305272,99.0232843372393));
#233958=CARTESIAN_POINT('Ctrl Pts',(-3.36248708663502,-7.17488946805482,
98.9981342048862));
#233959=CARTESIAN_POINT('Ctrl Pts',(-3.76405924365229,-6.97260634749538,
98.9828461197481));
#233960=CARTESIAN_POINT('Ctrl Pts',(-4.44829276479744,-6.55151445461675,
98.9555519163607));
#233961=CARTESIAN_POINT('Ctrl Pts',(-4.73742075356699,-6.34558668965958,
98.9435402885199));
#233962=CARTESIAN_POINT('Ctrl Pts',(-5.13331199052824,-6.02143794191036,
98.9250121428385));
#233963=CARTESIAN_POINT('Ctrl Pts',(-5.25188040644678,-5.91830670462849,
98.9191615399376));
#233964=CARTESIAN_POINT('Ctrl Pts',(-5.41408500718829,-5.76850599128377,
98.9105930697671));
#233965=CARTESIAN_POINT('Ctrl Pts',(-5.46035168459495,-5.72473028919786,
98.9080811320816));
#233966=CARTESIAN_POINT('Ctrl Pts',(-5.51268111550295,-5.67400672767969,
98.9051542295632));
#233967=CARTESIAN_POINT('Ctrl Pts',(-5.51926752755478,-5.66760014321294,
98.9047842535048));
#233968=CARTESIAN_POINT('Ctrl Pts',(-5.5292703590938,-5.65783644499864,
98.904219971643));
#233969=CARTESIAN_POINT('Ctrl Pts',(-5.53269494532087,-5.65448765001137,
98.9040263546194));
#233970=CARTESIAN_POINT('Ctrl Pts',(-5.53889840986603,-5.64841044645443,
98.903674853146));
#233971=CARTESIAN_POINT('Ctrl Pts',(-5.54167832137827,-5.64568308964385,
98.9035170549776));
#233972=CARTESIAN_POINT('Ctrl Pts',(-5.54723310881171,-5.64022526074605,
98.9032011813543));
#233973=CARTESIAN_POINT('Ctrl Pts',(-5.55000798553273,-5.6374947907625,
98.9030431060562));
#233974=CARTESIAN_POINT('Ctrl Pts',(-5.55781025307834,-5.62980604018116,
98.9025978474072));
#233975=CARTESIAN_POINT('Ctrl Pts',(-5.5628330116419,-5.62484308610008,
98.9023102850551));
#233976=CARTESIAN_POINT('Ctrl Pts',(-5.58344643933767,-5.60442048115203,
98.9011263504067));
#233977=CARTESIAN_POINT('Ctrl Pts',(-5.59897922821195,-5.58890281309652,
98.9002253240061));
#233978=CARTESIAN_POINT('Ctrl Pts',(-5.86631334291494,-5.31959600633263,
98.8845666665892));
#233979=CARTESIAN_POINT('Ctrl Pts',(-6.10066765185181,-5.04911259935259,
98.8685226913661));
#233980=CARTESIAN_POINT('Ctrl Pts',(-6.69309835078859,-4.26365127268738,
98.8232132369111));
#233981=CARTESIAN_POINT('Ctrl Pts',(-7.00960794333514,-3.72045981521665,
98.7934149495998));
#233982=CARTESIAN_POINT('Ctrl Pts',(-7.35484544840114,-2.92380076940478,
98.75492403291));
#233983=CARTESIAN_POINT('Ctrl Pts',(-7.44075692707853,-2.69768646678838,
98.7444989868383));
#233984=CARTESIAN_POINT('Ctrl Pts',(-7.550036890349,-2.36487633127673,98.72989041988));
#233985=CARTESIAN_POINT('Ctrl Pts',(-7.58176676333027,-2.26108626392274,
98.7254343652156));
#233986=CARTESIAN_POINT('Ctrl Pts',(-7.61601334419074,-2.14022290563121,
98.7203565950744));
#233987=CARTESIAN_POINT('Ctrl Pts',(-7.62062124952954,-2.12375731209143,
98.7196672013442));
#233988=CARTESIAN_POINT('Ctrl Pts',(-7.62753875605779,-2.09872633275612,
98.7186227498849));
#233989=CARTESIAN_POINT('Ctrl Pts',(-7.62988737694411,-2.09017183761961,
98.7182664330955));
#233990=CARTESIAN_POINT('Ctrl Pts',(-7.63411346212787,-2.07467692449907,
98.7176221671726));
#233991=CARTESIAN_POINT('Ctrl Pts',(-7.63599586152115,-2.06773786947747,
98.7173340592915));
#233992=CARTESIAN_POINT('Ctrl Pts',(-7.63973606186033,-2.05387567444613,
98.7167593245844));
#233993=CARTESIAN_POINT('Ctrl Pts',(-7.64159391833699,-2.04695255649828,
98.7164726961863));
#233994=CARTESIAN_POINT('Ctrl Pts',(-7.64678290024241,-2.02751081094486,
98.7156689171046));
#233995=CARTESIAN_POINT('Ctrl Pts',(-7.65009269695545,-2.01498648679361,
98.7151524516002));
#233996=CARTESIAN_POINT('Ctrl Pts',(-7.66348630798549,-1.96379615665739,
98.7130468941747));
#233997=CARTESIAN_POINT('Ctrl Pts',(-7.67330793795192,-1.92506183944342,
98.7114662001646));
#233998=CARTESIAN_POINT('Ctrl Pts',(-7.83465082278898,-1.26790187120604,
98.6848547863644));
#233999=CARTESIAN_POINT('Ctrl Pts',(-7.91126395176661,-0.633492366055027,
98.6625003051799));
#234000=CARTESIAN_POINT('Ctrl Pts',(-7.91075951849226,0.580304530698811,
98.6204359102891));
#234001=CARTESIAN_POINT('Ctrl Pts',(-7.84739031158016,1.15557940886955,
98.6006317366358));
#234002=CARTESIAN_POINT('Ctrl Pts',(-7.71335515118168,1.757743456605,98.5762582055363));
#234003=CARTESIAN_POINT('Ctrl Pts',(-7.70440106902857,1.79658393760866,
98.5746717819013));
#234004=CARTESIAN_POINT('Ctrl Pts',(-7.69227254215473,1.84743562531875,
98.572577199154));
#234005=CARTESIAN_POINT('Ctrl Pts',(-7.68936269813695,1.85950975985054,
98.5720785621658));
#234006=CARTESIAN_POINT('Ctrl Pts',(-7.68482596966916,1.87814175921411,
98.5713071280592));
#234007=CARTESIAN_POINT('Ctrl Pts',(-7.68321908987238,1.88470450429724,
98.5710350280134));
#234008=CARTESIAN_POINT('Ctrl Pts',(-7.6800154285328,1.89771656496042,98.57049478961));
#234009=CARTESIAN_POINT('Ctrl Pts',(-7.67841892584772,1.90416594400465,
98.5702266609676));
#234010=CARTESIAN_POINT('Ctrl Pts',(-7.67484704966503,1.9185176865934,98.5696292010279));
#234011=CARTESIAN_POINT('Ctrl Pts',(-7.67286759325506,1.92641902123219,
98.5692997326672));
#234012=CARTESIAN_POINT('Ctrl Pts',(-7.66713118536377,1.9491677574386,98.568349633106));
#234013=CARTESIAN_POINT('Ctrl Pts',(-7.66334332624633,1.96400728635094,
98.5677279860783));
#234014=CARTESIAN_POINT('Ctrl Pts',(-7.63762184366257,2.06356786049756,
98.5635449985875));
#234015=CARTESIAN_POINT('Ctrl Pts',(-7.6143271519258,2.14792951666858,98.559940960607));
#234016=CARTESIAN_POINT('Ctrl Pts',(-7.53290945425882,2.42479444226227,
98.5479441496123));
#234017=CARTESIAN_POINT('Ctrl Pts',(-7.46884772032344,2.61546608751238,
98.5394126252318));
#234018=CARTESIAN_POINT('Ctrl Pts',(-7.18228964197923,3.37161084358709,
98.5048277067009));
#234019=CARTESIAN_POINT('Ctrl Pts',(-6.90223805758939,3.91308229123864,
98.4785408188109));
#234020=CARTESIAN_POINT('Ctrl Pts',(-6.35227453621796,4.73021506270681,
98.4372334871509));
#234021=CARTESIAN_POINT('Ctrl Pts',(-6.11943619234049,5.02780619090267,
98.4216783506842));
#234022=CARTESIAN_POINT('Ctrl Pts',(-5.76790613931722,5.41633309822399,
98.4002314792745));
#234023=CARTESIAN_POINT('Ctrl Pts',(-5.66656294665684,5.52227043042734,
98.3942629212634));
#234024=CARTESIAN_POINT('Ctrl Pts',(-5.53481890949836,5.65253907112872,
98.386770247152));
#234025=CARTESIAN_POINT('Ctrl Pts',(-5.50710436812444,5.67954397892837,
98.3852082756454));
#234026=CARTESIAN_POINT('Ctrl Pts',(-5.46285891864407,5.72202815476593,
98.3827369772734));
#234027=CARTESIAN_POINT('Ctrl Pts',(-5.44645781661382,5.73764159080866,
98.3818256973729));
#234028=CARTESIAN_POINT('Ctrl Pts',(-5.41692386788539,5.76551642164585,
98.3801932629011));
#234029=CARTESIAN_POINT('Ctrl Pts',(-5.40381587091827,5.77780389368341,
98.3794717259426));
#234030=CARTESIAN_POINT('Ctrl Pts',(-5.3730905909535,5.80640983352979,98.3777873636261));
#234031=CARTESIAN_POINT('Ctrl Pts',(-5.35544062395208,5.82269296644172,
98.3768250709696));
#234032=CARTESIAN_POINT('Ctrl Pts',(-5.30448889330591,5.86927128003635,
98.3740621746716));
#234033=CARTESIAN_POINT('Ctrl Pts',(-5.27100222259598,5.89936296373868,
98.3722646494586));
#234034=CARTESIAN_POINT('Ctrl Pts',(-5.018182867237,6.12267944868293,98.3588280874195));
#234035=CARTESIAN_POINT('Ctrl Pts',(-4.78854518601225,6.30390394360081,
98.347384382168));
#234036=CARTESIAN_POINT('Ctrl Pts',(-4.23922784188059,6.69003833336223,
98.3213739389234));
#234037=CARTESIAN_POINT('Ctrl Pts',(-3.91378536103238,6.88548817053646,
98.3069321195091));
#234038=CARTESIAN_POINT('Ctrl Pts',(-3.37027584951745,7.16087537501986,
98.2833691991164));
#234039=CARTESIAN_POINT('Ctrl Pts',(-3.16052785769293,7.25589094003613,
98.2743920270559));
#234040=CARTESIAN_POINT('Ctrl Pts',(-2.9239651804909,7.35084768426346,98.264196330924));
#234041=CARTESIAN_POINT('Ctrl Pts',(-2.9009441869084,7.359963102801,98.2632033756447));
#234042=CARTESIAN_POINT('Ctrl Pts',(-2.86635641441423,7.37347102613003,
98.2617100591796));
#234043=CARTESIAN_POINT('Ctrl Pts',(-2.85482152969534,7.37794470702236,
98.26121181385));
#234044=CARTESIAN_POINT('Ctrl Pts',(-2.83385991618032,7.38601792542614,
98.2603059996657));
#234045=CARTESIAN_POINT('Ctrl Pts',(-2.82443669508371,7.38962652466335,
98.2598986532406));
#234046=CARTESIAN_POINT('Ctrl Pts',(-2.80414202162799,7.39735382921292,
98.2590210746002));
#234047=CARTESIAN_POINT('Ctrl Pts',(-2.793268346663,7.4014666178071,98.258550703452));
#234048=CARTESIAN_POINT('Ctrl Pts',(-2.76347310470483,7.41266116696907,
98.2572613925988));
#234049=CARTESIAN_POINT('Ctrl Pts',(-2.74453345209575,7.41969442105172,
98.256441350015));
#234050=CARTESIAN_POINT('Ctrl Pts',(-2.64429797543389,7.45648063494276,
98.2520992652728));
#234051=CARTESIAN_POINT('Ctrl Pts',(-2.56254564372747,7.48496992095989,
98.248550527013));
#234052=CARTESIAN_POINT('Ctrl Pts',(-1.74597568241153,7.75458437176633,
98.2130885188211));
#234053=CARTESIAN_POINT('Ctrl Pts',(-0.979994912125664,7.88807472567979,
98.1800996860991));
#234054=CARTESIAN_POINT('Ctrl Pts',(-0.11266906910052,7.91075844304539,
98.1447001808409));
#234055=CARTESIAN_POINT('Ctrl Pts',(-0.0184703696052005,7.91153920400532,
98.140874882418));
#234056=CARTESIAN_POINT('Ctrl Pts',(0.112854666247831,7.91028216295921,
98.1355653958916));
#234057=CARTESIAN_POINT('Ctrl Pts',(0.149985983955524,7.9096652453795,98.1340667765302));
#234058=CARTESIAN_POINT('Ctrl Pts',(0.209845807586467,7.90824903923447,
98.1316547065531));
#234059=CARTESIAN_POINT('Ctrl Pts',(0.232577541969286,7.90761315569268,
98.1307396243286));
#234060=CARTESIAN_POINT('Ctrl Pts',(0.2798873420992,7.90608556337504,98.1288369007036));
#234061=CARTESIAN_POINT('Ctrl Pts',(0.304464636199621,7.90517723706595,
98.1278494343586));
#234062=CARTESIAN_POINT('Ctrl Pts',(0.362583305398953,7.90275784954741,
98.1255165253629));
#234063=CARTESIAN_POINT('Ctrl Pts',(0.396120120879567,7.90114783703582,
98.1241720635184));
#234064=CARTESIAN_POINT('Ctrl Pts',(0.50912983468625,7.89500121727345,98.1196467527056));
#234065=CARTESIAN_POINT('Ctrl Pts',(0.58854453687307,7.88947861837628,98.1164753329699));
#234066=CARTESIAN_POINT('Ctrl Pts',(1.4058058867571,7.82023655966428,98.0838966156612));
#234067=CARTESIAN_POINT('Ctrl Pts',(2.13136554546537,7.65439675169261,98.0555044122154));
#234068=CARTESIAN_POINT('Ctrl Pts',(3.27965524196717,7.21571060593309,98.0097666865299));
#234069=CARTESIAN_POINT('Ctrl Pts',(3.71888922375843,6.9994590252055,97.9919305696375));
#234070=CARTESIAN_POINT('Ctrl Pts',(4.20739686260769,6.69991615517711,97.9695994867845));
#234071=CARTESIAN_POINT('Ctrl Pts',(4.27873687350113,6.6545830104007,97.9662686094557));
#234072=CARTESIAN_POINT('Ctrl Pts',(4.360714858569,6.60062667585319,97.9623450994737));
#234073=CARTESIAN_POINT('Ctrl Pts',(4.37207501447554,6.59310751139124,97.9617992255817));
#234074=CARTESIAN_POINT('Ctrl Pts',(4.39013133139129,6.58108904169181,97.9609280440195));
#234075=CARTESIAN_POINT('Ctrl Pts',(4.39684015749924,6.57660875454432,97.9606035740156));
#234076=CARTESIAN_POINT('Ctrl Pts',(4.40865086101335,6.56869518262951,97.9600309538032));
#234077=CARTESIAN_POINT('Ctrl Pts',(4.41375561663168,6.56526619208987,97.9597829971299));
#234078=CARTESIAN_POINT('Ctrl Pts',(4.42428499844677,6.55817551511852,97.9592705819181));
#234079=CARTESIAN_POINT('Ctrl Pts',(4.42970908801492,6.55451304292014,97.9590060874393));
#234080=CARTESIAN_POINT('Ctrl Pts',(4.44355022691304,6.54514215382548,97.9583297838862));
#234081=CARTESIAN_POINT('Ctrl Pts',(4.45196080951082,6.53942423934994,97.9579175317485));
#234082=CARTESIAN_POINT('Ctrl Pts',(4.48598101578233,6.51619963353444,97.9562446562215));
#234083=CARTESIAN_POINT('Ctrl Pts',(4.51149836492469,6.49855874815916,97.9549775978314));
#234084=CARTESIAN_POINT('Ctrl Pts',(4.67020082270343,6.38745788995528,97.9470161588127));
#234085=CARTESIAN_POINT('Ctrl Pts',(4.80056165880585,6.29007078007476,97.9400957798574));
#234086=CARTESIAN_POINT('Ctrl Pts',(5.0105694808423,6.12285096499516,97.9283795543114));
#234087=CARTESIAN_POINT('Ctrl Pts',(5.09198896246024,6.05530822655395,97.9236909798669));
#234088=CARTESIAN_POINT('Ctrl Pts',(5.92484526801671,5.3357218490174,97.8743665997887));
#234089=CARTESIAN_POINT('Ctrl Pts',(6.54849355655855,4.54882784412921,97.8269174948143));
#234090=CARTESIAN_POINT('Ctrl Pts',(7.03460941131951,3.61953669074862,97.7839044136457));
#234091=CARTESIAN_POINT('Ctrl Pts',(7.05889369760388,3.57194559470995,97.7817293111931));
#234092=CARTESIAN_POINT('Ctrl Pts',(7.0892341465826,3.51096792056043,97.7789770680554));
#234093=CARTESIAN_POINT('Ctrl Pts',(7.09573739736807,3.49780607163347,97.7783850472086));
#234094=CARTESIAN_POINT('Ctrl Pts',(7.1060076491603,3.47687371902962,97.7774467335431));
#234095=CARTESIAN_POINT('Ctrl Pts',(7.10979861526511,3.4691150483896,97.7770996449198));
#234096=CARTESIAN_POINT('Ctrl Pts',(7.11684287507102,3.45463807229611,97.7764533121912));
#234097=CARTESIAN_POINT('Ctrl Pts',(7.12009937642411,3.44792134324858,97.7761539619172));
#234098=CARTESIAN_POINT('Ctrl Pts',(7.12730666041352,3.43300213477449,97.7754901991866));
#234099=CARTESIAN_POINT('Ctrl Pts',(7.13125280234399,3.42479741863431,97.7751259406742));
#234100=CARTESIAN_POINT('Ctrl Pts',(7.14262458273126,3.40104863639578,97.7740738110491));
#234101=CARTESIAN_POINT('Ctrl Pts',(7.15001364417631,3.38548706239659,97.7733871494345));
#234102=CARTESIAN_POINT('Ctrl Pts',(7.20007158751687,3.27916872577874,97.7687144354425));
#234103=CARTESIAN_POINT('Ctrl Pts',(7.24106301463303,3.18763010576617,97.7647838694452));
#234104=CARTESIAN_POINT('Ctrl Pts',(7.34321002655226,2.94737780978454,97.7546939204284));
#234105=CARTESIAN_POINT('Ctrl Pts',(7.40159291619605,2.79753372194274,97.748622991563));
#234106=CARTESIAN_POINT('Ctrl Pts',(7.63187235469365,2.14870062388225,97.723145516042));
#234107=CARTESIAN_POINT('Ctrl Pts',(7.75817701686813,1.63496272931137,97.7050806169576));
#234108=CARTESIAN_POINT('Ctrl Pts',(7.90389431250101,0.609046105023389,
97.6692394029842));
#234109=CARTESIAN_POINT('Ctrl Pts',(7.92668861058478,0.0999348723505103,
97.6515101950275));
#234110=CARTESIAN_POINT('Ctrl Pts',(7.89887480416477,-0.438943935195724,
97.6301551041058));
#234111=CARTESIAN_POINT('Ctrl Pts',(7.89708177687097,-0.470100303620692,
97.628911041364));
#234112=CARTESIAN_POINT('Ctrl Pts',(7.89451090860682,-0.510594041807843,
97.6272826608688));
#234113=CARTESIAN_POINT('Ctrl Pts',(7.8939007354984,-0.519942245465121,
97.6269059444848));
#234114=CARTESIAN_POINT('Ctrl Pts',(7.8928946411101,-0.534946097686244,
97.6263000617729));
#234115=CARTESIAN_POINT('Ctrl Pts',(7.89250924110129,-0.540602462055626,
97.62607136149));
#234116=CARTESIAN_POINT('Ctrl Pts',(7.89177204775266,-0.551253129868674,
97.6256401971175));
#234117=CARTESIAN_POINT('Ctrl Pts',(7.89142159289779,-0.556247525711506,
97.625437791544));
#234118=CARTESIAN_POINT('Ctrl Pts',(7.89080204757728,-0.564958343760852,
97.6250843914673));
#234119=CARTESIAN_POINT('Ctrl Pts',(7.89053507191685,-0.568674918575564,
97.6249334881673));
#234120=CARTESIAN_POINT('Ctrl Pts',(7.88962166897656,-0.581265941003144,
97.6244218509768));
#234121=CARTESIAN_POINT('Ctrl Pts',(7.88896289663079,-0.590139465232265,
97.6240605902673));
#234122=CARTESIAN_POINT('Ctrl Pts',(7.8861055456265,-0.627767454678214,
97.6225258225581));
#234123=CARTESIAN_POINT('Ctrl Pts',(7.88376473312284,-0.656510667787545,
97.6213463887688));
#234124=CARTESIAN_POINT('Ctrl Pts',(7.86570444006156,-0.864230520872862,
97.6127749223484));
#234125=CARTESIAN_POINT('Ctrl Pts',(7.84404957395355,-1.04263214272784,
97.6051567750496));
#234126=CARTESIAN_POINT('Ctrl Pts',(7.78432733841987,-1.42522089297506,
97.5884649572146));
#234127=CARTESIAN_POINT('Ctrl Pts',(7.74425435782694,-1.6289653605696,97.5793562952375));
#234128=CARTESIAN_POINT('Ctrl Pts',(7.60156699884515,-2.22875593543653,
97.5522195903049));
#234129=CARTESIAN_POINT('Ctrl Pts',(7.47620376402859,-2.61869773090331,
97.5341911939636));
#234130=CARTESIAN_POINT('Ctrl Pts',(7.20091743896093,-3.29113722886374,
97.5031479440812));
#234131=CARTESIAN_POINT('Ctrl Pts',(7.06299073186216,-3.57756580146288,
97.4899292018986));
#234132=CARTESIAN_POINT('Ctrl Pts',(6.89052104924574,-3.88663843036336,
97.4755994736329));
#234133=CARTESIAN_POINT('Ctrl Pts',(6.87261491027139,-3.91821425397549,
97.4741344588587));
#234134=CARTESIAN_POINT('Ctrl Pts',(6.84616946736213,-3.96410929476055,
97.4720031321892));
#234135=CARTESIAN_POINT('Ctrl Pts',(6.83780129532769,-3.97852640116299,
97.4713333309792));
#234136=CARTESIAN_POINT('Ctrl Pts',(6.82290663583917,-4.00400186264425,
97.4701492163409));
#234137=CARTESIAN_POINT('Ctrl Pts',(6.81639868405345,-4.01507096557286,
97.469634531202));
#234138=CARTESIAN_POINT('Ctrl Pts',(6.8028344951548,-4.03801369523629,97.4685673344463));
#234139=CARTESIAN_POINT('Ctrl Pts',(6.79577405242389,-4.04988478862642,
97.4680149089954));
#234140=CARTESIAN_POINT('Ctrl Pts',(6.77748307365309,-4.08045585650678,
97.4665916220001));
#234141=CARTESIAN_POINT('Ctrl Pts',(6.76620620198897,-4.09912801067916,
97.465721677794));
#234142=CARTESIAN_POINT('Ctrl Pts',(6.7201009909639,-4.17476000254316,97.4621950614631));
#234143=CARTESIAN_POINT('Ctrl Pts',(6.68462906274458,-4.23132519085822,
97.459550601175));
#234144=CARTESIAN_POINT('Ctrl Pts',(6.45728884726687,-4.58385741142495,
97.4430216263116));
#234145=CARTESIAN_POINT('Ctrl Pts',(6.24651789831679,-4.86717169079069,
97.4295475751767));
#234146=CARTESIAN_POINT('Ctrl Pts',(5.91429754827461,-5.25645286689566,
97.4104048282614));
#234147=CARTESIAN_POINT('Ctrl Pts',(5.80743553853075,-5.37428187207255,
97.4045137992596));
#234148=CARTESIAN_POINT('Ctrl Pts',(5.31623529636951,-5.88412160894045,
97.3784050879208));
#234149=CARTESIAN_POINT('Ctrl Pts',(4.89529163319778,-6.23869281471567,
97.3586364561451));
#234150=CARTESIAN_POINT('Ctrl Pts',(4.37641363173298,-6.59067753915491,
97.3341219362174));
#234151=CARTESIAN_POINT('Ctrl Pts',(4.31110396341263,-6.63358190113328,
97.3310320996757));
#234152=CARTESIAN_POINT('Ctrl Pts',(4.23324072961883,-6.6830976208728,97.3273329669173));
#234153=CARTESIAN_POINT('Ctrl Pts',(4.22129038384432,-6.69065231327108,
97.3267648059197));
#234154=CARTESIAN_POINT('Ctrl Pts',(4.20316790516017,-6.70204098425758,
97.3259024807639));
#234155=CARTESIAN_POINT('Ctrl Pts',(4.19701060101924,-6.70589858319689,
97.3256093713385));
#234156=CARTESIAN_POINT('Ctrl Pts',(4.18597430524439,-6.7127917541905,97.3250837675339));
#234157=CARTESIAN_POINT('Ctrl Pts',(4.18109729939925,-6.71583050649923,
97.3248514172835));
#234158=CARTESIAN_POINT('Ctrl Pts',(4.17158418683911,-6.72174353327335,
97.3243980255361));
#234159=CARTESIAN_POINT('Ctrl Pts',(4.16694840879681,-6.72461833215975,
97.3241770082256));
#234160=CARTESIAN_POINT('Ctrl Pts',(4.15419726639016,-6.73250748792315,
97.3235688575524));
#234161=CARTESIAN_POINT('Ctrl Pts',(4.14607581571627,-6.73751195414856,
97.3231812679069));
#234162=CARTESIAN_POINT('Ctrl Pts',(4.11422975906141,-6.75705621947615,
97.321660411413));
#234163=CARTESIAN_POINT('Ctrl Pts',(4.09043774722936,-6.7714853815049,97.3205219548706));
#234164=CARTESIAN_POINT('Ctrl Pts',(3.94713314485832,-6.85736460318705,
97.3136489570119));
#234165=CARTESIAN_POINT('Ctrl Pts',(3.82584460669583,-6.92576468231635,
97.3077515178323));
#234166=CARTESIAN_POINT('Ctrl Pts',(3.65800909225906,-7.01466045760386,
97.2995043446516));
#234167=CARTESIAN_POINT('Ctrl Pts',(3.61297598823876,-7.03796108349436,
97.2972843908482));
#234168=CARTESIAN_POINT('Ctrl Pts',(3.3912744158515,-7.14998333623823,97.2863318644217));
#234169=CARTESIAN_POINT('Ctrl Pts',(3.21155198915956,-7.23249142353882,
97.2773820831093));
#234170=CARTESIAN_POINT('Ctrl Pts',(2.4974465171754,-7.52845837444701,97.2420287634282));
#234171=CARTESIAN_POINT('Ctrl Pts',(1.94345023894368,-7.69012622675716,
97.2151970324276));
#234172=CARTESIAN_POINT('Ctrl Pts',(1.11296720159382,-7.8369004144202,97.1784567016048));
#234173=CARTESIAN_POINT('Ctrl Pts',(0.846919968658294,-7.87009843947016,
97.1671615363555));
#234174=CARTESIAN_POINT('Ctrl Pts',(0.557157220673652,-7.89138814892926,
97.1553923440016));
#234175=CARTESIAN_POINT('Ctrl Pts',(0.534625753112108,-7.89294662348092,
97.1544806030023));
#234176=CARTESIAN_POINT('Ctrl Pts',(0.503146392704338,-7.89498859990009,
97.1532115153219));
#234177=CARTESIAN_POINT('Ctrl Pts',(0.494203994516476,-7.8955534129998,
97.1528515363164));
#234178=CARTESIAN_POINT('Ctrl Pts',(0.47874625648298,-7.89650337930094,
97.1522301985457));
#234179=CARTESIAN_POINT('Ctrl Pts',(0.472231372786632,-7.89689566400964,
97.1519686087453));
#234180=CARTESIAN_POINT('Ctrl Pts',(0.458734057238549,-7.89769162361928,
97.151427238254));
#234181=CARTESIAN_POINT('Ctrl Pts',(0.451751558753382,-7.89809410215934,
97.1511474965939));
#234182=CARTESIAN_POINT('Ctrl Pts',(0.43541242072116,-7.89901416874995,
97.1504936506222));
#234183=CARTESIAN_POINT('Ctrl Pts',(0.426055367752419,-7.89952439319272,
97.1501197857091));
#234184=CARTESIAN_POINT('Ctrl Pts',(0.395900672461138,-7.90111494442952,
97.148916796736));
#234185=CARTESIAN_POINT('Ctrl Pts',(0.375099582037465,-7.90212977746612,
97.148089801807));
#234186=CARTESIAN_POINT('Ctrl Pts',(-0.0983086388039994,-7.92335268774623,
97.1293323925826));
#234187=CARTESIAN_POINT('Ctrl Pts',(-0.55183535311112,-7.90472804229589,
97.112765214267));
#234188=CARTESIAN_POINT('Ctrl Pts',(-1.0870814065756,-7.83643092504216,
97.0939974216306));
#234189=CARTESIAN_POINT('Ctrl Pts',(-1.17265761534474,-7.82408269597081,
97.0910185094886));
#234190=CARTESIAN_POINT('Ctrl Pts',(-1.32685541977588,-7.79924596596974,
97.0856747036307));
#234191=CARTESIAN_POINT('Ctrl Pts',(-1.39554654178061,-7.78724809551117,
97.0833027570642));
#234192=CARTESIAN_POINT('Ctrl Pts',(-1.52138513928129,-7.76355007276849,
97.078964124061));
#234193=CARTESIAN_POINT('Ctrl Pts',(-1.57857888554986,-7.75212301359285,
97.0769947437771));
#234194=CARTESIAN_POINT('Ctrl Pts',(-1.68441625714541,-7.72975731292474,
97.073349291532));
#234195=CARTESIAN_POINT('Ctrl Pts',(-1.73309285279156,-7.71898927457733,
97.0716722408739));
#234196=CARTESIAN_POINT('Ctrl Pts',(-1.82377949637822,-7.69802687663649,
97.0685431431637));
#234197=CARTESIAN_POINT('Ctrl Pts',(-1.86581403278651,-7.68794689375911,
97.067090872675));
#234198=CARTESIAN_POINT('Ctrl Pts',(-1.94450794494458,-7.668392487707,97.0643658513458));
#234199=CARTESIAN_POINT('Ctrl Pts',(-1.98118600098433,-7.65899840184089,
97.0630932223467));
#234200=CARTESIAN_POINT('Ctrl Pts',(-2.05011182788473,-7.64081667948913,
97.0606950561623));
#234201=CARTESIAN_POINT('Ctrl Pts',(-2.08237409248248,-7.63208727479302,
97.0595697927056));
#234202=CARTESIAN_POINT('Ctrl Pts',(-2.38991179157687,-7.54677965773142,
97.0488104032862));
#234203=CARTESIAN_POINT('Ctrl Pts',(-2.66089297880733,-7.45554804472596,
97.0390838333108));
#234204=CARTESIAN_POINT('Ctrl Pts',(-2.95544793416656,-7.33827163696595,
97.0277046475114));
#234205=CARTESIAN_POINT('Ctrl Pts',(-2.98449431646108,-7.32650644949623,
97.0265735405876));
#234206=CARTESIAN_POINT('Ctrl Pts',(-3.20204233674662,-7.23688061067491,
97.0180291766725));
#234207=CARTESIAN_POINT('Ctrl Pts',(-3.387527165248,-7.15193429327303,97.0103331980211));
#234208=CARTESIAN_POINT('Ctrl Pts',(-3.58147309248776,-7.05387490738756,
97.0016389137599));
#234209=CARTESIAN_POINT('Ctrl Pts',(-3.59342140412005,-7.04779563618024,
97.0011006137207));
#234210=CARTESIAN_POINT('Ctrl Pts',(-3.609831478186,-7.03939365292522,97.00035754079));
#234211=CARTESIAN_POINT('Ctrl Pts',(-3.6143066253133,-7.0370969809812,97.000154513961));
#234212=CARTESIAN_POINT('Ctrl Pts',(-3.62195261705451,-7.03316379535545,
96.9998069694008));
#234213=CARTESIAN_POINT('Ctrl Pts',(-3.62512455528011,-7.03152939914952,
96.9996625950277));
#234214=CARTESIAN_POINT('Ctrl Pts',(-3.63128403903065,-7.0283503426705,
96.9993818570926));
#234215=CARTESIAN_POINT('Ctrl Pts',(-3.63427170745572,-7.02680592216284,
96.9992455098853));
#234216=CARTESIAN_POINT('Ctrl Pts',(-3.64043672014641,-7.02361404807074,
96.9989637966468));
#234217=CARTESIAN_POINT('Ctrl Pts',(-3.64361393596606,-7.02196634108187,
96.9988184131689));
#234218=CARTESIAN_POINT('Ctrl Pts',(-3.65358671515299,-7.01678585785531,
96.998361449238));
#234219=CARTESIAN_POINT('Ctrl Pts',(-3.66037824053363,-7.01324538252634,
96.9980493384985));
#234220=CARTESIAN_POINT('Ctrl Pts',(-3.6990555269746,-6.99301112497675,
96.996266720671));
#234221=CARTESIAN_POINT('Ctrl Pts',(-3.73083172242819,-6.97611001635202,
96.9947821322729));
#234222=CARTESIAN_POINT('Ctrl Pts',(-3.82266437292896,-6.92645922350291,
96.9904361626955));
#234223=CARTESIAN_POINT('Ctrl Pts',(-3.88241162748855,-6.89314730079322,
96.9875392229692));
#234224=CARTESIAN_POINT('Ctrl Pts',(-4.12028799247174,-6.75644625445476,
96.9757511101894));
#234225=CARTESIAN_POINT('Ctrl Pts',(-4.29477302543572,-6.64689805947475,
96.9665269777069));
#234226=CARTESIAN_POINT('Ctrl Pts',(-5.08515710944068,-6.10654252811286,
96.9227603463567));
#234227=CARTESIAN_POINT('Ctrl Pts',(-5.64209332043876,-5.59605366965307,
96.8865898642591));
#234228=CARTESIAN_POINT('Ctrl Pts',(-6.13647518402876,-4.99283365392006,
96.8528472234301));
#234229=CARTESIAN_POINT('Ctrl Pts',(-6.15422668879896,-4.97093647769951,
96.8516322777974));
#234230=CARTESIAN_POINT('Ctrl Pts',(-6.29891077143058,-4.79050002478239,
96.8417023983538));
#234231=CARTESIAN_POINT('Ctrl Pts',(-6.41981772064854,-4.62721477507735,
96.8332327952869));
#234232=CARTESIAN_POINT('Ctrl Pts',(-6.54584743837429,-4.44254667765714,
96.8242003543207));
#234233=CARTESIAN_POINT('Ctrl Pts',(-6.55731602983917,-4.42560122054253,
96.8233763921531));
#234234=CARTESIAN_POINT('Ctrl Pts',(-6.57339052286024,-4.40165063478374,
96.8222186196142));
#234235=CARTESIAN_POINT('Ctrl Pts',(-6.5780511785332,-4.39468246519611,
96.8218825865981));
#234236=CARTESIAN_POINT('Ctrl Pts',(-6.58614125202555,-4.3825452522256,
96.8212986836526));
#234237=CARTESIAN_POINT('Ctrl Pts',(-6.58957567821953,-4.37737956552921,
96.8210506110078));
#234238=CARTESIAN_POINT('Ctrl Pts',(-6.59672942018752,-4.36659219452174,
96.8205334843954));
#234239=CARTESIAN_POINT('Ctrl Pts',(-6.60044763497629,-4.36096978373847,
96.8202644750014));
#234240=CARTESIAN_POINT('Ctrl Pts',(-6.60922164385051,-4.34766544655475,
96.8196291391425));
#234241=CARTESIAN_POINT('Ctrl Pts',(-6.61427124313944,-4.33997943493695,
96.8192630625266));
#234242=CARTESIAN_POINT('Ctrl Pts',(-6.63088592528815,-4.31459382460092,
96.81805713107));
#234243=CARTESIAN_POINT('Ctrl Pts',(-6.64239350312258,-4.29685659344748,
96.8172195869929));
#234244=CARTESIAN_POINT('Ctrl Pts',(-6.86078402861689,-3.95726591806099,
96.8012797745708));
#234245=CARTESIAN_POINT('Ctrl Pts',(-7.04412841430869,-3.62085730145171,
96.7871615447161));
#234246=CARTESIAN_POINT('Ctrl Pts',(-7.47772863296214,-2.66654043363741,
96.7501634853319));
#234247=CARTESIAN_POINT('Ctrl Pts',(-7.67544320725768,-2.02837060757967,
96.7288386857934));
#234248=CARTESIAN_POINT('Ctrl Pts',(-7.7952034678766,-1.34882487862752,
96.7037970958478));
#234249=CARTESIAN_POINT('Ctrl Pts',(-7.79935834272993,-1.32458864760173,
96.702900643586));
#234250=CARTESIAN_POINT('Ctrl Pts',(-7.83365740191113,-1.11875740237589,
96.695256090629));
#234251=CARTESIAN_POINT('Ctrl Pts',(-7.85756594021687,-0.936191805727175,
96.6882699676156));
#234252=CARTESIAN_POINT('Ctrl Pts',(-7.87632171246219,-0.740031256710166,
96.6803832776849));
#234253=CARTESIAN_POINT('Ctrl Pts',(-7.87752705804985,-0.727088321453079,
96.6798611270636));
#234254=CARTESIAN_POINT('Ctrl Pts',(-7.87915986638815,-0.709074532588748,
96.6791319020082));
#234255=CARTESIAN_POINT('Ctrl Pts',(-7.87961432542802,-0.704006374364151,
96.6789264618666));
#234256=CARTESIAN_POINT('Ctrl Pts',(-7.88039063958191,-0.695253942890348,
96.67857120983));
#234257=CARTESIAN_POINT('Ctrl Pts',(-7.88071480206095,-0.691569870654439,
96.6784215339873));
#234258=CARTESIAN_POINT('Ctrl Pts',(-7.88136168965207,-0.684158544125279,
96.6781201416991));
#234259=CARTESIAN_POINT('Ctrl Pts',(-7.88168435440607,-0.680431285311236,
96.6779684217495));
#234260=CARTESIAN_POINT('Ctrl Pts',(-7.88233353941262,-0.672869810082374,
96.6776603346862));
#234261=CARTESIAN_POINT('Ctrl Pts',(-7.88265990628726,-0.669035581699117,
96.6775039587012));
#234262=CARTESIAN_POINT('Ctrl Pts',(-7.8834049525076,-0.660206391793181,
96.677143517224));
#234263=CARTESIAN_POINT('Ctrl Pts',(-7.88382168202179,-0.655211271916484,
96.6769393393908));
#234264=CARTESIAN_POINT('Ctrl Pts',(-7.88488188966348,-0.642355655122257,
96.676413202506));
#234265=CARTESIAN_POINT('Ctrl Pts',(-7.88551835968058,-0.634494601941113,
96.6760908436201));
#234266=CARTESIAN_POINT('Ctrl Pts',(-7.88854611848681,-0.596390395890846,
96.6745252785793));
#234267=CARTESIAN_POINT('Ctrl Pts',(-7.89077515304799,-0.566134970075116,
96.6732729651777));
#234268=CARTESIAN_POINT('Ctrl Pts',(-7.90491782061927,-0.35782676751667,
96.6645907929568));
#234269=CARTESIAN_POINT('Ctrl Pts',(-7.91097706688777,-0.179439737976786,
96.6568546686882));
#234270=CARTESIAN_POINT('Ctrl Pts',(-7.91099993502481,-0.00101392183331238,
96.6489153477367));
#234271=CARTESIAN_POINT('',(-7.91099714745356,0.0067181084832415,92.642331465206));
#234272=CARTESIAN_POINT('Ctrl Pts',(-7.91099992838748,-0.00106444979291354,
96.6489175960477));
#234273=CARTESIAN_POINT('Ctrl Pts',(-7.91112606604236,0.936391675789824,
96.6072042977785));
#234274=CARTESIAN_POINT('Ctrl Pts',(-7.74464776818924,1.86658964603236,
96.5613040616377));
#234275=CARTESIAN_POINT('Ctrl Pts',(-7.37225732492007,2.87261232096405,
96.515391247615));
#234276=CARTESIAN_POINT('Ctrl Pts',(-7.32225597777836,2.997774072022,96.5097266405357));
#234277=CARTESIAN_POINT('Ctrl Pts',(-7.24051843157264,3.18811121311503,
96.5011836088845));
#234278=CARTESIAN_POINT('Ctrl Pts',(-7.21104498509999,3.25422661382722,
96.4982295178264));
#234279=CARTESIAN_POINT('Ctrl Pts',(-7.17426417101405,3.33377975320426,
96.4946900890407));
#234280=CARTESIAN_POINT('Ctrl Pts',(-7.16782048081803,3.34761159582746,
96.4940752459597));
#234281=CARTESIAN_POINT('Ctrl Pts',(-7.15773495856991,3.3690982649268,96.4931209798907));
#234282=CARTESIAN_POINT('Ctrl Pts',(-7.15412079098113,3.37676599196542,
96.4927806083711));
#234283=CARTESIAN_POINT('Ctrl Pts',(-7.14772809875032,3.3902722360213,96.4921813557626));
#234284=CARTESIAN_POINT('Ctrl Pts',(-7.14495473036879,3.39611317674163,
96.4919222979246));
#234285=CARTESIAN_POINT('Ctrl Pts',(-7.1386091011567,3.40943541241606,96.491331646539));
#234286=CARTESIAN_POINT('Ctrl Pts',(-7.13503223232001,3.41691451090665,
96.4910002117557));
#234287=CARTESIAN_POINT('Ctrl Pts',(-7.12536407475329,3.43704888841134,
96.4901083768383));
#234288=CARTESIAN_POINT('Ctrl Pts',(-7.11925081768732,3.44969361778151,
96.4895487330531));
#234289=CARTESIAN_POINT('Ctrl Pts',(-7.09094902630095,3.50783771305206,
96.4869773193002));
#234290=CARTESIAN_POINT('Ctrl Pts',(-7.06835754716253,3.55314019128705,
96.4849794532567));
#234291=CARTESIAN_POINT('Ctrl Pts',(-6.61660128359404,4.43768038779073,
96.446068835574));
#234292=CARTESIAN_POINT('Ctrl Pts',(-6.04138787031093,5.19363179699353,
96.415640779593));
#234293=CARTESIAN_POINT('Ctrl Pts',(-5.26929880219813,5.90164866033169,
96.3779414276778));
#234294=CARTESIAN_POINT('Ctrl Pts',(-5.19043195064273,5.97112903773125,
96.3741077306436));
#234295=CARTESIAN_POINT('Ctrl Pts',(-4.97893972581641,6.15009343639504,
96.3638096700428));
#234296=CARTESIAN_POINT('Ctrl Pts',(-4.84410764189707,6.2568448589424,96.3572078913845));
#234297=CARTESIAN_POINT('Ctrl Pts',(-4.68436825884356,6.37505544805819,
96.3493060686769));
#234298=CARTESIAN_POINT('Ctrl Pts',(-4.66276429612681,6.39087373120974,
96.3482363535364));
#234299=CARTESIAN_POINT('Ctrl Pts',(-4.6328027838359,6.41257856468144,96.346751778361));
#234300=CARTESIAN_POINT('Ctrl Pts',(-4.62451337066542,6.41855915027333,
96.3463409337103));
#234301=CARTESIAN_POINT('Ctrl Pts',(-4.61112630960793,6.42817815409404,
96.3456772852174));
#234302=CARTESIAN_POINT('Ctrl Pts',(-4.60603587731121,6.43182662395389,
96.3454248975896));
#234303=CARTESIAN_POINT('Ctrl Pts',(-4.59549690655387,6.4393613014867,96.3449023016151));
#234304=CARTESIAN_POINT('Ctrl Pts',(-4.59004775928498,6.4432466471813,96.3446320585883));
#234305=CARTESIAN_POINT('Ctrl Pts',(-4.57735381027875,6.45227339910649,
96.3440024452216));
#234306=CARTESIAN_POINT('Ctrl Pts',(-4.57010527186256,6.45740952121629,
96.3436428652483));
#234307=CARTESIAN_POINT('Ctrl Pts',(-4.5475074369631,6.47336464001756,96.342521704661));
#234308=CARTESIAN_POINT('Ctrl Pts',(-4.53212831028888,6.48414116322664,
96.3417584835249));
#234309=CARTESIAN_POINT('Ctrl Pts',(-4.3909636874175,6.58231102930137,96.3347518365509));
#234310=CARTESIAN_POINT('Ctrl Pts',(-4.26270643225895,6.66608669771378,
96.3283788878));
#234311=CARTESIAN_POINT('Ctrl Pts',(-4.02232137531487,6.81332703208748,
96.3165035678335));
#234312=CARTESIAN_POINT('Ctrl Pts',(-3.9109166285087,6.87787937850078,96.3110259757728));
#234313=CARTESIAN_POINT('Ctrl Pts',(-3.46203577043441,7.12354535458856,
96.289141026107));
#234314=CARTESIAN_POINT('Ctrl Pts',(-3.11317458882525,7.28277005616153,
96.2725728543569));
#234315=CARTESIAN_POINT('Ctrl Pts',(-2.08033885132131,7.66633901058044,
96.2255394957139));
#234316=CARTESIAN_POINT('Ctrl Pts',(-1.37554052595554,7.8235868619562,96.1958601734888));
#234317=CARTESIAN_POINT('Ctrl Pts',(-0.602047832060468,7.88826666571952,
96.1643803485787));
#234318=CARTESIAN_POINT('Ctrl Pts',(-0.544824503784611,7.89242541302795,
96.1620596381402));
#234319=CARTESIAN_POINT('Ctrl Pts',(-0.461180203914722,7.89759029111265,
96.1586792652638));
#234320=CARTESIAN_POINT('Ctrl Pts',(-0.43479160321472,7.8990870266449,96.1576145229645));
#234321=CARTESIAN_POINT('Ctrl Pts',(-0.388289055237259,7.90149087051021,
96.1557412037622));
#234322=CARTESIAN_POINT('Ctrl Pts',(-0.368178241835084,7.90245348939801,
96.1549320402608));
#234323=CARTESIAN_POINT('Ctrl Pts',(-0.328934248886238,7.90418179919584,
96.1533549476245));
#234324=CARTESIAN_POINT('Ctrl Pts',(-0.309801532411928,7.90495481756091,
96.1525869441367));
#234325=CARTESIAN_POINT('Ctrl Pts',(-0.263717667904164,7.90664917616683,
96.1507391886713));
#234326=CARTESIAN_POINT('Ctrl Pts',(-0.236764218452382,7.90750219189215,
96.149660198029));
#234327=CARTESIAN_POINT('Ctrl Pts',(-0.137199209179035,7.91014367509163,
96.1456806500123));
#234328=CARTESIAN_POINT('Ctrl Pts',(-0.0645680399432022,7.91106994535592,
96.1427898437642));
#234329=CARTESIAN_POINT('Ctrl Pts',(0.498073740995025,7.9104962780555,96.120481805984));
#234330=CARTESIAN_POINT('Ctrl Pts',(0.98697778256932,7.86447193005222,96.1016773502992));
#234331=CARTESIAN_POINT('Ctrl Pts',(1.79946607830078,7.71098572564421,96.0699039738262));
#234332=CARTESIAN_POINT('Ctrl Pts',(2.12610682622432,7.62738718828368,96.0569589182298));
#234333=CARTESIAN_POINT('Ctrl Pts',(2.47688655717082,7.51332022770222,96.0422997172878));
#234334=CARTESIAN_POINT('Ctrl Pts',(2.50729986178603,7.50322565586212,96.0410222380319));
#234335=CARTESIAN_POINT('Ctrl Pts',(2.56067202756923,7.4851500005111,96.0387680455842));
#234336=CARTESIAN_POINT('Ctrl Pts',(2.58365709671294,7.47724733882676,96.0377932027137));
#234337=CARTESIAN_POINT('Ctrl Pts',(2.61821093918432,7.46518878328519,96.0363212942662));
#234338=CARTESIAN_POINT('Ctrl Pts',(2.62980701394639,7.46111165713496,96.0358262512677));
#234339=CARTESIAN_POINT('Ctrl Pts',(2.65090079563317,7.45363989612313,96.0349238126177));
#234340=CARTESIAN_POINT('Ctrl Pts',(2.66040161203556,7.45025408904559,96.0345166311289));
#234341=CARTESIAN_POINT('Ctrl Pts',(2.68060190583431,7.44301174081976,96.0336493938243));
#234342=CARTESIAN_POINT('Ctrl Pts',(2.69129959076237,7.43915027831298,96.0331892230564));
#234343=CARTESIAN_POINT('Ctrl Pts',(2.71412200616947,7.43085657169618,96.032205605208));
#234344=CARTESIAN_POINT('Ctrl Pts',(2.72624428552801,7.4264176927865,96.0316820082028));
#234345=CARTESIAN_POINT('Ctrl Pts',(2.77985113925099,7.40663924567325,96.0293616004284));
#234346=CARTESIAN_POINT('Ctrl Pts',(2.82121726741933,7.39098169060062,96.0275578514512));
#234347=CARTESIAN_POINT('Ctrl Pts',(3.19822882969589,7.24465222577795,96.0110046246551));
#234348=CARTESIAN_POINT('Ctrl Pts',(3.52470983348601,7.0915488473174,95.9958584135305));
#234349=CARTESIAN_POINT('Ctrl Pts',(4.18664986221276,6.7240932347035,95.9640538006204));
#234350=CARTESIAN_POINT('Ctrl Pts',(4.51870293257877,6.50559800253946,95.9474516459493));
#234351=CARTESIAN_POINT('Ctrl Pts',(4.95021052194207,6.17262273574143,95.9250761000726));
#234352=CARTESIAN_POINT('Ctrl Pts',(5.06490071532491,6.0788681044449,95.9190394777778));
#234353=CARTESIAN_POINT('Ctrl Pts',(5.2089409687579,5.95421290498354,95.9113300281022));
#234354=CARTESIAN_POINT('Ctrl Pts',(5.24076595283447,5.92622051441109,95.909618272721));
#234355=CARTESIAN_POINT('Ctrl Pts',(5.2920429269082,5.88038258476053,95.9068460750739));
#234356=CARTESIAN_POINT('Ctrl Pts',(5.31163317732874,5.86269312505263,95.9057835474417));
#234357=CARTESIAN_POINT('Ctrl Pts',(5.34913245400674,5.82849006121531,95.9037429265578));
#234358=CARTESIAN_POINT('Ctrl Pts',(5.36705445168012,5.81199113223914,95.9027646502257));
#234359=CARTESIAN_POINT('Ctrl Pts',(5.40801773433818,5.77392942592453,95.9005215797971));
#234360=CARTESIAN_POINT('Ctrl Pts',(5.43100679776116,5.75231101404095,95.8992575449625));
#234361=CARTESIAN_POINT('Ctrl Pts',(5.50440143074161,5.68246010973172,95.8952047075492));
#234362=CARTESIAN_POINT('Ctrl Pts',(5.55429872883775,5.63369805110749,95.8924229352468));
#234363=CARTESIAN_POINT('Ctrl Pts',(5.69604626380118,5.49146156812846,95.8844377955807));
#234364=CARTESIAN_POINT('Ctrl Pts',(5.78622769704016,5.39635642092132,95.879254874931));
#234365=CARTESIAN_POINT('Ctrl Pts',(6.07802218370891,5.07290204212425,95.8620839095294));
#234366=CARTESIAN_POINT('Ctrl Pts',(6.26881218279405,4.83515163644925,95.8502122673796));
#234367=CARTESIAN_POINT('Ctrl Pts',(6.74045963660932,4.17241449987347,95.8190606844011));
#234368=CARTESIAN_POINT('Ctrl Pts',(6.99480803763235,3.73034910938752,95.8003027982792));
#234369=CARTESIAN_POINT('Ctrl Pts',(7.28775531029806,3.08427629279857,95.7739133009784));
#234370=CARTESIAN_POINT('Ctrl Pts',(7.36359426547428,2.89855381132946,95.766419754105));
#234371=CARTESIAN_POINT('Ctrl Pts',(7.49385953923858,2.54131603198224,95.7519303800023));
#234372=CARTESIAN_POINT('Ctrl Pts',(7.54965268590818,2.37043403216245,95.7449673268109));
#234373=CARTESIAN_POINT('Ctrl Pts',(7.60415937881971,2.18196087762608,95.7371294163135));
#234374=CARTESIAN_POINT('Ctrl Pts',(7.60869274489973,2.16609968348544,95.7364685886054));
#234375=CARTESIAN_POINT('Ctrl Pts',(7.61532303176484,2.14262420739654,95.7354885867236));
#234376=CARTESIAN_POINT('Ctrl Pts',(7.61745822982439,2.13502072321874,95.7351708731105));
#234377=CARTESIAN_POINT('Ctrl Pts',(7.62119291660905,2.12164450619232,95.7346113982401));
#234378=CARTESIAN_POINT('Ctrl Pts',(7.62279724313438,2.11587312300213,95.7343698252611));
#234379=CARTESIAN_POINT('Ctrl Pts',(7.62612263656586,2.10385752474214,95.7338665069474));
#234380=CARTESIAN_POINT('Ctrl Pts',(7.62784259260812,2.09761300873886,95.7336047180498));
#234381=CARTESIAN_POINT('Ctrl Pts',(7.63221434299466,2.0816643402125,95.7329355410488));
#234382=CARTESIAN_POINT('Ctrl Pts',(7.63485529473338,2.07195724617636,95.732527719397));
#234383=CARTESIAN_POINT('Ctrl Pts',(7.64502282531641,2.03430202973873,95.7309435835658));
#234384=CARTESIAN_POINT('Ctrl Pts',(7.65241445697131,2.0063179448237,95.7297617478609));
#234385=CARTESIAN_POINT('Ctrl Pts',(7.76121732718517,1.58504988589116,95.711894281484));
#234386=CARTESIAN_POINT('Ctrl Pts',(7.83232820882552,1.18464516550145,95.6937280205191));
#234387=CARTESIAN_POINT('Ctrl Pts',(7.91015132266054,0.39983138607443,95.6576537711324));
#234388=CARTESIAN_POINT('Ctrl Pts',(7.92023283714517,0.0167780115089239,
95.6398635594541));
#234389=CARTESIAN_POINT('Ctrl Pts',(7.88516424848162,-0.741448352493183,
95.6054171829064));
#234390=CARTESIAN_POINT('Ctrl Pts',(7.84097021598678,-1.11570189230857,
95.5887936846303));
#234391=CARTESIAN_POINT('Ctrl Pts',(7.74314841723535,-1.62741318513683,
95.5668612218789));
#234392=CARTESIAN_POINT('Ctrl Pts',(7.71211531104413,-1.76864391508049,
95.5608899635125));
#234393=CARTESIAN_POINT('Ctrl Pts',(7.67268046905092,-1.92723911293059,
95.5542734488224));
#234394=CARTESIAN_POINT('Ctrl Pts',(7.66806746468618,-1.9455121540871,95.5535124401826));
#234395=CARTESIAN_POINT('Ctrl Pts',(7.66104546727304,-1.97291472005736,
95.552373193876));
#234396=CARTESIAN_POINT('Ctrl Pts',(7.65868537131834,-1.9820566410106,95.5519934541954));
#234397=CARTESIAN_POINT('Ctrl Pts',(7.6546005299008,-1.99776319822395,95.5513415947661));
#234398=CARTESIAN_POINT('Ctrl Pts',(7.65288369451128,-2.00432986982757,
95.5510692319275));
#234399=CARTESIAN_POINT('Ctrl Pts',(7.64933285576365,-2.01784029117552,
95.5505092134893));
#234400=CARTESIAN_POINT('Ctrl Pts',(7.64749784344183,-2.02478376964562,
95.5502215893161));
#234401=CARTESIAN_POINT('Ctrl Pts',(7.64306137320567,-2.04147880356667,
95.5495304717041));
#234402=CARTESIAN_POINT('Ctrl Pts',(7.64045070154433,-2.05122790987058,
95.5491272627168));
#234403=CARTESIAN_POINT('Ctrl Pts',(7.63239534645694,-2.08108050505075,
95.5478937279424));
#234404=CARTESIAN_POINT('Ctrl Pts',(7.62688990363295,-2.10116757996013,
95.5470652784247));
#234405=CARTESIAN_POINT('Ctrl Pts',(7.56374376454962,-2.32804319796375,
95.5377255944393));
#234406=CARTESIAN_POINT('Ctrl Pts',(7.49778631868551,-2.53243227134478,
95.5294778723722));
#234407=CARTESIAN_POINT('Ctrl Pts',(7.15868178240451,-3.45323355992984,
95.4928152974298));
#234408=CARTESIAN_POINT('Ctrl Pts',(6.79065580776811,-4.13018923469821,
95.4676558548608));
#234409=CARTESIAN_POINT('Ctrl Pts',(6.13344078174204,-5.00733610958948,
95.4286956010771));
#234410=CARTESIAN_POINT('Ctrl Pts',(5.91956726488576,-5.25844314229553,
95.4165614002616));
#234411=CARTESIAN_POINT('Ctrl Pts',(5.68023469576563,-5.50627644462431,
95.4027889115777));
#234412=CARTESIAN_POINT('Ctrl Pts',(5.66977288703903,-5.51704829490635,
95.4021866736221));
#234413=CARTESIAN_POINT('Ctrl Pts',(5.65447897966661,-5.53270600051181,
95.4013060602173));
#234414=CARTESIAN_POINT('Ctrl Pts',(5.64967103983775,-5.53761549412487,
95.4010291914705));
#234415=CARTESIAN_POINT('Ctrl Pts',(5.64129585698006,-5.54614531779369,
95.4005468573699));
#234416=CARTESIAN_POINT('Ctrl Pts',(5.63773150519665,-5.54976849131596,
95.4003415697169));
#234417=CARTESIAN_POINT('Ctrl Pts',(5.63039136479274,-5.55721539593551,
95.3999187938522));
#234418=CARTESIAN_POINT('Ctrl Pts',(5.62661516729661,-5.56103871920512,
95.3997012807777));
#234419=CARTESIAN_POINT('Ctrl Pts',(5.61713125484368,-5.57062143881782,
95.3991549729164));
#234420=CARTESIAN_POINT('Ctrl Pts',(5.61141858342267,-5.57637590462522,
95.3988258803135));
#234421=CARTESIAN_POINT('Ctrl Pts',(5.59023512029023,-5.59764883397976,
95.397605508479));
#234422=CARTESIAN_POINT('Ctrl Pts',(5.57470880854338,-5.6131116909807,95.3967109529389));
#234423=CARTESIAN_POINT('Ctrl Pts',(5.53746368343128,-5.64989763898267,
95.3945652868947));
#234424=CARTESIAN_POINT('Ctrl Pts',(5.51568574554323,-5.67116020753079,
95.393310859427));
#234425=CARTESIAN_POINT('Ctrl Pts',(5.47610709162652,-5.70935861366829,
95.3910323080453));
#234426=CARTESIAN_POINT('Ctrl Pts',(5.45834906073824,-5.72633828666108,
95.3900104089556));
#234427=CARTESIAN_POINT('Ctrl Pts',(4.98593981003197,-6.17384712607264,
95.3628433557496));
#234428=CARTESIAN_POINT('Ctrl Pts',(4.48185296354909,-6.54897051752987,
95.3345431406337));
#234429=CARTESIAN_POINT('Ctrl Pts',(3.56009478625329,-7.07815934688124,
95.2883918433917));
#234430=CARTESIAN_POINT('Ctrl Pts',(3.16401394654728,-7.26386119618355,
95.2699906132983));
#234431=CARTESIAN_POINT('Ctrl Pts',(2.71754108066484,-7.4297008454467,95.2506916782674));
#234432=CARTESIAN_POINT('Ctrl Pts',(2.68037536293075,-7.44318964732422,
95.2490951157419));
#234433=CARTESIAN_POINT('Ctrl Pts',(2.62666406241629,-7.46222898019171,
95.2468015484371));
#234434=CARTESIAN_POINT('Ctrl Pts',(2.61019896470891,-7.46800420574946,
95.2461003132636));
#234435=CARTESIAN_POINT('Ctrl Pts',(2.58150971520609,-7.47796065094888,
95.2448816232682));
#234436=CARTESIAN_POINT('Ctrl Pts',(2.56929419624123,-7.48216648044811,
95.2443637152936));
#234437=CARTESIAN_POINT('Ctrl Pts',(2.54571295048071,-7.49022099566367,
95.2433658170558));
#234438=CARTESIAN_POINT('Ctrl Pts',(2.5343486649334,-7.49407378103334,95.2428857534428));
#234439=CARTESIAN_POINT('Ctrl Pts',(2.50742182570655,-7.50313441842114,
95.2417502455319));
#234440=CARTESIAN_POINT('Ctrl Pts',(2.49185173220609,-7.50831973612383,
95.2410952060604));
#234441=CARTESIAN_POINT('Ctrl Pts',(2.43756177918868,-7.52621247840697,
95.2388164978652));
#234442=CARTESIAN_POINT('Ctrl Pts',(2.39875971449485,-7.53866921695688,
95.2371971626599));
#234443=CARTESIAN_POINT('Ctrl Pts',(1.84431488878029,-7.71195011490613,
95.2141861639005));
#234444=CARTESIAN_POINT('Ctrl Pts',(1.31361063968508,-7.81985605369122,
95.1938664240161));
#234445=CARTESIAN_POINT('Ctrl Pts',(0.370468989098573,-7.91282198341236,
95.1589041990029));
#234446=CARTESIAN_POINT('Ctrl Pts',(-0.0375636228363237,-7.92139958600949,
95.1441088451984));
#234447=CARTESIAN_POINT('Ctrl Pts',(-0.599349254782895,-7.889789511908,
95.1228751832535));
#234448=CARTESIAN_POINT('Ctrl Pts',(-0.753977925213433,-7.87651652901819,
95.1169357260577));
#234449=CARTESIAN_POINT('Ctrl Pts',(-0.979708179982585,-7.85043230877517,
95.1080297989279));
#234450=CARTESIAN_POINT('Ctrl Pts',(-1.05118730491298,-7.84118106037849,
95.1051748027151));
#234451=CARTESIAN_POINT('Ctrl Pts',(-1.13554506277208,-7.8290887923174,
95.1017559347112));
#234452=CARTESIAN_POINT('Ctrl Pts',(-1.1485567254491,-7.82719051470026,
95.1012271993877));
#234453=CARTESIAN_POINT('Ctrl Pts',(-1.16853655918385,-7.82422475419203,
95.1004130982736));
#234454=CARTESIAN_POINT('Ctrl Pts',(-1.17550817160751,-7.82318037835862,
95.1001286181859));
#234455=CARTESIAN_POINT('Ctrl Pts',(-1.18819096737012,-7.82126310800646,
95.0996103253936));
#234456=CARTESIAN_POINT('Ctrl Pts',(-1.19390261284005,-7.82039327210771,
95.0993766318645));
#234457=CARTESIAN_POINT('Ctrl Pts',(-1.20632168409,-7.81848802878117,95.0988678798762));
#234458=CARTESIAN_POINT('Ctrl Pts',(-1.21302873682976,-7.81745024576097,
95.0985927279567));
#234459=CARTESIAN_POINT('Ctrl Pts',(-1.23122537547122,-7.81461069612075,
95.0978451362602));
#234460=CARTESIAN_POINT('Ctrl Pts',(-1.24271230964406,-7.81279222625603,
95.0973720289084));
#234461=CARTESIAN_POINT('Ctrl Pts',(-1.29684933164786,-7.80409950590402,
95.095136617336));
#234462=CARTESIAN_POINT('Ctrl Pts',(-1.339446092445,-7.79690139389565,95.0933610546442));
#234463=CARTESIAN_POINT('Ctrl Pts',(-2.16340539959627,-7.65071518909409,
95.0586629026643));
#234464=CARTESIAN_POINT('Ctrl Pts',(-2.91942620267822,-7.3953036560385,
95.020389810409));
#234465=CARTESIAN_POINT('Ctrl Pts',(-3.79709335058799,-6.94288160360653,
94.9760591146227));
#234466=CARTESIAN_POINT('Ctrl Pts',(-3.96613406190936,-6.84772294323324,
94.9674986720219));
#234467=CARTESIAN_POINT('Ctrl Pts',(-4.26507314195986,-6.66465302452364,
94.9523845130701));
#234468=CARTESIAN_POINT('Ctrl Pts',(-4.39617833532916,-6.57891089801474,
94.9457644321755));
#234469=CARTESIAN_POINT('Ctrl Pts',(-4.59032185486511,-6.44354517049231,
94.9359820711478));
#234470=CARTESIAN_POINT('Ctrl Pts',(-4.65528919948562,-6.39676575101305,
94.9327120108043));
#234471=CARTESIAN_POINT('Ctrl Pts',(-4.73177696848006,-6.33990854298436,
94.9288655419062));
#234472=CARTESIAN_POINT('Ctrl Pts',(-4.74399095416185,-6.33077431624114,
94.9282514208236));
#234473=CARTESIAN_POINT('Ctrl Pts',(-4.76277516646231,-6.31664166012848,
94.9273070967002));
#234474=CARTESIAN_POINT('Ctrl Pts',(-4.76936407885932,-6.31166819728203,
94.9269758857795));
#234475=CARTESIAN_POINT('Ctrl Pts',(-4.78137133039626,-6.30257530922573,
94.9263723555379));
#234476=CARTESIAN_POINT('Ctrl Pts',(-4.78679215669524,-6.29845919066783,
94.9260999025356));
#234477=CARTESIAN_POINT('Ctrl Pts',(-4.79860650162472,-6.28946431118315,
94.9255061470036));
#234478=CARTESIAN_POINT('Ctrl Pts',(-4.80499790990156,-6.28458278372031,
94.9251849575151));
#234479=CARTESIAN_POINT('Ctrl Pts',(-4.82241370065629,-6.27123913142877,
94.9243098195065));
#234480=CARTESIAN_POINT('Ctrl Pts',(-4.83342327031411,-6.26275767026416,
94.9237566615132));
#234481=CARTESIAN_POINT('Ctrl Pts',(-4.88621376775106,-6.22186724335033,
94.9211045844746));
#234482=CARTESIAN_POINT('Ctrl Pts',(-4.9276918808517,-6.18906857678055,
94.9190217227572));
#234483=CARTESIAN_POINT('Ctrl Pts',(-5.7128860395509,-5.55528133793307,
94.8795995642244));
#234484=CARTESIAN_POINT('Ctrl Pts',(-6.34176891206572,-4.82493001242914,
94.8494209936139));
#234485=CARTESIAN_POINT('Ctrl Pts',(-6.92332855934655,-3.83263788035091,
94.809624523115));
#234486=CARTESIAN_POINT('Ctrl Pts',(-7.0152673793104,-3.66164016699497,
94.8027556528994));
#234487=CARTESIAN_POINT('Ctrl Pts',(-7.16716401441824,-3.35236174937193,
94.7900332542353));
#234488=CARTESIAN_POINT('Ctrl Pts',(-7.22963522771145,-3.21542204489982,
94.7843003702489));
#234489=CARTESIAN_POINT('Ctrl Pts',(-7.29732526497413,-3.05508106954919,
94.7773856129795));
#234490=CARTESIAN_POINT('Ctrl Pts',(-7.30639360304725,-3.03332966533883,
94.7764433395965));
#234491=CARTESIAN_POINT('Ctrl Pts',(-7.31793311761285,-3.00529888929421,
94.7752232247743));
#234492=CARTESIAN_POINT('Ctrl Pts',(-7.32049372070677,-2.99905622027662,
94.7749511256988));
#234493=CARTESIAN_POINT('Ctrl Pts',(-7.32460511466163,-2.98899613448557,
94.7745120299967));
#234494=CARTESIAN_POINT('Ctrl Pts',(-7.32616092007986,-2.98518075678214,
94.7743453585601));
#234495=CARTESIAN_POINT('Ctrl Pts',(-7.3291168040358,-2.97791566931651,
94.774027719301));
#234496=CARTESIAN_POINT('Ctrl Pts',(-7.33051743008273,-2.97446618200943,
94.7738767872619));
#234497=CARTESIAN_POINT('Ctrl Pts',(-7.33370471017912,-2.96660056601358,
94.773532361148));
#234498=CARTESIAN_POINT('Ctrl Pts',(-7.3354897991977,-2.96218383969471,
94.7733387659113));
#234499=CARTESIAN_POINT('Ctrl Pts',(-7.34099629414028,-2.94852398550127,
94.7727394274853));
#234500=CARTESIAN_POINT('Ctrl Pts',(-7.34470419931075,-2.93927550706612,
94.7723328024397));
#234501=CARTESIAN_POINT('Ctrl Pts',(-7.37323238705918,-2.86772774479975,
94.7691807564148));
#234502=CARTESIAN_POINT('Ctrl Pts',(-7.39727637142868,-2.80512388474049,
94.7663856983754));
#234503=CARTESIAN_POINT('Ctrl Pts',(-7.61554935348937,-2.21447216511167,
94.7397271656991));
#234504=CARTESIAN_POINT('Ctrl Pts',(-7.75371053990945,-1.66745036305818,
94.7130116411022));
#234505=CARTESIAN_POINT('Ctrl Pts',(-7.88453464447883,-0.744659888212214,
94.6695735779369));
#234506=CARTESIAN_POINT('Ctrl Pts',(-7.9107087703331,-0.375673156917667,
94.6525943800661));
#234507=CARTESIAN_POINT('Ctrl Pts',(-7.91122201221791,0.280936946069419,
94.623756332697));
#234508=CARTESIAN_POINT('Ctrl Pts',(-7.89581557996747,0.567873452934318,
94.6116136198462));
#234509=CARTESIAN_POINT('Ctrl Pts',(-7.86242790963038,0.875584398980283,
94.5990981324223));
#234510=CARTESIAN_POINT('Ctrl Pts',(-7.85992245178328,0.897797158235373,
94.5981974599803));
#234511=CARTESIAN_POINT('Ctrl Pts',(-7.85631024691878,0.928647469896319,
94.5969503791823));
#234512=CARTESIAN_POINT('Ctrl Pts',(-7.8552833490821,0.937294150986242,
94.5966012667754));
#234513=CARTESIAN_POINT('Ctrl Pts',(-7.85349040312374,0.952181188843237,
94.5960009134457));
#234514=CARTESIAN_POINT('Ctrl Pts',(-7.85273118888152,0.958422351461388,
94.595749441133));
#234515=CARTESIAN_POINT('Ctrl Pts',(-7.85114927927588,0.971298457531457,
94.5952310752899));
#234516=CARTESIAN_POINT('Ctrl Pts',(-7.85032561128993,0.977933277945624,
94.5949642149399));
#234517=CARTESIAN_POINT('Ctrl Pts',(-7.84838972364556,0.993367206418321,
94.5943440092636));
#234518=CARTESIAN_POINT('Ctrl Pts',(-7.84727111468852,1.00216551242569,
94.5939908807898));
#234519=CARTESIAN_POINT('Ctrl Pts',(-7.8436644668592,1.03015692778844,94.5928687707562));
#234520=CARTESIAN_POINT('Ctrl Pts',(-7.84112078192757,1.04934286821054,
94.5921016757835));
#234521=CARTESIAN_POINT('Ctrl Pts',(-7.79599753792367,1.38036059113958,
94.5789013097026));
#234522=CARTESIAN_POINT('Ctrl Pts',(-7.73491601324756,1.68940011153656,
94.5671229575886));
#234523=CARTESIAN_POINT('Ctrl Pts',(-7.50536082086748,2.57073160343405,
94.5344139622122));
#234524=CARTESIAN_POINT('Ctrl Pts',(-7.29046929547689,3.12859702176804,
94.5149473897396));
#234525=CARTESIAN_POINT('Ctrl Pts',(-6.85953880646736,3.95521445890848,
94.4824994298255));
#234526=CARTESIAN_POINT('Ctrl Pts',(-6.68525380758608,4.24315121881615,
94.4703740778455));
#234527=CARTESIAN_POINT('Ctrl Pts',(-6.48045185030031,4.53741810511691,
94.4561222977885));
#234528=CARTESIAN_POINT('Ctrl Pts',(-6.46762349377499,4.55568497405468,
94.4552295474633));
#234529=CARTESIAN_POINT('Ctrl Pts',(-6.45066188073635,4.57962132901756,
94.4540487470388));
#234530=CARTESIAN_POINT('Ctrl Pts',(-6.44659815367386,4.58533995045091,
94.4537658194258));
#234531=CARTESIAN_POINT('Ctrl Pts',(-6.44027350929476,4.59421518885608,
94.4533254485057));
#234532=CARTESIAN_POINT('Ctrl Pts',(-6.43801785676583,4.59737557220386,
94.4531683861077));
#234533=CARTESIAN_POINT('Ctrl Pts',(-6.43349447941282,4.60370339603459,
94.4528534101656));
#234534=CARTESIAN_POINT('Ctrl Pts',(-6.431226739806,4.60687082480029,94.4526954955576));
#234535=CARTESIAN_POINT('Ctrl Pts',(-6.4261559439075,4.61394233639957,94.4523423800092));
#234536=CARTESIAN_POINT('Ctrl Pts',(-6.42335166963501,4.61784553953872,
94.4521470920519));
#234537=CARTESIAN_POINT('Ctrl Pts',(-6.41513421398519,4.62926125392239,
94.4515748205565));
#234538=CARTESIAN_POINT('Ctrl Pts',(-6.4097114136782,4.6367667972927,94.4511971552335));
#234539=CARTESIAN_POINT('Ctrl Pts',(-6.37004643354941,4.69146341368938,
94.4484347146137));
#234540=CARTESIAN_POINT('Ctrl Pts',(-6.33529745322873,4.73828306195219,
94.4460145727601));
#234541=CARTESIAN_POINT('Ctrl Pts',(-6.22106550429026,4.88869234459986,
94.4380700166816));
#234542=CARTESIAN_POINT('Ctrl Pts',(-6.13953740350233,4.99069596489229,
94.4324173013784));
#234543=CARTESIAN_POINT('Ctrl Pts',(-5.9120210914342,5.26133651859309,94.4167930238903));
#234544=CARTESIAN_POINT('Ctrl Pts',(-5.7613674939071,5.42589080614565,94.4066063155981));
#234545=CARTESIAN_POINT('Ctrl Pts',(-5.42125914027264,5.76722458469051,
94.3843126146277));
#234546=CARTESIAN_POINT('Ctrl Pts',(-5.22965678887514,5.94151659274608,
94.3721757143731));
#234547=CARTESIAN_POINT('Ctrl Pts',(-4.92331560667846,6.19386287784564,
94.35371361287));
#234548=CARTESIAN_POINT('Ctrl Pts',(-4.81449526407076,6.27882237541689,
94.3473218559523));
#234549=CARTESIAN_POINT('Ctrl Pts',(-4.55761183383273,6.46877257752144,
94.3326639334802));
#234550=CARTESIAN_POINT('Ctrl Pts',(-4.40804484790486,6.57160477402897,
94.3244455144689));
#234551=CARTESIAN_POINT('Ctrl Pts',(-4.24042784836438,6.67854731801089,
94.3156103218769));
#234552=CARTESIAN_POINT('Ctrl Pts',(-4.22575609915171,6.68784030992249,
94.3148400144216));
#234553=CARTESIAN_POINT('Ctrl Pts',(-4.16886558809881,6.72361244143509,
94.3118649551015));
#234554=CARTESIAN_POINT('Ctrl Pts',(-4.12642719504461,6.74974097780123,
94.3096708344453));
#234555=CARTESIAN_POINT('Ctrl Pts',(-3.84115024000805,6.92168456783268,
94.2950914254933));
#234556=CARTESIAN_POINT('Ctrl Pts',(-3.59086528591821,7.05477575493315,
94.283126780237));
#234557=CARTESIAN_POINT('Ctrl Pts',(-3.31246037903762,7.18415543647104,
94.2706781561009));
#234558=CARTESIAN_POINT('Ctrl Pts',(-3.29091508140821,7.1940503916617,94.2697201186449));
#234559=CARTESIAN_POINT('Ctrl Pts',(-3.26078498605123,7.20772434532195,
94.268387722456));
#234560=CARTESIAN_POINT('Ctrl Pts',(-3.25223756431176,7.21158510935278,
94.2680105683121));
#234561=CARTESIAN_POINT('Ctrl Pts',(-3.23746076469172,7.21822799180887,
94.2673599623386));
#234562=CARTESIAN_POINT('Ctrl Pts',(-3.23123462486104,7.22101726518295,
94.2670862666242));
#234563=CARTESIAN_POINT('Ctrl Pts',(-3.21833691026475,7.22677534281028,
94.2665201902334));
#234564=CARTESIAN_POINT('Ctrl Pts',(-3.21166481579589,7.22974297155696,
94.2662278497354));
#234565=CARTESIAN_POINT('Ctrl Pts',(-3.1960575149201,7.23665895205102,94.2655451635215));
#234566=CARTESIAN_POINT('Ctrl Pts',(-3.18711907641673,7.24060000418424,
94.265155065939));
#234567=CARTESIAN_POINT('Ctrl Pts',(-3.15834831084868,7.25322174079708,
94.2639022562941));
#234568=CARTESIAN_POINT('Ctrl Pts',(-3.13848756604615,7.26183761048352,
94.2630417389403));
#234569=CARTESIAN_POINT('Ctrl Pts',(-2.68902687998292,7.45463164397244,
94.2436638462352));
#234570=CARTESIAN_POINT('Ctrl Pts',(-2.24395415014403,7.6004689903636,94.2265305156132));
#234571=CARTESIAN_POINT('Ctrl Pts',(-1.3296458246873,7.81267736419065,94.1934214767998));
#234572=CARTESIAN_POINT('Ctrl Pts',(-0.862131941818696,7.87798156403184,
94.1775059102993));
#234573=CARTESIAN_POINT('Ctrl Pts',(-0.272659089714595,7.90719670582171,
94.1564748440106));
#234574=CARTESIAN_POINT('Ctrl Pts',(-0.1536026088649,7.91040502904463,94.152175192663));
#234575=CARTESIAN_POINT('Ctrl Pts',(0.173987047569121,7.91183457340231,
94.1401085122769));
#234576=CARTESIAN_POINT('Ctrl Pts',(0.382413096933918,7.90450208480821,
94.1321371875806));
#234577=CARTESIAN_POINT('Ctrl Pts',(0.610010060304839,7.88747096059922,
94.1230303318664));
#234578=CARTESIAN_POINT('Ctrl Pts',(0.629683288720923,7.88592476350584,
94.1222402588328));
#234579=CARTESIAN_POINT('Ctrl Pts',(0.658252937186033,7.88357177065612,
94.1210888734911));
#234580=CARTESIAN_POINT('Ctrl Pts',(0.667154185192994,7.88282348431344,
94.1207295751329));
#234581=CARTESIAN_POINT('Ctrl Pts',(0.682843879193456,7.88147775969365,
94.1200952758218));
#234582=CARTESIAN_POINT('Ctrl Pts',(0.689632865342825,7.88088662211402,
94.1198204867809));
#234583=CARTESIAN_POINT('Ctrl Pts',(0.703650088699174,7.87964784870312,
94.1192524667211));
#234584=CARTESIAN_POINT('Ctrl Pts',(0.710878214463638,7.87899903735989,
94.1189591971604));
#234585=CARTESIAN_POINT('Ctrl Pts',(0.729346540244259,7.87731566187197,
94.118208957556));
#234586=CARTESIAN_POINT('Ctrl Pts',(0.740585419917201,7.87626698677392,
94.1177515317865));
#234587=CARTESIAN_POINT('Ctrl Pts',(0.786208646362108,7.87191146949555,
94.1158912075553));
#234588=CARTESIAN_POINT('Ctrl Pts',(0.820573170336826,7.86840351364132,
94.1144820194374));
#234589=CARTESIAN_POINT('Ctrl Pts',(1.28752181315138,7.81764479271208,94.0952332723437));
#234590=CARTESIAN_POINT('Ctrl Pts',(1.7155016658782,7.73500590644631,94.0764696006769));
#234591=CARTESIAN_POINT('Ctrl Pts',(2.83724127996136,7.42068775152626,94.0263430553656));
#234592=CARTESIAN_POINT('Ctrl Pts',(3.50939901040711,7.12746512953161,93.99562021129));
#234593=CARTESIAN_POINT('Ctrl Pts',(4.32027635140846,6.63083506586048,93.9565187478429));
#234594=CARTESIAN_POINT('Ctrl Pts',(4.50382027500275,6.50756229891525,93.9474824738646));
#234595=CARTESIAN_POINT('Ctrl Pts',(4.71589951209192,6.35184896037064,93.9368345450673));
#234596=CARTESIAN_POINT('Ctrl Pts',(4.74963557114221,6.3266622628682,93.9351341412914));
#234597=CARTESIAN_POINT('Ctrl Pts',(4.80175903272139,6.28709598381034,93.9324965560913));
#234598=CARTESIAN_POINT('Ctrl Pts',(4.82028647950243,6.27290235677451,93.9315569489415));
#234599=CARTESIAN_POINT('Ctrl Pts',(4.85399777920864,6.24683903919197,93.9298434857699));
#234600=CARTESIAN_POINT('Ctrl Pts',(4.86920157744939,6.23499546292231,93.9290692832884));
#234601=CARTESIAN_POINT('Ctrl Pts',(4.90254001282529,6.20882890938538,93.9273684571031));
#234602=CARTESIAN_POINT('Ctrl Pts',(4.92065548939076,6.19448178318537,93.9264421766341));
#234603=CARTESIAN_POINT('Ctrl Pts',(4.97057067787954,6.15459273426823,93.9238840693339));
#234604=CARTESIAN_POINT('Ctrl Pts',(5.0022361887982,6.12888388883201,93.9222546363481));
#234605=CARTESIAN_POINT('Ctrl Pts',(5.18338321580237,5.97947370517252,93.9128940434347));
#234606=CARTESIAN_POINT('Ctrl Pts',(5.32847424731431,5.85054970465887,93.9052434734407));
#234607=CARTESIAN_POINT('Ctrl Pts',(5.78435237888315,5.41442849967996,93.8805882002261));
#234608=CARTESIAN_POINT('Ctrl Pts',(6.07446599011095,5.08680976318078,93.8639396131964));
#234609=CARTESIAN_POINT('Ctrl Pts',(6.42623309184015,4.61629002832633,93.8412951881687));
#234610=CARTESIAN_POINT('Ctrl Pts',(6.51295253341472,4.49311179998054,93.8354669276539));
#234611=CARTESIAN_POINT('Ctrl Pts',(6.66866209012494,4.25795029522806,93.8244363427727));
#234612=CARTESIAN_POINT('Ctrl Pts',(6.73847891609442,4.14657634858243,93.8192504351364));
#234613=CARTESIAN_POINT('Ctrl Pts',(6.81572015897925,4.01625229528203,93.8131858969797));
#234614=CARTESIAN_POINT('Ctrl Pts',(6.82588706981406,3.99894854842869,93.8123807425546));
#234615=CARTESIAN_POINT('Ctrl Pts',(6.84233364529022,3.97071155448646,93.8110667822638));
#234616=CARTESIAN_POINT('Ctrl Pts',(6.84865319825554,3.9598016782416,93.8105591017631));
#234617=CARTESIAN_POINT('Ctrl Pts',(6.85999224575863,3.94011796308261,93.8096431594107));
#234618=CARTESIAN_POINT('Ctrl Pts',(6.86502106191644,3.93134951303079,93.8092351443102));
#234619=CARTESIAN_POINT('Ctrl Pts',(6.87571337677937,3.9126228799643,93.808363789536));
#234620=CARTESIAN_POINT('Ctrl Pts',(6.8813720760621,3.90266198769901,93.8079003286378));
#234621=CARTESIAN_POINT('Ctrl Pts',(6.89638197394832,3.87610622965771,93.8066648367283));
#234622=CARTESIAN_POINT('Ctrl Pts',(6.90569488926282,3.85948985309928,93.8058918683782));
#234623=CARTESIAN_POINT('Ctrl Pts',(6.94834410286881,3.78274529019253,93.8023225813965));
#234624=CARTESIAN_POINT('Ctrl Pts',(6.98095541691311,3.72221828863484,93.7995096908244));
#234625=CARTESIAN_POINT('Ctrl Pts',(7.07125692281705,3.5492555711758,93.7914857241954));
#234626=CARTESIAN_POINT('Ctrl Pts',(7.12704743643019,3.43585268210878,93.7862417623378));
#234627=CARTESIAN_POINT('Ctrl Pts',(7.35122789373618,2.95119201350464,93.7639673073234));
#234628=CARTESIAN_POINT('Ctrl Pts',(7.49350800194589,2.56854587001984,93.7467441039212));
#234629=CARTESIAN_POINT('Ctrl Pts',(7.64593524376229,2.03593124103031,93.7236458965112));
#234630=CARTESIAN_POINT('Ctrl Pts',(7.68229223272481,1.89413005387359,93.7175737724449));
#234631=CARTESIAN_POINT('Ctrl Pts',(7.71960480154008,1.72977298279587,93.7106255511862));
#234632=CARTESIAN_POINT('Ctrl Pts',(7.72442378518012,1.70812471857691,93.7097121331885));
#234633=CARTESIAN_POINT('Ctrl Pts',(7.76451305479354,1.52439270026603,93.7019746958401));
#234634=CARTESIAN_POINT('Ctrl Pts',(7.79476892142191,1.36125493476479,93.6952034887261));
#234635=CARTESIAN_POINT('Ctrl Pts',(7.82666707831053,1.15291719469416,93.6866679830586));
#234636=CARTESIAN_POINT('Ctrl Pts',(7.83308239195482,1.1084926169771,93.6848542737141));
#234637=CARTESIAN_POINT('Ctrl Pts',(7.84272740284494,1.03743314714883,93.6819627300506));
#234638=CARTESIAN_POINT('Ctrl Pts',(7.84620026418977,1.01083236508913,93.6808824325776));
#234639=CARTESIAN_POINT('Ctrl Pts',(7.85247858747658,0.96076000607758,93.6788527840488));
#234640=CARTESIAN_POINT('Ctrl Pts',(7.8553142823438,0.937292529382736,93.6779031400515));
#234641=CARTESIAN_POINT('Ctrl Pts',(7.86148233222033,0.884252322759162,
93.6757602553155));
#234642=CARTESIAN_POINT('Ctrl Pts',(7.86475308579494,0.854672766203541,
93.6745676348455));
#234643=CARTESIAN_POINT('Ctrl Pts',(7.87395177301604,0.766954777258875,
93.6710377259206));
#234644=CARTESIAN_POINT('Ctrl Pts',(7.87940250714819,0.708768184263577,
93.6687050577511));
#234645=CARTESIAN_POINT('Ctrl Pts',(7.91181445717617,0.315943863752889,
93.6530090742436));
#234646=CARTESIAN_POINT('Ctrl Pts',(7.91809547976187,-0.0200691808325795,
93.6397912824133));
#234647=CARTESIAN_POINT('Ctrl Pts',(7.88246650305884,-0.812204302438391,
93.6090295604024));
#234648=CARTESIAN_POINT('Ctrl Pts',(7.82236783998412,-1.26630810601944,
93.5918342402346));
#234649=CARTESIAN_POINT('Ctrl Pts',(7.63483161802273,-2.11200403984446,
93.5596322899469));
#234650=CARTESIAN_POINT('Ctrl Pts',(7.51545073566851,-2.50383510961908,
93.544615627285));
#234651=CARTESIAN_POINT('Ctrl Pts',(7.35759270602529,-2.90694396725511,
93.5279838569819));
#234652=CARTESIAN_POINT('Ctrl Pts',(7.34876577606518,-2.92918678397641,
93.5270620579119));
#234653=CARTESIAN_POINT('Ctrl Pts',(7.29645218561974,-3.05928595740922,
93.5216449017439));
#234654=CARTESIAN_POINT('Ctrl Pts',(7.25069345143284,-3.16621037333604,
93.5170899067403));
#234655=CARTESIAN_POINT('Ctrl Pts',(7.19573428570986,-3.28718790017869,
93.5117818568856));
#234656=CARTESIAN_POINT('Ctrl Pts',(7.18882533294422,-3.30226990554375,
93.5111173324279));
#234657=CARTESIAN_POINT('Ctrl Pts',(7.17858516789987,-3.32443939852791,
93.5101362872784));
#234658=CARTESIAN_POINT('Ctrl Pts',(7.17529076425434,-3.33154390262833,
93.5098212556013));
#234659=CARTESIAN_POINT('Ctrl Pts',(7.16940624213313,-3.34418487774112,
93.5092595592789));
#234660=CARTESIAN_POINT('Ctrl Pts',(7.16682024312357,-3.34972326674019,
93.5090130649506));
#234661=CARTESIAN_POINT('Ctrl Pts',(7.16140827480436,-3.36127902985214,
93.5084979161466));
#234662=CARTESIAN_POINT('Ctrl Pts',(7.15858113491976,-3.367295848212,93.5082292126132));
#234663=CARTESIAN_POINT('Ctrl Pts',(7.15121190364722,-3.38292808023746,
93.5075298386109));
#234664=CARTESIAN_POINT('Ctrl Pts',(7.14665801132307,-3.39253789288611,
93.5070986638222));
#234665=CARTESIAN_POINT('Ctrl Pts',(7.12706014445318,-3.43367955364797,
93.5052472872058));
#234666=CARTESIAN_POINT('Ctrl Pts',(7.11182690932603,-3.46512042168759,
93.5038187703604));
#234667=CARTESIAN_POINT('Ctrl Pts',(7.0087836114271,-3.67425630091621,93.4942189738057));
#234668=CARTESIAN_POINT('Ctrl Pts',(6.91454293229927,-3.84867293255867,
93.4857067873669));
#234669=CARTESIAN_POINT('Ctrl Pts',(6.5249394799104,-4.50915438052681,93.4518608291704));
#234670=CARTESIAN_POINT('Ctrl Pts',(6.18404803753021,-4.96637298060165,
93.4250847676656));
#234671=CARTESIAN_POINT('Ctrl Pts',(5.44609423212617,-5.76108094856937,
93.3757759149911));
#234672=CARTESIAN_POINT('Ctrl Pts',(5.0589376286557,-6.10387315705764,93.3532033669588));
#234673=CARTESIAN_POINT('Ctrl Pts',(4.61462806830041,-6.42574496260809,
93.3308621108159));
#234674=CARTESIAN_POINT('Ctrl Pts',(4.58802473122907,-6.4447668406944,93.3295364440292));
#234675=CARTESIAN_POINT('Ctrl Pts',(4.55132901054998,-6.47066258500791,
93.3277241909724));
#234676=CARTESIAN_POINT('Ctrl Pts',(4.54133771000652,-6.47767873984393,
93.3272324102615));
#234677=CARTESIAN_POINT('Ctrl Pts',(4.52542961294611,-6.48879492937695,
93.3264520081732));
#234678=CARTESIAN_POINT('Ctrl Pts',(4.51952341173672,-6.49291005238266,
93.3261628377541));
#234679=CARTESIAN_POINT('Ctrl Pts',(4.50804243261533,-6.50088612502279,
93.325601826317));
#234680=CARTESIAN_POINT('Ctrl Pts',(4.50246829152182,-6.50474797889296,
93.3253299525591));
#234681=CARTESIAN_POINT('Ctrl Pts',(4.48915680725946,-6.51394507889376,
93.324681894441));
#234682=CARTESIAN_POINT('Ctrl Pts',(4.48141490093967,-6.51927371855084,
93.3243059497563));
#234683=CARTESIAN_POINT('Ctrl Pts',(4.45829414707282,-6.5351267446416,93.3231860741039));
#234684=CARTESIAN_POINT('Ctrl Pts',(4.44288754249752,-6.54561063315618,
93.3224436074644));
#234685=CARTESIAN_POINT('Ctrl Pts',(4.31559528936557,-6.63157400682703,
93.3163399831584));
#234686=CARTESIAN_POINT('Ctrl Pts',(4.20182912189778,-6.704235276218,93.3110808125507));
#234687=CARTESIAN_POINT('Ctrl Pts',(3.79935886917099,-6.94701768958947,
93.2931017066865));
#234688=CARTESIAN_POINT('Ctrl Pts',(3.50174532691547,-7.10168883375342,
93.2809131527402));
#234689=CARTESIAN_POINT('Ctrl Pts',(2.97881577772075,-7.33256636260571,
93.2607083088823));
#234690=CARTESIAN_POINT('Ctrl Pts',(2.75824760198039,-7.41835195616723,
93.2525243664555));
#234691=CARTESIAN_POINT('Ctrl Pts',(1.98418392025008,-7.68010433793855,
93.224300440226));
#234692=CARTESIAN_POINT('Ctrl Pts',(1.41545544807959,-7.80495566424273,
93.2044710471174));
#234693=CARTESIAN_POINT('Ctrl Pts',(0.800849768687063,-7.87044959479491,
93.1800964019728));
#234694=CARTESIAN_POINT('Ctrl Pts',(0.763402977698106,-7.87416998292571,
93.1785993274632));
#234695=CARTESIAN_POINT('Ctrl Pts',(0.715853097766556,-7.87855175660551,
93.1766840017607));
#234696=CARTESIAN_POINT('Ctrl Pts',(0.705772841400102,-7.87946115759324,
93.1762771552465));
#234697=CARTESIAN_POINT('Ctrl Pts',(0.689790695397059,-7.88087208881772,
93.1756308497309));
#234698=CARTESIAN_POINT('Ctrl Pts',(0.683889916658087,-7.88138634158845,
93.1753919558666));
#234699=CARTESIAN_POINT('Ctrl Pts',(0.672955053347862,-7.88232694196387,
93.1749487612706));
#234700=CARTESIAN_POINT('Ctrl Pts',(0.66792112377951,-7.88275509552809,
93.174744539621));
#234701=CARTESIAN_POINT('Ctrl Pts',(0.656732302666678,-7.88369594975943,
93.1742901931732));
#234702=CARTESIAN_POINT('Ctrl Pts',(0.650577217806672,-7.88420626499466,
93.1740399655663));
#234703=CARTESIAN_POINT('Ctrl Pts',(0.632905151774223,-7.88565061249343,
93.1733207171843));
#234704=CARTESIAN_POINT('Ctrl Pts',(0.62138674353115,-7.88656661839868,
93.1728509315357));
#234705=CARTESIAN_POINT('Ctrl Pts',(0.546025504451834,-7.89239362782978,
93.169770983005));
#234706=CARTESIAN_POINT('Ctrl Pts',(0.482128174153243,-7.89655451092597,
93.1671300400059));
#234707=CARTESIAN_POINT('Ctrl Pts',(0.281070754108038,-7.90719762179349,
93.1587416628477));
#234708=CARTESIAN_POINT('Ctrl Pts',(0.143790888509328,-7.91088471384464,
93.152899873522));
#234709=CARTESIAN_POINT('Ctrl Pts',(-0.106758280771778,-7.9110902322365,
93.1421039948765));
#234710=CARTESIAN_POINT('Ctrl Pts',(-0.219993158767414,-7.9087513727691,
93.1371747867954));
#234711=CARTESIAN_POINT('Ctrl Pts',(-0.41923005130492,-7.90035393812578,
93.1284483179304));
#234712=CARTESIAN_POINT('Ctrl Pts',(-0.505257665495175,-7.89531891209549,
93.1246626849966));
#234713=CARTESIAN_POINT('Ctrl Pts',(-0.788410399395188,-7.8740997076641,
93.1121688126791));
#234714=CARTESIAN_POINT('Ctrl Pts',(-0.985013203383412,-7.85192887484135,
93.1034420305356));
#234715=CARTESIAN_POINT('Ctrl Pts',(-1.71091301869714,-7.74237420288489,
93.071276949285));
#234716=CARTESIAN_POINT('Ctrl Pts',(-2.23176868919481,-7.60860577114906,
93.0484443528242));
#234717=CARTESIAN_POINT('Ctrl Pts',(-2.77033914028371,-7.41016540461729,
93.0251942740174));
#234718=CARTESIAN_POINT('Ctrl Pts',(-2.80547177393867,-7.39693574603399,
93.0236785411096));
#234719=CARTESIAN_POINT('Ctrl Pts',(-2.85654121518628,-7.37728868596842,
93.0214761654429));
#234720=CARTESIAN_POINT('Ctrl Pts',(-2.87255324179364,-7.37106871124965,
93.0207857770316));
#234721=CARTESIAN_POINT('Ctrl Pts',(-2.90037999603011,-7.36015478738467,
93.0195861473025));
#234722=CARTESIAN_POINT('Ctrl Pts',(-2.91220388562658,-7.35548442628075,
93.0190764660169));
#234723=CARTESIAN_POINT('Ctrl Pts',(-2.92462211874586,-7.35054466603471,
93.018541207372));
#234724=CARTESIAN_POINT('Ctrl Pts',(-2.92522772180758,-7.35030368082826,
93.0185151043867));
#234725=CARTESIAN_POINT('Ctrl Pts',(-2.9259183300222,-7.35002877099245,
93.0184853375885));
#234726=CARTESIAN_POINT('Ctrl Pts',(-2.92600335660089,-7.34999492282369,
93.0184816727501));
#234727=CARTESIAN_POINT('Ctrl Pts',(-2.92617008948289,-7.34992854490085,
93.0184744861885));
#234728=CARTESIAN_POINT('Ctrl Pts',(-2.92625179421347,-7.34989601590352,
93.018470964533));
#234729=CARTESIAN_POINT('Ctrl Pts',(-2.9264120154653,-7.34983222413143,
93.0184640586447));
#234730=CARTESIAN_POINT('Ctrl Pts',(-2.92649053034446,-7.34980096213115,
93.0184606744825));
#234731=CARTESIAN_POINT('Ctrl Pts',(-2.92664450045386,-7.34973965352225,
93.0184540380389));
#234732=CARTESIAN_POINT('Ctrl Pts',(-2.92671995391438,-7.34970960772961,
93.0184507858338));
#234733=CARTESIAN_POINT('Ctrl Pts',(-2.9268679244604,-7.34965068277773,
93.0184444079907));
#234734=CARTESIAN_POINT('Ctrl Pts',(-2.92694043955458,-7.34962180451414,
93.0184412824384));
#234735=CARTESIAN_POINT('Ctrl Pts',(-2.92708265159954,-7.34956516784023,
93.0184351528047));
#234736=CARTESIAN_POINT('Ctrl Pts',(-2.92715234623792,-7.34953741044554,
93.0184321488227));
#234737=CARTESIAN_POINT('Ctrl Pts',(-2.92728903056338,-7.34948297070887,
93.0184262574505));
#234738=CARTESIAN_POINT('Ctrl Pts',(-2.92735601784517,-7.34945628941226,
93.0184233701637));
#234739=CARTESIAN_POINT('Ctrl Pts',(-2.92748739593124,-7.34940395892512,
93.0184177075061));
#234740=CARTESIAN_POINT('Ctrl Pts',(-2.92755178413494,-7.34937831085107,
93.0184149322473));
#234741=CARTESIAN_POINT('Ctrl Pts',(-2.92767806810214,-7.34932800560629,
93.0184094891609));
#234742=CARTESIAN_POINT('Ctrl Pts',(-2.92773996101404,-7.34930334964586,
93.0184068214562));
#234743=CARTESIAN_POINT('Ctrl Pts',(-2.92786135409999,-7.34925498913091,
93.0184015891805));
#234744=CARTESIAN_POINT('Ctrl Pts',(-2.92792085122977,-7.34923128585779,
93.0183990247407));
#234745=CARTESIAN_POINT('Ctrl Pts',(-2.9280231723058,-7.34919052036077,
93.0183946145088));
#234746=CARTESIAN_POINT('Ctrl Pts',(-2.92806603591217,-7.34917344273937,
93.0183927670066));
#234747=CARTESIAN_POINT('Ctrl Pts',(-2.92815134395272,-7.34913945363636,
93.0183890900708));
#234748=CARTESIAN_POINT('Ctrl Pts',(-2.9281937880129,-7.34912254231274,
93.018387260653));
#234749=CARTESIAN_POINT('Ctrl Pts',(-2.92827827463916,-7.34908887878788,
93.0183836191236));
#234750=CARTESIAN_POINT('Ctrl Pts',(-2.92832031680441,-7.34907212675436,
93.0183818070292));
#234751=CARTESIAN_POINT('Ctrl Pts',(-2.92840400405459,-7.34903878007497,
93.0183781999564));
#234752=CARTESIAN_POINT('Ctrl Pts',(-2.92844564855556,-7.34902218566965,
93.018376405003));
#234753=CARTESIAN_POINT('Ctrl Pts',(-2.92852854487242,-7.34898915251876,
93.0183728320227));
#234754=CARTESIAN_POINT('Ctrl Pts',(-2.92856979595827,-7.3489727140718,
93.0183710540272));
#234755=CARTESIAN_POINT('Ctrl Pts',(-2.92865190960521,-7.34893999120279,
93.0183675147833));
#234756=CARTESIAN_POINT('Ctrl Pts',(-2.92869277154966,-7.34892370703401,
93.0183657535615));
#234757=CARTESIAN_POINT('Ctrl Pts',(-2.92877411094629,-7.34889129113694,
93.0183622476909));
#234758=CARTESIAN_POINT('Ctrl Pts',(-2.92881458788457,-7.34887515962082,
93.0183605030644));
#234759=CARTESIAN_POINT('Ctrl Pts',(-2.9288951615487,-7.34884304734552,
93.0183570302));
#234760=CARTESIAN_POINT('Ctrl Pts',(-2.92893525742463,-7.3488270669323,
93.0183553019988));
#234761=CARTESIAN_POINT('Ctrl Pts',(-2.92901507292009,-7.34879525530777,
93.0183518618147));
#234762=CARTESIAN_POINT('Ctrl Pts',(-2.92905479198797,-7.34877942432342,
93.0183501498554));
#234763=CARTESIAN_POINT('Ctrl Pts',(-2.92913385788524,-7.34874790997645,
93.0183467419819));
#234764=CARTESIAN_POINT('Ctrl Pts',(-2.92917320398037,-7.34873222691344,
93.0183450460993));
#234765=CARTESIAN_POINT('Ctrl Pts',(-2.92925152789791,-7.34870100684924,
93.0183416702081));
#234766=CARTESIAN_POINT('Ctrl Pts',(-2.92929050505235,-7.34868547012113,
93.0183399902283));
#234767=CARTESIAN_POINT('Ctrl Pts',(-2.92936809499878,-7.34865454118845,
93.018336645974));
#234768=CARTESIAN_POINT('Ctrl Pts',(-2.92940670707883,-7.34863914927437,
93.0183349817304));
#234769=CARTESIAN_POINT('Ctrl Pts',(-2.92948357075744,-7.34860850844271,
93.0183316687811));
#234770=CARTESIAN_POINT('Ctrl Pts',(-2.92952182163013,-7.34859325982102,
93.0183300201068));
#234771=CARTESIAN_POINT('Ctrl Pts',(-2.92959796681332,-7.34856290403137,
93.0183267381275));
#234772=CARTESIAN_POINT('Ctrl Pts',(-2.92963586024538,-7.34854779721999,
93.0183251048604));
#234773=CARTESIAN_POINT('Ctrl Pts',(-2.92971129424774,-7.34851772359494,
93.0183218535356));
#234774=CARTESIAN_POINT('Ctrl Pts',(-2.92974883411642,-7.34850275706726,
93.0183202355083));
#234775=CARTESIAN_POINT('Ctrl Pts',(-2.92982356494667,-7.34847296245176,
93.018317014493));
#234776=CARTESIAN_POINT('Ctrl Pts',(-2.92986075477214,-7.34845813482306,
93.0183154115538));
#234777=CARTESIAN_POINT('Ctrl Pts',(-2.92993478907014,-7.34842861660696,
93.0183122205616));
#234778=CARTESIAN_POINT('Ctrl Pts',(-2.929971632813,-7.34841392631652,93.0183106325399));
#234779=CARTESIAN_POINT('Ctrl Pts',(-2.93004497881007,-7.34838468125426,
93.018307471216));
#234780=CARTESIAN_POINT('Ctrl Pts',(-2.93008147979078,-7.34837012699614,
93.0183058979686));
#234781=CARTESIAN_POINT('Ctrl Pts',(-2.93015414359627,-7.34834115268741,
93.0183027660496));
#234782=CARTESIAN_POINT('Ctrl Pts',(-2.93019030581279,-7.34832673288514,
93.0183012074042));
#234783=CARTESIAN_POINT('Ctrl Pts',(-2.93026229579386,-7.34829802602852,
93.0182981045294));
#234784=CARTESIAN_POINT('Ctrl Pts',(-2.9302981223905,-7.34828373944558,
93.0182965603505));
#234785=CARTESIAN_POINT('Ctrl Pts',(-2.93036944483893,-7.3482552975664,
93.0182934862488));
#234786=CARTESIAN_POINT('Ctrl Pts',(-2.93040493950912,-7.34824114274692,
93.018291956377));
#234787=CARTESIAN_POINT('Ctrl Pts',(-2.93047560123915,-7.3482129631614,
93.0182889107545));
#234788=CARTESIAN_POINT('Ctrl Pts',(-2.93051076762822,-7.34819893866832,
93.0182873950328));
#234789=CARTESIAN_POINT('Ctrl Pts',(-2.93058077644006,-7.34817101829869,
93.0182843775534));
#234790=CARTESIAN_POINT('Ctrl Pts',(-2.9306156176142,-7.34815712292548,
93.0182828758496));
#234791=CARTESIAN_POINT('Ctrl Pts',(-2.93068497957464,-7.34812945938451,
93.0182798862517));
#234792=CARTESIAN_POINT('Ctrl Pts',(-2.93071949911866,-7.34811569171746,
93.0182783984113));
#234793=CARTESIAN_POINT('Ctrl Pts',(-2.93078822079913,-7.34808828241595,
93.0182754364117));
#234794=CARTESIAN_POINT('Ctrl Pts',(-2.93082242224484,-7.34807464106212,
93.0182739622823));
#234795=CARTESIAN_POINT('Ctrl Pts',(-2.93089051117575,-7.34804748302762,
93.0182710275563));
#234796=CARTESIAN_POINT('Ctrl Pts',(-2.9309243974905,-7.34803396681884,
93.0182695670102));
#234797=CARTESIAN_POINT('Ctrl Pts',(-2.930991859484,-7.34800705776353,93.0182666593073));
#234798=CARTESIAN_POINT('Ctrl Pts',(-2.9310254341537,-7.34799366532444,
93.0182652121941));
#234799=CARTESIAN_POINT('Ctrl Pts',(-2.93109227624601,-7.34796700247158,
93.018262331211));
#234800=CARTESIAN_POINT('Ctrl Pts',(-2.93112554234659,-7.34795373259001,
93.0182608973981));
#234801=CARTESIAN_POINT('Ctrl Pts',(-2.9311917704262,-7.34792731361997,
93.018258042881));
#234802=CARTESIAN_POINT('Ctrl Pts',(-2.93122473134648,-7.3479141649586,
93.0182566222223));
#234803=CARTESIAN_POINT('Ctrl Pts',(-2.93129035228967,-7.34788798715706,
93.0182537938747));
#234804=CARTESIAN_POINT('Ctrl Pts',(-2.93132301102421,-7.34787495853552,
93.0182523862413));
#234805=CARTESIAN_POINT('Ctrl Pts',(-2.93138803078484,-7.34784901955548,
93.0182495838066));
#234806=CARTESIAN_POINT('Ctrl Pts',(-2.93142039053799,-7.34783610970937,
93.0182481890602));
#234807=CARTESIAN_POINT('Ctrl Pts',(-2.9314848154289,-7.34781040705996,
93.0182454122662));
#234808=CARTESIAN_POINT('Ctrl Pts',(-2.93151687927568,-7.34779761477617,
93.0182440302743));
#234809=CARTESIAN_POINT('Ctrl Pts',(-2.9315807153871,-7.34777214605471,
93.0182412788586));
#234810=CARTESIAN_POINT('Ctrl Pts',(-2.93161248639493,-7.34775947012286,
93.0182399094889));
#234811=CARTESIAN_POINT('Ctrl Pts',(-2.93167574011761,-7.34773423280616,
93.018237183176));
#234812=CARTESIAN_POINT('Ctrl Pts',(-2.93170722114656,-7.34772167209827,
93.0182358263053));
#234813=CARTESIAN_POINT('Ctrl Pts',(-2.93176989766444,-7.34769666414404,
93.0182331248716));
#234814=CARTESIAN_POINT('Ctrl Pts',(-2.93180109202279,-7.34768421735301,
93.0182317803573));
#234815=CARTESIAN_POINT('Ctrl Pts',(-2.93186319813986,-7.34765943607196,
93.0182291035097));
#234816=CARTESIAN_POINT('Ctrl Pts',(-2.93189410849655,-7.34764710214551,
93.0182277712367));
#234817=CARTESIAN_POINT('Ctrl Pts',(-2.93195564958619,-7.3476225454186,
93.0182251187434));
#234818=CARTESIAN_POINT('Ctrl Pts',(-2.93198627895568,-7.34761032316627,
93.0182237985818));
#234819=CARTESIAN_POINT('Ctrl Pts',(-2.93204726107688,-7.34758598860034,
93.0182211701817));
#234820=CARTESIAN_POINT('Ctrl Pts',(-2.93207761225227,-7.34757387691973,
93.0182198620111));
#234821=CARTESIAN_POINT('Ctrl Pts',(-2.94508423646356,-7.34238347122519,
93.01765926164));
#234822=CARTESIAN_POINT('Ctrl Pts',(-2.95804679217719,-7.33717080182073,
93.01710060554));
#234823=CARTESIAN_POINT('Ctrl Pts',(-2.99278063307489,-7.32309617591512,
93.0156037252995));
#234824=CARTESIAN_POINT('Ctrl Pts',(-3.01452638219254,-7.31417146483269,
93.0146666483168));
#234825=CARTESIAN_POINT('Ctrl Pts',(-3.11057424210187,-7.27425118977034,
93.0105275947787));
#234826=CARTESIAN_POINT('Ctrl Pts',(-3.18444140432334,-7.24221897759433,
93.007343811271));
#234827=CARTESIAN_POINT('Ctrl Pts',(-3.76730389164086,-6.97882090731071,
92.9822086001764));
#234828=CARTESIAN_POINT('Ctrl Pts',(-4.2509630499662,-6.69521294122317,
92.9614140314136));
#234829=CARTESIAN_POINT('Ctrl Pts',(-4.96390796320805,-6.16851943345574,
92.9288120420773));
#234830=CARTESIAN_POINT('Ctrl Pts',(-5.21479734809276,-5.95792697041818,
92.9168513746901));
#234831=CARTESIAN_POINT('Ctrl Pts',(-5.55549784949814,-5.63389724494306,
92.8991416086831));
#234832=CARTESIAN_POINT('Ctrl Pts',(-5.65638669784677,-5.53259812691413,
92.8936890529697));
#234833=CARTESIAN_POINT('Ctrl Pts',(-5.81709500917299,-5.36224342708556,
92.8845699390677));
#234834=CARTESIAN_POINT('Ctrl Pts',(-5.87856229826783,-5.29478549852349,
92.880971040315));
#234835=CARTESIAN_POINT('Ctrl Pts',(-5.94872114677814,-5.21506098677468,
92.8767153443157));
#234836=CARTESIAN_POINT('Ctrl Pts',(-5.95856302462046,-5.20381312652112,
92.8761148784572));
#234837=CARTESIAN_POINT('Ctrl Pts',(-5.97331343209403,-5.18685880837321,
92.8752095975896));
#234838=CARTESIAN_POINT('Ctrl Pts',(-5.97824581915656,-5.18117308929882,
92.8749059772487));
#234839=CARTESIAN_POINT('Ctrl Pts',(-5.98701232997471,-5.17103846959063,
92.8743647162705));
#234840=CARTESIAN_POINT('Ctrl Pts',(-5.9908496323154,-5.16659231757277,
92.8741272371414));
#234841=CARTESIAN_POINT('Ctrl Pts',(-5.99891256148631,-5.15722901508154,
92.8736270656217));
#234842=CARTESIAN_POINT('Ctrl Pts',(-6.00313710043055,-5.15231093660539,
92.8733643178286));
#234843=CARTESIAN_POINT('Ctrl Pts',(-6.0142413949916,-5.13935146083918,
92.8726718602992));
#234844=CARTESIAN_POINT('Ctrl Pts',(-6.0211110547341,-5.13130145872978,
92.8722416282666));
#234845=CARTESIAN_POINT('Ctrl Pts',(-6.05173131863672,-5.09527387727819,
92.8703155891476));
#234846=CARTESIAN_POINT('Ctrl Pts',(-6.07530296155246,-5.06714532043659,
92.8688103649413));
#234847=CARTESIAN_POINT('Ctrl Pts',(-6.23932736486503,-4.86862161718658,
92.8581700690522));
#234848=CARTESIAN_POINT('Ctrl Pts',(-6.37276443058871,-4.69260352104712,
92.8486005879175));
#234849=CARTESIAN_POINT('Ctrl Pts',(-6.63473670391265,-4.31522186172175,
92.8281266604278));
#234850=CARTESIAN_POINT('Ctrl Pts',(-6.76187851940734,-4.11313299884776,
92.8172018949812));
#234851=CARTESIAN_POINT('Ctrl Pts',(-6.93258929471882,-3.81242820574652,
92.8012972668138));
#234852=CARTESIAN_POINT('Ctrl Pts',(-6.98359222133139,-3.71817735566706,
92.7963592173527));
#234853=CARTESIAN_POINT('Ctrl Pts',(-7.05855329049864,-3.57266596325531,
92.7888296792713));
#234854=CARTESIAN_POINT('Ctrl Pts',(-7.08390243797734,-3.52213613161424,
92.7862319367448));
#234855=CARTESIAN_POINT('Ctrl Pts',(-7.13736990450129,-3.41264390853482,
92.7806434982027));
#234856=CARTESIAN_POINT('Ctrl Pts',(-7.16530403736545,-3.35359594421681,
92.777654715863));
#234857=CARTESIAN_POINT('Ctrl Pts',(-7.40717742334856,-2.82549479661754,
92.751169486616));
#234858=CARTESIAN_POINT('Ctrl Pts',(-7.57554356132076,-2.33687131199937,
92.7284906711403));
#234859=CARTESIAN_POINT('Ctrl Pts',(-7.7030955993067,-1.80205595855616,
92.7061131792509));
#234860=CARTESIAN_POINT('Ctrl Pts',(-7.71080382685018,-1.76878259633902,
92.7047302386655));
#234861=CARTESIAN_POINT('Ctrl Pts',(-7.72089515083701,-1.72390237647433,
92.7028772502103));
#234862=CARTESIAN_POINT('Ctrl Pts',(-7.72346794420973,-1.71233882460143,
92.702400923816));
#234863=CARTESIAN_POINT('Ctrl Pts',(-7.72746610123569,-1.69417656325994,
92.7016545075691));
#234864=CARTESIAN_POINT('Ctrl Pts',(-7.7289090035783,-1.68758175741215,
92.7013838367324));
#234865=CARTESIAN_POINT('Ctrl Pts',(-7.73166375920978,-1.67491346715052,
92.7008645747515));
#234866=CARTESIAN_POINT('Ctrl Pts',(-7.73297690164791,-1.66884026998875,
92.7006159410307));
#234867=CARTESIAN_POINT('Ctrl Pts',(-7.73604615324661,-1.65456377712249,
92.7000321747194));
#234868=CARTESIAN_POINT('Ctrl Pts',(-7.73779637321535,-1.64635921504607,
92.6996972375978));
#234869=CARTESIAN_POINT('Ctrl Pts',(-7.74137901547739,-1.62943283568601,
92.6990073731598));
#234870=CARTESIAN_POINT('Ctrl Pts',(-7.74320975716889,-1.62071067265692,
92.6986525019206));
#234871=CARTESIAN_POINT('Ctrl Pts',(-7.74788943436624,-1.59822646151356,
92.6977392871197));
#234872=CARTESIAN_POINT('Ctrl Pts',(-7.75071644955372,-1.58445985457751,
92.6971816703276));
#234873=CARTESIAN_POINT('Ctrl Pts',(-7.77421687419262,-1.46845275206103,
92.6924955646544));
#234874=CARTESIAN_POINT('Ctrl Pts',(-7.79290344259698,-1.36581788638988,
92.6884332824482));
#234875=CARTESIAN_POINT('Ctrl Pts',(-7.87742479802568,-0.843127933224769,
92.66814279541));
#234876=CARTESIAN_POINT('Ctrl Pts',(-7.91135110646884,-0.418615950099376,
92.6530110698391));
#234877=CARTESIAN_POINT('Ctrl Pts',(-7.91099726067231,0.00658343642006579,
92.6384370102158));
#234878=CARTESIAN_POINT('',(-7.91923391390641,-9.72790312405945E-5,90.6423314461212));
#234879=CARTESIAN_POINT('Ctrl Pts',(-7.91099714745356,0.0067181084832415,
92.642331465206));
#234880=CARTESIAN_POINT('Ctrl Pts',(-7.91079160367377,0.248758894166455,
92.6326073364901));
#234881=CARTESIAN_POINT('Ctrl Pts',(-7.89947448308587,0.490284791307527,
92.6228832077741));
#234882=CARTESIAN_POINT('Ctrl Pts',(-7.87720914932586,0.730408801820563,
92.6131590790582));
#234883=CARTESIAN_POINT('Ctrl Pts',(-7.85470833965837,0.973072339469931,
92.603332108945));
#234884=CARTESIAN_POINT('Ctrl Pts',(-7.82102660107798,1.21430427540786,
92.5935051388318));
#234885=CARTESIAN_POINT('Ctrl Pts',(-7.77638033720727,1.45321362885717,
92.5836781687186));
#234886=CARTESIAN_POINT('Ctrl Pts',(-7.73122410802533,1.69485188887608,
92.5737389515004));
#234887=CARTESIAN_POINT('Ctrl Pts',(-7.67485145389126,1.93411430807153,
92.5637997342821));
#234888=CARTESIAN_POINT('Ctrl Pts',(-7.60753419602398,2.17010240687525,
92.5538605170639));
#234889=CARTESIAN_POINT('Ctrl Pts',(-7.5741006142655,2.28730752849412,92.5489241360821));
#234890=CARTESIAN_POINT('Ctrl Pts',(-7.53796808386738,2.40370532976846,
92.5439877551003));
#234891=CARTESIAN_POINT('Ctrl Pts',(-7.49917423568835,2.51918772281624,
92.5390513741185));
#234892=CARTESIAN_POINT('Ctrl Pts',(-7.43818801125248,2.70073287678758,
92.5312910911719));
#234893=CARTESIAN_POINT('Ctrl Pts',(-7.37049778424932,2.88038206616635,
92.5235308082253));
#234894=CARTESIAN_POINT('Ctrl Pts',(-7.29623629942042,3.0575900416864,92.5157705252788));
#234895=CARTESIAN_POINT('Ctrl Pts',(-7.22206419200328,3.23458473854346,
92.5080195822209));
#234896=CARTESIAN_POINT('Ctrl Pts',(-7.14133670557192,3.4091437429375,92.500268639163));
#234897=CARTESIAN_POINT('Ctrl Pts',(-7.05423680001995,3.58073514368827,
92.4925176961052));
#234898=CARTESIAN_POINT('Ctrl Pts',(-6.96722404488927,3.75215485351964,
92.4847745084857));
#234899=CARTESIAN_POINT('Ctrl Pts',(-6.87385172440213,3.92061255348817,
92.4770313208662));
#234900=CARTESIAN_POINT('Ctrl Pts',(-6.77435153654204,4.08559448053162,
92.4692881332468));
#234901=CARTESIAN_POINT('Ctrl Pts',(-6.67493074056457,4.25044476736347,
92.4615511239699));
#234902=CARTESIAN_POINT('Ctrl Pts',(-6.56939199619968,4.41182449723104,
92.4538141146929));
#234903=CARTESIAN_POINT('Ctrl Pts',(-6.45801379380717,4.56924269863139,
92.446077105416));
#234904=CARTESIAN_POINT('Ctrl Pts',(-6.34670191090367,4.72656716629882,
92.4383447030953));
#234905=CARTESIAN_POINT('Ctrl Pts',(-6.22955770038984,4.87993451051667,
92.4306123007746));
#234906=CARTESIAN_POINT('Ctrl Pts',(-6.10690404949791,5.02888098191098,
92.4228798984539));
#234907=CARTESIAN_POINT('Ctrl Pts',(-5.98429861673466,5.1777688988304,92.4151505359283));
#234908=CARTESIAN_POINT('Ctrl Pts',(-5.8561882852263,5.32223912764058,92.4074211734027));
#234909=CARTESIAN_POINT('Ctrl Pts',(-5.72293751723684,5.46185931472087,
92.3996918108771));
#234910=CARTESIAN_POINT('Ctrl Pts',(-5.58968680123665,5.60147944732678,
92.3919624513673));
#234911=CARTESIAN_POINT('Ctrl Pts',(-5.45129589232242,5.73624927436528,
92.3842330918574));
#234912=CARTESIAN_POINT('Ctrl Pts',(-5.30816784116512,5.86577148975482,
92.3765037323475));
#234913=CARTESIAN_POINT('Ctrl Pts',(-5.16503261591601,5.99530019726283,
92.3687739854144));
#234914=CARTESIAN_POINT('Ctrl Pts',(-5.0171600413678,6.11958052746997,92.3610442384812));
#234915=CARTESIAN_POINT('Ctrl Pts',(-4.86498801307516,6.23825397307893,
92.353314491548));
#234916=CARTESIAN_POINT('Ctrl Pts',(-4.71278047387849,6.35695511235396,
92.3455829407992));
#234917=CARTESIAN_POINT('Ctrl Pts',(-4.55627176615189,6.47004654044728,
92.3378513900503));
#234918=CARTESIAN_POINT('Ctrl Pts',(-4.39593068929494,6.57721174776325,
92.3301198393014));
#234919=CARTESIAN_POINT('Ctrl Pts',(-4.23552280536625,6.68442160610585,
92.3223850671555));
#234920=CARTESIAN_POINT('Ctrl Pts',(-4.07127967099671,6.78570012743835,
92.3146502950096));
#234921=CARTESIAN_POINT('Ctrl Pts',(-3.90369674888765,6.88077558802233,
92.3069155228637));
#234922=CARTESIAN_POINT('Ctrl Pts',(-3.73591398405815,6.97596442614174,
92.2991715269981));
#234923=CARTESIAN_POINT('Ctrl Pts',(-3.56478378998337,7.06493525327135,
92.2914275311324));
#234924=CARTESIAN_POINT('Ctrl Pts',(-3.39082472169122,7.14746309586609,
92.2836835352668));
#234925=CARTESIAN_POINT('Ctrl Pts',(-3.216752745237,7.23004450317073,92.2759345131593));
#234926=CARTESIAN_POINT('Ctrl Pts',(-3.0398485657435,7.3061744546806,92.2681854910519));
#234927=CARTESIAN_POINT('Ctrl Pts',(-2.86064801984975,7.37567718291207,
92.2604364689444));
#234928=CARTESIAN_POINT('Ctrl Pts',(-2.68117361330881,7.44528612768456,
92.2526756045058));
#234929=CARTESIAN_POINT('Ctrl Pts',(-2.49939616920984,7.50824750455819,
92.2449147400672));
#234930=CARTESIAN_POINT('Ctrl Pts',(-2.3158650600953,7.56443586947697,92.2371538756286));
#234931=CARTESIAN_POINT('Ctrl Pts',(-2.18965234228518,7.60307611025098,
92.2318167979088));
#234932=CARTESIAN_POINT('Ctrl Pts',(-2.06261051400034,7.63851433241825,
92.2264797201889));
#234933=CARTESIAN_POINT('Ctrl Pts',(-1.93491995010981,7.67072394149777,
92.2211426424691));
#234934=CARTESIAN_POINT('Ctrl Pts',(-1.74318830671347,7.719087744537,92.213128842146));
#234935=CARTESIAN_POINT('Ctrl Pts',(-1.54940556761321,7.7603185217876,92.2051150418229));
#234936=CARTESIAN_POINT('Ctrl Pts',(-1.3541383791836,7.79424340459175,92.1971012414999));
#234937=CARTESIAN_POINT('Ctrl Pts',(-1.15909377229931,7.82812961703403,
92.1890965759632));
#234938=CARTESIAN_POINT('Ctrl Pts',(-0.962568414586113,7.85472647235197,
92.1810919104265));
#234939=CARTESIAN_POINT('Ctrl Pts',(-0.765142846728391,7.87391118975191,
92.1730872448899));
#234940=CARTESIAN_POINT('Ctrl Pts',(-0.567908804462299,7.89307729576129,
92.1650903448028));
#234941=CARTESIAN_POINT('Ctrl Pts',(-0.369776623316966,7.90484556132773,
92.1570934447159));
#234942=CARTESIAN_POINT('Ctrl Pts',(-0.171336154412708,7.90914438622732,
92.1490965446288));
#234943=CARTESIAN_POINT('Ctrl Pts',(0.0269454712136357,7.91343977009775,
92.1411060457251));
#234944=CARTESIAN_POINT('Ctrl Pts',(0.225534559741134,7.91027762249422,
92.1331155468214));
#234945=CARTESIAN_POINT('Ctrl Pts',(0.423836614784747,7.89963818943424,
92.1251250479177));
#234946=CARTESIAN_POINT('Ctrl Pts',(0.622013562858758,7.88900546869616,
92.1171395901474));
#234947=CARTESIAN_POINT('Ctrl Pts',(0.81990350528098,7.87090488351985,92.109154132377));
#234948=CARTESIAN_POINT('Ctrl Pts',(1.0169120070025,7.84536875933911,92.1011686746067));
#234949=CARTESIAN_POINT('Ctrl Pts',(1.22037994612897,7.81899536674473,92.0929213927822));
#234950=CARTESIAN_POINT('Ctrl Pts',(1.42290729803654,7.78469056794254,92.0846741109578));
#234951=CARTESIAN_POINT('Ctrl Pts',(1.62384370156454,7.74254820023028,92.0764268291333));
#234952=CARTESIAN_POINT('Ctrl Pts',(1.81826927566203,7.70177134799036,92.0684467793498));
#234953=CARTESIAN_POINT('Ctrl Pts',(2.01120503667431,7.65365695866286,92.0604667295663));
#234954=CARTESIAN_POINT('Ctrl Pts',(2.2020710068714,7.59834220607998,92.0524866797829));
#234955=CARTESIAN_POINT('Ctrl Pts',(2.39292181993292,7.54303184617749,92.0445072637148));
#234956=CARTESIAN_POINT('Ctrl Pts',(2.58170284843214,7.48052235570758,92.0365278476466));
#234957=CARTESIAN_POINT('Ctrl Pts',(2.76784823604333,7.41100108907237,92.0285484315785));
#234958=CARTESIAN_POINT('Ctrl Pts',(2.95400744904045,7.34147465895525,92.0205684228634));
#234959=CARTESIAN_POINT('Ctrl Pts',(3.13753031764566,7.26493553203591,92.0125884141483));
#234960=CARTESIAN_POINT('Ctrl Pts',(3.31786960790439,7.18161975218295,92.0046084054332));
#234961=CARTESIAN_POINT('Ctrl Pts',(3.49825000805026,7.09828497978377,91.9966265776067));
#234962=CARTESIAN_POINT('Ctrl Pts',(3.67544507989323,7.00817061607556,91.9886447497801));
#234963=CARTESIAN_POINT('Ctrl Pts',(3.8489305540484,6.91155949045602,91.9806629219536));
#234964=CARTESIAN_POINT('Ctrl Pts',(4.022545022454,6.81487653012067,91.9726751592792));
#234965=CARTESIAN_POINT('Ctrl Pts',(4.19244409089721,6.71168732123721,91.9646873966048));
#234966=CARTESIAN_POINT('Ctrl Pts',(4.35813006549708,6.60231954181335,91.9566996339304));
#234967=CARTESIAN_POINT('Ctrl Pts',(4.52388901409126,6.49290359293077,91.9487083531614));
#234968=CARTESIAN_POINT('Ctrl Pts',(4.68543089476072,6.37730383867855,91.9407170723923));
#234969=CARTESIAN_POINT('Ctrl Pts',(4.84228921294199,6.25588971915471,91.9327257916232));
#234970=CARTESIAN_POINT('Ctrl Pts',(4.99929511394555,6.13436136508704,91.9247269921214));
#234971=CARTESIAN_POINT('Ctrl Pts',(5.15160839303579,6.00700793154305,91.9167281926196));
#234972=CARTESIAN_POINT('Ctrl Pts',(5.29879693936175,5.87423799274515,91.9087293931178));
#234973=CARTESIAN_POINT('Ctrl Pts',(5.33250499978858,5.84383197793232,91.906897565685));
#234974=CARTESIAN_POINT('Ctrl Pts',(5.36594444023649,5.8131420336051,91.9050657382523));
#234975=CARTESIAN_POINT('Ctrl Pts',(5.39911035365196,5.7821733274858,91.9032339108195));
#234976=CARTESIAN_POINT('Ctrl Pts',(5.54624641353908,5.64478487865534,91.8951072577865));
#234977=CARTESIAN_POINT('Ctrl Pts',(5.68825553927663,5.50166497693222,91.8869806047535));
#234978=CARTESIAN_POINT('Ctrl Pts',(5.82468286059035,5.35322244760527,91.8788539517205));
#234979=CARTESIAN_POINT('Ctrl Pts',(5.96099404885058,5.20490627921566,91.870734216459));
#234980=CARTESIAN_POINT('Ctrl Pts',(6.09173269064198,5.05127674977003,91.8626144811975));
#234981=CARTESIAN_POINT('Ctrl Pts',(6.21647985837717,4.89278031086529,91.8544947459359));
#234982=CARTESIAN_POINT('Ctrl Pts',(6.34113654498359,4.73439883197893,91.8463809000491));
#234983=CARTESIAN_POINT('Ctrl Pts',(6.45981022575428,4.57115773181444,91.8382670541622));
#234984=CARTESIAN_POINT('Ctrl Pts',(6.5721210880426,4.40353782816791,91.8301532082754));
#234985=CARTESIAN_POINT('Ctrl Pts',(6.68435214928241,4.2360370247027,91.8220451275781));
#234986=CARTESIAN_POINT('Ctrl Pts',(6.79022923455868,4.06416388914116,91.8139370468808));
#234987=CARTESIAN_POINT('Ctrl Pts',(6.88941462589896,3.88842990324494,91.8058289661835));
#234988=CARTESIAN_POINT('Ctrl Pts',(6.9885574166138,3.71277139598132,91.7977243679477));
#234989=CARTESIAN_POINT('Ctrl Pts',(7.08101408766959,3.533255621941,91.7896197697119));
#234990=CARTESIAN_POINT('Ctrl Pts',(7.16649139146795,3.35042118785323,91.7815151714761));
#234991=CARTESIAN_POINT('Ctrl Pts',(7.2519419775556,3.16764390247395,91.7734131065012));
#234992=CARTESIAN_POINT('Ctrl Pts',(7.33041741232535,2.98155031436175,91.7653110415264));
#234993=CARTESIAN_POINT('Ctrl Pts',(7.40167113613748,2.79270216680357,91.7572089765515));
#234994=CARTESIAN_POINT('Ctrl Pts',(7.43957382506254,2.69224632803443,91.7528991660326));
#234995=CARTESIAN_POINT('Ctrl Pts',(7.47543385802744,2.59101143369428,91.7485893555137));
#234996=CARTESIAN_POINT('Ctrl Pts',(7.50921967833794,2.48908433414023,91.7442795449949));
#234997=CARTESIAN_POINT('Ctrl Pts',(7.57419722825957,2.29305614424353,91.7359908331753));
#234998=CARTESIAN_POINT('Ctrl Pts',(7.63147188357436,2.09455103469157,91.7277021213557));
#234999=CARTESIAN_POINT('Ctrl Pts',(7.68088318079123,1.89418968507339,91.7194134095361));
#235000=CARTESIAN_POINT('Ctrl Pts',(7.73032296313793,1.69371282909579,91.7111199193552));
#235001=CARTESIAN_POINT('Ctrl Pts',(7.77189026893824,1.4913778811092,91.7028264291743));
#235002=CARTESIAN_POINT('Ctrl Pts',(7.80547566980551,1.28781620120039,91.6945329389933));
#235003=CARTESIAN_POINT('Ctrl Pts',(7.83908245720586,1.08412489715467,91.6862341676784));
#235004=CARTESIAN_POINT('Ctrl Pts',(7.86469714640173,0.879205590369583,
91.6779353963635));
#235005=CARTESIAN_POINT('Ctrl Pts',(7.8822620206768,0.673696101663093,91.6696366250486));
#235006=CARTESIAN_POINT('Ctrl Pts',(7.8998473414792,0.467947388051725,91.6613281934849));
#235007=CARTESIAN_POINT('Ctrl Pts',(7.90936409203439,0.261607411075234,
91.6530197619213));
#235008=CARTESIAN_POINT('Ctrl Pts',(7.91080659728757,0.0553170887840625,
91.6447113303576));
#235009=CARTESIAN_POINT('Ctrl Pts',(7.91224999237583,-0.15110048737013,
91.6363977735898));
#235010=CARTESIAN_POINT('Ctrl Pts',(7.90560920453027,-0.35746805535786,
91.6280842168221));
#235011=CARTESIAN_POINT('Ctrl Pts',(7.8909306428383,-0.563147041114041,
91.6197706600543));
#235012=CARTESIAN_POINT('Ctrl Pts',(7.87623603319375,-0.769050894039098,
91.6114480141422));
#235013=CARTESIAN_POINT('Ctrl Pts',(7.85348611317857,-0.974264368778665,
91.6031253682302));
#235014=CARTESIAN_POINT('Ctrl Pts',(7.82277907762377,-1.17815470235951,
91.5948027223181));
#235015=CARTESIAN_POINT('Ctrl Pts',(7.81112303868708,-1.25554913735121,
91.5916435412688));
#235016=CARTESIAN_POINT('Ctrl Pts',(7.79832100536156,-1.33275302809533,
91.5884843602194));
#235017=CARTESIAN_POINT('Ctrl Pts',(7.78438026655081,-1.40973219645945,
91.58532517917));
#235018=CARTESIAN_POINT('Ctrl Pts',(7.74599703014416,-1.6216800464133,91.5766269606096));
#235019=CARTESIAN_POINT('Ctrl Pts',(7.69894391847647,-1.83211167553014,
91.5679287420491));
#235020=CARTESIAN_POINT('Ctrl Pts',(7.64335825120228,-2.04034204087895,
91.5592305234887));
#235021=CARTESIAN_POINT('Ctrl Pts',(7.58782142338809,-2.24838944793834,
91.5505399474793));
#235022=CARTESIAN_POINT('Ctrl Pts',(7.52376706861353,-2.45423923232996,
91.54184937147));
#235023=CARTESIAN_POINT('Ctrl Pts',(7.45138307374014,-2.65721871293632,
91.5331587954606));
#235024=CARTESIAN_POINT('Ctrl Pts',(7.37726312337087,-2.86506616671167,
91.5242597969509));
#235025=CARTESIAN_POINT('Ctrl Pts',(7.29440904556744,-3.06990368582867,
91.5153607984413));
#235026=CARTESIAN_POINT('Ctrl Pts',(7.20307723345002,-3.27102420794376,
91.5064617999317));
#235027=CARTESIAN_POINT('Ctrl Pts',(7.11414729877863,-3.46685558890633,
91.4977968305442));
#235028=CARTESIAN_POINT('Ctrl Pts',(7.01717995027879,-3.6591627506936,91.4891318611568));
#235029=CARTESIAN_POINT('Ctrl Pts',(6.91246148452419,-3.84731038843626,
91.4804668917693));
#235030=CARTESIAN_POINT('Ctrl Pts',(6.80350056224454,-4.04308044661513,
91.4714508786986));
#235031=CARTESIAN_POINT('Ctrl Pts',(6.68614748120441,-4.23434671547093,
91.4624348656279));
#235032=CARTESIAN_POINT('Ctrl Pts',(6.5607799042522,-4.42041718030781,91.4534188525572));
#235033=CARTESIAN_POINT('Ctrl Pts',(6.43541232730008,-4.60648764514457,
91.4444028394866));
#235034=CARTESIAN_POINT('Ctrl Pts',(6.30203035495867,-4.78736203649927,
91.4353868264159));
#235035=CARTESIAN_POINT('Ctrl Pts',(6.16106651317211,-4.96237648917021,
91.4263708133453));
#235036=CARTESIAN_POINT('Ctrl Pts',(6.03895158395946,-5.11398896814523,
91.4185603721431));
#235037=CARTESIAN_POINT('Ctrl Pts',(5.91119909586136,-5.26113814216653,
91.410749930941));
#235038=CARTESIAN_POINT('Ctrl Pts',(5.77817932597718,-5.40338455755741,
91.4029394897388));
#235039=CARTESIAN_POINT('Ctrl Pts',(5.64516914655071,-5.54562071726802,
91.3951296116537));
#235040=CARTESIAN_POINT('Ctrl Pts',(5.50689268232727,-5.68295456522088,
91.3873197335687));
#235041=CARTESIAN_POINT('Ctrl Pts',(5.36375856562433,-5.81498194749491,
91.3795098554836));
#235042=CARTESIAN_POINT('Ctrl Pts',(5.22060950466014,-5.9470231144049,91.3716991619894));
#235043=CARTESIAN_POINT('Ctrl Pts',(5.07260204044028,-6.0737564739082,91.3638884684953));
#235044=CARTESIAN_POINT('Ctrl Pts',(4.92017961795182,-6.19481666614045,
91.3560777750011));
#235045=CARTESIAN_POINT('Ctrl Pts',(4.76764902803233,-6.31596276942031,
91.3482615386043));
#235046=CARTESIAN_POINT('Ctrl Pts',(4.61069749646039,-6.43142744275326,
91.3404453022075));
#235047=CARTESIAN_POINT('Ctrl Pts',(4.4498000294716,-6.5408868433657,91.3326290658107));
#235048=CARTESIAN_POINT('Ctrl Pts',(4.28884307636006,-6.65038671270313,
91.3248099396382));
#235049=CARTESIAN_POINT('Ctrl Pts',(4.12393757723136,-6.75387669527379,
91.3169908134656));
#235050=CARTESIAN_POINT('Ctrl Pts',(3.95558523923625,-6.85107775573569,
91.3091716872931));
#235051=CARTESIAN_POINT('Ctrl Pts',(3.78704569837821,-6.94838690092639,
91.3013438664815));
#235052=CARTESIAN_POINT('Ctrl Pts',(3.61505197141565,-7.03939298604097,
91.2935160456699));
#235053=CARTESIAN_POINT('Ctrl Pts',(3.4401289372587,-7.12386369149743,91.2856882248584));
#235054=CARTESIAN_POINT('Ctrl Pts',(3.30402657414807,-7.18958781228949,
91.2795976324124));
#235055=CARTESIAN_POINT('Ctrl Pts',(3.16615130851551,-7.25135639975824,
91.2735070399665));
#235056=CARTESIAN_POINT('Ctrl Pts',(3.02675743534559,-7.30908068279317,
91.2674164475206));
#235057=CARTESIAN_POINT('Ctrl Pts',(2.84098615749911,-7.38601027502208,
91.2592994685186));
#235058=CARTESIAN_POINT('Ctrl Pts',(2.65214791877309,-7.45590820058209,
91.2511824895166));
#235059=CARTESIAN_POINT('Ctrl Pts',(2.46080376501156,-7.51853481937172,
91.2430655105146));
#235060=CARTESIAN_POINT('Ctrl Pts',(2.26959957285665,-7.58111562896357,
91.234954468801));
#235061=CARTESIAN_POINT('Ctrl Pts',(2.07589342409468,-7.63643563719126,
91.2268434270874));
#235062=CARTESIAN_POINT('Ctrl Pts',(1.88026521682142,-7.68430372346197,
91.2187323853738));
#235063=CARTESIAN_POINT('Ctrl Pts',(1.68475228992261,-7.73214360188379,
91.210626123359));
#235064=CARTESIAN_POINT('Ctrl Pts',(1.48731987376807,-7.77254023878968,
91.2025198613443));
#235065=CARTESIAN_POINT('Ctrl Pts',(1.28856242101603,-7.80535251523884,
91.1944135993296));
#235066=CARTESIAN_POINT('Ctrl Pts',(1.08989386305475,-7.83815011631151,
91.1863109628618));
#235067=CARTESIAN_POINT('Ctrl Pts',(0.889901766226695,-7.8633700695686,
91.178208326394));
#235068=CARTESIAN_POINT('Ctrl Pts',(0.689190725560644,-7.88092235362088,
91.1701056899262));
#235069=CARTESIAN_POINT('Ctrl Pts',(0.488540969893319,-7.89846927826839,
91.1620055275129));
#235070=CARTESIAN_POINT('Ctrl Pts',(0.287173027364239,-7.90835317547818,
91.1539053650996));
#235071=CARTESIAN_POINT('Ctrl Pts',(0.0856971434646774,-7.91053582253453,
91.1458052026864));
#235072=CARTESIAN_POINT('Ctrl Pts',(-0.117741213928936,-7.91273972963904,
91.1376261407357));
#235073=CARTESIAN_POINT('Ctrl Pts',(-0.321289296473831,-7.90709153012045,
91.1294470787851));
#235074=CARTESIAN_POINT('Ctrl Pts',(-0.524317403790099,-7.89360578316924,
91.1212680168345));
#235075=CARTESIAN_POINT('Ctrl Pts',(-0.725385892030624,-7.88025020010186,
91.1131678988588));
#235076=CARTESIAN_POINT('Ctrl Pts',(-0.925944074935925,-7.85920774109845,
91.1050677808831));
#235077=CARTESIAN_POINT('Ctrl Pts',(-1.12538375364369,-7.83054483462261,
91.0969676629074));
#235078=CARTESIAN_POINT('Ctrl Pts',(-1.32485027342461,-7.80187807062366,
91.0888664547983));
#235079=CARTESIAN_POINT('Ctrl Pts',(-1.52319767124596,-7.76558885942882,
91.0807652466892));
#235080=CARTESIAN_POINT('Ctrl Pts',(-1.71982572413473,-7.7217951590679,
91.0726640385801));
#235081=CARTESIAN_POINT('Ctrl Pts',(-1.91650563407373,-7.67798990892003,
91.0645606939256));
#235082=CARTESIAN_POINT('Ctrl Pts',(-2.11146498173309,-7.62667629233913,
91.0564573492712));
#235083=CARTESIAN_POINT('Ctrl Pts',(-2.30411600173069,-7.56802288914143,
91.0483540046167));
#235084=CARTESIAN_POINT('Ctrl Pts',(-2.49994911305512,-7.50840068502274,
91.0401168138879));
#235085=CARTESIAN_POINT('Ctrl Pts',(-2.69339664437544,-7.44119420382474,
91.0318796231591));
#235086=CARTESIAN_POINT('Ctrl Pts',(-2.88385978677335,-7.36663245521531,
91.0236424324303));
#235087=CARTESIAN_POINT('Ctrl Pts',(-3.0714720878476,-7.29318674255606,
91.0155285354969));
#235088=CARTESIAN_POINT('Ctrl Pts',(-3.25618843353923,-7.21260456913757,
91.0074146385636));
#235089=CARTESIAN_POINT('Ctrl Pts',(-3.43745874062739,-7.12515251812088,
90.9993007416302));
#235090=CARTESIAN_POINT('Ctrl Pts',(-3.62286075613152,-7.03570716560334,
90.9910019040037));
#235091=CARTESIAN_POINT('Ctrl Pts',(-3.8046574518437,-6.93907520016753,
90.9827030663772));
#235092=CARTESIAN_POINT('Ctrl Pts',(-3.98228874073508,-6.83559049281148,
90.9744042287506));
#235093=CARTESIAN_POINT('Ctrl Pts',(-4.15992002962658,-6.73210578545535,
90.9661053911241));
#235094=CARTESIAN_POINT('Ctrl Pts',(-4.33338563008723,-6.62176855699551,
90.9578065534975));
#235095=CARTESIAN_POINT('Ctrl Pts',(-4.50215861176599,-6.50495878807094,
90.949507715871));
#235096=CARTESIAN_POINT('Ctrl Pts',(-4.66330827066495,-6.39342521065219,
90.9415837292265));
#235097=CARTESIAN_POINT('Ctrl Pts',(-4.82052558239728,-6.27575117870101,
90.933659742582));
#235098=CARTESIAN_POINT('Ctrl Pts',(-4.97331335357888,-6.15224148478536,
90.9257357559375));
#235099=CARTESIAN_POINT('Ctrl Pts',(-5.1259375334243,-6.02886403388696,
90.9178202535818));
#235100=CARTESIAN_POINT('Ctrl Pts',(-5.27414135532592,-5.89966357935469,
90.909904751226));
#235101=CARTESIAN_POINT('Ctrl Pts',(-5.41745581421224,-5.76498859505012,
90.9019892488702));
#235102=CARTESIAN_POINT('Ctrl Pts',(-5.56064046996523,-5.63043558891217,
90.8940809157632));
#235103=CARTESIAN_POINT('Ctrl Pts',(-5.69894433647337,-5.49041816343139,
90.8861725826561));
#235104=CARTESIAN_POINT('Ctrl Pts',(-5.83193056651693,-5.34532570264203,
90.8782642495491));
#235105=CARTESIAN_POINT('Ctrl Pts',(-5.96479952625543,-5.20036118770943,
90.8703628901915));
#235106=CARTESIAN_POINT('Ctrl Pts',(-6.09235996748979,-5.05033081057702,
90.8624615308338));
#235107=CARTESIAN_POINT('Ctrl Pts',(-6.21421105581252,-4.89566154404259,
90.8545601714762));
#235108=CARTESIAN_POINT('Ctrl Pts',(-6.33599940615083,-4.74107191272658,
90.8466628803248));
#235109=CARTESIAN_POINT('Ctrl Pts',(-6.45208404818364,-4.58184841806269,
90.8387655891734));
#235110=CARTESIAN_POINT('Ctrl Pts',(-6.56210327760371,-4.41845239581266,
90.830868298022));
#235111=CARTESIAN_POINT('Ctrl Pts',(-6.67208510415121,-4.25511192276645,
90.8229736916865));
#235112=CARTESIAN_POINT('Ctrl Pts',(-6.77600543513875,-4.08760203167126,
90.815079085351));
#235113=CARTESIAN_POINT('Ctrl Pts',(-6.87354472814376,-3.9164146703595,
90.8071844790155));
#235114=CARTESIAN_POINT('Ctrl Pts',(-6.94203826633047,-3.79620436630813,
90.8016407693591));
#235115=CARTESIAN_POINT('Ctrl Pts',(-7.00738614932013,-3.67418133657432,
90.7960970597027));
#235116=CARTESIAN_POINT('Ctrl Pts',(-7.06949083333909,-3.5505239553247,
90.7905533500463));
#235117=CARTESIAN_POINT('Ctrl Pts',(-7.16340878593694,-3.36352279343119,
90.7821698622474));
#235118=CARTESIAN_POINT('Ctrl Pts',(-7.24982532033329,-3.17294811778614,
90.7737863744485));
#235119=CARTESIAN_POINT('Ctrl Pts',(-7.3285066088175,-2.97941468824301,
90.7654028866496));
#235120=CARTESIAN_POINT('Ctrl Pts',(-7.40729971606535,-2.78560621657449,
90.7570074845665));
#235121=CARTESIAN_POINT('Ctrl Pts',(-7.47833551473938,-2.58883084456481,
90.7486120824832));
#235122=CARTESIAN_POINT('Ctrl Pts',(-7.54142969395733,-2.38971947539844,
90.7402166804001));
#235123=CARTESIAN_POINT('Ctrl Pts',(-7.60467134316919,-2.19014272332732,
90.7318016557477));
#235124=CARTESIAN_POINT('Ctrl Pts',(-7.65993415822487,-1.98821931382836,
90.7233866310954));
#235125=CARTESIAN_POINT('Ctrl Pts',(-7.70708407564648,-1.78459408575633,
90.7149716064431));
#235126=CARTESIAN_POINT('Ctrl Pts',(-7.75428929441626,-1.58073002906592,
90.7065467119493));
#235127=CARTESIAN_POINT('Ctrl Pts',(-7.79336255777397,-1.37516043548086,
90.6981218174556));
#235128=CARTESIAN_POINT('Ctrl Pts',(-7.82422139285953,-1.16853780234929,
90.6896969229619));
#235129=CARTESIAN_POINT('Ctrl Pts',(-7.85514399266982,-0.961488217413219,
90.6812546198046));
#235130=CARTESIAN_POINT('Ctrl Pts',(-7.87781818003956,-0.753381513032924,
90.6728123166472));
#235131=CARTESIAN_POINT('Ctrl Pts',(-7.89221335862975,-0.544875492076966,
90.6643700134899));
#235132=CARTESIAN_POINT('Ctrl Pts',(-7.90473949093695,-0.363441549526122,
90.6570238450722));
#235133=CARTESIAN_POINT('Ctrl Pts',(-7.910997733292,-0.181705379616724,
90.6496776766546));
#235134=CARTESIAN_POINT('Ctrl Pts',(-7.91099999938413,-9.87136388252182E-5,
90.6423315082369));
#235135=CARTESIAN_POINT('',(-7.91135449193049,-0.00500362976431777,88.6423315082369));
#235136=CARTESIAN_POINT('Ctrl Pts',(-7.92012792240699,-9.7123266765243E-5,
90.6423314393769));
#235137=CARTESIAN_POINT('Ctrl Pts',(-7.92010724319683,0.0884449210834555,
90.6387539543251));
#235138=CARTESIAN_POINT('Ctrl Pts',(-7.91850031101797,0.17698031386293,
90.6351764692733));
#235139=CARTESIAN_POINT('Ctrl Pts',(-7.82012699933287,2.88639504458979,
90.5256294070049));
#235140=CARTESIAN_POINT('Ctrl Pts',(-4.81214997345493,8.03372540585939,
90.3136902525721));
#235141=CARTESIAN_POINT('Ctrl Pts',(4.17302520961857,8.37571682006808,89.9957815209222));
#235142=CARTESIAN_POINT('Ctrl Pts',(8.41895931796156,2.27239210928254,89.7308575778813));
#235143=CARTESIAN_POINT('Ctrl Pts',(7.62246482467963,-3.11822080623645,
89.518918423448));
#235144=CARTESIAN_POINT('Ctrl Pts',(5.21197134772341,-6.39936160446069,
89.3599640576236));
#235145=CARTESIAN_POINT('Ctrl Pts',(1.51916769345805,-8.09428556441293,
89.2010096917984));
#235146=CARTESIAN_POINT('Ctrl Pts',(-3.93614139152924,-7.78672095142201,
88.9890705373658));
#235147=CARTESIAN_POINT('Ctrl Pts',(-7.51177695944173,-3.99820861181208,
88.8028444761783));
#235148=CARTESIAN_POINT('Ctrl Pts',(-7.91518164929367,-0.685376453820117,
88.6696032035994));
#235149=CARTESIAN_POINT('Ctrl Pts',(-7.91142808499138,-0.00604239087124009,
88.6423315082369));
#235150=CARTESIAN_POINT('',(-7.911,2.36866082303777E-12,86.6423315082369));
#235151=CARTESIAN_POINT('Ctrl Pts',(-7.911,2.76390021980433E-12,88.6423315082369));
#235152=CARTESIAN_POINT('Ctrl Pts',(-7.91099999999923,2.20167589666949,
88.5537440725042));
#235153=CARTESIAN_POINT('Ctrl Pts',(-6.94214576672222,4.38610418338917,
88.4651566367715));
#235154=CARTESIAN_POINT('Ctrl Pts',(-3.67820201488045,7.34180684107751,
88.287981765306));
#235155=CARTESIAN_POINT('Ctrl Pts',(-1.40868175871484,8.0899266657138,88.1993943295733));
#235156=CARTESIAN_POINT('Ctrl Pts',(2.9730927052151,7.65454228025164,88.0222194581079));
#235157=CARTESIAN_POINT('Ctrl Pts',(5.05102072675798,6.47444880834072,87.9336320223751));
#235158=CARTESIAN_POINT('Ctrl Pts',(7.66951518847956,2.93425195367483,87.7564571509097));
#235159=CARTESIAN_POINT('Ctrl Pts',(8.18956872247087,0.601881960096832,
87.6678697151769));
#235160=CARTESIAN_POINT('Ctrl Pts',(7.3230668976124,-3.7153719823265,87.4906948437115));
#235161=CARTESIAN_POINT('Ctrl Pts',(5.94329958850049,-5.66643518936669,
87.4021074079788));
#235162=CARTESIAN_POINT('Ctrl Pts',(2.16154501637644,-7.92205913233052,
87.2249325365133));
#235163=CARTESIAN_POINT('Ctrl Pts',(-0.210816529302415,-8.20894963712996,
87.1363451007806));
#235164=CARTESIAN_POINT('Ctrl Pts',(-4.42123908576601,-6.91982244717725,
86.9591702293152));
#235165=CARTESIAN_POINT('Ctrl Pts',(-6.22631625634311,-5.35390358803376,
86.8705827935824));
#235166=CARTESIAN_POINT('Ctrl Pts',(-7.65317280859549,-2.31334857514328,
86.7354407413121));
#235167=CARTESIAN_POINT('Ctrl Pts',(-7.91100000000035,-1.15702837836302,
86.6888861247745));
#235168=CARTESIAN_POINT('Ctrl Pts',(-7.911,2.36866082303777E-12,86.6423315082369));
#235169=CARTESIAN_POINT('',(-7.911,1.97397653778353E-12,84.6423315082369));
#235170=CARTESIAN_POINT('Ctrl Pts',(-7.911,2.36866082303777E-12,86.6423315082369));
#235171=CARTESIAN_POINT('Ctrl Pts',(-7.91099999999934,2.20167589666909,
86.5537440725042));
#235172=CARTESIAN_POINT('Ctrl Pts',(-6.94214576672244,4.38610418338882,
86.4651566367715));
#235173=CARTESIAN_POINT('Ctrl Pts',(-3.67820201488082,7.34180684107733,
86.2879817653061));
#235174=CARTESIAN_POINT('Ctrl Pts',(-1.40868175871525,8.08992666571373,
86.1993943295733));
#235175=CARTESIAN_POINT('Ctrl Pts',(2.97309270521472,7.65454228025179,86.0222194581079));
#235176=CARTESIAN_POINT('Ctrl Pts',(5.05102072675766,6.47444880834097,85.9336320223751));
#235177=CARTESIAN_POINT('Ctrl Pts',(7.66951518847941,2.93425195367521,85.7564571509097));
#235178=CARTESIAN_POINT('Ctrl Pts',(8.18956872247084,0.601881960097242,
85.667869715177));
#235179=CARTESIAN_POINT('Ctrl Pts',(7.32306689761258,-3.71537198232613,
85.4906948437115));
#235180=CARTESIAN_POINT('Ctrl Pts',(5.94329958850078,-5.66643518936639,
85.4021074079788));
#235181=CARTESIAN_POINT('Ctrl Pts',(2.16154501637684,-7.92205913233041,
85.2249325365134));
#235182=CARTESIAN_POINT('Ctrl Pts',(-0.210816529302006,-8.20894963712997,
85.1363451007806));
#235183=CARTESIAN_POINT('Ctrl Pts',(-4.42123908576567,-6.91982244717747,
84.9591702293152));
#235184=CARTESIAN_POINT('Ctrl Pts',(-6.22631625634284,-5.35390358803407,
84.8705827935825));
#235185=CARTESIAN_POINT('Ctrl Pts',(-7.65317280859537,-2.31334857514366,
84.7354407413121));
#235186=CARTESIAN_POINT('Ctrl Pts',(-7.91100000000029,-1.15702837836341,
84.6888861247746));
#235187=CARTESIAN_POINT('Ctrl Pts',(-7.911,1.97397653778353E-12,84.6423315082369));
#235188=CARTESIAN_POINT('',(-7.911,1.80300219199125E-12,82.642331508237));
#235189=CARTESIAN_POINT('Ctrl Pts',(-7.911,1.97397653778353E-12,84.6423315082369));
#235190=CARTESIAN_POINT('Ctrl Pts',(-7.91099999999945,2.20167589666877,
84.5537440725042));
#235191=CARTESIAN_POINT('Ctrl Pts',(-6.94214576672259,4.38610418338862,
84.4651566367715));
#235192=CARTESIAN_POINT('Ctrl Pts',(-3.67820201488093,7.3418068410773,84.2879817653061));
#235193=CARTESIAN_POINT('Ctrl Pts',(-1.40868175871527,8.08992666571375,
84.1993943295733));
#235194=CARTESIAN_POINT('Ctrl Pts',(2.97309270521485,7.65454228025176,84.0222194581079));
#235195=CARTESIAN_POINT('Ctrl Pts',(5.05102072675784,6.47444880834085,83.9336320223751));
#235196=CARTESIAN_POINT('Ctrl Pts',(7.66951518847956,2.93425195367488,83.7564571509097));
#235197=CARTESIAN_POINT('Ctrl Pts',(8.1895687224709,0.601881960096794,83.667869715177));
#235198=CARTESIAN_POINT('Ctrl Pts',(7.32306689761233,-3.71537198232667,
83.4906948437115));
#235199=CARTESIAN_POINT('Ctrl Pts',(5.94329958850032,-5.6664351893669,83.4021074079788));
#235200=CARTESIAN_POINT('Ctrl Pts',(2.16154501637605,-7.92205913233065,
83.2249325365133));
#235201=CARTESIAN_POINT('Ctrl Pts',(-0.210816529302923,-8.20894963712997,
83.1363451007806));
#235202=CARTESIAN_POINT('Ctrl Pts',(-4.42123908576658,-6.91982244717691,
82.9591702293151));
#235203=CARTESIAN_POINT('Ctrl Pts',(-6.22631625634361,-5.35390358803321,
82.8705827935824));
#235204=CARTESIAN_POINT('Ctrl Pts',(-7.65317280859553,-2.31334857514293,
82.7354407413121));
#235205=CARTESIAN_POINT('Ctrl Pts',(-7.91100000000026,-1.15702837836313,
82.6888861247745));
#235206=CARTESIAN_POINT('Ctrl Pts',(-7.911,1.80300219199125E-12,82.642331508237));
#235207=CARTESIAN_POINT('',(-7.91099999999884,-4.25400661031056E-6,80.6423316794028));
#235208=CARTESIAN_POINT('Ctrl Pts',(-7.911,1.80300219199125E-12,82.642331508237));
#235209=CARTESIAN_POINT('Ctrl Pts',(-7.9109999999995,2.20167589666852,82.5537440725042));
#235210=CARTESIAN_POINT('Ctrl Pts',(-6.94214576672275,4.38610418338832,
82.4651566367715));
#235211=CARTESIAN_POINT('Ctrl Pts',(-3.67820201488135,7.34180684107707,
82.2879817653061));
#235212=CARTESIAN_POINT('Ctrl Pts',(-1.40868175871583,8.08992666571363,
82.1993943295733));
#235213=CARTESIAN_POINT('Ctrl Pts',(2.97309270521417,7.654542280252,82.0222194581079));
#235214=CARTESIAN_POINT('Ctrl Pts',(5.05102072675719,6.47444880834133,81.9336320223752));
#235215=CARTESIAN_POINT('Ctrl Pts',(7.6695151884792,2.93425195367576,81.7564571509097));
#235216=CARTESIAN_POINT('Ctrl Pts',(8.1895687224708,0.601881960097828,81.667869715177));
#235217=CARTESIAN_POINT('Ctrl Pts',(7.32306689761285,-3.71537198232561,
81.4906948437116));
#235218=CARTESIAN_POINT('Ctrl Pts',(5.94329958850118,-5.66643518936597,
81.4021074079788));
#235219=CARTESIAN_POINT('Ctrl Pts',(2.16154501637741,-7.92205913233026,
81.2249325365134));
#235220=CARTESIAN_POINT('Ctrl Pts',(-0.210816529301418,-8.20894963712999,
81.1363451007806));
#235221=CARTESIAN_POINT('Ctrl Pts',(-4.42123908576517,-6.91982244717778,
80.9591702293152));
#235222=CARTESIAN_POINT('Ctrl Pts',(-6.22631625634246,-5.35390358803451,
80.8705827935825));
#235223=CARTESIAN_POINT('Ctrl Pts',(-7.65317220619433,-2.31334985882827,
80.7354407983674));
#235224=CARTESIAN_POINT('Ctrl Pts',(-7.91099936803671,-1.15703121263333,
80.6888862388851));
#235225=CARTESIAN_POINT('Ctrl Pts',(-7.91099999999884,-4.25400661031052E-6,
80.6423316794028));
#235226=CARTESIAN_POINT('',(-7.92502143214218,0.00372523665453262,76.642331508237));
#235227=CARTESIAN_POINT('Ctrl Pts',(-7.91099999985351,-4.81432872164594E-5,
80.6412939480464));
#235228=CARTESIAN_POINT('Ctrl Pts',(-7.91100257635899,0.423328323470568,
80.6236424389112));
#235229=CARTESIAN_POINT('Ctrl Pts',(-7.87701747137843,0.846047094394404,
80.6062432736875));
#235230=CARTESIAN_POINT('Ctrl Pts',(-7.80305174663063,1.30302162523151,
80.5874701706095));
#235231=CARTESIAN_POINT('Ctrl Pts',(-7.79644699090499,1.34197475883232,
80.585870859129));
#235232=CARTESIAN_POINT('Ctrl Pts',(-7.78515772330068,1.40565771452233,
80.5832577175704));
#235233=CARTESIAN_POINT('Ctrl Pts',(-7.78064651787767,1.430417476116,80.5822421092159));
#235234=CARTESIAN_POINT('Ctrl Pts',(-7.77242693172883,1.4743410640839,80.5804410733706));
#235235=CARTESIAN_POINT('Ctrl Pts',(-7.76876563614406,1.49351346675973,
80.5796551494238));
#235236=CARTESIAN_POINT('Ctrl Pts',(-7.76132384667845,1.53171456920015,
80.5780896112955));
#235237=CARTESIAN_POINT('Ctrl Pts',(-7.75754423629362,1.55074330528034,
80.5773099930788));
#235238=CARTESIAN_POINT('Ctrl Pts',(-7.74987263149103,1.58863658699438,
80.5757578771316));
#235239=CARTESIAN_POINT('Ctrl Pts',(-7.7459816604466,1.60750120630538,80.5749853735629));
#235240=CARTESIAN_POINT('Ctrl Pts',(-7.73523236771968,1.65867173192364,
80.5728904426931));
#235241=CARTESIAN_POINT('Ctrl Pts',(-7.72824056966414,1.69094926191849,
80.5715695322991));
#235242=CARTESIAN_POINT('Ctrl Pts',(-7.70089308969035,1.81348487054252,
80.5665566893789));
#235243=CARTESIAN_POINT('Ctrl Pts',(-7.67915652412774,1.90342772299259,
80.5628808929967));
#235244=CARTESIAN_POINT('Ctrl Pts',(-7.60503027982869,2.18817832085411,
80.5512472965636));
#235245=CARTESIAN_POINT('Ctrl Pts',(-7.54676532599002,2.38137467340516,
80.5433614393516));
#235246=CARTESIAN_POINT('Ctrl Pts',(-7.43900827308007,2.69479122276379,
80.5305034948555));
#235247=CARTESIAN_POINT('Ctrl Pts',(-7.39382718649918,2.81639197050389,
80.5254976881248));
#235248=CARTESIAN_POINT('Ctrl Pts',(-7.2247862680274,3.23920193124665,80.5079672303777));
#235249=CARTESIAN_POINT('Ctrl Pts',(-7.08534255681913,3.5338197360161,80.4955359681529));
#235250=CARTESIAN_POINT('Ctrl Pts',(-6.85053571361749,3.95978856190524,
80.4766238781403));
#235251=CARTESIAN_POINT('Ctrl Pts',(-6.76865720522682,4.09817551814219,
80.4703190822393));
#235252=CARTESIAN_POINT('Ctrl Pts',(-6.66474863924903,4.26217805596696,
80.4625754928917));
#235253=CARTESIAN_POINT('Ctrl Pts',(-6.64669745716633,4.29027377824695,
80.4612389976533));
#235254=CARTESIAN_POINT('Ctrl Pts',(-6.62252910084508,4.32737191885125,
80.4594602801798));
#235255=CARTESIAN_POINT('Ctrl Pts',(-6.61657037883429,4.33647735338772,
80.4590225830894));
#235256=CARTESIAN_POINT('Ctrl Pts',(-6.6054303851961,4.35342379663038,80.4582058924342));
#235257=CARTESIAN_POINT('Ctrl Pts',(-6.600253885955,4.36126793112905,80.457827031843));
#235258=CARTESIAN_POINT('Ctrl Pts',(-6.58945431135344,4.37756964857835,
80.4570379642866));
#235259=CARTESIAN_POINT('Ctrl Pts',(-6.58382890329585,4.38602566351143,
80.4566276945091));
#235260=CARTESIAN_POINT('Ctrl Pts',(-6.57093528839604,4.40532642046014,
80.4556890723732));
#235261=CARTESIAN_POINT('Ctrl Pts',(-6.56365649496654,4.41616404243629,
80.4551604415119));
#235262=CARTESIAN_POINT('Ctrl Pts',(-6.54122689357849,4.44938222256679,
80.4535353428928));
#235263=CARTESIAN_POINT('Ctrl Pts',(-6.52598824372088,4.47170312814809,
80.4524366453631));
#235264=CARTESIAN_POINT('Ctrl Pts',(-6.38244623284158,4.67966064377969,
80.4421390890349));
#235265=CARTESIAN_POINT('Ctrl Pts',(-6.24637185614294,4.85980225658652,
80.4327625313605));
#235266=CARTESIAN_POINT('Ctrl Pts',(-6.0262532818032,5.12666157701905,80.4182891288265));
#235267=CARTESIAN_POINT('Ctrl Pts',(-5.94761361306142,5.21768911102217,
80.4132398388784));
#235268=CARTESIAN_POINT('Ctrl Pts',(-5.65471827256188,5.54149401266744,
80.3948989761496));
#235269=CARTESIAN_POINT('Ctrl Pts',(-5.42862294397031,5.76316344153982,
80.3816157447365));
#235270=CARTESIAN_POINT('Ctrl Pts',(-5.06385277380281,6.08022949783928,
80.3615685954509));
#235271=CARTESIAN_POINT('Ctrl Pts',(-4.93440742059983,6.18574332417144,
80.3546908858447));
#235272=CARTESIAN_POINT('Ctrl Pts',(-4.74354907268072,6.33151014012456,
80.3448753352736));
#235273=CARTESIAN_POINT('Ctrl Pts',(-4.68476521366669,6.3751277225059,80.3418944079285));
#235274=CARTESIAN_POINT('Ctrl Pts',(-4.57865220080663,6.45160315123772,
80.3365862683638));
#235275=CARTESIAN_POINT('Ctrl Pts',(-4.53155354618199,6.48477152379194,
80.3342552166449));
#235276=CARTESIAN_POINT('Ctrl Pts',(-4.45977733010866,6.53415476987012,
80.3307392659494));
#235277=CARTESIAN_POINT('Ctrl Pts',(-4.43536451914986,6.55075064256006,
80.3295496881913));
#235278=CARTESIAN_POINT('Ctrl Pts',(-4.39125503082659,6.58037673377982,
80.3274114085475));
#235279=CARTESIAN_POINT('Ctrl Pts',(-4.37159182949589,6.59345611834209,
80.326462123681));
#235280=CARTESIAN_POINT('Ctrl Pts',(-4.32907239210385,6.62146498146732,
80.3244177025369));
#235281=CARTESIAN_POINT('Ctrl Pts',(-4.30619683396836,6.63636460044106,
80.3233229281999));
#235282=CARTESIAN_POINT('Ctrl Pts',(-4.244044172706,6.67639004371176,80.3203620100793));
#235283=CARTESIAN_POINT('Ctrl Pts',(-4.2046212443013,6.70128757598071,80.3184984988389));
#235284=CARTESIAN_POINT('Ctrl Pts',(-4.0066949056698,6.82385366516267,80.309212211609));
#235285=CARTESIAN_POINT('Ctrl Pts',(-3.84499736244249,6.91625471228844,
80.3018465740832));
#235286=CARTESIAN_POINT('Ctrl Pts',(-3.11019412057477,7.3024131202901,80.269161658121));
#235287=CARTESIAN_POINT('Ctrl Pts',(-2.50574480187838,7.53125801775332,
80.2447614219016));
#235288=CARTESIAN_POINT('Ctrl Pts',(-1.64465310842037,7.7419545602089,80.2118252192316));
#235289=CARTESIAN_POINT('Ctrl Pts',(-1.40654390082939,7.78873394545177,
80.2028586642778));
#235290=CARTESIAN_POINT('Ctrl Pts',(-0.967204309309037,7.8542412640535,
80.1862134935696));
#235291=CARTESIAN_POINT('Ctrl Pts',(-0.766684728600054,7.87634304806157,
80.1785770654113));
#235292=CARTESIAN_POINT('Ctrl Pts',(-0.473931471669022,7.89732527160054,
80.1671581433925));
#235293=CARTESIAN_POINT('Ctrl Pts',(-0.382210604030192,7.90229535083546,
80.163541787853));
#235294=CARTESIAN_POINT('Ctrl Pts',(-0.275984242953884,7.90619773009887,
80.1592906049665));
#235295=CARTESIAN_POINT('Ctrl Pts',(-0.261540979114007,7.90668869772354,
80.1587112382315));
#235296=CARTESIAN_POINT('Ctrl Pts',(-0.239616753261383,7.90737382529358,
80.1578296457148));
#235297=CARTESIAN_POINT('Ctrl Pts',(-0.232136685368093,7.90759695231192,
80.1575284875577));
#235298=CARTESIAN_POINT('Ctrl Pts',(-0.218599416794738,7.90798153834219,
80.1569827578653));
#235299=CARTESIAN_POINT('Ctrl Pts',(-0.21254232003349,7.90814665251786,
80.1567383237233));
#235300=CARTESIAN_POINT('Ctrl Pts',(-0.200452568070444,7.90846231473651,
80.1562499262384));
#235301=CARTESIAN_POINT('Ctrl Pts',(-0.194419918685007,7.90861291950778,
80.1560059652401));
#235302=CARTESIAN_POINT('Ctrl Pts',(-0.177491679939836,7.90901615129111,
80.1553206535));
#235303=CARTESIAN_POINT('Ctrl Pts',(-0.166595757152461,7.90925316512054,
80.1548786993345));
#235304=CARTESIAN_POINT('Ctrl Pts',(-0.122185546973423,7.91012738878037,
80.1530737780868));
#235305=CARTESIAN_POINT('Ctrl Pts',(-0.0886681787073125,7.91057409549701,
80.1517032565867));
#235306=CARTESIAN_POINT('Ctrl Pts',(0.431899376155758,7.91420317672486,
80.1302756713965));
#235307=CARTESIAN_POINT('Ctrl Pts',(0.918131024994542,7.87261122472651,
80.1081097101464));
#235308=CARTESIAN_POINT('Ctrl Pts',(1.71809507071396,7.7290528431356,80.0707080044382));
#235309=CARTESIAN_POINT('Ctrl Pts',(2.03498180807262,7.65172974046777,80.0556413150283));
#235310=CARTESIAN_POINT('Ctrl Pts',(2.68233236071016,7.45069759872589,80.0250012436343));
#235311=CARTESIAN_POINT('Ctrl Pts',(3.01114398170241,7.32399138363621,80.0095231287553));
#235312=CARTESIAN_POINT('Ctrl Pts',(3.45681372319178,7.11714605858283,79.9888680857794));
#235313=CARTESIAN_POINT('Ctrl Pts',(3.58161216926669,7.05516731874095,79.983118444383));
#235314=CARTESIAN_POINT('Ctrl Pts',(3.72122728119742,6.98117023537433,79.976721489916));
#235315=CARTESIAN_POINT('Ctrl Pts',(3.73771061874789,6.97235897455571,79.9759668055988));
#235316=CARTESIAN_POINT('Ctrl Pts',(3.76244541255824,6.95902393023984,79.9748351427937));
#235317=CARTESIAN_POINT('Ctrl Pts',(3.77072022316311,6.95454373366976,79.9744566919036));
#235318=CARTESIAN_POINT('Ctrl Pts',(3.78494593744594,6.94680871027184,79.9738063063536));
#235319=CARTESIAN_POINT('Ctrl Pts',(3.79090067570193,6.94356097933376,79.9735341316392));
#235320=CARTESIAN_POINT('Ctrl Pts',(3.80316252834932,6.93685285534439,79.9729738183408));
#235321=CARTESIAN_POINT('Ctrl Pts',(3.80946911460674,6.93339150913244,79.9726857125224));
#235322=CARTESIAN_POINT('Ctrl Pts',(3.82465128253924,6.9250318653289,79.9719923249827));
#235323=CARTESIAN_POINT('Ctrl Pts',(3.83352219802981,6.9201250947534,79.9715873318625));
#235324=CARTESIAN_POINT('Ctrl Pts',(3.86074978334397,6.90499627561509,79.9703447389674));
#235325=CARTESIAN_POINT('Ctrl Pts',(3.8790752457855,6.89471810168413,79.9695090536308));
#235326=CARTESIAN_POINT('Ctrl Pts',(4.09045781241781,6.77505076225895,79.9598764872261));
#235327=CARTESIAN_POINT('Ctrl Pts',(4.27887820668434,6.65765484623747,79.9513616254832));
#235328=CARTESIAN_POINT('Ctrl Pts',(4.48253568863013,6.51854323401972,79.9421648413862));
#235329=CARTESIAN_POINT('Ctrl Pts',(4.50288303615596,6.5045043213996,79.9412460240785));
#235330=CARTESIAN_POINT('Ctrl Pts',(4.82464981636451,6.28026379596321,79.9267145857753));
#235331=CARTESIAN_POINT('Ctrl Pts',(5.11113909994778,6.04939959666413,79.913780307824));
#235332=CARTESIAN_POINT('Ctrl Pts',(5.57536377624048,5.61870627584345,79.891820816936));
#235333=CARTESIAN_POINT('Ctrl Pts',(5.76094534645344,5.42826383098148,79.8827114818377));
#235334=CARTESIAN_POINT('Ctrl Pts',(6.10323751740224,5.03964112773595,79.8646307840982));
#235335=CARTESIAN_POINT('Ctrl Pts',(6.26073855914029,4.84258537352525,79.8556848526237));
#235336=CARTESIAN_POINT('Ctrl Pts',(6.43649506144405,4.59975251369358,79.844551666801));
#235337=CARTESIAN_POINT('Ctrl Pts',(6.46408545864606,4.56089804033258,79.8427670650363));
#235338=CARTESIAN_POINT('Ctrl Pts',(6.5425873724176,4.44820363061286,79.8375755182173));
#235339=CARTESIAN_POINT('Ctrl Pts',(6.59259530718062,4.37374568099061,79.834126561785));
#235340=CARTESIAN_POINT('Ctrl Pts',(6.66678331916852,4.25912156138608,79.8287668203078));
#235341=CARTESIAN_POINT('Ctrl Pts',(6.6918901701621,4.2195642002757,79.8269076790374));
#235342=CARTESIAN_POINT('Ctrl Pts',(6.72231500356361,4.17067346886978,79.8245988157248));
#235343=CARTESIAN_POINT('Ctrl Pts',(6.72796707284153,4.16154962197275,79.8241674932859));
#235344=CARTESIAN_POINT('Ctrl Pts',(6.73674887488235,4.14730895566075,79.8234936132373));
#235345=CARTESIAN_POINT('Ctrl Pts',(6.73989139932079,4.14220000748476,79.8232517207053));
#235346=CARTESIAN_POINT('Ctrl Pts',(6.74542980994529,4.13317296648359,79.8228240912561));
#235347=CARTESIAN_POINT('Ctrl Pts',(6.74782810292229,4.12925634770371,79.822638477466));
#235348=CARTESIAN_POINT('Ctrl Pts',(6.75290514234691,4.12094887056766,79.8222446187083));
#235349=CARTESIAN_POINT('Ctrl Pts',(6.75558301909624,4.11655748499725,79.8220363300023));
#235350=CARTESIAN_POINT('Ctrl Pts',(6.76317037186138,4.10408782590624,79.8214446237769));
#235351=CARTESIAN_POINT('Ctrl Pts',(6.76806964329129,4.09600337695679,79.8210606994604));
#235352=CARTESIAN_POINT('Ctrl Pts',(6.78866293344535,4.06188388592323,79.8194391755199));
#235353=CARTESIAN_POINT('Ctrl Pts',(6.80422117769425,4.03576749292719,79.8181950205303));
#235354=CARTESIAN_POINT('Ctrl Pts',(7.1577974729009,3.43439040158215,79.7894893387484));
#235355=CARTESIAN_POINT('Ctrl Pts',(7.42184596227242,2.81874919018932,79.7592267335175));
#235356=CARTESIAN_POINT('Ctrl Pts',(7.7155513250587,1.79279676379647,79.7128722242424));
#235357=CARTESIAN_POINT('Ctrl Pts',(7.79630955076411,1.40051685731983,79.6959556403277));
#235358=CARTESIAN_POINT('Ctrl Pts',(7.85288679114162,0.958227425595022,
79.6777616786957));
#235359=CARTESIAN_POINT('Ctrl Pts',(7.85831801615514,0.912616439820966,
79.6758950882937));
#235360=CARTESIAN_POINT('Ctrl Pts',(7.86721243164276,0.831943879952323,
79.6726098102521));
#235361=CARTESIAN_POINT('Ctrl Pts',(7.87083919714595,0.796901763602491,
79.6711881468534));
#235362=CARTESIAN_POINT('Ctrl Pts',(7.87582995958644,0.745317959853305,
79.6691029065887));
#235363=CARTESIAN_POINT('Ctrl Pts',(7.87737615106156,0.728794477709592,
79.6684360894341));
#235364=CARTESIAN_POINT('Ctrl Pts',(7.87995923823529,0.700221159929094,
79.6672848994107));
#235365=CARTESIAN_POINT('Ctrl Pts',(7.8810205151654,0.688173604213696,79.666800101242));
#235366=CARTESIAN_POINT('Ctrl Pts',(7.88308006429568,0.664163975256677,
79.6658350872083));
#235367=CARTESIAN_POINT('Ctrl Pts',(7.88407874628551,0.652201969783695,
79.6653548655072));
#235368=CARTESIAN_POINT('Ctrl Pts',(7.88637958287595,0.623865288765077,
79.6642185808774));
#235369=CARTESIAN_POINT('Ctrl Pts',(7.88765797153187,0.607488724261065,
79.6635629240978));
#235370=CARTESIAN_POINT('Ctrl Pts',(7.8913172211549,0.558652660618702,79.6616106933338));
#235371=CARTESIAN_POINT('Ctrl Pts',(7.89354879507739,0.526182206988769,
79.6603165896497));
#235372=CARTESIAN_POINT('Ctrl Pts',(7.91035217541734,0.257450696571845,
79.6496370096787));
#235373=CARTESIAN_POINT('Ctrl Pts',(7.914514015212,0.0206532130825134,79.6404289131966));
#235374=CARTESIAN_POINT('Ctrl Pts',(7.90442008748098,-0.34893111664469,
79.6262990780623));
#235375=CARTESIAN_POINT('Ctrl Pts',(7.89743684061129,-0.481769775350074,
79.6212683118086));
#235376=CARTESIAN_POINT('Ctrl Pts',(7.85275791172879,-1.05534427903552,
79.5996837703251));
#235377=CARTESIAN_POINT('Ctrl Pts',(7.78148690974655,-1.49265501324453,
79.5836255446691));
#235378=CARTESIAN_POINT('Ctrl Pts',(7.60879453376141,-2.18227279752326,
79.5573263957851));
#235379=CARTESIAN_POINT('Ctrl Pts',(7.530320658477,-2.43932957341266,79.5472816890605));
#235380=CARTESIAN_POINT('Ctrl Pts',(7.40486466137258,-2.78602270606196,
79.5329561659184));
#235381=CARTESIAN_POINT('Ctrl Pts',(7.36901680874553,-2.87950229486924,
79.5290128007756));
#235382=CARTESIAN_POINT('Ctrl Pts',(7.32600733100514,-2.98558939354802,
79.524423554775));
#235383=CARTESIAN_POINT('Ctrl Pts',(7.3205728097602,-2.99888999038699,79.5238461099371));
#235384=CARTESIAN_POINT('Ctrl Pts',(7.31232034250548,-3.01893119898145,
79.5229728099676));
#235385=CARTESIAN_POINT('Ctrl Pts',(7.30952922738296,-3.02568287320149,
79.5226780531907));
#235386=CARTESIAN_POINT('Ctrl Pts',(7.30469928457368,-3.03732075913274,
79.5221690161413));
#235387=CARTESIAN_POINT('Ctrl Pts',(7.30266489409153,-3.04220881537479,
79.5219549206508));
#235388=CARTESIAN_POINT('Ctrl Pts',(7.29845227240776,-3.05230196165035,
79.5215122311074));
#235389=CARTESIAN_POINT('Ctrl Pts',(7.2962733764268,-3.05750677087776,79.521283609091));
#235390=CARTESIAN_POINT('Ctrl Pts',(7.29099426339513,-3.07007940409096,
79.5207305314863));
#235391=CARTESIAN_POINT('Ctrl Pts',(7.28788844837573,-3.07744485891418,
79.5204058371182));
#235392=CARTESIAN_POINT('Ctrl Pts',(7.27636477087859,-3.10465803496324,
79.519203622789));
#235393=CARTESIAN_POINT('Ctrl Pts',(7.26787699818645,-3.12447591116916,
79.5183230660393));
#235394=CARTESIAN_POINT('Ctrl Pts',(7.14598847550664,-3.4058860801337,79.5057446697801));
#235395=CARTESIAN_POINT('Ctrl Pts',(7.01863244436319,-3.66114058369329,
79.4933052538471));
#235396=CARTESIAN_POINT('Ctrl Pts',(6.6638642419253,-4.28535949515461,79.4609930872312));
#235397=CARTESIAN_POINT('Ctrl Pts',(6.41938218852172,-4.64359018436774,
79.4407712517041));
#235398=CARTESIAN_POINT('Ctrl Pts',(5.93785470884569,-5.23793751246095,
79.4059340337106));
#235399=CARTESIAN_POINT('Ctrl Pts',(5.71285582396468,-5.48246441320965,
79.3911363733515));
#235400=CARTESIAN_POINT('Ctrl Pts',(5.39597936913816,-5.78608228231994,
79.3723863000397));
#235401=CARTESIAN_POINT('Ctrl Pts',(5.31732396739807,-5.85844762209079,
79.3678840072062));
#235402=CARTESIAN_POINT('Ctrl Pts',(5.16785720904836,-5.99047067243447,
79.359608960847));
#235403=CARTESIAN_POINT('Ctrl Pts',(5.0974186777621,-6.05052151638252,79.3558198943539));
#235404=CARTESIAN_POINT('Ctrl Pts',(5.01367545102962,-6.11941432893087,
79.3514419098783));
#235405=CARTESIAN_POINT('Ctrl Pts',(5.00137958796215,-6.12946779732583,
79.3508022347687));
#235406=CARTESIAN_POINT('Ctrl Pts',(4.98254204400987,-6.14477551880341,
79.3498270059289));
#235407=CARTESIAN_POINT('Ctrl Pts',(4.97602217775554,-6.15005647810439,
79.3494903377724));
#235408=CARTESIAN_POINT('Ctrl Pts',(4.96465938491203,-6.15923021155808,
79.3489051013172));
#235409=CARTESIAN_POINT('Ctrl Pts',(4.95982025685341,-6.16312766597506,
79.3486563381076));
#235410=CARTESIAN_POINT('Ctrl Pts',(4.94971464922073,-6.17124715535377,
79.3481378303156));
#235411=CARTESIAN_POINT('Ctrl Pts',(4.94444734628547,-6.17546816049518,
79.3478681286437));
#235412=CARTESIAN_POINT('Ctrl Pts',(4.9299235427613,-6.18707645960809,79.3471259994543));
#235413=CARTESIAN_POINT('Ctrl Pts',(4.92065582837977,-6.19444973139401,
79.3466541544731));
#235414=CARTESIAN_POINT('Ctrl Pts',(4.88461966789591,-6.22298772222383,
79.3448260664416));
#235415=CARTESIAN_POINT('Ctrl Pts',(4.85773075959416,-6.24400011183762,
79.343476133452));
#235416=CARTESIAN_POINT('Ctrl Pts',(4.44257708384931,-6.56411781486267,
79.3228475060404));
#235417=CARTESIAN_POINT('Ctrl Pts',(4.02746558814835,-6.82669241445261,
79.3051735298626));
#235418=CARTESIAN_POINT('Ctrl Pts',(3.12409367736634,-7.28684725121567,
79.2703020286636));
#235419=CARTESIAN_POINT('Ctrl Pts',(2.63509451321552,-7.4775892494324,79.2532958375807));
#235420=CARTESIAN_POINT('Ctrl Pts',(1.95333413901935,-7.66827145460961,
79.2285687687574));
#235421=CARTESIAN_POINT('Ctrl Pts',(1.77413567222701,-7.7117013662272,79.221968771558));
#235422=CARTESIAN_POINT('Ctrl Pts',(1.46953484973944,-7.77434432124202,
79.2103517689428));
#235423=CARTESIAN_POINT('Ctrl Pts',(1.34488785193147,-7.7968734734457,79.2054870339007));
#235424=CARTESIAN_POINT('Ctrl Pts',(1.19883743826907,-7.81966483963672,
79.1996049120491));
#235425=CARTESIAN_POINT('Ctrl Pts',(1.17790219098917,-7.82284576220844,
79.1987574087489));
#235426=CARTESIAN_POINT('Ctrl Pts',(1.15053644910662,-7.82689139904885,
79.1976436343297));
#235427=CARTESIAN_POINT('Ctrl Pts',(1.14411713083316,-7.82783233620028,
79.1973819433387));
#235428=CARTESIAN_POINT('Ctrl Pts',(1.13367661474274,-7.82934957933406,
79.1969556187056));
#235429=CARTESIAN_POINT('Ctrl Pts',(1.12965610628783,-7.82993068830342,
79.1967912766765));
#235430=CARTESIAN_POINT('Ctrl Pts',(1.12193501216123,-7.8310405951247,79.1964753406692));
#235431=CARTESIAN_POINT('Ctrl Pts',(1.11823449465726,-7.83156986745732,
79.1963237757331));
#235432=CARTESIAN_POINT('Ctrl Pts',(1.1097815650264,-7.83277274770226,79.1959772285256));
#235433=CARTESIAN_POINT('Ctrl Pts',(1.10502894572362,-7.83344464895138,
79.1957821423553));
#235434=CARTESIAN_POINT('Ctrl Pts',(1.08994656561594,-7.83556292039606,
79.195162270552));
#235435=CARTESIAN_POINT('Ctrl Pts',(1.07961462924598,-7.8369931763136,79.1947364975708));
#235436=CARTESIAN_POINT('Ctrl Pts',(0.991580744751443,-7.84900236585298,
79.1910991662262));
#235437=CARTESIAN_POINT('Ctrl Pts',(0.913730813428599,-7.85844550016604,
79.1878195622358));
#235438=CARTESIAN_POINT('Ctrl Pts',(0.481019336274078,-7.90441647989722,
79.1692962945861));
#235439=CARTESIAN_POINT('Ctrl Pts',(0.124164678765431,-7.9180631132183,
79.1529414613027));
#235440=CARTESIAN_POINT('Ctrl Pts',(-0.767699417545959,-7.89185622959243,
79.1114295054131));
#235441=CARTESIAN_POINT('Ctrl Pts',(-1.3001184343718,-7.82179971853014,
79.0861683142335));
#235442=CARTESIAN_POINT('Ctrl Pts',(-2.13250282279253,-7.62486456022967,
79.0483503196822));
#235443=CARTESIAN_POINT('Ctrl Pts',(-2.43888402928554,-7.53246351013656,
79.034780303191));
#235444=CARTESIAN_POINT('Ctrl Pts',(-2.75705437964557,-7.41504876749888,
79.0210884355062));
#235445=CARTESIAN_POINT('Ctrl Pts',(-2.77522312111499,-7.40826792929645,
79.0203079235865));
#235446=CARTESIAN_POINT('Ctrl Pts',(-2.80167151291123,-7.39828605320154,
79.0191736570398));
#235447=CARTESIAN_POINT('Ctrl Pts',(-2.80997092654295,-7.39513780696166,
79.0188180060387));
#235448=CARTESIAN_POINT('Ctrl Pts',(-2.82451322249321,-7.3895934103642,
79.0181953149664));
#235449=CARTESIAN_POINT('Ctrl Pts',(-2.83075838963008,-7.38720330398279,
79.0179280577578));
#235450=CARTESIAN_POINT('Ctrl Pts',(-2.84286757000561,-7.38255135313997,
79.0174101562369));
#235451=CARTESIAN_POINT('Ctrl Pts',(-2.84873193109052,-7.38029043380816,
79.0171594789088));
#235452=CARTESIAN_POINT('Ctrl Pts',(-2.86270705814136,-7.37488338766276,
79.0165624253177));
#235453=CARTESIAN_POINT('Ctrl Pts',(-2.8708153500614,-7.37173086248394,
79.0162162799106));
#235454=CARTESIAN_POINT('Ctrl Pts',(-2.89969454680459,-7.36044768148992,
79.0149843427614));
#235455=CARTESIAN_POINT('Ctrl Pts',(-2.92043634053296,-7.35224252379918,
79.0141012398959));
#235456=CARTESIAN_POINT('Ctrl Pts',(-3.20672902961346,-7.2375865348228,
79.0019350136791));
#235457=CARTESIAN_POINT('Ctrl Pts',(-3.46636045451847,-7.11689080592085,
78.991187772922));
#235458=CARTESIAN_POINT('Ctrl Pts',(-4.27564698419196,-6.68585520810151,
78.958048068381));
#235459=CARTESIAN_POINT('Ctrl Pts',(-4.79488337505931,-6.32383238140299,
78.9375323694199));
#235460=CARTESIAN_POINT('Ctrl Pts',(-5.46526740481459,-5.72593604239941,
78.9061854508312));
#235461=CARTESIAN_POINT('Ctrl Pts',(-5.65574917677674,-5.53786716356691,
78.896564437832));
#235462=CARTESIAN_POINT('Ctrl Pts',(-5.88727373553365,-5.28484861679749,
78.8833381906605));
#235463=CARTESIAN_POINT('Ctrl Pts',(-5.93742176319132,-5.22844518350846,
78.8803727788504));
#235464=CARTESIAN_POINT('Ctrl Pts',(-5.99299078540164,-5.16411400801576,
78.8769598301381));
#235465=CARTESIAN_POINT('Ctrl Pts',(-5.99921485851653,-5.15688211226937,
78.8765757217058));
#235466=CARTESIAN_POINT('Ctrl Pts',(-6.00859111333249,-5.14594767539056,
78.8759943171108));
#235467=CARTESIAN_POINT('Ctrl Pts',(-6.01175300872925,-5.14225343666563,
78.8757977775455));
#235468=CARTESIAN_POINT('Ctrl Pts',(-6.01720492091928,-5.13587172799162,
78.8754580741461));
#235469=CARTESIAN_POINT('Ctrl Pts',(-6.01949655169882,-5.13318563182078,
78.8753150343466));
#235470=CARTESIAN_POINT('Ctrl Pts',(-6.02423033276859,-5.12762948145548,
78.8750190429693));
#235471=CARTESIAN_POINT('Ctrl Pts',(-6.02667223140632,-5.12475921545978,
78.8748660723277));
#235472=CARTESIAN_POINT('Ctrl Pts',(-6.03328149009823,-5.11697927815517,
78.874451271254));
#235473=CARTESIAN_POINT('Ctrl Pts',(-6.03744489983618,-5.11206627038428,
78.8741891426256));
#235474=CARTESIAN_POINT('Ctrl Pts',(-6.05291506732474,-5.09376552880462,
78.873212062682));
#235475=CARTESIAN_POINT('Ctrl Pts',(-6.06418325770431,-5.08034540977162,
78.8724942438912));
#235476=CARTESIAN_POINT('Ctrl Pts',(-6.25581268021518,-4.85057386957689,
78.8601834129765));
#235477=CARTESIAN_POINT('Ctrl Pts',(-6.42452196940388,-4.62479710659329,
78.8477772305291));
#235478=CARTESIAN_POINT('Ctrl Pts',(-6.91605885169952,-3.88804887516201,
78.8075644717317));
#235479=CARTESIAN_POINT('Ctrl Pts',(-7.19265416543083,-3.34881960892385,
78.7786731520798));
#235480=CARTESIAN_POINT('Ctrl Pts',(-7.51847192423664,-2.48196618427648,
78.7367703242711));
#235481=CARTESIAN_POINT('Ctrl Pts',(-7.61325003217029,-2.17394363535585,
78.7226463554586));
#235482=CARTESIAN_POINT('Ctrl Pts',(-7.7197734472994,-1.73382083693689,
78.7036368541788));
#235483=CARTESIAN_POINT('Ctrl Pts',(-7.74739104815025,-1.60591746136991,
78.6982454112363));
#235484=CARTESIAN_POINT('Ctrl Pts',(-7.77516574206615,-1.45980778080906,
78.6922314416077));
#235485=CARTESIAN_POINT('Ctrl Pts',(-7.7784472043781,-1.44222056831505,
78.6915099033989));
#235486=CARTESIAN_POINT('Ctrl Pts',(-7.78329611464803,-1.41573452026112,
78.6904268021478));
#235487=CARTESIAN_POINT('Ctrl Pts',(-7.78490801280894,-1.40684394051464,
78.690063833907));
#235488=CARTESIAN_POINT('Ctrl Pts',(-7.78765758572965,-1.39152897701073,
78.6894396050717));
#235489=CARTESIAN_POINT('Ctrl Pts',(-7.78880254938341,-1.38510592136462,
78.6891781145601));
#235490=CARTESIAN_POINT('Ctrl Pts',(-7.79114732821199,-1.37185725872576,
78.6886393808551));
#235491=CARTESIAN_POINT('Ctrl Pts',(-7.79234612276966,-1.36503147636626,
78.6883621700734));
#235492=CARTESIAN_POINT('Ctrl Pts',(-7.79521555091207,-1.34856635811974,
78.6876943186785));
#235493=CARTESIAN_POINT('Ctrl Pts',(-7.79687727840027,-1.33892546988532,
78.687303958776));
#235494=CARTESIAN_POINT('Ctrl Pts',(-7.80291825239022,-1.3034847726411,
78.6858714832853));
#235495=CARTESIAN_POINT('Ctrl Pts',(-7.8071873819504,-1.27766623398238,
78.6848328300586));
#235496=CARTESIAN_POINT('Ctrl Pts',(-7.87778852099861,-0.837119134097701,
78.6671922038647));
#235497=CARTESIAN_POINT('Ctrl Pts',(-7.911121397185,-0.417763042855495,
78.6516890751607));
#235498=CARTESIAN_POINT('Ctrl Pts',(-7.9107657971752,0.80931778776061,78.6081113855084));
#235499=CARTESIAN_POINT('Ctrl Pts',(-7.78704841551942,1.6115456588928,78.5820400313291));
#235500=CARTESIAN_POINT('Ctrl Pts',(-7.53082472263949,2.42333607253993,
78.5484743041727));
#235501=CARTESIAN_POINT('Ctrl Pts',(-7.51715341849031,2.46541743113994,
78.5467151783887));
#235502=CARTESIAN_POINT('Ctrl Pts',(-7.499029366238,2.51965214900101,78.5444248247676));
#235503=CARTESIAN_POINT('Ctrl Pts',(-7.49489865287078,2.53191282799997,
78.5439055131511));
#235504=CARTESIAN_POINT('Ctrl Pts',(-7.48828552227743,2.5513837591298,78.5430784072745));
#235505=CARTESIAN_POINT('Ctrl Pts',(-7.48582271498667,2.55860067787781,
78.5427713151707));
#235506=CARTESIAN_POINT('Ctrl Pts',(-7.48119017256368,2.57211176395077,
78.5421954243522));
#235507=CARTESIAN_POINT('Ctrl Pts',(-7.47902291793581,2.5784067788096,78.5419267128522));
#235508=CARTESIAN_POINT('Ctrl Pts',(-7.47412353219476,2.59257940028668,
78.5413208529498));
#235509=CARTESIAN_POINT('Ctrl Pts',(-7.4713868901299,2.60045543294256,78.5409835491894));
#235510=CARTESIAN_POINT('Ctrl Pts',(-7.46328682472605,2.62364901726336,
78.5399884594607));
#235511=CARTESIAN_POINT('Ctrl Pts',(-7.45788872603031,2.63895436488957,
78.5393295047075));
#235512=CARTESIAN_POINT('Ctrl Pts',(-7.41555206744036,2.75782500631194,
78.5341942217659));
#235513=CARTESIAN_POINT('Ctrl Pts',(-7.37650576635252,2.86062455612321,
78.5296503343627));
#235514=CARTESIAN_POINT('Ctrl Pts',(-7.22611765951461,3.23298532077706,
78.5128748958965));
#235515=CARTESIAN_POINT('Ctrl Pts',(-7.10203775847234,3.49714497454862,
78.5003688941416));
#235516=CARTESIAN_POINT('Ctrl Pts',(-6.8402469213909,3.98278658660264,78.4766408397171));
#235517=CARTESIAN_POINT('Ctrl Pts',(-6.70561605141231,4.20550622628523,
78.4654390629343));
#235518=CARTESIAN_POINT('Ctrl Pts',(-6.29207492979483,4.81912761399631,
78.4338346590945));
#235519=CARTESIAN_POINT('Ctrl Pts',(-5.98823420232389,5.19184709871647,
78.4137858705275));
#235520=CARTESIAN_POINT('Ctrl Pts',(-5.46609483454463,5.72509420642991,
78.3830335675215));
#235521=CARTESIAN_POINT('Ctrl Pts',(-5.27020516023182,5.90591560128893,
78.3721171287573));
#235522=CARTESIAN_POINT('Ctrl Pts',(-5.0347744450086,6.10217781708426,78.3597096312445));
#235523=CARTESIAN_POINT('Ctrl Pts',(-5.00378990464858,6.12761082591003,
78.3580900394602));
#235524=CARTESIAN_POINT('Ctrl Pts',(-4.95292916997448,6.16871576432185,
78.3554530592206));
#235525=CARTESIAN_POINT('Ctrl Pts',(-4.93316876673269,6.18452968850247,
78.3544337749786));
#235526=CARTESIAN_POINT('Ctrl Pts',(-4.89766319142676,6.21266577136493,
78.3526116238218));
#235527=CARTESIAN_POINT('Ctrl Pts',(-4.88194656594312,6.22502357049801,
78.3518082751982));
#235528=CARTESIAN_POINT('Ctrl Pts',(-4.84851235110195,6.25110800612759,
78.3501061071544));
#235529=CARTESIAN_POINT('Ctrl Pts',(-4.83078292597097,6.26481920321393,
78.3492075066009));
#235530=CARTESIAN_POINT('Ctrl Pts',(-4.78314784508848,6.30133573965823,
78.3468038436816));
#235531=CARTESIAN_POINT('Ctrl Pts',(-4.75313737576229,6.32400351967549,
78.3453007116829));
#235532=CARTESIAN_POINT('Ctrl Pts',(-4.60424474404896,6.43480785322636,
78.3378974764269));
#235533=CARTESIAN_POINT('Ctrl Pts',(-4.48306613196376,6.5198114146002,78.3320424486548));
#235534=CARTESIAN_POINT('Ctrl Pts',(-4.13228734119325,6.75146734349418,
78.3155318469041));
#235535=CARTESIAN_POINT('Ctrl Pts',(-3.89739906897396,6.8897310964753,78.3049938746325));
#235536=CARTESIAN_POINT('Ctrl Pts',(-3.23618606759972,7.23429034581969,
78.2762950372691));
#235537=CARTESIAN_POINT('Ctrl Pts',(-2.79776825957793,7.41487130966066,
78.2583349141204));
#235538=CARTESIAN_POINT('Ctrl Pts',(-2.30838193095897,7.56682459580615,
78.2379294587511));
#235539=CARTESIAN_POINT('Ctrl Pts',(-2.27081093874057,7.57818442915298,
78.2363603435014));
#235540=CARTESIAN_POINT('Ctrl Pts',(-2.22027471909584,7.59305482003728,
78.2342450520417));
#235541=CARTESIAN_POINT('Ctrl Pts',(-2.20738264520811,7.59681269896384,
78.2337050130071));
#235542=CARTESIAN_POINT('Ctrl Pts',(-2.18521852349263,7.60321208123391,
78.232775891817));
#235543=CARTESIAN_POINT('Ctrl Pts',(-2.17595107506911,7.60586950097858,
78.2323871958483));
#235544=CARTESIAN_POINT('Ctrl Pts',(-2.15685052196758,7.61130877408096,
78.2315856766973));
#235545=CARTESIAN_POINT('Ctrl Pts',(-2.14701683936376,7.61408852846327,
78.2311728051457));
#235546=CARTESIAN_POINT('Ctrl Pts',(-2.12417473523376,7.62049769278045,
78.2302132836744));
#235547=CARTESIAN_POINT('Ctrl Pts',(-2.1111623622684,7.62411285790008,78.2296663117233));
#235548=CARTESIAN_POINT('Ctrl Pts',(-2.06981910273436,7.6354850987078,78.2279273727684));
#235549=CARTESIAN_POINT('Ctrl Pts',(-2.04145433828004,7.64311768715359,
78.2267327072821));
#235550=CARTESIAN_POINT('Ctrl Pts',(-1.73442159322066,7.72390510879834,
78.213786200451));
#235551=CARTESIAN_POINT('Ctrl Pts',(-1.45200411177264,7.78194096436413,
78.2017515388553));
#235552=CARTESIAN_POINT('Ctrl Pts',(-0.605069694275399,7.90826592748787,
78.1658190384286));
#235553=CARTESIAN_POINT('Ctrl Pts',(-0.0356587227971045,7.93130212082995,
78.1419641412425));
#235554=CARTESIAN_POINT('Ctrl Pts',(0.616461942412507,7.88740643699264,
78.1153283554771));
#235555=CARTESIAN_POINT('Ctrl Pts',(0.701521487471995,7.88029653188009,
78.1118647858669));
#235556=CARTESIAN_POINT('Ctrl Pts',(0.818403494797568,7.86861918915918,
78.1071174435052));
#235557=CARTESIAN_POINT('Ctrl Pts',(0.850337445200649,7.86523225747011,
78.1058216273433));
#235558=CARTESIAN_POINT('Ctrl Pts',(0.905114269513804,7.8590850942827,78.1036007797293));
#235559=CARTESIAN_POINT('Ctrl Pts',(0.927967309322415,7.85641947942028,
78.1026748004428));
#235560=CARTESIAN_POINT('Ctrl Pts',(0.975057181542259,7.85071850932886,
78.1007678267073));
#235561=CARTESIAN_POINT('Ctrl Pts',(0.99929224543791,7.84767052268173,78.0997869689415));
#235562=CARTESIAN_POINT('Ctrl Pts',(1.05578587534189,7.84029951371488,78.0975017076958));
#235563=CARTESIAN_POINT('Ctrl Pts',(1.08803268423936,7.83588955813799,78.0961981751708));
#235564=CARTESIAN_POINT('Ctrl Pts',(1.19297609672135,7.82087758083035,78.0919583618356));
#235565=CARTESIAN_POINT('Ctrl Pts',(1.26555265697937,7.80946186874416,78.0890299493468));
#235566=CARTESIAN_POINT('Ctrl Pts',(1.96005892667254,7.69028561773148,78.0610211727918));
#235567=CARTESIAN_POINT('Ctrl Pts',(2.56719061568457,7.50945698518855,78.0365610937451));
#235568=CARTESIAN_POINT('Ctrl Pts',(3.75430902966473,6.99486333160442,77.9880309348258));
#235569=CARTESIAN_POINT('Ctrl Pts',(4.3266598225274,6.65603450387533,77.9643123682345));
#235570=CARTESIAN_POINT('Ctrl Pts',(4.85716263129601,6.24435535651387,77.937716232328));
#235571=CARTESIAN_POINT('Ctrl Pts',(4.86429161791076,6.23880354719328,77.9373578472209));
#235572=CARTESIAN_POINT('Ctrl Pts',(4.89394142995364,6.21563157999836,77.935863148741));
#235573=CARTESIAN_POINT('Ctrl Pts',(4.91637599876954,6.19790171527143,77.9347221742175));
#235574=CARTESIAN_POINT('Ctrl Pts',(4.94652685155057,6.17380702120838,77.9331745442123));
#235575=CARTESIAN_POINT('Ctrl Pts',(4.95432805678311,6.16754850267817,77.9327728171101));
#235576=CARTESIAN_POINT('Ctrl Pts',(4.96714959248495,6.15722239932323,77.9321103966097));
#235577=CARTESIAN_POINT('Ctrl Pts',(4.97217685776037,6.15316341760033,77.9318501137829));
#235578=CARTESIAN_POINT('Ctrl Pts',(4.98173259231435,6.14542882115636,77.9313543130794));
#235579=CARTESIAN_POINT('Ctrl Pts',(4.98626198224929,6.14175434720168,77.9311188506904));
#235580=CARTESIAN_POINT('Ctrl Pts',(4.99687068215286,6.13312855396817,77.9305662767521));
#235581=CARTESIAN_POINT('Ctrl Pts',(5.00294669666433,6.12817320442411,77.9302489660994));
#235582=CARTESIAN_POINT('Ctrl Pts',(5.02155863991474,6.11294793426166,77.9292744052347));
#235583=CARTESIAN_POINT('Ctrl Pts',(5.03407033909408,6.10264855918488,77.9286156674493));
#235584=CARTESIAN_POINT('Ctrl Pts',(5.18986049198327,5.97360018148361,77.9203671823294));
#235585=CARTESIAN_POINT('Ctrl Pts',(5.32891286915862,5.84989086019136,77.9124805312862));
#235586=CARTESIAN_POINT('Ctrl Pts',(5.54037521264345,5.64796173067632,77.8997081696442));
#235587=CARTESIAN_POINT('Ctrl Pts',(5.61579207381601,5.57298012158283,77.8949908963749));
#235588=CARTESIAN_POINT('Ctrl Pts',(6.3783837759318,4.78358785604404,77.8457688143051));
#235589=CARTESIAN_POINT('Ctrl Pts',(6.92722129838556,3.94727381964114,77.7985246399713));
#235590=CARTESIAN_POINT('Ctrl Pts',(7.32769944034608,2.98187889484434,77.7556581509835));
#235591=CARTESIAN_POINT('Ctrl Pts',(7.34768933672887,2.93227597320367,77.7534809687233));
#235592=CARTESIAN_POINT('Ctrl Pts',(7.37252596337561,2.86879723817412,77.7507264683992));
#235593=CARTESIAN_POINT('Ctrl Pts',(7.37783886699982,2.85510601026992,77.7501342403285));
#235594=CARTESIAN_POINT('Ctrl Pts',(7.38621557058701,2.833339925244,77.7491956752947));
#235595=CARTESIAN_POINT('Ctrl Pts',(7.38930431330969,2.82527473939298,77.748848541775));
#235596=CARTESIAN_POINT('Ctrl Pts',(7.39503798290656,2.8102295186254,77.74820217218));
#235597=CARTESIAN_POINT('Ctrl Pts',(7.39768624846209,2.80325077110061,77.747902829809));
#235598=CARTESIAN_POINT('Ctrl Pts',(7.40354210686122,2.7877532404858,77.7472391429869));
#235599=CARTESIAN_POINT('Ctrl Pts',(7.40674488397886,2.77923264269852,77.7468749523237));
#235600=CARTESIAN_POINT('Ctrl Pts',(7.41596365377168,2.75457811302087,77.7458231936916));
#235601=CARTESIAN_POINT('Ctrl Pts',(7.42194170262774,2.73842999950355,77.7451368339324));
#235602=CARTESIAN_POINT('Ctrl Pts',(7.46232174785929,2.62825046578179,77.7404707599168));
#235603=CARTESIAN_POINT('Ctrl Pts',(7.49498925943941,2.53359097958229,77.7365463514109));
#235604=CARTESIAN_POINT('Ctrl Pts',(7.57260763905175,2.29402402573444,77.726812988313));
#235605=CARTESIAN_POINT('Ctrl Pts',(7.61520423068091,2.14839472556766,77.7210768150218));
#235606=CARTESIAN_POINT('Ctrl Pts',(7.75536601047227,1.61246018307754,77.7005290190709));
#235607=CARTESIAN_POINT('Ctrl Pts',(7.8273168071756,1.21608559964228,77.686436597197));
#235608=CARTESIAN_POINT('Ctrl Pts',(7.90472703122433,0.469559889352466,
77.6604627762765));
#235609=CARTESIAN_POINT('Ctrl Pts',(7.91773313791556,0.121186773139081,
77.6485554836024));
#235610=CARTESIAN_POINT('Ctrl Pts',(7.90243346081503,-0.412028849165187,
77.6295378106966));
#235611=CARTESIAN_POINT('Ctrl Pts',(7.89062212084517,-0.596908325641212,
77.6227942936502));
#235612=CARTESIAN_POINT('Ctrl Pts',(7.85929075439808,-0.91264384301077,
77.6108087508214));
#235613=CARTESIAN_POINT('Ctrl Pts',(7.84295670697803,-1.04374330969894,
77.6056902902278));
#235614=CARTESIAN_POINT('Ctrl Pts',(7.82123619263469,-1.18843918424695,
77.5998393713379));
#235615=CARTESIAN_POINT('Ctrl Pts',(7.8190869927813,-1.20249817920185,77.5992688801238));
#235616=CARTESIAN_POINT('Ctrl Pts',(7.81597399459382,-1.22250062100783,
77.5984544373));
#235617=CARTESIAN_POINT('Ctrl Pts',(7.81504129596696,-1.2284489385268,77.5982118889174));
#235618=CARTESIAN_POINT('Ctrl Pts',(7.81329442963293,-1.2395071317363,77.5977603373753));
#235619=CARTESIAN_POINT('Ctrl Pts',(7.81248203709536,-1.24461728801893,
77.5975514131976));
#235620=CARTESIAN_POINT('Ctrl Pts',(7.81090337322782,-1.25448504018068,
77.5971474903222));
#235621=CARTESIAN_POINT('Ctrl Pts',(7.81013776701363,-1.25924274151509,
77.5969525208757));
#235622=CARTESIAN_POINT('Ctrl Pts',(7.80819330922427,-1.27125618240845,
77.5964596636944));
#235623=CARTESIAN_POINT('Ctrl Pts',(7.80700869243913,-1.27851097421516,
77.5961615261888));
#235624=CARTESIAN_POINT('Ctrl Pts',(7.80293571402801,-1.30323783670821,
77.5951436676677));
#235625=CARTESIAN_POINT('Ctrl Pts',(7.79999880958345,-1.32070177547351,
77.5944218827913));
#235626=CARTESIAN_POINT('Ctrl Pts',(7.7928480186949,-1.36236713931284,77.5926931657397));
#235627=CARTESIAN_POINT('Ctrl Pts',(7.78858000921853,-1.38655900952019,
77.5916840397113));
#235628=CARTESIAN_POINT('Ctrl Pts',(7.73414629470008,-1.68691610221818,
77.5790912538922));
#235629=CARTESIAN_POINT('Ctrl Pts',(7.66943194442527,-1.96023048788132,
77.5669693061806));
#235630=CARTESIAN_POINT('Ctrl Pts',(7.43972373944825,-2.74226805759188,
77.5313010349159));
#235631=CARTESIAN_POINT('Ctrl Pts',(7.23752780369644,-3.23848376741513,
77.5075350869696));
#235632=CARTESIAN_POINT('Ctrl Pts',(6.8508420050389,-3.96660545301836,77.4724651936643));
#235633=CARTESIAN_POINT('Ctrl Pts',(6.70086303092373,-4.21502598328224,
77.4604301065471));
#235634=CARTESIAN_POINT('Ctrl Pts',(6.51751906717591,-4.48409800608915,
77.4472500496257));
#235635=CARTESIAN_POINT('Ctrl Pts',(6.49726339263907,-4.51339762827026,
77.4458126449998));
#235636=CARTESIAN_POINT('Ctrl Pts',(6.46731197051676,-4.55610255684141,
77.4437139447329));
#235637=CARTESIAN_POINT('Ctrl Pts',(6.45777103912562,-4.56961572138255,
77.4430493106526));
#235638=CARTESIAN_POINT('Ctrl Pts',(6.44076050364316,-4.59354868235458,
77.4418711736407));
#235639=CARTESIAN_POINT('Ctrl Pts',(6.4333078312704,-4.60398042042706,77.4413573113864));
#235640=CARTESIAN_POINT('Ctrl Pts',(6.41774058016381,-4.62565878298052,
77.4402886988107));
#235641=CARTESIAN_POINT('Ctrl Pts',(6.4096217176148,-4.63690228162128,77.4397340414066));
#235642=CARTESIAN_POINT('Ctrl Pts',(6.3885066861093,-4.66598225008422,77.4382983443235));
#235643=CARTESIAN_POINT('Ctrl Pts',(6.37546535135251,-4.6837858187223,77.4374182527858));
#235644=CARTESIAN_POINT('Ctrl Pts',(6.32151530668096,-4.75679369269768,
77.4338042765838));
#235645=CARTESIAN_POINT('Ctrl Pts',(6.27996224929837,-4.81151913011076,
77.4310833767849));
#235646=CARTESIAN_POINT('Ctrl Pts',(6.01025098885638,-5.15728221383457,
77.4138110050535));
#235647=CARTESIAN_POINT('Ctrl Pts',(5.76262969289628,-5.43256809781041,
77.3997148571322));
#235648=CARTESIAN_POINT('Ctrl Pts',(5.04355695442311,-6.1272632909503,77.3623997314067));
#235649=CARTESIAN_POINT('Ctrl Pts',(4.53982978152938,-6.50927652500992,
77.339990075988));
#235650=CARTESIAN_POINT('Ctrl Pts',(3.89154994654811,-6.88871952010248,
77.3110870268858));
#235651=CARTESIAN_POINT('Ctrl Pts',(3.78553334723148,-6.94754296678254,
77.3063520837916));
#235652=CARTESIAN_POINT('Ctrl Pts',(3.65627492423814,-7.01542504296894,
77.3005302852983));
#235653=CARTESIAN_POINT('Ctrl Pts',(3.63428586580618,-7.02684147280587,
77.2995382200967));
#235654=CARTESIAN_POINT('Ctrl Pts',(3.60403485241907,-7.04236742279755,
77.2981707185742));
#235655=CARTESIAN_POINT('Ctrl Pts',(3.59581866938999,-7.04656613047035,
77.2977990338594));
#235656=CARTESIAN_POINT('Ctrl Pts',(3.58290827693169,-7.05313525557956,
77.2972145437632));
#235657=CARTESIAN_POINT('Ctrl Pts',(3.5782190027728,-7.05551539027658,77.2970021543736));
#235658=CARTESIAN_POINT('Ctrl Pts',(3.56843965912522,-7.0604668344007,77.2965590238204));
#235659=CARTESIAN_POINT('Ctrl Pts',(3.56334917687087,-7.06303731860187,
77.2963282471859));
#235660=CARTESIAN_POINT('Ctrl Pts',(3.55169673038865,-7.06890552134831,
77.295799720181));
#235661=CARTESIAN_POINT('Ctrl Pts',(3.5451329504574,-7.07219960814905,77.295501811451));
#235662=CARTESIAN_POINT('Ctrl Pts',(3.52554709553433,-7.08199481194364,
77.2946122801777));
#235663=CARTESIAN_POINT('Ctrl Pts',(3.51251170045875,-7.08846911466292,
77.2940194711463));
#235664=CARTESIAN_POINT('Ctrl Pts',(3.40090217233104,-7.14351887065642,
77.2889366581301));
#235665=CARTESIAN_POINT('Ctrl Pts',(3.30135504972178,-7.1900661783184,77.2843516872889));
#235666=CARTESIAN_POINT('Ctrl Pts',(3.11084011433444,-7.27435805145224,
77.2754578721429));
#235667=CARTESIAN_POINT('Ctrl Pts',(3.02008551882568,-7.31250255167785,
77.2711771876931));
#235668=CARTESIAN_POINT('Ctrl Pts',(2.7452032725329,-7.4220465724783,77.2581308631111));
#235669=CARTESIAN_POINT('Ctrl Pts',(2.55909403969478,-7.4882540376892,77.2491918114139));
#235670=CARTESIAN_POINT('Ctrl Pts',(1.82925535387079,-7.71750251658468,
77.214206600622));
#235671=CARTESIAN_POINT('Ctrl Pts',(1.27100822792951,-7.82883558825758,
77.1877376174386));
#235672=CARTESIAN_POINT('Ctrl Pts',(0.430699374555759,-7.90408857817761,
77.1509129639977));
#235673=CARTESIAN_POINT('Ctrl Pts',(0.154646174034814,-7.91430497799267,
77.1392607489023));
#235674=CARTESIAN_POINT('Ctrl Pts',(-0.144142949810752,-7.90971942074254,
77.1271552551416));
#235675=CARTESIAN_POINT('Ctrl Pts',(-0.166887518147169,-7.90927222143669,
77.1262368631341));
#235676=CARTESIAN_POINT('Ctrl Pts',(-0.19861546211328,-7.90851147079419,
77.1249600396358));
#235677=CARTESIAN_POINT('Ctrl Pts',(-0.207600598885092,-7.90828070932663,
77.1245989335158));
#235678=CARTESIAN_POINT('Ctrl Pts',(-0.223116893656547,-7.90785574886825,
77.123976173667));
#235679=CARTESIAN_POINT('Ctrl Pts',(-0.229648231400032,-7.90766877045632,
77.1237142864249));
#235680=CARTESIAN_POINT('Ctrl Pts',(-0.24316595350552,-7.90726502498545,
77.1231727894401));
#235681=CARTESIAN_POINT('Ctrl Pts',(-0.250152299030421,-7.90704709002894,
77.1228932177665));
#235682=CARTESIAN_POINT('Ctrl Pts',(-0.266477462127926,-7.90651617801907,
77.1222406102038));
#235683=CARTESIAN_POINT('Ctrl Pts',(-0.275816041442402,-7.90619591353404,
77.1218678109886));
#235684=CARTESIAN_POINT('Ctrl Pts',(-0.305820475653556,-7.90511369262563,
77.1206716738303));
#235685=CARTESIAN_POINT('Ctrl Pts',(-0.326483998381034,-7.90428724579868,
77.1198504308232));
#235686=CARTESIAN_POINT('Ctrl Pts',(-0.763086382203918,-7.88511013841454,
77.1025508603036));
#235687=CARTESIAN_POINT('Ctrl Pts',(-1.17695459106484,-7.83403434255653,
77.0872118346868));
#235688=CARTESIAN_POINT('Ctrl Pts',(-1.68121039943816,-7.73091923439417,
77.069161214131));
#235689=CARTESIAN_POINT('Ctrl Pts',(-1.77712688897886,-7.70943584865565,
77.0657542522054));
#235690=CARTESIAN_POINT('Ctrl Pts',(-1.95474462927927,-7.66616196928083,
77.0594723494524));
#235691=CARTESIAN_POINT('Ctrl Pts',(-2.03654452042719,-7.64483829336407,
77.0565900791355));
#235692=CARTESIAN_POINT('Ctrl Pts',(-2.18518747594735,-7.60353478318354,
77.051356486278));
#235693=CARTESIAN_POINT('Ctrl Pts',(-2.25213774819018,-7.58397396754472,
77.0490006799641));
#235694=CARTESIAN_POINT('Ctrl Pts',(-2.37554030182798,-7.54614131523068,
77.0446513062508));
#235695=CARTESIAN_POINT('Ctrl Pts',(-2.43206244761335,-7.52811482018747,
77.0426563428677));
#235696=CARTESIAN_POINT('Ctrl Pts',(-2.5372073317395,-7.49327339825308,
77.0389334112788));
#235697=CARTESIAN_POINT('Ctrl Pts',(-2.58587911634988,-7.47661664517903,
77.0372052789929));
#235698=CARTESIAN_POINT('Ctrl Pts',(-2.67701312719155,-7.44443184642277,
77.0339559704908));
#235699=CARTESIAN_POINT('Ctrl Pts',(-2.71951140998211,-7.42901221425867,
77.0324351507376));
#235700=CARTESIAN_POINT('Ctrl Pts',(-2.90857263975468,-7.35857549968119,
77.0256369752713));
#235701=CARTESIAN_POINT('Ctrl Pts',(-3.05361358118064,-7.2995801864152,
77.0203345320018));
#235702=CARTESIAN_POINT('Ctrl Pts',(-3.46098547768449,-7.11961457491311,
77.0049763286912));
#235703=CARTESIAN_POINT('Ctrl Pts',(-3.71855780394466,-6.9885360624109,
76.9947038083995));
#235704=CARTESIAN_POINT('Ctrl Pts',(-4.0434594698607,-6.80013906846717,
76.9803157999025));
#235705=CARTESIAN_POINT('Ctrl Pts',(-4.11782739016114,-6.75536471025688,
76.9769197222449));
#235706=CARTESIAN_POINT('Ctrl Pts',(-4.20068641771042,-6.70360152903413,
76.9730025614776));
#235707=CARTESIAN_POINT('Ctrl Pts',(-4.20991996119274,-6.69780663784926,
76.9725641580478));
#235708=CARTESIAN_POINT('Ctrl Pts',(-4.22331485818136,-6.68936147546022,
76.9719253881815));
#235709=CARTESIAN_POINT('Ctrl Pts',(-4.22748579266486,-6.68672634502883,
76.9717260929184));
#235710=CARTESIAN_POINT('Ctrl Pts',(-4.23483171764353,-6.68207568546012,
76.9713743917217));
#235711=CARTESIAN_POINT('Ctrl Pts',(-4.23800774498987,-6.68006178835826,
76.971222102372));
#235712=CARTESIAN_POINT('Ctrl Pts',(-4.24410476732026,-6.6761896100594,
76.970929307124));
#235713=CARTESIAN_POINT('Ctrl Pts',(-4.24702598169726,-6.67433167412037,
76.9707888260713));
#235714=CARTESIAN_POINT('Ctrl Pts',(-4.25324772295441,-6.67036881524532,
76.9704892018728));
#235715=CARTESIAN_POINT('Ctrl Pts',(-4.25654789250817,-6.66826336933369,
76.9703300204901));
#235716=CARTESIAN_POINT('Ctrl Pts',(-4.26913289940549,-6.66022122303928,
76.9697220274329));
#235717=CARTESIAN_POINT('Ctrl Pts',(-4.27840684348422,-6.65426760295549,
76.969271992865));
#235718=CARTESIAN_POINT('Ctrl Pts',(-4.3001165353017,-6.64026642497335,
76.9682138578564));
#235719=CARTESIAN_POINT('Ctrl Pts',(-4.31254214509926,-6.63220330302189,
76.9676046549331));
#235720=CARTESIAN_POINT('Ctrl Pts',(-4.35530968798281,-6.60427994463422,
76.9654957263624));
#235721=CARTESIAN_POINT('Ctrl Pts',(-4.38553727003681,-6.58424626172705,
76.9639840542439));
#235722=CARTESIAN_POINT('Ctrl Pts',(-4.51833140011995,-6.49491526874732,
76.9572538114778));
#235723=CARTESIAN_POINT('Ctrl Pts',(-4.61939701760682,-6.42342676278368,
76.9518950872519));
#235724=CARTESIAN_POINT('Ctrl Pts',(-4.87761245171966,-6.2315325976487,
76.9376770125713));
#235725=CARTESIAN_POINT('Ctrl Pts',(-5.03199220126173,-6.10754855743923,
76.9286502255891));
#235726=CARTESIAN_POINT('Ctrl Pts',(-5.83964539130386,-5.40748851329033,
76.8792491002531));
#235727=CARTESIAN_POINT('Ctrl Pts',(-6.39925362171106,-4.73209035673655,
76.8379236073619));
#235728=CARTESIAN_POINT('Ctrl Pts',(-6.8654387019972,-3.93099949669461,
76.7999503332903));
#235729=CARTESIAN_POINT('Ctrl Pts',(-6.89286745075898,-3.8827031946666,
76.7976946304945));
#235730=CARTESIAN_POINT('Ctrl Pts',(-6.92586940484383,-3.8231415816002,
76.7949532412712));
#235731=CARTESIAN_POINT('Ctrl Pts',(-6.93192695229304,-3.812147333986,76.7944488939623));
#235732=CARTESIAN_POINT('Ctrl Pts',(-6.94189496342214,-3.79395340536654,
76.7936170244948));
#235733=CARTESIAN_POINT('Ctrl Pts',(-6.94582044419765,-3.78676200503892,
76.793288925647));
#235734=CARTESIAN_POINT('Ctrl Pts',(-6.95288917055197,-3.77376427126368,
76.7926971957264));
#235735=CARTESIAN_POINT('Ctrl Pts',(-6.95603632939854,-3.76796008171878,
76.7924334147918));
#235736=CARTESIAN_POINT('Ctrl Pts',(-6.962748624193,-3.75554377239112,76.7918701122475));
#235737=CARTESIAN_POINT('Ctrl Pts',(-6.96631161743391,-3.74893049805985,
76.7915706727517));
#235738=CARTESIAN_POINT('Ctrl Pts',(-6.97591714162689,-3.73104069995804,
76.7907622410929));
#235739=CARTESIAN_POINT('Ctrl Pts',(-6.98194175947876,-3.71975455385849,
76.7902539329127));
#235740=CARTESIAN_POINT('Ctrl Pts',(-7.01148694758599,-3.66408176330713,
76.7877548877017));
#235741=CARTESIAN_POINT('Ctrl Pts',(-7.03461201682153,-3.61948591418087,
76.7857792028819));
#235742=CARTESIAN_POINT('Ctrl Pts',(-7.22313578221371,-3.24729211351989,
76.7695012767698));
#235743=CARTESIAN_POINT('Ctrl Pts',(-7.36598791958262,-2.90875467002388,
76.7560765859012));
#235744=CARTESIAN_POINT('Ctrl Pts',(-7.73503805004267,-1.8303709722937,
76.7160351704568));
#235745=CARTESIAN_POINT('Ctrl Pts',(-7.87673204921938,-1.06667459132602,
76.6917928232895));
#235746=CARTESIAN_POINT('Ctrl Pts',(-7.90668256405158,-0.26321844054238,
76.6609546739394));
#235747=CARTESIAN_POINT('Ctrl Pts',(-7.90766789019368,-0.231736072585083,
76.6597372276119));
#235748=CARTESIAN_POINT('Ctrl Pts',(-7.90985546229389,-0.145341961306333,
76.6563692697658));
#235749=CARTESIAN_POINT('Ctrl Pts',(-7.91067387089617,-0.0904231612133168,
76.6541983792898));
#235750=CARTESIAN_POINT('Ctrl Pts',(-7.91096236434687,-0.0261373439966448,
76.6516174170969));
#235751=CARTESIAN_POINT('Ctrl Pts',(-7.91098776064491,-0.0167731570304957,
76.6512404679346));
#235752=CARTESIAN_POINT('Ctrl Pts',(-7.91100010611559,-0.00359118555788957,
76.650708449942));
#235753=CARTESIAN_POINT('Ctrl Pts',(-7.91100091797001,0.00022660524541699,
76.6505542023486));
#235754=CARTESIAN_POINT('Ctrl Pts',(-7.91099896618133,0.00404438844160049,
76.6503997926682));
#235755=CARTESIAN_POINT('',(-7.90827614865568,-0.00626907122509836,74.6423315082369));
#235756=CARTESIAN_POINT('Ctrl Pts',(-7.92502143214218,0.00372523665453262,
76.642331508237));
#235757=CARTESIAN_POINT('Ctrl Pts',(-7.9241870030526,2.61244749534328,76.5367896921557));
#235758=CARTESIAN_POINT('Ctrl Pts',(-5.79219513848909,6.51283346952887,
76.378263087466));
#235759=CARTESIAN_POINT('Ctrl Pts',(-0.626326385655128,8.21169917704909,
76.1667516941681));
#235760=CARTESIAN_POINT('Ctrl Pts',(3.3870778892776,7.52640590708394,76.0077973283437));
#235761=CARTESIAN_POINT('Ctrl Pts',(6.55629850510655,4.98354837003805,75.8488429625187));
#235762=CARTESIAN_POINT('Ctrl Pts',(8.72532350098204,-0.030839795427598,
75.6369038080857));
#235763=CARTESIAN_POINT('Ctrl Pts',(6.69212697694097,-5.60207094650804,
75.4249646536528));
#235764=CARTESIAN_POINT('Ctrl Pts',(1.80805205364573,-8.025049431192,75.2130254992196));
#235765=CARTESIAN_POINT('Ctrl Pts',(-3.62141351739191,-7.93641147911786,
75.0010863447868));
#235766=CARTESIAN_POINT('Ctrl Pts',(-7.450008814502,-4.19522544625671,74.8108550144591));
#235767=CARTESIAN_POINT('Ctrl Pts',(-7.91343195938039,-0.787962566203169,
74.6736084727398));
#235768=CARTESIAN_POINT('Ctrl Pts',(-7.90689550057179,-0.00944669734432524,
74.6423315082369));
#235769=CARTESIAN_POINT('',(-7.90134992664127,0.00118378181009326,72.642331508237));
#235770=CARTESIAN_POINT('Ctrl Pts',(-7.911,1.34503519433338E-12,74.642331508237));
#235771=CARTESIAN_POINT('Ctrl Pts',(-7.91099999999962,2.20167589666814,
74.5537440725043));
#235772=CARTESIAN_POINT('Ctrl Pts',(-6.94214576672294,4.38610418338807,
74.4651566367715));
#235773=CARTESIAN_POINT('Ctrl Pts',(-3.67820201488151,7.34180684107701,
74.2879817653061));
#235774=CARTESIAN_POINT('Ctrl Pts',(-1.40868175871591,8.08992666571364,
74.1993943295733));
#235775=CARTESIAN_POINT('Ctrl Pts',(2.97309270521424,7.654542280252,74.0222194581079));
#235776=CARTESIAN_POINT('Ctrl Pts',(5.05102072675732,6.47444880834125,73.9336320223751));
#235777=CARTESIAN_POINT('Ctrl Pts',(7.66951518847933,2.93425195367549,73.7564571509097));
#235778=CARTESIAN_POINT('Ctrl Pts',(8.18956872247085,0.601881960097444,
73.667869715177));
#235779=CARTESIAN_POINT('Ctrl Pts',(7.32306689761263,-3.71537198232609,
73.4906948437115));
#235780=CARTESIAN_POINT('Ctrl Pts',(5.94329958850077,-5.66643518936643,
73.4021074079788));
#235781=CARTESIAN_POINT('Ctrl Pts',(2.16154501637667,-7.92205913233048,
73.2249325365133));
#235782=CARTESIAN_POINT('Ctrl Pts',(-0.210816529302271,-8.20894963712998,
73.1363451007806));
#235783=CARTESIAN_POINT('Ctrl Pts',(-4.42123908576603,-6.91982244717726,
72.9591702293152));
#235784=CARTESIAN_POINT('Ctrl Pts',(-6.22631625634318,-5.3539035880337,
72.8705827935824));
#235785=CARTESIAN_POINT('Ctrl Pts',(-7.65317280859534,-2.31334857514354,
72.7354407413121));
#235786=CARTESIAN_POINT('Ctrl Pts',(-7.91100000000017,-1.15702837836376,
72.6888861247746));
#235787=CARTESIAN_POINT('Ctrl Pts',(-7.911,1.17517107156573E-12,72.642331508237));
#235788=CARTESIAN_POINT('',(-7.921302937514,0.00357332256267995,70.6425359502471));
#235789=CARTESIAN_POINT('Ctrl Pts',(-7.89504541711033,0.00195716076996755,
72.642331508237));
#235790=CARTESIAN_POINT('Ctrl Pts',(-7.89841756211971,1.09499239008904,
72.5984880988909));
#235791=CARTESIAN_POINT('Ctrl Pts',(-7.4313217434443,3.50649690015027,72.5016599009365));
#235792=CARTESIAN_POINT('Ctrl Pts',(-5.03519156416044,6.50517613243061,
72.3518469143741));
#235793=CARTESIAN_POINT('Ctrl Pts',(-0.0564887115056478,8.72723159946603,
72.139907759941));
#235794=CARTESIAN_POINT('Ctrl Pts',(5.53353127081588,6.74627697064648,71.9279686055081));
#235795=CARTESIAN_POINT('Ctrl Pts',(8.01779672670277,1.88035637415614,71.7160294510749));
#235796=CARTESIAN_POINT('Ctrl Pts',(7.95963757450901,-2.18248761478921,
71.5570750852503));
#235797=CARTESIAN_POINT('Ctrl Pts',(5.9317470407567,-5.71302591978898,71.3981207194254));
#235798=CARTESIAN_POINT('Ctrl Pts',(1.32250398506214,-8.61939107734134,
71.1861815649926));
#235799=CARTESIAN_POINT('Ctrl Pts',(-5.61612825759075,-7.27095079450261,
70.9343199752662));
#235800=CARTESIAN_POINT('Ctrl Pts',(-7.90096779956093,-2.29930440440434,
70.7354431741484));
#235801=CARTESIAN_POINT('Ctrl Pts',(-7.921302937514,0.00357332256267995,
70.6425359502471));
#235802=CARTESIAN_POINT('',(-7.9109998986396,0.00126638231751385,66.6333051339456));
#235803=CARTESIAN_POINT('Ctrl Pts',(-7.91099908888364,0.00379679894604718,
70.6484690865411));
#235804=CARTESIAN_POINT('Ctrl Pts',(-7.91085111670076,0.312111202886401,
70.6376639763182));
#235805=CARTESIAN_POINT('Ctrl Pts',(-7.89267928218732,0.620131437501612,
70.6264055364096));
#235806=CARTESIAN_POINT('Ctrl Pts',(-7.85564523625669,0.934250163225403,
70.6137358191232));
#235807=CARTESIAN_POINT('Ctrl Pts',(-7.85469315267901,0.94222127003831,
70.6134135179521));
#235808=CARTESIAN_POINT('Ctrl Pts',(-7.85313376871219,0.955110237079679,
70.6128910660888));
#235809=CARTESIAN_POINT('Ctrl Pts',(-7.85253397562235,0.960029018171404,
70.6126913770645));
#235810=CARTESIAN_POINT('Ctrl Pts',(-7.85147662380977,0.968632858645214,
70.6123415421385));
#235811=CARTESIAN_POINT('Ctrl Pts',(-7.85102109270882,0.972318153061019,
70.6121915223589));
#235812=CARTESIAN_POINT('Ctrl Pts',(-7.85009695676984,0.979751517934062,
70.6118885756235));
#235813=CARTESIAN_POINT('Ctrl Pts',(-7.84962826330846,0.983499565505954,
70.6117356437699));
#235814=CARTESIAN_POINT('Ctrl Pts',(-7.84872081693304,0.990714261547698,
70.6114409170494));
#235815=CARTESIAN_POINT('Ctrl Pts',(-7.84828245104744,0.994180958727498,
70.6112991460335));
#235816=CARTESIAN_POINT('Ctrl Pts',(-7.84724280810808,1.00235915238736,
70.6109643378259));
#235817=CARTESIAN_POINT('Ctrl Pts',(-7.84663958513004,1.00707039507899,
70.6107711816911));
#235818=CARTESIAN_POINT('Ctrl Pts',(-7.84484102864902,1.02101761368873,
70.6101985312313));
#235819=CARTESIAN_POINT('Ctrl Pts',(-7.84363363211445,1.03025199631504,
70.6098183059978));
#235820=CARTESIAN_POINT('Ctrl Pts',(-7.83289144343958,1.1112966609469,70.6064719804277));
#235821=CARTESIAN_POINT('Ctrl Pts',(-7.82238731904701,1.18297278297795,
70.6034482681321));
#235822=CARTESIAN_POINT('Ctrl Pts',(-7.78662004678917,1.40567213821601,
70.5938754768716));
#235823=CARTESIAN_POINT('Ctrl Pts',(-7.75795657129801,1.55610757728357,
70.5871532256732));
#235824=CARTESIAN_POINT('Ctrl Pts',(-7.72306885283454,1.71411915122023,
70.5798893732315));
#235825=CARTESIAN_POINT('Ctrl Pts',(-7.7211756080123,1.72262712148943,70.5794976307331));
#235826=CARTESIAN_POINT('Ctrl Pts',(-7.70632924678631,1.78882834170141,
70.5764446503151));
#235827=CARTESIAN_POINT('Ctrl Pts',(-7.69274391390513,1.84637703676291,
70.5737623187859));
#235828=CARTESIAN_POINT('Ctrl Pts',(-7.67210176582676,1.92963356519597,
70.5698455637178));
#235829=CARTESIAN_POINT('Ctrl Pts',(-7.66555796445398,1.95546727875049,
70.5686251484955));
#235830=CARTESIAN_POINT('Ctrl Pts',(-7.50309063339445,2.58350894708661,
70.5388393957115));
#235831=CARTESIAN_POINT('Ctrl Pts',(-7.2768080497462,3.16529005472852,70.5088561641687));
#235832=CARTESIAN_POINT('Ctrl Pts',(-6.84381644008412,3.97945882441195,
70.4671975057645));
#235833=CARTESIAN_POINT('Ctrl Pts',(-6.68799608508582,4.23611270602389,
70.454075784752));
#235834=CARTESIAN_POINT('Ctrl Pts',(-6.44887509277901,4.58375298753841,
70.4363977074597));
#235835=CARTESIAN_POINT('Ctrl Pts',(-6.3774759807538,4.68258297951504,70.4313817155536));
#235836=CARTESIAN_POINT('Ctrl Pts',(-6.2935320512866,4.79329377436658,70.4257691237696));
#235837=CARTESIAN_POINT('Ctrl Pts',(-6.2832012834344,4.80682769866909,70.4250831122121));
#235838=CARTESIAN_POINT('Ctrl Pts',(-6.26756868077619,4.82717083824188,
70.4240520819537));
#235839=CARTESIAN_POINT('Ctrl Pts',(-6.26229929776086,4.83400485888472,
70.4237057423555));
#235840=CARTESIAN_POINT('Ctrl Pts',(-6.25319835101844,4.84576829432973,
70.4231096196414));
#235841=CARTESIAN_POINT('Ctrl Pts',(-6.24937212040819,4.85070181318161,
70.4228596192865));
#235842=CARTESIAN_POINT('Ctrl Pts',(-6.24146264280682,4.86087535418988,
70.4223441057653));
#235843=CARTESIAN_POINT('Ctrl Pts',(-6.23737862691588,4.86611477416117,
70.4220786243237));
#235844=CARTESIAN_POINT('Ctrl Pts',(-6.22632701103339,4.88025621712261,
70.4213621019252));
#235845=CARTESIAN_POINT('Ctrl Pts',(-6.21934690939891,4.88914847545498,
70.4209115730244));
#235846=CARTESIAN_POINT('Ctrl Pts',(-6.19346844107335,4.92197109669149,
70.4192486787925));
#235847=CARTESIAN_POINT('Ctrl Pts',(-6.17445070852578,4.945807242751,70.4180412131867));
#235848=CARTESIAN_POINT('Ctrl Pts',(-5.86704150791861,5.32656625209827,
70.3987532337327));
#235849=CARTESIAN_POINT('Ctrl Pts',(-5.54825549440634,5.65786199287062,
70.3820450583095));
#235850=CARTESIAN_POINT('Ctrl Pts',(-5.01234261201949,6.12568958486638,
70.357097805476));
#235851=CARTESIAN_POINT('Ctrl Pts',(-4.81432370874393,6.28251065701358,
70.3484290460469));
#235852=CARTESIAN_POINT('Ctrl Pts',(-4.18589931810519,6.73300550330014,
70.3217290308855));
#235853=CARTESIAN_POINT('Ctrl Pts',(-3.73370988021265,6.99389512970278,
70.3035642305113));
#235854=CARTESIAN_POINT('Ctrl Pts',(-3.24188190811885,7.21626510581342,
70.2819974320534));
#235855=CARTESIAN_POINT('Ctrl Pts',(-3.22458010991415,7.22401297686637,
70.2812371534633));
#235856=CARTESIAN_POINT('Ctrl Pts',(-3.1997706770104,7.23501593439064,70.2801448440562));
#235857=CARTESIAN_POINT('Ctrl Pts',(-3.19228549784985,7.23832171541877,
70.279815010035));
#235858=CARTESIAN_POINT('Ctrl Pts',(-3.17942350359844,7.24397830071323,
70.2792477859357));
#235859=CARTESIAN_POINT('Ctrl Pts',(-3.17404916783322,7.24633475050503,
70.2790106355001));
#235860=CARTESIAN_POINT('Ctrl Pts',(-3.16313491866869,7.25110577823717,
70.2785287542763));
#235861=CARTESIAN_POINT('Ctrl Pts',(-3.15759485083167,7.25351999229542,
70.2782840085017));
#235862=CARTESIAN_POINT('Ctrl Pts',(-3.14396060201519,7.25944285461772,
70.2776813389419));
#235863=CARTESIAN_POINT('Ctrl Pts',(-3.13586331859388,7.26294431155796,
70.2773231199561));
#235864=CARTESIAN_POINT('Ctrl Pts',(-3.10730635666155,7.27523635899781,
70.2760587630225));
#235865=CARTESIAN_POINT('Ctrl Pts',(-3.08681554067741,7.28395405524975,
70.2751497022249));
#235866=CARTESIAN_POINT('Ctrl Pts',(-2.67460507172667,7.45727478235392,
70.2568287150775));
#235867=CARTESIAN_POINT('Ctrl Pts',(-2.27030736478798,7.59013373184248,
70.2382873801141));
#235868=CARTESIAN_POINT('Ctrl Pts',(-1.51413666916433,7.77277038709964,
70.2042132127489));
#235869=CARTESIAN_POINT('Ctrl Pts',(-1.16577580760339,7.83259525855842,
70.1887346706286));
#235870=CARTESIAN_POINT('Ctrl Pts',(-0.467377151526313,7.90489220096417,
70.1586024307851));
#235871=CARTESIAN_POINT('Ctrl Pts',(-0.118163842135427,7.91781675258459,
70.1439741788804));
#235872=CARTESIAN_POINT('Ctrl Pts',(0.297091073903576,7.90569788941216,
70.1270506555417));
#235873=CARTESIAN_POINT('Ctrl Pts',(0.363378115011865,7.90292848884497,
70.1243626356777));
#235874=CARTESIAN_POINT('Ctrl Pts',(0.451347280069408,7.89814408432846,
70.1208117156702));
#235875=CARTESIAN_POINT('Ctrl Pts',(0.473066739764483,7.89687293865306,
70.119936344933));
#235876=CARTESIAN_POINT('Ctrl Pts',(0.50855295312103,7.89464915702493,70.118508341239));
#235877=CARTESIAN_POINT('Ctrl Pts',(0.522322907349464,7.89375007208344,
70.1179547687966));
#235878=CARTESIAN_POINT('Ctrl Pts',(0.54890553671837,7.89194454462674,70.1168871637592));
#235879=CARTESIAN_POINT('Ctrl Pts',(0.561718492308982,7.89104291714704,
70.1163730468352));
#235880=CARTESIAN_POINT('Ctrl Pts',(0.591182860446031,7.88889742865696,
70.1151918867361));
#235881=CARTESIAN_POINT('Ctrl Pts',(0.607832659738781,7.88763204483272,
70.114525235612));
#235882=CARTESIAN_POINT('Ctrl Pts',(0.660816081482424,7.88343654857742,
70.1124063517427));
#235883=CARTESIAN_POINT('Ctrl Pts',(0.697133653399223,7.88030801462151,
70.1109577816051));
#235884=CARTESIAN_POINT('Ctrl Pts',(1.05634167683523,7.84686180562356,70.0966678279628));
#235885=CARTESIAN_POINT('Ctrl Pts',(1.37710928346311,7.79696641204329,70.0842275348371));
#235886=CARTESIAN_POINT('Ctrl Pts',(2.05243821633732,7.64892982110479,70.0583750390849));
#235887=CARTESIAN_POINT('Ctrl Pts',(2.40505424527053,7.5454853662534,70.0450873164853));
#235888=CARTESIAN_POINT('Ctrl Pts',(3.15287494442057,7.26833028500581,70.016060340955));
#235889=CARTESIAN_POINT('Ctrl Pts',(3.54362151929933,7.0860378322976,70.0003463056089));
#235890=CARTESIAN_POINT('Ctrl Pts',(3.93709124265025,6.86175916029078,69.9823070155802));
#235891=CARTESIAN_POINT('Ctrl Pts',(3.95657128074476,6.85054522739924,69.9814078100892));
#235892=CARTESIAN_POINT('Ctrl Pts',(3.98299501487949,6.83518376637818,69.9801794085816));
#235893=CARTESIAN_POINT('Ctrl Pts',(3.98998065230025,6.83110831434241,69.9798538285351));
#235894=CARTESIAN_POINT('Ctrl Pts',(4.00155282443592,6.82433325076383,69.9793130901883));
#235895=CARTESIAN_POINT('Ctrl Pts',(4.00614291704869,6.82163970407463,69.9790982425227));
#235896=CARTESIAN_POINT('Ctrl Pts',(4.01513314368848,6.81635187838577,69.9786767176554));
#235897=CARTESIAN_POINT('Ctrl Pts',(4.01953349069685,6.81375796521284,69.9784700594784));
#235898=CARTESIAN_POINT('Ctrl Pts',(4.02984062073914,6.80766866697595,69.9779851926491));
#235899=CARTESIAN_POINT('Ctrl Pts',(4.03574536688144,6.80416985686918,69.9777068039797));
#235900=CARTESIAN_POINT('Ctrl Pts',(4.05436845635412,6.79310212386769,69.9768268127022));
#235901=CARTESIAN_POINT('Ctrl Pts',(4.06707006324639,6.78550522372069,69.9762237141692));
#235902=CARTESIAN_POINT('Ctrl Pts',(4.21455721300191,6.69672947493527,69.9691859233771));
#235903=CARTESIAN_POINT('Ctrl Pts',(4.34689781450766,6.611591881653,69.9625175395935));
#235904=CARTESIAN_POINT('Ctrl Pts',(4.49141693563802,6.51240492171535,69.954896315438));
#235905=CARTESIAN_POINT('Ctrl Pts',(4.506199088833,6.50218530335804,69.9541127497701));
#235906=CARTESIAN_POINT('Ctrl Pts',(4.88080318364001,6.24131237997012,69.9341556396123));
#235907=CARTESIAN_POINT('Ctrl Pts',(5.21918581026922,5.96123222998659,69.9138075111628));
#235908=CARTESIAN_POINT('Ctrl Pts',(5.55480054094463,5.63285685444536,69.892170887116));
#235909=CARTESIAN_POINT('Ctrl Pts',(5.57686955544724,5.61100805194178,69.8907405711576));
#235910=CARTESIAN_POINT('Ctrl Pts',(5.6224270433021,5.56537084882231,69.887772777617));
#235911=CARTESIAN_POINT('Ctrl Pts',(5.64589455701557,5.54156234309739,69.8862354991175));
#235912=CARTESIAN_POINT('Ctrl Pts',(6.11017327219273,5.0645268526137,69.8556585526467));
#235913=CARTESIAN_POINT('Ctrl Pts',(6.49529097694306,4.56016125646242,69.8275820506758));
#235914=CARTESIAN_POINT('Ctrl Pts',(6.82785898509628,3.99559549115742,69.8010072135642));
#235915=CARTESIAN_POINT('Ctrl Pts',(6.83935515565928,3.97588514861531,69.8000847404929));
#235916=CARTESIAN_POINT('Ctrl Pts',(6.85587192229252,3.94728329816932,69.7987537622991));
#235917=CARTESIAN_POINT('Ctrl Pts',(6.86096078464382,3.93843145978668,69.7983428975758));
#235918=CARTESIAN_POINT('Ctrl Pts',(6.86980668222111,3.9229752587709,69.7976273148951));
#235919=CARTESIAN_POINT('Ctrl Pts',(6.87357136062883,3.91637529901719,69.7973223334946));
#235920=CARTESIAN_POINT('Ctrl Pts',(6.88082279752194,3.90361994501233,69.7967340300147));
#235921=CARTESIAN_POINT('Ctrl Pts',(6.88431081815265,3.89746527955838,69.7964506646591));
#235922=CARTESIAN_POINT('Ctrl Pts',(6.8925556290906,3.88287158476477,69.7957799425493));
#235923=CARTESIAN_POINT('Ctrl Pts',(6.89730518859998,3.87442847140674,69.7953928345009));
#235924=CARTESIAN_POINT('Ctrl Pts',(6.91391020143407,3.84478306459198,69.7940368882096));
#235925=CARTESIAN_POINT('Ctrl Pts',(6.9256835489925,3.82353481471798,69.793070865673));
#235926=CARTESIAN_POINT('Ctrl Pts',(7.072789262075,3.55513326023804,69.7809411441152));
#235927=CARTESIAN_POINT('Ctrl Pts',(7.19492659274341,3.30096485789362,69.7702396350478));
#235928=CARTESIAN_POINT('Ctrl Pts',(7.58128415428314,2.37303127808974,69.7333540655585));
#235929=CARTESIAN_POINT('Ctrl Pts',(7.76640568090853,1.67033374921405,69.7096243617332));
#235930=CARTESIAN_POINT('Ctrl Pts',(7.89055629463045,0.646484163189275,
69.6728061963327));
#235931=CARTESIAN_POINT('Ctrl Pts',(7.9097448885582,0.33876422807075,69.6613867989229));
#235932=CARTESIAN_POINT('Ctrl Pts',(7.91102115814423,0.00989856671989338,
69.6482873074684));
#235933=CARTESIAN_POINT('Ctrl Pts',(7.91101983562758,-0.0109039421744316,
69.6474554331701));
#235934=CARTESIAN_POINT('Ctrl Pts',(7.91090166082746,-0.0403895646851279,
69.6462719175508));
#235935=CARTESIAN_POINT('Ctrl Pts',(7.91085256132498,-0.0490729706879633,
69.6459228342876));
#235936=CARTESIAN_POINT('Ctrl Pts',(7.91074445807252,-0.0638797135054466,
69.6453266790896));
#235937=CARTESIAN_POINT('Ctrl Pts',(7.91069264120539,-0.0700031059670321,
69.6450798721526));
#235938=CARTESIAN_POINT('Ctrl Pts',(7.91057391319928,-0.0823406590634978,
69.644582074641));
#235939=CARTESIAN_POINT('Ctrl Pts',(7.91050678939655,-0.0885548133708192,
69.6443310765237));
#235940=CARTESIAN_POINT('Ctrl Pts',(7.91032545937528,-0.103690573067891,
69.6437190782218));
#235941=CARTESIAN_POINT('Ctrl Pts',(7.91020348221067,-0.112612066136967,
69.6433578017747));
#235942=CARTESIAN_POINT('Ctrl Pts',(7.909732101786,-0.143292135664065,69.6421135738512));
#235943=CARTESIAN_POINT('Ctrl Pts',(7.90930801361072,-0.165049366286971,
69.641228034447));
#235944=CARTESIAN_POINT('Ctrl Pts',(7.8983543625057,-0.628797282299028,
69.622288809918));
#235945=CARTESIAN_POINT('Ctrl Pts',(7.85088131162575,-1.06912505287338,
69.6031252746552));
#235946=CARTESIAN_POINT('Ctrl Pts',(7.66733155680383,-2.01753142667131,
69.5613877935405));
#235947=CARTESIAN_POINT('Ctrl Pts',(7.51692779039415,-2.52076444398268,
69.5389928345805));
#235948=CARTESIAN_POINT('Ctrl Pts',(7.17939710997416,-3.34260898662557,
69.5021188216819));
#235949=CARTESIAN_POINT('Ctrl Pts',(7.01778261593823,-3.66981115299856,
69.4872559492473));
#235950=CARTESIAN_POINT('Ctrl Pts',(6.80359677257546,-4.03716230087435,
69.470035079886));
#235951=CARTESIAN_POINT('Ctrl Pts',(6.77240716139427,-4.08926763381848,
69.4675810678151));
#235952=CARTESIAN_POINT('Ctrl Pts',(6.72480803686864,-4.16674818254992,
69.4639147372843));
#235953=CARTESIAN_POINT('Ctrl Pts',(6.70884811750134,-4.19239674802439,
69.462698194935));
#235954=CARTESIAN_POINT('Ctrl Pts',(6.68109670412087,-4.23643067305631,
69.4606046164647));
#235955=CARTESIAN_POINT('Ctrl Pts',(6.66937527225629,-4.25485975068267,
69.4597268905245));
#235956=CARTESIAN_POINT('Ctrl Pts',(6.64496603678464,-4.292888594775,69.4579125011512));
#235957=CARTESIAN_POINT('Ctrl Pts',(6.63226747718221,-4.31248121522757,
69.4569759586562));
#235958=CARTESIAN_POINT('Ctrl Pts',(6.59739156685677,-4.36577289285717,
69.4544237054893));
#235959=CARTESIAN_POINT('Ctrl Pts',(6.5750428482299,-4.39935904425975,69.4528098497111));
#235960=CARTESIAN_POINT('Ctrl Pts',(6.4869714695125,-4.52954443347194,69.4465328692085));
#235961=CARTESIAN_POINT('Ctrl Pts',(6.41936854251691,-4.62485454626016,
69.4418912884152));
#235962=CARTESIAN_POINT('Ctrl Pts',(6.24335135893663,-4.86171394576476,
69.4302256310461));
#235963=CARTESIAN_POINT('Ctrl Pts',(6.13221700718403,-5.00116132434242,
69.4232359555068));
#235964=CARTESIAN_POINT('Ctrl Pts',(5.71411960026755,-5.49086303833126,
69.3981324807483));
#235965=CARTESIAN_POINT('Ctrl Pts',(5.38110225772349,-5.81760006731186,
69.3803421874458));
#235966=CARTESIAN_POINT('Ctrl Pts',(4.88353924823955,-6.22629454296176,
69.3551939352448));
#235967=CARTESIAN_POINT('Ctrl Pts',(4.74200440747497,-6.33475263811398,
69.3481745377593));
#235968=CARTESIAN_POINT('Ctrl Pts',(4.57707525233675,-6.45251100880464,
69.3400585268874));
#235969=CARTESIAN_POINT('Ctrl Pts',(4.55715494757008,-6.46659531431703,
69.3390792766886));
#235970=CARTESIAN_POINT('Ctrl Pts',(4.52691008564798,-6.48777025922047,
69.3375937031529));
#235971=CARTESIAN_POINT('Ctrl Pts',(4.51663325988129,-6.49492893374636,
69.3370891347679));
#235972=CARTESIAN_POINT('Ctrl Pts',(4.4988316047149,-6.50726660255448,69.3362154308485));
#235973=CARTESIAN_POINT('Ctrl Pts',(4.49131471512252,-6.51245703045414,
69.3358465995636));
#235974=CARTESIAN_POINT('Ctrl Pts',(4.47456368880782,-6.52398085342755,
69.3350248686121));
#235975=CARTESIAN_POINT('Ctrl Pts',(4.46532506753547,-6.53030768198174,
69.3345717922119));
#235976=CARTESIAN_POINT('Ctrl Pts',(4.44075388331292,-6.54705809399899,
69.3333670728325));
#235977=CARTESIAN_POINT('Ctrl Pts',(4.42539817090038,-6.55744735109239,
69.3326144633712));
#235978=CARTESIAN_POINT('Ctrl Pts',(4.35164699687575,-6.60696834574201,
69.3290011023577));
#235979=CARTESIAN_POINT('Ctrl Pts',(4.29276886255612,-6.64537414912787,
69.3261206439571));
#235980=CARTESIAN_POINT('Ctrl Pts',(3.62946871326175,-7.06554634934173,
69.2937579911157));
#235981=CARTESIAN_POINT('Ctrl Pts',(2.97646681887383,-7.36449029828657,
69.2630367198319));
#235982=CARTESIAN_POINT('Ctrl Pts',(2.1564026146062,-7.61275088441271,69.2278140258897));
#235983=CARTESIAN_POINT('Ctrl Pts',(2.01953500521352,-7.65019788485756,
69.2220273593962));
#235984=CARTESIAN_POINT('Ctrl Pts',(1.84569791994503,-7.69276910910477,
69.2147845329974));
#235985=CARTESIAN_POINT('Ctrl Pts',(1.80960141012084,-7.70134015173828,
69.2132863100638));
#235986=CARTESIAN_POINT('Ctrl Pts',(1.75171301175758,-7.71465617064854,
69.2108924238215));
#235987=CARTESIAN_POINT('Ctrl Pts',(1.72995911662299,-7.71956344398234,
69.2099948138479));
#235988=CARTESIAN_POINT('Ctrl Pts',(1.6886430240166,-7.72870016824137,69.208293708787));
#235989=CARTESIAN_POINT('Ctrl Pts',(1.6690849658518,-7.73294749320868,69.2074900069883));
#235990=CARTESIAN_POINT('Ctrl Pts',(1.62457083606776,-7.74243765749569,
69.2056642451202));
#235991=CARTESIAN_POINT('Ctrl Pts',(1.59960508898883,-7.74763414511772,
69.204642737016));
#235992=CARTESIAN_POINT('Ctrl Pts',(1.53470577950242,-7.76081552327239,
69.2019934865123));
#235993=CARTESIAN_POINT('Ctrl Pts',(1.49473483680088,-7.768612952506,69.2003679146869));
#235994=CARTESIAN_POINT('Ctrl Pts',(1.18069502603767,-7.82736159315848,
69.1876409838368));
#235995=CARTESIAN_POINT('Ctrl Pts',(0.904163748080776,-7.86410337357121,
69.1767025735591));
#235996=CARTESIAN_POINT('Ctrl Pts',(0.621624658355644,-7.88654078051388,
69.1656400708757));
#235997=CARTESIAN_POINT('Ctrl Pts',(0.616980776040272,-7.88690544007183,
69.1654582820691));
#235998=CARTESIAN_POINT('Ctrl Pts',(0.531838900574727,-7.8935155232476,
69.1621260156729));
#235999=CARTESIAN_POINT('Ctrl Pts',(0.45124995457206,-7.89853236491864,
69.1589832594708));
#236000=CARTESIAN_POINT('Ctrl Pts',(0.251691676715693,-7.90789112937733,
69.1512305752475));
#236001=CARTESIAN_POINT('Ctrl Pts',(0.132673820317266,-7.91078307719717,
69.1466329624234));
#236002=CARTESIAN_POINT('Ctrl Pts',(-0.545637791419402,-7.91195219904935,
69.1205705481882));
#236003=CARTESIAN_POINT('Ctrl Pts',(-1.10343012256314,-7.85360758320182,
69.0998390865875));
#236004=CARTESIAN_POINT('Ctrl Pts',(-1.97053418125241,-7.66864170349043,
69.0665704858109));
#236005=CARTESIAN_POINT('Ctrl Pts',(-2.28610841791605,-7.58055139623021,
69.0541934288714));
#236006=CARTESIAN_POINT('Ctrl Pts',(-2.63689963190927,-7.45872780315692,
69.0394963005347));
#236007=CARTESIAN_POINT('Ctrl Pts',(-2.67837611881163,-7.44393453748252,
69.0377430158081));
#236008=CARTESIAN_POINT('Ctrl Pts',(-2.73131691926864,-7.42455259460387,
69.0354831449151));
#236009=CARTESIAN_POINT('Ctrl Pts',(-2.74289735383468,-7.4202821676794,
69.0349874612163));
#236010=CARTESIAN_POINT('Ctrl Pts',(-2.76149128906497,-7.41337595137857,
69.0341893427003));
#236011=CARTESIAN_POINT('Ctrl Pts',(-2.7685111439795,-7.41075726098834,
69.0338875130375));
#236012=CARTESIAN_POINT('Ctrl Pts',(-2.78184230787428,-7.40576261109921,
69.0333133298286));
#236013=CARTESIAN_POINT('Ctrl Pts',(-2.78815432213501,-7.40338854535371,
69.0330410447723));
#236014=CARTESIAN_POINT('Ctrl Pts',(-2.80249444477008,-7.39797401874605,
69.0324214739287));
#236015=CARTESIAN_POINT('Ctrl Pts',(-2.81052064815655,-7.39492855818234,
69.0320740048296));
#236016=CARTESIAN_POINT('Ctrl Pts',(-2.8348322985067,-7.3856584541668,69.0310193684614));
#236017=CARTESIAN_POINT('Ctrl Pts',(-2.85110208063233,-7.37939305649343,
69.0303106729056));
#236018=CARTESIAN_POINT('Ctrl Pts',(-2.96595560202251,-7.33472710653747,
69.0252864238742));
#236019=CARTESIAN_POINT('Ctrl Pts',(-3.06377951558409,-7.29440671601176,
69.0208947170862));
#236020=CARTESIAN_POINT('Ctrl Pts',(-3.93189530091721,-6.91604768375778,
68.9807317531754));
#236021=CARTESIAN_POINT('Ctrl Pts',(-4.64451042085152,-6.4591221896803,
68.940188298803));
#236022=CARTESIAN_POINT('Ctrl Pts',(-5.51179424836091,-5.68398191777587,
68.889063945931));
#236023=CARTESIAN_POINT('Ctrl Pts',(-5.7384876831185,-5.4550266989416,68.875406972553));
#236024=CARTESIAN_POINT('Ctrl Pts',(-5.96577117693623,-5.19557736253906,
68.8614291078675));
#236025=CARTESIAN_POINT('Ctrl Pts',(-5.98084945682748,-5.17821297862073,
68.8605002544851));
#236026=CARTESIAN_POINT('Ctrl Pts',(-6.00238416534003,-5.15319372810005,
68.8591714073106));
#236027=CARTESIAN_POINT('Ctrl Pts',(-6.00890204324818,-5.14559204594074,
68.8587689064738));
#236028=CARTESIAN_POINT('Ctrl Pts',(-6.02017523553975,-5.13239369770441,
68.858072222402));
#236029=CARTESIAN_POINT('Ctrl Pts',(-6.02493721449291,-5.12680275577525,
68.8577777679882));
#236030=CARTESIAN_POINT('Ctrl Pts',(-6.03406862283743,-5.11605146335431,
68.8572128151506));
#236031=CARTESIAN_POINT('Ctrl Pts',(-6.0384392334869,-5.11089212804968,
68.8569422688286));
#236032=CARTESIAN_POINT('Ctrl Pts',(-6.04870417595842,-5.0987432165907,
68.8563065236597));
#236033=CARTESIAN_POINT('Ctrl Pts',(-6.05459302189567,-5.0917490056895,
68.855941547384));
#236034=CARTESIAN_POINT('Ctrl Pts',(-6.07483120582013,-5.06762726285238,
68.8546863338634));
#236035=CARTESIAN_POINT('Ctrl Pts',(-6.08912015881404,-5.05044908461893,
68.8537985395635));
#236036=CARTESIAN_POINT('Ctrl Pts',(-6.24603173697941,-4.86017607374578,
68.8440316301716));
#236037=CARTESIAN_POINT('Ctrl Pts',(-6.38130966668222,-4.68114520520416,
68.8354525716006));
#236038=CARTESIAN_POINT('Ctrl Pts',(-6.95852273651041,-3.84563205055615,
68.7977957767436));
#236039=CARTESIAN_POINT('Ctrl Pts',(-7.30799760753928,-3.13096923991101,
68.7724221487529));
#236040=CARTESIAN_POINT('Ctrl Pts',(-7.60119969975605,-2.19997506153997,
68.7380424742427));
#236041=CARTESIAN_POINT('Ctrl Pts',(-7.65055087496772,-2.02168066318905,
68.7313765766411));
#236042=CARTESIAN_POINT('Ctrl Pts',(-7.72310567619308,-1.71860796796184,
68.7196855727966));
#236043=CARTESIAN_POINT('Ctrl Pts',(-7.74963866285949,-1.59470134302498,
68.7148062357184));
#236044=CARTESIAN_POINT('Ctrl Pts',(-7.77718748041658,-1.44904797793527,
68.7089031571398));
#236045=CARTESIAN_POINT('Ctrl Pts',(-7.78110480732217,-1.42786312669663,
68.7080404538159));
#236046=CARTESIAN_POINT('Ctrl Pts',(-7.78613365936787,-1.40003180079594,
68.7069014025436));
#236047=CARTESIAN_POINT('Ctrl Pts',(-7.78732332842077,-1.39339936230936,
68.7066295336714));
#236048=CARTESIAN_POINT('Ctrl Pts',(-7.7892500135189,-1.38257850158291,
68.70618527683));
#236049=CARTESIAN_POINT('Ctrl Pts',(-7.78999213058395,-1.37839097916684,
68.706013184408));
#236050=CARTESIAN_POINT('Ctrl Pts',(-7.79141470495349,-1.37032601706327,
68.7056814100224));
#236051=CARTESIAN_POINT('Ctrl Pts',(-7.79209564555216,-1.36644866279891,
68.7055217563068));
#236052=CARTESIAN_POINT('Ctrl Pts',(-7.79364838751152,-1.3575682680243,
68.7051557555815));
#236053=CARTESIAN_POINT('Ctrl Pts',(-7.79451826528301,-1.35256489768235,
68.7049492957716));
#236054=CARTESIAN_POINT('Ctrl Pts',(-7.79724410386461,-1.33679643801509,
68.7042978316842));
#236055=CARTESIAN_POINT('Ctrl Pts',(-7.79908255431624,-1.3260285221321,
68.7038517934315));
#236056=CARTESIAN_POINT('Ctrl Pts',(-7.81539748347536,-1.22926329773904,
68.6998329420114));
#236057=CARTESIAN_POINT('Ctrl Pts',(-7.82847281469493,-1.14303908846525,
68.6961775526228));
#236058=CARTESIAN_POINT('Ctrl Pts',(-7.88740909033609,-0.705731820042474,
68.6773319981908));
#236059=CARTESIAN_POINT('Ctrl Pts',(-7.91108580357871,-0.352087788226273,
68.6611133316053));
#236060=CARTESIAN_POINT('Ctrl Pts',(-7.91084325809914,0.645895155136899,
68.6148376959662));
#236061=CARTESIAN_POINT('Ctrl Pts',(-7.83205366977351,1.287551949809,68.5847248809791));
#236062=CARTESIAN_POINT('Ctrl Pts',(-7.63369955591107,2.08365798852378,
68.5497839632651));
#236063=CARTESIAN_POINT('Ctrl Pts',(-7.58537104474223,2.25325349927394,
68.5424652438616));
#236064=CARTESIAN_POINT('Ctrl Pts',(-7.52587968753853,2.43831558495546,
68.5346147344285));
#236065=CARTESIAN_POINT('Ctrl Pts',(-7.52028676259635,2.45551114384552,
68.5338865712244));
#236066=CARTESIAN_POINT('Ctrl Pts',(-7.51187300612227,2.48108101839664,
68.5328056859826));
#236067=CARTESIAN_POINT('Ctrl Pts',(-7.5090970412129,2.48946996492996,68.5324513744765));
#236068=CARTESIAN_POINT('Ctrl Pts',(-7.50431104024997,2.50385238634467,
68.531844444626));
#236069=CARTESIAN_POINT('Ctrl Pts',(-7.50230786784703,2.50984812642866,
68.5315915828493));
#236070=CARTESIAN_POINT('Ctrl Pts',(-7.49838886895656,2.52153155639669,
68.5310991515472));
#236071=CARTESIAN_POINT('Ctrl Pts',(-7.49647375244883,2.52721947980096,
68.5308595569587));
#236072=CARTESIAN_POINT('Ctrl Pts',(-7.49186518133804,2.54085566966443,
68.5302854864449));
#236073=CARTESIAN_POINT('Ctrl Pts',(-7.48916554563593,2.54880184793873,
68.5299512307098));
#236074=CARTESIAN_POINT('Ctrl Pts',(-7.48098809720297,2.57274640082559,
68.5289448143863));
#236075=CARTESIAN_POINT('Ctrl Pts',(-7.47547161086222,2.58873157232257,
68.5282740319635));
#236076=CARTESIAN_POINT('Ctrl Pts',(-7.42484094801648,2.73393306583911,
68.5221907492286));
#236077=CARTESIAN_POINT('Ctrl Pts',(-7.37643059836866,2.86197959399821,
68.5168973318535));
#236078=CARTESIAN_POINT('Ctrl Pts',(-7.18770085984096,3.32451778395482,
68.4979868977521));
#236079=CARTESIAN_POINT('Ctrl Pts',(-7.02774493570683,3.65051939847605,
68.4850943589469));
#236080=CARTESIAN_POINT('Ctrl Pts',(-6.46714848361543,4.61858929916125,
68.4465955539818));
#236081=CARTESIAN_POINT('Ctrl Pts',(-5.99659176041218,5.21496642466577,
68.4228305182593));
#236082=CARTESIAN_POINT('Ctrl Pts',(-5.41788882742592,5.76473850535748,
68.3915206899993));
#236083=CARTESIAN_POINT('Ctrl Pts',(-5.38682320073879,5.79377813267851,
68.3898335427166));
#236084=CARTESIAN_POINT('Ctrl Pts',(-5.34981284122671,5.82781981604779,
68.3878138226306));
#236085=CARTESIAN_POINT('Ctrl Pts',(-5.34409242871493,5.83306586256276,
68.3875013778873));
#236086=CARTESIAN_POINT('Ctrl Pts',(-5.33487166866519,5.84149704069829,
68.3869972913447));
#236087=CARTESIAN_POINT('Ctrl Pts',(-5.3313761754734,5.84468745724451,68.3868060917488));
#236088=CARTESIAN_POINT('Ctrl Pts',(-5.32512137080621,5.85038608050914,
68.3864637726194));
#236089=CARTESIAN_POINT('Ctrl Pts',(-5.32236315397001,5.85289546822741,
68.386312753173));
#236090=CARTESIAN_POINT('Ctrl Pts',(-5.31657188311358,5.85815680776679,
68.3859955319414));
#236091=CARTESIAN_POINT('Ctrl Pts',(-5.31353846519703,5.86090835548905,
68.3858292970307));
#236092=CARTESIAN_POINT('Ctrl Pts',(-5.30558421956702,5.86811222855474,
68.3853931962922));
#236093=CARTESIAN_POINT('Ctrl Pts',(-5.30065993322906,5.87256071144008,
68.3851230177142));
#236094=CARTESIAN_POINT('Ctrl Pts',(-5.27900601782652,5.892072917125,68.3839340940201));
#236095=CARTESIAN_POINT('Ctrl Pts',(-5.26221788567267,5.9070712455425,68.3830101099492));
#236096=CARTESIAN_POINT('Ctrl Pts',(-5.14075676246417,6.01465454940284,
68.3763107600704));
#236097=CARTESIAN_POINT('Ctrl Pts',(-5.03371623520933,6.10451848928488,
68.3703303829838));
#236098=CARTESIAN_POINT('Ctrl Pts',(-4.77474578021259,6.31048865462766,
68.3558044740933));
#236099=CARTESIAN_POINT('Ctrl Pts',(-4.6208761656869,6.42401436851056,68.3471303453423));
#236100=CARTESIAN_POINT('Ctrl Pts',(-4.33253868812151,6.62102837346934,
68.3310162513777));
#236101=CARTESIAN_POINT('Ctrl Pts',(-4.19938133625408,6.70627339560469,
68.3236257276589));
#236102=CARTESIAN_POINT('Ctrl Pts',(-3.52426352970285,7.11047675268893,
68.2866947621455));
#236103=CARTESIAN_POINT('Ctrl Pts',(-2.94809399222469,7.3680567226221,68.2570999017098));
#236104=CARTESIAN_POINT('Ctrl Pts',(-2.13510524297085,7.6206754193539,68.220337585186));
#236105=CARTESIAN_POINT('Ctrl Pts',(-1.92005578446264,7.67767967531091,
68.2110276529885));
#236106=CARTESIAN_POINT('Ctrl Pts',(-1.6817592873947,7.73020532118632,68.2011469955851));
#236107=CARTESIAN_POINT('Ctrl Pts',(-1.66062283922999,7.73477345526727,
68.2002742771485));
#236108=CARTESIAN_POINT('Ctrl Pts',(-1.63086435372124,7.7410774315269,68.1990506728259));
#236109=CARTESIAN_POINT('Ctrl Pts',(-1.6222578449535,7.74288562657803,68.1986973927864));
#236110=CARTESIAN_POINT('Ctrl Pts',(-1.60730074638774,7.74600202372101,
68.1980844725638));
#236111=CARTESIAN_POINT('Ctrl Pts',(-1.6009515384415,7.7473167750308,68.1978246161593));
#236112=CARTESIAN_POINT('Ctrl Pts',(-1.58772188685668,7.75003932455502,
68.1972838356279));
#236113=CARTESIAN_POINT('Ctrl Pts',(-1.58084116856165,7.75144576980837,
68.1970029563248));
#236114=CARTESIAN_POINT('Ctrl Pts',(-1.56460831498766,7.7547413142814,68.196341203234));
#236115=CARTESIAN_POINT('Ctrl Pts',(-1.55525460735049,7.75662266311267,
68.195960584998));
#236116=CARTESIAN_POINT('Ctrl Pts',(-1.52455636074935,7.7627393637063,68.1947136965083));
#236117=CARTESIAN_POINT('Ctrl Pts',(-1.50319766024456,7.7669035870237,68.1938497643134));
#236118=CARTESIAN_POINT('Ctrl Pts',(-1.09001668140545,7.84569167623016,
68.1772058223454));
#236119=CARTESIAN_POINT('Ctrl Pts',(-0.693102082096715,7.89066962607179,
68.1624523967294));
#236120=CARTESIAN_POINT('Ctrl Pts',(0.518826306966947,7.93581068196543,
68.1193688038403));
#236121=CARTESIAN_POINT('Ctrl Pts',(1.33185625649462,7.8404272380676,68.0934236979002));
#236122=CARTESIAN_POINT('Ctrl Pts',(2.15882597486057,7.61087176665246,68.0595964409431));
#236123=CARTESIAN_POINT('Ctrl Pts',(2.20157469328526,7.59861615004263,68.0578270142458));
#236124=CARTESIAN_POINT('Ctrl Pts',(2.25549151259314,7.58266557825635,68.0555706305791));
#236125=CARTESIAN_POINT('Ctrl Pts',(2.26675834935077,7.57930510130921,68.0550977520128));
#236126=CARTESIAN_POINT('Ctrl Pts',(2.2845453985948,7.57395667973757,68.0543490884008));
#236127=CARTESIAN_POINT('Ctrl Pts',(2.29107063191087,7.57198539512595,68.0540739861473));
#236128=CARTESIAN_POINT('Ctrl Pts',(2.3026149309014,7.56848155311092,68.0535864878864));
#236129=CARTESIAN_POINT('Ctrl Pts',(2.30763504028592,7.56695242884955,68.0533742304613));
#236130=CARTESIAN_POINT('Ctrl Pts',(2.3191571192757,7.5634302736231,68.0528864547944));
#236131=CARTESIAN_POINT('Ctrl Pts',(2.32565804258392,7.56143385320787,68.0526108015917));
#236132=CARTESIAN_POINT('Ctrl Pts',(2.34362876407849,7.55588971326031,68.0518475907835));
#236133=CARTESIAN_POINT('Ctrl Pts',(2.35509304675062,7.55232427017967,68.0513593383043));
#236134=CARTESIAN_POINT('Ctrl Pts',(2.41729797498816,7.53282284874805,68.0487027932394));
#236135=CARTESIAN_POINT('Ctrl Pts',(2.46788439207697,7.51640180130833,68.0465160422651));
#236136=CARTESIAN_POINT('Ctrl Pts',(3.22548813931363,7.26200069613366,68.0134002662275));
#236137=CARTESIAN_POINT('Ctrl Pts',(3.89554266051209,6.92569504630479,67.9796939332058));
#236138=CARTESIAN_POINT('Ctrl Pts',(4.63242835971799,6.4146120779616,67.9412275467244));
#236139=CARTESIAN_POINT('Ctrl Pts',(4.75380603533181,6.32518541293356,67.9348230245944));
#236140=CARTESIAN_POINT('Ctrl Pts',(5.05832033635982,6.08711073318702,67.918582951615));
#236141=CARTESIAN_POINT('Ctrl Pts',(5.23750254302279,5.93364103221607,67.9088616113184));
#236142=CARTESIAN_POINT('Ctrl Pts',(5.41567130776306,5.76667107307951,67.8989808521852));
#236143=CARTESIAN_POINT('Ctrl Pts',(5.42176614128831,5.76094114605455,67.8986425720489));
#236144=CARTESIAN_POINT('Ctrl Pts',(5.43678649319039,5.74677513561423,67.8978082089299));
#236145=CARTESIAN_POINT('Ctrl Pts',(5.44570149350094,5.73832789901608,67.8973123840569));
#236146=CARTESIAN_POINT('Ctrl Pts',(5.47090459495785,5.71433555745963,67.8959089413582));
#236147=CARTESIAN_POINT('Ctrl Pts',(5.48714609095306,5.6987415920491,67.8950024820675));
#236148=CARTESIAN_POINT('Ctrl Pts',(5.51380260885289,5.67292822845103,67.8935113786188));
#236149=CARTESIAN_POINT('Ctrl Pts',(5.52425629561685,5.66274900349271,67.8929257618603));
#236150=CARTESIAN_POINT('Ctrl Pts',(5.54374434100569,5.64366729638782,67.8918324270314));
#236151=CARTESIAN_POINT('Ctrl Pts',(5.55278556266505,5.63477190016757,67.8913245352481));
#236152=CARTESIAN_POINT('Ctrl Pts',(5.57288692944677,5.61489938408339,67.8901938796729));
#236153=CARTESIAN_POINT('Ctrl Pts',(5.5839361206637,5.60391124342665,67.8895713978223));
#236154=CARTESIAN_POINT('Ctrl Pts',(5.61610563523402,5.57172986683852,67.8877561524365));
#236155=CARTESIAN_POINT('Ctrl Pts',(5.63713834095591,5.55044931108714,67.886565656977));
#236156=CARTESIAN_POINT('Ctrl Pts',(5.79534439179082,5.38855210386681,67.8775827990193));
#236157=CARTESIAN_POINT('Ctrl Pts',(5.9273611497005,5.2429862098085,67.8699288770248));
#236158=CARTESIAN_POINT('Ctrl Pts',(6.21560181621193,4.90034377436125,67.8527884688161));
#236159=CARTESIAN_POINT('Ctrl Pts',(6.36812510144712,4.70043234225726,67.8433996656303));
#236160=CARTESIAN_POINT('Ctrl Pts',(6.86166339913433,3.9853326508953,67.8114045045014));
#236161=CARTESIAN_POINT('Ctrl Pts',(7.15169314247932,3.43779787194358,67.7897652418953));
#236162=CARTESIAN_POINT('Ctrl Pts',(7.40411086386661,2.78738218927188,67.7626460621131));
#236163=CARTESIAN_POINT('Ctrl Pts',(7.43199621842302,2.71215574210869,67.7594860116449));
#236164=CARTESIAN_POINT('Ctrl Pts',(7.46310073176604,2.62416087587781,67.7557492950604));
#236165=CARTESIAN_POINT('Ctrl Pts',(7.46743872021903,2.61179091655468,67.7552230818424));
#236166=CARTESIAN_POINT('Ctrl Pts',(7.47391137600378,2.59318591228022,67.7544301739916));
#236167=CARTESIAN_POINT('Ctrl Pts',(7.47606904369181,2.5869588488368,67.7541645440067));
#236168=CARTESIAN_POINT('Ctrl Pts',(7.47989447129947,2.57587384769939,67.753691239994));
#236169=CARTESIAN_POINT('Ctrl Pts',(7.48156528791305,2.57101696290537,67.7534837095705));
#236170=CARTESIAN_POINT('Ctrl Pts',(7.4850685414005,2.56080104803721,67.7530468652586));
#236171=CARTESIAN_POINT('Ctrl Pts',(7.48689995501814,2.5554416722729,67.7528175029956));
#236172=CARTESIAN_POINT('Ctrl Pts',(7.49170082834321,2.54134312707155,67.7522136272554));
#236173=CARTESIAN_POINT('Ctrl Pts',(7.49466074578937,2.53260073744806,67.7518386560696));
#236174=CARTESIAN_POINT('Ctrl Pts',(7.50776894091152,2.4936602502621,67.7501660925996));
#236175=CARTESIAN_POINT('Ctrl Pts',(7.51774999166424,2.46340637151654,67.7488603165306));
#236176=CARTESIAN_POINT('Ctrl Pts',(7.59199058480113,2.23371947549876,67.7388936186771));
#236177=CARTESIAN_POINT('Ctrl Pts',(7.64848278157567,2.03187680548405,67.7298350987098));
#236178=CARTESIAN_POINT('Ctrl Pts',(7.78404461885729,1.46110020072928,67.7037944316538));
#236179=CARTESIAN_POINT('Ctrl Pts',(7.84484058863892,1.08840438157273,67.6863213086827));
#236180=CARTESIAN_POINT('Ctrl Pts',(7.91970559817353,0.260905781299018,
67.6480283852549));
#236181=CARTESIAN_POINT('Ctrl Pts',(7.92163796314033,-0.19371067842184,
67.627348210896));
#236182=CARTESIAN_POINT('Ctrl Pts',(7.86449376201347,-0.891154691847469,
67.5970828419961));
#236183=CARTESIAN_POINT('Ctrl Pts',(7.83298589056546,-1.13523765259873,
67.5867576918236));
#236184=CARTESIAN_POINT('Ctrl Pts',(7.78606359973278,-1.40060215981521,
67.5758230196328));
#236185=CARTESIAN_POINT('Ctrl Pts',(7.78187043760458,-1.4237153133273,67.5748729991635));
#236186=CARTESIAN_POINT('Ctrl Pts',(7.77582802194223,-1.45619736074891,
67.5735411965354));
#236187=CARTESIAN_POINT('Ctrl Pts',(7.77406467610899,-1.46558199795021,
67.573156804087));
#236188=CARTESIAN_POINT('Ctrl Pts',(7.77097199400565,-1.48187881184072,
67.5724899616385));
#236189=CARTESIAN_POINT('Ctrl Pts',(7.76965041770098,-1.48879244075826,
67.5722072757499));
#236190=CARTESIAN_POINT('Ctrl Pts',(7.76697205574318,-1.50270319278436,
67.5716389104792));
#236191=CARTESIAN_POINT('Ctrl Pts',(7.76561503747972,-1.50970026505496,
67.5713532384681));
#236192=CARTESIAN_POINT('Ctrl Pts',(7.76236061450086,-1.52636026625445,
67.5706735620396));
#236193=CARTESIAN_POINT('Ctrl Pts',(7.76045461798794,-1.53602151513891,
67.570279819889));
#236194=CARTESIAN_POINT('Ctrl Pts',(7.75640532548546,-1.55634692269173,
67.5694523117242));
#236195=CARTESIAN_POINT('Ctrl Pts',(7.75425806357083,-1.5670102749158,67.5690186674246));
#236196=CARTESIAN_POINT('Ctrl Pts',(7.74847284088452,-1.59543674119386,
67.5678639559954));
#236197=CARTESIAN_POINT('Ctrl Pts',(7.744795783556,-1.61319187868022,67.5671440814746));
#236198=CARTESIAN_POINT('Ctrl Pts',(7.66177140262123,-2.00725835167057,
67.5511964517676));
#236199=CARTESIAN_POINT('Ctrl Pts',(7.5551464194602,-2.37731544702658,67.5368542951744));
#236200=CARTESIAN_POINT('Ctrl Pts',(7.27803714832115,-3.12843892931088,
67.5081715834628));
#236201=CARTESIAN_POINT('Ctrl Pts',(7.10349990748246,-3.50674368655629,
67.4939707732165));
#236202=CARTESIAN_POINT('Ctrl Pts',(6.65822959460662,-4.30072865049707,
67.4624694079441));
#236203=CARTESIAN_POINT('Ctrl Pts',(6.3765508535052,-4.70827814437532,67.4451175111969));
#236204=CARTESIAN_POINT('Ctrl Pts',(6.03842161946734,-5.11100567077535,
67.4242934243672));
#236205=CARTESIAN_POINT('Ctrl Pts',(6.01800884669077,-5.13502522921731,
67.4230373549509));
#236206=CARTESIAN_POINT('Ctrl Pts',(5.99052112417736,-5.16698080711528,
67.4213480677093));
#236207=CARTESIAN_POINT('Ctrl Pts',(5.983572767746,-5.17502569385177,67.4209212287185));
#236208=CARTESIAN_POINT('Ctrl Pts',(5.97268994167827,-5.1875747346744,67.4202530052911));
#236209=CARTESIAN_POINT('Ctrl Pts',(5.96876652872789,-5.19208849044048,
67.4200121640985));
#236210=CARTESIAN_POINT('Ctrl Pts',(5.96088997743894,-5.20112947349032,
67.4195287897648));
#236211=CARTESIAN_POINT('Ctrl Pts',(5.956936790921,-5.2056566532824,67.4192862543255));
#236212=CARTESIAN_POINT('Ctrl Pts',(5.94799858625355,-5.21586915012669,
67.41873803718));
#236213=CARTESIAN_POINT('Ctrl Pts',(5.94301057178462,-5.22155183029942,
67.4184322125625));
#236214=CARTESIAN_POINT('Ctrl Pts',(5.92821800532219,-5.2383558580165,67.4175256009208));
#236215=CARTESIAN_POINT('Ctrl Pts',(5.91839035565772,-5.2494567727006,67.4169237327513));
#236216=CARTESIAN_POINT('Ctrl Pts',(5.83934248656592,-5.3382419020652,67.4120866847747));
#236217=CARTESIAN_POINT('Ctrl Pts',(5.76862843463035,-5.41457960198394,
67.4077844279173));
#236218=CARTESIAN_POINT('Ctrl Pts',(5.49525043649536,-5.69826288487768,
67.3913073584511));
#236219=CARTESIAN_POINT('Ctrl Pts',(5.2827497805174,-5.8958056576766,67.3788221045699));
#236220=CARTESIAN_POINT('Ctrl Pts',(4.91033953277173,-6.20566977208771,
67.3578988476421));
#236221=CARTESIAN_POINT('Ctrl Pts',(4.75624558076615,-6.32454744690161,
67.3494844691928));
#236222=CARTESIAN_POINT('Ctrl Pts',(4.41520973029936,-6.56812451273447,
67.3314609039004));
#236223=CARTESIAN_POINT('Ctrl Pts',(4.22701782039174,-6.69078923241248,
67.321876788765));
#236224=CARTESIAN_POINT('Ctrl Pts',(3.87301218074517,-6.90062749869307,
67.3045099823536));
#236225=CARTESIAN_POINT('Ctrl Pts',(3.70883279735146,-6.99023925194473,
67.2966985582147));
#236226=CARTESIAN_POINT('Ctrl Pts',(3.3663107793293,-7.16172562026536,67.2808366552323));
#236227=CARTESIAN_POINT('Ctrl Pts',(3.18778794893457,-7.24295325504262,
67.2727987430975));
#236228=CARTESIAN_POINT('Ctrl Pts',(2.88571549354815,-7.36706174915327,
67.2594685839598));
#236229=CARTESIAN_POINT('Ctrl Pts',(2.76379140836478,-7.41366375249362,
67.2541562109715));
#236230=CARTESIAN_POINT('Ctrl Pts',(2.57474960784972,-7.48060764359384,
67.2460268532089));
#236231=CARTESIAN_POINT('Ctrl Pts',(2.50842154757325,-7.50310920089263,
67.2431944827879));
#236232=CARTESIAN_POINT('Ctrl Pts',(2.41174137160759,-7.53448229359034,
67.2390948005035));
#236233=CARTESIAN_POINT('Ctrl Pts',(2.38162131187042,-7.54405725129403,
67.237821590573));
#236234=CARTESIAN_POINT('Ctrl Pts',(2.32817880693739,-7.56069429348718,
67.2355695773614));
#236235=CARTESIAN_POINT('Ctrl Pts',(2.30487961443618,-7.56782959132862,
67.2345901390223));
#236236=CARTESIAN_POINT('Ctrl Pts',(2.25629547181174,-7.58246314034823,
67.2325526728384));
#236237=CARTESIAN_POINT('Ctrl Pts',(2.23100523278638,-7.58994283160633,
67.2314948249496));
#236238=CARTESIAN_POINT('Ctrl Pts',(2.16507175965,-7.60908490712997,67.2287440050897));
#236239=CARTESIAN_POINT('Ctrl Pts',(2.12437152213732,-7.62054817614524,
67.2270529135127));
#236240=CARTESIAN_POINT('Ctrl Pts',(1.94170960640497,-7.67041802224471,
67.2194937961042));
#236241=CARTESIAN_POINT('Ctrl Pts',(1.79878421685514,-7.70518818957733,
67.213661751069));
#236242=CARTESIAN_POINT('Ctrl Pts',(1.26644595277864,-7.81907259721831,
67.1922041651124));
#236243=CARTESIAN_POINT('Ctrl Pts',(0.872208364421169,-7.87280390998333,
67.1768562486777));
#236244=CARTESIAN_POINT('Ctrl Pts',(0.115187498727938,-7.91839769503541,
67.1475423368327));
#236245=CARTESIAN_POINT('Ctrl Pts',(-0.246280254805599,-7.91540411195282,
67.1336047765581));
#236246=CARTESIAN_POINT('Ctrl Pts',(-0.650359760800838,-7.88434581558507,
67.11745972163));
#236247=CARTESIAN_POINT('Ctrl Pts',(-0.694424185768638,-7.88058701861995,
67.1156913336023));
#236248=CARTESIAN_POINT('Ctrl Pts',(-0.754816962548265,-7.87492491628468,
67.1132553269076));
#236249=CARTESIAN_POINT('Ctrl Pts',(-0.771174579355153,-7.87333987894532,
67.1125942822825));
#236250=CARTESIAN_POINT('Ctrl Pts',(-0.797194739895476,-7.87073668378792,
67.1115406771385));
#236251=CARTESIAN_POINT('Ctrl Pts',(-0.806860579378988,-7.86975167357119,
67.111148832676));
#236252=CARTESIAN_POINT('Ctrl Pts',(-0.826660213310985,-7.86769710457302,
67.1103452112875));
#236253=CARTESIAN_POINT('Ctrl Pts',(-0.836793803397933,-7.86662576759878,
67.109933395696));
#236254=CARTESIAN_POINT('Ctrl Pts',(-0.860155655201863,-7.86411026888412,
67.1089827750946));
#236255=CARTESIAN_POINT('Ctrl Pts',(-0.87338238647685,-7.86265230553085,
67.1084436572655));
#236256=CARTESIAN_POINT('Ctrl Pts',(-0.916897752826008,-7.85774451182423,
67.1066668870606));
#236257=CARTESIAN_POINT('Ctrl Pts',(-0.947169944042841,-7.85415300164765,
67.1054258724911));
#236258=CARTESIAN_POINT('Ctrl Pts',(-1.01999709800712,-7.84508558242687,
67.1024290527674));
#236259=CARTESIAN_POINT('Ctrl Pts',(-1.06252967968555,-7.83943827748803,
67.1006695849004));
#236260=CARTESIAN_POINT('Ctrl Pts',(-1.17140803015429,-7.82407950639369,
67.0961439175717));
#236261=CARTESIAN_POINT('Ctrl Pts',(-1.23767983905098,-7.81387006290142,
67.0933686134213));
#236262=CARTESIAN_POINT('Ctrl Pts',(-1.65065436978689,-7.74486402374802,
67.0759636208372));
#236263=CARTESIAN_POINT('Ctrl Pts',(-1.99324281375658,-7.66384753182314,
67.0610552886069));
#236264=CARTESIAN_POINT('Ctrl Pts',(-2.60648305526845,-7.47491071474089,
67.0340408817409));
#236265=CARTESIAN_POINT('Ctrl Pts',(-2.87876478489771,-7.37433145914516,
67.0219181510309));
#236266=CARTESIAN_POINT('Ctrl Pts',(-3.28341458512829,-7.19902028550096,
67.0037632786462));
#236267=CARTESIAN_POINT('Ctrl Pts',(-3.42017267821847,-7.13506303561728,
66.9976002800569));
#236268=CARTESIAN_POINT('Ctrl Pts',(-3.58996201886375,-7.04965415284804,
66.9899047700633));
#236269=CARTESIAN_POINT('Ctrl Pts',(-3.62477425119955,-7.03181787458476,
66.9883245217964));
#236270=CARTESIAN_POINT('Ctrl Pts',(-3.67981942301247,-7.00309772379881,
66.9858216165665));
#236271=CARTESIAN_POINT('Ctrl Pts',(-3.70013961194555,-6.99238268199853,
66.9848967372731));
#236272=CARTESIAN_POINT('Ctrl Pts',(-3.73799612759249,-6.97220932820111,
66.9831718698131));
#236273=CARTESIAN_POINT('Ctrl Pts',(-3.75554394271261,-6.96277298662633,
66.9823715997999));
#236274=CARTESIAN_POINT('Ctrl Pts',(-3.79457688114165,-6.94159252744235,
66.980589778873));
#236275=CARTESIAN_POINT('Ctrl Pts',(-3.81604352203695,-6.9298147426119,
66.9796086773805));
#236276=CARTESIAN_POINT('Ctrl Pts',(-3.87886938903857,-6.89496455059312,
66.9767336664274));
#236277=CARTESIAN_POINT('Ctrl Pts',(-3.92007662618697,-6.87162012708803,
66.9748433019408));
#236278=CARTESIAN_POINT('Ctrl Pts',(-4.28352552292124,-6.66138841428367,
66.9581235603776));
#236279=CARTESIAN_POINT('Ctrl Pts',(-4.59241135603751,-6.45232162554097,
66.9435541900578));
#236280=CARTESIAN_POINT('Ctrl Pts',(-5.16438029798295,-6.00324015328831,
66.9153596901105));
#236281=CARTESIAN_POINT('Ctrl Pts',(-5.42830392819344,-5.76569536736933,
66.9018413220092));
#236282=CARTESIAN_POINT('Ctrl Pts',(-6.01510779270623,-5.16141238266864,
66.8701310419566));
#236283=CARTESIAN_POINT('Ctrl Pts',(-6.32173135975657,-4.78093977203577,
66.8521917083083));
#236284=CARTESIAN_POINT('Ctrl Pts',(-6.65037668706667,-4.28576695019923,
66.8294430839026));
#236285=CARTESIAN_POINT('Ctrl Pts',(-6.70758099838292,-4.19567215426284,
66.8253222176226));
#236286=CARTESIAN_POINT('Ctrl Pts',(-6.79020240723264,-4.0595359946907,
66.8190916298904));
#236287=CARTESIAN_POINT('Ctrl Pts',(-6.81701214001228,-4.01435257407538,
66.8170230632416));
#236288=CARTESIAN_POINT('Ctrl Pts',(-6.86182486254777,-3.937084424497,66.8134801002833));
#236289=CARTESIAN_POINT('Ctrl Pts',(-6.88005786729249,-3.90513481283901,
66.8120135391104));
#236290=CARTESIAN_POINT('Ctrl Pts',(-6.90394769607149,-3.8625861131279,
66.8100571457601));
#236291=CARTESIAN_POINT('Ctrl Pts',(-6.90980430047521,-3.85209940147315,
66.8095747006156));
#236292=CARTESIAN_POINT('Ctrl Pts',(-6.91888011065777,-3.83576115231996,
66.8088225906709));
#236293=CARTESIAN_POINT('Ctrl Pts',(-6.92211583982343,-3.82991878544161,
66.808553553146));
#236294=CARTESIAN_POINT('Ctrl Pts',(-6.92826774671569,-3.81877776385261,
66.8080403301961));
#236295=CARTESIAN_POINT('Ctrl Pts',(-6.93118525482455,-3.81347984693081,
66.8077961962578));
#236296=CARTESIAN_POINT('Ctrl Pts',(-6.93795838617441,-3.8011470357459,
66.8072276912746));
#236297=CARTESIAN_POINT('Ctrl Pts',(-6.94180938619317,-3.79410961898137,
66.806903140264));
#236298=CARTESIAN_POINT('Ctrl Pts',(-6.9527057334131,-3.77412522921682,
66.8059810556304));
#236299=CARTESIAN_POINT('Ctrl Pts',(-6.95972558992607,-3.76116444344953,
66.8053825113967));
#236300=CARTESIAN_POINT('Ctrl Pts',(-7.00273206607491,-3.68122877388018,
66.8016873501654));
#236301=CARTESIAN_POINT('Ctrl Pts',(-7.03778704183263,-3.61375907952109,
66.7985527768892));
#236302=CARTESIAN_POINT('Ctrl Pts',(-7.12631986249401,-3.43718604694469,
66.7902866330243));
#236303=CARTESIAN_POINT('Ctrl Pts',(-7.17826298639787,-3.32734414118199,
66.785076987381));
#236304=CARTESIAN_POINT('Ctrl Pts',(-7.40924686813812,-2.80828752368348,
66.760272536044));
#236305=CARTESIAN_POINT('Ctrl Pts',(-7.5559495747517,-2.38558591839174,
66.7395918553351));
#236306=CARTESIAN_POINT('Ctrl Pts',(-7.8204588902342,-1.34718028490491,
66.6905596538628));
#236307=CARTESIAN_POINT('Ctrl Pts',(-7.90244011495927,-0.725350257540262,
66.6627612647477));
#236308=CARTESIAN_POINT('Ctrl Pts',(-7.91067278101759,-0.0759547027280309,
66.6364173843223));
#236309=CARTESIAN_POINT('Ctrl Pts',(-7.91086896929252,-0.0516248923044945,
66.6354339224731));
#236310=CARTESIAN_POINT('Ctrl Pts',(-7.91098474343785,-0.0180691788099223,
66.6340823436002));
#236311=CARTESIAN_POINT('Ctrl Pts',(-7.91100043565217,-0.00884386686046784,
66.6337112621352));
#236312=CARTESIAN_POINT('Ctrl Pts',(-7.91099997657907,0.000676441821172982,
66.6333288303818));
#236313=CARTESIAN_POINT('Ctrl Pts',(-7.91099994585805,0.000971412062998885,
66.6333169819085));
#236314=CARTESIAN_POINT('Ctrl Pts',(-7.9109998986396,0.00126638231751385,
66.6333051339456));
#236315=CARTESIAN_POINT('',(-7.91295189375223,-0.00166598417887076,62.642331508237));
#236316=CARTESIAN_POINT('Ctrl Pts',(-7.91099989836148,0.00126811855402201,
66.6333050642068));
#236317=CARTESIAN_POINT('Ctrl Pts',(-7.91099928203754,0.00511297881132095,
66.6331506291295));
#236318=CARTESIAN_POINT('Ctrl Pts',(-7.91099586272661,0.00895784202195827,
66.6329962807285));
#236319=CARTESIAN_POINT('Ctrl Pts',(-7.91097834218039,0.0197840586746226,
66.6325619164758));
#236320=CARTESIAN_POINT('Ctrl Pts',(-7.91095780249242,0.0267654053171677,
66.6322820999343));
#236321=CARTESIAN_POINT('Ctrl Pts',(-7.91089836532715,0.0406987012629768,
66.6317242134853));
#236322=CARTESIAN_POINT('Ctrl Pts',(-7.91085954540913,0.047650644824675,
66.6314461414183));
#236323=CARTESIAN_POINT('Ctrl Pts',(-7.91073262647501,0.0660386498407756,
66.6307113806948));
#236324=CARTESIAN_POINT('Ctrl Pts',(-7.91062889268007,0.0774746058023487,
66.6302551764811));
#236325=CARTESIAN_POINT('Ctrl Pts',(-7.91015231993077,0.11987607945988,
66.6285665006553));
#236326=CARTESIAN_POINT('Ctrl Pts',(-7.90962245622959,0.150839737555361,
66.6273388995308));
#236327=CARTESIAN_POINT('Ctrl Pts',(-7.900197246448,0.56086867718257,66.6111548963665));
#236328=CARTESIAN_POINT('Ctrl Pts',(-7.86424286935362,0.938836404484335,
66.5970875613475));
#236329=CARTESIAN_POINT('Ctrl Pts',(-7.70243067570597,1.90040547374632,
66.5624471197628));
#236330=CARTESIAN_POINT('Ctrl Pts',(-7.53748570971118,2.4749239617006,66.5429463969361));
#236331=CARTESIAN_POINT('Ctrl Pts',(-7.25936725899302,3.14686696985364,
66.517503072867));
#236332=CARTESIAN_POINT('Ctrl Pts',(-7.20610266127692,3.26699670417725,
66.5128375697959));
#236333=CARTESIAN_POINT('Ctrl Pts',(-7.0557477649952,3.58451016725992,66.5000658262069));
#236334=CARTESIAN_POINT('Ctrl Pts',(-6.95338151991874,3.77925408040659,
66.4917655908));
#236335=CARTESIAN_POINT('Ctrl Pts',(-6.83680463494965,3.98022336468596,
66.4824551501055));
#236336=CARTESIAN_POINT('Ctrl Pts',(-6.83053945494455,3.99096559749898,
66.4819551777497));
#236337=CARTESIAN_POINT('Ctrl Pts',(-6.82150622353697,4.00637033272666,
66.4812348190924));
#236338=CARTESIAN_POINT('Ctrl Pts',(-6.81875864010727,4.01104487738425,
66.4810157790753));
#236339=CARTESIAN_POINT('Ctrl Pts',(-6.81398665178543,4.01914452824442,
66.4806354617301));
#236340=CARTESIAN_POINT('Ctrl Pts',(-6.8119644618798,4.02257094401138,66.4804743316456));
#236341=CARTESIAN_POINT('Ctrl Pts',(-6.80807525375481,4.02914950840103,
66.4801644986259));
#236342=CARTESIAN_POINT('Ctrl Pts',(-6.80620862838498,4.03230188957265,
66.4800158220113));
#236343=CARTESIAN_POINT('Ctrl Pts',(-6.80181285901613,4.03971377338867,
66.4796657618743));
#236344=CARTESIAN_POINT('Ctrl Pts',(-6.79928190530546,4.0439721947542,66.4794642562782));
#236345=CARTESIAN_POINT('Ctrl Pts',(-6.79050903273192,4.05870135320307,
66.4787659501721));
#236346=CARTESIAN_POINT('Ctrl Pts',(-6.78424703371935,4.06915983701979,
66.4782677726274));
#236347=CARTESIAN_POINT('Ctrl Pts',(-6.70459932645225,4.20148862680312,
66.4719347984187));
#236348=CARTESIAN_POINT('Ctrl Pts',(-6.62796735928221,4.32136586863604,
66.4658800091696));
#236349=CARTESIAN_POINT('Ctrl Pts',(-6.10163134736442,5.09776724849869,
66.4249191932295));
#236350=CARTESIAN_POINT('Ctrl Pts',(-5.5582836757307,5.68532501686529,66.3860779366209));
#236351=CARTESIAN_POINT('Ctrl Pts',(-4.68822999498538,6.38006278782248,
66.3368595153382));
#236352=CARTESIAN_POINT('Ctrl Pts',(-4.42844028077415,6.56305198266711,
66.3233670828882));
#236353=CARTESIAN_POINT('Ctrl Pts',(-4.13860033191449,6.74213958633559,
66.3095880541551));
#236354=CARTESIAN_POINT('Ctrl Pts',(-4.11881635283361,6.75424390834694,
66.3086535133726));
#236355=CARTESIAN_POINT('Ctrl Pts',(-4.09081125123776,6.77120930915872,
66.3073390191198));
#236356=CARTESIAN_POINT('Ctrl Pts',(-4.0826342200968,6.776142710088,66.306956213113));
#236357=CARTESIAN_POINT('Ctrl Pts',(-4.06913154967501,6.78425588433564,
66.3063257396477));
#236358=CARTESIAN_POINT('Ctrl Pts',(-4.06381108015922,6.78744421544092,
66.3060777354332));
#236359=CARTESIAN_POINT('Ctrl Pts',(-4.05276234629888,6.79404760358914,
66.3055635915211));
#236360=CARTESIAN_POINT('Ctrl Pts',(-4.04703350102776,6.79746168192765,
66.3052974903903));
#236361=CARTESIAN_POINT('Ctrl Pts',(-4.03336998583586,6.80558099321663,
66.3046639841671));
#236362=CARTESIAN_POINT('Ctrl Pts',(-4.02543138095227,6.81027960482649,
66.304296839007));
#236363=CARTESIAN_POINT('Ctrl Pts',(-3.99942013968801,6.82561347232907,
66.303096890346));
#236364=CARTESIAN_POINT('Ctrl Pts',(-3.98131335864025,6.83619080168214,
66.3022663543023));
#236365=CARTESIAN_POINT('Ctrl Pts',(-3.77014495245343,6.95842423393827,
66.2926352106638));
#236366=CARTESIAN_POINT('Ctrl Pts',(-3.57247956996298,7.06194452791223,
66.2841568519467));
#236367=CARTESIAN_POINT('Ctrl Pts',(-3.20557481006159,7.23474410184379,
66.2692402124052));
#236368=CARTESIAN_POINT('Ctrl Pts',(-3.03781151028347,7.30677338981285,
66.2627147438363));
#236369=CARTESIAN_POINT('Ctrl Pts',(-2.62643559355724,7.46677790479841,
66.2472545881585));
#236370=CARTESIAN_POINT('Ctrl Pts',(-2.38070502022569,7.54872072244702,
66.2384668475955));
#236371=CARTESIAN_POINT('Ctrl Pts',(-2.03806315190372,7.64458058863521,
66.22644987999));
#236372=CARTESIAN_POINT('Ctrl Pts',(-1.94425863543611,7.6689746459748,66.2231829139045));
#236373=CARTESIAN_POINT('Ctrl Pts',(-1.64561615009179,7.74080556166402,
66.212800418588));
#236374=CARTESIAN_POINT('Ctrl Pts',(-1.43932818698111,7.78180272575495,
66.2056576871965));
#236375=CARTESIAN_POINT('Ctrl Pts',(-1.02568775950608,7.84699707928779,
66.1910044271717));
#236376=CARTESIAN_POINT('Ctrl Pts',(-0.818525101462187,7.87130267727842,
66.1835025596205));
#236377=CARTESIAN_POINT('Ctrl Pts',(-0.537657481213367,7.89304797240223,
66.1728266623332));
#236378=CARTESIAN_POINT('Ctrl Pts',(-0.464585112626584,7.89768585935518,
66.1700030700877));
#236379=CARTESIAN_POINT('Ctrl Pts',(-0.37212503434688,7.90226668471457,
66.1663600701291));
#236380=CARTESIAN_POINT('Ctrl Pts',(-0.352785772343109,7.90315367330225,
66.1655942055975));
#236381=CARTESIAN_POINT('Ctrl Pts',(-0.312288023977738,7.9048621458896,
66.1639819344647));
#236382=CARTESIAN_POINT('Ctrl Pts',(-0.291129141340385,7.90566968455202,
66.1631347154703));
#236383=CARTESIAN_POINT('Ctrl Pts',(-0.263566195959512,7.90661083426472,
66.162024448216));
#236384=CARTESIAN_POINT('Ctrl Pts',(-0.257164659908958,7.90682163462554,
66.1617661215252));
#236385=CARTESIAN_POINT('Ctrl Pts',(-0.24673449880566,7.90715241608655,
66.1613444561081));
#236386=CARTESIAN_POINT('Ctrl Pts',(-0.242706034707053,7.90727709295163,
66.1611814090509));
#236387=CARTESIAN_POINT('Ctrl Pts',(-0.23493035481804,7.90751179462669,
66.1608663409477));
#236388=CARTESIAN_POINT('Ctrl Pts',(-0.23118315154687,7.90762223453531,
66.1607143453585));
#236389=CARTESIAN_POINT('Ctrl Pts',(-0.22257610304206,7.90786978365866,
66.1603648573397));
#236390=CARTESIAN_POINT('Ctrl Pts',(-0.217716211496125,7.9080050763785,
66.1601672545491));
#236391=CARTESIAN_POINT('Ctrl Pts',(-0.204782576827038,7.90835319943292,
66.1596406678069));
#236392=CARTESIAN_POINT('Ctrl Pts',(-0.196708648547469,7.908558145283,66.1593112093463));
#236393=CARTESIAN_POINT('Ctrl Pts',(-0.142664636460765,7.90984716841232,
66.157101096545));
#236394=CARTESIAN_POINT('Ctrl Pts',(-0.0966870669104941,7.91054276674534,
66.1551974468075));
#236395=CARTESIAN_POINT('Ctrl Pts',(0.784336770407963,7.916189966033,66.1183063194036));
#236396=CARTESIAN_POINT('Ctrl Pts',(1.61495909087095,7.78930491016547,66.0769702379401));
#236397=CARTESIAN_POINT('Ctrl Pts',(2.74337863430935,7.42832616514622,66.0228037514143));
#236398=CARTESIAN_POINT('Ctrl Pts',(3.06897096605148,7.2998365964352,66.0073414646339));
#236399=CARTESIAN_POINT('Ctrl Pts',(3.46645458437597,7.11166161473437,65.9888374481187));
#236400=CARTESIAN_POINT('Ctrl Pts',(3.54722350984455,7.07172146107949,65.9850960529864));
#236401=CARTESIAN_POINT('Ctrl Pts',(3.65807087227756,7.01453047736543,65.9799856604118));
#236402=CARTESIAN_POINT('Ctrl Pts',(3.6887429159825,6.9984495472949,65.9785741896009));
#236403=CARTESIAN_POINT('Ctrl Pts',(3.73428230750769,6.9741913136386,65.9764822545273));
#236404=CARTESIAN_POINT('Ctrl Pts',(3.74923033272093,6.96616686194565,65.9757961878894));
#236405=CARTESIAN_POINT('Ctrl Pts',(3.77306354010134,6.95327370148798,65.9747032491939));
#236406=CARTESIAN_POINT('Ctrl Pts',(3.7819653411453,6.94843592507324,65.9742952399416));
#236407=CARTESIAN_POINT('Ctrl Pts',(3.79877940121627,6.93925626531247,65.9735249624555));
#236408=CARTESIAN_POINT('Ctrl Pts',(3.80669356665319,6.93491791913281,65.9731625647043));
#236409=CARTESIAN_POINT('Ctrl Pts',(3.82062462348474,6.92725023175208,65.972524928024));
#236410=CARTESIAN_POINT('Ctrl Pts',(3.82664462262819,6.92392657523965,65.9722494799569));
#236411=CARTESIAN_POINT('Ctrl Pts',(3.83833922737884,6.91745004442073,65.9717145649138));
#236412=CARTESIAN_POINT('Ctrl Pts',(3.84401429917232,6.91429802724052,65.9714550666749));
#236413=CARTESIAN_POINT('Ctrl Pts',(3.85739474054517,6.90684477085534,65.9708434222208));
#236414=CARTESIAN_POINT('Ctrl Pts',(3.86509681365737,6.90253761270633,65.9704914948044));
#236415=CARTESIAN_POINT('Ctrl Pts',(3.89179799179613,6.88754705905246,65.9692719545442));
#236416=CARTESIAN_POINT('Ctrl Pts',(3.91076022011657,6.8767979910971,65.9684067691432));
#236417=CARTESIAN_POINT('Ctrl Pts',(4.13112974345136,6.75067143333191,65.9583618148099));
#236418=CARTESIAN_POINT('Ctrl Pts',(4.32741716910721,6.62655784617023,65.9495150714584));
#236419=CARTESIAN_POINT('Ctrl Pts',(4.91624813205686,6.21689834753972,65.9230084970337));
#236420=CARTESIAN_POINT('Ctrl Pts',(5.28820020181546,5.90375139299988,65.9063730017569));
#236421=CARTESIAN_POINT('Ctrl Pts',(5.65162805358483,5.53570661753152,65.8885165635819));
#236422=CARTESIAN_POINT('Ctrl Pts',(5.67399994904702,5.51277352929593,65.8874098645691));
#236423=CARTESIAN_POINT('Ctrl Pts',(5.75178649667698,5.43206059529895,65.8835334024997));
#236424=CARTESIAN_POINT('Ctrl Pts',(5.8064625906904,5.37357630103937,65.8807575013142));
#236425=CARTESIAN_POINT('Ctrl Pts',(5.92370363505261,5.24429034524188,65.8746704726075));
#236426=CARTESIAN_POINT('Ctrl Pts',(5.98590662511264,5.17317769427676,65.8713534892865));
#236427=CARTESIAN_POINT('Ctrl Pts',(6.14748598072484,4.98163735349226,65.8624553818891));
#236428=CARTESIAN_POINT('Ctrl Pts',(6.24459398723676,4.85935565593164,65.8568115363913));
#236429=CARTESIAN_POINT('Ctrl Pts',(6.42786497879458,4.61400190357871,65.8453985960173));
#236430=CARTESIAN_POINT('Ctrl Pts',(6.51425770860047,4.49120333136278,65.8396355619922));
#236431=CARTESIAN_POINT('Ctrl Pts',(6.61321598982625,4.3416755354502,65.8325103234027));
#236432=CARTESIAN_POINT('Ctrl Pts',(6.62918256095405,4.31725731520878,65.8313441141959));
#236433=CARTESIAN_POINT('Ctrl Pts',(6.65028531994971,4.2845910596706,65.8297809597431));
#236434=CARTESIAN_POINT('Ctrl Pts',(6.65554204018736,4.27642087913969,65.8293897476216));
#236435=CARTESIAN_POINT('Ctrl Pts',(6.66417745756557,4.26294491882118,65.8287440891936));
#236436=CARTESIAN_POINT('Ctrl Pts',(6.66756490942522,4.25764474153666,65.8284900486614));
#236437=CARTESIAN_POINT('Ctrl Pts',(6.67413739240925,4.24733402468319,65.8279956645578));
#236438=CARTESIAN_POINT('Ctrl Pts',(6.67732311226754,4.24232392729733,65.8277553525936));
#236439=CARTESIAN_POINT('Ctrl Pts',(6.68469547941161,4.23070072314486,65.827197649648));
#236440=CARTESIAN_POINT('Ctrl Pts',(6.68887795458565,4.22408498605188,65.8268800720807));
#236441=CARTESIAN_POINT('Ctrl Pts',(6.70013946230265,4.20621314231168,65.8260217988697));
#236442=CARTESIAN_POINT('Ctrl Pts',(6.70719992764468,4.19494540379365,65.8254802899347));
#236443=CARTESIAN_POINT('Ctrl Pts',(6.75873844780945,4.11223275967713,65.8215026515674));
#236444=CARTESIAN_POINT('Ctrl Pts',(6.80210144272694,4.04010136496564,65.8180196892364));
#236445=CARTESIAN_POINT('Ctrl Pts',(7.24065206580134,3.28352160419392,65.7814270655434));
#236446=CARTESIAN_POINT('Ctrl Pts',(7.53231534395515,2.54419596747898,65.7456725481299));
#236447=CARTESIAN_POINT('Ctrl Pts',(7.77155637413643,1.50442303144175,65.7003807247599));
#236448=CARTESIAN_POINT('Ctrl Pts',(7.81938947944227,1.23188340388941,65.6888851675731));
#236449=CARTESIAN_POINT('Ctrl Pts',(7.85982094405236,0.900249459188929,
65.6753002819525));
#236450=CARTESIAN_POINT('Ctrl Pts',(7.86616328224149,0.843035979820562,
65.6729705514301));
#236451=CARTESIAN_POINT('Ctrl Pts',(7.87391858335319,0.765341831523711,
65.6698247753664));
#236452=CARTESIAN_POINT('Ctrl Pts',(7.87587707093603,0.744917676290511,
65.6689995147185));
#236453=CARTESIAN_POINT('Ctrl Pts',(7.87899502240439,0.711014386863049,
65.6676324427726));
#236454=CARTESIAN_POINT('Ctrl Pts',(7.88019940390992,0.697539516696597,
65.6670898403142));
#236455=CARTESIAN_POINT('Ctrl Pts',(7.88247817201753,0.671284844822668,
65.6660340688051));
#236456=CARTESIAN_POINT('Ctrl Pts',(7.88355605841738,0.658505391141245,
65.6655208386094));
#236457=CARTESIAN_POINT('Ctrl Pts',(7.88599635894217,0.62870810953524,65.6643257163679));
#236458=CARTESIAN_POINT('Ctrl Pts',(7.8873347722423,0.611688363108186,65.6636442618971));
#236459=CARTESIAN_POINT('Ctrl Pts',(7.8914037080637,0.557711225864623,65.6614868090556));
#236460=CARTESIAN_POINT('Ctrl Pts',(7.89392965852056,0.520738773124853,
65.6600145891226));
#236461=CARTESIAN_POINT('Ctrl Pts',(7.92087864991314,0.0808532449232036,
65.6425642329164));
#236462=CARTESIAN_POINT('Ctrl Pts',(7.91469074364,-0.323351698443158,65.6272324544178));
#236463=CARTESIAN_POINT('Ctrl Pts',(7.81449491258237,-1.41154484888727,
65.5868366513968));
#236464=CARTESIAN_POINT('Ctrl Pts',(7.66193549870036,-2.0864613413608,65.5629317880082));
#236465=CARTESIAN_POINT('Ctrl Pts',(7.40816993040214,-2.77579159953614,
65.5339807770892));
#236466=CARTESIAN_POINT('Ctrl Pts',(7.3920456843472,-2.81845014259915,65.5321683622193));
#236467=CARTESIAN_POINT('Ctrl Pts',(7.37177970755783,-2.8706957080847,65.5299203969703));
#236468=CARTESIAN_POINT('Ctrl Pts',(7.3679864400656,-2.88041762990786,65.529500885432));
#236469=CARTESIAN_POINT('Ctrl Pts',(7.36200658283733,-2.89565454958236,
65.5288414607508));
#236470=CARTESIAN_POINT('Ctrl Pts',(7.35983299816663,-2.90117466469663,
65.5286021617375));
#236471=CARTESIAN_POINT('Ctrl Pts',(7.35596745099794,-2.9109594483682,65.5281772715641));
#236472=CARTESIAN_POINT('Ctrl Pts',(7.35427798244231,-2.91522510400344,
65.527991799937));
#236473=CARTESIAN_POINT('Ctrl Pts',(7.35038044619573,-2.92504085019539,
65.5275644477046));
#236474=CARTESIAN_POINT('Ctrl Pts',(7.34816980341883,-2.93058990972043,
65.5273224424164));
#236475=CARTESIAN_POINT('Ctrl Pts',(7.34211661805863,-2.94573444241638,
65.5266608170033));
#236476=CARTESIAN_POINT('Ctrl Pts',(7.33826156049309,-2.95532487328022,
65.5262405819904));
#236477=CARTESIAN_POINT('Ctrl Pts',(7.31939539675772,-3.00199471076699,
65.5241893624855));
#236478=CARTESIAN_POINT('Ctrl Pts',(7.30412229548273,-3.0389667149656,65.5225450339597));
#236479=CARTESIAN_POINT('Ctrl Pts',(7.03961936363086,-3.66574160539814,
65.4943238568259));
#236480=CARTESIAN_POINT('Ctrl Pts',(6.71998699924606,-4.22321951402725,
65.4642357622994));
#236481=CARTESIAN_POINT('Ctrl Pts',(6.11980284778448,-5.02625157361758,
65.4181668020994));
#236482=CARTESIAN_POINT('Ctrl Pts',(5.88320586771784,-5.30123688484211,
65.4017552329232));
#236483=CARTESIAN_POINT('Ctrl Pts',(5.45352556843373,-5.73629129457823,
65.3751420655827));
#236484=CARTESIAN_POINT('Ctrl Pts',(5.27019089291166,-5.90517408834029,
65.3646112288012));
#236485=CARTESIAN_POINT('Ctrl Pts',(5.05751703092292,-6.08327550843033,
65.3532774873575));
#236486=CARTESIAN_POINT('Ctrl Pts',(5.03575641648895,-6.10130123532264,
65.352127534126));
#236487=CARTESIAN_POINT('Ctrl Pts',(5.00235494679588,-6.12866941044458,
65.3503770989181));
#236488=CARTESIAN_POINT('Ctrl Pts',(4.99078356062493,-6.13809605743508,
65.3497733587277));
#236489=CARTESIAN_POINT('Ctrl Pts',(4.9717771332771,-6.15349039382,65.3487860422892));
#236490=CARTESIAN_POINT('Ctrl Pts',(4.9643578828676,-6.15947746983601,65.3484017188756));
#236491=CARTESIAN_POINT('Ctrl Pts',(4.95000934790789,-6.17101347108987,
65.3476605309133));
#236492=CARTESIAN_POINT('Ctrl Pts',(4.94308151263521,-6.17656417151403,
65.3473035983366));
#236493=CARTESIAN_POINT('Ctrl Pts',(4.93042689498891,-6.18666834109502,
65.3466533065276));
#236494=CARTESIAN_POINT('Ctrl Pts',(4.92470311532453,-6.19122554554482,
65.3463598042737));
#236495=CARTESIAN_POINT('Ctrl Pts',(4.91222316801581,-6.2011336725963,65.345721228352));
#236496=CARTESIAN_POINT('Ctrl Pts',(4.9054645580108,-6.20648151116878,65.3453762727331));
#236497=CARTESIAN_POINT('Ctrl Pts',(4.88722625516582,-6.22086440501052,
65.3444477358294));
#236498=CARTESIAN_POINT('Ctrl Pts',(4.87573022864699,-6.22987874320063,
65.3438649443551));
#236499=CARTESIAN_POINT('Ctrl Pts',(4.82261822988918,-6.27128820355819,
65.3411838167773));
#236500=CARTESIAN_POINT('Ctrl Pts',(4.78070351486427,-6.30329884715531,
65.3391000675235));
#236501=CARTESIAN_POINT('Ctrl Pts',(4.05126906247565,-6.84891292170329,
65.3033767281313));
#236502=CARTESIAN_POINT('Ctrl Pts',(3.2850770636264,-7.24766466795618,65.2747982818525));
#236503=CARTESIAN_POINT('Ctrl Pts',(2.27660726844952,-7.57907220430775,
65.237707518615));
#236504=CARTESIAN_POINT('Ctrl Pts',(2.08104168511736,-7.63508588872774,
65.2305004234966));
#236505=CARTESIAN_POINT('Ctrl Pts',(1.69202090815529,-7.73045089168454,
65.215825977187));
#236506=CARTESIAN_POINT('Ctrl Pts',(1.49881412551783,-7.77022281110548,
65.2083709582009));
#236507=CARTESIAN_POINT('Ctrl Pts',(1.26996042998991,-7.80847840608513,
65.1991945472144));
#236508=CARTESIAN_POINT('Ctrl Pts',(1.23556445814071,-7.81399481257133,
65.1978072648243));
#236509=CARTESIAN_POINT('Ctrl Pts',(1.19063388305767,-7.82089667498545,
65.1959854634914));
#236510=CARTESIAN_POINT('Ctrl Pts',(1.18013101345366,-7.82248839142609,
65.1955589176149));
#236511=CARTESIAN_POINT('Ctrl Pts',(1.16305265320631,-7.82504144953598,
65.1948642434667));
#236512=CARTESIAN_POINT('Ctrl Pts',(1.15647908122443,-7.82601567181203,
65.194596598369));
#236513=CARTESIAN_POINT('Ctrl Pts',(1.14385606947641,-7.82787018690325,
65.1940821575163));
#236514=CARTESIAN_POINT('Ctrl Pts',(1.13780681934505,-7.82875175313959,
65.1938354087939));
#236515=CARTESIAN_POINT('Ctrl Pts',(1.12400070550152,-7.83074739882598,
65.193271772735));
#236516=CARTESIAN_POINT('Ctrl Pts',(1.11624320215771,-7.83185696519682,
65.192954722555));
#236517=CARTESIAN_POINT('Ctrl Pts',(1.0920313312266,-7.83528331878388,65.1919641146372));
#236518=CARTESIAN_POINT('Ctrl Pts',(1.07557135900134,-7.83755978355911,
65.1912891340108));
#236519=CARTESIAN_POINT('Ctrl Pts',(0.943143109205395,-7.85544998778699,
65.185846842098));
#236520=CARTESIAN_POINT('Ctrl Pts',(0.826851201363329,-7.86854047155583,
65.1809955164232));
#236521=CARTESIAN_POINT('Ctrl Pts',(0.226765852880969,-7.92263960998303,
65.1557123925149));
#236522=CARTESIAN_POINT('Ctrl Pts',(-0.259767247274056,-7.92162645311127,
65.1344753582925));
#236523=CARTESIAN_POINT('Ctrl Pts',(-1.16466782515643,-7.83624542502699,
65.0954252437204));
#236524=CARTESIAN_POINT('Ctrl Pts',(-1.58234017973066,-7.76269407223206,
65.0775692808003));
#236525=CARTESIAN_POINT('Ctrl Pts',(-2.3004596274304,-7.5758371962115,65.0469227699631));
#236526=CARTESIAN_POINT('Ctrl Pts',(-2.60366799199404,-7.47705444288822,
65.0339376002999));
#236527=CARTESIAN_POINT('Ctrl Pts',(-2.95311059273801,-7.33936687585642,
65.0187334165742));
#236528=CARTESIAN_POINT('Ctrl Pts',(-3.00590153086049,-7.31790436822573,
65.0164312375924));
#236529=CARTESIAN_POINT('Ctrl Pts',(-3.08563336799752,-7.28448049730058,
65.0129461245992));
#236530=CARTESIAN_POINT('Ctrl Pts',(-3.11274677424793,-7.27293592184086,
65.0117595566524));
#236531=CARTESIAN_POINT('Ctrl Pts',(-3.15976184372643,-7.25260637999799,
65.009699503751));
#236532=CARTESIAN_POINT('Ctrl Pts',(-3.17969292700168,-7.24389032943898,
65.0088253922964));
#236533=CARTESIAN_POINT('Ctrl Pts',(-3.22440136764305,-7.22411883525122,
65.0068628137169));
#236534=CARTESIAN_POINT('Ctrl Pts',(-3.2491583299682,-7.21301790359976,
65.0057747927955));
#236535=CARTESIAN_POINT('Ctrl Pts',(-3.31551299794478,-7.1828537709395,
65.0028551647272));
#236536=CARTESIAN_POINT('Ctrl Pts',(-3.35700331006319,-7.16355662619601,
65.0010259001361));
#236537=CARTESIAN_POINT('Ctrl Pts',(-3.54766651296,-7.07285892776174,64.9926018252344));
#236538=CARTESIAN_POINT('Ctrl Pts',(-3.69474612390494,-6.99715109128936,
64.9860532675792));
#236539=CARTESIAN_POINT('Ctrl Pts',(-3.86041590981725,-6.9051930250294,
64.978600167615));
#236540=CARTESIAN_POINT('Ctrl Pts',(-3.88143212040733,-6.89340165722562,
64.9776532297877));
#236541=CARTESIAN_POINT('Ctrl Pts',(-4.46523745561113,-6.56233521067544,
64.951305526274));
#236542=CARTESIAN_POINT('Ctrl Pts',(-4.98678148426048,-6.17531866429517,
64.9268440402243));
#236543=CARTESIAN_POINT('Ctrl Pts',(-5.52640283470541,-5.66148555973626,
64.8974466264646));
#236544=CARTESIAN_POINT('Ctrl Pts',(-5.59619010341347,-5.59251310861638,
64.8935498954053));
#236545=CARTESIAN_POINT('Ctrl Pts',(-5.67933048548015,-5.50722861263397,
64.8887747536335));
#236546=CARTESIAN_POINT('Ctrl Pts',(-5.69392548568271,-5.49213749944513,
64.8879313871));
#236547=CARTESIAN_POINT('Ctrl Pts',(-5.71662920404554,-5.4684742633342,
64.8866112483937));
#236548=CARTESIAN_POINT('Ctrl Pts',(-5.72477914102156,-5.45994175891446,
64.8861356913924));
#236549=CARTESIAN_POINT('Ctrl Pts',(-5.73985646487481,-5.44408581706135,
64.8852527715162));
#236550=CARTESIAN_POINT('Ctrl Pts',(-5.74678900610458,-5.43676730599287,
64.8848455656542));
#236551=CARTESIAN_POINT('Ctrl Pts',(-5.7620538604238,-5.42059076131024,
64.8839461601382));
#236552=CARTESIAN_POINT('Ctrl Pts',(-5.77037976917114,-5.41172673093397,
64.8834537642825));
#236553=CARTESIAN_POINT('Ctrl Pts',(-5.79426869206136,-5.38617600687318,
64.8820356093829));
#236554=CARTESIAN_POINT('Ctrl Pts',(-5.8097798774938,-5.36944125715782,
64.8811081784051));
#236555=CARTESIAN_POINT('Ctrl Pts',(-5.92998476284706,-5.23862361500082,
64.8738699495423));
#236556=CARTESIAN_POINT('Ctrl Pts',(-6.03137917850009,-5.12155835328291,
64.8674622120488));
#236557=CARTESIAN_POINT('Ctrl Pts',(-6.20399539181202,-4.91002356757783,
64.8560679488168));
#236558=CARTESIAN_POINT('Ctrl Pts',(-6.2766579606571,-4.81678883532281,
64.8511052233825));
#236559=CARTESIAN_POINT('Ctrl Pts',(-6.55468348287408,-4.44307031719229,
64.8314950433296));
#236560=CARTESIAN_POINT('Ctrl Pts',(-6.74355947346076,-4.15080245219404,
64.8167854207848));
#236561=CARTESIAN_POINT('Ctrl Pts',(-7.00393904565052,-3.68293868639049,
64.7944465436555));
#236562=CARTESIAN_POINT('Ctrl Pts',(-7.08940470736722,-3.51561412131933,
64.7866736813764));
#236563=CARTESIAN_POINT('Ctrl Pts',(-7.20087746185788,-3.2767401758236,
64.7758745818195));
#236564=CARTESIAN_POINT('Ctrl Pts',(-7.23193200219774,-3.20761937840966,
64.7727834161222));
#236565=CARTESIAN_POINT('Ctrl Pts',(-7.28481692959007,-3.08523502747364,
64.7673673641284));
#236566=CARTESIAN_POINT('Ctrl Pts',(-7.3070678769772,-3.03215962371616,
64.7650371399895));
#236567=CARTESIAN_POINT('Ctrl Pts',(-7.33871275733246,-2.95430496410741,
64.7616451002709));
#236568=CARTESIAN_POINT('Ctrl Pts',(-7.34856437555683,-2.92971404416638,
64.7605774682573));
#236569=CARTESIAN_POINT('Ctrl Pts',(-7.3656892497325,-2.88633827197494,
64.758700762772));
#236570=CARTESIAN_POINT('Ctrl Pts',(-7.37301461314857,-2.86757428170369,
64.7578910411445));
#236571=CARTESIAN_POINT('Ctrl Pts',(-7.38716037181644,-2.83092722492057,
64.7563136796715));
#236572=CARTESIAN_POINT('Ctrl Pts',(-7.39398769174374,-2.81304698299139,
64.7555459589759));
#236573=CARTESIAN_POINT('Ctrl Pts',(-7.41026741896729,-2.76994284460643,
64.7536996437646));
#236574=CARTESIAN_POINT('Ctrl Pts',(-7.41965602483305,-2.74469507646945,
64.7526218331671));
#236575=CARTESIAN_POINT('Ctrl Pts',(-7.45400825882142,-2.65085089625082,
64.7486288216142));
#236576=CARTESIAN_POINT('Ctrl Pts',(-7.47815115241558,-2.58195760249436,
64.7457234382332));
#236577=CARTESIAN_POINT('Ctrl Pts',(-7.77295151158238,-1.70188357189728,
64.7089081060041));
#236578=CARTESIAN_POINT('Ctrl Pts',(-7.91131782727057,-0.852277164320057,
64.6763923099968));
#236579=CARTESIAN_POINT('Ctrl Pts',(-7.91088452321688,0.311667010540729,
64.6328655054235));
#236580=CARTESIAN_POINT('Ctrl Pts',(-7.89269817734012,0.620111447589521,
64.6213625335678));
#236581=CARTESIAN_POINT('Ctrl Pts',(-7.83374141446319,1.11994740556406,
64.6021363242674));
#236582=CARTESIAN_POINT('Ctrl Pts',(-7.8038251575381,1.31228593576899,64.5945909225753));
#236583=CARTESIAN_POINT('Ctrl Pts',(-7.76339308421455,1.52117708106424,
64.5860954253086));
#236584=CARTESIAN_POINT('Ctrl Pts',(-7.75987480568725,1.53902400439993,
64.5853671660829));
#236585=CARTESIAN_POINT('Ctrl Pts',(-7.75453739664275,1.56561506436483,
64.5842782962087));
#236586=CARTESIAN_POINT('Ctrl Pts',(-7.75276494974449,1.5743685715218,64.583919236688));
#236587=CARTESIAN_POINT('Ctrl Pts',(-7.74969348264725,1.58940652656909,
64.5833013162439));
#236588=CARTESIAN_POINT('Ctrl Pts',(-7.7484016299389,1.59569243984903,64.5830426990774));
#236589=CARTESIAN_POINT('Ctrl Pts',(-7.74572574363282,1.60863292998275,
64.5825096185403));
#236590=CARTESIAN_POINT('Ctrl Pts',(-7.74434077983235,1.61528730710124,
64.5822351232398));
#236591=CARTESIAN_POINT('Ctrl Pts',(-7.7411066582929,1.63072661701824,64.5815973743376));
#236592=CARTESIAN_POINT('Ctrl Pts',(-7.73925112113987,1.6395101944426,64.5812338968571));
#236593=CARTESIAN_POINT('Ctrl Pts',(-7.7333282067922,1.66731344925635,64.580081236042));
#236594=CARTESIAN_POINT('Ctrl Pts',(-7.72920565433316,1.68632121403199,
64.5792900717738));
#236595=CARTESIAN_POINT('Ctrl Pts',(-7.61964723618212,2.1826171870924,64.5585467086464));
#236596=CARTESIAN_POINT('Ctrl Pts',(-7.47029854184898,2.64900880987656,
64.5365118008296));
#236597=CARTESIAN_POINT('Ctrl Pts',(-6.98700272257376,3.7843477583362,64.4800097007572));
#236598=CARTESIAN_POINT('Ctrl Pts',(-6.59953943876348,4.425600854941,64.4459557794708));
#236599=CARTESIAN_POINT('Ctrl Pts',(-6.09867470119871,5.0390709755064,64.4135720494977));
#236600=CARTESIAN_POINT('Ctrl Pts',(-6.06904562698734,5.07471720188722,
64.4116892524954));
#236601=CARTESIAN_POINT('Ctrl Pts',(-6.03023008971474,5.12058930394145,
64.4092646601659));
#236602=CARTESIAN_POINT('Ctrl Pts',(-6.02132819513371,5.13105413375027,
64.4087114214991));
#236603=CARTESIAN_POINT('Ctrl Pts',(-6.00710868876948,5.14768224173842,
64.407832158859));
#236604=CARTESIAN_POINT('Ctrl Pts',(-6.00180876674147,5.1538605713166,64.4075054178816));
#236605=CARTESIAN_POINT('Ctrl Pts',(-5.99227266719119,5.1649425236226,64.4069192695422));
#236606=CARTESIAN_POINT('Ctrl Pts',(-5.98803998670627,5.16984913785188,
64.4066597201374));
#236607=CARTESIAN_POINT('Ctrl Pts',(-5.97813586475046,5.18130172807505,
64.4060538353673));
#236608=CARTESIAN_POINT('Ctrl Pts',(-5.97245968736258,5.18784360772507,
64.4057076940662));
#236609=CARTESIAN_POINT('Ctrl Pts',(-5.95619543940933,5.20652632700762,
64.4047190088754));
#236610=CARTESIAN_POINT('Ctrl Pts',(-5.94558098562208,5.21864419687512,
64.404077549144));
#236611=CARTESIAN_POINT('Ctrl Pts',(-5.87742621538128,5.29597447208053,
64.3999827998908));
#236612=CARTESIAN_POINT('Ctrl Pts',(-5.81884984861185,5.36026786319395,
64.3965726682081));
#236613=CARTESIAN_POINT('Ctrl Pts',(-5.64343061171831,5.54654298153605,
64.3866675365612));
#236614=CARTESIAN_POINT('Ctrl Pts',(-5.52372580413826,5.66576608137955,
64.380296229468));
#236615=CARTESIAN_POINT('Ctrl Pts',(-5.14903647954631,6.01577594695166,
64.3613944307476));
#236616=CARTESIAN_POINT('Ctrl Pts',(-4.88273942192422,6.23386005454693,
64.3493547610119));
#236617=CARTESIAN_POINT('Ctrl Pts',(-4.49141430599195,6.513829352766,64.3328450612914));
#236618=CARTESIAN_POINT('Ctrl Pts',(-4.37767901909459,6.59080435594572,
64.328172106331));
#236619=CARTESIAN_POINT('Ctrl Pts',(-4.13509885122626,6.74592966002602,
64.3183782047864));
#236620=CARTESIAN_POINT('Ctrl Pts',(-4.00590909727489,6.82343764363281,
64.3132598398298));
#236621=CARTESIAN_POINT('Ctrl Pts',(-3.52795224875502,7.09193536610502,
64.2944501692724));
#236622=CARTESIAN_POINT('Ctrl Pts',(-3.16715975809274,7.26023678687777,
64.2805024216922));
#236623=CARTESIAN_POINT('Ctrl Pts',(-2.73330756054947,7.42410534870174,
64.2625000156496));
#236624=CARTESIAN_POINT('Ctrl Pts',(-2.67103830963621,7.44673514644921,
64.259887416779));
#236625=CARTESIAN_POINT('Ctrl Pts',(-2.5986505932255,7.47201745195604,64.2568098429536));
#236626=CARTESIAN_POINT('Ctrl Pts',(-2.58880062590436,7.47543584183412,
64.2563902086264));
#236627=CARTESIAN_POINT('Ctrl Pts',(-2.57417535563201,7.48047910779384,
64.2557658200017));
#236628=CARTESIAN_POINT('Ctrl Pts',(-2.5694051764208,7.48211891664661,64.2555619622406));
#236629=CARTESIAN_POINT('Ctrl Pts',(-2.56092520692506,7.4850249465483,64.2551991904726));
#236630=CARTESIAN_POINT('Ctrl Pts',(-2.55721603360747,7.4862929760509,64.2550403859401));
#236631=CARTESIAN_POINT('Ctrl Pts',(-2.54942625954005,7.48894954760442,
64.2547066059428));
#236632=CARTESIAN_POINT('Ctrl Pts',(-2.54534546472459,7.49033751205245,
64.2545315954107));
#236633=CARTESIAN_POINT('Ctrl Pts',(-2.53463841993553,7.49396944368319,
64.2540719988585));
#236634=CARTESIAN_POINT('Ctrl Pts',(-2.52801033725516,7.49620795314431,
64.2537870787175));
#236635=CARTESIAN_POINT('Ctrl Pts',(-2.49789626663681,7.50633392847157,
64.2524906681492));
#236636=CARTESIAN_POINT('Ctrl Pts',(-2.47437673242937,7.51411967858739,
64.2514728550875));
#236637=CARTESIAN_POINT('Ctrl Pts',(-1.96485324271369,7.68013738295354,
64.229315268551));
#236638=CARTESIAN_POINT('Ctrl Pts',(-1.46472098892859,7.7909991326682,64.2055252919042));
#236639=CARTESIAN_POINT('Ctrl Pts',(-0.739842015891198,7.87937876971255,
64.1715611967195));
#236640=CARTESIAN_POINT('Ctrl Pts',(-0.521225950115917,7.8968540061067,
64.161371288666));
#236641=CARTESIAN_POINT('Ctrl Pts',(0.193036051719969,7.92415537853956,
64.1286366094361));
#236642=CARTESIAN_POINT('Ctrl Pts',(0.688967922225117,7.89651497230842,
64.1068719336869));
#236643=CARTESIAN_POINT('Ctrl Pts',(1.21106283397772,7.81781884766206,64.0854307964007));
#236644=CARTESIAN_POINT('Ctrl Pts',(1.24297912746055,7.81280792329007,64.0841255360625));
#236645=CARTESIAN_POINT('Ctrl Pts',(1.28601085931369,7.80578148763414,64.0823729608116));
#236646=CARTESIAN_POINT('Ctrl Pts',(1.2971537384086,7.80393751534287,64.081919797525));
#236647=CARTESIAN_POINT('Ctrl Pts',(1.31466232940341,7.80100158140838,64.0812087793723));
#236648=CARTESIAN_POINT('Ctrl Pts',(1.32103069581015,7.79992568006176,64.0809503761468));
#236649=CARTESIAN_POINT('Ctrl Pts',(1.333271633079,7.79784221784928,64.0804540970928));
#236650=CARTESIAN_POINT('Ctrl Pts',(1.33914439562785,7.79683581909488,64.0802161817315));
#236651=CARTESIAN_POINT('Ctrl Pts',(1.35296391955941,7.79445153181023,64.0796567555466));
#236652=CARTESIAN_POINT('Ctrl Pts',(1.36090972923312,7.79306812229849,64.0793354338041));
#236653=CARTESIAN_POINT('Ctrl Pts',(1.3839543322968,7.78901960978687,64.0784044862969));
#236654=CARTESIAN_POINT('Ctrl Pts',(1.39904755217002,7.78632275377439,64.0777959478075));
#236655=CARTESIAN_POINT('Ctrl Pts',(1.50368860764358,7.76731140934583,64.0735851390602));
#236656=CARTESIAN_POINT('Ctrl Pts',(1.59295865842962,7.74949607460564,64.0700345685605));
#236657=CARTESIAN_POINT('Ctrl Pts',(1.86265693665639,7.69081586198631,64.0594233756925));
#236658=CARTESIAN_POINT('Ctrl Pts',(2.04198101920279,7.64515914530808,64.0525275766075));
#236659=CARTESIAN_POINT('Ctrl Pts',(2.72267036632174,7.4461901613614,64.0267759468229));
#236660=CARTESIAN_POINT('Ctrl Pts',(3.20994556004413,7.24947889792212,64.0093433961322));
#236661=CARTESIAN_POINT('Ctrl Pts',(4.09201404819325,6.78689572801275,63.97560782675));
#236662=CARTESIAN_POINT('Ctrl Pts',(4.48937105846307,6.5308479562568,63.9593846957629));
#236663=CARTESIAN_POINT('Ctrl Pts',(4.88486812349987,6.22276963296857,63.9395619379357));
#236664=CARTESIAN_POINT('Ctrl Pts',(4.90813447434176,6.20443506084648,63.9383810993536));
#236665=CARTESIAN_POINT('Ctrl Pts',(4.93716121914123,6.18129568449885,63.9368886015499));
#236666=CARTESIAN_POINT('Ctrl Pts',(4.943018773897,6.17661255407107,63.9365864259829));
#236667=CARTESIAN_POINT('Ctrl Pts',(4.95223049162175,6.16922626553811,63.9361096388008));
#236668=CARTESIAN_POINT('Ctrl Pts',(4.95558912758511,6.16652867956016,63.9359354682787));
#236669=CARTESIAN_POINT('Ctrl Pts',(4.96180051683923,6.16153147015002,63.9356127495189));
#236670=CARTESIAN_POINT('Ctrl Pts',(4.96465388512767,6.15923260052334,63.9354642607764));
#236671=CARTESIAN_POINT('Ctrl Pts',(4.97098192222929,6.15412704449034,63.935134421878));
#236672=CARTESIAN_POINT('Ctrl Pts',(4.97445581093696,6.15131939796065,63.9349529964619));
#236673=CARTESIAN_POINT('Ctrl Pts',(4.98439031213249,6.14327627298296,63.9344331523627));
#236674=CARTESIAN_POINT('Ctrl Pts',(4.99084503241679,6.1380335622422,63.934094170832));
#236675=CARTESIAN_POINT('Ctrl Pts',(5.03207959109769,6.10443361509594,63.9319208897339));
#236676=CARTESIAN_POINT('Ctrl Pts',(5.06662521464639,6.07579159826939,63.9300647209231));
#236677=CARTESIAN_POINT('Ctrl Pts',(5.17021671041445,5.98840531852886,63.9243960563845));
#236678=CARTESIAN_POINT('Ctrl Pts',(5.23849654846711,5.92876815388919,63.9205200854795));
#236679=CARTESIAN_POINT('Ctrl Pts',(5.43622834644156,5.74998200376512,63.9089196701358));
#236680=CARTESIAN_POINT('Ctrl Pts',(5.56274431072916,5.62767635967614,63.9010089206926));
#236681=CARTESIAN_POINT('Ctrl Pts',(5.98025080605423,5.19622005337958,63.8735075503733));
#236682=CARTESIAN_POINT('Ctrl Pts',(6.25039723339212,4.86791909241502,63.8532886931837));
#236683=CARTESIAN_POINT('Ctrl Pts',(6.69776412054272,4.22521799154917,63.816774740303));
#236684=CARTESIAN_POINT('Ctrl Pts',(6.88239357752927,3.91729600835116,63.8003939042679));
#236685=CARTESIAN_POINT('Ctrl Pts',(7.16526266729727,3.36337188954451,63.773238266434));
#236686=CARTESIAN_POINT('Ctrl Pts',(7.27324335869973,3.12301282987252,63.7621409097484));
#236687=CARTESIAN_POINT('Ctrl Pts',(7.37725852280909,2.85665677018606,63.7505574922953));
#236688=CARTESIAN_POINT('Ctrl Pts',(7.38538498199774,2.83558105053327,63.7496456210783));
#236689=CARTESIAN_POINT('Ctrl Pts',(7.39660898458209,2.80609636703977,63.7483763903276));
#236690=CARTESIAN_POINT('Ctrl Pts',(7.39978263573776,2.79771661117309,63.7480163932658));
#236691=CARTESIAN_POINT('Ctrl Pts',(7.40524330114572,2.78322389486852,63.7473950327189));
#236692=CARTESIAN_POINT('Ctrl Pts',(7.40753699731173,2.77711347119247,63.7471334383312));
#236693=CARTESIAN_POINT('Ctrl Pts',(7.41227289254228,2.76444939922472,63.7465920669997));
#236694=CARTESIAN_POINT('Ctrl Pts',(7.41471396852983,2.75789533514638,63.7463123289699));
#236695=CARTESIAN_POINT('Ctrl Pts',(7.42040503433178,2.74255317526491,63.7456585240878));
#236696=CARTESIAN_POINT('Ctrl Pts',(7.42364811224973,2.73376251693251,63.7452846954732));
#236697=CARTESIAN_POINT('Ctrl Pts',(7.43404694913998,2.70542056150309,63.7440819492995));
#236698=CARTESIAN_POINT('Ctrl Pts',(7.44114117546848,2.68584669556688,63.7432551448048));
#236699=CARTESIAN_POINT('Ctrl Pts',(7.60519834971592,2.22755280643899,63.7239856024463));
#236700=CARTESIAN_POINT('Ctrl Pts',(7.72318299393176,1.7758206661223,63.7069714200375));
#236701=CARTESIAN_POINT('Ctrl Pts',(7.88627796430435,0.809277563742729,
63.6725580291106));
#236702=CARTESIAN_POINT('Ctrl Pts',(7.92219366569465,0.295151974411452,
63.6553774165823));
#236703=CARTESIAN_POINT('Ctrl Pts',(7.90394648209241,-0.36435426003187,
63.631617934523));
#236704=CARTESIAN_POINT('Ctrl Pts',(7.89590136726839,-0.509767217034449,
63.6262657892029));
#236705=CARTESIAN_POINT('Ctrl Pts',(7.8736856866521,-0.777217438749315,
63.6160892520921));
#236706=CARTESIAN_POINT('Ctrl Pts',(7.86067791206208,-0.899295806154468,
63.6113060764793));
#236707=CARTESIAN_POINT('Ctrl Pts',(7.84261612746838,-1.03806969694013,
63.6057094774505));
#236708=CARTESIAN_POINT('Ctrl Pts',(7.84034227950658,-1.0551063228355,63.6050198106969));
#236709=CARTESIAN_POINT('Ctrl Pts',(7.83703858600898,-1.07925849102365,
63.6040385156898));
#236710=CARTESIAN_POINT('Ctrl Pts',(7.83605452272862,-1.08638032265145,
63.6037487159174));
#236711=CARTESIAN_POINT('Ctrl Pts',(7.83423431804553,-1.09942230161413,
63.6032172152205));
#236712=CARTESIAN_POINT('Ctrl Pts',(7.83340117040299,-1.10534286562151,
63.6029756320097));
#236713=CARTESIAN_POINT('Ctrl Pts',(7.83170255168003,-1.11731531648677,
63.6024865023705));
#236714=CARTESIAN_POINT('Ctrl Pts',(7.83083677554566,-1.12336715678453,
63.6022389442311));
#236715=CARTESIAN_POINT('Ctrl Pts',(7.82871998363456,-1.13804232999326,
63.6016378874268));
#236716=CARTESIAN_POINT('Ctrl Pts',(7.82746173544444,-1.14666460066037,
63.6012841130634));
#236717=CARTESIAN_POINT('Ctrl Pts',(7.82296046374832,-1.17715734632519,
63.6000307959122));
#236718=CARTESIAN_POINT('Ctrl Pts',(7.81964001966288,-1.1990161743014,63.5991283633749));
#236719=CARTESIAN_POINT('Ctrl Pts',(7.75138199030471,-1.63601962491467,
63.5810101149756));
#236720=CARTESIAN_POINT('Ctrl Pts',(7.65356508486526,-2.04533395711269,
63.5626869635745));
#236721=CARTESIAN_POINT('Ctrl Pts',(7.35580361962639,-2.96163149438161,
63.5204903009965));
#236722=CARTESIAN_POINT('Ctrl Pts',(7.13509633721601,-3.45970773442877,
63.4967404827161));
#236723=CARTESIAN_POINT('Ctrl Pts',(6.76173981293107,-4.11169516212418,
63.4653177398487));
#236724=CARTESIAN_POINT('Ctrl Pts',(6.65132737813032,-4.288007855659,63.4567666073274));
#236725=CARTESIAN_POINT('Ctrl Pts',(6.51446899673032,-4.488521630452,63.4469460817995));
#236726=CARTESIAN_POINT('Ctrl Pts',(6.49465540634456,-4.51714333560683,
63.4455418108436));
#236727=CARTESIAN_POINT('Ctrl Pts',(6.4652269591121,-4.55906026576051,63.4434815785605));
#236728=CARTESIAN_POINT('Ctrl Pts',(6.45575866501371,-4.57245778560391,
63.4428225343282));
#236729=CARTESIAN_POINT('Ctrl Pts',(6.43882889960544,-4.59625578493807,
63.4416508965721));
#236730=CARTESIAN_POINT('Ctrl Pts',(6.43138374031643,-4.60666777887235,
63.4411379515988));
#236731=CARTESIAN_POINT('Ctrl Pts',(6.41578064898209,-4.6283770202616,63.4400677498301));
#236732=CARTESIAN_POINT('Ctrl Pts',(6.40761806898652,-4.63967087852325,
63.4395105979607));
#236733=CARTESIAN_POINT('Ctrl Pts',(6.38653989593425,-4.66867321159473,
63.4380788212037));
#236734=CARTESIAN_POINT('Ctrl Pts',(6.37358044992413,-4.68634971520397,
63.4372051863992));
#236735=CARTESIAN_POINT('Ctrl Pts',(6.31813531142907,-4.76132070407994,
63.4334956269971));
#236736=CARTESIAN_POINT('Ctrl Pts',(6.27494889077715,-4.81809353198969,
63.4306759929381));
#236737=CARTESIAN_POINT('Ctrl Pts',(6.16251638105853,-4.96182095090556,
63.42350924253));
#236738=CARTESIAN_POINT('Ctrl Pts',(6.09219424850501,-5.04791494560045,
63.4191891293314));
#236739=CARTESIAN_POINT('Ctrl Pts',(5.88157056536384,-5.29496248111823,
63.4066978852439));
#236740=CARTESIAN_POINT('Ctrl Pts',(5.73653870245759,-5.45175459549485,
63.3986512425307));
#236741=CARTESIAN_POINT('Ctrl Pts',(5.2847659106428,-5.90214411618888,63.3749627627332));
#236742=CARTESIAN_POINT('Ctrl Pts',(4.96057340594551,-6.17711606949194,
63.3597493638944));
#236743=CARTESIAN_POINT('Ctrl Pts',(4.34783412448755,-6.61734113997531,
63.3320745106633));
#236744=CARTESIAN_POINT('Ctrl Pts',(4.06800329417708,-6.79295111586457,
63.3197635675601));
#236745=CARTESIAN_POINT('Ctrl Pts',(3.76149356967338,-6.95955761019976,
63.3058443043063));
#236746=CARTESIAN_POINT('Ctrl Pts',(3.74490748890894,-6.96849653047752,
63.3050897596108));
#236747=CARTESIAN_POINT('Ctrl Pts',(3.72212545680307,-6.98066987698059,
63.304051313161));
#236748=CARTESIAN_POINT('Ctrl Pts',(3.71595683018655,-6.98395551842405,
63.3037699324163));
#236749=CARTESIAN_POINT('Ctrl Pts',(3.70542622505697,-6.98954661138202,
63.3032892208275));
#236750=CARTESIAN_POINT('Ctrl Pts',(3.70106642277654,-6.9918561681456,63.3030900951225));
#236751=CARTESIAN_POINT('Ctrl Pts',(3.69260927855222,-6.99632611957984,
63.3027036221987));
#236752=CARTESIAN_POINT('Ctrl Pts',(3.6885121938096,-6.99848699731127,63.3025162995028));
#236753=CARTESIAN_POINT('Ctrl Pts',(3.67875456597198,-7.00362240079776,
63.3020699400994));
#236754=CARTESIAN_POINT('Ctrl Pts',(3.67309231547932,-7.00659366106113,
63.3018107373652));
#236755=CARTESIAN_POINT('Ctrl Pts',(3.65649026926341,-7.01527991253892,
63.3010501809444));
#236756=CARTESIAN_POINT('Ctrl Pts',(3.64554072945608,-7.02097615205138,
63.3005478612281));
#236757=CARTESIAN_POINT('Ctrl Pts',(3.62079133826501,-7.033777932925,63.2994107635638));
#236758=CARTESIAN_POINT('Ctrl Pts',(3.60698384511422,-7.04086851606291,
63.2987751977599));
#236759=CARTESIAN_POINT('Ctrl Pts',(3.56302228508351,-7.06328091069434,
63.2967475841615));
#236760=CARTESIAN_POINT('Ctrl Pts',(3.53279182429359,-7.07844946583242,
63.295347039574));
#236761=CARTESIAN_POINT('Ctrl Pts',(3.41031140286582,-7.13892568544084,
63.289649011473));
#236762=CARTESIAN_POINT('Ctrl Pts',(3.31728258414977,-7.18262616307382,
63.2852679933985));
#236763=CARTESIAN_POINT('Ctrl Pts',(3.03941027153567,-7.30660740985964,
63.2720774540956));
#236764=CARTESIAN_POINT('Ctrl Pts',(2.85232621806612,-7.38164984952312,
63.2630628956661));
#236765=CARTESIAN_POINT('Ctrl Pts',(2.46773212219431,-7.51911163645617,
63.2445108097419));
#236766=CARTESIAN_POINT('Ctrl Pts',(2.27021833357291,-7.58108487706883,
63.2349731810248));
#236767=CARTESIAN_POINT('Ctrl Pts',(1.81916341428423,-7.70340080464544,
63.2134207403243));
#236768=CARTESIAN_POINT('Ctrl Pts',(1.56460325517156,-7.75910833493442,
63.2014185806682));
#236769=CARTESIAN_POINT('Ctrl Pts',(0.834881445589659,-7.88142027242494,
63.1679151538222));
#236770=CARTESIAN_POINT('Ctrl Pts',(0.35574036248254,-7.91753495177006,
63.147043840901));
#236771=CARTESIAN_POINT('Ctrl Pts',(-0.155828194711189,-7.90953009500481,
63.1262136662988));
#236772=CARTESIAN_POINT('Ctrl Pts',(-0.187879696822543,-7.90883366874564,
63.12491429725));
#236773=CARTESIAN_POINT('Ctrl Pts',(-0.23202914836037,-7.90760583653871,
63.1231322284744));
#236774=CARTESIAN_POINT('Ctrl Pts',(-0.244131221362002,-7.90724146211114,
63.1226445372684));
#236775=CARTESIAN_POINT('Ctrl Pts',(-0.263407239634278,-7.90661679594143,
63.121869019027));
#236776=CARTESIAN_POINT('Ctrl Pts',(-0.270581726987097,-7.9063745206703,
63.121580653234));
#236777=CARTESIAN_POINT('Ctrl Pts',(-0.284540352484606,-7.90588412978552,
63.1210201539704));
#236778=CARTESIAN_POINT('Ctrl Pts',(-0.291324520084976,-7.90563704644275,
63.1207479898238));
#236779=CARTESIAN_POINT('Ctrl Pts',(-0.307552031188192,-7.90502511429534,
63.1200975764195));
#236780=CARTESIAN_POINT('Ctrl Pts',(-0.316995064710479,-7.90465207578622,
63.1197195726926));
#236781=CARTESIAN_POINT('Ctrl Pts',(-0.345310423768705,-7.90348268225755,
63.118587547154));
#236782=CARTESIAN_POINT('Ctrl Pts',(-0.364180647064771,-7.90263565273551,
63.1178350434298));
#236783=CARTESIAN_POINT('Ctrl Pts',(-0.528940873703219,-7.89464865451438,
63.1112812460149));
#236784=CARTESIAN_POINT('Ctrl Pts',(-0.674614125503046,-7.88353691317266,
63.1056002782559));
#236785=CARTESIAN_POINT('Ctrl Pts',(-1.23059885112246,-7.82560231641964,
63.0842897814308));
#236786=CARTESIAN_POINT('Ctrl Pts',(-1.63733325522774,-7.75071606027826,
63.0695147263373));
#236787=CARTESIAN_POINT('Ctrl Pts',(-2.13083361138616,-7.61925348107716,
63.0517066338229));
#236788=CARTESIAN_POINT('Ctrl Pts',(-2.22481279927818,-7.59234375462168,
63.0483186790001));
#236789=CARTESIAN_POINT('Ctrl Pts',(-2.56836552838068,-7.4870450350955,
63.0358962081762));
#236790=CARTESIAN_POINT('Ctrl Pts',(-2.81450281443147,-7.39803459814459,
63.0269267700972));
#236791=CARTESIAN_POINT('Ctrl Pts',(-3.42130712582622,-7.14392217001038,
63.0038838816257));
#236792=CARTESIAN_POINT('Ctrl Pts',(-3.7748223836862,-6.96359738829807,
62.9895666291405));
#236793=CARTESIAN_POINT('Ctrl Pts',(-4.13479609800248,-6.74448020904884,
62.9728232014384));
#236794=CARTESIAN_POINT('Ctrl Pts',(-4.15619181354347,-6.73131648732427,
62.971820274038));
#236795=CARTESIAN_POINT('Ctrl Pts',(-4.18574355174824,-6.71294016043397,
62.9704246304117));
#236796=CARTESIAN_POINT('Ctrl Pts',(-4.19395338992532,-6.70781407320363,
62.9700357853563));
#236797=CARTESIAN_POINT('Ctrl Pts',(-4.20706114099578,-6.69959633885935,
62.9694131936411));
#236798=CARTESIAN_POINT('Ctrl Pts',(-4.21196511642709,-6.69651434744451,
62.9691798687378));
#236799=CARTESIAN_POINT('Ctrl Pts',(-4.22153172220577,-6.69048737622925,
62.9687239344762));
#236800=CARTESIAN_POINT('Ctrl Pts',(-4.22619466705786,-6.68754290072226,
62.9685013468812));
#236801=CARTESIAN_POINT('Ctrl Pts',(-4.23739375870245,-6.68045470199821,
62.9679659025585));
#236802=CARTESIAN_POINT('Ctrl Pts',(-4.24392690555339,-6.67630626256486,
62.9676528457913));
#236803=CARTESIAN_POINT('Ctrl Pts',(-4.25752219552345,-6.66764546072879,
62.9669999443457));
#236804=CARTESIAN_POINT('Ctrl Pts',(-4.26458327482654,-6.66313145051145,
62.9666600312947));
#236805=CARTESIAN_POINT('Ctrl Pts',(-4.30680165549954,-6.63604746372577,
62.9646228786255));
#236806=CARTESIAN_POINT('Ctrl Pts',(-4.34178655075259,-6.61321071158007,
62.9629148000786));
#236807=CARTESIAN_POINT('Ctrl Pts',(-4.43693757067343,-6.5500194126596,
62.9582174495099));
#236808=CARTESIAN_POINT('Ctrl Pts',(-4.49673235460716,-6.50911415824023,
62.9552083411964));
#236809=CARTESIAN_POINT('Ctrl Pts',(-4.80376571761989,-6.29282449872205,
62.9394865049185));
#236810=CARTESIAN_POINT('Ctrl Pts',(-5.04133224417852,-6.10415977446242,
62.9264124402159));
#236811=CARTESIAN_POINT('Ctrl Pts',(-5.47447485390096,-5.71760592375576,
62.9013320093905));
#236812=CARTESIAN_POINT('Ctrl Pts',(-5.67161080174227,-5.52211260611122,
62.8893447842702));
#236813=CARTESIAN_POINT('Ctrl Pts',(-6.26986270417766,-4.86293970858322,
62.8513369290645));
#236814=CARTESIAN_POINT('Ctrl Pts',(-6.62755587378424,-4.36290146828069,
62.8261463124174));
#236815=CARTESIAN_POINT('Ctrl Pts',(-6.96576978193879,-3.75092595174726,
62.7977563571408));
#236816=CARTESIAN_POINT('Ctrl Pts',(-7.00634198489996,-3.67458382499478,
62.7942559518159));
#236817=CARTESIAN_POINT('Ctrl Pts',(-7.0602495353255,-3.5690093098751,62.789471352245));
#236818=CARTESIAN_POINT('Ctrl Pts',(-7.07467001517772,-3.54033828040014,
62.7881775800957));
#236819=CARTESIAN_POINT('Ctrl Pts',(-7.09912530616854,-3.49096976723562,
62.7859593714696));
#236820=CARTESIAN_POINT('Ctrl Pts',(-7.10924503446923,-3.47031483751352,
62.7850341544154));
#236821=CARTESIAN_POINT('Ctrl Pts',(-7.12993344383466,-3.42761835629211,
62.7831274353452));
#236822=CARTESIAN_POINT('Ctrl Pts',(-7.14049033714466,-3.40557135572353,
62.7821460549402));
#236823=CARTESIAN_POINT('Ctrl Pts',(-7.16114439327719,-3.36191919788908,
62.7802092004797));
#236824=CARTESIAN_POINT('Ctrl Pts',(-7.17124638279738,-3.3403166070579,
62.7792536884135));
#236825=CARTESIAN_POINT('Ctrl Pts',(-7.19441010128287,-3.29019275181924,
62.7770435189253));
#236826=CARTESIAN_POINT('Ctrl Pts',(-7.20740018771078,-3.26163878935312,
62.7757895847122));
#236827=CARTESIAN_POINT('Ctrl Pts',(-7.24061068202721,-3.18747038019025,
62.7725455988817));
#236828=CARTESIAN_POINT('Ctrl Pts',(-7.26057004381556,-3.14174046452932,
62.770558208481));
#236829=CARTESIAN_POINT('Ctrl Pts',(-7.39687529743503,-2.82120704187418,
62.7567143853091));
#236830=CARTESIAN_POINT('Ctrl Pts',(-7.49802459475522,-2.54019811410001,
62.7450275291352));
#236831=CARTESIAN_POINT('Ctrl Pts',(-7.71525783041505,-1.80941381150031,
62.7154074416694));
#236832=CARTESIAN_POINT('Ctrl Pts',(-7.80807617666539,-1.35392540913555,
62.6976887149269));
#236833=CARTESIAN_POINT('Ctrl Pts',(-7.86860920784648,-0.821062540347037,
62.6766127570459));
#236834=CARTESIAN_POINT('Ctrl Pts',(-7.8757884283724,-0.749073443795881,
62.6737571195273));
#236835=CARTESIAN_POINT('Ctrl Pts',(-7.88710793826565,-0.617285281893133,
62.6685050860276));
#236836=CARTESIAN_POINT('Ctrl Pts',(-7.89155790886853,-0.557518070914136,
62.6661141194771));
#236837=CARTESIAN_POINT('Ctrl Pts',(-7.89649509437854,-0.479197428151138,
62.6629651230745));
#236838=CARTESIAN_POINT('Ctrl Pts',(-7.8975967833046,-0.460684268224057,
62.6622196185075));
#236839=CARTESIAN_POINT('Ctrl Pts',(-7.89919993510043,-0.432046457029626,
62.6610644797303));
#236840=CARTESIAN_POINT('Ctrl Pts',(-7.89974705693606,-0.421924390696138,
62.66065582272));
#236841=CARTESIAN_POINT('Ctrl Pts',(-7.90079530384688,-0.401814113693694,
62.6598431448212));
#236842=CARTESIAN_POINT('Ctrl Pts',(-7.9012969467538,-0.391825948337949,
62.6594391360707));
#236843=CARTESIAN_POINT('Ctrl Pts',(-7.90224314638702,-0.372245175815101,
62.6586463530874));
#236844=CARTESIAN_POINT('Ctrl Pts',(-7.90268917938739,-0.362652656010148,
62.6582576128334));
#236845=CARTESIAN_POINT('Ctrl Pts',(-7.90364951877993,-0.341155774561508,
62.6573856093179));
#236846=CARTESIAN_POINT('Ctrl Pts',(-7.90415439594652,-0.329251063018407,
62.6569021269899));
#236847=CARTESIAN_POINT('Ctrl Pts',(-7.90536890445572,-0.298999329113977,
62.6556720296713));
#236848=CARTESIAN_POINT('Ctrl Pts',(-7.9060415591867,-0.28065098335316,
62.6549245682616));
#236849=CARTESIAN_POINT('Ctrl Pts',(-7.90953206395998,-0.175435025194458,
62.6506308328613));
#236850=CARTESIAN_POINT('Ctrl Pts',(-7.91098204786704,-0.0885293612401188,
62.6470549677864));
#236851=CARTESIAN_POINT('Ctrl Pts',(-7.91099983433237,-0.00161900995920416,
62.6434563298346));
#236852=CARTESIAN_POINT('',(-7.91119476205495,-0.00157576206492399,60.642331508237));
#236853=CARTESIAN_POINT('Ctrl Pts',(-7.91295189375223,-0.00166598417887076,
62.642331508237));
#236854=CARTESIAN_POINT('Ctrl Pts',(-7.911044428271,1.20131615954359,62.5937797499043));
#236855=CARTESIAN_POINT('Ctrl Pts',(-7.31720135608686,3.72124015044939,
62.4922432029633));
#236856=CARTESIAN_POINT('Ctrl Pts',(-3.88587637449001,7.80657458159615,
62.2847370788058));
#236857=CARTESIAN_POINT('Ctrl Pts',(3.49765847362659,8.67946754426088,62.0198131357647));
#236858=CARTESIAN_POINT('Ctrl Pts',(9.20349395763675,1.7300954411653,61.7019044041151));
#236859=CARTESIAN_POINT('Ctrl Pts',(6.8843891943671,-5.35210690193868,61.436980461074));
#236860=CARTESIAN_POINT('Ctrl Pts',(2.11872085160187,-7.94981861215979,
61.2250413066407));
#236861=CARTESIAN_POINT('Ctrl Pts',(-3.33448788563662,-8.06506802945827,
61.0131021522079));
#236862=CARTESIAN_POINT('Ctrl Pts',(-7.3506215263508,-4.4053455900463,60.8188655527398));
#236863=CARTESIAN_POINT('Ctrl Pts',(-7.9145503126708,-0.881728631901568,
60.6776137418802));
#236864=CARTESIAN_POINT('Ctrl Pts',(-7.91119476205495,-0.00157576206492399,
60.642331508237));
#236865=CARTESIAN_POINT('',(-7.911,2.06501482580279E-13,58.642331508237));
#236866=CARTESIAN_POINT('Ctrl Pts',(-7.911,1.51545442861334E-13,60.642331508237));
#236867=CARTESIAN_POINT('Ctrl Pts',(-7.91099999999996,2.20167589666687,
60.5537440725043));
#236868=CARTESIAN_POINT('Ctrl Pts',(-6.94214576672367,4.38610418338687,
60.4651566367716));
#236869=CARTESIAN_POINT('Ctrl Pts',(-3.67820201488288,7.3418068410763,60.2879817653061));
#236870=CARTESIAN_POINT('Ctrl Pts',(-1.40868175871752,8.08992666571334,
60.1993943295734));
#236871=CARTESIAN_POINT('Ctrl Pts',(2.97309270521258,7.65454228025262,60.022219458108));
#236872=CARTESIAN_POINT('Ctrl Pts',(5.05102072675584,6.47444880834238,59.9336320223752));
#236873=CARTESIAN_POINT('Ctrl Pts',(7.66951518847859,2.93425195367736,59.7564571509098));
#236874=CARTESIAN_POINT('Ctrl Pts',(8.18956872247067,0.601881960099537,
59.6678697151771));
#236875=CARTESIAN_POINT('Ctrl Pts',(7.32306689761363,-3.71537198232408,
59.4906948437116));
#236876=CARTESIAN_POINT('Ctrl Pts',(5.94329958850236,-5.66643518936472,
59.4021074079789));
#236877=CARTESIAN_POINT('Ctrl Pts',(2.16154501637906,-7.9220591323298,59.2249325365134));
#236878=CARTESIAN_POINT('Ctrl Pts',(-0.210816529299704,-8.20894963713003,
59.1363451007807));
#236879=CARTESIAN_POINT('Ctrl Pts',(-4.42123908576373,-6.91982244717871,
58.9591702293153));
#236880=CARTESIAN_POINT('Ctrl Pts',(-6.22631625634134,-5.35390358803581,
58.8705827935825));
#236881=CARTESIAN_POINT('Ctrl Pts',(-7.65317280859479,-2.31334857514567,
58.7354407413122));
#236882=CARTESIAN_POINT('Ctrl Pts',(-7.91100000000003,-1.15702837836533,
58.6888861247746));
#236883=CARTESIAN_POINT('Ctrl Pts',(-7.911,2.06501482580279E-13,58.642331508237));
#236884=CARTESIAN_POINT('',(-7.91885212407836,0.00556268397477262,56.6423315082371));
#236885=CARTESIAN_POINT('Ctrl Pts',(-7.91099992802374,0.00106714965019804,
58.642331508237));
#236886=CARTESIAN_POINT('Ctrl Pts',(-7.91096940833068,0.227315913889333,
58.6332491561257));
#236887=CARTESIAN_POINT('Ctrl Pts',(-7.90122887744838,0.453290643197541,
58.6241668040144));
#236888=CARTESIAN_POINT('Ctrl Pts',(-7.88187379827257,0.67822299290445,
58.615084451903));
#236889=CARTESIAN_POINT('Ctrl Pts',(-7.86241477327814,0.904363334426611,
58.6059533233172));
#236890=CARTESIAN_POINT('Ctrl Pts',(-7.83323770277879,1.12944994568909,
58.5968221947314));
#236891=CARTESIAN_POINT('Ctrl Pts',(-7.79449038791976,1.35271600590314,
58.5876910661456));
#236892=CARTESIAN_POINT('Ctrl Pts',(-7.75565473134637,1.57649110026798,
58.5785391190965));
#236893=CARTESIAN_POINT('Ctrl Pts',(-7.70720520429141,1.79843721837864,
58.5693871720473));
#236894=CARTESIAN_POINT('Ctrl Pts',(-7.64934062386123,2.01779806228132,
58.5602352249982));
#236895=CARTESIAN_POINT('Ctrl Pts',(-7.59135757699637,2.23760800469804,
58.5510645411237));
#236896=CARTESIAN_POINT('Ctrl Pts',(-7.52392093810813,2.45482196310906,
58.5418938572492));
#236897=CARTESIAN_POINT('Ctrl Pts',(-7.44728003336618,2.66869651789509,
58.5327231733748));
#236898=CARTESIAN_POINT('Ctrl Pts',(-7.41968444052939,2.7457049398585,58.5294211447898));
#236899=CARTESIAN_POINT('Ctrl Pts',(-7.39089601295679,2.82228059530343,
58.5261191162049));
#236900=CARTESIAN_POINT('Ctrl Pts',(-7.36092793096881,2.89838937948014,
58.5228170876199));
#236901=CARTESIAN_POINT('Ctrl Pts',(-7.28988374893415,3.0788175536841,58.5149890951589));
#236902=CARTESIAN_POINT('Ctrl Pts',(-7.21211428983778,3.2568539712332,58.5071611026978));
#236903=CARTESIAN_POINT('Ctrl Pts',(-7.12780410353066,3.4319571182769,58.4993331102368));
#236904=CARTESIAN_POINT('Ctrl Pts',(-7.04356512704589,3.60691237021398,
58.4915117294318));
#236905=CARTESIAN_POINT('Ctrl Pts',(-6.95279657486164,3.77893896953824,
58.4836903486268));
#236906=CARTESIAN_POINT('Ctrl Pts',(-6.85573177582579,3.94751349813177,
58.4758689678218));
#236907=CARTESIAN_POINT('Ctrl Pts',(-6.75873181828307,4.11597541510663,
58.4680528118771));
#236908=CARTESIAN_POINT('Ctrl Pts',(-6.65544416528475,4.28098955002536,
58.4602366559323));
#236909=CARTESIAN_POINT('Ctrl Pts',(-6.5461490106616,4.44205516964998,58.4524204999875));
#236910=CARTESIAN_POINT('Ctrl Pts',(-6.43690636184094,4.60304341274642,
58.4446080989534));
#236911=CARTESIAN_POINT('Ctrl Pts',(-6.32166215730543,4.76008662815491,
58.4367956979194));
#236912=CARTESIAN_POINT('Ctrl Pts',(-6.2007411113375,4.91271113237578,58.4289832968852));
#236913=CARTESIAN_POINT('Ctrl Pts',(-6.07985540926239,5.06529102613143,
58.4211731793301));
#236914=CARTESIAN_POINT('Ctrl Pts',(-5.95329639023129,5.21345450622929,
58.413363061775));
#236915=CARTESIAN_POINT('Ctrl Pts',(-5.82143053108722,5.35675905485076,
58.4055529442198));
#236916=CARTESIAN_POINT('Ctrl Pts',(-5.68955715861867,5.50007176853921,
58.3977423816674));
#236917=CARTESIAN_POINT('Ctrl Pts',(-5.55237657564755,5.63852473403909,
58.389931819115));
#236918=CARTESIAN_POINT('Ctrl Pts',(-5.41029407527172,5.77171023346458,
58.3821212565626));
#236919=CARTESIAN_POINT('Ctrl Pts',(-5.29957997260393,5.87549157893815,
58.3760350783068));
#236920=CARTESIAN_POINT('Ctrl Pts',(-5.18589028672745,5.97607523241643,
58.369948900051));
#236921=CARTESIAN_POINT('Ctrl Pts',(-5.06943163061923,6.07328444439063,
58.3638627217951));
#236922=CARTESIAN_POINT('Ctrl Pts',(-4.9040987450655,6.21128946741928,58.3552223557918));
#236923=CARTESIAN_POINT('Ctrl Pts',(-4.73326321401969,6.34242682809438,
58.3465819897885));
#236924=CARTESIAN_POINT('Ctrl Pts',(-4.55750201800622,6.46630469092427,
58.3379416237852));
#236925=CARTESIAN_POINT('Ctrl Pts',(-4.38144844489156,6.59038862341719,
58.329286884614));
#236926=CARTESIAN_POINT('Ctrl Pts',(-4.20045301627322,6.70718878691962,
58.3206321454429));
#236927=CARTESIAN_POINT('Ctrl Pts',(-4.01512042995576,6.81635745343155,
58.3119774062718));
#236928=CARTESIAN_POINT('Ctrl Pts',(-3.82405570793325,6.92890258828949,
58.3030549854133));
#236929=CARTESIAN_POINT('Ctrl Pts',(-3.62838151641226,7.03333651284979,
58.2941325645549));
#236930=CARTESIAN_POINT('Ctrl Pts',(-3.42878438433409,7.12933086942573,
58.2852101436964));
#236931=CARTESIAN_POINT('Ctrl Pts',(-3.23452569788872,7.22275775096684,
58.2765263628333));
#236932=CARTESIAN_POINT('Ctrl Pts',(-3.03655143037527,7.30819064082307,
58.2678425819702));
#236933=CARTESIAN_POINT('Ctrl Pts',(-2.83551318567347,7.3853764950659,58.259158801107));
#236934=CARTESIAN_POINT('Ctrl Pts',(-2.62618780777504,7.46574407951114,
58.2501170602509));
#236935=CARTESIAN_POINT('Ctrl Pts',(-2.41354078660347,7.53717026480837,
58.2410753193948));
#236936=CARTESIAN_POINT('Ctrl Pts',(-2.19832496958148,7.59942684207925,
58.2320335785387));
#236937=CARTESIAN_POINT('Ctrl Pts',(-1.9831091525595,7.66168341935013,58.2229918376826));
#236938=CARTESIAN_POINT('Ctrl Pts',(-1.76532481521441,7.71477034207186,
58.2139500968265));
#236939=CARTESIAN_POINT('Ctrl Pts',(-1.545738369841,7.75851879497635,58.2049083559704));
#236940=CARTESIAN_POINT('Ctrl Pts',(-1.3436316008017,7.79878475243088,58.1965863621979));
#236941=CARTESIAN_POINT('Ctrl Pts',(-1.13982650248577,7.83117396984472,
58.1882643684254));
#236942=CARTESIAN_POINT('Ctrl Pts',(-0.934949408664502,7.85555794347148,
58.1799423746529));
#236943=CARTESIAN_POINT('Ctrl Pts',(-0.730254536072288,7.87992022957056,
58.1716277826056));
#236944=CARTESIAN_POINT('Ctrl Pts',(-0.524489859309828,7.89629144106774,
58.1633131905582));
#236945=CARTESIAN_POINT('Ctrl Pts',(-0.31829045064656,7.90459437220072,
58.1549985985109));
#236946=CARTESIAN_POINT('Ctrl Pts',(-0.112261864260327,7.91289042491628,
58.1466908945412));
#236947=CARTESIAN_POINT('Ctrl Pts',(0.0942004442125806,7.91313151999478,
58.1383831905715));
#236948=CARTESIAN_POINT('Ctrl Pts',(0.300456894676682,7.90529231935425,
58.1300754866019));
#236949=CARTESIAN_POINT('Ctrl Pts',(0.506505241677638,7.89746102811387,
58.1217761647311));
#236950=CARTESIAN_POINT('Ctrl Pts',(0.71234785382415,7.88156572555374,58.1134768428604));
#236951=CARTESIAN_POINT('Ctrl Pts',(0.917345371216407,7.85763313408738,
58.1051775209896));
#236952=CARTESIAN_POINT('Ctrl Pts',(1.12221191552918,7.83371583317304,58.0968835015623));
#236953=CARTESIAN_POINT('Ctrl Pts',(1.32623415240593,7.80177151984718,58.0885894821349));
#236954=CARTESIAN_POINT('Ctrl Pts',(1.52877661383848,7.76187883601519,58.0802954627076));
#236955=CARTESIAN_POINT('Ctrl Pts',(1.73116887996143,7.72201573459252,58.0720075937083));
#236956=CARTESIAN_POINT('Ctrl Pts',(1.93208327441081,7.67421608263384,58.0637197247089));
#236957=CARTESIAN_POINT('Ctrl Pts',(2.13089277128065,7.61860991239897,58.0554318557095));
#236958=CARTESIAN_POINT('Ctrl Pts',(2.20667782066217,7.59741315659245,58.0522725671882));
#236959=CARTESIAN_POINT('Ctrl Pts',(2.28215710482043,7.57508257354178,58.0491132786669));
#236960=CARTESIAN_POINT('Ctrl Pts',(2.35729629640153,7.55162731939094,58.0459539901456));
#236961=CARTESIAN_POINT('Ctrl Pts',(2.54999823109176,7.49147398584543,58.0378516803192));
#236962=CARTESIAN_POINT('Ctrl Pts',(2.74038128870137,7.42394518745584,58.0297493704928));
#236963=CARTESIAN_POINT('Ctrl Pts',(2.92786907164504,7.34925191426341,58.0216470606664));
#236964=CARTESIAN_POINT('Ctrl Pts',(3.11539823756553,7.27454215450346,58.013542962469));
#236965=CARTESIAN_POINT('Ctrl Pts',(3.30003055800498,7.19266488408896,58.0054388642716));
#236966=CARTESIAN_POINT('Ctrl Pts',(3.48120979698936,7.10387917615054,57.9973347660743));
#236967=CARTESIAN_POINT('Ctrl Pts',(3.66245175319492,7.01506273404571,57.9892278625526));
#236968=CARTESIAN_POINT('Ctrl Pts',(3.84023795770216,6.91933322516687,57.981120959031));
#236969=CARTESIAN_POINT('Ctrl Pts',(4.01403644525848,6.81699584979606,57.9730140555094));
#236970=CARTESIAN_POINT('Ctrl Pts',(4.18799167277873,6.71456618158225,57.9648998407862));
#236971=CARTESIAN_POINT('Ctrl Pts',(4.35795172173338,6.60551690033114,57.956785626063));
#236972=CARTESIAN_POINT('Ctrl Pts',(4.52341217216975,6.49019747932731,57.9486714113399));
#236973=CARTESIAN_POINT('Ctrl Pts',(4.68895348846072,6.37482169800591,57.9405532309385));
#236974=CARTESIAN_POINT('Ctrl Pts',(4.84999056217602,6.25316985214359,57.9324350505371));
#236975=CARTESIAN_POINT('Ctrl Pts',(5.00605106612091,6.12563251618881,57.9243168701357));
#236976=CARTESIAN_POINT('Ctrl Pts',(5.16227939843205,5.99795802584719,57.9161899593962));
#236977=CARTESIAN_POINT('Ctrl Pts',(5.31352022438843,5.86438560526916,57.9080630486568));
#236978=CARTESIAN_POINT('Ctrl Pts',(5.45933613739997,5.72534452577998,57.8999361379174));
#236979=CARTESIAN_POINT('Ctrl Pts',(5.53670664146746,5.65156877535613,57.8956239667185));
#236980=CARTESIAN_POINT('Ctrl Pts',(5.61255044765232,5.57625398609848,57.8913117955197));
#236981=CARTESIAN_POINT('Ctrl Pts',(5.6868066934775,5.49946821347478,57.8869996243208));
#236982=CARTESIAN_POINT('Ctrl Pts',(5.8245298280504,5.35705356297878,57.8790018360174));
#236983=CARTESIAN_POINT('Ctrl Pts',(5.95702851641505,5.20932963798965,57.8710040477139));
#236984=CARTESIAN_POINT('Ctrl Pts',(6.08387878431521,5.05671236454668,57.8630062594104));
#236985=CARTESIAN_POINT('Ctrl Pts',(6.21062547912626,4.90421970292144,57.8550150012914));
#236986=CARTESIAN_POINT('Ctrl Pts',(6.33173273167485,4.74684191120925,57.8470237431723));
#236987=CARTESIAN_POINT('Ctrl Pts',(6.44681411763098,4.58503094130387,57.8390324850533));
#236988=CARTESIAN_POINT('Ctrl Pts',(6.56182105441875,4.42332465116092,57.8310463966888));
#236989=CARTESIAN_POINT('Ctrl Pts',(6.67080970098743,4.25719117061807,57.8230603083243));
#236990=CARTESIAN_POINT('Ctrl Pts',(6.77343431023401,4.08711495372282,57.8150742199598));
#236991=CARTESIAN_POINT('Ctrl Pts',(6.87600992375256,3.91711993575374,57.8070919443671));
#236992=CARTESIAN_POINT('Ctrl Pts',(6.97222738389496,3.74318621947823,57.7991096687743));
#236993=CARTESIAN_POINT('Ctrl Pts',(7.06178441053314,3.56582696427506,57.7911273931816));
#236994=CARTESIAN_POINT('Ctrl Pts',(7.15131385511121,3.38852233274378,57.7831475759957));
#236995=CARTESIAN_POINT('Ctrl Pts',(7.23418680508977,3.20779456389923,57.7751677588098));
#236996=CARTESIAN_POINT('Ctrl Pts',(7.31014687583093,3.02418148492767,57.7671879416239));
#236997=CARTESIAN_POINT('Ctrl Pts',(7.38871731538235,2.83425854013018,57.7589338979176));
#236998=CARTESIAN_POINT('Ctrl Pts',(7.45989114022406,2.64124878708016,57.7506798542112));
#236999=CARTESIAN_POINT('Ctrl Pts',(7.52343851156297,2.44577062757961,57.7424258105049));
#237000=CARTESIAN_POINT('Ctrl Pts',(7.58488293844788,2.25676133850973,57.7344449141384));
#237001=CARTESIAN_POINT('Ctrl Pts',(7.63919749948067,2.06544473941621,57.7264640177718));
#237002=CARTESIAN_POINT('Ctrl Pts',(7.68622497097408,1.87239597723734,57.7184831214053));
#237003=CARTESIAN_POINT('Ctrl Pts',(7.73326288316665,1.67930435576819,57.7105004531779));
#237004=CARTESIAN_POINT('Ctrl Pts',(7.77301040096005,1.4844801297399,57.7025177849505));
#237005=CARTESIAN_POINT('Ctrl Pts',(7.80536120397024,1.28850978869243,57.6945351167231));
#237006=CARTESIAN_POINT('Ctrl Pts',(7.83772416213384,1.0924658157924,57.6865494491711));
#237007=CARTESIAN_POINT('Ctrl Pts',(7.86268481042211,0.895275199482527,
57.6785637816192));
#237008=CARTESIAN_POINT('Ctrl Pts',(7.88018853644928,0.697531096090645,
57.6705781140673));
#237009=CARTESIAN_POINT('Ctrl Pts',(7.89770153022582,0.499682292545889,
57.6625882183204));
#237010=CARTESIAN_POINT('Ctrl Pts',(7.90774970095625,0.301279750613616,
57.6545983225735));
#237011=CARTESIAN_POINT('Ctrl Pts',(7.91033050948413,0.102918563556239,
57.6466084268267));
#237012=CARTESIAN_POINT('Ctrl Pts',(7.91291437519276,-0.0956775987018777,
57.6386090663887));
#237013=CARTESIAN_POINT('Ctrl Pts',(7.9080132038404,-0.294231973617734,
57.6306097059508));
#237014=CARTESIAN_POINT('Ctrl Pts',(7.8956765394065,-0.492151384297384,
57.6226103455129));
#237015=CARTESIAN_POINT('Ctrl Pts',(7.88333125094898,-0.69020915179793,
57.6146053930712));
#237016=CARTESIAN_POINT('Ctrl Pts',(7.86354013599447,-0.887630737857427,
57.6066004406296));
#237017=CARTESIAN_POINT('Ctrl Pts',(7.83640427237677,-1.08383074318602,
57.5985954881879));
#237018=CARTESIAN_POINT('Ctrl Pts',(7.80923299424253,-1.28028680553311,
57.5905800886301));
#237019=CARTESIAN_POINT('Ctrl Pts',(7.77469787875517,-1.47551777435169,
57.5825646890722));
#237020=CARTESIAN_POINT('Ctrl Pts',(7.73295074651253,-1.66894989499725,
57.5745492895143));
#237021=CARTESIAN_POINT('Ctrl Pts',(7.72347430418865,-1.71285826034864,
57.5727298239));
#237022=CARTESIAN_POINT('Ctrl Pts',(7.71362644739048,-1.75667400383091,
57.5709103582857));
#237023=CARTESIAN_POINT('Ctrl Pts',(7.70340930374815,-1.80039054066789,
57.5690908926713));
#237024=CARTESIAN_POINT('Ctrl Pts',(7.65982881545839,-1.98686027119019,
57.5613300935013));
#237025=CARTESIAN_POINT('Ctrl Pts',(7.60939621414596,-2.17207776286606,
57.5535692943313));
#237026=CARTESIAN_POINT('Ctrl Pts',(7.55219166053658,-2.35548766129687,
57.5458084951612));
#237027=CARTESIAN_POINT('Ctrl Pts',(7.49505655269008,-2.53867490192314,
57.5380571175247));
#237028=CARTESIAN_POINT('Ctrl Pts',(7.43116596132914,-2.72005857897147,
57.5303057398882));
#237029=CARTESIAN_POINT('Ctrl Pts',(7.36065130442519,-2.89909181894326,
57.5225543622517));
#237030=CARTESIAN_POINT('Ctrl Pts',(7.29020793793713,-3.07794405606126,
57.5148108212687));
#237031=CARTESIAN_POINT('Ctrl Pts',(7.21315396760143,-3.25445025561536,
57.5070672802857));
#237032=CARTESIAN_POINT('Ctrl Pts',(7.12967105811057,-3.42807695408672,
57.4993237393028));
#237033=CARTESIAN_POINT('Ctrl Pts',(7.04625562909086,-3.60156330752832,
57.4915864575385));
#237034=CARTESIAN_POINT('Ctrl Pts',(6.95642176167249,-3.77217447228026,
57.4838491757743));
#237035=CARTESIAN_POINT('Ctrl Pts',(6.86039987431697,-3.93939520287971,
57.4761118940101));
#237036=CARTESIAN_POINT('Ctrl Pts',(6.76443616110939,-4.10651462404036,
57.4683792998207));
#237037=CARTESIAN_POINT('Ctrl Pts',(6.66229207125565,-4.27024739094581,
57.4606467056312));
#237038=CARTESIAN_POINT('Ctrl Pts',(6.55424481595404,-4.43010111538547,
57.4529141114417));
#237039=CARTESIAN_POINT('Ctrl Pts',(6.44624115950998,-4.58989033619899,
57.4451846374821));
#237040=CARTESIAN_POINT('Ctrl Pts',(6.33233928253398,-4.74580333503905,
57.4374551635225));
#237041=CARTESIAN_POINT('Ctrl Pts',(6.21286077897892,-4.89737500514566,
57.4297256895629));
#237042=CARTESIAN_POINT('Ctrl Pts',(6.09338420221705,-5.04894423090243,
57.4219963402542));
#237043=CARTESIAN_POINT('Ctrl Pts',(5.96833139152503,-5.19617197859636,
57.4142669909454));
#237044=CARTESIAN_POINT('Ctrl Pts',(5.83806569384948,-5.33862435036384,
57.4065376416367));
#237045=CARTESIAN_POINT('Ctrl Pts',(5.70779472968696,-5.48108248131102,
57.3988079798395));
#237046=CARTESIAN_POINT('Ctrl Pts',(5.57231070061897,-5.61876458601279,
57.3910783180424));
#237047=CARTESIAN_POINT('Ctrl Pts',(5.43201534467499,-5.75127205887667,
57.3833486562453));
#237048=CARTESIAN_POINT('Ctrl Pts',(5.29168860988826,-5.88380916872407,
57.3756172656108));
#237049=CARTESIAN_POINT('Ctrl Pts',(5.14654866637825,-6.01116909522465,
57.3678858749764));
#237050=CARTESIAN_POINT('Ctrl Pts',(4.99703202626331,-6.1329920861272,57.360154484342));
#237051=CARTESIAN_POINT('Ctrl Pts',(4.84745453975904,-6.25486465337876,
57.3524199473875));
#237052=CARTESIAN_POINT('Ctrl Pts',(4.69349708817789,-6.37119557151886,
57.3446854104331));
#237053=CARTESIAN_POINT('Ctrl Pts',(4.5356270033007,-6.48166712250247,57.3369508734786));
#237054=CARTESIAN_POINT('Ctrl Pts',(4.37757100220106,-6.59226877066988,
57.3292072279213));
#237055=CARTESIAN_POINT('Ctrl Pts',(4.21559345993335,-6.69699706499938,
57.3214635823641));
#237056=CARTESIAN_POINT('Ctrl Pts',(4.05018915375438,-6.79557862281134,
57.3137199368068));
#237057=CARTESIAN_POINT('Ctrl Pts',(3.88467887056285,-6.89422334330164,
57.30597132978));
#237058=CARTESIAN_POINT('Ctrl Pts',(3.71573776374398,-6.9867133106257,57.2982227227533));
#237059=CARTESIAN_POINT('Ctrl Pts',(3.54388251592853,-7.07282247149581,
57.2904741157265));
#237060=CARTESIAN_POINT('Ctrl Pts',(3.37176687433982,-7.15906210431598,
57.2827137680689));
#237061=CARTESIAN_POINT('Ctrl Pts',(3.19672859841029,-7.23890147297845,
57.2749534204113));
#237062=CARTESIAN_POINT('Ctrl Pts',(3.01930264737507,-7.31216332719352,
57.2671930727537));
#237063=CARTESIAN_POINT('Ctrl Pts',(2.89728271706964,-7.36254719884934,
57.2618561021764));
#237064=CARTESIAN_POINT('Ctrl Pts',(2.77413383706884,-7.40982118990013,
57.2565191315991));
#237065=CARTESIAN_POINT('Ctrl Pts',(2.65003307283612,-7.45394162258297,
57.2511821610218));
#237066=CARTESIAN_POINT('Ctrl Pts',(2.46600626720784,-7.51936702378625,
57.2432680627231));
#237067=CARTESIAN_POINT('Ctrl Pts',(2.27929511676439,-7.57806579485747,
57.2353539644245));
#237068=CARTESIAN_POINT('Ctrl Pts',(2.09043302669929,-7.62981066350174,
57.2274398661259));
#237069=CARTESIAN_POINT('Ctrl Pts',(1.90178780376386,-7.68149611439238,
57.2195348554519));
#237070=CARTESIAN_POINT('Ctrl Pts',(1.71099689002177,-7.72624347717776,
57.2116298447778));
#237071=CARTESIAN_POINT('Ctrl Pts',(1.51861292999975,-7.7638737604908,57.2037248341038));
#237072=CARTESIAN_POINT('Ctrl Pts',(1.32641414860508,-7.80146782288288,
57.1958274323751));
#237073=CARTESIAN_POINT('Ctrl Pts',(1.13262571155332,-7.83195838650878,
57.1879300306464));
#237074=CARTESIAN_POINT('Ctrl Pts',(0.937814939473485,-7.85521636489412,
57.1800326289177));
#237075=CARTESIAN_POINT('Ctrl Pts',(0.74315551126932,-7.8784562747068,57.1721413624933));
#237076=CARTESIAN_POINT('Ctrl Pts',(0.547475671210005,-7.89447475287415,
57.164250096069));
#237077=CARTESIAN_POINT('Ctrl Pts',(0.351352718647428,-7.90319380169176,
57.1563588296447));
#237078=CARTESIAN_POINT('Ctrl Pts',(0.155345724235176,-7.91190769535155,
57.1484722289499));
#237079=CARTESIAN_POINT('Ctrl Pts',(-0.0411035170795087,-7.91333074393357,
57.1405856282551));
#237080=CARTESIAN_POINT('Ctrl Pts',(-0.237412516086123,-7.90743677162237,
57.1326990275604));
#237081=CARTESIAN_POINT('Ctrl Pts',(-0.433641879939017,-7.90154519027335,
57.1248156261619));
#237082=CARTESIAN_POINT('Ctrl Pts',(-0.629730770656352,-7.88834251389541,
57.1169322247635));
#237083=CARTESIAN_POINT('Ctrl Pts',(-0.825096346086271,-7.86785466437167,
57.109048823365));
#237084=CARTESIAN_POINT('Ctrl Pts',(-1.02044628527462,-7.84736845460952,
57.101166052921));
#237085=CARTESIAN_POINT('Ctrl Pts',(-1.21507268094227,-7.81959826266944,
57.0932832824769));
#237086=CARTESIAN_POINT('Ctrl Pts',(-1.40839693655226,-7.7846219605778,
57.0854005120329));
#237087=CARTESIAN_POINT('Ctrl Pts',(-1.60172168115791,-7.74964557001688,
57.0775177216501));
#237088=CARTESIAN_POINT('Ctrl Pts',(-1.79374393951702,-7.70746309385163,
57.0696349312673));
#237089=CARTESIAN_POINT('Ctrl Pts',(-1.9838943476887,-7.65820372001221,
57.0617521408846));
#237090=CARTESIAN_POINT('Ctrl Pts',(-2.17407721358866,-7.60893593784285,
57.0538680049487));
#237091=CARTESIAN_POINT('Ctrl Pts',(-2.36238725867034,-7.55258893756365,
57.0459838690128));
#237092=CARTESIAN_POINT('Ctrl Pts',(-2.54826910623883,-7.48934213146847,
57.038099733077));
#237093=CARTESIAN_POINT('Ctrl Pts',(-2.73421394201501,-7.42607389346368,
57.0302129255107));
#237094=CARTESIAN_POINT('Ctrl Pts',(-2.91772861443998,-7.3559013021761,
57.0223261179445));
#237095=CARTESIAN_POINT('Ctrl Pts',(-3.09827636154169,-7.27905245121314,
57.0144393103783));
#237096=CARTESIAN_POINT('Ctrl Pts',(-3.27900053039043,-7.20212850760149,
57.0065447962391));
#237097=CARTESIAN_POINT('Ctrl Pts',(-3.45675166563389,-7.11851540902328,
56.9986502821));
#237098=CARTESIAN_POINT('Ctrl Pts',(-3.63101535873538,-7.02848834847351,
56.9907557679609));
#237099=CARTESIAN_POINT('Ctrl Pts',(-3.80537650642813,-6.93841094151919,
56.9828568389226));
#237100=CARTESIAN_POINT('Ctrl Pts',(-3.97624602381833,-6.84191259040028,
56.9749579098842));
#237101=CARTESIAN_POINT('Ctrl Pts',(-4.14313703997129,-6.73931275932628,
56.9670589808458));
#237102=CARTESIAN_POINT('Ctrl Pts',(-4.31023184716961,-6.63658764333694,
56.9591504064051));
#237103=CARTESIAN_POINT('Ctrl Pts',(-4.47333816303147,-6.52774635631258,
56.9512418319643));
#237104=CARTESIAN_POINT('Ctrl Pts',(-4.63199996408114,-6.41315034384446,
56.9433332575236));
#237105=CARTESIAN_POINT('Ctrl Pts',(-4.69927337998713,-6.36456104788958,
56.9399799814732));
#237106=CARTESIAN_POINT('Ctrl Pts',(-4.76574818354377,-6.31493764713479,
56.9366267054228));
#237107=CARTESIAN_POINT('Ctrl Pts',(-4.83139155477593,-6.26430975003949,
56.9332734293723));
#237108=CARTESIAN_POINT('Ctrl Pts',(-4.99962145197458,-6.13456129617652,
56.9246797012525));
#237109=CARTESIAN_POINT('Ctrl Pts',(-5.16272509822018,-5.99795315184645,
56.9160859731326));
#237110=CARTESIAN_POINT('Ctrl Pts',(-5.32016110145686,-5.85489597299092,
56.9074922450127));
#237111=CARTESIAN_POINT('Ctrl Pts',(-5.47736979429696,-5.71204534399306,
56.898910924752));
#237112=CARTESIAN_POINT('Ctrl Pts',(-5.62892699136269,-5.56276442911684,
56.8903296044912));
#237113=CARTESIAN_POINT('Ctrl Pts',(-5.77432430049551,-5.40750403353591,
56.8817482842305));
#237114=CARTESIAN_POINT('Ctrl Pts',(-5.92600958060508,-5.24552911987293,
56.8727958491736));
#237115=CARTESIAN_POINT('Ctrl Pts',(-6.07099014928944,-5.07704620370147,
56.8638434141167));
#237116=CARTESIAN_POINT('Ctrl Pts',(-6.20872801391771,-4.90261332854157,
56.8548909790597));
#237117=CARTESIAN_POINT('Ctrl Pts',(-6.3402359125913,-4.7360701565984,56.8463434679921));
#237118=CARTESIAN_POINT('Ctrl Pts',(-6.46514155792974,-4.56410355985527,
56.8377959569244));
#237119=CARTESIAN_POINT('Ctrl Pts',(-6.58301392637842,-4.38723701720204,
56.8292484458567));
#237120=CARTESIAN_POINT('Ctrl Pts',(-6.70070507568962,-4.21064239240987,
56.8207140758891));
#237121=CARTESIAN_POINT('Ctrl Pts',(-6.81138438193963,-4.02916305574041,
56.8121797059214));
#237122=CARTESIAN_POINT('Ctrl Pts',(-6.91466186145532,-3.84335430863916,
56.8036453359538));
#237123=CARTESIAN_POINT('Ctrl Pts',(-7.01771448227365,-3.65795010968363,
56.7951295472618));
#237124=CARTESIAN_POINT('Ctrl Pts',(-7.11339731274083,-3.46823552599294,
56.7866137585697));
#237125=CARTESIAN_POINT('Ctrl Pts',(-7.20136432801631,-3.27479355306166,
56.7780979698777));
#237126=CARTESIAN_POINT('Ctrl Pts',(-7.21437620211279,-3.2461800711915,
56.7768383344343));
#237127=CARTESIAN_POINT('Ctrl Pts',(-7.22721933351794,-3.21748508828331,
56.7755786989909));
#237128=CARTESIAN_POINT('Ctrl Pts',(-7.23989268275838,-3.18871054536809,
56.7743190635475));
#237129=CARTESIAN_POINT('Ctrl Pts',(-7.31699601980963,-3.0136492226825,
56.7666555726807));
#237130=CARTESIAN_POINT('Ctrl Pts',(-7.38775912880493,-2.83575951975293,
56.7589920818139));
#237131=CARTESIAN_POINT('Ctrl Pts',(-7.45197484386047,-2.6555586844336,
56.7513285909471));
#237132=CARTESIAN_POINT('Ctrl Pts',(-7.51619454488105,-2.47534666378014,
56.743664624396));
#237133=CARTESIAN_POINT('Ctrl Pts',(-7.57386592148028,-2.29282356988889,
56.7360006578449));
#237134=CARTESIAN_POINT('Ctrl Pts',(-7.62483108905492,-2.10852362172718,
56.7283366912939));
#237135=CARTESIAN_POINT('Ctrl Pts',(-7.6758306922615,-1.92409914762978,
56.7206675464309));
#237136=CARTESIAN_POINT('Ctrl Pts',(-7.72011493821241,-1.73789577386895,
56.712998401568));
#237137=CARTESIAN_POINT('Ctrl Pts',(-7.75757652038701,-1.55046042527379,
56.705329256705));
#237138=CARTESIAN_POINT('Ctrl Pts',(-7.79505129506646,-1.3629590692758,
56.6976574110691));
#237139=CARTESIAN_POINT('Ctrl Pts',(-7.82569856089014,-1.17422523459191,
56.6899855654331));
#237140=CARTESIAN_POINT('Ctrl Pts',(-7.84946272487774,-0.98481263738586,
56.6823137197972));
#237141=CARTESIAN_POINT('Ctrl Pts',(-7.87325307651349,-0.795191311168729,
56.674633419936));
#237142=CARTESIAN_POINT('Ctrl Pts',(-7.89014514416397,-0.604890092031874,
56.6669531200748));
#237143=CARTESIAN_POINT('Ctrl Pts',(-7.90013541291234,-0.414465267119512,
56.6592728202137));
#237144=CARTESIAN_POINT('Ctrl Pts',(-7.90748097070979,-0.274451360317271,
56.6536257162215));
#237145=CARTESIAN_POINT('Ctrl Pts',(-7.91109634198683,-0.134370668405158,
56.6479786122293));
#237146=CARTESIAN_POINT('Ctrl Pts',(-7.91099804815405,0.00555716679354367,
56.6423315082371));
#237147=CARTESIAN_POINT('',(-7.91503681196177,-0.00538689920117852,54.6423315082371));
#237148=CARTESIAN_POINT('Ctrl Pts',(-7.9196338726488,0.00556323312257564,
56.6423315082371));
#237149=CARTESIAN_POINT('Ctrl Pts',(-7.92037954994029,0.228541081453708,
56.633342571399));
#237150=CARTESIAN_POINT('Ctrl Pts',(-7.91127946851613,0.451321298709539,
56.6243536345609));
#237151=CARTESIAN_POINT('Ctrl Pts',(-7.66531770480111,3.28740455581408,
56.5093951205063));
#237152=CARTESIAN_POINT('Ctrl Pts',(-5.21295917794468,6.99651976617628,
56.3504407546814));
#237153=CARTESIAN_POINT('Ctrl Pts',(0.108828255203027,8.23489439458598,
56.1385016002485));
#237154=CARTESIAN_POINT('Ctrl Pts',(4.03755664298072,7.19823663329124,55.9795472344238));
#237155=CARTESIAN_POINT('Ctrl Pts',(6.97493635397154,4.37898776636411,55.8205928685989));
#237156=CARTESIAN_POINT('Ctrl Pts',(8.6839076066132,-0.795229888551257,
55.6086537141659));
#237157=CARTESIAN_POINT('Ctrl Pts',(5.54732397292391,-7.53617730613503,
55.3437297711246));
#237158=CARTESIAN_POINT('Ctrl Pts',(-3.36342892092028,-8.73984422959885,
55.0258210394751));
#237159=CARTESIAN_POINT('Ctrl Pts',(-7.60611129338621,-3.71462797172983,
54.7920216185127));
#237160=CARTESIAN_POINT('Ctrl Pts',(-7.91792072111909,-0.547831146367218,
54.6641917747666));
#237161=CARTESIAN_POINT('Ctrl Pts',(-7.91503681196177,-0.00538689920117852,
54.6423315082371));
#237162=CARTESIAN_POINT('',(-7.89592422791155,-0.00169916443013902,52.6419012676071));
#237163=CARTESIAN_POINT('Ctrl Pts',(-7.91503681196177,-0.00538689920117852,
54.6423315082371));
#237164=CARTESIAN_POINT('Ctrl Pts',(-7.91093071864774,0.766942108068054,
54.6112069861583));
#237165=CARTESIAN_POINT('Ctrl Pts',(-7.59192480626818,2.8589101804051,54.5270976754714));
#237166=CARTESIAN_POINT('Ctrl Pts',(-5.11028731654404,7.07453852357992,
54.3370187875679));
#237167=CARTESIAN_POINT('Ctrl Pts',(0.58978711048592,8.70507802341358,54.1250796331348));
#237168=CARTESIAN_POINT('Ctrl Pts',(5.43791012976232,6.18501921579411,53.9131404787019));
#237169=CARTESIAN_POINT('Ctrl Pts',(7.74829280852149,2.84261021379085,53.754186112877));
#237170=CARTESIAN_POINT('Ctrl Pts',(8.14634157535645,-1.20929315616148,
53.5952317470524));
#237171=CARTESIAN_POINT('Ctrl Pts',(6.07974643190811,-6.25134587265489,
53.3832925926191));
#237172=CARTESIAN_POINT('Ctrl Pts',(-0.686725509353473,-9.33247982718465,
53.1183686495784));
#237173=CARTESIAN_POINT('Ctrl Pts',(-6.97348851421393,-5.26974137332134,
52.8537204811401));
#237174=CARTESIAN_POINT('Ctrl Pts',(-7.8979285753281,-1.31578168274657,
52.6950418899188));
#237175=CARTESIAN_POINT('Ctrl Pts',(-7.89517691866717,-0.00168164862291708,
52.6423328759138));
#237176=CARTESIAN_POINT('',(-7.91099629000672,-0.00766153195038582,48.6489215596253));
#237177=CARTESIAN_POINT('Ctrl Pts',(-7.91099973373757,-0.00205251166330671,
52.6331944121903));
#237178=CARTESIAN_POINT('Ctrl Pts',(-7.911012932558,0.048819727856465,52.6310900189783));
#237179=CARTESIAN_POINT('Ctrl Pts',(-7.91053542539201,0.099691711568022,
52.6290015797071));
#237180=CARTESIAN_POINT('Ctrl Pts',(-7.9089841469533,0.181189019281594,
52.6256809048648));
#237181=CARTESIAN_POINT('Ctrl Pts',(-7.90822311057975,0.211818222793782,
52.6244385547084));
#237182=CARTESIAN_POINT('Ctrl Pts',(-7.90695085357179,0.253313005621773,
52.6227630283582));
#237183=CARTESIAN_POINT('Ctrl Pts',(-7.90659513898706,0.264182870437372,
52.6223248131627));
#237184=CARTESIAN_POINT('Ctrl Pts',(-7.90595353200988,0.282625506951483,
52.6215824858392));
#237185=CARTESIAN_POINT('Ctrl Pts',(-7.90567917209676,0.290198648831562,
52.6212780004511));
#237186=CARTESIAN_POINT('Ctrl Pts',(-7.90515089134796,0.304223727932115,
52.6207147319171));
#237187=CARTESIAN_POINT('Ctrl Pts',(-7.90489995253835,0.310675767063107,
52.6204558524761));
#237188=CARTESIAN_POINT('Ctrl Pts',(-7.90438181296186,0.323590785070841,
52.6199381414412));
#237189=CARTESIAN_POINT('Ctrl Pts',(-7.90411458409236,0.330053757846875,
52.6196793109632));
#237190=CARTESIAN_POINT('Ctrl Pts',(-7.90347797628165,0.345005914195665,
52.619081065922));
#237191=CARTESIAN_POINT('Ctrl Pts',(-7.90310284587809,0.353494852114456,
52.6187418374667));
#237192=CARTESIAN_POINT('Ctrl Pts',(-7.90212204759867,0.374907361350196,
52.6178872178594));
#237193=CARTESIAN_POINT('Ctrl Pts',(-7.90149835139332,0.387830104258191,
52.6173724089325));
#237194=CARTESIAN_POINT('Ctrl Pts',(-7.89800117210295,0.456777265173465,
52.6146308309875));
#237195=CARTESIAN_POINT('Ctrl Pts',(-7.89456350284564,0.512772124101357,
52.6124222693121));
#237196=CARTESIAN_POINT('Ctrl Pts',(-7.88765463965521,0.608625931688615,
52.6086707946328));
#237197=CARTESIAN_POINT('Ctrl Pts',(-7.88447618195296,0.648503380186446,
52.607118765331));
#237198=CARTESIAN_POINT('Ctrl Pts',(-7.80108588307536,1.60324068771695,
52.5701585682059));
#237199=CARTESIAN_POINT('Ctrl Pts',(-7.56252295257933,2.49704936280296,
52.5409320553595));
#237200=CARTESIAN_POINT('Ctrl Pts',(-7.14668627840421,3.3931778602967,52.5051186023916));
#237201=CARTESIAN_POINT('Ctrl Pts',(-7.11650863425822,3.45602160025433,
52.502564424753));
#237202=CARTESIAN_POINT('Ctrl Pts',(-7.01475458183899,3.66093494270624,
52.4940712254409));
#237203=CARTESIAN_POINT('Ctrl Pts',(-6.93972760594997,3.80123753006522,
52.4879826079628));
#237204=CARTESIAN_POINT('Ctrl Pts',(-6.84545460471771,3.96542398621287,
52.4804634148356));
#237205=CARTESIAN_POINT('Ctrl Pts',(-6.83024115713981,3.99157134927366,
52.479254570032));
#237206=CARTESIAN_POINT('Ctrl Pts',(-6.80987565222271,4.02611619720566,
52.4776428955779));
#237207=CARTESIAN_POINT('Ctrl Pts',(-6.80485721505982,4.03459245942312,
52.4772462677514));
#237208=CARTESIAN_POINT('Ctrl Pts',(-6.79659298336621,4.04849166503751,
52.4765939828554));
#237209=CARTESIAN_POINT('Ctrl Pts',(-6.79335648938684,4.05392014613352,
52.4763387485088));
#237210=CARTESIAN_POINT('Ctrl Pts',(-6.78707359918654,4.06442961019123,
52.4758436994921));
#237211=CARTESIAN_POINT('Ctrl Pts',(-6.78402799294279,4.06951106248642,
52.475603920298));
#237212=CARTESIAN_POINT('Ctrl Pts',(-6.77698473842869,4.0812325253682,52.4750498616678));
#237213=CARTESIAN_POINT('Ctrl Pts',(-6.7729830379271,4.08787008580662,52.474735403034));
#237214=CARTESIAN_POINT('Ctrl Pts',(-6.76222473104568,4.1056555645672,52.4738909179498));
#237215=CARTESIAN_POINT('Ctrl Pts',(-6.75545032984012,4.11679265528246,
52.4733601178916));
#237216=CARTESIAN_POINT('Ctrl Pts',(-6.70742396134459,4.19531007673991,
52.4696040721258));
#237217=CARTESIAN_POINT('Ctrl Pts',(-6.66519295747925,4.26208460462532,
52.4663375849493));
#237218=CARTESIAN_POINT('Ctrl Pts',(-6.25122656140715,4.89543429045929,
52.4347230442141));
#237219=CARTESIAN_POINT('Ctrl Pts',(-5.80914108662441,5.4126731407887,52.4042669191825));
#237220=CARTESIAN_POINT('Ctrl Pts',(-5.02563446170886,6.12130554842635,
52.3587522616422));
#237221=CARTESIAN_POINT('Ctrl Pts',(-4.7268268451441,6.35488160224629,52.3428268930438));
#237222=CARTESIAN_POINT('Ctrl Pts',(-4.35455564355918,6.60504552102741,
52.3245429351046));
#237223=CARTESIAN_POINT('Ctrl Pts',(-4.29617994775286,6.6431633425181,52.3217170935278));
#237224=CARTESIAN_POINT('Ctrl Pts',(-4.21856134272978,6.6923952365298,52.3180118225116));
#237225=CARTESIAN_POINT('Ctrl Pts',(-4.19976504114966,6.70420669499665,
52.3171185393061));
#237226=CARTESIAN_POINT('Ctrl Pts',(-4.16912113100334,6.7232836571928,52.3156686985233));
#237227=CARTESIAN_POINT('Ctrl Pts',(-4.1573036904254,6.73059731131467,52.3151111463399));
#237228=CARTESIAN_POINT('Ctrl Pts',(-4.13455535827979,6.74459317698454,
52.3140408670323));
#237229=CARTESIAN_POINT('Ctrl Pts',(-4.12362738917688,6.75128004826359,
52.313528043546));
#237230=CARTESIAN_POINT('Ctrl Pts',(-4.09880695659685,6.76638503156501,
52.3123662772848));
#237231=CARTESIAN_POINT('Ctrl Pts',(-4.08490470061334,6.77478696728526,
52.3117176780363));
#237232=CARTESIAN_POINT('Ctrl Pts',(-4.04502346600183,6.79872211083111,
52.3098631110752));
#237233=CARTESIAN_POINT('Ctrl Pts',(-4.01898101152874,6.81414916370589,
52.3086594167013));
#237234=CARTESIAN_POINT('Ctrl Pts',(-3.8296951341968,6.92481588305789,52.2999633791836));
#237235=CARTESIAN_POINT('Ctrl Pts',(-3.66317036632227,7.01433007826407,
52.2925987961428));
#237236=CARTESIAN_POINT('Ctrl Pts',(-2.90958194048469,7.38525258431442,
52.2604216449909));
#237237=CARTESIAN_POINT('Ctrl Pts',(-2.29236121775071,7.59951780839213,
52.2373624417914));
#237238=CARTESIAN_POINT('Ctrl Pts',(-1.46689762266164,7.77621265400654,
52.2062514874439));
#237239=CARTESIAN_POINT('Ctrl Pts',(-1.27650168421947,7.80972537694599,
52.1990333042836));
#237240=CARTESIAN_POINT('Ctrl Pts',(-0.976792306665396,7.85122590302028,
52.18738148886));
#237241=CARTESIAN_POINT('Ctrl Pts',(-0.868211605161448,7.86397345849996,
52.1831009689399));
#237242=CARTESIAN_POINT('Ctrl Pts',(-0.746308312213926,7.87572968213505,
52.1781972640075));
#237243=CARTESIAN_POINT('Ctrl Pts',(-0.733208381019096,7.87696004750313,
52.1776690375182));
#237244=CARTESIAN_POINT('Ctrl Pts',(-0.713622888995197,7.87875026559636,
52.1768773264857));
#237245=CARTESIAN_POINT('Ctrl Pts',(-0.707139565301127,7.87933480759248,
52.1766149266276));
#237246=CARTESIAN_POINT('Ctrl Pts',(-0.696026919526955,7.88032290714134,
52.1761646011664));
#237247=CARTESIAN_POINT('Ctrl Pts',(-0.691397942095661,7.88073038994905,
52.1759768505676));
#237248=CARTESIAN_POINT('Ctrl Pts',(-0.681899812157914,7.88155806496639,
52.1755912599834));
#237249=CARTESIAN_POINT('Ctrl Pts',(-0.677030623872231,7.88197782409037,
52.1753934005481));
#237250=CARTESIAN_POINT('Ctrl Pts',(-0.665367713300532,7.88297236397686,
52.1749190227701));
#237251=CARTESIAN_POINT('Ctrl Pts',(-0.658573639667189,7.88354287397432,
52.1746423102084));
#237252=CARTESIAN_POINT('Ctrl Pts',(-0.634060227466214,7.88556939753143,
52.173642554381));
#237253=CARTESIAN_POINT('Ctrl Pts',(-0.616336827841533,7.88697445170266,
52.1729171579881));
#237254=CARTESIAN_POINT('Ctrl Pts',(-0.311729396845934,7.91008973390784,
52.1604037149726));
#237255=CARTESIAN_POINT('Ctrl Pts',(-0.02391435518396,7.91619088675665,
52.1478329046686));
#237256=CARTESIAN_POINT('Ctrl Pts',(0.977510641633306,7.88281018681442,
52.1027626971913));
#237257=CARTESIAN_POINT('Ctrl Pts',(1.68507174448236,7.76240544792788,52.0688797087307));
#237258=CARTESIAN_POINT('Ctrl Pts',(2.53646756300021,7.49545597042762,52.0298018758791));
#237259=CARTESIAN_POINT('Ctrl Pts',(2.70427238259385,7.43656128584124,52.022166253564));
#237260=CARTESIAN_POINT('Ctrl Pts',(2.95198964077305,7.34012447839218,52.0110078393031));
#237261=CARTESIAN_POINT('Ctrl Pts',(3.03348492028,7.30682147497035,52.0073554350284));
#237262=CARTESIAN_POINT('Ctrl Pts',(3.1462816874173,7.25851463621045,52.0023252688226));
#237263=CARTESIAN_POINT('Ctrl Pts',(3.17806443065659,7.24465525016644,52.0009107181923));
#237264=CARTESIAN_POINT('Ctrl Pts',(3.22560284890893,7.22355230455932,51.9987990074478));
#237265=CARTESIAN_POINT('Ctrl Pts',(3.24142729942536,7.21646524989355,51.9980967482958));
#237266=CARTESIAN_POINT('Ctrl Pts',(3.26684019746719,7.20498350935541,51.9969700465279));
#237267=CARTESIAN_POINT('Ctrl Pts',(3.27644333771793,7.20062159134022,51.996544530949));
#237268=CARTESIAN_POINT('Ctrl Pts',(3.29477899895547,7.19224893130617,51.9957325439315));
#237269=CARTESIAN_POINT('Ctrl Pts',(3.30351298769402,7.18824145968819,51.9953459659301));
#237270=CARTESIAN_POINT('Ctrl Pts',(3.31895722999937,7.18112098651579,51.9946627378169));
#237271=CARTESIAN_POINT('Ctrl Pts',(3.32567045165565,7.17801447232363,51.9943658746755));
#237272=CARTESIAN_POINT('Ctrl Pts',(3.33887941434223,7.17187957385656,51.9937819970591));
#237273=CARTESIAN_POINT('Ctrl Pts',(3.34537541624781,7.16885176929519,51.9934949638429));
#237274=CARTESIAN_POINT('Ctrl Pts',(3.36278060918614,7.16071035118143,51.9927261886038));
#237275=CARTESIAN_POINT('Ctrl Pts',(3.37368226673752,7.15558062799368,51.9922449790048));
#237276=CARTESIAN_POINT('Ctrl Pts',(3.41321054907595,7.13687036861615,51.9905012627755));
#237277=CARTESIAN_POINT('Ctrl Pts',(3.44176740661182,7.12314270936864,51.9892436298566));
#237278=CARTESIAN_POINT('Ctrl Pts',(3.92755276256321,6.88601588875911,51.9678835700672));
#237279=CARTESIAN_POINT('Ctrl Pts',(4.36227279624529,6.61917924942799,51.9493800873574));
#237280=CARTESIAN_POINT('Ctrl Pts',(4.89769438738188,6.21472233682185,51.9258878440039));
#237281=CARTESIAN_POINT('Ctrl Pts',(5.0239744011972,6.11308973187248,51.9202803036852));
#237282=CARTESIAN_POINT('Ctrl Pts',(5.18469766571331,5.97539032549101,51.9129735383617));
#237283=CARTESIAN_POINT('Ctrl Pts',(5.22204676123818,5.94277772198482,51.9112630277526));
#237284=CARTESIAN_POINT('Ctrl Pts',(5.3117648341662,5.86293849842565,51.9071187742434));
#237285=CARTESIAN_POINT('Ctrl Pts',(5.36381364818646,5.81535868234409,51.9046847813853));
#237286=CARTESIAN_POINT('Ctrl Pts',(5.47329053844085,5.71256135781169,51.8994886808603));
#237287=CARTESIAN_POINT('Ctrl Pts',(5.53053459284019,5.65715949723827,51.8967252600328));
#237288=CARTESIAN_POINT('Ctrl Pts',(5.77390838897745,5.41439277775362,51.8847351329297));
#237289=CARTESIAN_POINT('Ctrl Pts',(5.95142036700782,5.21864452628176,51.8753679638631));
#237290=CARTESIAN_POINT('Ctrl Pts',(6.18032618801816,4.93932286943376,51.8619196615312));
#237291=CARTESIAN_POINT('Ctrl Pts',(6.24046104693437,4.86312523879511,51.8582429853743));
#237292=CARTESIAN_POINT('Ctrl Pts',(6.3479983903071,4.72158344271387,51.8513661567181));
#237293=CARTESIAN_POINT('Ctrl Pts',(6.39583024176179,4.656585439111,51.8481880208492));
#237294=CARTESIAN_POINT('Ctrl Pts',(6.45071896206369,4.57955661949901,51.8444056087554));
#237295=CARTESIAN_POINT('Ctrl Pts',(6.45875024687003,4.56822276210144,51.8438486950927));
#237296=CARTESIAN_POINT('Ctrl Pts',(6.47099413354621,4.55084719267143,51.8429943997299));
#237297=CARTESIAN_POINT('Ctrl Pts',(6.47522824206945,4.54482061913332,51.8426980010337));
#237298=CARTESIAN_POINT('Ctrl Pts',(6.48259137154624,4.53430921024349,51.8421808781726));
#237299=CARTESIAN_POINT('Ctrl Pts',(6.48572417383986,4.52982702155779,51.8419603231061));
#237300=CARTESIAN_POINT('Ctrl Pts',(6.49225865331545,4.52045728196455,51.8414991721101));
#237301=CARTESIAN_POINT('Ctrl Pts',(6.49565946376103,4.51556913248198,51.8412585383494));
#237302=CARTESIAN_POINT('Ctrl Pts',(6.50503278325136,4.5020639060141,51.8405935652216));
#237303=CARTESIAN_POINT('Ctrl Pts',(6.51099367508337,4.49343880416742,51.8401687258356));
#237304=CARTESIAN_POINT('Ctrl Pts',(6.53425575421329,4.45963630486868,51.83850321145));
#237305=CARTESIAN_POINT('Ctrl Pts',(6.55142807729838,4.43437079552155,51.837257177257));
#237306=CARTESIAN_POINT('Ctrl Pts',(6.64990642672224,4.28765964077672,51.8300176659102));
#237307=CARTESIAN_POINT('Ctrl Pts',(6.72797896751328,4.16408181112704,51.823904307414));
#237308=CARTESIAN_POINT('Ctrl Pts',(6.9672158290295,3.76109508051637,51.8040607910132));
#237309=CARTESIAN_POINT('Ctrl Pts',(7.11473596704962,3.47396898476637,51.7900756821757));
#237310=CARTESIAN_POINT('Ctrl Pts',(7.44418052249601,2.72314570911304,51.7546708600605));
#237311=CARTESIAN_POINT('Ctrl Pts',(7.60064637513865,2.24979198825484,51.7334824488672));
#237312=CARTESIAN_POINT('Ctrl Pts',(7.79054781880554,1.42001356373868,51.6981947477973));
#237313=CARTESIAN_POINT('Ctrl Pts',(7.84625115385763,1.07024531693852,51.6837709687419));
#237314=CARTESIAN_POINT('Ctrl Pts',(7.88379256174759,0.65827318731429,51.6670194868207));
#237315=CARTESIAN_POINT('Ctrl Pts',(7.88855067119788,0.598562532219954,
51.6645990538531));
#237316=CARTESIAN_POINT('Ctrl Pts',(7.89467671610254,0.508825519669789,
51.6609726823818));
#237317=CARTESIAN_POINT('Ctrl Pts',(7.89655239903012,0.478836169824792,
51.6597626541195));
#237318=CARTESIAN_POINT('Ctrl Pts',(7.89949520658906,0.427051087437223,
51.6576763967149));
#237319=CARTESIAN_POINT('Ctrl Pts',(7.9006430899164,0.405260309788896,51.6567994916115));
#237320=CARTESIAN_POINT('Ctrl Pts',(7.90283589571974,0.360075236898814,
51.6549831519664));
#237321=CARTESIAN_POINT('Ctrl Pts',(7.90386713118382,0.336680481965398,
51.6540438452353));
#237322=CARTESIAN_POINT('Ctrl Pts',(7.90640606694132,0.272617432871721,
51.6514746819227));
#237323=CARTESIAN_POINT('Ctrl Pts',(7.90770385976311,0.231941468414489,
51.6498467243587));
#237324=CARTESIAN_POINT('Ctrl Pts',(7.91157557022579,0.0718421331945126,
51.6434515960189));
#237325=CARTESIAN_POINT('Ctrl Pts',(7.91175844709219,-0.047623919068554,
51.6387070502196));
#237326=CARTESIAN_POINT('Ctrl Pts',(7.90128752924617,-0.543387775044297,
51.6191102104846));
#237327=CARTESIAN_POINT('Ctrl Pts',(7.86648873491408,-0.91868269334451,
51.6045173183823));
#237328=CARTESIAN_POINT('Ctrl Pts',(7.74402111267489,-1.659624852261,51.5754834897492));
#237329=CARTESIAN_POINT('Ctrl Pts',(7.65677288121044,-2.02436018172972,
51.5610749480961));
#237330=CARTESIAN_POINT('Ctrl Pts',(7.5209905695871,-2.45448035999185,51.5432166453439));
#237331=CARTESIAN_POINT('Ctrl Pts',(7.49690482399161,-2.52709137195962,
51.5401705141228));
#237332=CARTESIAN_POINT('Ctrl Pts',(7.4653922553341,-2.6176738239576,51.5363232668059));
#237333=CARTESIAN_POINT('Ctrl Pts',(7.45894699663908,-2.63598320771407,
51.5355431878288));
#237334=CARTESIAN_POINT('Ctrl Pts',(7.44859284998366,-2.66505471852185,
51.5343005414809));
#237335=CARTESIAN_POINT('Ctrl Pts',(7.44472785746868,-2.67583243585648,
51.5338389677733));
#237336=CARTESIAN_POINT('Ctrl Pts',(7.43776005159926,-2.69513054207825,
51.5330108675046));
#237337=CARTESIAN_POINT('Ctrl Pts',(7.4346659584296,-2.70365406627205,51.5326445450864));
#237338=CARTESIAN_POINT('Ctrl Pts',(7.4273961559404,-2.72357387535458,51.5317870771952));
#237339=CARTESIAN_POINT('Ctrl Pts',(7.42320886504025,-2.73496589677564,
51.5312956552408));
#237340=CARTESIAN_POINT('Ctrl Pts',(7.41111685825313,-2.76763128935859,
51.5298834922547));
#237341=CARTESIAN_POINT('Ctrl Pts',(7.40314685501238,-2.78888018209056,
51.5289611020241));
#237342=CARTESIAN_POINT('Ctrl Pts',(7.34143011282637,-2.95129486509077,
51.5218825882311));
#237343=CARTESIAN_POINT('Ctrl Pts',(7.28374256217901,-3.090927042738,51.5156341740384));
#237344=CARTESIAN_POINT('Ctrl Pts',(7.02163824453983,-3.67719158960518,
51.488845155229));
#237345=CARTESIAN_POINT('Ctrl Pts',(6.77986210960784,-4.10592567801498,
51.4679287301087));
#237346=CARTESIAN_POINT('Ctrl Pts',(6.40063454518289,-4.65253886377285,
51.4402212244242));
#237347=CARTESIAN_POINT('Ctrl Pts',(6.29668123735791,-4.79229044014567,
51.4330262054818));
#237348=CARTESIAN_POINT('Ctrl Pts',(6.12043744610999,-5.0135812573942,51.4214460702434));
#237349=CARTESIAN_POINT('Ctrl Pts',(6.05092738978183,-5.09725708149458,
51.4170208994315));
#237350=CARTESIAN_POINT('Ctrl Pts',(5.95753905595361,-5.20507410811285,
51.411252632427));
#237351=CARTESIAN_POINT('Ctrl Pts',(5.93520051408025,-5.23053180335807,
51.4098856193712));
#237352=CARTESIAN_POINT('Ctrl Pts',(5.89835553087223,-5.27198151988611,
51.4076513758338));
#237353=CARTESIAN_POINT('Ctrl Pts',(5.88394592914525,-5.28805894644538,
51.4067826405154));
#237354=CARTESIAN_POINT('Ctrl Pts',(5.85591278059868,-5.31908031668289,
51.4051022089783));
#237355=CARTESIAN_POINT('Ctrl Pts',(5.84229739692514,-5.33403140580243,
51.4042903933297));
#237356=CARTESIAN_POINT('Ctrl Pts',(5.81067518429199,-5.36848951386144,
51.4024148543552));
#237357=CARTESIAN_POINT('Ctrl Pts',(5.79262717438009,-5.38795844293858,
51.4013517826696));
#237358=CARTESIAN_POINT('Ctrl Pts',(5.7337422832019,-5.45084147816368,51.3979068017594));
#237359=CARTESIAN_POINT('Ctrl Pts',(5.69251255569761,-5.49388517007,51.3955310038168));
#237360=CARTESIAN_POINT('Ctrl Pts',(5.34877993184729,-5.84471669441425,
51.3760094943302));
#237361=CARTESIAN_POINT('Ctrl Pts',(5.02202823518501,-6.12775747677063,
51.359168774521));
#237362=CARTESIAN_POINT('Ctrl Pts',(4.60152081278964,-6.43567854055421,
51.339091794929));
#237363=CARTESIAN_POINT('Ctrl Pts',(4.52832205492248,-6.48739174265638,
51.3356534581524));
#237364=CARTESIAN_POINT('Ctrl Pts',(4.01477254559888,-6.83727479690381,
51.3119056257524));
#237365=CARTESIAN_POINT('Ctrl Pts',(3.54622064757126,-7.09161757516245,
51.2922487525006));
#237366=CARTESIAN_POINT('Ctrl Pts',(2.83935122829312,-7.3876262975815,51.2634266808514));
#237367=CARTESIAN_POINT('Ctrl Pts',(2.61908206399757,-7.46855679499356,
51.2545316589161));
#237368=CARTESIAN_POINT('Ctrl Pts',(2.3024685659512,-7.5691544096621,51.2415801466397));
#237369=CARTESIAN_POINT('Ctrl Pts',(2.20884847374301,-7.59700254168023,
51.2377299068452));
#237370=CARTESIAN_POINT('Ctrl Pts',(2.09955003299581,-7.62732319452465,
51.2331916124215));
#237371=CARTESIAN_POINT('Ctrl Pts',(2.08434869705361,-7.63149133263188,
51.2325594542538));
#237372=CARTESIAN_POINT('Ctrl Pts',(2.06118168039161,-7.63776924120068,
51.2315944538325));
#237373=CARTESIAN_POINT('Ctrl Pts',(2.05322494974195,-7.63991205489974,
51.2312627396126));
#237374=CARTESIAN_POINT('Ctrl Pts',(2.03878084370208,-7.64377777841625,
51.2306600339215));
#237375=CARTESIAN_POINT('Ctrl Pts',(2.03229459027209,-7.64550487230856,
51.2303891883007));
#237376=CARTESIAN_POINT('Ctrl Pts',(2.01834559425839,-7.64920006459119,
51.2298062899027));
#237377=CARTESIAN_POINT('Ctrl Pts',(2.01088215753811,-7.65116550036741,
51.2294941434126));
#237378=CARTESIAN_POINT('Ctrl Pts',(1.99082946846771,-7.65641484645382,
51.2286547347505));
#237379=CARTESIAN_POINT('Ctrl Pts',(1.97823500038386,-7.65967861952292,
51.2281267493803));
#237380=CARTESIAN_POINT('Ctrl Pts',(1.92077462569151,-7.67441792425526,
51.225714153871));
#237381=CARTESIAN_POINT('Ctrl Pts',(1.87581709643743,-7.68553028374534,
51.2238161303691));
#237382=CARTESIAN_POINT('Ctrl Pts',(1.06177608986239,-7.87917245035684,
51.1892267695536));
#237383=CARTESIAN_POINT('Ctrl Pts',(0.269832480310142,-7.94579192008655,
51.1514267204623));
#237384=CARTESIAN_POINT('Ctrl Pts',(-0.90906387391072,-7.86832581836317,
51.0984082166215));
#237385=CARTESIAN_POINT('Ctrl Pts',(-1.29699672823081,-7.81375717549953,
51.0814342310139));
#237386=CARTESIAN_POINT('Ctrl Pts',(-1.73960975791977,-7.71760865638512,
51.0628256688525));
#237387=CARTESIAN_POINT('Ctrl Pts',(-1.79973014518173,-7.70381055776497,
51.0603136254667));
#237388=CARTESIAN_POINT('Ctrl Pts',(-1.87378158119324,-7.68590098525529,
51.0572383253472));
#237389=CARTESIAN_POINT('Ctrl Pts',(-1.88786988639595,-7.68245264639402,
51.0566540927801));
#237390=CARTESIAN_POINT('Ctrl Pts',(-1.91001542900665,-7.67696757355624,
51.0557370494918));
#237391=CARTESIAN_POINT('Ctrl Pts',(-1.91807904306189,-7.67495686304351,
51.0554034117045));
#237392=CARTESIAN_POINT('Ctrl Pts',(-1.93240428508631,-7.67136079192476,
51.054811181186));
#237393=CARTESIAN_POINT('Ctrl Pts',(-1.93866716185656,-7.66978046339651,
51.0545524283822));
#237394=CARTESIAN_POINT('Ctrl Pts',(-1.95312099129079,-7.66611445485102,
51.0539556441));
#237395=CARTESIAN_POINT('Ctrl Pts',(-1.96131055747216,-7.66402331280451,
51.0536177872915));
#237396=CARTESIAN_POINT('Ctrl Pts',(-1.98377329884904,-7.65824926371994,
51.0526918672706));
#237397=CARTESIAN_POINT('Ctrl Pts',(-1.99803958857213,-7.65453957413411,
51.0521046611031));
#237398=CARTESIAN_POINT('Ctrl Pts',(-2.06798410911439,-7.63614290635203,
51.049229861381));
#237399=CARTESIAN_POINT('Ctrl Pts',(-2.12351186249019,-7.62088802616805,
51.0469605243978));
#237400=CARTESIAN_POINT('Ctrl Pts',(-3.03593058252707,-7.35947666308705,
51.0098728557065));
#237401=CARTESIAN_POINT('Ctrl Pts',(-3.84521275693607,-6.9708696223835,
50.9808530086722));
#237402=CARTESIAN_POINT('Ctrl Pts',(-4.74724961333479,-6.33192697228394,
50.9425893048823));
#237403=CARTESIAN_POINT('Ctrl Pts',(-4.91671148246358,-6.201259475936,50.9350463544984));
#237404=CARTESIAN_POINT('Ctrl Pts',(-5.2124228427832,-5.95349620170652,
50.9208638412435));
#237405=CARTESIAN_POINT('Ctrl Pts',(-5.34054242286951,-5.83884140076207,
50.9143409400278));
#237406=CARTESIAN_POINT('Ctrl Pts',(-5.4836107516599,-5.70215832806318,
50.9064833612311));
#237407=CARTESIAN_POINT('Ctrl Pts',(-5.50231415306876,-5.68411254336957,
50.9054443874267));
#237408=CARTESIAN_POINT('Ctrl Pts',(-5.52609699011638,-5.66093853883887,
50.9041076843781));
#237409=CARTESIAN_POINT('Ctrl Pts',(-5.53125898143786,-5.65589490392956,
50.903816613114));
#237410=CARTESIAN_POINT('Ctrl Pts',(-5.53952835788207,-5.64779298321426,
50.9033487951516));
#237411=CARTESIAN_POINT('Ctrl Pts',(-5.54264013911168,-5.64473916998709,
50.9031724059919));
#237412=CARTESIAN_POINT('Ctrl Pts',(-5.54853717681745,-5.63894240784062,
50.9028374717575));
#237413=CARTESIAN_POINT('Ctrl Pts',(-5.55132292894481,-5.63619996273505,
50.9026789673142));
#237414=CARTESIAN_POINT('Ctrl Pts',(-5.5576342470128,-5.62997754137028,
50.902319221579));
#237415=CARTESIAN_POINT('Ctrl Pts',(-5.56115857629428,-5.6264963191132,
50.9021178788941));
#237416=CARTESIAN_POINT('Ctrl Pts',(-5.57021161430208,-5.61753719578666,
50.9015995054334));
#237417=CARTESIAN_POINT('Ctrl Pts',(-5.57573551316179,-5.61205444211983,
50.9012820757323));
#237418=CARTESIAN_POINT('Ctrl Pts',(-5.60981800342172,-5.5781258257499,
50.8993164612047));
#237419=CARTESIAN_POINT('Ctrl Pts',(-5.63816642790486,-5.54947069324606,
50.8976508544256));
#237420=CARTESIAN_POINT('Ctrl Pts',(-6.25134430504331,-4.92011052168407,
50.8609791270086));
#237421=CARTESIAN_POINT('Ctrl Pts',(-6.73724408125472,-4.23043507993487,
50.8197042175227));
#237422=CARTESIAN_POINT('Ctrl Pts',(-7.27560593288448,-3.1302872266117,
50.7647930121821));
#237423=CARTESIAN_POINT('Ctrl Pts',(-7.41976997593545,-2.77131964628872,
50.7482090714532));
#237424=CARTESIAN_POINT('Ctrl Pts',(-7.54348847028449,-2.38330429577554,
50.7317554182434));
#237425=CARTESIAN_POINT('Ctrl Pts',(-7.54975758804608,-2.36337005962162,
50.7309139765251));
#237426=CARTESIAN_POINT('Ctrl Pts',(-7.55865880549966,-2.33466953280044,
50.7297080135697));
#237427=CARTESIAN_POINT('Ctrl Pts',(-7.56135476331092,-2.32592323808961,
50.7293412386578));
#237428=CARTESIAN_POINT('Ctrl Pts',(-7.56600764361138,-2.31073465995964,
50.7287055770043));
#237429=CARTESIAN_POINT('Ctrl Pts',(-7.56797152810201,-2.30429453023421,
50.7284364449191));
#237430=CARTESIAN_POINT('Ctrl Pts',(-7.57173192344728,-2.29190647376306,
50.7279195084701));
#237431=CARTESIAN_POINT('Ctrl Pts',(-7.57352965271673,-2.28595892453885,
50.7276716613336));
#237432=CARTESIAN_POINT('Ctrl Pts',(-7.57774795541946,-2.27194363299604,
50.7270884030425));
#237433=CARTESIAN_POINT('Ctrl Pts',(-7.58016265699817,-2.26387412226327,
50.7267531987912));
#237434=CARTESIAN_POINT('Ctrl Pts',(-7.58846382173659,-2.23597089688677,
50.7255962282729));
#237435=CARTESIAN_POINT('Ctrl Pts',(-7.59428539129238,-2.21611787368668,
50.7247767449108));
#237436=CARTESIAN_POINT('Ctrl Pts',(-7.65879440192245,-1.9928864065297,
50.7156033858462));
#237437=CARTESIAN_POINT('Ctrl Pts',(-7.7093765445267,-1.7872464436281,50.707539029237));
#237438=CARTESIAN_POINT('Ctrl Pts',(-7.80701268840627,-1.30817640644099,
50.6894926242977));
#237439=CARTESIAN_POINT('Ctrl Pts',(-7.8480587307184,-1.03380809376537,
50.679706509675));
#237440=CARTESIAN_POINT('Ctrl Pts',(-7.89918585906256,-0.502552382104667,
50.6613253803921));
#237441=CARTESIAN_POINT('Ctrl Pts',(-7.91132569102394,-0.246219205752182,
50.6527051770111));
#237442=CARTESIAN_POINT('Ctrl Pts',(-7.91032769265032,0.523963540078032,
50.6266919225513));
#237443=CARTESIAN_POINT('Ctrl Pts',(-7.85962538591528,1.03633015157118,
50.6092764726127));
#237444=CARTESIAN_POINT('Ctrl Pts',(-7.75324523613621,1.57231962172495,
50.5877143879113));
#237445=CARTESIAN_POINT('Ctrl Pts',(-7.7466477853958,1.60450886891474,50.5864061596295));
#237446=CARTESIAN_POINT('Ctrl Pts',(-7.73838202077217,1.64359820378141,
50.5848002522428));
#237447=CARTESIAN_POINT('Ctrl Pts',(-7.73690461505836,1.65053880043261,
50.5845144492266));
#237448=CARTESIAN_POINT('Ctrl Pts',(-7.73445736620318,1.66196006796274,
50.5840430340289));
#237449=CARTESIAN_POINT('Ctrl Pts',(-7.73349296506658,1.666441890976,50.5838577649383));
#237450=CARTESIAN_POINT('Ctrl Pts',(-7.73174200886593,1.67454478566484,
50.5835223020355));
#237451=CARTESIAN_POINT('Ctrl Pts',(-7.73095680422824,1.67816614848497,
50.583372193434));
#237452=CARTESIAN_POINT('Ctrl Pts',(-7.72926968647717,1.68592082003794,
50.5830503661171));
#237453=CARTESIAN_POINT('Ctrl Pts',(-7.72836700197534,1.69005395782781,
50.5828785992936));
#237454=CARTESIAN_POINT('Ctrl Pts',(-7.72591061183009,1.70125795491553,
50.5824123394205));
#237455=CARTESIAN_POINT('Ctrl Pts',(-7.72435051820062,1.70832739321897,
50.582117450894));
#237456=CARTESIAN_POINT('Ctrl Pts',(-7.71653395414529,1.74351790172649,
50.5806461412921));
#237457=CARTESIAN_POINT('Ctrl Pts',(-7.71013368762364,1.77160645033107,
50.5794609390703));
#237458=CARTESIAN_POINT('Ctrl Pts',(-7.65421224601727,2.01098252167035,
50.5692717990256));
#237459=CARTESIAN_POINT('Ctrl Pts',(-7.59617324761271,2.22016964899762,
50.5597788778296));
#237460=CARTESIAN_POINT('Ctrl Pts',(-7.36614410463515,2.93391204623333,
50.5259758079177));
#237461=CARTESIAN_POINT('Ctrl Pts',(-7.15184277494405,3.42331255617383,
50.5003941302939));
#237462=CARTESIAN_POINT('Ctrl Pts',(-6.71616940725617,4.195483196243,50.4592358935602));
#237463=CARTESIAN_POINT('Ctrl Pts',(-6.52189909727086,4.49153442503722,
50.443210103376));
#237464=CARTESIAN_POINT('Ctrl Pts',(-6.17042207143741,4.95602026962088,
50.4180132197873));
#237465=CARTESIAN_POINT('Ctrl Pts',(-6.02454086189876,5.13236446589125,
50.4084264138683));
#237466=CARTESIAN_POINT('Ctrl Pts',(-5.85661189252792,5.31831671592667,
50.3982802325562));
#237467=CARTESIAN_POINT('Ctrl Pts',(-5.84194479643378,5.33442373235327,
50.3974010176935));
#237468=CARTESIAN_POINT('Ctrl Pts',(-5.82124448762606,5.35696849418104,
50.3961698295652));
#237469=CARTESIAN_POINT('Ctrl Pts',(-5.81526682006235,5.36345696771227,
50.3958154225556));
#237470=CARTESIAN_POINT('Ctrl Pts',(-5.80487224623932,5.37470197666532,
50.3952010890919));
#237471=CARTESIAN_POINT('Ctrl Pts',(-5.80046032227125,5.37946309432187,
50.3949409439696));
#237472=CARTESIAN_POINT('Ctrl Pts',(-5.79126625361084,5.38936039143677,
50.3944000802879));
#237473=CARTESIAN_POINT('Ctrl Pts',(-5.7864831229754,5.39449564990703,50.3941194055393));
#237474=CARTESIAN_POINT('Ctrl Pts',(-5.77520142776797,5.40657561943629,
50.3934590479722));
#237475=CARTESIAN_POINT('Ctrl Pts',(-5.76869715321432,5.41351499631357,
50.3930796176615));
#237476=CARTESIAN_POINT('Ctrl Pts',(-5.74738455181556,5.43617127392764,
50.3918405270949));
#237477=CARTESIAN_POINT('Ctrl Pts',(-5.7325243251148,5.45183933894015,50.3909831642796));
#237478=CARTESIAN_POINT('Ctrl Pts',(-5.44128433838478,5.75640451034283,
50.3743072158344));
#237479=CARTESIAN_POINT('Ctrl Pts',(-5.14344727488068,6.02401543239919,
50.3595204759108));
#237480=CARTESIAN_POINT('Ctrl Pts',(-4.62814530654299,6.42082155355519,
50.336419023468));
#237481=CARTESIAN_POINT('Ctrl Pts',(-4.42250903761971,6.5641523383706,50.3277523745125));
#237482=CARTESIAN_POINT('Ctrl Pts',(-3.99799616288946,6.83102501461066,
50.3104519248722));
#237483=CARTESIAN_POINT('Ctrl Pts',(-3.77934687143073,6.95438056092077,
50.3018271641067));
#237484=CARTESIAN_POINT('Ctrl Pts',(-3.25510236948542,7.21810828926355,
50.2810986754919));
#237485=CARTESIAN_POINT('Ctrl Pts',(-2.94568074263968,7.34981325299562,
50.2687920465069));
#237486=CARTESIAN_POINT('Ctrl Pts',(-2.60622576986852,7.46940972956807,
50.2544547284584));
#237487=CARTESIAN_POINT('Ctrl Pts',(-2.58360347089448,7.47726471109727,
50.2534961952832));
#237488=CARTESIAN_POINT('Ctrl Pts',(-2.55215747470383,7.48802373825333,
50.2521598443616));
#237489=CARTESIAN_POINT('Ctrl Pts',(-2.54336365864591,7.49101519016262,
50.2517857089474));
#237490=CARTESIAN_POINT('Ctrl Pts',(-2.52928229843265,7.49577768810581,
50.2511859487729));
#237491=CARTESIAN_POINT('Ctrl Pts',(-2.52399809898363,7.4975586487069,50.2509607319681));
#237492=CARTESIAN_POINT('Ctrl Pts',(-2.513668312286,7.50102799117831,50.2505201808872));
#237493=CARTESIAN_POINT('Ctrl Pts',(-2.50862289542961,7.5027168730374,50.2503048670463));
#237494=CARTESIAN_POINT('Ctrl Pts',(-2.49647650735981,7.50676908246108,
50.2497862016411));
#237495=CARTESIAN_POINT('Ctrl Pts',(-2.48937388533346,7.50912742385825,
50.249482650873));
#237496=CARTESIAN_POINT('Ctrl Pts',(-2.46779454181345,7.5162586075214,50.2485596246148));
#237497=CARTESIAN_POINT('Ctrl Pts',(-2.45330740933709,7.5209996747131,50.2479389042245));
#237498=CARTESIAN_POINT('Ctrl Pts',(-2.31130353353664,7.56701799353016,
50.2418447492537));
#237499=CARTESIAN_POINT('Ctrl Pts',(-2.18277465488257,7.60508894715016,
50.2362517768322));
#237500=CARTESIAN_POINT('Ctrl Pts',(-1.80580541054453,7.70640577991665,
50.2197201771648));
#237501=CARTESIAN_POINT('Ctrl Pts',(-1.55518467560398,7.76086443556248,
50.2085741784437));
#237502=CARTESIAN_POINT('Ctrl Pts',(-0.875789659399663,7.87425898133527,
50.1784472665762));
#237503=CARTESIAN_POINT('Ctrl Pts',(-0.444071036561553,7.91035947100023,
50.1594314781763));
#237504=CARTESIAN_POINT('Ctrl Pts',(0.339512619627885,7.91150462062581,
50.1259458845519));
#237505=CARTESIAN_POINT('Ctrl Pts',(0.690244517435434,7.88864753255679,
50.1113200870908));
#237506=CARTESIAN_POINT('Ctrl Pts',(1.07380501108117,7.83786612837951,50.0956499447213));
#237507=CARTESIAN_POINT('Ctrl Pts',(1.10926335960438,7.83292649469544,50.0942041296534));
#237508=CARTESIAN_POINT('Ctrl Pts',(1.1617684254719,7.82524843939604,50.0920672925894));
#237509=CARTESIAN_POINT('Ctrl Pts',(1.17884161369433,7.82269464220956,50.0913730977716));
#237510=CARTESIAN_POINT('Ctrl Pts',(1.2079903140451,7.81823700321695,50.0901890231708));
#237511=CARTESIAN_POINT('Ctrl Pts',(1.22007000279372,7.81636102202077,50.0896986495944));
#237512=CARTESIAN_POINT('Ctrl Pts',(1.24478919109654,7.81246342147455,50.0886958462254));
#237513=CARTESIAN_POINT('Ctrl Pts',(1.25742823206002,7.81043910958335,50.0881834665638));
#237514=CARTESIAN_POINT('Ctrl Pts',(1.28652792164341,7.80570593830926,50.0870046085689));
#237515=CARTESIAN_POINT('Ctrl Pts',(1.30298504155243,7.80297566781858,50.0863385241983));
#237516=CARTESIAN_POINT('Ctrl Pts',(1.35434261323166,7.79428833221164,50.0842617858416));
#237517=CARTESIAN_POINT('Ctrl Pts',(1.38921191795744,7.78814899648283,50.0828545323641));
#237518=CARTESIAN_POINT('Ctrl Pts',(1.46904279405581,7.77354021242246,50.0796389625636));
#237519=CARTESIAN_POINT('Ctrl Pts',(1.51397456855761,7.76491437330063,50.0778336754279));
#237520=CARTESIAN_POINT('Ctrl Pts',(1.94820642981538,7.67763972927537,50.0604295725632));
#237521=CARTESIAN_POINT('Ctrl Pts',(2.33114609284802,7.57016807343126,50.0454590821063));
#237522=CARTESIAN_POINT('Ctrl Pts',(3.04024702424708,7.31221771313176,50.0176853393892));
#237523=CARTESIAN_POINT('Ctrl Pts',(3.36741183720351,7.16743774627461,50.0048379230262));
#237524=CARTESIAN_POINT('Ctrl Pts',(3.91557611398751,6.87901567254248,49.9821106534605));
#237525=CARTESIAN_POINT('Ctrl Pts',(4.14127072079178,6.74555090909402,49.9723595492534));
#237526=CARTESIAN_POINT('Ctrl Pts',(4.3658750952618,6.5972044594386,49.9618747626815));
#237527=CARTESIAN_POINT('Ctrl Pts',(4.3718303212097,6.59325956331433,49.9615961788359));
#237528=CARTESIAN_POINT('Ctrl Pts',(4.39809625028165,6.57580909840806,49.9603648368023));
#237529=CARTESIAN_POINT('Ctrl Pts',(4.41834964992846,6.56221778673381,49.9594084116411));
#237530=CARTESIAN_POINT('Ctrl Pts',(4.46446058030299,6.53096419255763,49.9572142770302));
#237531=CARTESIAN_POINT('Ctrl Pts',(4.49027664649578,6.51324167822048,49.9559738027848));
#237532=CARTESIAN_POINT('Ctrl Pts',(4.53292881850131,6.48358721069017,49.9539031571463));
#237533=CARTESIAN_POINT('Ctrl Pts',(4.54982480756593,6.47174172857735,49.9530773339777));
#237534=CARTESIAN_POINT('Ctrl Pts',(4.57313044412891,6.45526618014219,49.951930232073));
#237535=CARTESIAN_POINT('Ctrl Pts',(4.57957987954209,6.45069233817113,49.9516119402214));
#237536=CARTESIAN_POINT('Ctrl Pts',(4.59036357911497,6.44302037834353,49.9510782996455));
#237537=CARTESIAN_POINT('Ctrl Pts',(4.59470159928951,6.43992753045374,49.9508632367408));
#237538=CARTESIAN_POINT('Ctrl Pts',(4.60318894763311,6.43386342392706,49.9504416903345));
#237539=CARTESIAN_POINT('Ctrl Pts',(4.60733853208254,6.43089252716621,49.9502352267515));
#237540=CARTESIAN_POINT('Ctrl Pts',(4.61717853573062,6.42383315986144,49.9497447644865));
#237541=CARTESIAN_POINT('Ctrl Pts',(4.62286639700492,6.41974114521041,49.9494605684063));
#237542=CARTESIAN_POINT('Ctrl Pts',(4.64131950506261,6.40642819591742,49.9485362775669));
#237543=CARTESIAN_POINT('Ctrl Pts',(4.65406259942769,6.3971767438836,49.9478944524473));
#237544=CARTESIAN_POINT('Ctrl Pts',(4.96909121374221,6.16702732253397,49.9319374506794));
#237545=CARTESIAN_POINT('Ctrl Pts',(5.25529737093517,5.92501932603227,49.9152954905421));
#237546=CARTESIAN_POINT('Ctrl Pts',(6.0141038076308,5.18503071401614,49.866980091659));
#237547=CARTESIAN_POINT('Ctrl Pts',(6.44071774748014,4.64449558108511,49.8347778215324));
#237548=CARTESIAN_POINT('Ctrl Pts',(6.91942068029469,3.84279043986989,49.7943738339742));
#237549=CARTESIAN_POINT('Ctrl Pts',(7.03648185979773,3.62399751143469,49.7839603918511));
#237550=CARTESIAN_POINT('Ctrl Pts',(7.15319544314933,3.37879714129683,49.7729410966472));
#237551=CARTESIAN_POINT('Ctrl Pts',(7.16321812964198,3.35749627089562,49.7719890155991));
#237552=CARTESIAN_POINT('Ctrl Pts',(7.17717621177664,3.32748463169668,49.7706548071203));
#237553=CARTESIAN_POINT('Ctrl Pts',(7.18119108074594,3.31881108405622,49.7702700568691));
#237554=CARTESIAN_POINT('Ctrl Pts',(7.18813635264969,3.3037352121519,49.76960276584));
#237555=CARTESIAN_POINT('Ctrl Pts',(7.19107394113495,3.29733622030934,49.7693199883963));
#237556=CARTESIAN_POINT('Ctrl Pts',(7.19717339632518,3.28400276903716,49.7687317171701));
#237557=CARTESIAN_POINT('Ctrl Pts',(7.20033379407984,3.27706764319233,49.7684262719303));
#237558=CARTESIAN_POINT('Ctrl Pts',(7.20776052589805,3.26070793313679,49.7677069879225));
#237559=CARTESIAN_POINT('Ctrl Pts',(7.21201840912271,3.25127951603576,49.7672934271915));
#237560=CARTESIAN_POINT('Ctrl Pts',(7.22591258531051,3.22035144058372,49.7659400070756));
#237561=CARTESIAN_POINT('Ctrl Pts',(7.23547136949463,3.1988169945158,49.7650026905068));
#237562=CARTESIAN_POINT('Ctrl Pts',(7.40862836498946,2.80397399893836,49.7479076508804));
#237563=CARTESIAN_POINT('Ctrl Pts',(7.54323930083466,2.4186009739306,49.7327504839495));
#237564=CARTESIAN_POINT('Ctrl Pts',(7.79928066207843,1.45142122964752,49.6970409681734));
#237565=CARTESIAN_POINT('Ctrl Pts',(7.8860908278076,0.863095349536447,49.6773337288548));
#237566=CARTESIAN_POINT('Ctrl Pts',(7.91712013831398,-0.043457692133003,
49.6449984011458));
#237567=CARTESIAN_POINT('Ctrl Pts',(7.90914648703363,-0.357892497832621,
49.6333669545769));
#237568=CARTESIAN_POINT('Ctrl Pts',(7.88076924122621,-0.69123696655325,
49.6200404118277));
#237569=CARTESIAN_POINT('Ctrl Pts',(7.87897113862675,-0.71143950147839,
49.6192293731651));
#237570=CARTESIAN_POINT('Ctrl Pts',(7.8762942947089,-0.74025955699584,49.618067759341));
#237571=CARTESIAN_POINT('Ctrl Pts',(7.87547905122072,-0.748882995955991,
49.6177195943124));
#237572=CARTESIAN_POINT('Ctrl Pts',(7.87405953616969,-0.763639575587852,
49.6171228149721));
#237573=CARTESIAN_POINT('Ctrl Pts',(7.87346225656381,-0.769773391818883,
49.6168744599458));
#237574=CARTESIAN_POINT('Ctrl Pts',(7.87225261495514,-0.782047211500224,
49.6163769188983));
#237575=CARTESIAN_POINT('Ctrl Pts',(7.87164023553197,-0.788187209220541,
49.6161277323885));
#237576=CARTESIAN_POINT('Ctrl Pts',(7.87012323044885,-0.803219288305605,
49.6155169655765));
#237577=CARTESIAN_POINT('Ctrl Pts',(7.86921071864419,-0.812110554272524,
49.6151551031322));
#237578=CARTESIAN_POINT('Ctrl Pts',(7.8659644398614,-0.843222166176726,
49.6138868343835));
#237579=CARTESIAN_POINT('Ctrl Pts',(7.86355162024573,-0.865434049971041,
49.6129776706834));
#237580=CARTESIAN_POINT('Ctrl Pts',(7.8171417592864,-1.27644744821703,49.5960891600648));
#237581=CARTESIAN_POINT('Ctrl Pts',(7.74445422984662,-1.66145453306334,
49.5792278055125));
#237582=CARTESIAN_POINT('Ctrl Pts',(7.5756321974535,-2.29416606638227,49.5509413922721));
#237583=CARTESIAN_POINT('Ctrl Pts',(7.49499028326708,-2.54529469133629,
49.5395459001544));
#237584=CARTESIAN_POINT('Ctrl Pts',(7.17778260874517,-3.38627525119422,
49.5010973471223));
#237585=CARTESIAN_POINT('Ctrl Pts',(6.88283161453795,-3.95146852869857,
49.4749551106286));
#237586=CARTESIAN_POINT('Ctrl Pts',(6.47433691152503,-4.54691360091522,
49.4456352480798));
#237587=CARTESIAN_POINT('Ctrl Pts',(6.42403646834625,-4.6177069351777,49.4421189710503));
#237588=CARTESIAN_POINT('Ctrl Pts',(6.35353751303947,-4.71354589265816,
49.4373167914929));
#237589=CARTESIAN_POINT('Ctrl Pts',(6.33433691373511,-4.73931742800615,
49.4360212169839));
#237590=CARTESIAN_POINT('Ctrl Pts',(6.30111903086722,-4.78334083237742,
49.4338007401467));
#237591=CARTESIAN_POINT('Ctrl Pts',(6.28717818388037,-4.80164982554388,
49.4328750536705));
#237592=CARTESIAN_POINT('Ctrl Pts',(6.25826854996638,-4.83927607814003,
49.4309681127715));
#237593=CARTESIAN_POINT('Ctrl Pts',(6.24328973703541,-4.85858533600675,
49.4299869785863));
#237594=CARTESIAN_POINT('Ctrl Pts',(6.20812014753273,-4.90349141679698,
49.4276992833118));
#237595=CARTESIAN_POINT('Ctrl Pts',(6.18786011692474,-4.92903347762713,
49.42639351928));
#237596=CARTESIAN_POINT('Ctrl Pts',(6.12158406150175,-5.01153583554654,
49.4221607916786));
#237597=CARTESIAN_POINT('Ctrl Pts',(6.07493478778017,-5.06798286160838,
49.4192413642065));
#237598=CARTESIAN_POINT('Ctrl Pts',(5.99205043746395,-5.16548639627903,
49.4141553483735));
#237599=CARTESIAN_POINT('Ctrl Pts',(5.95616035870386,-5.20682935974878,
49.4119848278126));
#237600=CARTESIAN_POINT('Ctrl Pts',(5.80392923001785,-5.37855562637706,
49.4029076878342));
#237601=CARTESIAN_POINT('Ctrl Pts',(5.68371296333561,-5.50543943382206,
49.3960511430872));
#237602=CARTESIAN_POINT('Ctrl Pts',(5.18398362418241,-5.99905588172231,
49.3686478983667));
#237603=CARTESIAN_POINT('Ctrl Pts',(4.7724237198176,-6.33137517358873,49.3485624053136));
#237604=CARTESIAN_POINT('Ctrl Pts',(4.22427297875216,-6.68996727406419,
49.3228349423994));
#237605=CARTESIAN_POINT('Ctrl Pts',(4.11601715674862,-6.75711077940484,
49.3177944058474));
#237606=CARTESIAN_POINT('Ctrl Pts',(3.98775570306799,-6.83243605543242,
49.3118365409727));
#237607=CARTESIAN_POINT('Ctrl Pts',(3.9692782329836,-6.84318699891152,49.310978576969));
#237608=CARTESIAN_POINT('Ctrl Pts',(3.9394676918288,-6.86037062519305,49.3095946975938));
#237609=CARTESIAN_POINT('Ctrl Pts',(3.92816187044759,-6.86685045184993,
49.3090699253161));
#237610=CARTESIAN_POINT('Ctrl Pts',(3.90796902303783,-6.87835760682458,
49.3081327244748));
#237611=CARTESIAN_POINT('Ctrl Pts',(3.89908816800399,-6.88339572520712,
49.3077205666184));
#237612=CARTESIAN_POINT('Ctrl Pts',(3.88061377750974,-6.89382904151755,
49.3068631960752));
#237613=CARTESIAN_POINT('Ctrl Pts',(3.87101868872506,-6.89922143828456,
49.3064179128951));
#237614=CARTESIAN_POINT('Ctrl Pts',(3.84605615133679,-6.91318180356323,
49.3052594465964));
#237615=CARTESIAN_POINT('Ctrl Pts',(3.83067142416883,-6.92171850085521,
49.3045454342996));
#237616=CARTESIAN_POINT('Ctrl Pts',(3.753683968429,-6.96410210704746,49.3009721450845));
#237617=CARTESIAN_POINT('Ctrl Pts',(3.69166125299304,-6.99717789300047,
49.2980929016583));
#237618=CARTESIAN_POINT('Ctrl Pts',(3.01317596259054,-7.34747173732453,
49.2666301737935));
#237619=CARTESIAN_POINT('Ctrl Pts',(2.35799642377459,-7.58317166646662,
49.236847120652));
#237620=CARTESIAN_POINT('Ctrl Pts',(1.66979020112909,-7.73277708092119,
49.2078242827824));
#237621=CARTESIAN_POINT('Ctrl Pts',(1.65909436721716,-7.73507896405873,
49.207373679671));
#237622=CARTESIAN_POINT('Ctrl Pts',(1.50187881343523,-7.76857271210901,
49.2007570896734));
#237623=CARTESIAN_POINT('Ctrl Pts',(1.35450498613362,-7.79561924610495,
49.1946411071309));
#237624=CARTESIAN_POINT('Ctrl Pts',(1.1678978778891,-7.82441417684245,49.1869961801491));
#237625=CARTESIAN_POINT('Ctrl Pts',(1.12930204155378,-7.83007787857513,
49.1854202533786));
#237626=CARTESIAN_POINT('Ctrl Pts',(1.06793728565388,-7.83861961996101,
49.1829226458428));
#237627=CARTESIAN_POINT('Ctrl Pts',(1.04519511005172,-7.8416844350422,49.1819987587911));
#237628=CARTESIAN_POINT('Ctrl Pts',(1.00268098972975,-7.84722555292625,
49.1802748066811));
#237629=CARTESIAN_POINT('Ctrl Pts',(0.982912411321682,-7.84972618886304,
49.1794744624347));
#237630=CARTESIAN_POINT('Ctrl Pts',(0.938799693025847,-7.85513699636905,
49.1776912880547));
#237631=CARTESIAN_POINT('Ctrl Pts',(0.914451029592729,-7.85800874362651,
49.1767089105883));
#237632=CARTESIAN_POINT('Ctrl Pts',(0.842875059848871,-7.86611342436338,
49.1738263708649));
#237633=CARTESIAN_POINT('Ctrl Pts',(0.795613374499294,-7.87103412298189,
49.1719297820021));
#237634=CARTESIAN_POINT('Ctrl Pts',(0.373760442075087,-7.9111173727665,
49.1550559330217));
#237635=CARTESIAN_POINT('Ctrl Pts',(-0.00286190810906917,-7.91994173535442,
49.1403425663408));
#237636=CARTESIAN_POINT('Ctrl Pts',(-0.948677347144523,-7.87461582484368,
49.1036414949084));
#237637=CARTESIAN_POINT('Ctrl Pts',(-1.51404753537399,-7.78570761869245,
49.0822651771676));
#237638=CARTESIAN_POINT('Ctrl Pts',(-2.43405743196127,-7.53694238822372,
49.046622632109));
#237639=CARTESIAN_POINT('Ctrl Pts',(-2.79544504176706,-7.41050590419739,
49.0323349507945));
#237640=CARTESIAN_POINT('Ctrl Pts',(-3.17626541325873,-7.24543504168874,
49.016064749451));
#237641=CARTESIAN_POINT('Ctrl Pts',(-3.20619573906016,-7.23224030114821,
49.014777365499));
#237642=CARTESIAN_POINT('Ctrl Pts',(-3.25151126837907,-7.21192642875092,
49.0128141209004));
#237643=CARTESIAN_POINT('Ctrl Pts',(-3.26695698304196,-7.20494277623656,
49.0121424509039));
#237644=CARTESIAN_POINT('Ctrl Pts',(-3.31236438508732,-7.18423615989473,
49.0101602344403));
#237645=CARTESIAN_POINT('Ctrl Pts',(-3.34226273619789,-7.17037563796252,
49.008845232795));
#237646=CARTESIAN_POINT('Ctrl Pts',(-3.38226084418731,-7.15152846668484,
49.0070719199289));
#237647=CARTESIAN_POINT('Ctrl Pts',(-3.39243802388179,-7.14670637990842,
49.006619484534));
#237648=CARTESIAN_POINT('Ctrl Pts',(-3.40910890443529,-7.1387638553658,
49.0058763015897));
#237649=CARTESIAN_POINT('Ctrl Pts',(-3.41560871748465,-7.13565624127435,
49.0055860260539));
#237650=CARTESIAN_POINT('Ctrl Pts',(-3.42795057044004,-7.12973477303732,
49.0050338564574));
#237651=CARTESIAN_POINT('Ctrl Pts',(-3.43379341576472,-7.12692260550121,
49.0047720257847));
#237652=CARTESIAN_POINT('Ctrl Pts',(-3.44739632784333,-7.12035489856849,
49.0041614490109));
#237653=CARTESIAN_POINT('Ctrl Pts',(-3.4551537185134,-7.11659385545897,
49.0038124931375));
#237654=CARTESIAN_POINT('Ctrl Pts',(-3.47874413845167,-7.10510876519192,
49.0027489586867));
#237655=CARTESIAN_POINT('Ctrl Pts',(-3.49455747017834,-7.09734453352809,
49.0020328132275));
#237656=CARTESIAN_POINT('Ctrl Pts',(-3.66522005895423,-7.01284179344709,
48.9942678563086));
#237657=CARTESIAN_POINT('Ctrl Pts',(-3.81751575097769,-6.93111497405427,
48.9869936551422));
#237658=CARTESIAN_POINT('Ctrl Pts',(-4.05434841994003,-6.79384779929839,
48.9751134531399));
#237659=CARTESIAN_POINT('Ctrl Pts',(-4.1406975149891,-6.74156748034654,
48.9706652642546));
#237660=CARTESIAN_POINT('Ctrl Pts',(-5.03963920542211,-6.17351361007708,
48.9232858178684));
#237661=CARTESIAN_POINT('Ctrl Pts',(-5.75291523545961,-5.51498231897554,
48.8775307954523));
#237662=CARTESIAN_POINT('Ctrl Pts',(-6.35899265573277,-4.70631580225002,
48.8361887343776));
#237663=CARTESIAN_POINT('Ctrl Pts',(-6.38725277906597,-4.66789010852951,
48.8342507130064));
#237664=CARTESIAN_POINT('Ctrl Pts',(-6.4232930267536,-4.61794550415109,
48.8317654075641));
#237665=CARTESIAN_POINT('Ctrl Pts',(-6.43139240891813,-4.60665884040604,
48.8312059664108));
#237666=CARTESIAN_POINT('Ctrl Pts',(-6.44421033575313,-4.58869708823273,
48.8303191376588));
#237667=CARTESIAN_POINT('Ctrl Pts',(-6.44894831899294,-4.58203594469263,
48.8299910115572));
#237668=CARTESIAN_POINT('Ctrl Pts',(-6.45779788168344,-4.56955340406677,
48.8293775354614));
#237669=CARTESIAN_POINT('Ctrl Pts',(-6.46191193305268,-4.56373377434584,
48.8290920918066));
#237670=CARTESIAN_POINT('Ctrl Pts',(-6.47115179674687,-4.55062576109939,
48.8284504484443));
#237671=CARTESIAN_POINT('Ctrl Pts',(-6.4762731748559,-4.5433342557451,48.8280944169137));
#237672=CARTESIAN_POINT('Ctrl Pts',(-6.49129377000335,-4.52187184686007,
48.8270490554321));
#237673=CARTESIAN_POINT('Ctrl Pts',(-6.50115890076761,-4.50767709133017,
48.8263610149082));
#237674=CARTESIAN_POINT('Ctrl Pts',(-6.57535144307397,-4.4001726203807,
48.8211751603362));
#237675=CARTESIAN_POINT('Ctrl Pts',(-6.63771500643069,-4.30552046751548,
48.8167516971204));
#237676=CARTESIAN_POINT('Ctrl Pts',(-6.86810291237869,-3.93893951383469,
48.8001313672972));
#237677=CARTESIAN_POINT('Ctrl Pts',(-7.02163131959227,-3.65825063119893,
48.7884701328979));
#237678=CARTESIAN_POINT('Ctrl Pts',(-7.45537879774512,-2.73671954071198,
48.7525506912303));
#237679=CARTESIAN_POINT('Ctrl Pts',(-7.66786858919159,-2.06783614009374,
48.7301321547401));
#237680=CARTESIAN_POINT('Ctrl Pts',(-7.79411041957937,-1.35513529185525,
48.7037779797173));
#237681=CARTESIAN_POINT('Ctrl Pts',(-7.79836362753557,-1.33044113327896,
48.7028615403327));
#237682=CARTESIAN_POINT('Ctrl Pts',(-7.81102040931224,-1.25480931528971,
48.700043608784));
#237683=CARTESIAN_POINT('Ctrl Pts',(-7.81904265379069,-1.20380981845328,
48.6981280387552));
#237684=CARTESIAN_POINT('Ctrl Pts',(-7.84210828712324,-1.0472044481388,
48.6921896832425));
#237685=CARTESIAN_POINT('Ctrl Pts',(-7.85551493416445,-0.941372934361506,
48.6880985486666));
#237686=CARTESIAN_POINT('Ctrl Pts',(-7.87078871851612,-0.797527018899254,
48.6823967410285));
#237687=CARTESIAN_POINT('Ctrl Pts',(-7.8745279592402,-0.759719505442483,
48.6808849382556));
#237688=CARTESIAN_POINT('Ctrl Pts',(-7.87870809856111,-0.714101410066124,
48.6790435066982));
#237689=CARTESIAN_POINT('Ctrl Pts',(-7.87940998446185,-0.706314676449113,
48.6787285779233));
#237690=CARTESIAN_POINT('Ctrl Pts',(-7.88053850701718,-0.69358378458703,
48.6782126763788));
#237691=CARTESIAN_POINT('Ctrl Pts',(-7.88097203785256,-0.688640229116838,
48.6780120968644));
#237692=CARTESIAN_POINT('Ctrl Pts',(-7.88173884250575,-0.679800785236281,
48.6776529961838));
#237693=CARTESIAN_POINT('Ctrl Pts',(-7.88207388037984,-0.675905047473435,
48.6774945764827));
#237694=CARTESIAN_POINT('Ctrl Pts',(-7.88271582337061,-0.668375304900736,
48.6771880762194));
#237695=CARTESIAN_POINT('Ctrl Pts',(-7.88302310419652,-0.664741332275987,
48.6770400174397));
#237696=CARTESIAN_POINT('Ctrl Pts',(-7.88368395296132,-0.656861085553477,
48.676718653775));
#237697=CARTESIAN_POINT('Ctrl Pts',(-7.88403660313302,-0.652614737967597,
48.6765452955303));
#237698=CARTESIAN_POINT('Ctrl Pts',(-7.88488459467025,-0.64230286066898,
48.6761238491736));
#237699=CARTESIAN_POINT('Ctrl Pts',(-7.88537636808917,-0.636237038868326,
48.6758755514612));
#237700=CARTESIAN_POINT('Ctrl Pts',(-7.88669645817127,-0.619717629343189,
48.6751982801246));
#237701=CARTESIAN_POINT('Ctrl Pts',(-7.8875109858695,-0.609263004909966,
48.6747684948195));
#237702=CARTESIAN_POINT('Ctrl Pts',(-7.90323768057082,-0.402089420018049,
48.6662291460158));
#237703=CARTESIAN_POINT('Ctrl Pts',(-7.91080563654813,-0.204897649807095,
48.6577000542341));
#237704=CARTESIAN_POINT('Ctrl Pts',(-7.91099630412092,-0.00764697228234312,
48.6489209116116));
#237705=CARTESIAN_POINT('',(-7.91143166941437,0.00169103298945927,44.6423315082371));
#237706=CARTESIAN_POINT('Ctrl Pts',(-7.91099626150122,-0.00769093712042951,
48.6489228683743));
#237707=CARTESIAN_POINT('Ctrl Pts',(-7.91164791772632,0.662610988365909,
48.6190895035468));
#237708=CARTESIAN_POINT('Ctrl Pts',(-7.82711173938375,1.33033400700045,
48.5868061908958));
#237709=CARTESIAN_POINT('Ctrl Pts',(-7.56272340494108,2.35334709170472,
48.5394353254642));
#237710=CARTESIAN_POINT('Ctrl Pts',(-7.43885343323155,2.71965928564517,
48.5228574067941));
#237711=CARTESIAN_POINT('Ctrl Pts',(-7.28054940035535,3.09482819938831,
48.5064056155218));
#237712=CARTESIAN_POINT('Ctrl Pts',(-7.27231631601591,3.11412532889468,
48.5055607992272));
#237713=CARTESIAN_POINT('Ctrl Pts',(-7.26037555434932,3.14180709915026,
48.5043508811569));
#237714=CARTESIAN_POINT('Ctrl Pts',(-7.25672995232899,3.15021831596243,
48.5039835051861));
#237715=CARTESIAN_POINT('Ctrl Pts',(-7.25038044184114,3.1647985426772,48.5033471375152));
#237716=CARTESIAN_POINT('Ctrl Pts',(-7.24768326417479,3.17097046180989,
48.5030778989516));
#237717=CARTESIAN_POINT('Ctrl Pts',(-7.24248427103993,3.18282596849578,
48.5025609929336));
#237718=CARTESIAN_POINT('Ctrl Pts',(-7.23998364027211,3.18851006754165,
48.5023132822061));
#237719=CARTESIAN_POINT('Ctrl Pts',(-7.2340808919189,3.20188465860019,48.5017307009548));
#237720=CARTESIAN_POINT('Ctrl Pts',(-7.23067319599463,3.20957268980701,
48.5013960361421));
#237721=CARTESIAN_POINT('Ctrl Pts',(-7.21887117103174,3.23608479888389,
48.5002426883938));
#237722=CARTESIAN_POINT('Ctrl Pts',(-7.21041550464177,3.25488157523169,
48.4994262692693));
#237723=CARTESIAN_POINT('Ctrl Pts',(-7.11550591576871,3.46367881514814,
48.4903713846731));
#237724=CARTESIAN_POINT('Ctrl Pts',(-7.02163462186226,3.65022614488148,
48.4824142806544));
#237725=CARTESIAN_POINT('Ctrl Pts',(-6.90912552480948,3.85336937889999,
48.4738349677696));
#237726=CARTESIAN_POINT('Ctrl Pts',(-6.89767092776954,3.87383619562231,
48.4729715458886));
#237727=CARTESIAN_POINT('Ctrl Pts',(-6.5165657367382,4.54773666085987,48.444569700496));
#237728=CARTESIAN_POINT('Ctrl Pts',(-6.05593026730365,5.14520197799945,
48.420740272478));
#237729=CARTESIAN_POINT('Ctrl Pts',(-5.42747543611767,5.75694397000242,
48.389967159942));
#237730=CARTESIAN_POINT('Ctrl Pts',(-5.33481663504837,5.84291221156716,
48.385453449272));
#237731=CARTESIAN_POINT('Ctrl Pts',(-5.10686044411135,6.04446425561905,
48.3742918660903));
#237732=CARTESIAN_POINT('Ctrl Pts',(-4.96965073242299,6.15777030377607,
48.3675276026204));
#237733=CARTESIAN_POINT('Ctrl Pts',(-4.81974343042241,6.27328649923102,
48.359945201152));
#237734=CARTESIAN_POINT('Ctrl Pts',(-4.81072369648317,6.28020602766404,
48.3594882579054));
#237735=CARTESIAN_POINT('Ctrl Pts',(-4.79855073843631,6.28950295375264,
48.3588705546121));
#237736=CARTESIAN_POINT('Ctrl Pts',(-4.79541056537802,6.29189749630896,
48.3587111189372));
#237737=CARTESIAN_POINT('Ctrl Pts',(-4.78951436177792,6.29638667502592,
48.3584115791611));
#237738=CARTESIAN_POINT('Ctrl Pts',(-4.78675875949195,6.29848184576806,
48.3582715183897));
#237739=CARTESIAN_POINT('Ctrl Pts',(-4.78101743996767,6.30284120693398,
48.357979556023));
#237740=CARTESIAN_POINT('Ctrl Pts',(-4.77803148816639,6.30510508549159,
48.3578276305779));
#237741=CARTESIAN_POINT('Ctrl Pts',(-4.77117625249734,6.31029489803012,
48.3574786514511));
#237742=CARTESIAN_POINT('Ctrl Pts',(-4.76730588703944,6.31321939359672,
48.3572814884621));
#237743=CARTESIAN_POINT('Ctrl Pts',(-4.75508028050654,6.32243955855908,
48.3566582778941));
#237744=CARTESIAN_POINT('Ctrl Pts',(-4.74671527130343,6.32872219146621,
48.3562312499412));
#237745=CARTESIAN_POINT('Ctrl Pts',(-4.67806032983215,6.3800735593634,48.3527216113364));
#237746=CARTESIAN_POINT('Ctrl Pts',(-4.61714431659378,6.424294879196,48.3495769969414));
#237747=CARTESIAN_POINT('Ctrl Pts',(-4.43471670617654,6.55279135583343,
48.3400937281315));
#237748=CARTESIAN_POINT('Ctrl Pts',(-4.31146699714319,6.6345334940547,48.3336019948001));
#237749=CARTESIAN_POINT('Ctrl Pts',(-4.00771767056835,6.82394808415077,
48.3175432042965));
#237750=CARTESIAN_POINT('Ctrl Pts',(-3.82507750996235,6.92797541912186,
48.3078395628417));
#237751=CARTESIAN_POINT('Ctrl Pts',(-3.49322621780812,7.09986381864569,
48.2903913324137));
#237752=CARTESIAN_POINT('Ctrl Pts',(-3.34563158485885,7.17059581106805,
48.2826917718914));
#237753=CARTESIAN_POINT('Ctrl Pts',(-2.87995336003558,7.37625375905966,
48.2587665527189));
#237754=CARTESIAN_POINT('Ctrl Pts',(-2.55513872036533,7.49496771270357,
48.2426164241586));
#237755=CARTESIAN_POINT('Ctrl Pts',(-1.92387198622441,7.67985509310382,
48.2129055711801));
#237756=CARTESIAN_POINT('Ctrl Pts',(-1.61920035885695,7.74981792725625,
48.1992684735961));
#237757=CARTESIAN_POINT('Ctrl Pts',(-1.20324504779625,7.81972491483518,
48.1816645555034));
#237758=CARTESIAN_POINT('Ctrl Pts',(-1.09495900617121,7.83562138489461,
48.1771710997982));
#237759=CARTESIAN_POINT('Ctrl Pts',(-0.969915592877777,7.85133491372611,
48.172081143961));
#237760=CARTESIAN_POINT('Ctrl Pts',(-0.953449816019706,7.85335149077491,
48.1714128576817));
#237761=CARTESIAN_POINT('Ctrl Pts',(-0.928498969036424,7.85632761390697,
48.1704031369641));
#237762=CARTESIAN_POINT('Ctrl Pts',(-0.920018538811382,7.85732523199819,
48.1700604622762));
#237763=CARTESIAN_POINT('Ctrl Pts',(-0.904758108076628,7.85909538882041,
48.1694447446672));
#237764=CARTESIAN_POINT('Ctrl Pts',(-0.89797869842171,7.85987288842498,
48.1691715405684));
#237765=CARTESIAN_POINT('Ctrl Pts',(-0.884419813309074,7.86141012363792,
48.1686257807841));
#237766=CARTESIAN_POINT('Ctrl Pts',(-0.877640344171195,7.86216986364495,
48.1683532251655));
#237767=CARTESIAN_POINT('Ctrl Pts',(-0.858733845965238,7.86426385788495,
48.1675940286768));
#237768=CARTESIAN_POINT('Ctrl Pts',(-0.846604676376769,7.86557883237744,
48.1671080138349));
#237769=CARTESIAN_POINT('Ctrl Pts',(-0.797959647548427,7.87073882099469,
48.1651629305347));
#237770=CARTESIAN_POINT('Ctrl Pts',(-0.761419986069347,7.87435767790698,
48.1637111886542));
#237771=CARTESIAN_POINT('Ctrl Pts',(-0.148815339735849,7.93072552491043,
48.1395236409995));
#237772=CARTESIAN_POINT('Ctrl Pts',(0.431333047120447,7.92039036244018,
48.1190414103495));
#237773=CARTESIAN_POINT('Ctrl Pts',(1.40121433934112,7.79614851755108,48.0852321336883));
#237774=CARTESIAN_POINT('Ctrl Pts',(1.79281738828514,7.71551123934827,48.0716489341533));
#237775=CARTESIAN_POINT('Ctrl Pts',(2.27466912532441,7.577611618939,48.0534932253593));
#237776=CARTESIAN_POINT('Ctrl Pts',(2.3721429801864,7.54766547611505,48.049742488657));
#237777=CARTESIAN_POINT('Ctrl Pts',(2.59564961580598,7.47424195990608,48.0409080683694));
#237778=CARTESIAN_POINT('Ctrl Pts',(2.7212016876782,7.42945150301658,48.0357623131637));
#237779=CARTESIAN_POINT('Ctrl Pts',(2.87083519215558,7.37176771595247,48.0293827703455));
#237780=CARTESIAN_POINT('Ctrl Pts',(2.89604598425466,7.36189999869819,48.0282998957074));
#237781=CARTESIAN_POINT('Ctrl Pts',(2.92997690475974,7.34841788575881,48.0268320155387));
#237782=CARTESIAN_POINT('Ctrl Pts',(2.93874212864078,7.3449169353033,48.0264518806728));
#237783=CARTESIAN_POINT('Ctrl Pts',(2.95256096566265,7.33936880623374,48.0258511071557));
#237784=CARTESIAN_POINT('Ctrl Pts',(2.95761878039787,7.33733206823279,48.0256309074573));
#237785=CARTESIAN_POINT('Ctrl Pts',(2.96801042737812,7.33313495171264,48.0251778558198));
#237786=CARTESIAN_POINT('Ctrl Pts',(2.97334401535499,7.3309739791643,48.0249449792933));
#237787=CARTESIAN_POINT('Ctrl Pts',(2.98546293331624,7.32604844083083,48.0244150627199));
#237788=CARTESIAN_POINT('Ctrl Pts',(2.99224678479662,7.32328026652157,48.0241178749044));
#237789=CARTESIAN_POINT('Ctrl Pts',(3.01237042260991,7.31503611566253,48.0232346662927));
#237790=CARTESIAN_POINT('Ctrl Pts',(3.02569905330234,7.30953310218356,48.0226475564617));
#237791=CARTESIAN_POINT('Ctrl Pts',(3.11585489173414,7.27202147060471,48.0186621665154));
#237792=CARTESIAN_POINT('Ctrl Pts',(3.19218638090611,7.23883923735941,48.0152183089434));
#237793=CARTESIAN_POINT('Ctrl Pts',(3.50128965375392,7.09862846713809,48.0010193650734));
#237794=CARTESIAN_POINT('Ctrl Pts',(3.72931472324528,6.98152976718042,47.9899568984898));
#237795=CARTESIAN_POINT('Ctrl Pts',(4.33540487570436,6.63210478696252,47.9594509675495));
#237796=CARTESIAN_POINT('Ctrl Pts',(4.7002752821341,6.37871321579496,47.9398839873903));
#237797=CARTESIAN_POINT('Ctrl Pts',(5.31550270848996,5.86986667640528,47.905593310329));
#237798=CARTESIAN_POINT('Ctrl Pts',(5.57349016989947,5.62548975807045,47.8907088750727));
#237799=CARTESIAN_POINT('Ctrl Pts',(5.85965286627001,5.31534392419588,47.8735155990729));
#237800=CARTESIAN_POINT('Ctrl Pts',(5.90447332132728,5.26551115058837,47.8707998545952));
#237801=CARTESIAN_POINT('Ctrl Pts',(5.96305759529284,5.19868660470533,47.8672178124476));
#237802=CARTESIAN_POINT('Ctrl Pts',(5.97739168188314,5.18219904920756,47.8663387721762));
#237803=CARTESIAN_POINT('Ctrl Pts',(6.00068108105965,5.15518559733434,47.864906287427));
#237804=CARTESIAN_POINT('Ctrl Pts',(6.00967740954633,5.14469526931984,47.8643518922996));
#237805=CARTESIAN_POINT('Ctrl Pts',(6.02697782338581,5.12441451524966,47.8632837344666));
#237806=CARTESIAN_POINT('Ctrl Pts',(6.03528565405263,5.11462734545,47.8627698849495));
#237807=CARTESIAN_POINT('Ctrl Pts',(6.05431508747019,5.09209849888594,47.8615907968072));
#237808=CARTESIAN_POINT('Ctrl Pts',(6.06502036613315,5.07934309351674,47.8609259456079));
#237809=CARTESIAN_POINT('Ctrl Pts',(6.09887349949267,5.03874725911853,47.8588185934831));
#237810=CARTESIAN_POINT('Ctrl Pts',(6.12187062922111,5.01078156875489,47.8573796978197));
#237811=CARTESIAN_POINT('Ctrl Pts',(6.34222752784816,4.73903477931616,47.8435205584969));
#237812=CARTESIAN_POINT('Ctrl Pts',(6.52512196159636,4.48387107694677,47.8314735615384));
#237813=CARTESIAN_POINT('Ctrl Pts',(6.98320898283572,3.75714588720639,47.7992953107247));
#237814=CARTESIAN_POINT('Ctrl Pts',(7.22552720475665,3.26696852218822,47.7799469547945));
#237815=CARTESIAN_POINT('Ctrl Pts',(7.5019114838266,2.52324829553692,47.7505871945972));
#237816=CARTESIAN_POINT('Ctrl Pts',(7.57733559644206,2.28679475633846,47.7412274259359));
#237817=CARTESIAN_POINT('Ctrl Pts',(7.65052373696703,2.01360801038185,47.7300284135753));
#237818=CARTESIAN_POINT('Ctrl Pts',(7.65930241548482,1.97995381891484,47.7286421611545));
#237819=CARTESIAN_POINT('Ctrl Pts',(7.67020179464787,1.93701216598482,47.7268637241967));
#237820=CARTESIAN_POINT('Ctrl Pts',(7.67252812342186,1.92777693106521,47.7264806794888));
#237821=CARTESIAN_POINT('Ctrl Pts',(7.67601634825423,1.91382278161091,47.7259010278631));
#237822=CARTESIAN_POINT('Ctrl Pts',(7.67719058741939,1.9091069384319,47.7257049808064));
#237823=CARTESIAN_POINT('Ctrl Pts',(7.67949766712264,1.89980496279101,47.7253179738754));
#237824=CARTESIAN_POINT('Ctrl Pts',(7.68063074680038,1.89521889161692,47.725127025079));
#237825=CARTESIAN_POINT('Ctrl Pts',(7.68313469287715,1.88504519627132,47.7247030967469));
#237826=CARTESIAN_POINT('Ctrl Pts',(7.6845035720382,1.87945708967914,47.724470025349));
#237827=CARTESIAN_POINT('Ctrl Pts',(7.6881695875273,1.86442053826833,47.7238422698674));
#237828=CARTESIAN_POINT('Ctrl Pts',(7.69045539647751,1.85496936459352,47.72344705524));
#237829=CARTESIAN_POINT('Ctrl Pts',(7.70075933444319,1.81201908242679,47.721648021481));
#237830=CARTESIAN_POINT('Ctrl Pts',(7.70857600681764,1.77847221666756,47.7202345300573));
#237831=CARTESIAN_POINT('Ctrl Pts',(7.8358553386864,1.21561856284086,47.6963657250822));
#237832=CARTESIAN_POINT('Ctrl Pts',(7.90075749779283,0.675494280796114,
47.6713061155912));
#237833=CARTESIAN_POINT('Ctrl Pts',(7.9181632415298,-0.359367472907174,
47.6235748808032));
#237834=CARTESIAN_POINT('Ctrl Pts',(7.88044781417404,-0.851513552323777,
47.6010161602236));
#237835=CARTESIAN_POINT('Ctrl Pts',(7.75897777392869,-1.55991840891451,
47.569917771904));
#237836=CARTESIAN_POINT('Ctrl Pts',(7.71120648062879,-1.78111952380973,
47.5603939626964));
#237837=CARTESIAN_POINT('Ctrl Pts',(7.64385662378762,-2.03887039919428,
47.5495188688549));
#237838=CARTESIAN_POINT('Ctrl Pts',(7.6333987453365,-2.07768145879723,47.5478872392832));
#237839=CARTESIAN_POINT('Ctrl Pts',(7.61922542006292,-2.12872929772349,
47.5457487453617));
#237840=CARTESIAN_POINT('Ctrl Pts',(7.61577554602076,-2.14103882712643,
47.5452336571527));
#237841=CARTESIAN_POINT('Ctrl Pts',(7.61008422704115,-2.16115827146161,
47.5443927080092));
#237842=CARTESIAN_POINT('Ctrl Pts',(7.60786056714314,-2.16897316912061,
47.5440662951332));
#237843=CARTESIAN_POINT('Ctrl Pts',(7.6035441152359,-2.18405473177788,47.5434368145077));
#237844=CARTESIAN_POINT('Ctrl Pts',(7.60145293653761,-2.19132184713629,
47.5431336969993));
#237845=CARTESIAN_POINT('Ctrl Pts',(7.59662367866529,-2.20801404286949,
47.5424379088335));
#237846=CARTESIAN_POINT('Ctrl Pts',(7.59387847075438,-2.21743705683769,
47.5420454606288));
#237847=CARTESIAN_POINT('Ctrl Pts',(7.58652246918227,-2.24251289709838,
47.5410019907324));
#237848=CARTESIAN_POINT('Ctrl Pts',(7.58188075924071,-2.25815664328931,
47.5403519334927));
#237849=CARTESIAN_POINT('Ctrl Pts',(7.55025697470046,-2.36354010844566,
47.5359789412157));
#237850=CARTESIAN_POINT('Ctrl Pts',(7.52173016133097,-2.45281029152105,
47.5323045272707));
#237851=CARTESIAN_POINT('Ctrl Pts',(7.18153029378573,-3.45560181924886,
47.4913244080797));
#237852=CARTESIAN_POINT('Ctrl Pts',(6.70684949520771,-4.30505050391386,
47.4604883065493));
#237853=CARTESIAN_POINT('Ctrl Pts',(6.02579664882594,-5.12680646109746,
47.421968628824));
#237854=CARTESIAN_POINT('Ctrl Pts',(5.95905156131876,-5.20423609343146,
47.4182276797094));
#237855=CARTESIAN_POINT('Ctrl Pts',(5.78953438319508,-5.39335167910168,
47.4087581054396));
#237856=CARTESIAN_POINT('Ctrl Pts',(5.685015814706,-5.50341220090058,47.4029404670049));
#237857=CARTESIAN_POINT('Ctrl Pts',(5.55631926246223,-5.63135154330612,
47.3957453489449));
#237858=CARTESIAN_POINT('Ctrl Pts',(5.53512836457719,-5.65218169444424,
47.3945603282218));
#237859=CARTESIAN_POINT('Ctrl Pts',(5.50664702358555,-5.6798644031683,47.3929678200024));
#237860=CARTESIAN_POINT('Ctrl Pts',(5.49946003904369,-5.68682339786983,
47.3925659833255));
#237861=CARTESIAN_POINT('Ctrl Pts',(5.48765159273853,-5.69821393008731,
47.3919058075313));
#237862=CARTESIAN_POINT('Ctrl Pts',(5.48303790423802,-5.70265353469084,
47.3916478833134));
#237863=CARTESIAN_POINT('Ctrl Pts',(5.47407735184347,-5.71125506022064,
47.3911469862032));
#237864=CARTESIAN_POINT('Ctrl Pts',(5.46973111745684,-5.71541763297707,
47.3909040464157));
#237865=CARTESIAN_POINT('Ctrl Pts',(5.45966980136849,-5.72503179397972,
47.3903416975435));
#237866=CARTESIAN_POINT('Ctrl Pts',(5.45395130169864,-5.73047978621501,
47.3900221113531));
#237867=CARTESIAN_POINT('Ctrl Pts',(5.43635448925281,-5.74719400138421,
47.3890388155757));
#237868=CARTESIAN_POINT('Ctrl Pts',(5.42444939345269,-5.75843188686159,
47.3883737446472));
#237869=CARTESIAN_POINT('Ctrl Pts',(5.32549952995165,-5.85125704755426,
47.3828480034995));
#237870=CARTESIAN_POINT('Ctrl Pts',(5.23665625844741,-5.93090078000216,
47.3778999382196));
#237871=CARTESIAN_POINT('Ctrl Pts',(5.13331565004882,-6.01940798472861,
47.3721876621747));
#237872=CARTESIAN_POINT('Ctrl Pts',(5.12054818087192,-6.03027266164513,
47.3714826526186));
#237873=CARTESIAN_POINT('Ctrl Pts',(5.1028638937583,-6.04522472376653,47.3705072298042));
#237874=CARTESIAN_POINT('Ctrl Pts',(5.09797647939127,-6.04934688164466,
47.3702377661627));
#237875=CARTESIAN_POINT('Ctrl Pts',(5.0778295247574,-6.06629753155847,47.369127464889));
#237876=CARTESIAN_POINT('Ctrl Pts',(5.06252655876757,-6.07907421084948,
47.3682852600263));
#237877=CARTESIAN_POINT('Ctrl Pts',(4.72676657057053,-6.35725825692849,
47.3498337452759));
#237878=CARTESIAN_POINT('Ctrl Pts',(4.38591508810346,-6.59702993310786,
47.331695768767));
#237879=CARTESIAN_POINT('Ctrl Pts',(3.65051488629766,-7.03205559198144,
47.2949343267975));
#237880=CARTESIAN_POINT('Ctrl Pts',(3.25533261519665,-7.22349662895991,
47.2764103480214));
#237881=CARTESIAN_POINT('Ctrl Pts',(2.54179739579593,-7.49864697020106,
47.2448001249646));
#237882=CARTESIAN_POINT('Ctrl Pts',(2.23029748456682,-7.59711921350632,
47.2314969827077));
#237883=CARTESIAN_POINT('Ctrl Pts',(1.85766486694136,-7.69001470722281,
47.2159496806692));
#237884=CARTESIAN_POINT('Ctrl Pts',(1.80157227704531,-7.7033487738541,47.2136203603499));
#237885=CARTESIAN_POINT('Ctrl Pts',(1.71646537542548,-7.72259955853075,
47.2101027701486));
#237886=CARTESIAN_POINT('Ctrl Pts',(1.68755550901289,-7.72896847820476,
47.2089107638258));
#237887=CARTESIAN_POINT('Ctrl Pts',(1.6373263615106,-7.73973883474461,47.2068446805466));
#237888=CARTESIAN_POINT('Ctrl Pts',(1.6160234249689,-7.74421481732105,47.2059699656311));
#237889=CARTESIAN_POINT('Ctrl Pts',(1.56821554746232,-7.75405392403873,
47.2040103654752));
#237890=CARTESIAN_POINT('Ctrl Pts',(1.54170101629998,-7.75936919097492,
47.2029259171615));
#237891=CARTESIAN_POINT('Ctrl Pts',(1.47065338736643,-7.7732332946957,47.2000262828967));
#237892=CARTESIAN_POINT('Ctrl Pts',(1.42607308470058,-7.78153537691466,
47.1982133825744));
#237893=CARTESIAN_POINT('Ctrl Pts',(1.22285735870231,-7.81757474965926,
47.1899782562534));
#237894=CARTESIAN_POINT('Ctrl Pts',(1.06346774005549,-7.84084769504832,
47.1835996718062));
#237895=CARTESIAN_POINT('Ctrl Pts',(0.585235132806012,-7.89582404324409,
47.164656810414));
#237896=CARTESIAN_POINT('Ctrl Pts',(0.265062059889638,-7.9130452019605,
47.1522415973748));
#237897=CARTESIAN_POINT('Ctrl Pts',(-0.424845421560862,-7.90822456977076,
47.1255668533777));
#237898=CARTESIAN_POINT('Ctrl Pts',(-0.793772353520196,-7.87974767875001,
47.1113520754224));
#237899=CARTESIAN_POINT('Ctrl Pts',(-1.24387748904195,-7.81306548385664,
47.0933639008474));
#237900=CARTESIAN_POINT('Ctrl Pts',(-1.32819992645492,-7.79917355143417,
47.0899648516399));
#237901=CARTESIAN_POINT('Ctrl Pts',(-1.43207723812229,-7.78032651164104,
47.0857309247119));
#237902=CARTESIAN_POINT('Ctrl Pts',(-1.45186091071279,-7.77665903421985,
47.0849224637683));
#237903=CARTESIAN_POINT('Ctrl Pts',(-1.48303493967257,-7.77075691907995,
47.0836450416208));
#237904=CARTESIAN_POINT('Ctrl Pts',(-1.49443477874304,-7.76857261141134,
47.0831771711006));
#237905=CARTESIAN_POINT('Ctrl Pts',(-1.51573727336818,-7.76444224444807,
47.0823014559511));
#237906=CARTESIAN_POINT('Ctrl Pts',(-1.5256410975579,-7.76250230853364,
47.081893748887));
#237907=CARTESIAN_POINT('Ctrl Pts',(-1.54770133499664,-7.75813735612915,
47.0809842890247));
#237908=CARTESIAN_POINT('Ctrl Pts',(-1.55985580622623,-7.75570270970725,
47.08048231615));
#237909=CARTESIAN_POINT('Ctrl Pts',(-1.59640447816599,-7.74829230069315,
47.0789701154108));
#237910=CARTESIAN_POINT('Ctrl Pts',(-1.62078077998999,-7.74322997723396,
47.0779577957333));
#237911=CARTESIAN_POINT('Ctrl Pts',(-1.8834225631919,-7.68739156593984,
47.0670115723598));
#237912=CARTESIAN_POINT('Ctrl Pts',(-2.11923978341215,-7.62575154262978,
47.0568413676541));
#237913=CARTESIAN_POINT('Ctrl Pts',(-2.70981564242152,-7.44186791529549,
47.0308351057076));
#237914=CARTESIAN_POINT('Ctrl Pts',(-3.05943082227927,-7.30509335568665,
47.0149493884497));
#237915=CARTESIAN_POINT('Ctrl Pts',(-3.56723494997244,-7.0635589243002,
46.9914902837725));
#237916=CARTESIAN_POINT('Ctrl Pts',(-3.73353259683494,-6.97708867872951,
46.9837365138791));
#237917=CARTESIAN_POINT('Ctrl Pts',(-3.96243897957423,-6.84753391324431,
46.9729613729912));
#237918=CARTESIAN_POINT('Ctrl Pts',(-4.02773512985558,-6.80933133599963,
46.9698753981089));
#237919=CARTESIAN_POINT('Ctrl Pts',(-4.14165889584774,-6.7404662846283,
46.9644676067707));
#237920=CARTESIAN_POINT('Ctrl Pts',(-4.19051880494137,-6.71019942766042,
46.962140475121));
#237921=CARTESIAN_POINT('Ctrl Pts',(-4.26139950981679,-6.66521539255381,
46.9587520799467));
#237922=CARTESIAN_POINT('Ctrl Pts',(-4.28368289485535,-6.65091594251652,
46.9576850178575));
#237923=CARTESIAN_POINT('Ctrl Pts',(-4.32279036419075,-6.62554225168772,
46.9558089649588));
#237924=CARTESIAN_POINT('Ctrl Pts',(-4.33964470428317,-6.61451513756861,
46.9549993274632));
#237925=CARTESIAN_POINT('Ctrl Pts',(-4.37243637290283,-6.59288158923538,
46.9534218702914));
#237926=CARTESIAN_POINT('Ctrl Pts',(-4.38837767427708,-6.58228143390373,
46.9526539703265));
#237927=CARTESIAN_POINT('Ctrl Pts',(-4.43118081515678,-6.55359491023963,
46.9505892352346));
#237928=CARTESIAN_POINT('Ctrl Pts',(-4.4579703826455,-6.53540126871248,
46.9492938854217));
#237929=CARTESIAN_POINT('Ctrl Pts',(-4.5580486311177,-6.46653328192752,
46.944442574614));
#237930=CARTESIAN_POINT('Ctrl Pts',(-4.63059159534863,-6.41478617760905,
46.9409012877639));
#237931=CARTESIAN_POINT('Ctrl Pts',(-5.26983038060739,-5.94230257982683,
46.9094336644822));
#237932=CARTESIAN_POINT('Ctrl Pts',(-5.7787648833409,-5.44867417119312,
46.8822996055486));
#237933=CARTESIAN_POINT('Ctrl Pts',(-6.41681003677691,-4.63836330232164,
46.8435641468412));
#237934=CARTESIAN_POINT('Ctrl Pts',(-6.60219645247315,-4.37045355110006,
46.8314778529121));
#237935=CARTESIAN_POINT('Ctrl Pts',(-6.88397742347322,-3.90421112663448,
46.8109531215989));
#237936=CARTESIAN_POINT('Ctrl Pts',(-6.98954822631143,-3.71190247040105,
46.8026152994368));
#237937=CARTESIAN_POINT('Ctrl Pts',(-7.12823091426804,-3.43232540823938,
46.7904336545306));
#237938=CARTESIAN_POINT('Ctrl Pts',(-7.1680041551118,-3.34846971559125,
46.7867720642286));
#237939=CARTESIAN_POINT('Ctrl Pts',(-7.21271025299846,-3.24976519090757,
46.7824361466163));
#237940=CARTESIAN_POINT('Ctrl Pts',(-7.21908655071576,-3.23557604752589,
46.781812220806));
#237941=CARTESIAN_POINT('Ctrl Pts',(-7.22875861268694,-3.21388193691375,
46.780857230924));
#237942=CARTESIAN_POINT('Ctrl Pts',(-7.23208465038839,-3.20639046187242,
46.7805272593346));
#237943=CARTESIAN_POINT('Ctrl Pts',(-7.23785002500948,-3.19335008355712,
46.7799525280505));
#237944=CARTESIAN_POINT('Ctrl Pts',(-7.24029464143683,-3.1878035142746,
46.7797079626353));
#237945=CARTESIAN_POINT('Ctrl Pts',(-7.24576104728485,-3.17536210780843,
46.7791591258388));
#237946=CARTESIAN_POINT('Ctrl Pts',(-7.24877937256675,-3.16846576081492,
46.7788547257878));
#237947=CARTESIAN_POINT('Ctrl Pts',(-7.25678380875276,-3.15010571740462,
46.7780438351657));
#237948=CARTESIAN_POINT('Ctrl Pts',(-7.26175258739268,-3.13863451761687,
46.7775366891549));
#237949=CARTESIAN_POINT('Ctrl Pts',(-7.2827125407002,-3.08992899004435,
46.7753810871942));
#237950=CARTESIAN_POINT('Ctrl Pts',(-7.29844451873437,-3.05258425654252,
46.7737225686046));
#237951=CARTESIAN_POINT('Ctrl Pts',(-7.64406237031845,-2.21420639352112,
46.7363329003107));
#237952=CARTESIAN_POINT('Ctrl Pts',(-7.84040113190449,-1.36462053495646,
46.6945171896527));
#237953=CARTESIAN_POINT('Ctrl Pts',(-7.90570422276263,-0.333951554203285,
46.6486976052779));
#237954=CARTESIAN_POINT('Ctrl Pts',(-7.9109843985096,-0.167369534641295,
46.6414201239052));
#237955=CARTESIAN_POINT('Ctrl Pts',(-7.91101914685337,0.204580413004452,
46.6254962739105));
#237956=CARTESIAN_POINT('Ctrl Pts',(-7.90304521296736,0.40983116605556,
46.616931548811));
#237957=CARTESIAN_POINT('Ctrl Pts',(-7.88553970957431,0.634495654482527,
46.6078024804637));
#237958=CARTESIAN_POINT('Ctrl Pts',(-7.88390990811863,0.654435493437473,
46.6069943435935));
#237959=CARTESIAN_POINT('Ctrl Pts',(-7.88137736095431,0.684036577842264,
46.6057977473433));
#237960=CARTESIAN_POINT('Ctrl Pts',(-7.88053245831373,0.69370261631616,
46.6054074976996));
#237961=CARTESIAN_POINT('Ctrl Pts',(-7.87905553467166,0.710248273071947,
46.6047403321912));
#237962=CARTESIAN_POINT('Ctrl Pts',(-7.87843228212967,0.717128652384837,
46.6044631445851));
#237963=CARTESIAN_POINT('Ctrl Pts',(-7.87720217828301,0.730513185691244,
46.6039244068364));
#237964=CARTESIAN_POINT('Ctrl Pts',(-7.87659628220425,0.737017421410841,
46.6036628272313));
#237965=CARTESIAN_POINT('Ctrl Pts',(-7.87512780889711,0.752572693193192,
46.6030377703939));
#237966=CARTESIAN_POINT('Ctrl Pts',(-7.87425768228362,0.761623016127559,
46.6026745281692));
#237967=CARTESIAN_POINT('Ctrl Pts',(-7.87160217877376,0.788752289338839,
46.6015869447471));
#237968=CARTESIAN_POINT('Ctrl Pts',(-7.86977012189251,0.806826666005331,
46.6008640573136));
#237969=CARTESIAN_POINT('Ctrl Pts',(-7.85327560144176,0.964152014989901,
46.594586404731));
#237970=CARTESIAN_POINT('Ctrl Pts',(-7.83498040868318,1.10300100843181,
46.5891462657306));
#237971=CARTESIAN_POINT('Ctrl Pts',(-7.77935501718813,1.45312032543868,
46.5756500914551));
#237972=CARTESIAN_POINT('Ctrl Pts',(-7.73709979674496,1.66349544685578,
46.5677487879319));
#237973=CARTESIAN_POINT('Ctrl Pts',(-7.51899058819125,2.55908857585947,
46.5346624953478));
#237974=CARTESIAN_POINT('Ctrl Pts',(-7.2602604731843,3.22066128629926,46.5119160306334));
#237975=CARTESIAN_POINT('Ctrl Pts',(-6.78241530144773,4.08163811306552,
46.4768525218232));
#237976=CARTESIAN_POINT('Ctrl Pts',(-6.63508911507151,4.31700060822855,
46.4665784875517));
#237977=CARTESIAN_POINT('Ctrl Pts',(-6.46600140977416,4.55796368165872,
46.4548228171509));
#237978=CARTESIAN_POINT('Ctrl Pts',(-6.45624040394983,4.57177941205441,
46.4541443030755));
#237979=CARTESIAN_POINT('Ctrl Pts',(-6.442756868781,4.59073471246363,46.4532070337478));
#237980=CARTESIAN_POINT('Ctrl Pts',(-6.43907229553737,4.5959013526013,46.4529509119981));
#237981=CARTESIAN_POINT('Ctrl Pts',(-6.43320054552772,4.60411400847454,
46.4525427478832));
#237982=CARTESIAN_POINT('Ctrl Pts',(-6.43101740611882,4.60716292137744,
46.4523909892367));
#237983=CARTESIAN_POINT('Ctrl Pts',(-6.42677073654578,4.61308480433933,
46.4520957810424));
#237984=CARTESIAN_POINT('Ctrl Pts',(-6.42470744569853,4.61595794491736,
46.4519523484376));
#237985=CARTESIAN_POINT('Ctrl Pts',(-6.41977611291144,4.62281513349123,
46.4516095316173));
#237986=CARTESIAN_POINT('Ctrl Pts',(-6.41690629109887,4.62679789372693,
46.4514100204948));
#237987=CARTESIAN_POINT('Ctrl Pts',(-6.40831368005967,4.63869941203079,
46.4508126314973));
#237988=CARTESIAN_POINT('Ctrl Pts',(-6.40257995358048,4.64661020477595,
46.4504139638445));
#237989=CARTESIAN_POINT('Ctrl Pts',(-6.34698984029864,4.72300934463816,
46.4465482775541));
#237990=CARTESIAN_POINT('Ctrl Pts',(-6.29605281505008,4.79070091192116,
46.4430028325326));
#237991=CARTESIAN_POINT('Ctrl Pts',(-6.08546707048257,5.0613936472923,46.4283823619154));
#237992=CARTESIAN_POINT('Ctrl Pts',(-5.91701729527572,5.25732855099089,
46.4167753595818));
#237993=CARTESIAN_POINT('Ctrl Pts',(-5.33373177489051,5.87217890901269,
46.3779072500078));
#237994=CARTESIAN_POINT('Ctrl Pts',(-4.88160528106935,6.25309762320797,
46.3499414274239));
#237995=CARTESIAN_POINT('Ctrl Pts',(-4.12016044708525,6.76125015596907,
46.3093915908466));
#237996=CARTESIAN_POINT('Ctrl Pts',(-3.83801486155599,6.92530890395117,
46.2955137683405));
#237997=CARTESIAN_POINT('Ctrl Pts',(-3.52595838988207,7.08181245173011,
46.2813933372183));
#237998=CARTESIAN_POINT('Ctrl Pts',(-3.50535082630986,7.09203537538503,
46.2804662759181));
#237999=CARTESIAN_POINT('Ctrl Pts',(-3.47678514542058,7.10605120695807,
46.2791886468821));
#238000=CARTESIAN_POINT('Ctrl Pts',(-3.46886494757564,7.109920863096,46.2788351960316));
#238001=CARTESIAN_POINT('Ctrl Pts',(-3.45525896034505,7.11654033966704,
46.2782293561906));
#238002=CARTESIAN_POINT('Ctrl Pts',(-3.44957632366842,7.11929659984846,
46.2779767257125));
#238003=CARTESIAN_POINT('Ctrl Pts',(-3.4378844952586,7.12495022453766,46.277457773404));
#238004=CARTESIAN_POINT('Ctrl Pts',(-3.43187492585763,7.12784679959228,
46.2771914812712));
#238005=CARTESIAN_POINT('Ctrl Pts',(-3.4179527872306,7.13453549524244,46.2765756068396));
#238006=CARTESIAN_POINT('Ctrl Pts',(-3.41003755145934,7.13832206382818,
46.2762262324559));
#238007=CARTESIAN_POINT('Ctrl Pts',(-3.38509523954811,7.15020326021038,
46.2751277142923));
#238008=CARTESIAN_POINT('Ctrl Pts',(-3.36804545601702,7.1582502230721,46.2743803510417));
#238009=CARTESIAN_POINT('Ctrl Pts',(-3.11999583824539,7.27423943376218,
46.2635583934711));
#238010=CARTESIAN_POINT('Ctrl Pts',(-2.88392894132317,7.37101769589469,
46.2539092775393));
#238011=CARTESIAN_POINT('Ctrl Pts',(-2.45816857229417,7.52196973683812,
46.2374324778464));
#238012=CARTESIAN_POINT('Ctrl Pts',(-2.27036081818771,7.58077092814684,
46.230467930732));
#238013=CARTESIAN_POINT('Ctrl Pts',(-1.5998579774445,7.76354365030446,46.2063476036101));
#238014=CARTESIAN_POINT('Ctrl Pts',(-1.10788731374773,7.84886694339196,
46.19005935218));
#238015=CARTESIAN_POINT('Ctrl Pts',(-0.490210998109943,7.8967293271967,
46.1685260140483));
#238016=CARTESIAN_POINT('Ctrl Pts',(-0.369051197926477,7.90331833395652,
46.1642462393734));
#238017=CARTESIAN_POINT('Ctrl Pts',(-0.0326616750813311,7.91386001225206,
46.1520963967267));
#238018=CARTESIAN_POINT('Ctrl Pts',(0.182637893657517,7.91181879906,46.1440174185811));
#238019=CARTESIAN_POINT('Ctrl Pts',(0.410882353412002,7.9003338149808,46.1348772701185));
#238020=CARTESIAN_POINT('Ctrl Pts',(0.424193995312145,7.89963025377752,
46.1343421139178));
#238021=CARTESIAN_POINT('Ctrl Pts',(0.442470771810868,7.89861794008617,
46.1336044048347));
#238022=CARTESIAN_POINT('Ctrl Pts',(0.447437560064625,7.89833814021777,
46.1334036305564));
#238023=CARTESIAN_POINT('Ctrl Pts',(0.455944787830551,7.89785084235624,
46.1330592239558));
#238024=CARTESIAN_POINT('Ctrl Pts',(0.459485340559439,7.89764564914033,
46.1329157355235));
#238025=CARTESIAN_POINT('Ctrl Pts',(0.466390677394443,7.89724079015637,
46.1326355858701));
#238026=CARTESIAN_POINT('Ctrl Pts',(0.469755474767058,7.89704135455257,
46.1324989387917));
#238027=CARTESIAN_POINT('Ctrl Pts',(0.477830560657102,7.89655755522796,
46.1321706756795));
#238028=CARTESIAN_POINT('Ctrl Pts',(0.482540719983266,7.89627112763345,
46.1319789339037));
#238029=CARTESIAN_POINT('Ctrl Pts',(0.496757000986494,7.89539385955919,
46.1313994143855));
#238030=CARTESIAN_POINT('Ctrl Pts',(0.506262282690488,7.89479006783097,
46.1310108547932));
#238031=CARTESIAN_POINT('Ctrl Pts',(0.592795251856389,7.88913642675631,
46.1274638362563));
#238032=CARTESIAN_POINT('Ctrl Pts',(0.669743771186503,7.88297673824935,
46.1242397146186));
#238033=CARTESIAN_POINT('Ctrl Pts',(1.00689969050782,7.851015574393,46.1098436161027));
#238034=CARTESIAN_POINT('Ctrl Pts',(1.26581026973013,7.81344969823005,46.0980864655485));
#238035=CARTESIAN_POINT('Ctrl Pts',(1.98903841689542,7.67162352792478,46.0641367407087));
#238036=CARTESIAN_POINT('Ctrl Pts',(2.44651220492522,7.53821461255747,46.041407712751));
#238037=CARTESIAN_POINT('Ctrl Pts',(3.31494170402759,7.1975129799865,45.998324135843));
#238038=CARTESIAN_POINT('Ctrl Pts',(3.72539586055095,6.9938938100647,45.9779972051401));
#238039=CARTESIAN_POINT('Ctrl Pts',(4.19582424969576,6.7072883231408,45.955107865128));
#238040=CARTESIAN_POINT('Ctrl Pts',(4.27478097233938,6.65724464373,45.9512779243765));
#238041=CARTESIAN_POINT('Ctrl Pts',(4.36572519529921,6.5973178527296,45.9468779184628));
#238042=CARTESIAN_POINT('Ctrl Pts',(4.37859130219193,6.58878574115383,45.9462557052739));
#238043=CARTESIAN_POINT('Ctrl Pts',(4.39905322189861,6.57513008952619,45.9452665573415));
#238044=CARTESIAN_POINT('Ctrl Pts',(4.40666521883834,6.57003094308754,45.9448986758088));
#238045=CARTESIAN_POINT('Ctrl Pts',(4.42006581944261,6.5610203443173,45.9442511880732));
#238046=CARTESIAN_POINT('Ctrl Pts',(4.42585812493511,6.55711443128995,45.943971366806));
#238047=CARTESIAN_POINT('Ctrl Pts',(4.43780448421693,6.54903562709445,45.9433943494475));
#238048=CARTESIAN_POINT('Ctrl Pts',(4.44395784547117,6.54486172147018,45.9430971933014));
#238049=CARTESIAN_POINT('Ctrl Pts',(4.4596560689931,6.53418106483038,45.9423392368472));
#238050=CARTESIAN_POINT('Ctrl Pts',(4.46919259595945,6.52766206106103,45.9418789149905));
#238051=CARTESIAN_POINT('Ctrl Pts',(4.50771455168816,6.50120513385387,45.9400199829574));
#238052=CARTESIAN_POINT('Ctrl Pts',(4.53658132250954,6.48109470829839,45.9386281199425));
#238053=CARTESIAN_POINT('Ctrl Pts',(4.72269177450918,6.34958567964282,45.9296604984897));
#238054=CARTESIAN_POINT('Ctrl Pts',(4.87595969684265,6.23266227309692,45.9223056904432));
#238055=CARTESIAN_POINT('Ctrl Pts',(5.16674075911856,5.99353631383202,45.9083098725554));
#238056=CARTESIAN_POINT('Ctrl Pts',(5.30456368744701,5.8719073179548,45.9016556888451));
#238057=CARTESIAN_POINT('Ctrl Pts',(5.85465228922296,5.35126441174039,45.8747259680411));
#238058=CARTESIAN_POINT('Ctrl Pts',(6.22712389008861,4.91282587417699,45.8557056279231));
#238059=CARTESIAN_POINT('Ctrl Pts',(6.62366873227137,4.3276662542269,45.8303253884603));
#238060=CARTESIAN_POINT('Ctrl Pts',(6.6956314675118,4.21547147514043,45.8254528399837));
#238061=CARTESIAN_POINT('Ctrl Pts',(6.84074938123687,3.97612521736984,45.8149379417926));
#238062=CARTESIAN_POINT('Ctrl Pts',(6.91326288913124,3.84866428299787,45.8092563409422));
#238063=CARTESIAN_POINT('Ctrl Pts',(6.99007950811927,3.70445549718361,45.8027195315619));
#238064=CARTESIAN_POINT('Ctrl Pts',(6.99791418982556,3.68963399900479,45.8020466369318));
#238065=CARTESIAN_POINT('Ctrl Pts',(7.00927705363812,3.66797156880741,45.8010617299988));
#238066=CARTESIAN_POINT('Ctrl Pts',(7.0128424899835,3.661150154579,45.8007513797536));
#238067=CARTESIAN_POINT('Ctrl Pts',(7.01913060688919,3.64907680369912,45.8002017310208));
#238068=CARTESIAN_POINT('Ctrl Pts',(7.02185736584784,3.64382698948614,45.7999626110031));
#238069=CARTESIAN_POINT('Ctrl Pts',(7.02749501516782,3.6329430258095,45.7994666267695));
#238070=CARTESIAN_POINT('Ctrl Pts',(7.03040502391157,3.62730842587836,45.7992097248701));
#238071=CARTESIAN_POINT('Ctrl Pts',(7.03777087237578,3.61300389845012,45.7985572037536));
#238072=CARTESIAN_POINT('Ctrl Pts',(7.04221746144918,3.60432923674784,45.7981611937507));
#238073=CARTESIAN_POINT('Ctrl Pts',(7.05991018090416,3.56965553636934,45.7965771364491));
#238074=CARTESIAN_POINT('Ctrl Pts',(7.07302836460833,3.54359170008807,45.7953838269835));
#238075=CARTESIAN_POINT('Ctrl Pts',(7.16179569425834,3.36476772815613,45.7871812659395));
#238076=CARTESIAN_POINT('Ctrl Pts',(7.2326319366691,3.20967452797392,45.7799920601974));
#238077=CARTESIAN_POINT('Ctrl Pts',(7.3735800497196,2.87266468595254,45.764351034622));
#238078=CARTESIAN_POINT('Ctrl Pts',(7.442091699172,2.6901958106158,45.7558715124615));
#238079=CARTESIAN_POINT('Ctrl Pts',(7.63710636232333,2.10611451611819,45.7289449002622));
#238080=CARTESIAN_POINT('Ctrl Pts',(7.73834115391352,1.69682317771659,45.7104284615116));
#238081=CARTESIAN_POINT('Ctrl Pts',(7.81970503848471,1.20114579350319,45.6889167994172));
#238082=CARTESIAN_POINT('Ctrl Pts',(7.83164257362626,1.1206752279207,45.6854509870675));
#238083=CARTESIAN_POINT('Ctrl Pts',(7.84605522142712,1.01199720991207,45.6808067636892));
#238084=CARTESIAN_POINT('Ctrl Pts',(7.8496230466261,0.983940510441004,45.6796110512966));
#238085=CARTESIAN_POINT('Ctrl Pts',(7.88472396204376,0.695564166980198,
45.6673545787445));
#238086=CARTESIAN_POINT('Ctrl Pts',(7.90344690351887,0.4338412695229,45.6565178200312));
#238087=CARTESIAN_POINT('Ctrl Pts',(7.90994359474025,0.134513873435497,
45.6443994715032));
#238088=CARTESIAN_POINT('Ctrl Pts',(7.91048814677211,0.0973599680355795,
45.6428999347237));
#238089=CARTESIAN_POINT('Ctrl Pts',(7.91089923204992,0.0433431444362618,
45.6407265153664));
#238090=CARTESIAN_POINT('Ctrl Pts',(7.91097364256311,0.0264823913665555,
45.6400490617653));
#238091=CARTESIAN_POINT('Ctrl Pts',(7.91100980263998,-0.00324919136649711,
45.6388561571947));
#238092=CARTESIAN_POINT('Ctrl Pts',(7.91099404652836,-0.0161199149451286,
45.6383403104487));
#238093=CARTESIAN_POINT('Ctrl Pts',(7.91089655275947,-0.0427240193872596,
45.6372751984862));
#238094=CARTESIAN_POINT('Ctrl Pts',(7.91081046290157,-0.0564573445869161,
45.6367260130036));
#238095=CARTESIAN_POINT('Ctrl Pts',(7.91050204921107,-0.0912165795131029,
45.635337629187));
#238096=CARTESIAN_POINT('Ctrl Pts',(7.91023165753433,-0.112241989610785,
45.6344993072133));
#238097=CARTESIAN_POINT('Ctrl Pts',(7.90880248143647,-0.197069300870259,
45.6311230988658));
#238098=CARTESIAN_POINT('Ctrl Pts',(7.90695557248555,-0.26085766336606,
45.6285980157543));
#238099=CARTESIAN_POINT('Ctrl Pts',(7.89003433165123,-0.672884988251195,
45.61237452518));
#238100=CARTESIAN_POINT('Ctrl Pts',(7.85273020113686,-1.019835340228,45.5991405529902));
#238101=CARTESIAN_POINT('Ctrl Pts',(7.71081289093464,-1.83109198658558,
45.5686189010716));
#238102=CARTESIAN_POINT('Ctrl Pts',(7.58699601374979,-2.290634514008,45.5516977672314));
#238103=CARTESIAN_POINT('Ctrl Pts',(7.33027569981168,-2.98703881584404,
45.5242204971208));
#238104=CARTESIAN_POINT('Ctrl Pts',(7.22519672387178,-3.23293335779673,
45.5141157504508));
#238105=CARTESIAN_POINT('Ctrl Pts',(7.10029097383133,-3.48856536984689,
45.5027540650829));
#238106=CARTESIAN_POINT('Ctrl Pts',(7.09264562335316,-3.50408309085231,
45.5020608967));
#238107=CARTESIAN_POINT('Ctrl Pts',(7.08195090117628,-3.52561170015096,
45.5010942266304));
#238108=CARTESIAN_POINT('Ctrl Pts',(7.07894461562811,-3.53164403010793,
45.5008228181208));
#238109=CARTESIAN_POINT('Ctrl Pts',(7.07375425597294,-3.54202560864643,
45.5003547725307));
#238110=CARTESIAN_POINT('Ctrl Pts',(7.07157386776715,-3.54637670288162,
45.500158317618));
#238111=CARTESIAN_POINT('Ctrl Pts',(7.06706629545426,-3.5553511453646,45.4997525130845));
#238112=CARTESIAN_POINT('Ctrl Pts',(7.06473858690384,-3.55997422598885,
45.4995431372866));
#238113=CARTESIAN_POINT('Ctrl Pts',(7.05931079486258,-3.57072811888522,
45.4990553253989));
#238114=CARTESIAN_POINT('Ctrl Pts',(7.0562072622968,-3.5768571775396,45.4987767146655));
#238115=CARTESIAN_POINT('Ctrl Pts',(7.04666549501679,-3.59564013405746,
45.4979210648263));
#238116=CARTESIAN_POINT('Ctrl Pts',(7.04020120188754,-3.60828069932307,
45.4973426836424));
#238117=CARTESIAN_POINT('Ctrl Pts',(6.97010061293252,-3.74445298009451,
45.4910837943756));
#238118=CARTESIAN_POINT('Ctrl Pts',(6.90326121295536,-3.86629122503848,
45.4852216459464));
#238119=CARTESIAN_POINT('Ctrl Pts',(6.75942538110885,-4.11285262353395,
45.4728876073449));
#238120=CARTESIAN_POINT('Ctrl Pts',(6.68209761614589,-4.23732892812539,
45.466404404723));
#238121=CARTESIAN_POINT('Ctrl Pts',(6.42420408684024,-4.62783623698831,
45.4453852478108));
#238122=CARTESIAN_POINT('Ctrl Pts',(6.2308640963602,-4.88503740364512,45.4305074192471));
#238123=CARTESIAN_POINT('Ctrl Pts',(5.72735472129881,-5.47616573367393,
45.3947180364904));
#238124=CARTESIAN_POINT('Ctrl Pts',(5.40293077719033,-5.79649772187217,
45.3739711690651));
#238125=CARTESIAN_POINT('Ctrl Pts',(5.04738372681391,-6.0916243331638,45.3539804182439));
#238126=CARTESIAN_POINT('Ctrl Pts',(5.04201908182731,-6.09606537701818,
45.3536793609821));
#238127=CARTESIAN_POINT('Ctrl Pts',(5.01527016786991,-6.11814961501412,
45.3521810927908));
#238128=CARTESIAN_POINT('Ctrl Pts',(4.99379900570893,-6.13568749836777,
45.3509874950553));
#238129=CARTESIAN_POINT('Ctrl Pts',(4.80591426104648,-6.28751428864805,
45.3406217088511));
#238130=CARTESIAN_POINT('Ctrl Pts',(4.63420465355468,-6.41512307387998,
45.3316878048027));
#238131=CARTESIAN_POINT('Ctrl Pts',(4.44033715162932,-6.54734754518713,
45.3221691602431));
#238132=CARTESIAN_POINT('Ctrl Pts',(4.4231019807628,-6.55900318445198,45.3213276669488));
#238133=CARTESIAN_POINT('Ctrl Pts',(4.39744280911085,-6.57620859568392,
45.3200818483037));
#238134=CARTESIAN_POINT('Ctrl Pts',(4.38905391772956,-6.58181042430696,
45.3196756464177));
#238135=CARTESIAN_POINT('Ctrl Pts',(4.37467526437712,-6.59137230701359,
45.3189812876583));
#238136=CARTESIAN_POINT('Ctrl Pts',(4.3686907922502,-6.59534027329059,45.3186928463632));
#238137=CARTESIAN_POINT('Ctrl Pts',(4.35703847309424,-6.60304345131603,
45.3181323000038));
#238138=CARTESIAN_POINT('Ctrl Pts',(4.35137120504217,-6.60677952653373,
45.317860164055));
#238139=CARTESIAN_POINT('Ctrl Pts',(4.33780644471185,-6.61569689935402,
45.3172099761898));
#238140=CARTESIAN_POINT('Ctrl Pts',(4.32990446010047,-6.62087136131351,
45.3168321693279));
#238141=CARTESIAN_POINT('Ctrl Pts',(4.30619259917828,-6.63633800968059,
45.3157013077879));
#238142=CARTESIAN_POINT('Ctrl Pts',(4.2903551073974,-6.64658784177486,45.3149497665221));
#238143=CARTESIAN_POINT('Ctrl Pts',(4.15228885468236,-6.73524354212397,
45.308430624798));
#238144=CARTESIAN_POINT('Ctrl Pts',(4.0279561475674,-6.81032893379145,45.3027819222614));
#238145=CARTESIAN_POINT('Ctrl Pts',(3.56926012949443,-7.07038000079558,
45.2826753791903));
#238146=CARTESIAN_POINT('Ctrl Pts',(3.22367015589914,-7.2344917770006,45.2689281102694));
#238147=CARTESIAN_POINT('Ctrl Pts',(2.52855275112702,-7.50484174369433,
45.2428137832711));
#238148=CARTESIAN_POINT('Ctrl Pts',(2.18086279749248,-7.61315069583241,
45.2304359977541));
#238149=CARTESIAN_POINT('Ctrl Pts',(1.64673179636296,-7.73992937044682,
45.2112850042528));
#238150=CARTESIAN_POINT('Ctrl Pts',(1.46506356731048,-7.77636274062096,
45.2047445353424));
#238151=CARTESIAN_POINT('Ctrl Pts',(1.03757546833957,-7.84658262609221,
45.1890153557494));
#238152=CARTESIAN_POINT('Ctrl Pts',(0.791113763081927,-7.87525001000017,
45.1796674161245));
#238153=CARTESIAN_POINT('Ctrl Pts',(0.52530832906285,-7.89356143452319,
45.1690424716581));
#238154=CARTESIAN_POINT('Ctrl Pts',(0.506909614258777,-7.89476431546944,
45.1683046517731));
#238155=CARTESIAN_POINT('Ctrl Pts',(0.480957323714662,-7.89636994244776,
45.1672607189268));
#238156=CARTESIAN_POINT('Ctrl Pts',(0.47340703412835,-7.89682619758156,
45.1669566259211));
#238157=CARTESIAN_POINT('Ctrl Pts',(0.460203647342578,-7.89760505878734,
45.1664241950331));
#238158=CARTESIAN_POINT('Ctrl Pts',(0.454550830320328,-7.89793242589721,
45.1661960332597));
#238159=CARTESIAN_POINT('Ctrl Pts',(0.442689811762091,-7.89860654752731,
45.1657168584562));
#238160=CARTESIAN_POINT('Ctrl Pts',(0.436481543543993,-7.89895205226282,
45.1654658000956));
#238161=CARTESIAN_POINT('Ctrl Pts',(0.421685784197907,-7.89975797455184,
45.1648668832787));
#238162=CARTESIAN_POINT('Ctrl Pts',(0.413097945615922,-7.90021170879171,
45.1645187863434));
#238163=CARTESIAN_POINT('Ctrl Pts',(0.385115460175408,-7.90164439805896,
45.1633830537415));
#238164=CARTESIAN_POINT('Ctrl Pts',(0.365718022450598,-7.90256593970965,
45.162593419539));
#238165=CARTESIAN_POINT('Ctrl Pts',(0.0741315556924383,-7.91534288226645,
45.1506899654776));
#238166=CARTESIAN_POINT('Ctrl Pts',(-0.198479376256622,-7.91320053288995,
45.1391311538104));
#238167=CARTESIAN_POINT('Ctrl Pts',(-1.03798266636762,-7.86319146982881,
45.1030281235171));
#238168=CARTESIAN_POINT('Ctrl Pts',(-1.60028562578764,-7.7682901021775,
45.078286348511));
#238169=CARTESIAN_POINT('Ctrl Pts',(-2.34249328756123,-7.55894653183966,
45.0458582466332));
#238170=CARTESIAN_POINT('Ctrl Pts',(-2.53525619925512,-7.49649426413489,
45.0374360336317));
#238171=CARTESIAN_POINT('Ctrl Pts',(-2.99457737418755,-7.32793515054033,
45.0172681513016));
#238172=CARTESIAN_POINT('Ctrl Pts',(-3.25817943566352,-7.21459622248732,
45.0055809705141));
#238173=CARTESIAN_POINT('Ctrl Pts',(-3.57153799931158,-7.05917939104955,
44.9914120968652));
#238174=CARTESIAN_POINT('Ctrl Pts',(-3.62769303037083,-7.03048651889441,
44.9888633056237));
#238175=CARTESIAN_POINT('Ctrl Pts',(-3.71063203770076,-6.9868498522256,
44.9850843294984));
#238176=CARTESIAN_POINT('Ctrl Pts',(-3.73768169953415,-6.97241683328406,
44.9838495330199));
#238177=CARTESIAN_POINT('Ctrl Pts',(-3.78591329980418,-6.94632033169141,
44.9816435883287));
#238178=CARTESIAN_POINT('Ctrl Pts',(-3.80712693898525,-6.93471629832611,
44.9806718822521));
#238179=CARTESIAN_POINT('Ctrl Pts',(-3.84798326401398,-6.9121235786435,
44.9787975552144));
#238180=CARTESIAN_POINT('Ctrl Pts',(-3.86763291042413,-6.90114796536284,
44.9778948141908));
#238181=CARTESIAN_POINT('Ctrl Pts',(-3.91027816743006,-6.87708845539374,
44.9759327566614));
#238182=CARTESIAN_POINT('Ctrl Pts',(-3.93325553581372,-6.86397274652391,
44.9748737772607));
#238183=CARTESIAN_POINT('Ctrl Pts',(-4.02507293746807,-6.8109500303309,
44.9706346606344));
#238184=CARTESIAN_POINT('Ctrl Pts',(-4.09337524098538,-6.77012051171215,
44.9674644089371));
#238185=CARTESIAN_POINT('Ctrl Pts',(-4.25557705942827,-6.66980792048567,
44.9598920416068));
#238186=CARTESIAN_POINT('Ctrl Pts',(-4.34886198285789,-6.60936257318151,
44.955501181235));
#238187=CARTESIAN_POINT('Ctrl Pts',(-4.70177928760292,-6.36997702317278,
44.9387291285415));
#238188=CARTESIAN_POINT('Ctrl Pts',(-4.95190290536343,-6.17753979015283,
44.9265110289741));
#238189=CARTESIAN_POINT('Ctrl Pts',(-5.45822152667925,-5.737434517197,44.9005739907985));
#238190=CARTESIAN_POINT('Ctrl Pts',(-5.71053168985345,-5.48636083463045,
44.8868933460029));
#238191=CARTESIAN_POINT('Ctrl Pts',(-6.00765592213653,-5.14791067155404,
44.8691207780525));
#238192=CARTESIAN_POINT('Ctrl Pts',(-6.06893232733867,-5.07552696022641,
44.8653541274941));
#238193=CARTESIAN_POINT('Ctrl Pts',(-6.14135536629102,-4.98678892817076,
44.860763292693));
#238194=CARTESIAN_POINT('Ctrl Pts',(-6.15376172311053,-4.97147123089405,
44.8599717804732));
#238195=CARTESIAN_POINT('Ctrl Pts',(-6.17404747217003,-4.94623284032787,
44.8586690057422));
#238196=CARTESIAN_POINT('Ctrl Pts',(-6.18196053394706,-4.93633927670484,
44.8581586555875));
#238197=CARTESIAN_POINT('Ctrl Pts',(-6.19578493978849,-4.91896948730705,
44.8572632017542));
#238198=CARTESIAN_POINT('Ctrl Pts',(-6.20170660918157,-4.91150149854571,
44.8568783866464));
#238199=CARTESIAN_POINT('Ctrl Pts',(-6.21344267413409,-4.8966457418733,
44.8561132176306));
#238200=CARTESIAN_POINT('Ctrl Pts',(-6.21925742486876,-4.88925827388927,
44.855732874729));
#238201=CARTESIAN_POINT('Ctrl Pts',(-6.23521012111914,-4.8689163416059,
44.8546859801475));
#238202=CARTESIAN_POINT('Ctrl Pts',(-6.24532078671114,-4.85594067769134,
44.8540186328727));
#238203=CARTESIAN_POINT('Ctrl Pts',(-6.28905064317848,-4.79945686536525,
44.8511154240065));
#238204=CARTESIAN_POINT('Ctrl Pts',(-6.32225586930292,-4.75563085296177,
44.8488676069389));
#238205=CARTESIAN_POINT('Ctrl Pts',(-6.41195798424915,-4.63463720616461,
44.8426797870547));
#238206=CARTESIAN_POINT('Ctrl Pts',(-6.46751630855158,-4.55678610336702,
44.8387180184373));
#238207=CARTESIAN_POINT('Ctrl Pts',(-6.65537496491862,-4.28319020282288,
44.8248919499331));
#238208=CARTESIAN_POINT('Ctrl Pts',(-6.78030859801647,-4.08254179281821,
44.8149238945223));
#238209=CARTESIAN_POINT('Ctrl Pts',(-7.13372370115756,-3.45385352866851,
44.784498602175));
#238210=CARTESIAN_POINT('Ctrl Pts',(-7.33200476137419,-3.01012614697774,
44.7641711620468));
#238211=CARTESIAN_POINT('Ctrl Pts',(-7.51194210097086,-2.48192977669456,
44.741441148462));
#238212=CARTESIAN_POINT('Ctrl Pts',(-7.53452375414921,-2.41250937540598,
44.7384799554686));
#238213=CARTESIAN_POINT('Ctrl Pts',(-7.56414407293966,-2.31697554156631,
44.7344389399165));
#238214=CARTESIAN_POINT('Ctrl Pts',(-7.57201431891645,-2.29112426063764,
44.7333488364948));
#238215=CARTESIAN_POINT('Ctrl Pts',(-7.5852391505688,-2.24687232741814,
44.7314884585909));
#238216=CARTESIAN_POINT('Ctrl Pts',(-7.59065960290408,-2.22849164736873,
44.7307173831222));
#238217=CARTESIAN_POINT('Ctrl Pts',(-7.60163615089809,-2.19076560450639,
44.7291380998129));
#238218=CARTESIAN_POINT('Ctrl Pts',(-7.60718531341491,-2.1714183647465,
44.7283299810722));
#238219=CARTESIAN_POINT('Ctrl Pts',(-7.61802338877394,-2.13307976462393,
44.7267320793164));
#238220=CARTESIAN_POINT('Ctrl Pts',(-7.62331526778823,-2.11408939373407,
44.7259422663055));
#238221=CARTESIAN_POINT('Ctrl Pts',(-7.63535777158823,-2.07024061416471,
44.7241223718093));
#238222=CARTESIAN_POINT('Ctrl Pts',(-7.64205808700295,-2.0453685979053,
44.7230928849345));
#238223=CARTESIAN_POINT('Ctrl Pts',(-7.659095115593,-1.98087349764613,44.7204303460047));
#238224=CARTESIAN_POINT('Ctrl Pts',(-7.66924589194999,-1.94120201785514,
44.7187994219176));
#238225=CARTESIAN_POINT('Ctrl Pts',(-7.83325781983586,-1.27883391880955,
44.6916758007861));
#238226=CARTESIAN_POINT('Ctrl Pts',(-7.91113768679704,-0.639744219957868,
44.6668472522222));
#238227=CARTESIAN_POINT('Ctrl Pts',(-7.91099981726586,0.00170035864730828,
44.6425804671265));
#238228=CARTESIAN_POINT('',(-7.91313519165583,0.000112501479813467,42.642361085604));
#238229=CARTESIAN_POINT('Ctrl Pts',(-7.91143166941437,0.00169103298945927,
44.6423315082371));
#238230=CARTESIAN_POINT('Ctrl Pts',(-7.91482057188058,0.894287429589468,
44.6064986371717));
#238231=CARTESIAN_POINT('Ctrl Pts',(-7.3389531910569,4.4250799800469,44.4646961888898));
#238232=CARTESIAN_POINT('Ctrl Pts',(-2.18951637767745,9.09795524730432,
44.2169241633916));
#238233=CARTESIAN_POINT('Ctrl Pts',(6.49039433236539,6.75072682562183,43.8990154317418));
#238234=CARTESIAN_POINT('Ctrl Pts',(8.71254627783232,-0.362491690837899,
43.6340914887007));
#238235=CARTESIAN_POINT('Ctrl Pts',(6.339535221574,-5.24393813728578,43.4221523342676));
#238236=CARTESIAN_POINT('Ctrl Pts',(1.9657803162333,-8.50293123149737,43.2102131798347));
#238237=CARTESIAN_POINT('Ctrl Pts',(-3.92045911912344,-7.79462844045021,
42.9982740254015));
#238238=CARTESIAN_POINT('Ctrl Pts',(-7.3291187982702,-3.69026847598658,
42.7913283977889));
#238239=CARTESIAN_POINT('Ctrl Pts',(-7.91165264643059,-1.18860184589039,
42.6903523473923));
#238240=CARTESIAN_POINT('Ctrl Pts',(-7.91313519165583,0.000112501479813467,
42.642361085604));
#238241=CARTESIAN_POINT('',(-7.91099999357494,-0.00031633835898803,38.6421995802722));
#238242=CARTESIAN_POINT('Ctrl Pts',(-7.91099999835655,0.000161253323083898,
42.6435915724384));
#238243=CARTESIAN_POINT('Ctrl Pts',(-7.91099870059755,0.0638286015180441,
42.6410668225085));
#238244=CARTESIAN_POINT('Ctrl Pts',(-7.91022881507591,0.127493277805992,
42.638529614139));
#238245=CARTESIAN_POINT('Ctrl Pts',(-7.90832539151437,0.206249592499511,
42.6353710381167));
#238246=CARTESIAN_POINT('Ctrl Pts',(-7.9079169564133,0.22135672748423,42.6347642479927));
#238247=CARTESIAN_POINT('Ctrl Pts',(-7.90714330592795,0.247228113755906,
42.6337234649721));
#238248=CARTESIAN_POINT('Ctrl Pts',(-7.90679939190703,0.257992976732809,
42.6332899181849));
#238249=CARTESIAN_POINT('Ctrl Pts',(-7.90611046252487,0.278260253947631,
42.6324727207975));
#238250=CARTESIAN_POINT('Ctrl Pts',(-7.90577029609844,0.287762817832992,
42.63208917522));
#238251=CARTESIAN_POINT('Ctrl Pts',(-7.9050362112272,0.307284959190939,
42.6313003848133));
#238252=CARTESIAN_POINT('Ctrl Pts',(-7.90464037354412,0.31730444560978,
42.6308950983097));
#238253=CARTESIAN_POINT('Ctrl Pts',(-7.9036728105286,0.340669235416282,
42.6299489135466));
#238254=CARTESIAN_POINT('Ctrl Pts',(-7.90308633337,0.354013883144208,42.6294076821203));
#238255=CARTESIAN_POINT('Ctrl Pts',(-7.90109918721431,0.396760740314834,
42.6276712079707));
#238256=CARTESIAN_POINT('Ctrl Pts',(-7.89956822106437,0.426156485313474,
42.6264728942297));
#238257=CARTESIAN_POINT('Ctrl Pts',(-7.89396496713785,0.523301666765553,
42.6224998320577));
#238258=CARTESIAN_POINT('Ctrl Pts',(-7.88918489844305,0.591006759762721,
42.6197100027726));
#238259=CARTESIAN_POINT('Ctrl Pts',(-7.84058482017965,1.17272008376745,
42.595588814592));
#238260=CARTESIAN_POINT('Ctrl Pts',(-7.74745509593689,1.68136534198015,
42.5735676573225));
#238261=CARTESIAN_POINT('Ctrl Pts',(-7.5220386691645,2.46875506434117,42.5393271557479));
#238262=CARTESIAN_POINT('Ctrl Pts',(-7.4219210303001,2.75516156289006,42.5268184404839));
#238263=CARTESIAN_POINT('Ctrl Pts',(-7.29236199789618,3.0670132149062,42.5131199356718));
#238264=CARTESIAN_POINT('Ctrl Pts',(-7.2789041760689,3.09881712585957,42.5117218180166));
#238265=CARTESIAN_POINT('Ctrl Pts',(-7.25607392047374,3.15180085256804,
42.5093905672729));
#238266=CARTESIAN_POINT('Ctrl Pts',(-7.24681597348907,3.17302940492572,
42.508455968599));
#238267=CARTESIAN_POINT('Ctrl Pts',(-7.22840792166405,3.21473841455266,
42.5066185157093));
#238268=CARTESIAN_POINT('Ctrl Pts',(-7.21926366441351,3.23522121402781,
42.5057155958044));
#238269=CARTESIAN_POINT('Ctrl Pts',(-7.20180576779138,3.273883669975,42.5040101146665));
#238270=CARTESIAN_POINT('Ctrl Pts',(-7.19351010009055,3.29207123923967,
42.5032073317));
#238271=CARTESIAN_POINT('Ctrl Pts',(-7.17456817545133,3.33318638862942,
42.5013913476605));
#238272=CARTESIAN_POINT('Ctrl Pts',(-7.16388077381466,3.35609479450021,
42.500378676122));
#238273=CARTESIAN_POINT('Ctrl Pts',(-7.13600576372836,3.41510489672469,
42.4977677206586));
#238274=CARTESIAN_POINT('Ctrl Pts',(-7.11865389642515,3.45112828501532,
42.4961715043756));
#238275=CARTESIAN_POINT('Ctrl Pts',(-6.98457416611006,3.72417073743901,
42.4840523910024));
#238276=CARTESIAN_POINT('Ctrl Pts',(-6.8563104951417,3.95534242720663,42.4736776131043));
#238277=CARTESIAN_POINT('Ctrl Pts',(-6.69361097697219,4.21680046069988,
42.4616474514794));
#238278=CARTESIAN_POINT('Ctrl Pts',(-6.67019486193765,4.25374359303614,
42.4599408199053));
#238279=CARTESIAN_POINT('Ctrl Pts',(-6.40972029917303,4.65724925413542,
42.4412270910775));
#238280=CARTESIAN_POINT('Ctrl Pts',(-6.14301203832827,5.00378929000388,
42.4245490659468));
#238281=CARTESIAN_POINT('Ctrl Pts',(-5.61542258507756,5.58313268729837,
42.3950732033718));
#238282=CARTESIAN_POINT('Ctrl Pts',(-5.3651465527745,5.82404849341945,42.3821969794744));
#238283=CARTESIAN_POINT('Ctrl Pts',(-4.92895650299121,6.19187285391271,
42.3607111520235));
#238284=CARTESIAN_POINT('Ctrl Pts',(-4.75201995878336,6.32868093484177,
42.3522170410829));
#238285=CARTESIAN_POINT('Ctrl Pts',(-4.5184609321609,6.49394689255161,42.3410525639834));
#238286=CARTESIAN_POINT('Ctrl Pts',(-4.4669619645894,6.52947823729085,42.3385934462071));
#238287=CARTESIAN_POINT('Ctrl Pts',(-4.38323240422503,6.58579264624337,
42.3345924147162));
#238288=CARTESIAN_POINT('Ctrl Pts',(-4.3512623082631,6.60695901010832,42.3330640497093));
#238289=CARTESIAN_POINT('Ctrl Pts',(-4.3117857028548,6.63268438148475,42.3311747304916));
#238290=CARTESIAN_POINT('Ctrl Pts',(-4.30442355069523,6.63746457220562,
42.3308222945574));
#238291=CARTESIAN_POINT('Ctrl Pts',(-4.29016086689439,6.646691517374,42.3301393242249));
#238292=CARTESIAN_POINT('Ctrl Pts',(-4.28326133731275,6.65113980507829,
42.3298088505483));
#238293=CARTESIAN_POINT('Ctrl Pts',(-4.2712542389336,6.65885463003269,42.3292335620636));
#238294=CARTESIAN_POINT('Ctrl Pts',(-4.26614980919285,6.66212605425707,
42.3289889427032));
#238295=CARTESIAN_POINT('Ctrl Pts',(-4.25550461176271,6.66893130024049,
42.3284786720217));
#238296=CARTESIAN_POINT('Ctrl Pts',(-4.24996319315084,6.67246409091946,
42.328212979319));
#238297=CARTESIAN_POINT('Ctrl Pts',(-4.23640167640157,6.68108614364804,
42.3275625691861));
#238298=CARTESIAN_POINT('Ctrl Pts',(-4.22837681288277,6.68616786732243,
42.327177543004));
#238299=CARTESIAN_POINT('Ctrl Pts',(-4.19765897270355,6.70554243936984,
42.3257030768762));
#238300=CARTESIAN_POINT('Ctrl Pts',(-4.17490267052612,6.71973421550902,
42.3246094136083));
#238301=CARTESIAN_POINT('Ctrl Pts',(-3.83400822828007,6.92993011537489,
42.3082004016254));
#238302=CARTESIAN_POINT('Ctrl Pts',(-3.50251849300235,7.10322450315396,
42.2916822566228));
#238303=CARTESIAN_POINT('Ctrl Pts',(-2.88859882580964,7.37072755434766,
42.2612754480296));
#238304=CARTESIAN_POINT('Ctrl Pts',(-2.61067170306401,7.47368859428964,
42.2476094290269));
#238305=CARTESIAN_POINT('Ctrl Pts',(-2.25540895700324,7.58305750969555,
42.2306489468922));
#238306=CARTESIAN_POINT('Ctrl Pts',(-2.18287539235076,7.60425446415045,
42.2272114130834));
#238307=CARTESIAN_POINT('Ctrl Pts',(-1.96843893145003,7.66359957183411,
42.2171339901846));
#238308=CARTESIAN_POINT('Ctrl Pts',(-1.82576177469744,7.69883797427789,
42.2105384219362));
#238309=CARTESIAN_POINT('Ctrl Pts',(-1.43063361459529,7.78482382225821,
42.1926305645198));
#238310=CARTESIAN_POINT('Ctrl Pts',(-1.17655050986805,7.82725612401495,
42.1815166821291));
#238311=CARTESIAN_POINT('Ctrl Pts',(-0.80939899044334,7.87028479958545,
42.166096023552));
#238312=CARTESIAN_POINT('Ctrl Pts',(-0.697695034915772,7.88097281613747,
42.1614872222848));
#238313=CARTESIAN_POINT('Ctrl Pts',(-0.568604925504825,7.8905580717715,
42.1562549250558));
#238314=CARTESIAN_POINT('Ctrl Pts',(-0.551407257854619,7.89177852490375,
42.1555597779375));
#238315=CARTESIAN_POINT('Ctrl Pts',(-0.525325112893288,7.89354380182114,
42.1545083907135));
#238316=CARTESIAN_POINT('Ctrl Pts',(-0.516443532063122,7.89412986366183,
42.1541508747595));
#238317=CARTESIAN_POINT('Ctrl Pts',(-0.501068162266608,7.89511836690642,
42.1535328328762));
#238318=CARTESIAN_POINT('Ctrl Pts',(-0.494574840011914,7.89552778847505,
42.1532720909362));
#238319=CARTESIAN_POINT('Ctrl Pts',(-0.481108193446497,7.89636021924944,
42.1527318893854));
#238320=CARTESIAN_POINT('Ctrl Pts',(-0.474134797297655,7.89678200283286,
42.1524524679748));
#238321=CARTESIAN_POINT('Ctrl Pts',(-0.45513379795647,7.89790601247448,
42.1516919459518));
#238322=CARTESIAN_POINT('Ctrl Pts',(-0.443105112664125,7.89859000180985,
42.1512114113679));
#238323=CARTESIAN_POINT('Ctrl Pts',(-0.397690237275794,7.90106836627447,
42.1494005753619));
#238324=CARTESIAN_POINT('Ctrl Pts',(-0.364294133291213,7.90267857579063,
42.1480759952152));
#238325=CARTESIAN_POINT('Ctrl Pts',(0.154392163748717,7.9243923523408,42.1276105879979));
#238326=CARTESIAN_POINT('Ctrl Pts',(0.640527675438196,7.89997628448017,
42.1099744137218));
#238327=CARTESIAN_POINT('Ctrl Pts',(1.37927812403532,7.79418870521098,42.0840395769463));
#238328=CARTESIAN_POINT('Ctrl Pts',(1.63517736337208,7.74454538581923,42.0752005077116));
#238329=CARTESIAN_POINT('Ctrl Pts',(2.27953144422728,7.58617691457483,42.052626486232));
#238330=CARTESIAN_POINT('Ctrl Pts',(2.66295556603332,7.46022598293077,42.038901452621));
#238331=CARTESIAN_POINT('Ctrl Pts',(3.14754722139484,7.25890471335881,42.019492909002));
#238332=CARTESIAN_POINT('Ctrl Pts',(3.25890930042056,7.20959492743243,42.0148818912178));
#238333=CARTESIAN_POINT('Ctrl Pts',(3.42049917552824,7.13353597706497,42.0079107646925));
#238334=CARTESIAN_POINT('Ctrl Pts',(3.47165056578738,7.10878275110357,42.0056619575579));
#238335=CARTESIAN_POINT('Ctrl Pts',(3.53076560766431,7.07938555444326,42.0030092680924));
#238336=CARTESIAN_POINT('Ctrl Pts',(3.53899435623791,7.07527558119831,42.0026387975371));
#238337=CARTESIAN_POINT('Ctrl Pts',(3.55150024029925,7.06900205248514,42.0020738823564));
#238338=CARTESIAN_POINT('Ctrl Pts',(3.55578263179744,7.06684893358418,42.0018801021677));
#238339=CARTESIAN_POINT('Ctrl Pts',(3.56354105169646,7.06293928482301,42.0015284161103));
#238340=CARTESIAN_POINT('Ctrl Pts',(3.56701774782794,7.06118407597467,42.0013705951262));
#238341=CARTESIAN_POINT('Ctrl Pts',(3.57447816624742,7.05741077037642,42.0010314540196));
#238342=CARTESIAN_POINT('Ctrl Pts',(3.57846147677908,7.05539186734896,42.0008500817292));
#238343=CARTESIAN_POINT('Ctrl Pts',(3.58912611960712,7.04997523984261,42.0003636894633));
#238344=CARTESIAN_POINT('Ctrl Pts',(3.59580432120636,7.04657139803977,42.0000582702541));
#238345=CARTESIAN_POINT('Ctrl Pts',(3.62705729328857,7.03058593637707,41.9986249740378));
#238346=CARTESIAN_POINT('Ctrl Pts',(3.65157054174572,7.01788541840043,41.9974892015698));
#238347=CARTESIAN_POINT('Ctrl Pts',(4.06845019056466,6.79912111484412,41.9779835261067));
#238348=CARTESIAN_POINT('Ctrl Pts',(4.44285243392775,6.56058896109704,41.9576218471729));
#238349=CARTESIAN_POINT('Ctrl Pts',(5.10703314298491,6.054401489337,41.9188452271468));
#238350=CARTESIAN_POINT('Ctrl Pts',(5.40071668941503,5.79394975465895,41.900530795568));
#238351=CARTESIAN_POINT('Ctrl Pts',(5.79814124642927,5.38491140359518,41.8748787660774));
#238352=CARTESIAN_POINT('Ctrl Pts',(5.91803707394898,5.25286161115937,41.8670006677436));
#238353=CARTESIAN_POINT('Ctrl Pts',(6.13349685031662,4.99880982487135,41.8526218867711));
#238354=CARTESIAN_POINT('Ctrl Pts',(6.23013733241971,4.87783516662728,41.8460793770987));
#238355=CARTESIAN_POINT('Ctrl Pts',(6.37079399765316,4.69075528225316,41.8364156828291));
#238356=CARTESIAN_POINT('Ctrl Pts',(6.41746445510188,4.62669987817769,41.833183577806));
#238357=CARTESIAN_POINT('Ctrl Pts',(6.47167544041893,4.54989623715831,41.8293971409052));
#238358=CARTESIAN_POINT('Ctrl Pts',(6.48015160032975,4.53781599616775,41.8288041511419));
#238359=CARTESIAN_POINT('Ctrl Pts',(6.49313774562894,4.51919752849987,41.8278941452395));
#238360=CARTESIAN_POINT('Ctrl Pts',(6.49767174606763,4.51267614239911,41.8275761411321));
#238361=CARTESIAN_POINT('Ctrl Pts',(6.50591270157564,4.50078476461483,41.826997619719));
#238362=CARTESIAN_POINT('Ctrl Pts',(6.50962284567701,4.49541699792591,41.82673697158));
#238363=CARTESIAN_POINT('Ctrl Pts',(6.51711626045318,4.48454693763668,41.8262101445558));
#238364=CARTESIAN_POINT('Ctrl Pts',(6.5208992145039,4.47904443187499,41.8259439787367));
#238365=CARTESIAN_POINT('Ctrl Pts',(6.53167685664295,4.46332518951311,41.8251850857048));
#238366=CARTESIAN_POINT('Ctrl Pts',(6.53865454718371,4.45309679004026,41.8246930537045));
#238367=CARTESIAN_POINT('Ctrl Pts',(6.56840559753406,4.40926487332594,41.8225920910825));
#238368=CARTESIAN_POINT('Ctrl Pts',(6.59094434609169,4.37550242949679,41.8209927214414));
#238369=CARTESIAN_POINT('Ctrl Pts',(6.93501445721856,3.85140321657824,41.7964521185822));
#238370=CARTESIAN_POINT('Ctrl Pts',(7.20133226115239,3.32695555952119,41.7759547822028));
#238371=CARTESIAN_POINT('Ctrl Pts',(7.53263720896423,2.44352334974857,41.7439858797529));
#238372=CARTESIAN_POINT('Ctrl Pts',(7.63523838939109,2.10108298526976,41.7321033063432));
#238373=CARTESIAN_POINT('Ctrl Pts',(7.78446248100036,1.44435950833828,41.7085545272018));
#238374=CARTESIAN_POINT('Ctrl Pts',(7.83599010499158,1.13192336618629,41.6970303396375));
#238375=CARTESIAN_POINT('Ctrl Pts',(7.86987714827276,0.805661861619268,
41.6838908718752));
#238376=CARTESIAN_POINT('Ctrl Pts',(7.87105781337322,0.79404424294889,41.6834215486685));
#238377=CARTESIAN_POINT('Ctrl Pts',(7.87271497859607,0.777370987452586,
41.682745855618));
#238378=CARTESIAN_POINT('Ctrl Pts',(7.87321234218713,0.772317422427499,
41.6825407751514));
#238379=CARTESIAN_POINT('Ctrl Pts',(7.87407027409981,0.763513271140609,
41.6821829985929));
#238380=CARTESIAN_POINT('Ctrl Pts',(7.87443302605777,0.759762933224345,
41.6820304400052));
#238381=CARTESIAN_POINT('Ctrl Pts',(7.87512830221276,0.752520781811202,
41.6817355416628));
#238382=CARTESIAN_POINT('Ctrl Pts',(7.87546118373133,0.749029002665477,
41.6815932238576));
#238383=CARTESIAN_POINT('Ctrl Pts',(7.87624427014324,0.740756542111757,
41.6812557407947));
#238384=CARTESIAN_POINT('Ctrl Pts',(7.87669244436285,0.735975675108506,
41.6810604519576));
#238385=CARTESIAN_POINT('Ctrl Pts',(7.87801595034233,0.721717583487722,
41.6804773021051));
#238386=CARTESIAN_POINT('Ctrl Pts',(7.8788785295607,0.712239214731559,41.6800886721552));
#238387=CARTESIAN_POINT('Ctrl Pts',(7.88665478920199,0.625047519095722,
41.6765048998713));
#238388=CARTESIAN_POINT('Ctrl Pts',(7.89243534955537,0.547239983336362,
41.6732428725542));
#238389=CARTESIAN_POINT('Ctrl Pts',(7.92032139550481,0.078054762570438,
41.653241515011));
#238390=CARTESIAN_POINT('Ctrl Pts',(7.91446008089835,-0.31440974453127,
41.6351453450269));
#238391=CARTESIAN_POINT('Ctrl Pts',(7.83315626379213,-1.22339376134746,
41.5924020090547));
#238392=CARTESIAN_POINT('Ctrl Pts',(7.73567680809133,-1.73620792553614,
41.5677256530961));
#238393=CARTESIAN_POINT('Ctrl Pts',(7.48743080959072,-2.57879933669016,
41.5284489605261));
#238394=CARTESIAN_POINT('Ctrl Pts',(7.36320480954451,-2.91463331157522,
41.5131310383426));
#238395=CARTESIAN_POINT('Ctrl Pts',(7.2053924350939,-3.26603699853198,41.4974969445848));
#238396=CARTESIAN_POINT('Ctrl Pts',(7.19399121978,-3.29107401465484,41.4963850956787));
#238397=CARTESIAN_POINT('Ctrl Pts',(7.17806155451168,-3.32557715373047,
41.4948556201981));
#238398=CARTESIAN_POINT('Ctrl Pts',(7.1736445943426,-3.33509434963568,41.49443402614));
#238399=CARTESIAN_POINT('Ctrl Pts',(7.16616169906272,-3.3511340535668,41.4937239787043));
#238400=CARTESIAN_POINT('Ctrl Pts',(7.1631057670378,-3.35766119682825,41.4934351692039));
#238401=CARTESIAN_POINT('Ctrl Pts',(7.15704573331951,-3.37055885260953,
41.4928647443787));
#238402=CARTESIAN_POINT('Ctrl Pts',(7.15404203568944,-3.37692954614723,
41.4925831150505));
#238403=CARTESIAN_POINT('Ctrl Pts',(7.14740906999548,-3.39094916852007,
41.4919636269054));
#238404=CARTESIAN_POINT('Ctrl Pts',(7.14377602061087,-3.39859630513791,
41.4916259033775));
#238405=CARTESIAN_POINT('Ctrl Pts',(7.13107999928208,-3.42520961341242,
41.4904511948363));
#238406=CARTESIAN_POINT('Ctrl Pts',(7.1219536790369,-3.44414556234178,41.4896164724179));
#238407=CARTESIAN_POINT('Ctrl Pts',(7.03091379201953,-3.63113248627902,
41.481384381308));
#238408=CARTESIAN_POINT('Ctrl Pts',(6.94314036340964,-3.79627178594612,
41.4742006783067));
#238409=CARTESIAN_POINT('Ctrl Pts',(6.78769803070729,-4.06526511745037,
41.4625704802281));
#238410=CARTESIAN_POINT('Ctrl Pts',(6.72329665144036,-4.1709121911696,41.4580213458165));
#238411=CARTESIAN_POINT('Ctrl Pts',(6.6478364102031,-4.28840829465699,41.4529618441489));
#238412=CARTESIAN_POINT('Ctrl Pts',(6.63918970967433,-4.30178272812262,
41.4523859189581));
#238413=CARTESIAN_POINT('Ctrl Pts',(6.49978840723532,-4.5159826465098,41.4431612410853));
#238414=CARTESIAN_POINT('Ctrl Pts',(6.36001271808578,-4.71079526743562,
41.4347640706728));
#238415=CARTESIAN_POINT('Ctrl Pts',(5.94762925884295,-5.23367366748182,
41.4116790647961));
#238416=CARTESIAN_POINT('Ctrl Pts',(5.65704299298588,-5.54648263022499,
41.3972455682058));
#238417=CARTESIAN_POINT('Ctrl Pts',(5.21342635695285,-5.95271591715908,
41.3755003212993));
#238418=CARTESIAN_POINT('Ctrl Pts',(5.08027153275409,-6.06675173383288,
41.3690001665635));
#238419=CARTESIAN_POINT('Ctrl Pts',(4.89991148103098,-6.21111084628582,
41.3600751269425));
#238420=CARTESIAN_POINT('Ctrl Pts',(4.85601160993663,-6.24549287430204,
41.3578928487773));
#238421=CARTESIAN_POINT('Ctrl Pts',(4.79307237772491,-6.29372163776929,
41.3547526931519));
#238422=CARTESIAN_POINT('Ctrl Pts',(4.77432808708408,-6.30795261333543,
41.3538161298554));
#238423=CARTESIAN_POINT('Ctrl Pts',(4.74130836388819,-6.33279024433729,
41.3521642232574));
#238424=CARTESIAN_POINT('Ctrl Pts',(4.72706007890023,-6.34343284695367,
41.3514507415207));
#238425=CARTESIAN_POINT('Ctrl Pts',(4.70639121606066,-6.35876292330278,
41.3504149017802));
#238426=CARTESIAN_POINT('Ctrl Pts',(4.69999920577254,-6.36348895328019,
41.3500944432749));
#238427=CARTESIAN_POINT('Ctrl Pts',(4.68880052635003,-6.37174278934834,
41.3495328147075));
#238428=CARTESIAN_POINT('Ctrl Pts',(4.68399696528157,-6.37527481592008,
41.3492918483111));
#238429=CARTESIAN_POINT('Ctrl Pts',(4.67475425839886,-6.38205483203358,
41.3488280839328));
#238430=CARTESIAN_POINT('Ctrl Pts',(4.67031570795626,-6.38530362969092,
41.3486053245037));
#238431=CARTESIAN_POINT('Ctrl Pts',(4.65985349837133,-6.39294470102254,
41.3480801420297));
#238432=CARTESIAN_POINT('Ctrl Pts',(4.65382701820704,-6.39733308971132,
41.347777537933));
#238433=CARTESIAN_POINT('Ctrl Pts',(4.6360065892842,-6.4102711407821,41.346882493395));
#238434=CARTESIAN_POINT('Ctrl Pts',(4.62419525341872,-6.41879672906169,
41.3462889530326));
#238435=CARTESIAN_POINT('Ctrl Pts',(4.51903066034954,-6.49426509022223,
41.3410019171923));
#238436=CARTESIAN_POINT('Ctrl Pts',(4.42425554580203,-6.55919801382446,
41.3362210729431));
#238437=CARTESIAN_POINT('Ctrl Pts',(3.92744505071731,-6.8839085622763,41.3111847583723));
#238438=CARTESIAN_POINT('Ctrl Pts',(3.50385539283111,-7.10886818793583,
41.2899831386461));
#238439=CARTESIAN_POINT('Ctrl Pts',(2.75467613367001,-7.42342047050458,
41.2545014273808));
#238440=CARTESIAN_POINT('Ctrl Pts',(2.43892351605282,-7.53306581064085,
41.2400869403296));
#238441=CARTESIAN_POINT('Ctrl Pts',(1.89677820470627,-7.68364994717669,
41.2163940378961));
#238442=CARTESIAN_POINT('Ctrl Pts',(1.67382248801716,-7.73528078587551,
41.2069344648335));
#238443=CARTESIAN_POINT('Ctrl Pts',(1.39850149706047,-7.78657475691858,
41.1955620038474));
#238444=CARTESIAN_POINT('Ctrl Pts',(1.34797686153379,-7.79548018567544,
41.1934873433383));
#238445=CARTESIAN_POINT('Ctrl Pts',(1.27808558524441,-7.80709935651474,
41.1906338361787));
#238446=CARTESIAN_POINT('Ctrl Pts',(1.25879034363712,-7.81023367130875,
41.1898477917781));
#238447=CARTESIAN_POINT('Ctrl Pts',(1.22632560953256,-7.81538380311779,
41.1885281828534));
#238448=CARTESIAN_POINT('Ctrl Pts',(1.2131623115111,-7.81743792414354,41.1879939372384));
#238449=CARTESIAN_POINT('Ctrl Pts',(1.18718525132024,-7.82142442930598,
41.1869412295709));
#238450=CARTESIAN_POINT('Ctrl Pts',(1.17437180631286,-7.82335860011679,
41.1864227367381));
#238451=CARTESIAN_POINT('Ctrl Pts',(1.14620406064931,-7.82753971898799,
41.1852846187976));
#238452=CARTESIAN_POINT('Ctrl Pts',(1.13084777436115,-7.82977299251159,
41.1846652457046));
#238453=CARTESIAN_POINT('Ctrl Pts',(1.07744740976148,-7.83737866167482,
41.1825152327377));
#238454=CARTESIAN_POINT('Ctrl Pts',(1.03937067696906,-7.84251910005954,
41.1809889051577));
#238455=CARTESIAN_POINT('Ctrl Pts',(0.506717972341742,-7.91048096006713,
41.159730455763));
#238456=CARTESIAN_POINT('Ctrl Pts',(0.00731260741647796,-7.92669320504271,
41.1410341984355));
#238457=CARTESIAN_POINT('Ctrl Pts',(-0.90201145808582,-7.87022465470477,
41.1076974136502));
#238458=CARTESIAN_POINT('Ctrl Pts',(-1.31105361893869,-7.81250146625802,
41.0929345420716));
#238459=CARTESIAN_POINT('Ctrl Pts',(-1.86351271515144,-7.68991452212968,
41.0717721792114));
#238460=CARTESIAN_POINT('Ctrl Pts',(-2.01230659331713,-7.65232540870932,
41.0659418603715));
#238461=CARTESIAN_POINT('Ctrl Pts',(-2.22716561755725,-7.59134653841591,
41.0572228361006));
#238462=CARTESIAN_POINT('Ctrl Pts',(-2.29416592661701,-7.57136785887135,
41.0544607076508));
#238463=CARTESIAN_POINT('Ctrl Pts',(-2.37218678289564,-7.54697230230424,
41.0511847181549));
#238464=CARTESIAN_POINT('Ctrl Pts',(-2.3834743888746,-7.54341506879274,
41.0507093013355));
#238465=CARTESIAN_POINT('Ctrl Pts',(-2.40069722003787,-7.53794486207966,
41.0499816058009));
#238466=CARTESIAN_POINT('Ctrl Pts',(-2.40663826782427,-7.53605016793063,
41.0497301680818));
#238467=CARTESIAN_POINT('Ctrl Pts',(-2.41743698034745,-7.532592215618,41.0492723738522));
#238468=CARTESIAN_POINT('Ctrl Pts',(-2.42229538866276,-7.53103127669919,
41.049066125727));
#238469=CARTESIAN_POINT('Ctrl Pts',(-2.43276060248113,-7.52765777468234,
41.0486212408881));
#238470=CARTESIAN_POINT('Ctrl Pts',(-2.4383668971224,-7.52584364682478,
41.0483825302795));
#238471=CARTESIAN_POINT('Ctrl Pts',(-2.45347245468287,-7.52093702365585,
41.0477383066767));
#238472=CARTESIAN_POINT('Ctrl Pts',(-2.46296787316416,-7.51783280301107,
41.0473322317163));
#238473=CARTESIAN_POINT('Ctrl Pts',(-2.50690719582342,-7.50337607847169,
41.0454478887469));
#238474=CARTESIAN_POINT('Ctrl Pts',(-2.54127835751409,-7.49180489411687,
41.0439588234731));
#238475=CARTESIAN_POINT('Ctrl Pts',(-3.33659015593797,-7.21795715504033,
41.0091334536547));
#238476=CARTESIAN_POINT('Ctrl Pts',(-4.05315067313634,-6.84132417149653,
40.9703917886254));
#238477=CARTESIAN_POINT('Ctrl Pts',(-4.97939950295789,-6.15708534962913,
40.9183549931759));
#238478=CARTESIAN_POINT('Ctrl Pts',(-5.24443306440607,-5.93296521418211,
40.9031176585472));
#238479=CARTESIAN_POINT('Ctrl Pts',(-5.59324502259268,-5.59630096841265,
40.8827411829602));
#238480=CARTESIAN_POINT('Ctrl Pts',(-5.69004090942325,-5.49785515395312,
40.8770448151079));
#238481=CARTESIAN_POINT('Ctrl Pts',(-5.79693849907084,-5.38328644139439,
40.8707011200634));
#238482=CARTESIAN_POINT('Ctrl Pts',(-5.80961431573372,-5.36960430390184,
40.8699480065784));
#238483=CARTESIAN_POINT('Ctrl Pts',(-5.82860683313839,-5.34895800861483,
40.8688182336109));
#238484=CARTESIAN_POINT('Ctrl Pts',(-5.83495965837832,-5.34202725368332,
40.8684401036363));
#238485=CARTESIAN_POINT('Ctrl Pts',(-5.84587360926192,-5.33007774199091,
40.8677900852868));
#238486=CARTESIAN_POINT('Ctrl Pts',(-5.85044065742265,-5.3250644226503,
40.8675179567374));
#238487=CARTESIAN_POINT('Ctrl Pts',(-5.85984123664472,-5.31471857015759,
40.8669575670575));
#238488=CARTESIAN_POINT('Ctrl Pts',(-5.86467394882794,-5.30938530085289,
40.8666693391533));
#238489=CARTESIAN_POINT('Ctrl Pts',(-5.87630393215415,-5.29651546766536,
40.8659753763027));
#238490=CARTESIAN_POINT('Ctrl Pts',(-5.88309399964106,-5.28897239495878,
40.8655699320696));
#238491=CARTESIAN_POINT('Ctrl Pts',(-5.90795268648622,-5.26124982671628,
40.8640845429697));
#238492=CARTESIAN_POINT('Ctrl Pts',(-5.92593223975613,-5.24099053542619,
40.8630081767097));
#238493=CARTESIAN_POINT('Ctrl Pts',(-6.22181759134387,-4.90411883986894,
40.8452596001976));
#238494=CARTESIAN_POINT('Ctrl Pts',(-6.47411235510459,-4.56588584959776,
40.8296579544249));
#238495=CARTESIAN_POINT('Ctrl Pts',(-7.04034076015635,-3.66480813162043,
40.7918176038611));
#238496=CARTESIAN_POINT('Ctrl Pts',(-7.31474470896616,-3.08085139283841,
40.7706197055535));
#238497=CARTESIAN_POINT('Ctrl Pts',(-7.57098143575211,-2.30125550977007,
40.7408230835879));
#238498=CARTESIAN_POINT('Ctrl Pts',(-7.62078809436649,-2.13052103914183,
40.7342001877652));
#238499=CARTESIAN_POINT('Ctrl Pts',(-7.68404135629249,-1.88294257598479,
40.7243011654923));
#238500=CARTESIAN_POINT('Ctrl Pts',(-7.70217209096954,-1.80734838724972,
40.7212374913821));
#238501=CARTESIAN_POINT('Ctrl Pts',(-7.72219683173286,-1.71807636936456,
40.7175785105827));
#238502=CARTESIAN_POINT('Ctrl Pts',(-7.72517332907833,-1.70464288098104,
40.717026843419));
#238503=CARTESIAN_POINT('Ctrl Pts',(-7.72968329499523,-1.68403414276137,
40.7161789388692));
#238504=CARTESIAN_POINT('Ctrl Pts',(-7.73124186100431,-1.67686437171393,
40.7158836613779));
#238505=CARTESIAN_POINT('Ctrl Pts',(-7.73406753038487,-1.66377794427556,
40.7153441936115));
#238506=CARTESIAN_POINT('Ctrl Pts',(-7.73533782557549,-1.6578619774857,
40.715100123017));
#238507=CARTESIAN_POINT('Ctrl Pts',(-7.73788008050035,-1.6459557590787,
40.7146085340985));
#238508=CARTESIAN_POINT('Ctrl Pts',(-7.73915187450848,-1.63996547649116,
40.7143610098755));
#238509=CARTESIAN_POINT('Ctrl Pts',(-7.74275558663714,-1.62289406768938,
40.713655058165));
#238510=CARTESIAN_POINT('Ctrl Pts',(-7.74507066474516,-1.61180942604657,
40.7131960228799));
#238511=CARTESIAN_POINT('Ctrl Pts',(-7.75486041985839,-1.56442775938644,
40.7112311692262));
#238512=CARTESIAN_POINT('Ctrl Pts',(-7.76210373800981,-1.52808371994476,
40.7097172880214));
#238513=CARTESIAN_POINT('Ctrl Pts',(-7.7699405016551,-1.4872679250133,40.7080104755257));
#238514=CARTESIAN_POINT('Ctrl Pts',(-7.77078586890594,-1.48284465118816,
40.7078254178229));
#238515=CARTESIAN_POINT('Ctrl Pts',(-7.83494860717424,-1.14555979643847,
40.6937077632809));
#238516=CARTESIAN_POINT('Ctrl Pts',(-7.87681762142771,-0.808984523196858,
40.6791532968308));
#238517=CARTESIAN_POINT('Ctrl Pts',(-7.90632403430723,-0.314033589777592,
40.6577503719093));
#238518=CARTESIAN_POINT('Ctrl Pts',(-7.91099952265989,-0.15704629847537,
40.6509581643851));
#238519=CARTESIAN_POINT('Ctrl Pts',(-7.91100234797369,0.772373789970606,
40.6108749923711));
#238520=CARTESIAN_POINT('Ctrl Pts',(-7.79788667119714,1.54064593551892,
40.578844518645));
#238521=CARTESIAN_POINT('Ctrl Pts',(-7.55062270443671,2.36205473388458,
40.5440179223328));
#238522=CARTESIAN_POINT('Ctrl Pts',(-7.52469935148756,2.44337995427355,
40.540562126901));
#238523=CARTESIAN_POINT('Ctrl Pts',(-7.48726342187173,2.55457034081584,
40.5358267958462));
#238524=CARTESIAN_POINT('Ctrl Pts',(-7.47687824320938,2.58480848789389,
40.5345379450999));
#238525=CARTESIAN_POINT('Ctrl Pts',(-7.45871756391708,2.63666093459443,
40.5323259268704));
#238526=CARTESIAN_POINT('Ctrl Pts',(-7.45103071614268,2.65830582374256,
40.5314019885384));
#238527=CARTESIAN_POINT('Ctrl Pts',(-7.43496316436037,2.70293213185022,
40.529495856555));
#238528=CARTESIAN_POINT('Ctrl Pts',(-7.42656991338957,2.72590878244444,
40.5285137882891));
#238529=CARTESIAN_POINT('Ctrl Pts',(-7.40668957857656,2.77955809941648,
40.5262191121037));
#238530=CARTESIAN_POINT('Ctrl Pts',(-7.39511829835713,2.81019912181624,
40.5249073162285));
#238531=CARTESIAN_POINT('Ctrl Pts',(-7.35675365339833,2.90991156737503,
40.5206342483615));
#238532=CARTESIAN_POINT('Ctrl Pts',(-7.3291801617614,2.97867888759196,40.5176807207594));
#238533=CARTESIAN_POINT('Ctrl Pts',(-7.04895884406455,3.65008135229361,
40.4887693267845));
#238534=CARTESIAN_POINT('Ctrl Pts',(-6.72353035685079,4.21960368041695,
40.46385531856));
#238535=CARTESIAN_POINT('Ctrl Pts',(-6.19674893016468,4.92290214617427,
40.4296839260125));
#238536=CARTESIAN_POINT('Ctrl Pts',(-6.05407085248918,5.09734090286663,
40.4208586935318));
#238537=CARTESIAN_POINT('Ctrl Pts',(-5.88616374296398,5.28561514880879,
40.4107634761776));
#238538=CARTESIAN_POINT('Ctrl Pts',(-5.86807612122627,5.3056888085986,40.4096795047913));
#238539=CARTESIAN_POINT('Ctrl Pts',(-5.84109823327695,5.33532218646695,
40.4080675396181));
#238540=CARTESIAN_POINT('Ctrl Pts',(-5.83228651665282,5.34495326363265,
40.4075417772004));
#238541=CARTESIAN_POINT('Ctrl Pts',(-5.81657685624194,5.36203858825917,
40.4066057133409));
#238542=CARTESIAN_POINT('Ctrl Pts',(-5.80968831254594,5.36950145329251,
40.4061956901212));
#238543=CARTESIAN_POINT('Ctrl Pts',(-5.79517818902847,5.38516072431975,
40.4053328871233));
#238544=CARTESIAN_POINT('Ctrl Pts',(-5.78755355013952,5.39335425988686,
40.4048800146035));
#238545=CARTESIAN_POINT('Ctrl Pts',(-5.76727022158068,5.4150584457735,40.4036765512428));
#238546=CARTESIAN_POINT('Ctrl Pts',(-5.75458154121131,5.42854078555881,
40.4029249978295));
#238547=CARTESIAN_POINT('Ctrl Pts',(-5.68454047870131,5.50244129261868,
40.3987835465537));
#238548=CARTESIAN_POINT('Ctrl Pts',(-5.62628457520848,5.56199444060645,
40.395365398516));
#238549=CARTESIAN_POINT('Ctrl Pts',(-5.44400371047081,5.74253974683037,
40.3847689166946));
#238550=CARTESIAN_POINT('Ctrl Pts',(-5.31693715025488,5.86038537166933,
40.3775195902244));
#238551=CARTESIAN_POINT('Ctrl Pts',(-4.79628416821656,6.31237380172243,
40.3485273933873));
#238552=CARTESIAN_POINT('Ctrl Pts',(-4.3742565208147,6.6118316471179,40.3266564531261));
#238553=CARTESIAN_POINT('Ctrl Pts',(-3.79644263484986,6.94213488557179,
40.2992621339574));
#238554=CARTESIAN_POINT('Ctrl Pts',(-3.66474689035937,7.01254910149011,
40.2931666450985));
#238555=CARTESIAN_POINT('Ctrl Pts',(-3.49626755928694,7.09658737874406,
40.2855436529132));
#238556=CARTESIAN_POINT('Ctrl Pts',(-3.46127141784807,7.11372191358679,
40.2839694948362));
#238557=CARTESIAN_POINT('Ctrl Pts',(-3.40547513865571,7.14053122766648,
40.2814740556934));
#238558=CARTESIAN_POINT('Ctrl Pts',(-3.38475713788507,7.15037525275031,
40.2805505748934));
#238559=CARTESIAN_POINT('Ctrl Pts',(-3.3459610811637,7.16860255018474,40.278826996598));
#238560=CARTESIAN_POINT('Ctrl Pts',(-3.32789360558772,7.17700788851833,
40.2780266210041));
#238561=CARTESIAN_POINT('Ctrl Pts',(-3.28751418085551,7.19560791417237,
40.2762428878666));
#238562=CARTESIAN_POINT('Ctrl Pts',(-3.26518616719312,7.20576727645902,
40.2752599843282));
#238563=CARTESIAN_POINT('Ctrl Pts',(-3.19941161439191,7.23532654752022,
40.2723743377453));
#238564=CARTESIAN_POINT('Ctrl Pts',(-3.15583677350629,7.25443858765414,
40.2704751798555));
#238565=CARTESIAN_POINT('Ctrl Pts',(-2.76477433797736,7.4217692765787,40.2535376005496));
#238566=CARTESIAN_POINT('Ctrl Pts',(-2.40724711869554,7.54531696811186,
40.2387646848321));
#238567=CARTESIAN_POINT('Ctrl Pts',(-1.69872307434632,7.73464329169606,
40.2103430583309));
#238568=CARTESIAN_POINT('Ctrl Pts',(-1.34938059035412,7.80317559349103,
40.1967986474047));
#238569=CARTESIAN_POINT('Ctrl Pts',(-0.497775541314349,7.9113201019901,
40.1644947463322));
#238570=CARTESIAN_POINT('Ctrl Pts',(0.00593936727166913,7.92696014748089,
40.1460161682002));
#238571=CARTESIAN_POINT('Ctrl Pts',(0.669194255993171,7.88430632434497,
40.1204784504287));
#238572=CARTESIAN_POINT('Ctrl Pts',(0.830320863652399,7.86896888133234,
40.1141705893205));
#238573=CARTESIAN_POINT('Ctrl Pts',(1.01010849946013,7.84627161771918,40.1069324370505));
#238574=CARTESIAN_POINT('Ctrl Pts',(1.02934969102803,7.84377056562541,40.1061552127109));
#238575=CARTESIAN_POINT('Ctrl Pts',(1.05737495349073,7.84002282632107,40.1050192000771));
#238576=CARTESIAN_POINT('Ctrl Pts',(1.06616650824992,7.83883209958511,40.1046622623202));
#238577=CARTESIAN_POINT('Ctrl Pts',(1.08169724998666,7.836702007757,40.1040306835718));
#238578=CARTESIAN_POINT('Ctrl Pts',(1.08843727092537,7.83576873101463,40.1037562486358));
#238579=CARTESIAN_POINT('Ctrl Pts',(1.10238863413474,7.83381856675941,40.1031874656906));
#238580=CARTESIAN_POINT('Ctrl Pts',(1.10959979136409,7.83280041493283,40.1028930744439));
#238581=CARTESIAN_POINT('Ctrl Pts',(1.1280979557436,7.8301625795568,40.1021368533298));
#238582=CARTESIAN_POINT('Ctrl Pts',(1.13938286488857,7.82852845084185,40.1016745182533));
#238583=CARTESIAN_POINT('Ctrl Pts',(1.18574710310853,7.82171223082387,40.099770787206));
#238584=CARTESIAN_POINT('Ctrl Pts',(1.2207946118134,7.81631875493454,40.0983217933654));
#238585=CARTESIAN_POINT('Ctrl Pts',(1.43957106662348,7.78114383205426,40.0892092610057));
#238586=CARTESIAN_POINT('Ctrl Pts',(1.6222076876335,7.74512698262287,40.0812696047363));
#238587=CARTESIAN_POINT('Ctrl Pts',(2.05357500590967,7.64413310936212,40.0618303084283));
#238588=CARTESIAN_POINT('Ctrl Pts',(2.30074261574574,7.57340838405021,40.0501737565286));
#238589=CARTESIAN_POINT('Ctrl Pts',(3.12962459886837,7.29190361439506,40.0101392731647));
#238590=CARTESIAN_POINT('Ctrl Pts',(3.68996569173267,7.02500741221093,39.981634394864));
#238591=CARTESIAN_POINT('Ctrl Pts',(4.36891174306192,6.5977452557836,39.947482330211));
#238592=CARTESIAN_POINT('Ctrl Pts',(4.52086260901511,6.49456999198483,39.9398489570674));
#238593=CARTESIAN_POINT('Ctrl Pts',(4.68616055607473,6.37371691234888,39.9315559304474));
#238594=CARTESIAN_POINT('Ctrl Pts',(4.70317852423507,6.36116968915161,39.9307022431757));
#238595=CARTESIAN_POINT('Ctrl Pts',(4.72794812632327,6.34275350588278,39.929459831041));
#238596=CARTESIAN_POINT('Ctrl Pts',(4.73573949836382,6.33693829274793,39.9290690440187));
#238597=CARTESIAN_POINT('Ctrl Pts',(4.74928361986323,6.32679049461528,39.9283897480596));
#238598=CARTESIAN_POINT('Ctrl Pts',(4.75504120159098,6.3224643958016,39.9281009894505));
#238599=CARTESIAN_POINT('Ctrl Pts',(4.76563212351459,6.31448399935484,39.9275698400554));
#238600=CARTESIAN_POINT('Ctrl Pts',(4.77046718520593,6.31083200139766,39.927327360621));
#238601=CARTESIAN_POINT('Ctrl Pts',(4.78346099146956,6.30099410991741,39.9266757317295));
#238602=CARTESIAN_POINT('Ctrl Pts',(4.79161194323275,6.29479791705815,39.9262669823544));
#238603=CARTESIAN_POINT('Ctrl Pts',(4.81905516219072,6.27385193398609,39.9248908127163));
#238604=CARTESIAN_POINT('Ctrl Pts',(4.83829162214233,6.25902907312811,39.9239262430707));
#238605=CARTESIAN_POINT('Ctrl Pts',(5.16869034430632,6.00200341938804,39.9073594147257));
#238606=CARTESIAN_POINT('Ctrl Pts',(5.46139734846983,5.736949378959,39.8927264229657));
#238607=CARTESIAN_POINT('Ctrl Pts',(6.01745508057288,5.15212604582466,39.8640915068873));
#238608=CARTESIAN_POINT('Ctrl Pts',(6.27794370802062,4.83131443334262,39.8501927590075));
#238609=CARTESIAN_POINT('Ctrl Pts',(6.79821587437285,4.07699817135065,39.8189553805546));
#238610=CARTESIAN_POINT('Ctrl Pts',(7.04392660354598,3.63601958059191,39.8015964760974));
#238611=CARTESIAN_POINT('Ctrl Pts',(7.25901019616077,3.14511343640741,39.7804013203069));
#238612=CARTESIAN_POINT('Ctrl Pts',(7.27181065256443,3.11540323767162,39.7791114907648));
#238613=CARTESIAN_POINT('Ctrl Pts',(7.28730603817542,3.07882220005217,39.7775138077519));
#238614=CARTESIAN_POINT('Ctrl Pts',(7.29017421320001,3.07202463761152,39.7772165189923));
#238615=CARTESIAN_POINT('Ctrl Pts',(7.29490271913841,3.06077418433231,39.7767238024391));
#238616=CARTESIAN_POINT('Ctrl Pts',(7.29676849669299,3.05632357491983,39.7765287104422));
#238617=CARTESIAN_POINT('Ctrl Pts',(7.3001335763186,3.04827589872604,39.7761756183));
#238618=CARTESIAN_POINT('Ctrl Pts',(7.30163429644865,3.04467942280767,39.7760177062426));
#238619=CARTESIAN_POINT('Ctrl Pts',(7.30483994126542,3.03698109386714,39.7756794403149));
#238620=CARTESIAN_POINT('Ctrl Pts',(7.30654406903454,3.03287891270207,39.7754990367912));
#238621=CARTESIAN_POINT('Ctrl Pts',(7.31114830290633,3.02176918531788,39.7750100400641));
#238622=CARTESIAN_POINT('Ctrl Pts',(7.31404178216675,3.01475891645706,39.7747010306974));
#238623=CARTESIAN_POINT('Ctrl Pts',(7.32895807282144,2.97847213023135,39.7730991453766));
#238624=CARTESIAN_POINT('Ctrl Pts',(7.34081498577084,2.94912833474925,39.7717957118249));
#238625=CARTESIAN_POINT('Ctrl Pts',(7.41214618164648,2.76950041500587,39.7637717178741));
#238626=CARTESIAN_POINT('Ctrl Pts',(7.46717632886497,2.61750169107085,39.7567906328849));
#238627=CARTESIAN_POINT('Ctrl Pts',(7.6425935150441,2.08230054402993,39.7318432890643));
#238628=CARTESIAN_POINT('Ctrl Pts',(7.73843080990549,1.69170914979968,39.7130258836722));
#238629=CARTESIAN_POINT('Ctrl Pts',(7.90947319428854,0.661372734536837,
39.6645049237019));
#238630=CARTESIAN_POINT('Ctrl Pts',(7.93707607450059,0.0166292319216803,
39.6354409402011));
#238631=CARTESIAN_POINT('Ctrl Pts',(7.88301626232736,-0.666127036516802,
39.6075237348211));
#238632=CARTESIAN_POINT('Ctrl Pts',(7.87938397631287,-0.707798594534086,
39.6058299266597));
#238633=CARTESIAN_POINT('Ctrl Pts',(7.87425824196206,-0.761661913541318,
39.6036534173758));
#238634=CARTESIAN_POINT('Ctrl Pts',(7.87306671358917,-0.773881293818122,
39.603160512756));
#238635=CARTESIAN_POINT('Ctrl Pts',(7.87111485122181,-0.793426902090646,
39.6023734446436));
#238636=CARTESIAN_POINT('Ctrl Pts',(7.87037272538773,-0.800754902556105,
39.6020786649584));
#238637=CARTESIAN_POINT('Ctrl Pts',(7.86896010012639,-0.814511954830978,
39.6015258399994));
#238638=CARTESIAN_POINT('Ctrl Pts',(7.86829195344806,-0.820941238776542,
39.6012677152625));
#238639=CARTESIAN_POINT('Ctrl Pts',(7.86677389097498,-0.83537678359513,
39.6006886786768));
#238640=CARTESIAN_POINT('Ctrl Pts',(7.86591963067793,-0.843382586103295,
39.600367914354));
#238641=CARTESIAN_POINT('Ctrl Pts',(7.86341024346504,-0.866564126086607,
39.5994401588033));
#238642=CARTESIAN_POINT('Ctrl Pts',(7.86172340541166,-0.88173643570895,
39.5988342432992));
#238643=CARTESIAN_POINT('Ctrl Pts',(7.84983915724431,-0.985883726085517,
39.5946838968042));
#238644=CARTESIAN_POINT('Ctrl Pts',(7.8381752333609,-1.07468657371834,39.5911894732191));
#238645=CARTESIAN_POINT('Ctrl Pts',(7.79976131148449,-1.33308578314917,
39.5811409899696));
#238646=CARTESIAN_POINT('Ctrl Pts',(7.76899527289545,-1.50203562170476,
39.5747231579468));
#238647=CARTESIAN_POINT('Ctrl Pts',(7.69079955105152,-1.86414336961229,
39.5612130823033));
#238648=CARTESIAN_POINT('Ctrl Pts',(7.64153601517832,-2.05678398142565,
39.554179662604));
#238649=CARTESIAN_POINT('Ctrl Pts',(7.35863999617281,-3.01158210706327,
39.5196356725454));
#238650=CARTESIAN_POINT('Ctrl Pts',(7.0180764893229,-3.73702445245757,39.4948757103241));
#238651=CARTESIAN_POINT('Ctrl Pts',(6.55071837234274,-4.43552897307171,
39.4619324958306));
#238652=CARTESIAN_POINT('Ctrl Pts',(6.52613167462745,-4.47162539624775,
39.4602004486837));
#238653=CARTESIAN_POINT('Ctrl Pts',(6.49678555560715,-4.51395168099094,
39.4581319095132));
#238654=CARTESIAN_POINT('Ctrl Pts',(6.49231374453956,-4.52038102105089,
39.4578166694836));
#238655=CARTESIAN_POINT('Ctrl Pts',(6.48511265210462,-4.53070165435446,
39.4573089578732));
#238656=CARTESIAN_POINT('Ctrl Pts',(6.4823894044477,-4.53459713756698,39.4571169389188));
#238657=CARTESIAN_POINT('Ctrl Pts',(6.47752182487494,-4.54154664551803,
39.4567736912171));
#238658=CARTESIAN_POINT('Ctrl Pts',(6.47537884746101,-4.54460160046006,
39.4566225646633));
#238659=CARTESIAN_POINT('Ctrl Pts',(6.47088541436579,-4.55099765345676,
39.4563056610577));
#238660=CARTESIAN_POINT('Ctrl Pts',(6.46853453141645,-4.55433844848692,
39.4561398520972));
#238661=CARTESIAN_POINT('Ctrl Pts',(6.46238463628175,-4.56306358014097,
39.4557060722785));
#238662=CARTESIAN_POINT('Ctrl Pts',(6.4585814894613,-4.56844498348352,39.4554377947126));
#238663=CARTESIAN_POINT('Ctrl Pts',(6.44200276932736,-4.59184157861496,
39.4542682334181));
#238664=CARTESIAN_POINT('Ctrl Pts',(6.42915862733806,-4.6098078146529,39.4533619183058));
#238665=CARTESIAN_POINT('Ctrl Pts',(6.33697283982645,-4.73762153613201,
39.4468569987781));
#238666=CARTESIAN_POINT('Ctrl Pts',(6.25489964491543,-4.84546272994121,
39.4410655121948));
#238667=CARTESIAN_POINT('Ctrl Pts',(6.04825966640609,-5.10297727938587,
39.4265959749351));
#238668=CARTESIAN_POINT('Ctrl Pts',(5.9208592967262,-5.25026091175052,39.4177677597876));
#238669=CARTESIAN_POINT('Ctrl Pts',(5.65165370940961,-5.53920886390032,
39.3995486536993));
#238670=CARTESIAN_POINT('Ctrl Pts',(5.50963163843938,-5.68049124530426,
39.3901556754905));
#238671=CARTESIAN_POINT('Ctrl Pts',(5.30779506440411,-5.86657906017108,
39.3772538121195));
#238672=CARTESIAN_POINT('Ctrl Pts',(5.25247838047507,-5.91615662337351,
39.3737608792202));
#238673=CARTESIAN_POINT('Ctrl Pts',(5.1346307563961,-6.01882170299738,39.3664193855873));
#238674=CARTESIAN_POINT('Ctrl Pts',(5.07195542982818,-6.07173088622744,
39.3625721246829));
#238675=CARTESIAN_POINT('Ctrl Pts',(4.98769380057236,-6.14064750997105,
39.357482595284));
#238676=CARTESIAN_POINT('Ctrl Pts',(4.96683279642721,-6.15753305064508,
39.3562291459551));
#238677=CARTESIAN_POINT('Ctrl Pts',(4.84816404091072,-6.25259176290216,
39.3491370728797));
#238678=CARTESIAN_POINT('Ctrl Pts',(4.7485956033084,-6.32854163513958,39.3433331587604));
#238679=CARTESIAN_POINT('Ctrl Pts',(4.25310540789064,-6.68821657910273,
39.3152339064891));
#238680=CARTESIAN_POINT('Ctrl Pts',(3.83332893144382,-6.93735195977141,
39.2939014058871));
#238681=CARTESIAN_POINT('Ctrl Pts',(3.36427164458332,-7.16007163635944,
39.2727834711049));
#238682=CARTESIAN_POINT('Ctrl Pts',(3.33521722870478,-7.17365148349033,
39.271485501209));
#238683=CARTESIAN_POINT('Ctrl Pts',(3.2958022348712,-7.19178257689446,39.2697381816599));
#238684=CARTESIAN_POINT('Ctrl Pts',(3.28551350961971,-7.19648872605534,
39.2692833065709));
#238685=CARTESIAN_POINT('Ctrl Pts',(3.26854048262703,-7.20420834464605,
39.2685349404013));
#238686=CARTESIAN_POINT('Ctrl Pts',(3.26186204141069,-7.20723461411041,
39.2682409944066));
#238687=CARTESIAN_POINT('Ctrl Pts',(3.24896859907966,-7.21305555768865,
39.2676744930654));
#238688=CARTESIAN_POINT('Ctrl Pts',(3.2427541770195,-7.21585149402628,39.2674018931087));
#238689=CARTESIAN_POINT('Ctrl Pts',(3.22845948657297,-7.22226063564699,
39.2667758639015));
#238690=CARTESIAN_POINT('Ctrl Pts',(3.22037674433235,-7.22586831951005,
39.2664226302322));
#238691=CARTESIAN_POINT('Ctrl Pts',(3.19519341552973,-7.23705810080611,
39.2653243750825));
#238692=CARTESIAN_POINT('Ctrl Pts',(3.1780719213602,-7.24459314151474,39.2645810140054));
#238693=CARTESIAN_POINT('Ctrl Pts',(2.98343878356135,-7.3294269522037,39.2561678659832));
#238694=CARTESIAN_POINT('Ctrl Pts',(2.8031676618595,-7.40024754997926,39.2487285214943));
#238695=CARTESIAN_POINT('Ctrl Pts',(2.30802229274416,-7.57407486475203,
39.2291011393963));
#238696=CARTESIAN_POINT('Ctrl Pts',(1.98898407430081,-7.66404182105322,
39.2173249318956));
#238697=CARTESIAN_POINT('Ctrl Pts',(1.30681986779557,-7.81092563168555,
39.1930191378243));
#238698=CARTESIAN_POINT('Ctrl Pts',(0.943482622422935,-7.86308904344701,
39.1805736772349));
#238699=CARTESIAN_POINT('Ctrl Pts',(0.359184972264966,-7.90588236407069,
39.1599403049664));
#238700=CARTESIAN_POINT('Ctrl Pts',(0.139962716899381,-7.91279922510106,
39.1520553092065));
#238701=CARTESIAN_POINT('Ctrl Pts',(-0.221047111317497,-7.90918244205259,
39.1384658144267));
#238702=CARTESIAN_POINT('Ctrl Pts',(-0.362756532939589,-7.90395047343957,
39.132964486278));
#238703=CARTESIAN_POINT('Ctrl Pts',(-0.519231561498289,-7.89395621367766,
39.1266913395954));
#238704=CARTESIAN_POINT('Ctrl Pts',(-0.534202161363723,-7.89295725090466,
39.1260892997371));
#238705=CARTESIAN_POINT('Ctrl Pts',(-0.55672519408571,-7.89138995483522,
39.1251808116274));
#238706=CARTESIAN_POINT('Ctrl Pts',(-0.564279852216511,-7.89085335112084,
39.1248756251144));
#238707=CARTESIAN_POINT('Ctrl Pts',(-0.577349614028726,-7.88990614698147,
39.1243468555256));
#238708=CARTESIAN_POINT('Ctrl Pts',(-0.582865086493773,-7.88950061003361,
39.1241234703382));
#238709=CARTESIAN_POINT('Ctrl Pts',(-0.594303099490266,-7.88864754585823,
39.123659713978));
#238710=CARTESIAN_POINT('Ctrl Pts',(-0.600225570156667,-7.88819913171024,
39.1234193087174));
#238711=CARTESIAN_POINT('Ctrl Pts',(-0.614102164234724,-7.8871327605112,
39.1228553858304));
#238712=CARTESIAN_POINT('Ctrl Pts',(-0.622055861457477,-7.88650944047409,
39.1225316646589));
#238713=CARTESIAN_POINT('Ctrl Pts',(-0.64777094388794,-7.88445504263871,
39.1214834637921));
#238714=CARTESIAN_POINT('Ctrl Pts',(-0.665528370603681,-7.88297599239676,
39.1207571980808));
#238715=CARTESIAN_POINT('Ctrl Pts',(-0.961642688585574,-7.85730438486096,
39.1086070511222));
#238716=CARTESIAN_POINT('Ctrl Pts',(-1.23851832859792,-7.81844267469711,
39.0966730025797));
#238717=CARTESIAN_POINT('Ctrl Pts',(-2.26868898926957,-7.61775005000018,
39.0511396957554));
#238718=CARTESIAN_POINT('Ctrl Pts',(-2.99919681267972,-7.36084965174593,
39.0170010411374));
#238719=CARTESIAN_POINT('Ctrl Pts',(-3.80154720339991,-6.93907036048083,
38.9795614679564));
#238720=CARTESIAN_POINT('Ctrl Pts',(-3.92040934276124,-6.87261599001586,
38.9740009093031));
#238721=CARTESIAN_POINT('Ctrl Pts',(-4.0630162838258,-6.78798203620403,
38.967300447851));
#238722=CARTESIAN_POINT('Ctrl Pts',(-4.0884479541028,-6.77269479515523,
38.9661043407375));
#238723=CARTESIAN_POINT('Ctrl Pts',(-4.1273302762464,-6.74902340832795,
38.9642738327391));
#238724=CARTESIAN_POINT('Ctrl Pts',(-4.14084268476378,-6.74074135667223,
38.9636373600786));
#238725=CARTESIAN_POINT('Ctrl Pts',(-4.16514113705716,-6.72574766766972,
38.9624922370781));
#238726=CARTESIAN_POINT('Ctrl Pts',(-4.17593606508903,-6.71905055511353,
38.961983286741));
#238727=CARTESIAN_POINT('Ctrl Pts',(-4.19893430486621,-6.70470574368689,
38.9608985301386));
#238728=CARTESIAN_POINT('Ctrl Pts',(-4.21113296480193,-6.69705066132884,
38.9603228824472));
#238729=CARTESIAN_POINT('Ctrl Pts',(-4.24399308143047,-6.67630451613915,
38.9587714914036));
#238730=CARTESIAN_POINT('Ctrl Pts',(-4.26461488405599,-6.6631508437261,
38.9577971021183));
#238731=CARTESIAN_POINT('Ctrl Pts',(-4.36662954372632,-6.59741292276161,
38.9529728854797));
#238732=CARTESIAN_POINT('Ctrl Pts',(-4.44711340348016,-6.54343134258716,
38.949154380549));
#238733=CARTESIAN_POINT('Ctrl Pts',(-5.13729534301404,-6.06189992185897,
38.9162852650773));
#238734=CARTESIAN_POINT('Ctrl Pts',(-5.68474661841976,-5.55176085948237,
38.8898898009307));
#238735=CARTESIAN_POINT('Ctrl Pts',(-6.345612358851,-4.73404902000102,38.8512052838017));
#238736=CARTESIAN_POINT('Ctrl Pts',(-6.52437542221823,-4.48447513137996,
38.8397045301339));
#238737=CARTESIAN_POINT('Ctrl Pts',(-6.69773345473422,-4.21006023195367,
38.8267469164493));
#238738=CARTESIAN_POINT('Ctrl Pts',(-6.70723004528729,-4.19491426605578,
38.8260307417187));
#238739=CARTESIAN_POINT('Ctrl Pts',(-6.72028619414195,-4.17393353813587,
38.8250371204291));
#238740=CARTESIAN_POINT('Ctrl Pts',(-6.72388969836193,-4.16812608204342,
38.8247619228636));
#238741=CARTESIAN_POINT('Ctrl Pts',(-6.73005956652532,-4.15815381665238,
38.824289074913));
#238742=CARTESIAN_POINT('Ctrl Pts',(-6.73262960495915,-4.15399127757514,
38.8240916153339));
#238743=CARTESIAN_POINT('Ctrl Pts',(-6.73763388694166,-4.14586929464999,
38.8237061550521));
#238744=CARTESIAN_POINT('Ctrl Pts',(-6.74006850512477,-4.14191008459247,
38.8235181741941));
#238745=CARTESIAN_POINT('Ctrl Pts',(-6.74590184169187,-4.13240506842805,
38.8230666818386));
#238746=CARTESIAN_POINT('Ctrl Pts',(-6.74929720889266,-4.12685721742079,
38.8228029933496));
#238747=CARTESIAN_POINT('Ctrl Pts',(-6.75952655077611,-4.11009662154917,
38.822005853868));
#238748=CARTESIAN_POINT('Ctrl Pts',(-6.76633942930401,-4.09887108278781,
38.8214712741906));
#238749=CARTESIAN_POINT('Ctrl Pts',(-6.83809994267305,-3.97996525406577,
38.8158009496879));
#238750=CARTESIAN_POINT('Ctrl Pts',(-6.90049212903592,-3.87077988264666,
38.810516976508));
#238751=CARTESIAN_POINT('Ctrl Pts',(-7.03306817711749,-3.62537485366121,
38.7985272381898));
#238752=CARTESIAN_POINT('Ctrl Pts',(-7.10195123930655,-3.48850621869802,
38.7917687265623));
#238753=CARTESIAN_POINT('Ctrl Pts',(-7.58304626281119,-2.45919381169649,
38.7408263405149));
#238754=CARTESIAN_POINT('Ctrl Pts',(-7.82978586759737,-1.49850900763372,
38.6938860509098));
#238755=CARTESIAN_POINT('Ctrl Pts',(-7.89711545381878,-0.470795646110987,
38.6514934850059));
#238756=CARTESIAN_POINT('Ctrl Pts',(-7.89974506321828,-0.424392577760123,
38.6495926731345));
#238757=CARTESIAN_POINT('Ctrl Pts',(-7.9032569944861,-0.350970695827668,
38.6466057750882));
#238758=CARTESIAN_POINT('Ctrl Pts',(-7.90440999868677,-0.323966265265489,
38.645511619673));
#238759=CARTESIAN_POINT('Ctrl Pts',(-7.90580520635408,-0.286823731104289,
38.6440126961079));
#238760=CARTESIAN_POINT('Ctrl Pts',(-7.90616634151718,-0.276690431204561,
38.6436043709949));
#238761=CARTESIAN_POINT('Ctrl Pts',(-7.90675041216298,-0.259365923096405,
38.6429073179335));
#238762=CARTESIAN_POINT('Ctrl Pts',(-7.90698302131279,-0.252175064862617,
38.6426183007084));
#238763=CARTESIAN_POINT('Ctrl Pts',(-7.90742979372104,-0.237754845543562,
38.6420393330728));
#238764=CARTESIAN_POINT('Ctrl Pts',(-7.90764385320122,-0.23052548772057,
38.6417493860273));
#238765=CARTESIAN_POINT('Ctrl Pts',(-7.90805392097528,-0.216003257010647,
38.6411675638293));
#238766=CARTESIAN_POINT('Ctrl Pts',(-7.90824975574135,-0.208710386087284,
38.6408756941452));
#238767=CARTESIAN_POINT('Ctrl Pts',(-7.90867410624758,-0.192048711219186,
38.6402095868746));
#238768=CARTESIAN_POINT('Ctrl Pts',(-7.90889606318929,-0.182679743604795,
38.6398355457794));
#238769=CARTESIAN_POINT('Ctrl Pts',(-7.90961151354725,-0.150029827977226,
38.6385338352241));
#238770=CARTESIAN_POINT('Ctrl Pts',(-7.91001886535678,-0.126747013976437,
38.63760874234));
#238771=CARTESIAN_POINT('Ctrl Pts',(-7.91077144928316,-0.069207562755391,
38.6353302278485));
#238772=CARTESIAN_POINT('Ctrl Pts',(-7.91099697586045,-0.0349497599870603,
38.6339803854939));
#238773=CARTESIAN_POINT('Ctrl Pts',(-7.91099996979002,-0.000691362661667347,
38.6326370762697));
#238774=CARTESIAN_POINT('',(-7.91099714850641,0.00671686857199988,36.6423315082371));
#238775=CARTESIAN_POINT('Ctrl Pts',(-7.91099999384339,-0.000312105552225759,
38.6423075098952));
#238776=CARTESIAN_POINT('Ctrl Pts',(-7.91100845698712,0.214204840705644,
38.633703106139));
#238777=CARTESIAN_POINT('Ctrl Pts',(-7.90228725669127,0.428551622663759,
38.6250987023827));
#238778=CARTESIAN_POINT('Ctrl Pts',(-7.88490367260169,0.642039775864754,
38.6164942986265));
#238779=CARTESIAN_POINT('Ctrl Pts',(-7.86749257111238,0.855865870816871,
38.607876274502));
#238780=CARTESIAN_POINT('Ctrl Pts',(-7.84139169850389,1.0688303849902,38.5992582503774));
#238781=CARTESIAN_POINT('Ctrl Pts',(-7.8067199407512,1.28025183720925,38.5906402262529));
#238782=CARTESIAN_POINT('Ctrl Pts',(-7.77197215411129,1.4921368983938,38.5820033043618));
#238783=CARTESIAN_POINT('Ctrl Pts',(-7.72861591878302,1.70247189396046,
38.5733663824707));
#238784=CARTESIAN_POINT('Ctrl Pts',(-7.67682144207909,1.9105846085517,38.5647294605796));
#238785=CARTESIAN_POINT('Ctrl Pts',(-7.62497517071932,2.11890543657738,
38.5560839017367));
#238786=CARTESIAN_POINT('Ctrl Pts',(-7.56467386178044,2.32499931604724,
38.5474383428938));
#238787=CARTESIAN_POINT('Ctrl Pts',(-7.49613763527628,2.5282091592656,38.538792784051));
#238788=CARTESIAN_POINT('Ctrl Pts',(-7.42750453073433,2.73170624576942,
38.5301350044481));
#238789=CARTESIAN_POINT('Ctrl Pts',(-7.35061330897551,2.93231092054215,
38.5214772248452));
#238790=CARTESIAN_POINT('Ctrl Pts',(-7.26573314758899,3.12938377768317,
38.5128194452423));
#238791=CARTESIAN_POINT('Ctrl Pts',(-7.20608463478069,3.26787435841868,
38.5067352947282));
#238792=CARTESIAN_POINT('Ctrl Pts',(-7.14249186566219,3.40462120763661,
38.5006511442142));
#238793=CARTESIAN_POINT('Ctrl Pts',(-7.0750620256049,3.53940931990685,38.4945669937001));
#238794=CARTESIAN_POINT('Ctrl Pts',(-6.9883054145714,3.7128304613219,38.4867390012391));
#238795=CARTESIAN_POINT('Ctrl Pts',(-6.89506198584002,3.88327317234364,
38.478911008778));
#238796=CARTESIAN_POINT('Ctrl Pts',(-6.79556355936849,4.05021442772887,
38.471083016317));
#238797=CARTESIAN_POINT('Ctrl Pts',(-6.69614917096623,4.2170146816804,38.4632616355119));
#238798=CARTESIAN_POINT('Ctrl Pts',(-6.59049048314436,4.38031906811435,
38.455440254707));
#238799=CARTESIAN_POINT('Ctrl Pts',(-6.47886629898294,4.53962690976947,
38.4476188739019));
#238800=CARTESIAN_POINT('Ctrl Pts',(-6.36731668231471,4.69882833016394,
38.4398027179572));
#238801=CARTESIAN_POINT('Ctrl Pts',(-6.24980970692534,4.85403823551805,
38.4319865620124));
#238802=CARTESIAN_POINT('Ctrl Pts',(-6.12666884578254,5.00478269799175,
38.4241704060676));
#238803=CARTESIAN_POINT('Ctrl Pts',(-6.00358714197187,5.15545474225958,
38.4163580050335));
#238804=CARTESIAN_POINT('Ctrl Pts',(-5.87487716579644,5.30166534453566,
38.4085456039994));
#238805=CARTESIAN_POINT('Ctrl Pts',(-5.74090433793375,5.44297146627589,
38.4007332029652));
#238806=CARTESIAN_POINT('Ctrl Pts',(-5.60697066885577,5.58423628579022,
38.3929230854101));
#238807=CARTESIAN_POINT('Ctrl Pts',(-5.4677774550567,5.72059922564389,38.3851129678549));
#238808=CARTESIAN_POINT('Ctrl Pts',(-5.32372895307522,5.85165199188987,
38.3773028502997));
#238809=CARTESIAN_POINT('Ctrl Pts',(-5.17967224363889,5.98271222513235,
38.3694922877473));
#238810=CARTESIAN_POINT('Ctrl Pts',(-5.03075994947666,6.1084614384403,38.3616817251948));
#238811=CARTESIAN_POINT('Ctrl Pts',(-4.8774319061609,6.22852944126971,38.3538711626424));
#238812=CARTESIAN_POINT('Ctrl Pts',(-4.75795500587992,6.32208931779827,
38.3477849843867));
#238813=CARTESIAN_POINT('Ctrl Pts',(-4.63579765713189,6.41220035023896,
38.341698806131));
#238814=CARTESIAN_POINT('Ctrl Pts',(-4.51118132570738,6.49870479761844,
38.3356126278753));
#238815=CARTESIAN_POINT('Ctrl Pts',(-4.33426723146526,6.6215125851782,38.326972261872));
#238816=CARTESIAN_POINT('Ctrl Pts',(-4.15248085579787,6.73699201908061,
38.3183318958687));
#238817=CARTESIAN_POINT('Ctrl Pts',(-3.96643163827274,6.84480394598041,
38.3096915298653));
#238818=CARTESIAN_POINT('Ctrl Pts',(-3.78007292961942,6.95279521700933,
38.3010367906942));
#238819=CARTESIAN_POINT('Ctrl Pts',(-3.58943740353826,7.05309337038577,
38.292382051523));
#238820=CARTESIAN_POINT('Ctrl Pts',(-3.39515819837377,7.14540564334982,
38.2837273123519));
#238821=CARTESIAN_POINT('Ctrl Pts',(-3.19487014829558,7.24057303470599,
38.2748048914935));
#238822=CARTESIAN_POINT('Ctrl Pts',(-2.99070969790356,7.32725258432475,
38.265882470635));
#238823=CARTESIAN_POINT('Ctrl Pts',(-2.78338977774932,7.40517807653,38.2569600497766));
#238824=CARTESIAN_POINT('Ctrl Pts',(-2.58161485771975,7.48101936542439,
38.2482762689134));
#238825=CARTESIAN_POINT('Ctrl Pts',(-2.37684751817603,7.54856879860471,
38.2395924880503));
#238826=CARTESIAN_POINT('Ctrl Pts',(-2.1697592267171,7.60763208219719,38.2309087071871));
#238827=CARTESIAN_POINT('Ctrl Pts',(-1.95413440900065,7.66913005327341,
38.221866966331));
#238828=CARTESIAN_POINT('Ctrl Pts',(-1.73599353148225,7.72142740611874,
38.2128252254749));
#238829=CARTESIAN_POINT('Ctrl Pts',(-1.51610670561192,7.76436355776818,
38.2037834846188));
#238830=CARTESIAN_POINT('Ctrl Pts',(-1.29621987974158,7.80729970941762,
38.1947417437627));
#238831=CARTESIAN_POINT('Ctrl Pts',(-1.07458738408571,7.84087463795251,
38.1857000029066));
#238832=CARTESIAN_POINT('Ctrl Pts',(-0.851987577295945,7.86498812256785,
38.1766582620505));
#238833=CARTESIAN_POINT('Ctrl Pts',(-0.647107318578418,7.88718210843792,
38.1683362682781));
#238834=CARTESIAN_POINT('Ctrl Pts',(-0.441233560333439,7.90137982551008,
38.1600142745056));
#238835=CARTESIAN_POINT('Ctrl Pts',(-0.235001561034966,7.90750879015073,
38.1516922807332));
#238836=CARTESIAN_POINT('Ctrl Pts',(-0.0289529880413066,7.9136323035843,
38.1433776886858));
#238837=CARTESIAN_POINT('Ctrl Pts',(0.177452899164308,7.91170137223193,
38.1350630966384));
#238838=CARTESIAN_POINT('Ctrl Pts',(0.383576684738589,7.90169538307602,
38.1267485045911));
#238839=CARTESIAN_POINT('Ctrl Pts',(0.589529710684304,7.89169768320603,
38.1184408006214));
#238840=CARTESIAN_POINT('Ctrl Pts',(0.795200810003176,7.87363828532877,
38.1101330966518));
#238841=CARTESIAN_POINT('Ctrl Pts',(0.99995067399829,7.84754863951606,38.1018253926821));
#238842=CARTESIAN_POINT('Ctrl Pts',(1.20449395460811,7.82148531698019,38.0935260708114));
#238843=CARTESIAN_POINT('Ctrl Pts',(1.40811756591243,7.78740795590163,38.0852267489406));
#238844=CARTESIAN_POINT('Ctrl Pts',(1.61018703286426,7.74539984243524,38.0769274270698));
#238845=CARTESIAN_POINT('Ctrl Pts',(1.81212739747043,7.70341856798647,38.0686334076425));
#238846=CARTESIAN_POINT('Ctrl Pts',(2.0125153127887,7.6535167074161,38.0603393882152));
#238847=CARTESIAN_POINT('Ctrl Pts',(2.21072478216942,7.59582891707692,38.0520453687879));
#238848=CARTESIAN_POINT('Ctrl Pts',(2.40878726936989,7.5381839051036,38.0437574997885));
#238849=CARTESIAN_POINT('Ctrl Pts',(2.60467425455987,7.47276456807297,38.0354696307892));
#238850=CARTESIAN_POINT('Ctrl Pts',(2.79777270488987,7.39975600217826,38.0271817617898));
#238851=CARTESIAN_POINT('Ctrl Pts',(2.8713807358158,7.37192555213036,38.0240224732685));
#238852=CARTESIAN_POINT('Ctrl Pts',(2.94458370948021,7.34299283840878,38.0208631847471));
#238853=CARTESIAN_POINT('Ctrl Pts',(3.0173482451762,7.31297002368614,38.0177038962258));
#238854=CARTESIAN_POINT('Ctrl Pts',(3.20396013851991,7.2359735274492,38.0096015863993));
#238855=CARTESIAN_POINT('Ctrl Pts',(3.3876085655808,7.15183612509522,38.0014992765729));
#238856=CARTESIAN_POINT('Ctrl Pts',(3.56773809816881,7.0608190645898,37.9933969667465));
#238857=CARTESIAN_POINT('Ctrl Pts',(3.74790738959376,6.96978191447212,37.9852928685491));
#238858=CARTESIAN_POINT('Ctrl Pts',(3.92455595283388,6.87186222152694,37.9771887703518));
#238859=CARTESIAN_POINT('Ctrl Pts',(4.09715270374799,6.76736734056683,37.9690846721544));
#238860=CARTESIAN_POINT('Ctrl Pts',(4.26980920095802,6.66283628753484,37.9609777686329));
#238861=CARTESIAN_POINT('Ctrl Pts',(4.43841081580003,6.55172567213123,37.9528708651113));
#238862=CARTESIAN_POINT('Ctrl Pts',(4.60245472775733,6.4343866435694,37.9447639615897));
#238863=CARTESIAN_POINT('Ctrl Pts',(4.76664658252704,6.31694179294026,37.9366497468665));
#238864=CARTESIAN_POINT('Ctrl Pts',(4.9262722610229,6.19325749019009,37.9285355321434));
#238865=CARTESIAN_POINT('Ctrl Pts',(5.08086030370299,6.06372654184332,37.9204213174202));
#238866=CARTESIAN_POINT('Ctrl Pts',(5.23552389854136,5.93413228754778,37.9123031370189));
#238867=CARTESIAN_POINT('Ctrl Pts',(5.38514470664768,5.79868589780636,37.9041849566175));
#238868=CARTESIAN_POINT('Ctrl Pts',(5.52928687788314,5.65781827404074,37.8960667762161));
#238869=CARTESIAN_POINT('Ctrl Pts',(5.67358406044154,5.51679916041943,37.8879398654766));
#238870=CARTESIAN_POINT('Ctrl Pts',(5.81239060997052,5.37034739094218,37.8798129547372));
#238871=CARTESIAN_POINT('Ctrl Pts',(5.94530888935037,5.21892931646056,37.8716860439978));
#238872=CARTESIAN_POINT('Ctrl Pts',(6.01583585765681,5.13858628320875,37.8673738727989));
#238873=CARTESIAN_POINT('Ctrl Pts',(6.08470572584131,5.05684558542534,37.8630617015999));
#238874=CARTESIAN_POINT('Ctrl Pts',(6.15186390298104,4.97378040520477,37.858749530401));
#238875=CARTESIAN_POINT('Ctrl Pts',(6.27642224235003,4.81971933106135,37.8507517420976));
#238876=CARTESIAN_POINT('Ctrl Pts',(6.39530611617561,4.66083294090514,37.8427539537941));
#238877=CARTESIAN_POINT('Ctrl Pts',(6.50813008396221,4.49757310226593,37.8347561654906));
#238878=CARTESIAN_POINT('Ctrl Pts',(6.62086193111673,4.33444656508584,37.8267649073716));
#238879=CARTESIAN_POINT('Ctrl Pts',(6.72754354352387,4.16695396967206,37.8187736492525));
#238880=CARTESIAN_POINT('Ctrl Pts',(6.82783007593749,3.99557973942749,37.8107823911334));
#238881=CARTESIAN_POINT('Ctrl Pts',(6.92805173036105,3.82431637567057,37.8027963027689));
#238882=CARTESIAN_POINT('Ctrl Pts',(7.02188638206704,3.64917666978696,37.7948102144045));
#238883=CARTESIAN_POINT('Ctrl Pts',(7.10903258373227,3.47067381403567,37.78682412604));
#238884=CARTESIAN_POINT('Ctrl Pts',(7.19613717947469,3.29225618031235,37.7788418504473));
#238885=CARTESIAN_POINT('Ctrl Pts',(7.27655954387214,3.11047889735802,37.7708595748546));
#238886=CARTESIAN_POINT('Ctrl Pts',(7.35004406976566,2.92587989714252,37.7628772992619));
#238887=CARTESIAN_POINT('Ctrl Pts',(7.42350596365979,2.74133775031768,37.754897482076));
#238888=CARTESIAN_POINT('Ctrl Pts',(7.49003415531645,2.55397592927376,37.7469176648901));
#238889=CARTESIAN_POINT('Ctrl Pts',(7.5494209388371,2.36435286880954,37.7389378477041));
#238890=CARTESIAN_POINT('Ctrl Pts',(7.61084854993877,2.16821340942876,37.7306838039978));
#238891=CARTESIAN_POINT('Ctrl Pts',(7.66463506173117,1.96965488086799,37.7224297602914));
#238892=CARTESIAN_POINT('Ctrl Pts',(7.71060635131985,1.7693136225627,37.7141757165851));
#238893=CARTESIAN_POINT('Ctrl Pts',(7.7550563337884,1.57560216702007,37.7061948202185));
#238894=CARTESIAN_POINT('Ctrl Pts',(7.79220000586526,1.38022442966616,37.698213923852));
#238895=CARTESIAN_POINT('Ctrl Pts',(7.82193174012489,1.18376722915736,37.6902330274855));
#238896=CARTESIAN_POINT('Ctrl Pts',(7.85167007520916,0.987266412641513,
37.6822503592581));
#238897=CARTESIAN_POINT('Ctrl Pts',(7.87399314149391,0.789685986156863,
37.6742676910307));
#238898=CARTESIAN_POINT('Ctrl Pts',(7.88884701985376,0.591619554565615,
37.6662850228033));
#238899=CARTESIAN_POINT('Ctrl Pts',(7.90370647925503,0.393478703558105,
37.6582993552513));
#238900=CARTESIAN_POINT('Ctrl Pts',(7.91109113082668,0.19485181704736,37.6503136876993));
#238901=CARTESIAN_POINT('Ctrl Pts',(7.91099915083615,-0.00366544263280774,
37.6423280201474));
#238902=CARTESIAN_POINT('Ctrl Pts',(7.9109071221447,-0.202287811830585,
37.6343381244005));
#238903=CARTESIAN_POINT('Ctrl Pts',(7.90333056992725,-0.40080010423743,
37.6263482286537));
#238904=CARTESIAN_POINT('Ctrl Pts',(7.88831971041271,-0.59860934365767,
37.6183583329068));
#238905=CARTESIAN_POINT('Ctrl Pts',(7.87329106929592,-0.796652904451298,
37.6103589724689));
#238906=CARTESIAN_POINT('Ctrl Pts',(7.85081055391816,-0.993991414902722,
37.602359612031));
#238907=CARTESIAN_POINT('Ctrl Pts',(7.82098008880441,-1.19003842396997,
37.594360251593));
#238908=CARTESIAN_POINT('Ctrl Pts',(7.79112877051456,-1.38622248094407,
37.5863552991514));
#238909=CARTESIAN_POINT('Ctrl Pts',(7.75391731762823,-1.58111290822961,
37.5783503467097));
#238910=CARTESIAN_POINT('Ctrl Pts',(7.70949829634302,-1.77413556942082,
37.570345394268));
#238911=CARTESIAN_POINT('Ctrl Pts',(7.66502130461008,-1.96741014093707,
37.5623299947102));
#238912=CARTESIAN_POINT('Ctrl Pts',(7.61331804226879,-2.1588117554832,37.5543145951523));
#238913=CARTESIAN_POINT('Ctrl Pts',(7.55459058646191,-2.34778237299396,
37.5462991955945));
#238914=CARTESIAN_POINT('Ctrl Pts',(7.54125967442368,-2.39067799387917,
37.5444797299801));
#238915=CARTESIAN_POINT('Ctrl Pts',(7.52756701912597,-2.43344843754376,
37.5426602643658));
#238916=CARTESIAN_POINT('Ctrl Pts',(7.51351532345902,-2.47608733370747,
37.5408407987515));
#238917=CARTESIAN_POINT('Ctrl Pts',(7.45357883045174,-2.65796046577115,
37.5330799995815));
#238918=CARTESIAN_POINT('Ctrl Pts',(7.38692818315501,-2.83797895846785,
37.5253192004114));
#238919=CARTESIAN_POINT('Ctrl Pts',(7.31369244998865,-3.01559674807144,
37.5175584012414));
#238920=CARTESIAN_POINT('Ctrl Pts',(7.24054562427867,-3.19299891143357,
37.5098070236049));
#238921=CARTESIAN_POINT('Ctrl Pts',(7.16082975950019,-3.36800584520122,
37.5020556459683));
#238922=CARTESIAN_POINT('Ctrl Pts',(7.07472422788984,-3.54008447629553,
37.4943042683318));
#238923=CARTESIAN_POINT('Ctrl Pts',(6.98870574909145,-3.71198913565495,
37.4865607273488));
#238924=CARTESIAN_POINT('Ctrl Pts',(6.89631062222946,-3.88097106769996,
37.4788171863659));
#238925=CARTESIAN_POINT('Ctrl Pts',(6.79776707992659,-4.04651501011258,
37.4710736453829));
#238926=CARTESIAN_POINT('Ctrl Pts',(6.69930319182685,-4.21192514090741,
37.4633363636186));
#238927=CARTESIAN_POINT('Ctrl Pts',(6.59470096549073,-4.37390250821271,
37.4555990818544));
#238928=CARTESIAN_POINT('Ctrl Pts',(6.4842355806927,-4.53195431729831,37.4478618000902));
#238929=CARTESIAN_POINT('Ctrl Pts',(6.37383712052952,-4.68991037186651,
37.4401292059008));
#238930=CARTESIAN_POINT('Ctrl Pts',(6.25758278008694,-4.84394531068987,
37.4323966117113));
#238931=CARTESIAN_POINT('Ctrl Pts',(6.13579232178727,-4.99359325374988,
37.4246640175219));
#238932=CARTESIAN_POINT('Ctrl Pts',(6.01405100795465,-5.14318081138638,
37.4169345435623));
#238933=CARTESIAN_POINT('Ctrl Pts',(5.88677825172797,-5.28838462093796,
37.4092050696027));
#238934=CARTESIAN_POINT('Ctrl Pts',(5.75433560554668,-5.42876991027781,
37.4014755956432));
#238935=CARTESIAN_POINT('Ctrl Pts',(5.62189509522726,-5.56915293566722,
37.3937462463344));
#238936=CARTESIAN_POINT('Ctrl Pts',(5.4842850992924,-5.70471732690519,37.3860168970257));
#238937=CARTESIAN_POINT('Ctrl Pts',(5.34190599268322,-5.83506309865927,
37.378287547717));
#238938=CARTESIAN_POINT('Ctrl Pts',(5.19952112985637,-5.96541414013762,
37.3705578859198));
#238939=CARTESIAN_POINT('Ctrl Pts',(5.05236703677377,-6.09054589860268,
37.3628282241227));
#238940=CARTESIAN_POINT('Ctrl Pts',(4.90087920027377,-6.21009694484103,
37.3550985623256));
#238941=CARTESIAN_POINT('Ctrl Pts',(4.74935748158953,-6.32967473019368,
37.3473671716911));
#238942=CARTESIAN_POINT('Ctrl Pts',(4.59350037119699,-6.44366909505734,
37.3396357810567));
#238943=CARTESIAN_POINT('Ctrl Pts',(4.43377454944196,-6.55176039280442,
37.3319043904223));
#238944=CARTESIAN_POINT('Ctrl Pts',(4.2739837266316,-6.65989567873293,37.3241698534678));
#238945=CARTESIAN_POINT('Ctrl Pts',(4.11032135462739,-6.7621229128854,37.3164353165133));
#238946=CARTESIAN_POINT('Ctrl Pts',(3.94328108648753,-6.85816704907002,
37.3087007795589));
#238947=CARTESIAN_POINT('Ctrl Pts',(3.77604410282847,-6.95432429194637,
37.3009571340016));
#238948=CARTESIAN_POINT('Ctrl Pts',(3.60542158991372,-7.04428371568233,
37.2932134884444));
#238949=CARTESIAN_POINT('Ctrl Pts',(3.43193060864663,-7.1278168675573,37.2854698428871));
#238950=CARTESIAN_POINT('Ctrl Pts',(3.25832846911384,-7.21140354037165,
37.2777212358604));
#238951=CARTESIAN_POINT('Ctrl Pts',(3.08185452803681,-7.28855559639948,
37.2699726288336));
#238952=CARTESIAN_POINT('Ctrl Pts',(2.90304347049441,-7.35909366759384,
37.2622240218069));
#238953=CARTESIAN_POINT('Ctrl Pts',(2.72396147978784,-7.42973861754103,
37.2544636741493));
#238954=CARTESIAN_POINT('Ctrl Pts',(2.54253563730978,-7.4937494487335,37.2467033264917));
#238955=CARTESIAN_POINT('Ctrl Pts',(2.35931450721544,-7.55099702397258,
37.2389429788341));
#238956=CARTESIAN_POINT('Ctrl Pts',(2.23330909823,-7.5903675055743,37.2336060082567));
#238957=CARTESIAN_POINT('Ctrl Pts',(2.10645482339439,-7.62654028306821,
37.2282690376794));
#238958=CARTESIAN_POINT('Ctrl Pts',(1.97893192261877,-7.65948754458419,
37.222932067102));
#238959=CARTESIAN_POINT('Ctrl Pts',(1.78983049186541,-7.70834444992577,
37.2150179688034));
#238960=CARTESIAN_POINT('Ctrl Pts',(1.59865148808939,-7.75026327553616,
37.2071038705047));
#238961=CARTESIAN_POINT('Ctrl Pts',(1.40594636116218,-7.78506492134361,
37.199189772206));
#238962=CARTESIAN_POINT('Ctrl Pts',(1.21346251425868,-7.81982660501237,
37.191284761532));
#238963=CARTESIAN_POINT('Ctrl Pts',(1.0194563706773,-7.84748732618165,37.183379750858));
#238964=CARTESIAN_POINT('Ctrl Pts',(0.82449426457881,-7.86791778094285,
37.175474740184));
#238965=CARTESIAN_POINT('Ctrl Pts',(0.629719818694653,-7.8883285704286,
37.1675773384552));
#238966=CARTESIAN_POINT('Ctrl Pts',(0.433991583861733,-7.9015229212864,
37.1596799367265));
#238967=CARTESIAN_POINT('Ctrl Pts',(0.237886089320525,-7.90742253888761,
37.1517825349978));
#238968=CARTESIAN_POINT('Ctrl Pts',(0.0419329444939414,-7.91331757321563,
37.1438912685734));
#238969=CARTESIAN_POINT('Ctrl Pts',(-0.154396533022881,-7.91192915444299,
37.136000002149));
#238970=CARTESIAN_POINT('Ctrl Pts',(-0.350520402733202,-7.90323076009221,
37.1281087357247));
#238971=CARTESIAN_POINT('Ctrl Pts',(-0.546528313749996,-7.8945375086873,
37.1202221350299));
#238972=CARTESIAN_POINT('Ctrl Pts',(-0.742330515623083,-7.87854290891249,
37.1123355343352));
#238973=CARTESIAN_POINT('Ctrl Pts',(-0.937344491595128,-7.85527251621968,
37.1044489336404));
#238974=CARTESIAN_POINT('Ctrl Pts',(-1.13227935775763,-7.83201156344688,
37.0965655322419));
#238975=CARTESIAN_POINT('Ctrl Pts',(-1.3264262933321,-7.8014807407568,37.0886821308434));
#238976=CARTESIAN_POINT('Ctrl Pts',(-1.51920704762722,-7.76375752754037,
37.0807987294449));
#238977=CARTESIAN_POINT('Ctrl Pts',(-1.71197237255739,-7.72603733353209,
37.0729159590008));
#238978=CARTESIAN_POINT('Ctrl Pts',(-1.90337139443323,-7.68112595550735,
37.0650331885567));
#238979=CARTESIAN_POINT('Ctrl Pts',(-2.09283469600871,-7.62915224223387,
37.0571504181127));
#238980=CARTESIAN_POINT('Ctrl Pts',(-2.28229847681395,-7.57717839749774,
37.0492676277299));
#238981=CARTESIAN_POINT('Ctrl Pts',(-2.46982619466817,-7.51814227264755,
37.0413848373471));
#238982=CARTESIAN_POINT('Ctrl Pts',(-2.65486217690922,-7.45222301206941,
37.0335020469643));
#238983=CARTESIAN_POINT('Ctrl Pts',(-2.83992974387146,-7.38629249940159,
37.0256179110284));
#238984=CARTESIAN_POINT('Ctrl Pts',(-3.02250440274074,-7.31347662573346,
37.0177337750925));
#238985=CARTESIAN_POINT('Ctrl Pts',(-3.20204886462847,-7.23400332240258,
37.0098496391567));
#238986=CARTESIAN_POINT('Ctrl Pts',(-3.38165416722836,-7.15450308862604,
37.0019628315904));
#238987=CARTESIAN_POINT('Ctrl Pts',(-3.55822691168626,-7.06834106985719,
36.9940760240241));
#238988=CARTESIAN_POINT('Ctrl Pts',(-3.73125266538508,-6.9757920372569,
36.9861892164578));
#238989=CARTESIAN_POINT('Ctrl Pts',(-3.90444749073451,-6.88315257061791,
36.9782947023187));
#238990=CARTESIAN_POINT('Ctrl Pts',(-4.07408809812436,-6.78411378700904,
36.9704001881795));
#238991=CARTESIAN_POINT('Ctrl Pts',(-4.23968649499488,-6.67899539033813,
36.9625056740404));
#238992=CARTESIAN_POINT('Ctrl Pts',(-4.40537750050749,-6.57381820763935,
36.9546067450021));
#238993=CARTESIAN_POINT('Ctrl Pts',(-4.56702150496516,-6.46255482837822,
36.9467078159637));
#238994=CARTESIAN_POINT('Ctrl Pts',(-4.72416186895681,-6.3455666126749,
36.9388088869254));
#238995=CARTESIAN_POINT('Ctrl Pts',(-4.88149411744783,-6.22843554236294,
36.9309003124846));
#238996=CARTESIAN_POINT('Ctrl Pts',(-5.03431147256526,-6.10556588780956,
36.9229917380439));
#238997=CARTESIAN_POINT('Ctrl Pts',(-5.18219174192037,-5.97735809116137,
36.9150831636031));
#238998=CARTESIAN_POINT('Ctrl Pts',(-5.24489373318827,-5.92299732903288,
36.9117298875529));
#238999=CARTESIAN_POINT('Ctrl Pts',(-5.3067085985598,-5.86767731612106,
36.9083766115027));
#239000=CARTESIAN_POINT('Ctrl Pts',(-5.36760627154116,-5.81143045331457,
36.9050233354525));
#239001=CARTESIAN_POINT('Ctrl Pts',(-5.52367396083747,-5.66728179411931,
36.8964296073328));
#239002=CARTESIAN_POINT('Ctrl Pts',(-5.6740275740787,-5.51675480152332,
36.887835879213));
#239003=CARTESIAN_POINT('Ctrl Pts',(-5.81816424798464,-5.36030650088904,
36.8792421510933));
#239004=CARTESIAN_POINT('Ctrl Pts',(-5.96209281342726,-5.20408408458074,
36.8706608308327));
#239005=CARTESIAN_POINT('Ctrl Pts',(-6.0998221849825,-5.04195760390072,
36.8620795105721));
#239006=CARTESIAN_POINT('Ctrl Pts',(-6.23088592796903,-4.87442115052008,
36.8534981903116));
#239007=CARTESIAN_POINT('Ctrl Pts',(-6.36761776080882,-4.69963927861393,
36.8445457552546));
#239008=CARTESIAN_POINT('Ctrl Pts',(-6.49709444095225,-4.51896928210813,
36.8355933201976));
#239009=CARTESIAN_POINT('Ctrl Pts',(-6.61882955468969,-4.33301469256294,
36.8266408851406));
#239010=CARTESIAN_POINT('Ctrl Pts',(-6.73505851645895,-4.15547094026742,
36.8180933740731));
#239011=CARTESIAN_POINT('Ctrl Pts',(-6.84423051064621,-3.97311029123179,
36.8095458630055));
#239012=CARTESIAN_POINT('Ctrl Pts',(-6.94596260802212,-3.78649236734456,
36.800998351938));
#239013=CARTESIAN_POINT('Ctrl Pts',(-7.0475383006116,-3.60016135326535,
36.7924639819702));
#239014=CARTESIAN_POINT('Ctrl Pts',(-7.1416967961109,-3.40958633864797,
36.7839296120024));
#239015=CARTESIAN_POINT('Ctrl Pts',(-7.22809886420539,-3.21535500517016,
36.7753952420347));
#239016=CARTESIAN_POINT('Ctrl Pts',(-7.31431281523246,-3.02154655773731,
36.7668794533426));
#239017=CARTESIAN_POINT('Ctrl Pts',(-7.39280393547199,-2.82409790275373,
36.7583636646506));
#239018=CARTESIAN_POINT('Ctrl Pts',(-7.46327923506166,-2.62362041071063,
36.7498478759585));
#239019=CARTESIAN_POINT('Ctrl Pts',(-7.47370377569695,-2.59396625138911,
36.7485882405149));
#239020=CARTESIAN_POINT('Ctrl Pts',(-7.48395301401652,-2.56424586810514,
36.7473286050713));
#239021=CARTESIAN_POINT('Ctrl Pts',(-7.49402608667908,-2.53446128638286,
36.7460689696277));
#239022=CARTESIAN_POINT('Ctrl Pts',(-7.55402569557346,-2.35705134263631,
36.7385660321927));
#239023=CARTESIAN_POINT('Ctrl Pts',(-7.60773975115643,-2.17745488740816,
36.7310630947577));
#239024=CARTESIAN_POINT('Ctrl Pts',(-7.65500905793486,-1.99618569350029,
36.7235601573226));
#239025=CARTESIAN_POINT('Ctrl Pts',(-7.70229117428998,-1.81486737719569,
36.7160551866559));
#239026=CARTESIAN_POINT('Ctrl Pts',(-7.74312495255439,-1.63187578218918,
36.7085502159892));
#239027=CARTESIAN_POINT('Ctrl Pts',(-7.77740159634273,-1.44773803196767,
36.7010452453225));
#239028=CARTESIAN_POINT('Ctrl Pts',(-7.81168274059985,-1.26357610475252,
36.693539289265));
#239029=CARTESIAN_POINT('Ctrl Pts',(-7.83940497754203,-1.07826809693323,
36.6860333332076));
#239030=CARTESIAN_POINT('Ctrl Pts',(-7.86051110285172,-0.892348699749605,
36.6785273771502));
#239031=CARTESIAN_POINT('Ctrl Pts',(-7.88163270239363,-0.706292993324796,
36.6710159180028));
#239032=CARTESIAN_POINT('Ctrl Pts',(-7.89612847385921,-0.519625379766348,
36.6635044588554));
#239033=CARTESIAN_POINT('Ctrl Pts',(-7.90399327063924,-0.332883429580984,
36.655992999708));
#239034=CARTESIAN_POINT('Ctrl Pts',(-7.90876131246361,-0.219670913892321,
36.6514391692177));
#239035=CARTESIAN_POINT('Ctrl Pts',(-7.911093217297,-0.106431084262574,
36.6468853387274));
#239036=CARTESIAN_POINT('Ctrl Pts',(-7.91099714850641,0.00671686857199988,
36.6423315082371));
#239037=CARTESIAN_POINT('',(-7.91099848652071,-0.00489349231630381,32.6423315082371));
#239038=CARTESIAN_POINT('Ctrl Pts',(-7.91099706278514,0.00681708184264343,
36.6450777990978));
#239039=CARTESIAN_POINT('Ctrl Pts',(-7.91070528407644,0.345416582456211,
36.6327147129114));
#239040=CARTESIAN_POINT('Ctrl Pts',(-7.88867503774943,0.68363518933523,
36.6202189618414));
#239041=CARTESIAN_POINT('Ctrl Pts',(-7.8393101641919,1.06354126535353,36.6051583824506));
#239042=CARTESIAN_POINT('Ctrl Pts',(-7.83319959704548,1.10764969224287,
36.6033937543779));
#239043=CARTESIAN_POINT('Ctrl Pts',(-7.82516509291598,1.16225036545417,
36.6011870502451));
#239044=CARTESIAN_POINT('Ctrl Pts',(-7.82359181834253,1.17279397243764,
36.6007598934203));
#239045=CARTESIAN_POINT('Ctrl Pts',(-7.82099482329918,1.18996045492925,
36.6000626940279));
#239046=CARTESIAN_POINT('Ctrl Pts',(-7.81998398707249,1.19658528818443,
36.5997932137383));
#239047=CARTESIAN_POINT('Ctrl Pts',(-7.81819033045375,1.2082412349205,36.5993183313836));
#239048=CARTESIAN_POINT('Ctrl Pts',(-7.81741106757056,1.21327289816011,
36.5991130871169));
#239049=CARTESIAN_POINT('Ctrl Pts',(-7.81582923860537,1.22342189954141,
36.598698601407));
#239050=CARTESIAN_POINT('Ctrl Pts',(-7.81502650307395,1.22853920872915,
36.5984893524356));
#239051=CARTESIAN_POINT('Ctrl Pts',(-7.81346128021241,1.23845363919506,
36.5980834414047));
#239052=CARTESIAN_POINT('Ctrl Pts',(-7.8126993992683,1.24325085575843,36.5978868069372));
#239053=CARTESIAN_POINT('Ctrl Pts',(-7.81087524324058,1.2546688398177,36.5974182393464));
#239054=CARTESIAN_POINT('Ctrl Pts',(-7.80980896897679,1.26128895607668,
36.5971461226603));
#239055=CARTESIAN_POINT('Ctrl Pts',(-7.80657916940378,1.28118050400872,
36.5963271396894));
#239056=CARTESIAN_POINT('Ctrl Pts',(-7.80439023056759,1.29444773456824,
36.5957790884124));
#239057=CARTESIAN_POINT('Ctrl Pts',(-7.77729701338445,1.45609361835273,
36.5890790050618));
#239058=CARTESIAN_POINT('Ctrl Pts',(-7.74820146872424,1.60372137993247,
36.5827132490778));
#239059=CARTESIAN_POINT('Ctrl Pts',(-7.67739188676139,1.91581287388975,
36.5688300730985));
#239060=CARTESIAN_POINT('Ctrl Pts',(-7.63455793024819,2.07995331249798,
36.5612754489659));
#239061=CARTESIAN_POINT('Ctrl Pts',(-7.56721709163401,2.30776211892767,
36.5505357530121));
#239062=CARTESIAN_POINT('Ctrl Pts',(-7.54711106335815,2.37268938563442,
36.5474452977945));
#239063=CARTESIAN_POINT('Ctrl Pts',(-7.5062612801121,2.49882744872548,36.5413918441512));
#239064=CARTESIAN_POINT('Ctrl Pts',(-7.48559901490657,2.56005943389883,
36.5384302709666));
#239065=CARTESIAN_POINT('Ctrl Pts',(-7.42557493208854,2.73099640628764,
36.5301077137671));
#239066=CARTESIAN_POINT('Ctrl Pts',(-7.38453563148447,2.84009467163069,
36.5247320885914));
#239067=CARTESIAN_POINT('Ctrl Pts',(-7.25264348142139,3.16850473520379,
36.5084111899047));
#239068=CARTESIAN_POINT('Ctrl Pts',(-7.15431598157754,3.38467532582889,
36.4974800345152));
#239069=CARTESIAN_POINT('Ctrl Pts',(-6.87964711060265,3.92287798540189,
36.4700808805751));
#239070=CARTESIAN_POINT('Ctrl Pts',(-6.69033849445937,4.23767954039783,
36.4538959396896));
#239071=CARTESIAN_POINT('Ctrl Pts',(-6.39792012662386,4.65520511985469,
36.4324424525915));
#239072=CARTESIAN_POINT('Ctrl Pts',(-6.31283878358843,4.76994610465057,
36.4265445986849));
#239073=CARTESIAN_POINT('Ctrl Pts',(-6.21309531438781,4.89711352397218,
36.4200011498997));
#239074=CARTESIAN_POINT('Ctrl Pts',(-6.20144313842409,4.9118608754035,36.4192422007314));
#239075=CARTESIAN_POINT('Ctrl Pts',(-6.18386521261576,4.93394578195421,
36.4181054288256));
#239076=CARTESIAN_POINT('Ctrl Pts',(-6.17797875491938,4.94131444573236,
36.417726108244));
#239077=CARTESIAN_POINT('Ctrl Pts',(-6.16783426400353,4.95396684888715,
36.4170747292975));
#239078=CARTESIAN_POINT('Ctrl Pts',(-6.16358259018361,4.95925566011073,
36.4168024279444));
#239079=CARTESIAN_POINT('Ctrl Pts',(-6.1548146619227,4.97013371181017,36.4162423150181));
#239080=CARTESIAN_POINT('Ctrl Pts',(-6.15029758631067,4.97572228284742,
36.4159545354244));
#239081=CARTESIAN_POINT('Ctrl Pts',(-6.1394086947008,4.98915664571703,36.4152626836935));
#239082=CARTESIAN_POINT('Ctrl Pts',(-6.13302943749608,4.99699640542645,
36.4148588983926));
#239083=CARTESIAN_POINT('Ctrl Pts',(-6.11342090119484,5.02100011653531,
36.413622432649));
#239084=CARTESIAN_POINT('Ctrl Pts',(-6.10014256949035,5.03712397360805,
36.4127916476173));
#239085=CARTESIAN_POINT('Ctrl Pts',(-5.94818684316513,5.22016147029716,
36.4033576641535));
#239086=CARTESIAN_POINT('Ctrl Pts',(-5.80275700278186,5.38135967587272,
36.3950247822911));
#239087=CARTESIAN_POINT('Ctrl Pts',(-5.14588127976912,6.05181976761474,
36.3599861980014));
#239088=CARTESIAN_POINT('Ctrl Pts',(-4.57277788374726,6.49571303085079,
36.3360812566952));
#239089=CARTESIAN_POINT('Ctrl Pts',(-3.73086370745845,6.98047578459952,
36.3019010940387));
#239090=CARTESIAN_POINT('Ctrl Pts',(-3.50849286935078,7.09484685526336,
36.2929146763334));
#239091=CARTESIAN_POINT('Ctrl Pts',(-3.2003601929441,7.23529459093938,36.2801137688988));
#239092=CARTESIAN_POINT('Ctrl Pts',(-3.11901344209155,7.27073230674187,
36.2767019812494));
#239093=CARTESIAN_POINT('Ctrl Pts',(-2.98953510491732,7.32456503420561,
36.2712015553313));
#239094=CARTESIAN_POINT('Ctrl Pts',(-2.94179175885726,7.34387051648252,
36.2691594814894));
#239095=CARTESIAN_POINT('Ctrl Pts',(-2.88252742754584,7.36716397294914,
36.2666104156077));
#239096=CARTESIAN_POINT('Ctrl Pts',(-2.87118049793392,7.37159358083965,
36.2661217223737));
#239097=CARTESIAN_POINT('Ctrl Pts',(-2.8543899213502,7.37810362748676,36.2653976770858));
#239098=CARTESIAN_POINT('Ctrl Pts',(-2.84895410211927,7.38020429831263,
36.2651631332968));
#239099=CARTESIAN_POINT('Ctrl Pts',(-2.8383888159033,7.38427383821025,36.2647069990688));
#239100=CARTESIAN_POINT('Ctrl Pts',(-2.83325960788966,7.38624337414168,
36.2644854349616));
#239101=CARTESIAN_POINT('Ctrl Pts',(-2.8226585010605,7.39030136664032,36.264027258876));
#239102=CARTESIAN_POINT('Ctrl Pts',(-2.8171863278237,7.39238909267262,36.2637906188887));
#239103=CARTESIAN_POINT('Ctrl Pts',(-2.80237120210787,7.39802247280592,
36.2631495946696));
#239104=CARTESIAN_POINT('Ctrl Pts',(-2.79302385720518,7.40155649809921,
36.2627447695621));
#239105=CARTESIAN_POINT('Ctrl Pts',(-2.75822707562884,7.41463709231251,
36.2612363913187));
#239106=CARTESIAN_POINT('Ctrl Pts',(-2.73273533494119,7.42407013571564,
36.2601286659647));
#239107=CARTESIAN_POINT('Ctrl Pts',(-2.56275942017937,7.4859744892282,36.2527266183532));
#239108=CARTESIAN_POINT('Ctrl Pts',(-2.4168244902327,7.53435508431277,36.2462962288376));
#239109=CARTESIAN_POINT('Ctrl Pts',(-2.2501326870075,7.58427556946827,36.2389246507686));
#239110=CARTESIAN_POINT('Ctrl Pts',(-2.23066531977546,7.59002406117988,
36.2380633286273));
#239111=CARTESIAN_POINT('Ctrl Pts',(-1.94716049245495,7.67255487476962,
36.2255152194321));
#239112=CARTESIAN_POINT('Ctrl Pts',(-1.67932009705048,7.73559391449341,
36.2136125196681));
#239113=CARTESIAN_POINT('Ctrl Pts',(-0.674306896117623,7.91746777695069,
36.1694908955377));
#239114=CARTESIAN_POINT('Ctrl Pts',(0.0752945901321078,7.94578121850872,
36.1381661598143));
#239115=CARTESIAN_POINT('Ctrl Pts',(0.975269774363557,7.85225137429399,
36.1012586174437));
#239116=CARTESIAN_POINT('Ctrl Pts',(1.13226772742942,7.8311540247008,36.0948222850803));
#239117=CARTESIAN_POINT('Ctrl Pts',(1.32016409661107,7.8001356336022,36.0871263490344));
#239118=CARTESIAN_POINT('Ctrl Pts',(1.35176862144557,7.79472069715811,36.0858320936758));
#239119=CARTESIAN_POINT('Ctrl Pts',(1.41261387819294,7.78391463573031,36.0833407779462));
#239120=CARTESIAN_POINT('Ctrl Pts',(1.44185885594751,7.77855051223805,36.0821435149027));
#239121=CARTESIAN_POINT('Ctrl Pts',(1.49247569249424,7.76897108963063,36.0800715763413));
#239122=CARTESIAN_POINT('Ctrl Pts',(1.51386164165528,7.76483215638587,36.0791962517859));
#239123=CARTESIAN_POINT('Ctrl Pts',(1.56167570972921,7.75537340872317,36.0772393869506));
#239124=CARTESIAN_POINT('Ctrl Pts',(1.58809429921554,7.75000672471615,36.0761582748788));
#239125=CARTESIAN_POINT('Ctrl Pts',(1.65850041301441,7.73532927117364,36.0732773020853));
#239126=CARTESIAN_POINT('Ctrl Pts',(1.70243694458549,7.72577834448097,36.0714796743983));
#239127=CARTESIAN_POINT('Ctrl Pts',(1.899000171306,7.68129119029673,36.0634376442952));
#239128=CARTESIAN_POINT('Ctrl Pts',(2.05065227578138,7.64220271131309,36.0572342714464));
#239129=CARTESIAN_POINT('Ctrl Pts',(2.56530279672973,7.49312740778367,36.0361407028324));
#239130=CARTESIAN_POINT('Ctrl Pts',(2.92150369899722,7.36155956161799,36.0214892748173));
#239131=CARTESIAN_POINT('Ctrl Pts',(3.44337623176874,7.12493015787836,35.9993411171139));
#239132=CARTESIAN_POINT('Ctrl Pts',(3.61685585972647,7.03845311696228,35.9918522997115));
#239133=CARTESIAN_POINT('Ctrl Pts',(3.906508794791,6.88052637567865,35.9789929104648));
#239134=CARTESIAN_POINT('Ctrl Pts',(4.02433036437457,6.81228437072018,35.9736566171887));
#239135=CARTESIAN_POINT('Ctrl Pts',(4.20271328177182,6.7027219634552,35.9653632212593));
#239136=CARTESIAN_POINT('Ctrl Pts',(4.26456040402482,6.66354297607204,35.9624468443415));
#239137=CARTESIAN_POINT('Ctrl Pts',(4.34186872616721,6.61305245898055,35.9587424974102));
#239138=CARTESIAN_POINT('Ctrl Pts',(4.35784524034377,6.60253524922748,35.9579737402198));
#239139=CARTESIAN_POINT('Ctrl Pts',(4.3818320997843,6.5866199032509,35.9568145392717));
#239140=CARTESIAN_POINT('Ctrl Pts',(4.389870993509,6.58126484502446,35.9564251979859));
#239141=CARTESIAN_POINT('Ctrl Pts',(4.40605915405835,6.5704383474748,35.9556394289025));
#239142=CARTESIAN_POINT('Ctrl Pts',(4.41420808517499,6.56496643762655,35.9552429891663));
#239143=CARTESIAN_POINT('Ctrl Pts',(4.43090275727621,6.55371102765095,35.9544289441032));
#239144=CARTESIAN_POINT('Ctrl Pts',(4.43944740730779,6.54792594608191,35.954011296441));
#239145=CARTESIAN_POINT('Ctrl Pts',(4.46354320839489,6.53154324601246,35.9528306526604));
#239146=CARTESIAN_POINT('Ctrl Pts',(4.47906777983703,6.52090691279368,35.9520665571161));
#239147=CARTESIAN_POINT('Ctrl Pts',(4.55966056972187,6.46526686856762,35.9480820921412));
#239148=CARTESIAN_POINT('Ctrl Pts',(4.62408819050632,6.41934484934875,35.9448365230807));
#239149=CARTESIAN_POINT('Ctrl Pts',(5.18428084240982,6.00724689531925,35.9161265688413));
#239150=CARTESIAN_POINT('Ctrl Pts',(5.63637242781823,5.58525948795938,35.8897185944934));
#239151=CARTESIAN_POINT('Ctrl Pts',(6.17641289500448,4.94810567346979,35.855077630033));
#239152=CARTESIAN_POINT('Ctrl Pts',(6.31094296593637,4.77533545081489,35.8461002761938));
#239153=CARTESIAN_POINT('Ctrl Pts',(6.4622622475926,4.56342097878544,35.8355491808253));
#239154=CARTESIAN_POINT('Ctrl Pts',(6.4861202828166,4.52944677518939,35.8338710112579));
#239155=CARTESIAN_POINT('Ctrl Pts',(6.52345037012987,4.47538836240697,35.8312214288481));
#239156=CARTESIAN_POINT('Ctrl Pts',(6.53709958358123,4.45542756257335,35.8302474870463));
#239157=CARTESIAN_POINT('Ctrl Pts',(6.56181905548895,4.41891932849473,35.8284740468403));
#239158=CARTESIAN_POINT('Ctrl Pts',(6.57291876927047,4.40239210022035,35.8276741390254));
#239159=CARTESIAN_POINT('Ctrl Pts',(6.5968268705265,4.3665014857691,35.8259433001152));
#239160=CARTESIAN_POINT('Ctrl Pts',(6.60961265409561,4.34712325015933,35.8250126878944));
#239161=CARTESIAN_POINT('Ctrl Pts',(6.64432298040021,4.29400884067751,35.8224724342672));
#239162=CARTESIAN_POINT('Ctrl Pts',(6.66607579817694,4.26016117844394,35.8208651307021));
#239163=CARTESIAN_POINT('Ctrl Pts',(6.78169813048691,4.07719735040688,35.812236493039));
#239164=CARTESIAN_POINT('Ctrl Pts',(6.87082502759339,3.92514109825721,35.8052782890374));
#239165=CARTESIAN_POINT('Ctrl Pts',(6.96672573649211,3.74823686309907,35.7973769699102));
#239166=CARTESIAN_POINT('Ctrl Pts',(6.97854604194942,3.72618333053912,35.7963952999387));
#239167=CARTESIAN_POINT('Ctrl Pts',(6.99169551014139,3.70136789216168,35.7952942750104));
#239168=CARTESIAN_POINT('Ctrl Pts',(6.99312791429543,3.69866088658637,35.7951742168448));
#239169=CARTESIAN_POINT('Ctrl Pts',(6.99607776725517,3.69307831571942,35.794926722603));
#239170=CARTESIAN_POINT('Ctrl Pts',(6.99759501600783,3.69020264531196,35.7947992878969));
#239171=CARTESIAN_POINT('Ctrl Pts',(7.00325608427099,3.67945706929135,35.7943232986429));
#239172=CARTESIAN_POINT('Ctrl Pts',(7.00738840503139,3.67158111006522,35.79397482051));
#239173=CARTESIAN_POINT('Ctrl Pts',(7.35164865905182,3.01274318125731,35.764856695746));
#239174=CARTESIAN_POINT('Ctrl Pts',(7.59949128928855,2.31757308743826,35.7371318304023));
#239175=CARTESIAN_POINT('Ctrl Pts',(7.83832611160117,1.15974337726697,35.6929232434117));
#239176=CARTESIAN_POINT('Ctrl Pts',(7.89138348015633,0.714408154638406,
35.6762316585544));
#239177=CARTESIAN_POINT('Ctrl Pts',(7.90742710246973,0.239341158786664,
35.6573115373116));
#239178=CARTESIAN_POINT('Ctrl Pts',(7.90821631719195,0.211665376319118,
35.6562051248054));
#239179=CARTESIAN_POINT('Ctrl Pts',(7.90910095356235,0.17363825722812,35.6546785923203));
#239180=CARTESIAN_POINT('Ctrl Pts',(7.90932137131331,0.163289871669249,
35.6542625337007));
#239181=CARTESIAN_POINT('Ctrl Pts',(7.90964343604327,0.146633932053922,
35.653591814127));
#239182=CARTESIAN_POINT('Ctrl Pts',(7.90975784931207,0.140326620285303,
35.6533375787019));
#239183=CARTESIAN_POINT('Ctrl Pts',(7.9099799510671,0.127218088190425,35.6528086788881));
#239184=CARTESIAN_POINT('Ctrl Pts',(7.91008641224594,0.120416853968545,
35.6525339732033));
#239185=CARTESIAN_POINT('Ctrl Pts',(7.91031128864618,0.104760419078613,
35.6519009170061));
#239186=CARTESIAN_POINT('Ctrl Pts',(7.91042360625605,0.095905148632572,
35.6515423571482));
#239187=CARTESIAN_POINT('Ctrl Pts',(7.91073366554095,0.0677289495780813,
35.6503998266645));
#239188=CARTESIAN_POINT('Ctrl Pts',(7.91087549124689,0.0484075584678235,
35.6496138939339));
#239189=CARTESIAN_POINT('Ctrl Pts',(7.91160936912533,-0.151196350409517,
35.6414677988726));
#239190=CARTESIAN_POINT('Ctrl Pts',(7.90611006295592,-0.331417862464458,
35.6338584674401));
#239191=CARTESIAN_POINT('Ctrl Pts',(7.84630317469573,-1.25483571835492,
35.5935749927134));
#239192=CARTESIAN_POINT('Ctrl Pts',(7.69335173637718,-1.98785632586977,
35.5580675828169));
#239193=CARTESIAN_POINT('Ctrl Pts',(7.35805813766003,-2.91567333815961,
35.5145506942186));
#239194=CARTESIAN_POINT('Ctrl Pts',(7.26568348756958,-3.13879380260562,
35.50416552714));
#239195=CARTESIAN_POINT('Ctrl Pts',(7.11749019147832,-3.45497880394309,
35.489617319248));
#239196=CARTESIAN_POINT('Ctrl Pts',(7.06974234676012,-3.55166010471907,
35.4851916942741));
#239197=CARTESIAN_POINT('Ctrl Pts',(7.01216272956621,-3.66248360727265,
35.480143991968));
#239198=CARTESIAN_POINT('Ctrl Pts',(7.00424452537631,-3.67760396901163,
35.479455848788));
#239199=CARTESIAN_POINT('Ctrl Pts',(6.99213954654262,-3.70053835876744,
35.4784128970207));
#239200=CARTESIAN_POINT('Ctrl Pts',(6.98798849329457,-3.70837112507276,
35.4780568434847));
#239201=CARTESIAN_POINT('Ctrl Pts',(6.98044705879823,-3.72254369302833,
35.4774128617745));
#239202=CARTESIAN_POINT('Ctrl Pts',(6.97706118731049,-3.72888587597723,
35.4771247762576));
#239203=CARTESIAN_POINT('Ctrl Pts',(6.97028074790042,-3.7415449645188,35.4765499401766));
#239204=CARTESIAN_POINT('Ctrl Pts',(6.96688622689929,-3.74786188751085,
35.4762631883492));
#239205=CARTESIAN_POINT('Ctrl Pts',(6.95732777245099,-3.76559152195833,
35.4754586240659));
#239206=CARTESIAN_POINT('Ctrl Pts',(6.95114434046665,-3.77699372565035,
35.47494149789));
#239207=CARTESIAN_POINT('Ctrl Pts',(6.92574442066891,-3.82355735052294,
35.4728308975617));
#239208=CARTESIAN_POINT('Ctrl Pts',(6.90628881316048,-3.85858801661332,
35.4712458812878));
#239209=CARTESIAN_POINT('Ctrl Pts',(6.58648689813112,-4.42423709558592,
35.4456945362196));
#239210=CARTESIAN_POINT('Ctrl Pts',(6.22605544251963,-4.91853791413004,
35.424191484825));
#239211=CARTESIAN_POINT('Ctrl Pts',(5.54496019890987,-5.65621281444071,
35.3898913364315));
#239212=CARTESIAN_POINT('Ctrl Pts',(5.25627045360818,-5.92544755955108,
35.3766914946964));
#239213=CARTESIAN_POINT('Ctrl Pts',(4.82439392239379,-6.2717255844288,35.3571269544986));
#239214=CARTESIAN_POINT('Ctrl Pts',(4.69707942914819,-6.36763375925413,
35.351375686854));
#239215=CARTESIAN_POINT('Ctrl Pts',(4.48115496048411,-6.52029247833874,
35.3415069429887));
#239216=CARTESIAN_POINT('Ctrl Pts',(4.39415213054745,-6.57923926471133,
35.3375010048448));
#239217=CARTESIAN_POINT('Ctrl Pts',(4.26270862701209,-6.66452547611605,
35.3313681142168));
#239218=CARTESIAN_POINT('Ctrl Pts',(4.21914015245588,-6.69219252665309,
35.3293223994837));
#239219=CARTESIAN_POINT('Ctrl Pts',(4.16769075057763,-6.72416204219813,
35.3268881070584));
#239220=CARTESIAN_POINT('Ctrl Pts',(4.16006849619777,-6.72888040225786,
35.3265269918238));
#239221=CARTESIAN_POINT('Ctrl Pts',(4.14840051546367,-6.73607576165551,
35.3259734572116));
#239222=CARTESIAN_POINT('Ctrl Pts',(4.14436053258067,-6.73856210769509,
35.325781661779));
#239223=CARTESIAN_POINT('Ctrl Pts',(4.13732260994436,-6.74288476699529,
35.3254472992998));
#239224=CARTESIAN_POINT('Ctrl Pts',(4.13432567424517,-6.74472272068568,
35.3253048425462));
#239225=CARTESIAN_POINT('Ctrl Pts',(4.12806855145587,-6.74855433689502,
35.3250072545488));
#239226=CARTESIAN_POINT('Ctrl Pts',(4.12480814373666,-6.75054763562258,
35.3248520988065));
#239227=CARTESIAN_POINT('Ctrl Pts',(4.11681640767235,-6.75542555077468,
35.3244715632216));
#239228=CARTESIAN_POINT('Ctrl Pts',(4.11208349665493,-6.75830755609491,
35.32424600627));
#239229=CARTESIAN_POINT('Ctrl Pts',(4.09363584923845,-6.76951430529142,
35.3233660747703));
#239230=CARTESIAN_POINT('Ctrl Pts',(4.07989911165069,-6.7778021230506,35.3227091690026));
#239231=CARTESIAN_POINT('Ctrl Pts',(3.85069589391009,-6.91513857648727,
35.3117215202549));
#239232=CARTESIAN_POINT('Ctrl Pts',(3.62924570567944,-7.03388618953717,
35.3007156549931));
#239233=CARTESIAN_POINT('Ctrl Pts',(2.86975921874841,-7.39572128763022,
35.2627369797264));
#239234=CARTESIAN_POINT('Ctrl Pts',(2.31023670295025,-7.58914336350543,
35.2345505280346));
#239235=CARTESIAN_POINT('Ctrl Pts',(1.43371657745948,-7.78609867108479,
35.1940773289123));
#239236=CARTESIAN_POINT('Ctrl Pts',(1.12935733332025,-7.83603576734698,
35.1806263670723));
#239237=CARTESIAN_POINT('Ctrl Pts',(0.71295788331513,-7.87958229016834,
35.1631645077018));
#239238=CARTESIAN_POINT('Ctrl Pts',(0.602849329554254,-7.88877050614783,
35.1586335269741));
#239239=CARTESIAN_POINT('Ctrl Pts',(0.476506946563828,-7.89665255111096,
35.1535312231086));
#239240=CARTESIAN_POINT('Ctrl Pts',(0.460429731994517,-7.89760627337691,
35.1528837340511));
#239241=CARTESIAN_POINT('Ctrl Pts',(0.43613530425295,-7.89897301460196,
35.1519079858912));
#239242=CARTESIAN_POINT('Ctrl Pts',(0.427920225573886,-7.89942231876122,
35.1515785024877));
#239243=CARTESIAN_POINT('Ctrl Pts',(0.413734661019399,-7.90017597077229,
35.1510103554901));
#239244=CARTESIAN_POINT('Ctrl Pts',(0.407764512162655,-7.90048636741614,
35.1507714879162));
#239245=CARTESIAN_POINT('Ctrl Pts',(0.395416977482603,-7.90111430024951,
35.1502779606968));
#239246=CARTESIAN_POINT('Ctrl Pts',(0.389039546091621,-7.90143088329806,
35.1500233333827));
#239247=CARTESIAN_POINT('Ctrl Pts',(0.371748224690901,-7.90226825926077,
35.1493337023921));
#239248=CARTESIAN_POINT('Ctrl Pts',(0.36083360822879,-7.90277416432851,
35.1488992014654));
#239249=CARTESIAN_POINT('Ctrl Pts',(0.320132635023746,-7.90457620622215,
35.1472819259567));
#239250=CARTESIAN_POINT('Ctrl Pts',(0.290339890298518,-7.90572657498813,
35.1461040724566));
#239251=CARTESIAN_POINT('Ctrl Pts',(-0.183792432772987,-7.92135013940513,
35.1274526735648));
#239252=CARTESIAN_POINT('Ctrl Pts',(-0.62859310451462,-7.89851235134479,
35.1113297268909));
#239253=CARTESIAN_POINT('Ctrl Pts',(-1.53153963099389,-7.77535110596137,
35.0797562554624));
#239254=CARTESIAN_POINT('Ctrl Pts',(-1.98741790875059,-7.67149589729444,
35.0644355819677));
#239255=CARTESIAN_POINT('Ctrl Pts',(-2.66568863962111,-7.45242264858109,
35.0397943035602));
#239256=CARTESIAN_POINT('Ctrl Pts',(-2.896230849264,-7.36588976150276,35.0310584726172));
#239257=CARTESIAN_POINT('Ctrl Pts',(-3.19666779003233,-7.23683483120016,
35.0187311737756));
#239258=CARTESIAN_POINT('Ctrl Pts',(-3.27048979546408,-7.20377394393731,
35.015623727536));
#239259=CARTESIAN_POINT('Ctrl Pts',(-3.3808162050088,-7.15231934167255,
35.010841528461));
#239260=CARTESIAN_POINT('Ctrl Pts',(-3.41770783065832,-7.13476441387362,
35.0092188377385));
#239261=CARTESIAN_POINT('Ctrl Pts',(-3.46163540585171,-7.11344255007217,
35.0072563825009));
#239262=CARTESIAN_POINT('Ctrl Pts',(-3.46880436200363,-7.10994942973714,
35.0069351417212));
#239263=CARTESIAN_POINT('Ctrl Pts',(-3.47988827015735,-7.10452796972739,
35.0064369522124));
#239264=CARTESIAN_POINT('Ctrl Pts',(-3.48380693615512,-7.10260721683944,
35.0062605247722));
#239265=CARTESIAN_POINT('Ctrl Pts',(-3.49071452737688,-7.09921433605655,
35.0059490113607));
#239266=CARTESIAN_POINT('Ctrl Pts',(-3.49370412388529,-7.09774355662329,
35.0058140176421));
#239267=CARTESIAN_POINT('Ctrl Pts',(-3.5000311779489,-7.09462589600445,
35.0055279618301));
#239268=CARTESIAN_POINT('Ctrl Pts',(-3.50336840323916,-7.09297854797006,
35.0053768679942));
#239269=CARTESIAN_POINT('Ctrl Pts',(-3.51280987839659,-7.08830968212789,
35.004948802898));
#239270=CARTESIAN_POINT('Ctrl Pts',(-3.51891137666305,-7.08528264179443,
35.0046714584796));
#239271=CARTESIAN_POINT('Ctrl Pts',(-3.54437500734256,-7.07260876633628,
35.003511064577));
#239272=CARTESIAN_POINT('Ctrl Pts',(-3.56370126849847,-7.06289049927954,
35.002623245603));
#239273=CARTESIAN_POINT('Ctrl Pts',(-3.88852100881482,-6.89788133903762,
34.9875847775401));
#239274=CARTESIAN_POINT('Ctrl Pts',(-4.18361746525914,-6.72299483106897,
34.9721887483753));
#239275=CARTESIAN_POINT('Ctrl Pts',(-5.03521647966954,-6.14047506005405,
34.9244906823409));
#239276=CARTESIAN_POINT('Ctrl Pts',(-5.55084173935188,-5.67866308281204,
34.8913218951509));
#239277=CARTESIAN_POINT('Ctrl Pts',(-6.20353054142754,-4.91910317391241,
34.847114686122));
#239278=CARTESIAN_POINT('Ctrl Pts',(-6.39279887307541,-4.67049468715187,
34.8338783030197));
#239279=CARTESIAN_POINT('Ctrl Pts',(-6.57808754008093,-4.39466588035967,
34.8204355997297));
#239280=CARTESIAN_POINT('Ctrl Pts',(-6.58921667738758,-4.37796156577782,
34.81962606533));
#239281=CARTESIAN_POINT('Ctrl Pts',(-6.60537072762976,-4.35351395425731,
34.8184478692966));
#239282=CARTESIAN_POINT('Ctrl Pts',(-6.6104458093076,-4.34580399952919,
34.8180772592681));
#239283=CARTESIAN_POINT('Ctrl Pts',(-6.61933032260097,-4.33225526518893,
34.8174276507688));
#239284=CARTESIAN_POINT('Ctrl Pts',(-6.62314554631107,-4.326420307271,34.8171484283016));
#239285=CARTESIAN_POINT('Ctrl Pts',(-6.63053911450104,-4.31507997197211,
34.8166068014018));
#239286=CARTESIAN_POINT('Ctrl Pts',(-6.63411832660669,-4.30957516958262,
34.8163443636169));
#239287=CARTESIAN_POINT('Ctrl Pts',(-6.64264709592539,-4.29642218032096,
34.815718440098));
#239288=CARTESIAN_POINT('Ctrl Pts',(-6.64759030920783,-4.28876987891027,
34.8153551985196));
#239289=CARTESIAN_POINT('Ctrl Pts',(-6.66249373418397,-4.26561108142173,
34.8142586447625));
#239290=CARTESIAN_POINT('Ctrl Pts',(-6.67241302042754,-4.2500782518517,
34.8135269006031));
#239291=CARTESIAN_POINT('Ctrl Pts',(-6.7730894822763,-4.09120556713317,
34.8060801099556));
#239292=CARTESIAN_POINT('Ctrl Pts',(-6.85927046892438,-3.94501166973401,
34.7995407344318));
#239293=CARTESIAN_POINT('Ctrl Pts',(-7.02716418806364,-3.63804363252641,
34.7863751107902));
#239294=CARTESIAN_POINT('Ctrl Pts',(-7.10821555084118,-3.47702080470081,
34.779772836855));
#239295=CARTESIAN_POINT('Ctrl Pts',(-7.45230308949078,-2.73100539348885,
34.7502718727135));
#239296=CARTESIAN_POINT('Ctrl Pts',(-7.64907637125781,-2.11819648010552,
34.7292064240524));
#239297=CARTESIAN_POINT('Ctrl Pts',(-7.81330498254887,-1.26089029544188,
34.6976758137546));
#239298=CARTESIAN_POINT('Ctrl Pts',(-7.84687314368932,-1.03158298422918,
34.6890136934493));
#239299=CARTESIAN_POINT('Ctrl Pts',(-7.87413990191499,-0.763712073946177,
34.6783598892406));
#239300=CARTESIAN_POINT('Ctrl Pts',(-7.87768143455745,-0.72627162633861,
34.6768601797615));
#239301=CARTESIAN_POINT('Ctrl Pts',(-7.8818854217051,-0.67817194338873,
34.6749208881759));
#239302=CARTESIAN_POINT('Ctrl Pts',(-7.88279347792796,-0.66753424522885,
34.6744912039117));
#239303=CARTESIAN_POINT('Ctrl Pts',(-7.8842200882024,-0.650412874666579,
34.6737983821548));
#239304=CARTESIAN_POINT('Ctrl Pts',(-7.88475218675746,-0.643930322195523,
34.6735357764512));
#239305=CARTESIAN_POINT('Ctrl Pts',(-7.88574915055482,-0.63159779361437,
34.6730356519341));
#239306=CARTESIAN_POINT('Ctrl Pts',(-7.8862155026584,-0.625747939483491,
34.6727981907134));
#239307=CARTESIAN_POINT('Ctrl Pts',(-7.8872621224248,-0.612432271626754,
34.6722571543863));
#239308=CARTESIAN_POINT('Ctrl Pts',(-7.88783829920551,-0.604966148034549,
34.6719534237771));
#239309=CARTESIAN_POINT('Ctrl Pts',(-7.88951901594675,-0.582776709622307,
34.6710496490344));
#239310=CARTESIAN_POINT('Ctrl Pts',(-7.89059293587748,-0.568051153424212,
34.670448461855));
#239311=CARTESIAN_POINT('Ctrl Pts',(-7.89775524617057,-0.465900514353901,
34.6662685496937));
#239312=CARTESIAN_POINT('Ctrl Pts',(-7.90243164160236,-0.378384321028612,
34.6626392711476));
#239313=CARTESIAN_POINT('Ctrl Pts',(-7.90918039501917,-0.19492018992749,
34.6549496850105));
#239314=CARTESIAN_POINT('Ctrl Pts',(-7.91096274880416,-0.0989752959457913,
34.6508818064442));
#239315=CARTESIAN_POINT('Ctrl Pts',(-7.91107275700221,0.188848524910494,
34.6385730740983));
#239316=CARTESIAN_POINT('Ctrl Pts',(-7.90416559975877,0.380656400235834,
34.6302310135188));
#239317=CARTESIAN_POINT('Ctrl Pts',(-7.8685506472537,0.871920452914543,
34.6087034270501));
#239318=CARTESIAN_POINT('Ctrl Pts',(-7.82972775036714,1.17034252646841,
34.5954787338032));
#239319=CARTESIAN_POINT('Ctrl Pts',(-7.74820065132595,1.60272043721625,
34.5763743909714));
#239320=CARTESIAN_POINT('Ctrl Pts',(-7.71877779695645,1.73890671062302,
34.5703635255649));
#239321=CARTESIAN_POINT('Ctrl Pts',(-7.60083664326615,2.22255112026571,
34.5490690659233));
#239322=CARTESIAN_POINT('Ctrl Pts',(-7.49231808227196,2.56469210752963,
34.534123361522));
#239323=CARTESIAN_POINT('Ctrl Pts',(-7.34633320136737,2.93545624937585,
34.5179843385539));
#239324=CARTESIAN_POINT('Ctrl Pts',(-7.33142549257565,2.97249309148422,
34.5163724530777));
#239325=CARTESIAN_POINT('Ctrl Pts',(-7.31022006699589,3.02404593784191,
34.5141291068849));
#239326=CARTESIAN_POINT('Ctrl Pts',(-7.30415823708213,3.03865820912228,
34.5134932865611));
#239327=CARTESIAN_POINT('Ctrl Pts',(-7.29302207540162,3.06527647961835,
34.5123351295118));
#239328=CARTESIAN_POINT('Ctrl Pts',(-7.287961828526,3.0772882991266,34.5118125258578));
#239329=CARTESIAN_POINT('Ctrl Pts',(-7.27770391914602,3.10147091021826,
34.5107604621578));
#239330=CARTESIAN_POINT('Ctrl Pts',(-7.27250535570819,3.11364127576453,
34.5102310215708));
#239331=CARTESIAN_POINT('Ctrl Pts',(-7.25972318197535,3.14335898981476,
34.5089383044952));
#239332=CARTESIAN_POINT('Ctrl Pts',(-7.25210645253976,3.16089202957714,
34.5081756843678));
#239333=CARTESIAN_POINT('Ctrl Pts',(-7.22449779041522,3.22381962951235,
34.5054388026399));
#239334=CARTESIAN_POINT('Ctrl Pts',(-7.20414246775042,3.2690537927787,34.5034718910792));
#239335=CARTESIAN_POINT('Ctrl Pts',(-7.08754882379454,3.52177278577797,
34.4924847062207));
#239336=CARTESIAN_POINT('Ctrl Pts',(-6.98277127782974,3.72520383142453,
34.483651956027));
#239337=CARTESIAN_POINT('Ctrl Pts',(-6.70768292456216,4.20679388393263,
34.4626499021831));
#239338=CARTESIAN_POINT('Ctrl Pts',(-6.52870899158561,4.47951930306538,
34.4506872206033));
#239339=CARTESIAN_POINT('Ctrl Pts',(-6.00972063840075,5.17290993479888,
34.4191427874257));
#239340=CARTESIAN_POINT('Ctrl Pts',(-5.64260555892777,5.57105305774826,
34.3998725866302));
#239341=CARTESIAN_POINT('Ctrl Pts',(-5.2164350660965,5.94756608199953,34.3772962545697));
#239342=CARTESIAN_POINT('Ctrl Pts',(-5.19492398685463,5.96636420611167,
34.3761559116807));
#239343=CARTESIAN_POINT('Ctrl Pts',(-5.16633446096287,5.99107622159623,
34.3746385933119));
#239344=CARTESIAN_POINT('Ctrl Pts',(-5.15934664326809,5.99709498582975,
34.3742675961681));
#239345=CARTESIAN_POINT('Ctrl Pts',(-5.14848061043203,6.00642109604818,
34.373690458721));
#239346=CARTESIAN_POINT('Ctrl Pts',(-5.14460968183564,6.00973694935427,
34.3734848118043));
#239347=CARTESIAN_POINT('Ctrl Pts',(-5.13689091832819,6.01633595123726,
34.3730746457925));
#239348=CARTESIAN_POINT('Ctrl Pts',(-5.13304313382562,6.01961915498458,
34.3728701301292));
#239349=CARTESIAN_POINT('Ctrl Pts',(-5.12441730400735,6.02696504300323,
34.3724115379909));
#239350=CARTESIAN_POINT('Ctrl Pts',(-5.11963757457088,6.03102573696138,
34.3721573441653));
#239351=CARTESIAN_POINT('Ctrl Pts',(-5.10569518660571,6.04284219286316,
34.3714156173279));
#239352=CARTESIAN_POINT('Ctrl Pts',(-5.09651972614669,6.05058276407319,
34.3709271769505));
#239353=CARTESIAN_POINT('Ctrl Pts',(-5.02677329272439,6.10915080374051,
34.367211687322));
#239354=CARTESIAN_POINT('Ctrl Pts',(-4.96546639655223,6.15908397527802,
34.3639277919866));
#239355=CARTESIAN_POINT('Ctrl Pts',(-4.82260776964509,6.27192001731401,
34.3562424610373));
#239356=CARTESIAN_POINT('Ctrl Pts',(-4.74055700436013,6.33416484679106,
34.3518065623045));
#239357=CARTESIAN_POINT('Ctrl Pts',(-4.55310333349143,6.47068715544381,
34.3416626361279));
#239358=CARTESIAN_POINT('Ctrl Pts',(-4.44705247423557,6.54402510220171,
34.3359172604791));
#239359=CARTESIAN_POINT('Ctrl Pts',(-3.76030904391294,6.99452808568198,
34.2988753894218));
#239360=CARTESIAN_POINT('Ctrl Pts',(-3.1339110057794,7.29671921277099,34.2661012541298));
#239361=CARTESIAN_POINT('Ctrl Pts',(-2.4009978845483,7.53826223019135,34.2322486332985));
#239362=CARTESIAN_POINT('Ctrl Pts',(-2.32544074441799,7.56191206343619,
34.2288048065048));
#239363=CARTESIAN_POINT('Ctrl Pts',(-2.02737730355157,7.65031767360384,
34.2154046424973));
#239364=CARTESIAN_POINT('Ctrl Pts',(-1.80241675960301,7.7064209923196,34.2056975034139));
#239365=CARTESIAN_POINT('Ctrl Pts',(-1.55263291173244,7.75717650079496,
34.1953564828679));
#239366=CARTESIAN_POINT('Ctrl Pts',(-1.52994111845616,7.76168386424671,
34.1944209241997));
#239367=CARTESIAN_POINT('Ctrl Pts',(-1.49791701752003,7.76789904687555,
34.1931060205783));
#239368=CARTESIAN_POINT('Ctrl Pts',(-1.488601014569,7.76968969869472,34.192724152463));
#239369=CARTESIAN_POINT('Ctrl Pts',(-1.47238266917604,7.77277682671952,
34.1920604714581));
#239370=CARTESIAN_POINT('Ctrl Pts',(-1.46548178808664,7.77408087503589,
34.1917784281484));
#239371=CARTESIAN_POINT('Ctrl Pts',(-1.45107502149182,7.77678343377511,
34.1911903466519));
#239372=CARTESIAN_POINT('Ctrl Pts',(-1.44356882723896,7.77818027145643,
34.1908843596391));
#239373=CARTESIAN_POINT('Ctrl Pts',(-1.42581032641579,7.78145838269297,
34.190161417822));
#239374=CARTESIAN_POINT('Ctrl Pts',(-1.41555628975377,7.78333026667,34.1897447490815));
#239375=CARTESIAN_POINT('Ctrl Pts',(-1.38168199248268,7.78944489595657,
34.1883708063087));
#239376=CARTESIAN_POINT('Ctrl Pts',(-1.3580460252912,7.79360044659157,34.1874161840546));
#239377=CARTESIAN_POINT('Ctrl Pts',(-0.994047170786951,7.85589062829521,
34.1727763021128));
#239378=CARTESIAN_POINT('Ctrl Pts',(-0.650240750991511,7.89179093117464,
34.1597969559625));
#239379=CARTESIAN_POINT('Ctrl Pts',(0.190528588098214,7.92424735389335,
34.1293710571656));
#239380=CARTESIAN_POINT('Ctrl Pts',(0.686931845273835,7.8967163559241,34.1125470744031));
#239381=CARTESIAN_POINT('Ctrl Pts',(1.63259166383128,7.75437875179024,34.0793509219251));
#239382=CARTESIAN_POINT('Ctrl Pts',(2.08086441694054,7.64628993356028,34.0630341684548));
#239383=CARTESIAN_POINT('Ctrl Pts',(2.54498181759764,7.49051720398846,34.0436254849891));
#239384=CARTESIAN_POINT('Ctrl Pts',(2.5727220039266,7.48103481448433,34.04245655637));
#239385=CARTESIAN_POINT('Ctrl Pts',(2.61015496918314,7.46800632938839,34.0408677353606));
#239386=CARTESIAN_POINT('Ctrl Pts',(2.61989466946123,7.46459506059157,34.0404532873622));
#239387=CARTESIAN_POINT('Ctrl Pts',(2.63520953950674,7.45919745755351,34.0397999743238));
#239388=CARTESIAN_POINT('Ctrl Pts',(2.64078922238311,7.45722390106425,34.0395616115591));
#239389=CARTESIAN_POINT('Ctrl Pts',(2.65152407730603,7.45341338030751,34.0391023718561));
#239390=CARTESIAN_POINT('Ctrl Pts',(2.65667956932722,7.45157732403126,34.0388815301399));
#239391=CARTESIAN_POINT('Ctrl Pts',(2.66882880136625,7.44723633411519,34.0383604289886));
#239392=CARTESIAN_POINT('Ctrl Pts',(2.6758209202681,7.44472689823923,34.0380599980318));
#239393=CARTESIAN_POINT('Ctrl Pts',(2.6961601773935,7.43739488674601,34.0371845637561));
#239394=CARTESIAN_POINT('Ctrl Pts',(2.7094978508953,7.43254625256531,34.0366085872982));
#239395=CARTESIAN_POINT('Ctrl Pts',(2.80456618666071,7.39769622873416,34.0324898830865));
#239396=CARTESIAN_POINT('Ctrl Pts',(2.88580824261921,7.36638385988909,34.0289002688795));
#239397=CARTESIAN_POINT('Ctrl Pts',(3.15499382992904,7.25749761817918,34.0168049709042));
#239398=CARTESIAN_POINT('Ctrl Pts',(3.34045900833821,7.17402168633489,34.0081420734133));
#239399=CARTESIAN_POINT('Ctrl Pts',(3.8280737800776,6.93153953925002,33.984745234026));
#239400=CARTESIAN_POINT('Ctrl Pts',(4.12349815824072,6.75996718491266,33.9699218826192));
#239401=CARTESIAN_POINT('Ctrl Pts',(4.96362336634729,6.19642852570688,33.9265330512412));
#239402=CARTESIAN_POINT('Ctrl Pts',(5.4706192272667,5.75375277790836,33.8988970267875));
#239403=CARTESIAN_POINT('Ctrl Pts',(5.97341324591713,5.18746622838379,33.868147655446));
#239404=CARTESIAN_POINT('Ctrl Pts',(6.03003200365184,5.12154135587622,33.864628982967));
#239405=CARTESIAN_POINT('Ctrl Pts',(6.10796387820317,5.02771602740295,33.8597058539575));
#239406=CARTESIAN_POINT('Ctrl Pts',(6.13019465424269,5.00058643576555,33.8582920184751));
#239407=CARTESIAN_POINT('Ctrl Pts',(6.16645993343334,4.95572438913711,33.855969874392));
#239408=CARTESIAN_POINT('Ctrl Pts',(6.18060009993573,4.93807804104071,33.8550604379545));
#239409=CARTESIAN_POINT('Ctrl Pts',(6.2100350099089,4.90101998598743,33.8531588436651));
#239410=CARTESIAN_POINT('Ctrl Pts',(6.22531485121378,4.88159674027004,33.8521668582874));
#239411=CARTESIAN_POINT('Ctrl Pts',(6.26154222050212,4.8350989468069,33.8498032345234));
#239412=CARTESIAN_POINT('Ctrl Pts',(6.28240554564411,4.80795937748013,33.8484325571041));
#239413=CARTESIAN_POINT('Ctrl Pts',(6.3531651268356,4.71466644131793,33.8437508988213));
#239414=CARTESIAN_POINT('Ctrl Pts',(6.40219810248842,4.64786471352681,33.8404499471088));
#239415=CARTESIAN_POINT('Ctrl Pts',(6.67390184188345,4.26524036482616,33.8218216826655));
#239416=CARTESIAN_POINT('Ctrl Pts',(6.87424867518735,3.93420342718045,33.8067889470348));
#239417=CARTESIAN_POINT('Ctrl Pts',(7.16543486055353,3.36238324148139,33.7819609615455));
#239418=CARTESIAN_POINT('Ctrl Pts',(7.27018813362744,3.12944738746237,33.7721276616706));
#239419=CARTESIAN_POINT('Ctrl Pts',(7.4453491631003,2.68343728213385,33.7534916224684));
#239420=CARTESIAN_POINT('Ctrl Pts',(7.51831423271007,2.47164040696927,33.744717833383));
#239421=CARTESIAN_POINT('Ctrl Pts',(7.5898989491045,2.23116201769167,33.734677095712));
#239422=CARTESIAN_POINT('Ctrl Pts',(7.5974696294702,2.20524493515027,33.7335939392209));
#239423=CARTESIAN_POINT('Ctrl Pts',(7.60850237886289,2.16674475890125,33.7319829535654));
#239424=CARTESIAN_POINT('Ctrl Pts',(7.61206625219226,2.15419095490056,33.7314573518577));
#239425=CARTESIAN_POINT('Ctrl Pts',(7.61834831644763,2.13185202713648,33.7305214688025));
#239426=CARTESIAN_POINT('Ctrl Pts',(7.62107876122559,2.12207036895957,33.7301114652925));
#239427=CARTESIAN_POINT('Ctrl Pts',(7.62677935013026,2.10149543439788,33.7292485964937));
#239428=CARTESIAN_POINT('Ctrl Pts',(7.62974543424081,2.09070106042789,33.7287956382194));
#239429=CARTESIAN_POINT('Ctrl Pts',(7.63755898236424,2.06202739017408,33.7275916640917));
#239430=CARTESIAN_POINT('Ctrl Pts',(7.64236653881737,2.04413743381336,33.7268396841063));
#239431=CARTESIAN_POINT('Ctrl Pts',(7.66848931408079,1.94554857884579,33.7226912053715));
#239432=CARTESIAN_POINT('Ctrl Pts',(7.68858892867833,1.8645341408897,33.7192663447152));
#239433=CARTESIAN_POINT('Ctrl Pts',(7.74657487058553,1.61390801926714,33.7086411952719));
#239434=CARTESIAN_POINT('Ctrl Pts',(7.78015706553231,1.44335566140471,33.7013695011496));
#239435=CARTESIAN_POINT('Ctrl Pts',(7.89433954600021,0.74236463259594,33.6715033267744));
#239436=CARTESIAN_POINT('Ctrl Pts',(7.92650776288397,0.205465166371491,
33.6487805333601));
#239437=CARTESIAN_POINT('Ctrl Pts',(7.89859463168227,-0.461981566028062,
33.6213452956789));
#239438=CARTESIAN_POINT('Ctrl Pts',(7.88982110678699,-0.593251939845101,
33.6159822584154));
#239439=CARTESIAN_POINT('Ctrl Pts',(7.87468374746445,-0.757904671680177,
33.6092899609492));
#239440=CARTESIAN_POINT('Ctrl Pts',(7.87137343804469,-0.791545214675656,
33.6079244379071));
#239441=CARTESIAN_POINT('Ctrl Pts',(7.86544596437889,-0.848063048106572,
33.6056330656535));
#239442=CARTESIAN_POINT('Ctrl Pts',(7.86294435175595,-0.870951937648596,
33.6047058599445));
#239443=CARTESIAN_POINT('Ctrl Pts',(7.85831997680068,-0.911618717420446,
33.6030597617128));
#239444=CARTESIAN_POINT('Ctrl Pts',(7.85623672504698,-0.929400917681355,
33.6023404116204));
#239445=CARTESIAN_POINT('Ctrl Pts',(7.85135358338842,-0.969892497417391,
33.6007033172868));
#239446=CARTESIAN_POINT('Ctrl Pts',(7.84851549640411,-0.992597126123971,
33.5997860230528));
#239447=CARTESIAN_POINT('Ctrl Pts',(7.84047361374117,-1.05474023500931,
33.5972770295948));
#239448=CARTESIAN_POINT('Ctrl Pts',(7.83507077710528,-1.09415236137217,
33.5956876252606));
#239449=CARTESIAN_POINT('Ctrl Pts',(7.80263041955931,-1.31822172075325,
33.586659953005));
#239450=CARTESIAN_POINT('Ctrl Pts',(7.76936231264552,-1.50191907340749,
33.5792934349324));
#239451=CARTESIAN_POINT('Ctrl Pts',(7.64068251027363,-2.09246990461497,
33.5555742754769));
#239452=CARTESIAN_POINT('Ctrl Pts',(7.51953730779798,-2.49299799263316,
33.5393798474998));
#239453=CARTESIAN_POINT('Ctrl Pts',(7.10139902132887,-3.56186232690879,
33.4957149213162));
#239454=CARTESIAN_POINT('Ctrl Pts',(6.74269472370014,-4.20150497822946,
33.4694002469612));
#239455=CARTESIAN_POINT('Ctrl Pts',(6.27066974870917,-4.82340275239621,
33.4388608412441));
#239456=CARTESIAN_POINT('Ctrl Pts',(6.23949773618388,-4.86365922976025,
33.4368571473716));
#239457=CARTESIAN_POINT('Ctrl Pts',(6.20040904514496,-4.91314525266786,
33.4343576677292));
#239458=CARTESIAN_POINT('Ctrl Pts',(6.19285651983289,-4.92266154880706,
33.4338753244391));
#239459=CARTESIAN_POINT('Ctrl Pts',(6.16692716522239,-4.95517881529396,
33.4322212567101));
#239460=CARTESIAN_POINT('Ctrl Pts',(6.14844398118256,-4.97809444857104,
33.4310454658514));
#239461=CARTESIAN_POINT('Ctrl Pts',(6.12289995151748,-5.00940490325771,
33.4294243208895));
#239462=CARTESIAN_POINT('Ctrl Pts',(6.115948810461,-5.01788914261537,33.4289835516718));
#239463=CARTESIAN_POINT('Ctrl Pts',(6.10486905471203,-5.03135535318596,
33.4282815566676));
#239464=CARTESIAN_POINT('Ctrl Pts',(6.10075192059565,-5.036346778003,33.4280208258888));
#239465=CARTESIAN_POINT('Ctrl Pts',(6.09274305434589,-5.04603212953442,
33.4275138692608));
#239466=CARTESIAN_POINT('Ctrl Pts',(6.08885200972897,-5.05072661920389,
33.4272676736596));
#239467=CARTESIAN_POINT('Ctrl Pts',(6.07955262351533,-5.06191983159958,
33.4266795201582));
#239468=CARTESIAN_POINT('Ctrl Pts',(6.07413928928858,-5.06841438492518,
33.4263373394146));
#239469=CARTESIAN_POINT('Ctrl Pts',(6.05794192546089,-5.08778367091741,
33.4253140352011));
#239470=CARTESIAN_POINT('Ctrl Pts',(6.0471273354793,-5.10063270953619,33.4246315154351));
#239471=CARTESIAN_POINT('Ctrl Pts',(5.95231133520476,-5.21256017194947,
33.4186530173416));
#239472=CARTESIAN_POINT('Ctrl Pts',(5.86593281889663,-5.30957862845449,
33.4132380705982));
#239473=CARTESIAN_POINT('Ctrl Pts',(5.73162163410296,-5.45315366801678,
33.4048292385462));
#239474=CARTESIAN_POINT('Ctrl Pts',(5.68543353193467,-5.50129227403439,
33.4019425125504));
#239475=CARTESIAN_POINT('Ctrl Pts',(5.35132360401761,-5.84080947781086,
33.3811305794373));
#239476=CARTESIAN_POINT('Ctrl Pts',(5.04177128796185,-6.1100113505011,33.3622403092658));
#239477=CARTESIAN_POINT('Ctrl Pts',(4.30504545794233,-6.65644130039882,
33.3202099944185));
#239478=CARTESIAN_POINT('Ctrl Pts',(3.8691073434636,-6.91894037269793,33.2972827902246));
#239479=CARTESIAN_POINT('Ctrl Pts',(3.26826795600276,-7.20606439880843,
33.2691241546764));
#239480=CARTESIAN_POINT('Ctrl Pts',(3.12353557052244,-7.26997034578886,
33.2625742465813));
#239481=CARTESIAN_POINT('Ctrl Pts',(2.95971212467584,-7.33650955533215,
33.2554156861002));
#239482=CARTESIAN_POINT('Ctrl Pts',(2.94242077799682,-7.34346160116359,
33.2546632260482));
#239483=CARTESIAN_POINT('Ctrl Pts',(2.91640742958189,-7.35381372700929,
33.2535358687255));
#239484=CARTESIAN_POINT('Ctrl Pts',(2.90770375475078,-7.35725951032207,
33.2531594524301));
#239485=CARTESIAN_POINT('Ctrl Pts',(2.89265050535234,-7.36318820451808,
33.2525097744516));
#239486=CARTESIAN_POINT('Ctrl Pts',(2.88630380784358,-7.36567836729344,
33.2522362718966));
#239487=CARTESIAN_POINT('Ctrl Pts',(2.87354018498532,-7.3706672171093,33.2516870672129));
#239488=CARTESIAN_POINT('Ctrl Pts',(2.8671231998896,-7.37316573644356,33.2514113708138));
#239489=CARTESIAN_POINT('Ctrl Pts',(2.85198900607451,-7.37903564599636,
33.2507621383588));
#239490=CARTESIAN_POINT('Ctrl Pts',(2.84326906030105,-7.38239997610226,
33.2503888370053));
#239491=CARTESIAN_POINT('Ctrl Pts',(2.8162721661635,-7.39276099202303,33.2492354725393));
#239492=CARTESIAN_POINT('Ctrl Pts',(2.79797513955904,-7.39970534038252,
33.2484571469723));
#239493=CARTESIAN_POINT('Ctrl Pts',(2.75574074133208,-7.41555569515303,
33.2466682485789));
#239494=CARTESIAN_POINT('Ctrl Pts',(2.73178557906378,-7.42441383994552,
33.2456592630205));
#239495=CARTESIAN_POINT('Ctrl Pts',(2.65222499606333,-7.45339657343536,
33.2423267522719));
#239496=CARTESIAN_POINT('Ctrl Pts',(2.59643629125748,-7.47301389554289,
33.2400199377527));
#239497=CARTESIAN_POINT('Ctrl Pts',(2.37704236793153,-7.54740725644711,
33.231061504581));
#239498=CARTESIAN_POINT('Ctrl Pts',(2.21187921263003,-7.59745228526428,
33.2245639999587));
#239499=CARTESIAN_POINT('Ctrl Pts',(1.82205695413581,-7.70177844077924,
33.2097171392192));
#239500=CARTESIAN_POINT('Ctrl Pts',(1.59639371773892,-7.75169767255701,
33.2014954827003));
#239501=CARTESIAN_POINT('Ctrl Pts',(0.565705906051421,-7.9327716704868,
33.1650180842437));
#239502=CARTESIAN_POINT('Ctrl Pts',(-0.254295056719606,-7.94882421314376,
33.1393353748658));
#239503=CARTESIAN_POINT('Ctrl Pts',(-1.10698695403444,-7.8332976042954,
33.1055569888184));
#239504=CARTESIAN_POINT('Ctrl Pts',(-1.15180529946786,-7.82683306810016,
33.1037594655331));
#239505=CARTESIAN_POINT('Ctrl Pts',(-1.20477604327292,-7.81872781773682,
33.1016064147208));
#239506=CARTESIAN_POINT('Ctrl Pts',(-1.21298522435998,-7.81745846467005,
33.1012719307997));
#239507=CARTESIAN_POINT('Ctrl Pts',(-1.22618854464113,-7.81539558974431,
33.1007326316085));
#239508=CARTESIAN_POINT('Ctrl Pts',(-1.23118396476856,-7.8146102024239,
33.1005282839324));
#239509=CARTESIAN_POINT('Ctrl Pts',(-1.24006366485248,-7.81320539717708,
33.100164492716));
#239510=CARTESIAN_POINT('Ctrl Pts',(-1.24394824663736,-7.81258787028632,
33.1000051588568));
#239511=CARTESIAN_POINT('Ctrl Pts',(-1.25204194133461,-7.81129503666675,
33.099672787477));
#239512=CARTESIAN_POINT('Ctrl Pts',(-1.25625097096794,-7.81061922452501,
33.0994997204936));
#239513=CARTESIAN_POINT('Ctrl Pts',(-1.26715663428347,-7.80885914105427,
33.0990507235426));
#239514=CARTESIAN_POINT('Ctrl Pts',(-1.27385241069877,-7.80776965950133,
33.0987744872436));
#239515=CARTESIAN_POINT('Ctrl Pts',(-1.30292340751619,-7.8030010753022,
33.0975726729861));
#239516=CARTESIAN_POINT('Ctrl Pts',(-1.32528370329718,-7.79923446590876,
33.0966418547931));
#239517=CARTESIAN_POINT('Ctrl Pts',(-1.48784462420015,-7.77113170041769,
33.0898295792521));
#239518=CARTESIAN_POINT('Ctrl Pts',(-1.62737531321939,-7.7431140196866,
33.0837382771522));
#239519=CARTESIAN_POINT('Ctrl Pts',(-1.90170194822282,-7.6802872753975,
33.0713916472817));
#239520=CARTESIAN_POINT('Ctrl Pts',(-2.03648968708364,-7.64565169904366,
33.0651449976961));
#239521=CARTESIAN_POINT('Ctrl Pts',(-2.51367454224812,-7.5095187469555,
33.0425606024695));
#239522=CARTESIAN_POINT('Ctrl Pts',(-2.8500298662681,-7.38842059827652,
33.0257893660323));
#239523=CARTESIAN_POINT('Ctrl Pts',(-3.35377556121985,-7.16752030909823,
33.0003370067336));
#239524=CARTESIAN_POINT('Ctrl Pts',(-3.52760930456423,-7.08358206223383,
32.9914835664204));
#239525=CARTESIAN_POINT('Ctrl Pts',(-4.01859904418437,-6.82393887190937,
32.966454707792));
#239526=CARTESIAN_POINT('Ctrl Pts',(-4.32699442876898,-6.63268024582356,
32.9507292024945));
#239527=CARTESIAN_POINT('Ctrl Pts',(-4.67033730848178,-6.38557225903462,
32.9333674822912));
#239528=CARTESIAN_POINT('Ctrl Pts',(-4.71905137201568,-6.34965652838012,
32.9309069465731));
#239529=CARTESIAN_POINT('Ctrl Pts',(-4.77768189135187,-6.30538217618281,
32.9279483816718));
#239530=CARTESIAN_POINT('Ctrl Pts',(-4.78799534936075,-6.29755422202991,
32.9274280596859));
#239531=CARTESIAN_POINT('Ctrl Pts',(-4.80490077869327,-6.28465740135022,
32.9265753338291));
#239532=CARTESIAN_POINT('Ctrl Pts',(-4.81150403756006,-6.27960341443356,
32.9262423010124));
#239533=CARTESIAN_POINT('Ctrl Pts',(-4.8230891819454,-6.27070740211041,
32.9256580791199));
#239534=CARTESIAN_POINT('Ctrl Pts',(-4.82807446967707,-6.2668698323316,
32.9254067013155));
#239535=CARTESIAN_POINT('Ctrl Pts',(-4.83874047572135,-6.25863908361579,
32.9248689268498));
#239536=CARTESIAN_POINT('Ctrl Pts',(-4.84441980298106,-6.25424410646158,
32.9245826070497));
#239537=CARTESIAN_POINT('Ctrl Pts',(-4.85919300959943,-6.24277958701514,
32.9238378969922));
#239538=CARTESIAN_POINT('Ctrl Pts',(-4.86827746307664,-6.2356978936318,
32.9233800254965));
#239539=CARTESIAN_POINT('Ctrl Pts',(-4.88808292797253,-6.22018908423993,
32.922381941198));
#239540=CARTESIAN_POINT('Ctrl Pts',(-4.89879769230012,-6.21175402981377,
32.92184206974));
#239541=CARTESIAN_POINT('Ctrl Pts',(-4.92998613446486,-6.18707046143443,
32.9202708581929));
#239542=CARTESIAN_POINT('Ctrl Pts',(-4.95040125335474,-6.17074806076066,
32.9192426907221));
#239543=CARTESIAN_POINT('Ctrl Pts',(-5.01960032552379,-6.11485723849423,
32.9157583943229));
#239544=CARTESIAN_POINT('Ctrl Pts',(-5.06799432180668,-6.07480866113479,
32.9133230221243));
#239545=CARTESIAN_POINT('Ctrl Pts',(-5.25347026708293,-5.91755837522489,
32.9039893140947));
#239546=CARTESIAN_POINT('Ctrl Pts',(-5.38700932170671,-5.79625590262394,
32.8972712509505));
#239547=CARTESIAN_POINT('Ctrl Pts',(-5.77102749514541,-5.42268040001609,
32.8778186098568));
#239548=CARTESIAN_POINT('Ctrl Pts',(-6.00878352578486,-5.15798010686436,
32.8656141319729));
#239549=CARTESIAN_POINT('Ctrl Pts',(-6.61625359361432,-4.38242722531574,
32.832262283388));
#239550=CARTESIAN_POINT('Ctrl Pts',(-6.94392670045103,-3.84215250971736,
32.811695866637));
#239551=CARTESIAN_POINT('Ctrl Pts',(-7.22018416563913,-3.23332405583869,
32.7854154625734));
#239552=CARTESIAN_POINT('Ctrl Pts',(-7.23604542286125,-3.19766952160274,
32.7838652966413));
#239553=CARTESIAN_POINT('Ctrl Pts',(-7.25465465695654,-3.15499027336271,
32.7819947604547));
#239554=CARTESIAN_POINT('Ctrl Pts',(-7.25765746243578,-3.14807655146799,
32.7816912813118));
#239555=CARTESIAN_POINT('Ctrl Pts',(-7.26252341858543,-3.13682910709141,
32.7811967981714));
#239556=CARTESIAN_POINT('Ctrl Pts',(-7.26439257762675,-3.13249800165178,
32.7810061981507));
#239557=CARTESIAN_POINT('Ctrl Pts',(-7.26772792946892,-3.12475048040685,
32.7806649176362));
#239558=CARTESIAN_POINT('Ctrl Pts',(-7.26919558695255,-3.12133470491688,
32.7805143362191));
#239559=CARTESIAN_POINT('Ctrl Pts',(-7.2722949430002,-3.11410732840079,
32.7801954815238));
#239560=CARTESIAN_POINT('Ctrl Pts',(-7.27392605338335,-3.11029547801546,
32.7800271693351));
#239561=CARTESIAN_POINT('Ctrl Pts',(-7.27824888268384,-3.10017117176651,
32.7795797564026));
#239562=CARTESIAN_POINT('Ctrl Pts',(-7.280935380527,-3.09385650548485,32.7793003128052));
#239563=CARTESIAN_POINT('Ctrl Pts',(-7.29325459756733,-3.06479503107134,
32.7780125054566));
#239564=CARTESIAN_POINT('Ctrl Pts',(-7.30278885919563,-3.04200691288834,
32.7769977724746));
#239565=CARTESIAN_POINT('Ctrl Pts',(-7.3742873870809,-2.86884281070689,
32.76925187874));
#239566=CARTESIAN_POINT('Ctrl Pts',(-7.43170412403889,-2.7166414463969,
32.762244000626));
#239567=CARTESIAN_POINT('Ctrl Pts',(-7.76625893670682,-1.73960537619222,
32.7165088511698));
#239568=CARTESIAN_POINT('Ctrl Pts',(-7.91041738305944,-0.875554323490879,
32.6734984947441));
#239569=CARTESIAN_POINT('Ctrl Pts',(-7.91099823792547,-0.00528010797013839,
32.6351117714718));
#239570=CARTESIAN_POINT('',(-7.90633320911253,0.0091686610735674,30.6423296657176));
#239571=CARTESIAN_POINT('Ctrl Pts',(-7.91099848652071,-0.00489349231630381,
32.6423315082371));
#239572=CARTESIAN_POINT('Ctrl Pts',(-7.91112000549778,0.191558526308438,
32.6344573356086));
#239573=CARTESIAN_POINT('Ctrl Pts',(-7.90391953153266,0.3880566740996,32.6265831629801));
#239574=CARTESIAN_POINT('Ctrl Pts',(-7.88941347252823,0.584017173968438,
32.6187089903516));
#239575=CARTESIAN_POINT('Ctrl Pts',(-7.87490737418884,0.779978205208178,
32.6108347963714));
#239576=CARTESIAN_POINT('Ctrl Pts',(-7.85309567576184,0.975401241513716,
32.6029606023911));
#239577=CARTESIAN_POINT('Ctrl Pts',(-7.82404679708957,1.16970625242088,
32.5950864084109));
#239578=CARTESIAN_POINT('Ctrl Pts',(-7.79499295893251,1.36404443682007,
32.5872108700777));
#239579=CARTESIAN_POINT('Ctrl Pts',(-7.75869952909333,1.55726387423657,
32.5793353317445));
#239580=CARTESIAN_POINT('Ctrl Pts',(-7.7152863595527,1.74879312387145,32.5714597934113));
#239581=CARTESIAN_POINT('Ctrl Pts',(-7.67185848387765,1.94038725370098,
32.5635815872534));
#239582=CARTESIAN_POINT('Ctrl Pts',(-7.62130613881505,2.1302897186296,32.5557033810955));
#239583=CARTESIAN_POINT('Ctrl Pts',(-7.56379956637718,2.31794243234649,
32.5478251749376));
#239584=CARTESIAN_POINT('Ctrl Pts',(-7.50623084948155,2.50579793290405,
32.539938455199));
#239585=CARTESIAN_POINT('Ctrl Pts',(-7.44169299101388,2.69139849450419,
32.5320517354603));
#239586=CARTESIAN_POINT('Ctrl Pts',(-7.37040551932443,2.87420310359445,
32.5241650157217));
#239587=CARTESIAN_POINT('Ctrl Pts',(-7.29907845676179,3.05710923675234,
32.516273915941));
#239588=CARTESIAN_POINT('Ctrl Pts',(-7.22099444403144,3.23721600540227,
32.5083828161603));
#239589=CARTESIAN_POINT('Ctrl Pts',(-7.13641997995962,3.41400510685517,
32.5004917163797));
#239590=CARTESIAN_POINT('Ctrl Pts',(-7.0517210203732,3.59105444584432,32.4925890007225));
#239591=CARTESIAN_POINT('Ctrl Pts',(-6.960512674969,3.76477605187092,32.4846862850654));
#239592=CARTESIAN_POINT('Ctrl Pts',(-6.86310673043122,3.93467749716667,
32.4767835694082));
#239593=CARTESIAN_POINT('Ctrl Pts',(-6.77073650364176,4.09579533353997,
32.4692894103919));
#239594=CARTESIAN_POINT('Ctrl Pts',(-6.67279342162344,4.25347781647384,
32.4617952513755));
#239595=CARTESIAN_POINT('Ctrl Pts',(-6.56957742872845,4.4073317787457,32.4543010923592));
#239596=CARTESIAN_POINT('Ctrl Pts',(-6.45121722598701,4.58375973003807,
32.4457073642394));
#239597=CARTESIAN_POINT('Ctrl Pts',(-6.32567389938808,4.75552543575751,
32.4371136361197));
#239598=CARTESIAN_POINT('Ctrl Pts',(-6.19332147061131,4.92206157637884,
32.4285199079999));
#239599=CARTESIAN_POINT('Ctrl Pts',(-6.06116013588264,5.08835726757617,
32.4199385877393));
#239600=CARTESIAN_POINT('Ctrl Pts',(-5.92220947264522,5.24943826804819,
32.4113572674787));
#239601=CARTESIAN_POINT('Ctrl Pts',(-5.77688574263718,5.40476753584419,
32.4027759472181));
#239602=CARTESIAN_POINT('Ctrl Pts',(-5.62527722371201,5.56681430023003,
32.3938235121611));
#239603=CARTESIAN_POINT('Ctrl Pts',(-5.46673230395977,5.72260058575925,
32.3848710771042));
#239604=CARTESIAN_POINT('Ctrl Pts',(-5.30177229556195,5.87155273552165,
32.3759186420472));
#239605=CARTESIAN_POINT('Ctrl Pts',(-5.14427352695691,6.01376769050683,
32.3673711309796));
#239606=CARTESIAN_POINT('Ctrl Pts',(-4.98092733305738,6.14975280576015,
32.358823619912));
#239607=CARTESIAN_POINT('Ctrl Pts',(-4.812227598083,6.27904344181885,32.3502761088444));
#239608=CARTESIAN_POINT('Ctrl Pts',(-4.64378722517104,6.40813530408562,
32.3417417388769));
#239609=CARTESIAN_POINT('Ctrl Pts',(-4.47000992688538,6.5305530686014,32.3332073689094));
#239610=CARTESIAN_POINT('Ctrl Pts',(-4.2914240497278,6.64587094558854,32.3246729989419));
#239611=CARTESIAN_POINT('Ctrl Pts',(-4.11322699487409,6.76093774917994,
32.3161572102499));
#239612=CARTESIAN_POINT('Ctrl Pts',(-3.93024246014209,6.86893537581798,
32.3076414215579));
#239613=CARTESIAN_POINT('Ctrl Pts',(-3.74302932750089,6.96948007052666,
32.299125632866));
#239614=CARTESIAN_POINT('Ctrl Pts',(-3.71533720103348,6.98435240540092,
32.2978659974221));
#239615=CARTESIAN_POINT('Ctrl Pts',(-3.68755261220178,6.99906174571603,
32.2966063619783));
#239616=CARTESIAN_POINT('Ctrl Pts',(-3.65967742918494,7.01360692613396,
32.2953467265344));
#239617=CARTESIAN_POINT('Ctrl Pts',(-3.48497466296167,7.10476626498729,
32.2874521847716));
#239618=CARTESIAN_POINT('Ctrl Pts',(-3.30687280924795,7.18938953503818,
32.2795576430088));
#239619=CARTESIAN_POINT('Ctrl Pts',(-3.12590476337168,7.2672305873923,32.271663101246));
#239620=CARTESIAN_POINT('Ctrl Pts',(-2.94489593494597,7.34508918182989,
32.2637667803871));
#239621=CARTESIAN_POINT('Ctrl Pts',(-2.76101994164748,7.41616237708621,
32.2558704595283));
#239622=CARTESIAN_POINT('Ctrl Pts',(-2.57482919663688,7.48025237596609,
32.2479741386694));
#239623=CARTESIAN_POINT('Ctrl Pts',(-2.38856579612657,7.54436738409599,
32.2400747365019));
#239624=CARTESIAN_POINT('Ctrl Pts',(-2.19998616738562,7.60149365387825,
32.2321753343345));
#239625=CARTESIAN_POINT('Ctrl Pts',(-2.00965766347297,7.65148332518894,
32.224275932167));
#239626=CARTESIAN_POINT('Ctrl Pts',(-1.81911972483716,7.70152800440836,
32.2163678376121));
#239627=CARTESIAN_POINT('Ctrl Pts',(-1.62682939779038,7.74442030912966,
32.2084597430572));
#239628=CARTESIAN_POINT('Ctrl Pts',(-1.43336521450231,7.78006331348626,
32.2005516485022));
#239629=CARTESIAN_POINT('Ctrl Pts',(-1.2397857683471,7.81572755337496,32.192638842431));
#239630=CARTESIAN_POINT('Ctrl Pts',(-1.04503140962768,7.84413383167741,
32.1847260363598));
#239631=CARTESIAN_POINT('Ctrl Pts',(-0.849685900793989,7.8652371146706,
32.1768132302886));
#239632=CARTESIAN_POINT('Ctrl Pts',(-0.654066647658819,7.88636997041156,
32.1688893357332));
#239633=CARTESIAN_POINT('Ctrl Pts',(-0.45785493019226,7.90017935774268,
32.1609654411779));
#239634=CARTESIAN_POINT('Ctrl Pts',(-0.261636014943777,7.90667234654911,
32.1530415466225));
#239635=CARTESIAN_POINT('Ctrl Pts',(-0.124208424811838,7.91121989897692,
32.1474918179849));
#239636=CARTESIAN_POINT('Ctrl Pts',(0.0132227108735123,7.91217962945228,
32.1419420893473));
#239637=CARTESIAN_POINT('Ctrl Pts',(0.150457961287746,7.90956910342688,
32.1363923607096));
#239638=CARTESIAN_POINT('Ctrl Pts',(0.351362711009467,7.90574743897704,
32.1282678676249));
#239639=CARTESIAN_POINT('Ctrl Pts',(0.552289511266152,7.89426372287408,
32.1201433745403));
#239640=CARTESIAN_POINT('Ctrl Pts',(0.75262882604898,7.87511719596605,32.1120188814556));
#239641=CARTESIAN_POINT('Ctrl Pts',(0.95279114157448,7.85598758496415,32.1039015663391));
#239642=CARTESIAN_POINT('Ctrl Pts',(1.15236668873377,7.82920869128804,32.0957842512227));
#239643=CARTESIAN_POINT('Ctrl Pts',(1.35074749380469,7.79483176264763,32.0876669361062));
#239644=CARTESIAN_POINT('Ctrl Pts',(1.54898127630582,7.76048031119182,32.0795556368366));
#239645=CARTESIAN_POINT('Ctrl Pts',(1.74602176733017,7.7185421071342,32.0714443375669));
#239646=CARTESIAN_POINT('Ctrl Pts',(1.9412670915232,7.66912009811876,32.0633330382973));
#239647=CARTESIAN_POINT('Ctrl Pts',(2.13639547986959,7.61972768881072,32.0552265970269));
#239648=CARTESIAN_POINT('Ctrl Pts',(2.32973053525365,7.56286049108492,32.0471201557565));
#239649=CARTESIAN_POINT('Ctrl Pts',(2.52068097188842,7.49867244503716,32.0390137144862));
#239650=CARTESIAN_POINT('Ctrl Pts',(2.71154416765701,7.43451372503252,32.0309109768626));
#239651=CARTESIAN_POINT('Ctrl Pts',(2.90002461400492,7.36304092931086,32.0228082392389));
#239652=CARTESIAN_POINT('Ctrl Pts',(3.08554602564457,7.28445788810869,32.0147055016153));
#239653=CARTESIAN_POINT('Ctrl Pts',(3.27274283328488,7.20516518373727,32.0065295902588));
#239654=CARTESIAN_POINT('Ctrl Pts',(3.45692658085326,7.11863327249783,31.9983536789023));
#239655=CARTESIAN_POINT('Ctrl Pts',(3.63752461481758,7.02512175528626,31.9901777675459));
#239656=CARTESIAN_POINT('Ctrl Pts',(3.81643807878664,6.93248248841233,31.9820781188964));
#239657=CARTESIAN_POINT('Ctrl Pts',(3.99183215466595,6.83299343225187,31.973978470247));
#239658=CARTESIAN_POINT('Ctrl Pts',(4.16317336433251,6.72695388259146,31.9658788215976));
#239659=CARTESIAN_POINT('Ctrl Pts',(4.3345134095745,6.62091505356946,31.9577792279929));
#239660=CARTESIAN_POINT('Ctrl Pts',(4.501800370889,6.50832598870004,31.9496796343882));
#239661=CARTESIAN_POINT('Ctrl Pts',(4.66452819305336,6.38953032203545,31.9415800407835));
#239662=CARTESIAN_POINT('Ctrl Pts',(4.82727591879314,6.27072012522794,31.9334794565008));
#239663=CARTESIAN_POINT('Ctrl Pts',(4.9854631345689,6.14570200217393,31.9253788722181));
#239664=CARTESIAN_POINT('Ctrl Pts',(5.13861498424679,6.01486134866585,31.9172782879354));
#239665=CARTESIAN_POINT('Ctrl Pts',(5.29426820851848,5.88188372138169,31.9090453996958));
#239666=CARTESIAN_POINT('Ctrl Pts',(5.44471989471052,5.74289193843662,31.9008125114562));
#239667=CARTESIAN_POINT('Ctrl Pts',(5.58950865835294,5.59833135480543,31.8925796232166));
#239668=CARTESIAN_POINT('Ctrl Pts',(5.73210667912259,5.45595806154336,31.8844713036298));
#239669=CARTESIAN_POINT('Ctrl Pts',(5.86921173082491,5.30818354979302,31.876362984043));
#239670=CARTESIAN_POINT('Ctrl Pts',(6.00042193345515,5.15546871006995,31.8682546644563));
#239671=CARTESIAN_POINT('Ctrl Pts',(6.13465582268388,4.99923461799452,31.8599594918903));
#239672=CARTESIAN_POINT('Ctrl Pts',(6.26271967295164,4.83783003424346,31.8516643193242));
#239673=CARTESIAN_POINT('Ctrl Pts',(6.38422822998997,4.671782412249,31.8433691467582));
#239674=CARTESIAN_POINT('Ctrl Pts',(6.50573678702833,4.50573479025451,31.8350739741922));
#239675=CARTESIAN_POINT('Ctrl Pts',(6.62068987352878,4.3350444414627,31.8267788016262));
#239676=CARTESIAN_POINT('Ctrl Pts',(6.72875067701665,4.16026866038096,31.8184836290601));
#239677=CARTESIAN_POINT('Ctrl Pts',(6.83072554834154,3.99533616671763,31.8106556365991));
#239678=CARTESIAN_POINT('Ctrl Pts',(6.92675804387642,3.82644917922782,31.802827644138));
#239679=CARTESIAN_POINT('Ctrl Pts',(7.01652494160159,3.65407973967219,31.794999651677));
#239680=CARTESIAN_POINT('Ctrl Pts',(7.10621602067271,3.4818558862874,31.787178270872));
#239681=CARTESIAN_POINT('Ctrl Pts',(7.18965187749445,3.30615574759313,31.779356890067));
#239682=CARTESIAN_POINT('Ctrl Pts',(7.26655298979631,3.12747959969082,31.771535509262));
#239683=CARTESIAN_POINT('Ctrl Pts',(7.34340273040609,2.9489228115192,31.7637193533173));
#239684=CARTESIAN_POINT('Ctrl Pts',(7.41372628156807,2.76739429547649,31.7559031973726));
#239685=CARTESIAN_POINT('Ctrl Pts',(7.47729035038828,2.58341828126812,31.7480870414278));
#239686=CARTESIAN_POINT('Ctrl Pts',(7.54082388279168,2.39953064982624,31.7402746403937));
#239687=CARTESIAN_POINT('Ctrl Pts',(7.59760428629726,2.21319819435234,31.7324622393596));
#239688=CARTESIAN_POINT('Ctrl Pts',(7.64744658960323,2.02496460689217,31.7246498383254));
#239689=CARTESIAN_POINT('Ctrl Pts',(7.69727432455182,1.83678603804048,31.7168397207703));
#239690=CARTESIAN_POINT('Ctrl Pts',(7.74016790974515,1.64670778446427,31.7090296032151));
#239691=CARTESIAN_POINT('Ctrl Pts',(7.77599234082576,1.45528832724622,31.7012194856599));
#239692=CARTESIAN_POINT('Ctrl Pts',(7.81181881307571,1.26385796351785,31.6934089231075));
#239693=CARTESIAN_POINT('Ctrl Pts',(7.84057525530673,1.07108658848957,31.6855983605551));
#239694=CARTESIAN_POINT('Ctrl Pts',(7.86217777683998,0.877542936478608,
31.6777877980026));
#239695=CARTESIAN_POINT('Ctrl Pts',(7.87901098135532,0.726729066351007,
31.6717016197469));
#239696=CARTESIAN_POINT('Ctrl Pts',(7.89150141216044,0.575446532133352,
31.6656154414912));
#239697=CARTESIAN_POINT('Ctrl Pts',(7.89963121182758,0.423966646234818,
31.6595292632355));
#239698=CARTESIAN_POINT('Ctrl Pts',(7.91117284628295,0.208915163791779,
31.6508888972321));
#239699=CARTESIAN_POINT('Ctrl Pts',(7.91391921597654,-0.00643163438786562,
31.6422485312288));
#239700=CARTESIAN_POINT('Ctrl Pts',(7.90790194795712,-0.221377012121736,
31.6336081652254));
#239701=CARTESIAN_POINT('Ctrl Pts',(7.90187467026881,-0.436679949474773,
31.6249534260543));
#239702=CARTESIAN_POINT('Ctrl Pts',(7.88705462113972,-0.651579901821391,
31.6162986868832));
#239703=CARTESIAN_POINT('Ctrl Pts',(7.86352535064658,-0.865384342207935,
31.6076439477121));
#239704=CARTESIAN_POINT('Ctrl Pts',(7.83926834535949,-1.08580152183831,
31.5987215268536));
#239705=CARTESIAN_POINT('Ctrl Pts',(7.80575485188671,-1.3050540693302,31.5897991059952));
#239706=CARTESIAN_POINT('Ctrl Pts',(7.76313293069965,-1.52239551375017,
31.5808766851367));
#239707=CARTESIAN_POINT('Ctrl Pts',(7.72165097984496,-1.73392392131651,
31.5721929042736));
#239708=CARTESIAN_POINT('Ctrl Pts',(7.67154163656631,-1.94364192956361,
31.5635091234104));
#239709=CARTESIAN_POINT('Ctrl Pts',(7.61299237196658,-2.150876134132,31.5548253425472));
#239710=CARTESIAN_POINT('Ctrl Pts',(7.55202960860712,-2.36665287974031,
31.5457836016911));
#239711=CARTESIAN_POINT('Ctrl Pts',(7.4819165041512,-2.57973645053514,31.536741860835));
#239712=CARTESIAN_POINT('Ctrl Pts',(7.40292104009272,-2.7893872219813,31.5277001199789));
#239713=CARTESIAN_POINT('Ctrl Pts',(7.32392557603425,-2.99903799342743,
31.5186583791228));
#239714=CARTESIAN_POINT('Ctrl Pts',(7.23604788008165,-3.20525571698875,
31.5096166382667));
#239715=CARTESIAN_POINT('Ctrl Pts',(7.13961162634878,-3.40732546506866,
31.5005748974106));
#239716=CARTESIAN_POINT('Ctrl Pts',(7.05085195984431,-3.59330991340587,
31.4922529036381));
#239717=CARTESIAN_POINT('Ctrl Pts',(6.95476663062083,-3.77593846816199,
31.4839309098656));
#239718=CARTESIAN_POINT('Ctrl Pts',(6.85162772868264,-3.9546325325556,31.4756089160932));
#239719=CARTESIAN_POINT('Ctrl Pts',(6.74858056026681,-4.13316766335924,
31.4672943240458));
#239720=CARTESIAN_POINT('Ctrl Pts',(6.63849247985562,-4.30777503239189,
31.4589797319984));
#239721=CARTESIAN_POINT('Ctrl Pts',(6.52168189619684,-4.47789975823694,
31.4506651399511));
#239722=CARTESIAN_POINT('Ctrl Pts',(6.40496808221328,-4.6478835472426,31.4423574359814));
#239723=CARTESIAN_POINT('Ctrl Pts',(6.28154304031016,-4.81339186116776,
31.4340497320117));
#239724=CARTESIAN_POINT('Ctrl Pts',(6.1517694211802,-4.97389726357836,31.425742028042));
#239725=CARTESIAN_POINT('Ctrl Pts',(6.02212673778417,-5.1342407232705,31.4174427061712));
#239726=CARTESIAN_POINT('Ctrl Pts',(5.88614844625316,-5.28959112027977,
31.4091433843005));
#239727=CARTESIAN_POINT('Ctrl Pts',(5.74423876278191,-5.43945236546417,
31.4008440624297));
#239728=CARTESIAN_POINT('Ctrl Pts',(5.60241974552068,-5.58921786417942,
31.3925500430023));
#239729=CARTESIAN_POINT('Ctrl Pts',(5.4546770957743,-5.73350099465784,31.3842560235749));
#239730=CARTESIAN_POINT('Ctrl Pts',(5.3014542838967,-5.87183987143326,31.3759620041475));
#239731=CARTESIAN_POINT('Ctrl Pts',(5.14834509435641,-6.01007616304967,
31.3676741351482));
#239732=CARTESIAN_POINT('Ctrl Pts',(4.9897640699021,-6.14237680291009,31.3593862661488));
#239733=CARTESIAN_POINT('Ctrl Pts',(4.82619078682655,-6.26831743685261,
31.3510983971494));
#239734=CARTESIAN_POINT('Ctrl Pts',(4.76383758172261,-6.31632529016147,
31.3479391086282));
#239735=CARTESIAN_POINT('Ctrl Pts',(4.70075932402139,-6.36340937113779,
31.344779820107));
#239736=CARTESIAN_POINT('Ctrl Pts',(4.63698390055644,-6.40954766781404,
31.3416205315859));
#239737=CARTESIAN_POINT('Ctrl Pts',(4.47342548012091,-6.52787392134491,
31.3335182217594));
#239738=CARTESIAN_POINT('Ctrl Pts',(4.30534816810133,-6.63992687499192,
31.325415911933));
#239739=CARTESIAN_POINT('Ctrl Pts',(4.13326606970902,-6.74537119786541,
31.3173136021066));
#239740=CARTESIAN_POINT('Ctrl Pts',(3.96114598873752,-6.85083879478879,
31.3092095039092));
#239741=CARTESIAN_POINT('Ctrl Pts',(3.78501963037437,-6.94969468511056,
31.3011054057118));
#239742=CARTESIAN_POINT('Ctrl Pts',(3.60542753985813,-7.04164847566481,
31.2930013075145));
#239743=CARTESIAN_POINT('Ctrl Pts',(3.42577328152959,-7.1336340970529,31.2848944039928));
#239744=CARTESIAN_POINT('Ctrl Pts',(3.24265118208867,-7.21871270823087,
31.2767875004711));
#239745=CARTESIAN_POINT('Ctrl Pts',(3.05662419990538,-7.29664097380108,
31.2686805969494));
#239746=CARTESIAN_POINT('Ctrl Pts',(2.87042944950575,-7.37463951888646,
31.2605663822263));
#239747=CARTESIAN_POINT('Ctrl Pts',(2.68132487568337,-7.44547470887926,
31.2524521675032));
#239748=CARTESIAN_POINT('Ctrl Pts',(2.48989240424191,-7.5089517787304,31.24433795278));
#239749=CARTESIAN_POINT('Ctrl Pts',(2.29836637358184,-7.57245987187143,
31.2362197723787));
#239750=CARTESIAN_POINT('Ctrl Pts',(2.10451048050494,-7.62860257782504,
31.2281015919773));
#239751=CARTESIAN_POINT('Ctrl Pts',(1.90892035503056,-7.67723544501209,
31.2199834115759));
#239752=CARTESIAN_POINT('Ctrl Pts',(1.71311989080711,-7.72592061226503,
31.2118565008365));
#239753=CARTESIAN_POINT('Ctrl Pts',(1.5155817785933,-7.76707973273538,31.2037295900971));
#239754=CARTESIAN_POINT('Ctrl Pts',(1.31691173377675,-7.80061949369671,
31.1956026793576));
#239755=CARTESIAN_POINT('Ctrl Pts',(1.21149661691418,-7.81841582441454,
31.1912905081588));
#239756=CARTESIAN_POINT('Ctrl Pts',(1.10576292376352,-7.83406787061175,
31.18697833696));
#239757=CARTESIAN_POINT('Ctrl Pts',(0.999801603749123,-7.84756763291281,
31.1826661657612));
#239758=CARTESIAN_POINT('Ctrl Pts',(0.803275035865438,-7.87260565576786,
31.1746683774577));
#239759=CARTESIAN_POINT('Ctrl Pts',(0.605624164434566,-7.89028031150178,
31.1666705891542));
#239760=CARTESIAN_POINT('Ctrl Pts',(0.407435973534077,-7.90050105546923,
31.1586728008507));
#239761=CARTESIAN_POINT('Ctrl Pts',(0.209409603049642,-7.91071345421169,
31.1506815427317));
#239762=CARTESIAN_POINT('Ctrl Pts',(0.0108471198679824,-7.91348405289138,
31.1426902846126));
#239763=CARTESIAN_POINT('Ctrl Pts',(-0.187658120185684,-7.90877395238531,
31.1346990264935));
#239764=CARTESIAN_POINT('Ctrl Pts',(-0.386034941989788,-7.90406689896688,
31.126712938129));
#239765=CARTESIAN_POINT('Ctrl Pts',(-0.584354261112515,-7.89188879974217,
31.1187268497645));
#239766=CARTESIAN_POINT('Ctrl Pts',(-0.78202104470825,-7.8722527960955,
31.1107407614));
#239767=CARTESIAN_POINT('Ctrl Pts',(-0.979593456904803,-7.85262616720115,
31.1027584858073));
#239768=CARTESIAN_POINT('Ctrl Pts',(-1.17651362232059,-7.82554876433088,
31.0947762102146));
#239769=CARTESIAN_POINT('Ctrl Pts',(-1.37218954246306,-7.7910857304714,
31.0867939346219));
#239770=CARTESIAN_POINT('Ctrl Pts',(-1.56780519770736,-7.75663331064774,
31.0788141174361));
#239771=CARTESIAN_POINT('Ctrl Pts',(-1.76217704252591,-7.71479985261514,
31.0708343002502));
#239772=CARTESIAN_POINT('Ctrl Pts',(-1.95472080065425,-7.66570202861353,
31.0628544830644));
#239773=CARTESIAN_POINT('Ctrl Pts',(-2.15388132751438,-7.61491695725678,
31.054600439358));
#239774=CARTESIAN_POINT('Ctrl Pts',(-2.35108552174003,-7.55635943088405,
31.0463463956517));
#239775=CARTESIAN_POINT('Ctrl Pts',(-2.54570046579419,-7.49021562696664,
31.0380923519453));
#239776=CARTESIAN_POINT('Ctrl Pts',(-2.73387510541626,-7.42626069007378,
31.0301114555788));
#239777=CARTESIAN_POINT('Ctrl Pts',(-2.91962879532448,-7.3552136682197,
31.0221305592123));
#239778=CARTESIAN_POINT('Ctrl Pts',(-3.10240674042604,-7.27729300062593,
31.0141496628458));
#239779=CARTESIAN_POINT('Ctrl Pts',(-3.28522526456568,-7.19935503364881,
31.0061669946183));
#239780=CARTESIAN_POINT('Ctrl Pts',(-3.46506641872656,-7.11454050960702,
30.9981843263909));
#239781=CARTESIAN_POINT('Ctrl Pts',(-3.64139680113664,-7.02311542954207,
30.9902016581635));
#239782=CARTESIAN_POINT('Ctrl Pts',(-3.81779343608521,-6.93165599837124,
30.9822159906116));
#239783=CARTESIAN_POINT('Ctrl Pts',(-3.99067637246239,-6.83358121347228,
30.9742303230596));
#239784=CARTESIAN_POINT('Ctrl Pts',(-4.15953782867062,-6.72920248260209,
30.9662446555077));
#239785=CARTESIAN_POINT('Ctrl Pts',(-4.32848869245094,-6.62476848601813,
30.9582547597609));
#239786=CARTESIAN_POINT('Ctrl Pts',(-4.49341354679249,-6.51402406493902,
30.9502648640141));
#239787=CARTESIAN_POINT('Ctrl Pts',(-4.65383423728175,-6.39732349439233,
30.9422749682673));
#239788=CARTESIAN_POINT('Ctrl Pts',(-4.81444495932278,-6.28048468238537,
30.9342756078293));
#239789=CARTESIAN_POINT('Ctrl Pts',(-4.97054058840902,-6.15767582334372,
30.9262762473914));
#239790=CARTESIAN_POINT('Ctrl Pts',(-5.12167568950783,-6.02929176035664,
30.9182768869534));
#239791=CARTESIAN_POINT('Ctrl Pts',(-5.27291644255949,-5.90081794967448,
30.9102719345117));
#239792=CARTESIAN_POINT('Ctrl Pts',(-5.4191895056411,-5.76676138739371,
30.9022669820701));
#239793=CARTESIAN_POINT('Ctrl Pts',(-5.56008652872081,-5.62755353534175,
30.8942620296284));
#239794=CARTESIAN_POINT('Ctrl Pts',(-5.70116743391328,-5.48816400568305,
30.8862466300705));
#239795=CARTESIAN_POINT('Ctrl Pts',(-5.83685805631752,-5.34361000062216,
30.8782312305126));
#239796=CARTESIAN_POINT('Ctrl Pts',(-5.96678975451033,-5.19435665173952,
30.8702158309548));
#239797=CARTESIAN_POINT('Ctrl Pts',(-5.99628376231048,-5.16047670175525,
30.8683963653404));
#239798=CARTESIAN_POINT('Ctrl Pts',(-6.02548120320849,-5.12635472781571,
30.866576899726));
#239799=CARTESIAN_POINT('Ctrl Pts',(-6.05437807709909,-5.09199637662302,
30.8647574341116));
#239800=CARTESIAN_POINT('Ctrl Pts',(-6.17670551434893,-4.94654918861768,
30.8570551973017));
#239801=CARTESIAN_POINT('Ctrl Pts',(-6.29402186928434,-4.79641363535212,
30.8493529604917));
#239802=CARTESIAN_POINT('Ctrl Pts',(-6.40593152587227,-4.64197827287416,
30.8416507236818));
#239803=CARTESIAN_POINT('Ctrl Pts',(-6.51769924070127,-4.48773879006967,
30.8339582560828));
#239804=CARTESIAN_POINT('Ctrl Pts',(-6.62407369436811,-4.3292106427767,
30.8262657884838));
#239805=CARTESIAN_POINT('Ctrl Pts',(-6.72469650293035,-4.16681868377739,
30.8185733208848));
#239806=CARTESIAN_POINT('Ctrl Pts',(-6.82518779454681,-4.00463897580518,
30.8108909075653));
#239807=CARTESIAN_POINT('Ctrl Pts',(-6.91994222679607,-3.83860582307059,
30.8032084942458));
#239808=CARTESIAN_POINT('Ctrl Pts',(-7.00864229111484,-3.66917623387001,
30.7955260809263));
#239809=CARTESIAN_POINT('Ctrl Pts',(-7.09727541642188,-3.49987450758978,
30.7878494652707));
#239810=CARTESIAN_POINT('Ctrl Pts',(-7.17986309738958,-3.32718176537128,
30.780172849615));
#239811=CARTESIAN_POINT('Ctrl Pts',(-7.25613136580334,-3.15158350709686,
30.7724962339594));
#239812=CARTESIAN_POINT('Ctrl Pts',(-7.33235639994112,-2.97608479039744,
30.7648239699552));
#239813=CARTESIAN_POINT('Ctrl Pts',(-7.4022690064745,-2.79768416835301,
30.757151705951));
#239814=CARTESIAN_POINT('Ctrl Pts',(-7.46564138949943,-2.61689121734033,
30.7494794419468));
#239815=CARTESIAN_POINT('Ctrl Pts',(-7.52898973886491,-2.43616683115052,
30.7418100876104));
#239816=CARTESIAN_POINT('Ctrl Pts',(-7.58580268248014,-2.25305226534913,
30.7341407332739));
#239817=CARTESIAN_POINT('Ctrl Pts',(-7.63590076839302,-2.06807651097701,
30.7264713789375));
#239818=CARTESIAN_POINT('Ctrl Pts',(-7.68599815158814,-1.88310335122995,
30.7188021321778));
#239819=CARTESIAN_POINT('Ctrl Pts',(-7.72938075927012,-1.69626940359867,
30.7111328854182));
#239820=CARTESIAN_POINT('Ctrl Pts',(-7.76591910683258,-1.50811850533461,
30.7034636386586));
#239821=CARTESIAN_POINT('Ctrl Pts',(-7.80245646267677,-1.31997271383357,
30.6957946000564));
#239822=CARTESIAN_POINT('Ctrl Pts',(-7.8321498640609,-1.13051040154314,
30.6881255614543));
#239823=CARTESIAN_POINT('Ctrl Pts',(-7.85492108572722,-0.940284923306739,
30.6804565228522));
#239824=CARTESIAN_POINT('Ctrl Pts',(-7.87770307273813,-0.749969513890778,
30.6727838586281));
#239825=CARTESIAN_POINT('Ctrl Pts',(-7.89355630427478,-0.558890580240167,
30.6651111944039));
#239826=CARTESIAN_POINT('Ctrl Pts',(-7.90245446202203,-0.367606414073757,
30.6574385301797));
#239827=CARTESIAN_POINT('Ctrl Pts',(-7.90829444408519,-0.242064011802341,
30.6524028561988));
#239828=CARTESIAN_POINT('Ctrl Pts',(-7.91113961314385,-0.11643327993427,
30.6473671822179));
#239829=CARTESIAN_POINT('Ctrl Pts',(-7.91099473374487,0.00912812472498083,
30.642331508237));
#239830=CARTESIAN_POINT('',(-7.92501410677892,-0.00343255291858106,28.642331508237));
#239831=CARTESIAN_POINT('Ctrl Pts',(-7.90633320911253,0.0091686610735674,
30.6423296657176));
#239832=CARTESIAN_POINT('Ctrl Pts',(-7.91336746977763,0.802296278954325,
30.6105026779658));
#239833=CARTESIAN_POINT('Ctrl Pts',(-7.44150124210029,4.22685934970188,
30.4727061129974));
#239834=CARTESIAN_POINT('Ctrl Pts',(-3.57838467684135,7.95204539560988,
30.2819247594207));
#239835=CARTESIAN_POINT('Ctrl Pts',(1.84890739308732,8.01686568835012,30.0699856049879));
#239836=CARTESIAN_POINT('Ctrl Pts',(6.72176570595038,5.56614746243324,29.8580464505547));
#239837=CARTESIAN_POINT('Ctrl Pts',(8.72502379230441,-0.0138583237335466,
29.6461072961218));
#239838=CARTESIAN_POINT('Ctrl Pts',(6.53049753724295,-5.01776157217315,
29.4341681416887));
#239839=CARTESIAN_POINT('Ctrl Pts',(3.34789267773502,-7.54374501772842,
29.2752137758639));
#239840=CARTESIAN_POINT('Ctrl Pts',(-0.668896594127559,-8.20840108341964,
29.1162594100393));
#239841=CARTESIAN_POINT('Ctrl Pts',(-5.81251715635164,-6.4871340805156,
28.9052986541635));
#239842=CARTESIAN_POINT('Ctrl Pts',(-7.92294825320361,-2.5984269134878,
28.7473226868962));
#239843=CARTESIAN_POINT('Ctrl Pts',(-7.92501410677892,-0.00343255291858106,
28.642331508237));
#239844=CARTESIAN_POINT('',(-7.911,-2.20934381900406E-13,24.642331508237));
#239845=CARTESIAN_POINT('Ctrl Pts',(-7.91099939187997,-0.00310188245014101,
28.6503955877365));
#239846=CARTESIAN_POINT('Ctrl Pts',(-7.91100069750583,0.000227968239218608,
28.6502613150879));
#239847=CARTESIAN_POINT('Ctrl Pts',(-7.91099990075837,0.0035578146403876,
28.6501269234759));
#239848=CARTESIAN_POINT('Ctrl Pts',(-7.91099372550141,0.0106505683740582,
28.6498404065745));
#239849=CARTESIAN_POINT('Ctrl Pts',(-7.91098776457367,0.0144134729226244,
28.649688248172));
#239850=CARTESIAN_POINT('Ctrl Pts',(-7.91097028956923,0.0220191955620909,
28.6493803880486));
#239851=CARTESIAN_POINT('Ctrl Pts',(-7.91095866021637,0.0258620120489566,
28.6492246797667));
#239852=CARTESIAN_POINT('Ctrl Pts',(-7.91092980626999,0.0335463549286024,
28.6489129912032));
#239853=CARTESIAN_POINT('Ctrl Pts',(-7.91091258351208,0.0373878802412497,
28.6487570110713));
#239854=CARTESIAN_POINT('Ctrl Pts',(-7.91086330887346,0.0468424567040657,
28.6483727184439));
#239855=CARTESIAN_POINT('Ctrl Pts',(-7.91082808115321,0.0524554816042823,
28.6481442216884));
#239856=CARTESIAN_POINT('Ctrl Pts',(-7.91066499237011,0.0746734089642306,
28.6472383724012));
#239857=CARTESIAN_POINT('Ctrl Pts',(-7.91049082701998,0.0912775885031617,
28.6465582915197));
#239858=CARTESIAN_POINT('Ctrl Pts',(-7.90633603099997,0.395923944287139,
28.6340247013134));
#239859=CARTESIAN_POINT('Ctrl Pts',(-7.88667765437492,0.68351374242021,
28.6212865391246));
#239860=CARTESIAN_POINT('Ctrl Pts',(-7.79356480844529,1.43768529788987,
28.5867060414319));
#239861=CARTESIAN_POINT('Ctrl Pts',(-7.69395872348861,1.89989813937944,
28.564366966351));
#239862=CARTESIAN_POINT('Ctrl Pts',(-7.47299284271564,2.61001391222413,
28.530404667836));
#239863=CARTESIAN_POINT('Ctrl Pts',(-7.37891251455699,2.86521594782051,
28.5182597392054));
#239864=CARTESIAN_POINT('Ctrl Pts',(-7.19952949890077,3.28396891102393,
28.4986198111455));
#239865=CARTESIAN_POINT('Ctrl Pts',(-7.12131958148455,3.45028848752972,
28.4908970527732));
#239866=CARTESIAN_POINT('Ctrl Pts',(-7.01483659852659,3.65765294324576,
28.4813718555403));
#239867=CARTESIAN_POINT('Ctrl Pts',(-6.99187752568665,3.70135196213072,
28.4793704019216));
#239868=CARTESIAN_POINT('Ctrl Pts',(-6.96249123284194,3.75603494812408,
28.476872918965));
#239869=CARTESIAN_POINT('Ctrl Pts',(-6.95644479396315,3.76722159284334,
28.4763623751625));
#239870=CARTESIAN_POINT('Ctrl Pts',(-6.94679207522196,3.78497781054658,
28.4755525886451));
#239871=CARTESIAN_POINT('Ctrl Pts',(-6.9432034003835,3.79155689711105,28.4752526719134));
#239872=CARTESIAN_POINT('Ctrl Pts',(-6.93643485370573,3.80392378079822,
28.4746891485306));
#239873=CARTESIAN_POINT('Ctrl Pts',(-6.93325707452281,3.80971271209514,
28.47442546189));
#239874=CARTESIAN_POINT('Ctrl Pts',(-6.92610911208688,3.82269552560342,
28.4738343116019));
#239875=CARTESIAN_POINT('Ctrl Pts',(-6.92213495926728,3.82988722030503,
28.4735070010147));
#239876=CARTESIAN_POINT('Ctrl Pts',(-6.91202366550362,3.84811763914778,
28.4726776711487));
#239877=CARTESIAN_POINT('Ctrl Pts',(-6.90587126957856,3.85914790170746,
28.4721762402867));
#239878=CARTESIAN_POINT('Ctrl Pts',(-6.87205461697762,3.91943592520712,
28.4694374658705));
#239879=CARTESIAN_POINT('Ctrl Pts',(-6.84388939434853,3.96841161772681,
28.4672195356385));
#239880=CARTESIAN_POINT('Ctrl Pts',(-6.31375551053387,4.86781301471811,
28.4266031238632));
#239881=CARTESIAN_POINT('Ctrl Pts',(-5.65763198849656,5.6169207411592,28.3961955078519));
#239882=CARTESIAN_POINT('Ctrl Pts',(-4.77148256975636,6.31158599312026,
28.3560885092999));
#239883=CARTESIAN_POINT('Ctrl Pts',(-4.66008259963891,6.39427798120392,
28.351033313477));
#239884=CARTESIAN_POINT('Ctrl Pts',(-4.47982046028401,6.5208728543024,28.34273272976));
#239885=CARTESIAN_POINT('Ctrl Pts',(-4.41235100523158,6.5667139369484,28.3396001284843));
#239886=CARTESIAN_POINT('Ctrl Pts',(-4.32160497183233,6.62633998329858,
28.3353352864027));
#239887=CARTESIAN_POINT('Ctrl Pts',(-4.29894738683064,6.64106184566675,
28.3342662304549));
#239888=CARTESIAN_POINT('Ctrl Pts',(-4.26619511427759,6.66210492949661,
28.3327141437806));
#239889=CARTESIAN_POINT('Ctrl Pts',(-4.25616066497755,6.66852001838038,
28.332237719767));
#239890=CARTESIAN_POINT('Ctrl Pts',(-4.24060053424063,6.67841828388974,
28.331497479866));
#239891=CARTESIAN_POINT('Ctrl Pts',(-4.23508492323408,6.68191734145765,
28.3312348027027));
#239892=CARTESIAN_POINT('Ctrl Pts',(-4.22477576473722,6.68843949326119,
28.3307432938459));
#239893=CARTESIAN_POINT('Ctrl Pts',(-4.21998328506552,6.69146427855042,
28.3305145844437));
#239894=CARTESIAN_POINT('Ctrl Pts',(-4.21225805610636,6.69632847559487,
28.3301455592729));
#239895=CARTESIAN_POINT('Ctrl Pts',(-4.20932736072825,6.69817110519297,
28.3300054810382));
#239896=CARTESIAN_POINT('Ctrl Pts',(-4.20321049616838,6.70201138966755,
28.3297129436406));
#239897=CARTESIAN_POINT('Ctrl Pts',(-4.20002411095955,6.70400869701049,
28.3295604594732));
#239898=CARTESIAN_POINT('Ctrl Pts',(-4.19265385197047,6.70862124597143,
28.3292075365407));
#239899=CARTESIAN_POINT('Ctrl Pts',(-4.18846895727958,6.71123484449945,
28.3290069803148));
#239900=CARTESIAN_POINT('Ctrl Pts',(-4.17502757636155,6.71961194097316,
28.3283623000814));
#239901=CARTESIAN_POINT('Ctrl Pts',(-4.16576165487082,6.72536019355585,
28.3279170975541));
#239902=CARTESIAN_POINT('Ctrl Pts',(-4.08255166408519,6.77674281183797,
28.3239122518502));
#239903=CARTESIAN_POINT('Ctrl Pts',(-4.00787495439204,6.82117353949541,
28.3202698307919));
#239904=CARTESIAN_POINT('Ctrl Pts',(-3.68396626654726,7.00673566293631,
28.3043184548576));
#239905=CARTESIAN_POINT('Ctrl Pts',(-3.42791732057716,7.13549647419334,
28.2913323050295));
#239906=CARTESIAN_POINT('Ctrl Pts',(-3.02332581642951,7.31214607335183,
28.2708728029163));
#239907=CARTESIAN_POINT('Ctrl Pts',(-2.87938443717211,7.37001513697177,
28.2636040263249));
#239908=CARTESIAN_POINT('Ctrl Pts',(-2.69194493070265,7.43904203987247,
28.2542205246128));
#239909=CARTESIAN_POINT('Ctrl Pts',(-2.64992268633678,7.45411455049617,
28.2521219780601));
#239910=CARTESIAN_POINT('Ctrl Pts',(-2.55986721172178,7.48555781691231,
28.247638093769));
#239911=CARTESIAN_POINT('Ctrl Pts',(-2.51179939178841,7.50182376477952,
28.2452528610037));
#239912=CARTESIAN_POINT('Ctrl Pts',(-2.40804899529163,7.53582349122296,
28.2401251985732));
#239913=CARTESIAN_POINT('Ctrl Pts',(-2.35231952535368,7.55340509646899,
28.2373835780121));
#239914=CARTESIAN_POINT('Ctrl Pts',(-2.23080304102068,7.590265984888,28.2314377861457));
#239915=CARTESIAN_POINT('Ctrl Pts',(-2.16494959868516,7.60931096031932,
28.2282359341819));
#239916=CARTESIAN_POINT('Ctrl Pts',(-2.01905068141353,7.64945792625273,
28.2211938629336));
#239917=CARTESIAN_POINT('Ctrl Pts',(-1.93890422734654,7.6701644660312,28.2173594750244));
#239918=CARTESIAN_POINT('Ctrl Pts',(-1.57656917404609,7.75773462790546,
28.2001981828266));
#239919=CARTESIAN_POINT('Ctrl Pts',(-1.29114372364367,7.81031283063245,
28.1871621729531));
#239920=CARTESIAN_POINT('Ctrl Pts',(-0.845272370409721,7.86732907906118,
28.1677053388765));
#239921=CARTESIAN_POINT('Ctrl Pts',(-0.686507738654565,7.88277003708533,
28.1609501978895));
#239922=CARTESIAN_POINT('Ctrl Pts',(-0.445220905622621,7.89889101406481,
28.1509437282521));
#239923=CARTESIAN_POINT('Ctrl Pts',(-0.362981612354909,7.90309722944765,
28.1475785115249));
#239924=CARTESIAN_POINT('Ctrl Pts',(-0.265322876925592,7.90656443802844,
28.1436342470231));
#239925=CARTESIAN_POINT('Ctrl Pts',(-0.249954281716337,7.90706521424777,
28.1430150582266));
#239926=CARTESIAN_POINT('Ctrl Pts',(-0.226305744770819,7.90776677097254,
28.1420645967093));
#239927=CARTESIAN_POINT('Ctrl Pts',(-0.218026827105749,7.90799936124399,
28.1417322949427));
#239928=CARTESIAN_POINT('Ctrl Pts',(-0.202942505682139,7.90839943860257,
28.1411276282901));
#239929=CARTESIAN_POINT('Ctrl Pts',(-0.196137227451665,7.90857114334941,
28.1408551273204));
#239930=CARTESIAN_POINT('Ctrl Pts',(-0.181315439582044,7.90892597063747,
28.1402622615986));
#239931=CARTESIAN_POINT('Ctrl Pts',(-0.173298851774147,7.90910568940206,
28.1399420070591));
#239932=CARTESIAN_POINT('Ctrl Pts',(-0.151489154864978,7.90956145189505,
28.1390718297102));
#239933=CARTESIAN_POINT('Ctrl Pts',(-0.137695544958028,7.90981360493365,
28.1385226779377));
#239934=CARTESIAN_POINT('Ctrl Pts',(-0.0720454124986548,7.91084193694461,
28.1359146394308));
#239935=CARTESIAN_POINT('Ctrl Pts',(-0.0201821841223189,7.91114426013311,
28.1338710242911));
#239936=CARTESIAN_POINT('Ctrl Pts',(0.889310074192833,7.90750201682776,
28.0983136759724));
#239937=CARTESIAN_POINT('Ctrl Pts',(1.74055375587961,7.76465212691922,28.0702090047863));
#239938=CARTESIAN_POINT('Ctrl Pts',(2.87982968575234,7.37633129990284,28.0277447212724));
#239939=CARTESIAN_POINT('Ctrl Pts',(3.19971383537684,7.24330910870905,28.0150769246642));
#239940=CARTESIAN_POINT('Ctrl Pts',(3.52884280033714,7.08036987832201,28.000421018349));
#239941=CARTESIAN_POINT('Ctrl Pts',(3.5477762884037,7.07090181794877,27.9995727016386));
#239942=CARTESIAN_POINT('Ctrl Pts',(3.57431102841773,7.05749919770662,27.9983766604006));
#239943=CARTESIAN_POINT('Ctrl Pts',(3.58194434888166,7.05362806889196,27.9980317579995));
#239944=CARTESIAN_POINT('Ctrl Pts',(3.59495913966229,7.04700123019173,27.9974422916614));
#239945=CARTESIAN_POINT('Ctrl Pts',(3.60034377055346,7.0442517195044,27.997197998491));
#239946=CARTESIAN_POINT('Ctrl Pts',(3.61058757890795,7.0390061924101,27.9967324720837));
#239947=CARTESIAN_POINT('Ctrl Pts',(3.61544733526907,7.03651130941019,27.9965112877436));
#239948=CARTESIAN_POINT('Ctrl Pts',(3.62754904745606,7.03028273220812,27.9959596693016));
#239949=CARTESIAN_POINT('Ctrl Pts',(3.63478781743424,7.02654288452659,27.9956289734115));
#239950=CARTESIAN_POINT('Ctrl Pts',(3.65842088096235,7.01428677469717,27.9945469285674));
#239951=CARTESIAN_POINT('Ctrl Pts',(3.67479105506096,7.00572430192148,27.9937936496346));
#239952=CARTESIAN_POINT('Ctrl Pts',(3.88328972352501,6.89573653676422,27.9841525100428));
#239953=CARTESIAN_POINT('Ctrl Pts',(4.07118341144484,6.78649975393642,27.9749558601663));
#239954=CARTESIAN_POINT('Ctrl Pts',(4.30261350486665,6.63887921920449,27.9631400393756));
#239955=CARTESIAN_POINT('Ctrl Pts',(4.35055670117626,6.60756056031079,27.960664578983));
#239956=CARTESIAN_POINT('Ctrl Pts',(4.55366275659396,6.47171362983408,27.9500676087089));
#239957=CARTESIAN_POINT('Ctrl Pts',(4.70543037963849,6.36222017369908,27.9418736171299));
#239958=CARTESIAN_POINT('Ctrl Pts',(4.99867963181355,6.13441700950387,27.9256026940386));
#239959=CARTESIAN_POINT('Ctrl Pts',(5.14019499050633,6.01633331953407,27.9175307793291));
#239960=CARTESIAN_POINT('Ctrl Pts',(5.38352493741036,5.79843526414609,27.9033205736802));
#239961=CARTESIAN_POINT('Ctrl Pts',(5.48700882673113,5.70060764310326,27.8971619471324));
#239962=CARTESIAN_POINT('Ctrl Pts',(5.83170193321483,5.35666803760051,27.8762779111186));
#239963=CARTESIAN_POINT('Ctrl Pts',(6.05945537562609,5.09761339391123,27.8618454937884));
#239964=CARTESIAN_POINT('Ctrl Pts',(6.30974284918697,4.77235775333514,27.8451284060405));
#239965=CARTESIAN_POINT('Ctrl Pts',(6.34923124628318,4.71969448759089,27.8424616701445));
#239966=CARTESIAN_POINT('Ctrl Pts',(6.40085069594386,4.64903233855344,27.8389346455726));
#239967=CARTESIAN_POINT('Ctrl Pts',(6.41357127967324,4.63146788422882,27.8380620939076));
#239968=CARTESIAN_POINT('Ctrl Pts',(6.4342586784555,4.6026542625308,27.8366375130033));
#239969=CARTESIAN_POINT('Ctrl Pts',(6.44226857953668,4.59143621889701,27.8360845528981));
#239970=CARTESIAN_POINT('Ctrl Pts',(6.45768930546228,4.56971935430552,27.8350173152911));
#239971=CARTESIAN_POINT('Ctrl Pts',(6.46510394679604,4.55922330022064,27.8345029554047));
#239972=CARTESIAN_POINT('Ctrl Pts',(6.48211518649803,4.53501750364098,27.8333200830842));
#239973=CARTESIAN_POINT('Ctrl Pts',(6.49169393295344,4.52129527157791,27.8326519664111));
#239974=CARTESIAN_POINT('Ctrl Pts',(6.52133881547096,4.47853845602889,27.8305777998808));
#239975=CARTESIAN_POINT('Ctrl Pts',(6.54125431669742,4.44939980640473,27.8291751185168));
#239976=CARTESIAN_POINT('Ctrl Pts',(6.72601630461986,4.17515018047701,27.8160741977128));
#239977=CARTESIAN_POINT('Ctrl Pts',(6.87721269275172,3.92111378965817,27.8047042179514));
#239978=CARTESIAN_POINT('Ctrl Pts',(7.23137641049123,3.24226353805426,27.7759364261887));
#239979=CARTESIAN_POINT('Ctrl Pts',(7.41128504969639,2.80676536531833,27.7590609056798));
#239980=CARTESIAN_POINT('Ctrl Pts',(7.6103324652913,2.16928357363508,27.7346436666831));
#239981=CARTESIAN_POINT('Ctrl Pts',(7.66212917370045,1.97856616625083,27.727360824489));
#239982=CARTESIAN_POINT('Ctrl Pts',(7.73347120397359,1.67073959523631,27.7154092046737));
#239983=CARTESIAN_POINT('Ctrl Pts',(7.75761585171015,1.55478050873955,27.710862680265));
#239984=CARTESIAN_POINT('Ctrl Pts',(7.7896233363017,1.38166895679634,27.7039578000215));
#239985=CARTESIAN_POINT('Ctrl Pts',(7.7994795879539,1.3248995266088,27.7016747728488));
#239986=CARTESIAN_POINT('Ctrl Pts',(7.81051183161563,1.25696127301639,27.6989152843981));
#239987=CARTESIAN_POINT('Ctrl Pts',(7.81228546354891,1.24589026315899,27.6984647424382));
#239988=CARTESIAN_POINT('Ctrl Pts',(7.8149880761139,1.22878786235243,27.6977673663296));
#239989=CARTESIAN_POINT('Ctrl Pts',(7.81593362837821,1.22275907559367,27.6975212683163));
#239990=CARTESIAN_POINT('Ctrl Pts',(7.81757444252269,1.21221767136442,27.6970904906555));
#239991=CARTESIAN_POINT('Ctrl Pts',(7.81827277608412,1.20770552940837,27.6969059493699));
#239992=CARTESIAN_POINT('Ctrl Pts',(7.81982717575409,1.19760423881393,27.6964924752013));
#239993=CARTESIAN_POINT('Ctrl Pts',(7.82068115612301,1.19201477570479,27.6962634476173));
#239994=CARTESIAN_POINT('Ctrl Pts',(7.82292447625388,1.17722563820278,27.6956568316467));
#239995=CARTESIAN_POINT('Ctrl Pts',(7.82430357745864,1.16802443940177,27.6952787723308));
#239996=CARTESIAN_POINT('Ctrl Pts',(7.8301579471061,1.12848912754554,27.6936514842474));
#239997=CARTESIAN_POINT('Ctrl Pts',(7.83447303613741,1.09813177915668,27.6923947362356));
#239998=CARTESIAN_POINT('Ctrl Pts',(7.90005308046722,0.616692937639541,
27.6723391194829));
#239999=CARTESIAN_POINT('Ctrl Pts',(7.92244177925405,0.161212538544038,
27.6516666678638));
#240000=CARTESIAN_POINT('Ctrl Pts',(7.88794912182902,-0.767502434094909,
27.6089087074514));
#240001=CARTESIAN_POINT('Ctrl Pts',(7.82777272970739,-1.23888115495861,
27.586914023236));
#240002=CARTESIAN_POINT('Ctrl Pts',(7.70578328661029,-1.79260254353746,
27.561801987866));
#240003=CARTESIAN_POINT('Ctrl Pts',(7.6842413581143,-1.88280517663804,27.5577321030192));
#240004=CARTESIAN_POINT('Ctrl Pts',(7.61629433043974,-2.14669424541121,
27.5458953573642));
#240005=CARTESIAN_POINT('Ctrl Pts',(7.56554840994925,-2.31920633322945,
27.5382481571461));
#240006=CARTESIAN_POINT('Ctrl Pts',(7.47872827294973,-2.58104149531858,
27.5267894275504));
#240007=CARTESIAN_POINT('Ctrl Pts',(7.44683034956438,-2.67167931200832,
27.5228503468896));
#240008=CARTESIAN_POINT('Ctrl Pts',(7.40734466260113,-2.77767095780826,
27.518274687283));
#240009=CARTESIAN_POINT('Ctrl Pts',(7.40134923865544,-2.79360705046267,
27.5175875461814));
#240010=CARTESIAN_POINT('Ctrl Pts',(7.39208419796691,-2.81799473472111,
27.5165372208217));
#240011=CARTESIAN_POINT('Ctrl Pts',(7.38885144732317,-2.82646022523184,
27.5161728590177));
#240012=CARTESIAN_POINT('Ctrl Pts',(7.38292997659567,-2.84188698729883,
27.5155092913804));
#240013=CARTESIAN_POINT('Ctrl Pts',(7.38024594061698,-2.84885003892416,
27.5152099360156));
#240014=CARTESIAN_POINT('Ctrl Pts',(7.37442223215794,-2.86389471028146,
27.514563465398));
#240015=CARTESIAN_POINT('Ctrl Pts',(7.37127911684671,-2.87197499150922,
27.5142164610236));
#240016=CARTESIAN_POINT('Ctrl Pts',(7.36272382273786,-2.89386226936205,
27.5132770731304));
#240017=CARTESIAN_POINT('Ctrl Pts',(7.35728608196858,-2.90765927078222,
27.5126855112933));
#240018=CARTESIAN_POINT('Ctrl Pts',(7.33154433578997,-2.97243840514617,
27.5099107843658));
#240019=CARTESIAN_POINT('Ctrl Pts',(7.31074879325445,-3.02322421407497,
27.5077434782227));
#240020=CARTESIAN_POINT('Ctrl Pts',(6.9476543563465,-3.88429474074423,27.4711220894172));
#240021=CARTESIAN_POINT('Ctrl Pts',(6.47315210377507,-4.63205170740908,
27.4420193411361));
#240022=CARTESIAN_POINT('Ctrl Pts',(5.61792701522823,-5.58417432911609,
27.397134420406));
#240023=CARTESIAN_POINT('Ctrl Pts',(5.32826474102179,-5.86120416465559,
27.3826192214403));
#240024=CARTESIAN_POINT('Ctrl Pts',(5.00548171015029,-6.12612227622994,
27.3659543503292));
#240025=CARTESIAN_POINT('Ctrl Pts',(4.99205054272018,-6.1370719945937,27.3652605393221));
#240026=CARTESIAN_POINT('Ctrl Pts',(4.97232073780811,-6.15304903479525,
27.3642409358957));
#240027=CARTESIAN_POINT('Ctrl Pts',(4.96605016825652,-6.15811104722852,
27.3639168207194));
#240028=CARTESIAN_POINT('Ctrl Pts',(4.95508593623094,-6.16693445263731,
27.3633500037873));
#240029=CARTESIAN_POINT('Ctrl Pts',(4.95039569180073,-6.17070009584951,
27.3631075026071));
#240030=CARTESIAN_POINT('Ctrl Pts',(4.94070029229818,-6.17846604553034,
27.3626061636518));
#240031=CARTESIAN_POINT('Ctrl Pts',(4.93569456348985,-6.18246562705647,
27.3623472926453));
#240032=CARTESIAN_POINT('Ctrl Pts',(4.92304151301149,-6.19255026388212,
27.3616928757877));
#240033=CARTESIAN_POINT('Ctrl Pts',(4.91538777538602,-6.19862722916318,
27.3612969639971));
#240034=CARTESIAN_POINT('Ctrl Pts',(4.88651731079452,-6.22146289674119,
27.3598033866403));
#240035=CARTESIAN_POINT('Ctrl Pts',(4.86522610182895,-6.23812687928477,
27.3587015707564));
#240036=CARTESIAN_POINT('Ctrl Pts',(4.7235934993176,-6.3478122585053,27.3513719085748));
#240037=CARTESIAN_POINT('Ctrl Pts',(4.60067922769253,-6.43745322224898,
27.3450107756092));
#240038=CARTESIAN_POINT('Ctrl Pts',(3.9360669171789,-6.89339211330293,27.3108767433396));
#240039=CARTESIAN_POINT('Ctrl Pts',(3.35307889087473,-7.19502786354673,
27.2821516336935));
#240040=CARTESIAN_POINT('Ctrl Pts',(2.26597366979905,-7.59632626646408,
27.2333002017464));
#240041=CARTESIAN_POINT('Ctrl Pts',(1.77669114644166,-7.72542560950767,
27.2126610815678));
#240042=CARTESIAN_POINT('Ctrl Pts',(1.21024481498384,-7.8181841746075,27.1893957300751));
#240043=CARTESIAN_POINT('Ctrl Pts',(1.14190591260103,-7.82845752778553,
27.1866013212568));
#240044=CARTESIAN_POINT('Ctrl Pts',(1.04195581519104,-7.84214632516268,
27.1825324351451));
#240045=CARTESIAN_POINT('Ctrl Pts',(1.0104449481947,-7.84626866229335,27.1812522692178));
#240046=CARTESIAN_POINT('Ctrl Pts',(0.954781625108807,-7.85320980754346,
27.1789954539141));
#240047=CARTESIAN_POINT('Ctrl Pts',(0.930639433645672,-7.85610733641379,
27.1780181473124));
#240048=CARTESIAN_POINT('Ctrl Pts',(0.883385639279105,-7.86155782626504,
27.1761081845053));
#240049=CARTESIAN_POINT('Ctrl Pts',(0.860275379822527,-7.86412028885816,
27.1751754544352));
#240050=CARTESIAN_POINT('Ctrl Pts',(0.79753688709894,-7.87079686016875,
27.1726469927131));
#240051=CARTESIAN_POINT('Ctrl Pts',(0.757888261979526,-7.87471356304108,
27.171053053983));
#240052=CARTESIAN_POINT('Ctrl Pts',(0.605608998775533,-7.88859578560043,
27.1649459215727));
#240053=CARTESIAN_POINT('Ctrl Pts',(0.492798413333528,-7.89644577318701,
27.1604527576214));
#240054=CARTESIAN_POINT('Ctrl Pts',(0.302136363620833,-7.90561124475939,
27.1529038368206));
#240055=CARTESIAN_POINT('Ctrl Pts',(0.224363953506112,-7.90820058383713,
27.1498371403737));
#240056=CARTESIAN_POINT('Ctrl Pts',(-0.513661300400068,-7.92187618780069,
27.1208349444013));
#240057=CARTESIAN_POINT('Ctrl Pts',(-1.17280383165529,-7.85139858238789,
27.0958899741146));
#240058=CARTESIAN_POINT('Ctrl Pts',(-1.90840247602796,-7.67795765219672,
27.066060416114));
#240059=CARTESIAN_POINT('Ctrl Pts',(-2.00091005091787,-7.65437079275459,
27.0622678420703));
#240060=CARTESIAN_POINT('Ctrl Pts',(-2.11304730774199,-7.62360712828126,
27.0576056288537));
#240061=CARTESIAN_POINT('Ctrl Pts',(-2.13310584498613,-7.61801903512717,
27.056769127253));
#240062=CARTESIAN_POINT('Ctrl Pts',(-2.16445974210661,-7.60915063350176,
27.0554573841175));
#240063=CARTESIAN_POINT('Ctrl Pts',(-2.17577028932236,-7.60592420324783,
27.0549833328181));
#240064=CARTESIAN_POINT('Ctrl Pts',(-2.19676285101964,-7.59988523779251,
27.0541018532935));
#240065=CARTESIAN_POINT('Ctrl Pts',(-2.20644677106315,-7.59707939256954,
27.0536945783104));
#240066=CARTESIAN_POINT('Ctrl Pts',(-2.22784103102108,-7.59083620477417,
27.0527933419118));
#240067=CARTESIAN_POINT('Ctrl Pts',(-2.23954882583235,-7.5873902629724,
27.0522991798805));
#240068=CARTESIAN_POINT('Ctrl Pts',(-2.27333823279566,-7.57736004352931,
27.0508701217227));
#240069=CARTESIAN_POINT('Ctrl Pts',(-2.29539894767959,-7.57070641398238,
27.04993351194));
#240070=CARTESIAN_POINT('Ctrl Pts',(-2.47229480477882,-7.51650940813083,
27.0423951007361));
#240071=CARTESIAN_POINT('Ctrl Pts',(-2.62566279256396,-7.46431832394128,
27.0356873226902));
#240072=CARTESIAN_POINT('Ctrl Pts',(-3.22788148345043,-7.23852530562619,
27.0088253168393));
#240073=CARTESIAN_POINT('Ctrl Pts',(-3.66209650357547,-7.02883565103473,
26.9883448860614));
#240074=CARTESIAN_POINT('Ctrl Pts',(-4.22296367476717,-6.69182120773536,
26.9610970086187));
#240075=CARTESIAN_POINT('Ctrl Pts',(-4.36839439778994,-6.59780459234992,
26.9539441038624));
#240076=CARTESIAN_POINT('Ctrl Pts',(-4.59960920893525,-6.43733239431023,
26.9424241406506));
#240077=CARTESIAN_POINT('Ctrl Pts',(-4.68731619086642,-6.37375247603161,
26.9380175595952));
#240078=CARTESIAN_POINT('Ctrl Pts',(-4.80065776835905,-6.28798454442269,
26.9322697292135));
#240079=CARTESIAN_POINT('Ctrl Pts',(-4.82749367379495,-6.26740532304475,
26.9309047760873));
#240080=CARTESIAN_POINT('Ctrl Pts',(-4.87123570090996,-6.23341394281793,
26.9286730362737));
#240081=CARTESIAN_POINT('Ctrl Pts',(-4.8882203086831,-6.22010360474032,
26.9278047513385));
#240082=CARTESIAN_POINT('Ctrl Pts',(-4.92101901566706,-6.19418291149676,
26.9261245897198));
#240083=CARTESIAN_POINT('Ctrl Pts',(-4.93683962822205,-6.18158107459217,
26.9253125950674));
#240084=CARTESIAN_POINT('Ctrl Pts',(-4.97333466322978,-6.15228165452778,
26.9234357721402));
#240085=CARTESIAN_POINT('Ctrl Pts',(-4.99397364343534,-6.13554027647342,
26.922371598295));
#240086=CARTESIAN_POINT('Ctrl Pts',(-5.06074754575701,-6.08081625645618,
26.9189192799987));
#240087=CARTESIAN_POINT('Ctrl Pts',(-5.10653670357011,-6.04241466888241,
26.9165372834474));
#240088=CARTESIAN_POINT('Ctrl Pts',(-5.48073507461986,-5.72129727413463,
26.8969392517743));
#240089=CARTESIAN_POINT('Ctrl Pts',(-5.78585522984609,-5.41254083981036,
26.8800300446694));
#240090=CARTESIAN_POINT('Ctrl Pts',(-6.11997531801542,-5.01371911638406,
26.859991588568));
#240091=CARTESIAN_POINT('Ctrl Pts',(-6.17469694995096,-4.94616973211665,
26.8566566265284));
#240092=CARTESIAN_POINT('Ctrl Pts',(-6.55640491701762,-4.45877318992151,
26.8329965411742));
#240093=CARTESIAN_POINT('Ctrl Pts',(-6.84140072411021,-4.00778435727092,
26.8133260798258));
#240094=CARTESIAN_POINT('Ctrl Pts',(-7.18377333489709,-3.32151283187578,
26.7844826260153));
#240095=CARTESIAN_POINT('Ctrl Pts',(-7.27917941520453,-3.1068613735164,
26.7755791547357));
#240096=CARTESIAN_POINT('Ctrl Pts',(-7.40058591975522,-2.79728532262134,
26.7626154389189));
#240097=CARTESIAN_POINT('Ctrl Pts',(-7.43458566182813,-2.70562606258487,
26.7587617960729));
#240098=CARTESIAN_POINT('Ctrl Pts',(-7.47208565803646,-2.59848138100245,
26.7542198530485));
#240099=CARTESIAN_POINT('Ctrl Pts',(-7.47724938449326,-2.58358495248393,
26.7535875511159));
#240100=CARTESIAN_POINT('Ctrl Pts',(-7.48504434582995,-2.56087876614334,
26.7526223759556));
#240101=CARTESIAN_POINT('Ctrl Pts',(-7.48770797918858,-2.553080126387,26.7522906313868));
#240102=CARTESIAN_POINT('Ctrl Pts',(-7.49251902831954,-2.53892194944552,
26.7516878934578));
#240103=CARTESIAN_POINT('Ctrl Pts',(-7.49467054710605,-2.53256380869944,
26.751417046023));
#240104=CARTESIAN_POINT('Ctrl Pts',(-7.49927832456228,-2.51888966964696,
26.7508341692596));
#240105=CARTESIAN_POINT('Ctrl Pts',(-7.50173197396476,-2.51157280352617,
26.7505220462804));
#240106=CARTESIAN_POINT('Ctrl Pts',(-7.50829264793326,-2.49191326541878,
26.7496827613901));
#240107=CARTESIAN_POINT('Ctrl Pts',(-7.51237993343311,-2.47956406304294,
26.7491548766488));
#240108=CARTESIAN_POINT('Ctrl Pts',(-7.53087234844916,-2.42322619320042,
26.7467433192638));
#240109=CARTESIAN_POINT('Ctrl Pts',(-7.5449215185686,-2.37912224858076,
26.7448462473919));
#240110=CARTESIAN_POINT('Ctrl Pts',(-7.79195640446019,-1.57941559712661,
26.7102474342051));
#240111=CARTESIAN_POINT('Ctrl Pts',(-7.91071778081479,-0.793331051394151,
26.6724337110449));
#240112=CARTESIAN_POINT('Ctrl Pts',(-7.91115323352253,0.428571442726039,
26.6176012636813));
#240113=CARTESIAN_POINT('Ctrl Pts',(-7.87602182063576,0.859285952645077,
26.5989630286065));
#240114=CARTESIAN_POINT('Ctrl Pts',(-7.8013956521794,1.31260341219004,26.5803038022687));
#240115=CARTESIAN_POINT('Ctrl Pts',(-7.796710534783,1.3401517441448,26.5791734450176));
#240116=CARTESIAN_POINT('Ctrl Pts',(-7.79014045727208,1.37758260871179,
26.577642393961));
#240117=CARTESIAN_POINT('Ctrl Pts',(-7.7883824932134,1.38748705514272,26.5772377261131));
#240118=CARTESIAN_POINT('Ctrl Pts',(-7.78536810985002,1.40428397343252,
26.5765522244372));
#240119=CARTESIAN_POINT('Ctrl Pts',(-7.78412141900727,1.41117816678409,
26.57627108558));
#240120=CARTESIAN_POINT('Ctrl Pts',(-7.78170024028225,1.4244664382731,26.5757296268643));
#240121=CARTESIAN_POINT('Ctrl Pts',(-7.78052702603791,1.4308607412084,26.5754692672213));
#240122=CARTESIAN_POINT('Ctrl Pts',(-7.77773672550261,1.44596365213746,
26.5748547619746));
#240123=CARTESIAN_POINT('Ctrl Pts',(-7.77611289134087,1.45467101308581,
26.5745008290344));
#240124=CARTESIAN_POINT('Ctrl Pts',(-7.77132358543822,1.48011515408911,
26.5734676074171));
#240125=CARTESIAN_POINT('Ctrl Pts',(-7.76811866960463,1.49684450712406,
26.5727895627329));
#240126=CARTESIAN_POINT('Ctrl Pts',(-7.74440299081455,1.6185103149424,26.5678677109966));
#240127=CARTESIAN_POINT('Ctrl Pts',(-7.7218202765575,1.72303396548536,26.5636898858591));
#240128=CARTESIAN_POINT('Ctrl Pts',(-7.64260808230237,2.05674095974465,
26.5504972332984));
#240129=CARTESIAN_POINT('Ctrl Pts',(-7.57783716017767,2.28386416534251,
26.541744589189));
#240130=CARTESIAN_POINT('Ctrl Pts',(-7.29347674395331,3.13464536068801,
26.509439043966));
#240131=CARTESIAN_POINT('Ctrl Pts',(-7.0062335019558,3.73275205311661,26.4879507496564));
#240132=CARTESIAN_POINT('Ctrl Pts',(-6.49866984652717,4.51963317915568,
26.4551303542329));
#240133=CARTESIAN_POINT('Ctrl Pts',(-6.33738410007175,4.74313564605484,
26.4451699102142));
#240134=CARTESIAN_POINT('Ctrl Pts',(-6.1203941954405,5.0129545588054,26.431761006296));
#240135=CARTESIAN_POINT('Ctrl Pts',(-6.07526472610776,5.06755330212035,
26.4289716620884));
#240136=CARTESIAN_POINT('Ctrl Pts',(-6.02252159938466,5.12964597027968,
26.4257022383939));
#240137=CARTESIAN_POINT('Ctrl Pts',(-6.0156174334469,5.13774085448112,26.4252740818744));
#240138=CARTESIAN_POINT('Ctrl Pts',(-6.00542409335878,5.14964346107971,
26.4246416419693));
#240139=CARTESIAN_POINT('Ctrl Pts',(-6.00214755812901,5.15346204095446,
26.4244383046035));
#240140=CARTESIAN_POINT('Ctrl Pts',(-5.99630559980613,5.16025731876955,
26.4240756726765));
#240141=CARTESIAN_POINT('Ctrl Pts',(-5.99374159486631,5.16323523927039,
26.4239164853653));
#240142=CARTESIAN_POINT('Ctrl Pts',(-5.98838367736504,5.16944873343351,
26.4235837713961));
#240143=CARTESIAN_POINT('Ctrl Pts',(-5.98558935970127,5.17268395437235,
26.4234102138374));
#240144=CARTESIAN_POINT('Ctrl Pts',(-5.97831889980753,5.18108780884048,
26.4229585384681));
#240145=CARTESIAN_POINT('Ctrl Pts',(-5.97383868510563,5.18625289727279,
26.4226801073904));
#240146=CARTESIAN_POINT('Ctrl Pts',(-5.95413400648279,5.20891034676229,
26.4214550601818));
#240147=CARTESIAN_POINT('Ctrl Pts',(-5.93883967053494,5.22634117666884,
26.4205029479036));
#240148=CARTESIAN_POINT('Ctrl Pts',(-5.82563916825739,5.35421636913377,
26.4134484972194));
#240149=CARTESIAN_POINT('Ctrl Pts',(-5.72474082912931,5.46196321994297,
26.4071206215268));
#240150=CARTESIAN_POINT('Ctrl Pts',(-5.35545475970595,5.83483650152617,
26.384051665594));
#240151=CARTESIAN_POINT('Ctrl Pts',(-5.07119699638799,6.08351455379554,
26.366480565096));
#240152=CARTESIAN_POINT('Ctrl Pts',(-4.62748775459407,6.41890386143699,
26.3406119496773));
#240153=CARTESIAN_POINT('Ctrl Pts',(-4.48104928751347,6.52197583467332,
26.3322947385368));
#240154=CARTESIAN_POINT('Ctrl Pts',(-4.13640591247933,6.74746441238821,
26.3133645062173));
#240155=CARTESIAN_POINT('Ctrl Pts',(-3.9360333499996,6.86627854841027,26.3028240628792));
#240156=CARTESIAN_POINT('Ctrl Pts',(-3.64585238949148,7.02146280099603,
26.28832383032));
#240157=CARTESIAN_POINT('Ctrl Pts',(-3.56017993803925,7.06528832928464,
26.2841321990931));
#240158=CARTESIAN_POINT('Ctrl Pts',(-3.28468301116491,7.19993421645528,
26.2709448387543));
#240159=CARTESIAN_POINT('Ctrl Pts',(-3.09201949013388,7.28475259347493,
26.2621591220722));
#240160=CARTESIAN_POINT('Ctrl Pts',(-2.87698347807668,7.36934957183451,
26.2528226897495));
#240161=CARTESIAN_POINT('Ctrl Pts',(-2.85774597391413,7.37683095933883,
26.2519914478159));
#240162=CARTESIAN_POINT('Ctrl Pts',(-2.83062494197478,7.38725620541511,
26.2508251683409));
#240163=CARTESIAN_POINT('Ctrl Pts',(-2.82276574945083,7.39026287292216,
26.2504878620272));
#240164=CARTESIAN_POINT('Ctrl Pts',(-2.80909707415674,7.39546707157249,
26.2499023648688));
#240165=CARTESIAN_POINT('Ctrl Pts',(-2.80328978017355,7.39767030810257,
26.2496539682316));
#240166=CARTESIAN_POINT('Ctrl Pts',(-2.79118048021438,7.4022481639531,26.2491367599536));
#240167=CARTESIAN_POINT('Ctrl Pts',(-2.78487802287419,7.40462158060136,
26.2488679918123));
#240168=CARTESIAN_POINT('Ctrl Pts',(-2.76999458486316,7.41020478363784,
26.2482342770542));
#240169=CARTESIAN_POINT('Ctrl Pts',(-2.7614110349545,7.41340772063927,26.2478695773413));
#240170=CARTESIAN_POINT('Ctrl Pts',(-2.7331826597784,7.42388526217052,26.2466727410348));
#240171=CARTESIAN_POINT('Ctrl Pts',(-2.71351442084337,7.43109677872282,
26.245842873794));
#240172=CARTESIAN_POINT('Ctrl Pts',(-2.33321914023445,7.56882391637849,
26.2298740519594));
#240173=CARTESIAN_POINT('Ctrl Pts',(-1.96358772280067,7.6730289495587,26.2157282373308));
#240174=CARTESIAN_POINT('Ctrl Pts',(-1.10543592251756,7.84884663629935,
26.1848831318124));
#240175=CARTESIAN_POINT('Ctrl Pts',(-0.614898182543244,7.90242192526621,
26.1686941642928));
#240176=CARTESIAN_POINT('Ctrl Pts',(0.270674092557271,7.9161436271238,26.1383674843764));
#240177=CARTESIAN_POINT('Ctrl Pts',(0.663780681655991,7.89290336375354,
26.1244810596426));
#240178=CARTESIAN_POINT('Ctrl Pts',(1.07782696147844,7.83727079501794,26.1079073636825));
#240179=CARTESIAN_POINT('Ctrl Pts',(1.10215822685561,7.83388611670848,26.1069261417326));
#240180=CARTESIAN_POINT('Ctrl Pts',(1.13347515830392,7.82938088928804,26.1056533618288));
#240181=CARTESIAN_POINT('Ctrl Pts',(1.14047587960559,7.82836418490359,26.1053682049606));
#240182=CARTESIAN_POINT('Ctrl Pts',(1.15119111929889,7.82679334795556,26.1049307621782));
#240183=CARTESIAN_POINT('Ctrl Pts',(1.15490663674343,7.82624595607969,26.1047788973489));
#240184=CARTESIAN_POINT('Ctrl Pts',(1.16191463398962,7.82520839748316,26.1044921185943));
#240185=CARTESIAN_POINT('Ctrl Pts',(1.16520719882351,7.82471879778873,26.1043572398327));
#240186=CARTESIAN_POINT('Ctrl Pts',(1.17276523294139,7.82359005260197,26.1040473041234));
#240187=CARTESIAN_POINT('Ctrl Pts',(1.17703048652175,7.82294949724309,26.1038721603524));
#240188=CARTESIAN_POINT('Ctrl Pts',(1.18882107218922,7.82116892725666,26.1033873544864));
#240189=CARTESIAN_POINT('Ctrl Pts',(1.19634526829126,7.82002154271879,26.1030772420138));
#240190=CARTESIAN_POINT('Ctrl Pts',(1.23699814748896,7.81376223249415,26.1013978062007));
#240191=CARTESIAN_POINT('Ctrl Pts',(1.27009527117754,7.80845071555044,26.1000164646679));
#240192=CARTESIAN_POINT('Ctrl Pts',(1.77675059669189,7.7238348624857,26.0786661570943));
#240193=CARTESIAN_POINT('Ctrl Pts',(2.2421162159693,7.60179529812355,26.0563598131128));
#240194=CARTESIAN_POINT('Ctrl Pts',(3.09447293763029,7.29314924779506,26.0138061286022));
#240195=CARTESIAN_POINT('Ctrl Pts',(3.48308121579645,7.11575536627994,25.9936815251743));
#240196=CARTESIAN_POINT('Ctrl Pts',(4.01138527105143,6.8208926187245,25.9663143425586));
#240197=CARTESIAN_POINT('Ctrl Pts',(4.16427924726478,6.72863816026076,25.9583855005607));
#240198=CARTESIAN_POINT('Ctrl Pts',(4.51625888036789,6.49966074398804,25.9401587881319));
#240199=CARTESIAN_POINT('Ctrl Pts',(4.71247010742161,6.3588382451958,25.9300219980779));
#240200=CARTESIAN_POINT('Ctrl Pts',(4.91928730015014,6.19556466398832,25.9193502384425));
#240201=CARTESIAN_POINT('Ctrl Pts',(4.93656956896215,6.18180313085005,25.9184585274147));
#240202=CARTESIAN_POINT('Ctrl Pts',(4.96071364762451,6.16241185512859,25.9172127881281));
#240203=CARTESIAN_POINT('Ctrl Pts',(4.96762389100698,6.15684274966645,25.9168562490253));
#240204=CARTESIAN_POINT('Ctrl Pts',(4.97958242596478,6.14717188405658,25.9162392386036));
#240205=CARTESIAN_POINT('Ctrl Pts',(4.98463505079739,6.14307550985348,25.9159785439694));
#240206=CARTESIAN_POINT('Ctrl Pts',(4.99512108339739,6.13455258989415,25.9154375048495));
#240207=CARTESIAN_POINT('Ctrl Pts',(5.00055367419677,6.1301250450378,25.9151572022822));
#240208=CARTESIAN_POINT('Ctrl Pts',(5.01330222177585,6.11970679400144,25.9144994146451));
#240209=CARTESIAN_POINT('Ctrl Pts',(5.02061334293253,6.11371017247318,25.9141221764823));
#240210=CARTESIAN_POINT('Ctrl Pts',(5.04434985878454,6.09417006001401,25.912897392132));
#240211=CARTESIAN_POINT('Ctrl Pts',(5.06073140497371,6.08057331788893,25.9120520698406));
#240212=CARTESIAN_POINT('Ctrl Pts',(5.38637643554274,5.80805921374848,25.895246213873));
#240213=CARTESIAN_POINT('Ctrl Pts',(5.6754623561066,5.5259184381252,25.8803370786886));
#240214=CARTESIAN_POINT('Ctrl Pts',(6.27011228381404,4.84942489064089,25.8483637678578));
#240215=CARTESIAN_POINT('Ctrl Pts',(6.56247372882423,4.44580122646084,25.8316935546056));
#240216=CARTESIAN_POINT('Ctrl Pts',(6.91781220683121,3.84301683863817,25.8069848401363));
#240217=CARTESIAN_POINT('Ctrl Pts',(7.01388183108026,3.66474540948979,25.7996869988365));
#240218=CARTESIAN_POINT('Ctrl Pts',(7.13427751659233,3.41921785981841,25.7894099858113));
#240219=CARTESIAN_POINT('Ctrl Pts',(7.16468960440114,3.35502442328154,25.7867027369443));
#240220=CARTESIAN_POINT('Ctrl Pts',(7.22672273303816,3.21939457384322,25.7809237749373));
#240221=CARTESIAN_POINT('Ctrl Pts',(7.25815764873642,3.14788332052009,25.777841874611));
#240222=CARTESIAN_POINT('Ctrl Pts',(7.29359559588401,3.06391158548436,25.774190479926));
#240223=CARTESIAN_POINT('Ctrl Pts',(7.2986342281089,3.05188946745068,25.7736669462404));
#240224=CARTESIAN_POINT('Ctrl Pts',(7.30662467730634,3.03269138425578,25.772829743969));
#240225=CARTESIAN_POINT('Ctrl Pts',(7.30959570315216,3.02552340315881,25.7725168978054));
#240226=CARTESIAN_POINT('Ctrl Pts',(7.31481714431917,3.01287342281304,25.7719643433128));
#240227=CARTESIAN_POINT('Ctrl Pts',(7.31707195767473,3.00739323712137,25.7717248196948));
#240228=CARTESIAN_POINT('Ctrl Pts',(7.32171729765526,2.99606687270199,25.7712294772718));
#240229=CARTESIAN_POINT('Ctrl Pts',(7.32410698440346,2.99022035529244,25.7709736240022));
#240230=CARTESIAN_POINT('Ctrl Pts',(7.3301988727343,2.97526505751482,25.7703187452598));
#240231=CARTESIAN_POINT('Ctrl Pts',(7.33389109293483,2.9661522402239,25.7699193147646));
#240232=CARTESIAN_POINT('Ctrl Pts',(7.34799805010092,2.93114730523009,25.7683835500981));
#240233=CARTESIAN_POINT('Ctrl Pts',(7.35829266765072,2.90520719786508,25.7672424692423));
#240234=CARTESIAN_POINT('Ctrl Pts',(7.42680005071799,2.72988389094158,25.7595119491278));
#240235=CARTESIAN_POINT('Ctrl Pts',(7.48059552369722,2.57881991545966,25.7527627603881));
#240236=CARTESIAN_POINT('Ctrl Pts',(7.57801063966181,2.27649401736567,25.7391903386938));
#240237=CARTESIAN_POINT('Ctrl Pts',(7.62178083557579,2.12535300142618,25.732373834178));
#240238=CARTESIAN_POINT('Ctrl Pts',(7.75338882681451,1.61433155697979,25.7093683059126));
#240239=CARTESIAN_POINT('Ctrl Pts',(7.82046110818994,1.24960009383117,25.6930391849767));
#240240=CARTESIAN_POINT('Ctrl Pts',(7.91356405651987,0.41926592395969,25.6568611486482));
#240241=CARTESIAN_POINT('Ctrl Pts',(7.92452867562839,-0.0466752222971706,
25.6372781353941));
#240242=CARTESIAN_POINT('Ctrl Pts',(7.89186314670459,-0.551421332796872,
25.6167844943394));
#240243=CARTESIAN_POINT('Ctrl Pts',(7.8889292064818,-0.591916736334149,
25.6151447841897));
#240244=CARTESIAN_POINT('Ctrl Pts',(7.88437398432118,-0.648718964333772,
25.6128509140851));
#240245=CARTESIAN_POINT('Ctrl Pts',(7.88301359124601,-0.665045969766149,
25.6121922921765));
#240246=CARTESIAN_POINT('Ctrl Pts',(7.88056957172468,-0.693316700811977,
25.6110531187557));
#240247=CARTESIAN_POINT('Ctrl Pts',(7.87950948889312,-0.705262389321949,
25.6105721526273));
#240248=CARTESIAN_POINT('Ctrl Pts',(7.87732643998743,-0.729242932820919,
25.6096074094877));
#240249=CARTESIAN_POINT('Ctrl Pts',(7.87620304738806,-0.74127771750638,
25.6091236414423));
#240250=CARTESIAN_POINT('Ctrl Pts',(7.87346876379282,-0.769861738101626,
25.6079755734287));
#240251=CARTESIAN_POINT('Ctrl Pts',(7.8718332691595,-0.786408580381014,
25.6073117219543));
#240252=CARTESIAN_POINT('Ctrl Pts',(7.86655258293882,-0.838167419799401,
25.6052375182829));
#240253=CARTESIAN_POINT('Ctrl Pts',(7.86272318943543,-0.873360312132879,
25.6038305727208));
#240254=CARTESIAN_POINT('Ctrl Pts',(7.85335165086542,-0.954423125706396,
25.6005975743449));
#240255=CARTESIAN_POINT('Ctrl Pts',(7.84764361275078,-1.00027268178144,
25.5987747009162));
#240256=CARTESIAN_POINT('Ctrl Pts',(7.78810478296598,-1.44658680221168,
25.5810845557414));
#240257=CARTESIAN_POINT('Ctrl Pts',(7.70406824708064,-1.84243034530877,
25.5658698828461));
#240258=CARTESIAN_POINT('Ctrl Pts',(7.40337791033981,-2.86581218369819,
25.5266429365841));
#240259=CARTESIAN_POINT('Ctrl Pts',(7.13751549315792,-3.47542187534271,
25.5035403828359));
#240260=CARTESIAN_POINT('Ctrl Pts',(6.78327536612906,-4.07087513869016,
25.4760585818342));
#240261=CARTESIAN_POINT('Ctrl Pts',(6.76754866782858,-4.09696644855851,
25.4748432087378));
#240262=CARTESIAN_POINT('Ctrl Pts',(6.74674109882409,-4.13104043233352,
25.4732404550622));
#240263=CARTESIAN_POINT('Ctrl Pts',(6.74179592184971,-4.13910597292978,
25.4728599251289));
#240264=CARTESIAN_POINT('Ctrl Pts',(6.7341391328884,-4.15154400318084,25.4722712997907));
#240265=CARTESIAN_POINT('Ctrl Pts',(6.73143769275227,-4.155922768755,25.4720637305759));
#240266=CARTESIAN_POINT('Ctrl Pts',(6.7263168678056,-4.16420502432065,25.4716704614654));
#240267=CARTESIAN_POINT('Ctrl Pts',(6.72389835107848,-4.16810905026834,
25.4714848070942));
#240268=CARTESIAN_POINT('Ctrl Pts',(6.7183144432621,-4.17710521666728,25.4710563512632));
#240269=CARTESIAN_POINT('Ctrl Pts',(6.71514666252388,-4.18219586463287,
25.4708134231343));
#240270=CARTESIAN_POINT('Ctrl Pts',(6.70629777858811,-4.19638011548431,
25.4701351954627));
#240271=CARTESIAN_POINT('Ctrl Pts',(6.70060398527656,-4.20546575297769,
25.4696992129861));
#240272=CARTESIAN_POINT('Ctrl Pts',(6.66786980790264,-4.25746473442685,
25.4671949545672));
#240273=CARTESIAN_POINT('Ctrl Pts',(6.64043742628702,-4.30012608767705,
25.4651044659931));
#240274=CARTESIAN_POINT('Ctrl Pts',(6.55823600476274,-4.42529868456959,
25.4588618965666));
#240275=CARTESIAN_POINT('Ctrl Pts',(6.50232854621353,-4.50704449709793,
25.4546462635495));
#240276=CARTESIAN_POINT('Ctrl Pts',(6.39493788545992,-4.65790875222603,
25.4466322764198));
#240277=CARTESIAN_POINT('Ctrl Pts',(6.3438302323843,-4.72727847542925,25.4428513684603));
#240278=CARTESIAN_POINT('Ctrl Pts',(6.04035596901734,-5.12540596672461,
25.4206450382768));
#240279=CARTESIAN_POINT('Ctrl Pts',(5.76360505415213,-5.43475171000619,
25.4013764489329));
#240280=CARTESIAN_POINT('Ctrl Pts',(5.01942047650561,-6.1454956440562,25.3540120357548));
#240281=CARTESIAN_POINT('Ctrl Pts',(4.52692046934216,-6.51681590509685,
25.3264482449478));
#240282=CARTESIAN_POINT('Ctrl Pts',(3.94139570983323,-6.85954613464755,
25.2985278931954));
#240283=CARTESIAN_POINT('Ctrl Pts',(3.88607054964027,-6.8910397790384,25.2959311305616));
#240284=CARTESIAN_POINT('Ctrl Pts',(3.81788358005277,-6.92877259244427,
25.2927803022379));
#240285=CARTESIAN_POINT('Ctrl Pts',(3.80537799203041,-6.93564870859802,
25.292204457958));
#240286=CARTESIAN_POINT('Ctrl Pts',(3.78469697854054,-6.9469472556835,25.2912554804291));
#240287=CARTESIAN_POINT('Ctrl Pts',(3.77653226797111,-6.95138917212442,
25.2908816827509));
#240288=CARTESIAN_POINT('Ctrl Pts',(3.76178497541852,-6.95937861546379,
25.290208051278));
#240289=CARTESIAN_POINT('Ctrl Pts',(3.75520516225295,-6.9629312149718,25.2899080449809));
#240290=CARTESIAN_POINT('Ctrl Pts',(3.74114027095115,-6.97049945301062,
25.2892679245558));
#240291=CARTESIAN_POINT('Ctrl Pts',(3.73365373916137,-6.97451237779075,
25.2889279028926));
#240292=CARTESIAN_POINT('Ctrl Pts',(3.71342776775083,-6.9853119876847,25.288011179519));
#240293=CARTESIAN_POINT('Ctrl Pts',(3.70067616664857,-6.99207589088613,
25.2874352509688));
#240294=CARTESIAN_POINT('Ctrl Pts',(3.63807612165887,-7.02506196361125,
25.2846177705243));
#240295=CARTESIAN_POINT('Ctrl Pts',(3.58796657139059,-7.05078644554548,
25.2823930629384));
#240296=CARTESIAN_POINT('Ctrl Pts',(3.17202403732779,-7.2587341389627,25.2641713853836));
#240297=CARTESIAN_POINT('Ctrl Pts',(2.79283639816729,-7.41289855684044,
25.2491540744402));
#240298=CARTESIAN_POINT('Ctrl Pts',(2.06802766020124,-7.64402357077033,
25.2222185966223));
#240299=CARTESIAN_POINT('Ctrl Pts',(1.72588399181924,-7.7284644605348,25.210178402911));
#240300=CARTESIAN_POINT('Ctrl Pts',(0.892907146292186,-7.87595001267056,
25.1809104913779));
#240301=CARTESIAN_POINT('Ctrl Pts',(0.399564734553673,-7.91632554801724,
25.1635904060704));
#240302=CARTESIAN_POINT('Ctrl Pts',(-0.128326483362468,-7.91003230056521,
25.1427104788361));
#240303=CARTESIAN_POINT('Ctrl Pts',(-0.162345484888009,-7.90940722041612,
25.1413556328557));
#240304=CARTESIAN_POINT('Ctrl Pts',(-0.207319566408222,-7.90829057411755,
25.1395530951377));
#240305=CARTESIAN_POINT('Ctrl Pts',(-0.2182794854113,-7.90799565452776,
25.1391129322763));
#240306=CARTESIAN_POINT('Ctrl Pts',(-0.235283884072636,-7.90750270746726,
25.1384286609986));
#240307=CARTESIAN_POINT('Ctrl Pts',(-0.241328833869524,-7.90732053026867,
25.1381851413681));
#240308=CARTESIAN_POINT('Ctrl Pts',(-0.25282129510099,-7.90696099014185,
25.1377216713262));
#240309=CARTESIAN_POINT('Ctrl Pts',(-0.258268845628237,-7.90678492878626,
25.1375017685695));
#240310=CARTESIAN_POINT('Ctrl Pts',(-0.2709042296182,-7.90636348921582,
25.136991224677));
#240311=CARTESIAN_POINT('Ctrl Pts',(-0.278091913268336,-7.90611393875588,
25.1367004336836));
#240312=CARTESIAN_POINT('Ctrl Pts',(-0.298356904620666,-7.90538268559308,
25.1358795602324));
#240313=CARTESIAN_POINT('Ctrl Pts',(-0.31143334100732,-7.90487833682059,
25.1353486805052));
#240314=CARTESIAN_POINT('Ctrl Pts',(-0.389438147581476,-7.9016758921437,
25.1321749217301));
#240315=CARTESIAN_POINT('Ctrl Pts',(-0.454331603766616,-7.89821033573475,
25.1295061030923));
#240316=CARTESIAN_POINT('Ctrl Pts',(-0.767204610793201,-7.87763310944881,
25.1165213591357));
#240317=CARTESIAN_POINT('Ctrl Pts',(-1.01432200024726,-7.8496401047812,
25.1059149459615));
#240318=CARTESIAN_POINT('Ctrl Pts',(-1.42060480679042,-7.78410984820686,
25.0882062682119));
#240319=CARTESIAN_POINT('Ctrl Pts',(-1.58066643160403,-7.75319143955675,
25.0811573547996));
#240320=CARTESIAN_POINT('Ctrl Pts',(-2.41718768415652,-7.56462143454308,
25.0441163516376));
#240321=CARTESIAN_POINT('Ctrl Pts',(-3.07169686577322,-7.32332428500461,
25.0148602313158));
#240322=CARTESIAN_POINT('Ctrl Pts',(-3.85920077119008,-6.90859483200105,
24.9784786209216));
#240323=CARTESIAN_POINT('Ctrl Pts',(-4.02868505155801,-6.81115347557454,
24.9705249472782));
#240324=CARTESIAN_POINT('Ctrl Pts',(-4.23443943109837,-6.68249019055684,
24.960712382342));
#240325=CARTESIAN_POINT('Ctrl Pts',(-4.27426643629504,-6.65708636716249,
24.9588055484855));
#240326=CARTESIAN_POINT('Ctrl Pts',(-4.33708197457112,-6.6162231048759,
24.9557861183175));
#240327=CARTESIAN_POINT('Ctrl Pts',(-4.36022087023407,-6.60099706073905,
24.9546712660697));
#240328=CARTESIAN_POINT('Ctrl Pts',(-4.40311666151133,-6.57244646316064,
24.9525996083202));
#240329=CARTESIAN_POINT('Ctrl Pts',(-4.42289423302735,-6.55915356223814,
24.9516424911782));
#240330=CARTESIAN_POINT('Ctrl Pts',(-4.46667809829981,-6.52943747718006,
24.9495192162957));
#240331=CARTESIAN_POINT('Ctrl Pts',(-4.49065450569651,-6.51297083667225,
24.9483535355956));
#240332=CARTESIAN_POINT('Ctrl Pts',(-4.56012943768581,-6.46469045543939,
24.9449670642311));
#240333=CARTESIAN_POINT('Ctrl Pts',(-4.60538467697536,-6.43252945560772,
24.9427501575247));
#240334=CARTESIAN_POINT('Ctrl Pts',(-4.70686112012858,-6.35879454162698,
24.9377532698846));
#240335=CARTESIAN_POINT('Ctrl Pts',(-4.76287733930216,-6.31694619033517,
24.9349766274018));
#240336=CARTESIAN_POINT('Ctrl Pts',(-4.94234353897597,-6.17912693867589,
24.9260174705253));
#240337=CARTESIAN_POINT('Ctrl Pts',(-5.06350578203972,-6.08023679844488,
24.9198707185008));
#240338=CARTESIAN_POINT('Ctrl Pts',(-5.42453302331702,-5.76729328858461,
24.901192208494));
#240339=CARTESIAN_POINT('Ctrl Pts',(-5.65435206053312,-5.54215984406977,
24.8887963742496));
#240340=CARTESIAN_POINT('Ctrl Pts',(-6.01740140029522,-5.14035484515502,
24.8678586022022));
#240341=CARTESIAN_POINT('Ctrl Pts',(-6.15808236656568,-4.97095432613832,
24.8593393837935));
#240342=CARTESIAN_POINT('Ctrl Pts',(-6.37749611203214,-4.68311645786316,
24.8451500723635));
#240343=CARTESIAN_POINT('Ctrl Pts',(-6.46042724311262,-4.56803184101864,
24.8395461789172));
#240344=CARTESIAN_POINT('Ctrl Pts',(-6.55272448061564,-4.43240532886357,
24.8329766340643));
#240345=CARTESIAN_POINT('Ctrl Pts',(-6.56515298355492,-4.41397569249168,
24.8320846448784));
#240346=CARTESIAN_POINT('Ctrl Pts',(-6.58488513591073,-4.38444811181062,
24.8306564116691));
#240347=CARTESIAN_POINT('Ctrl Pts',(-6.59223881665402,-4.37338368782955,
24.8301214305637));
#240348=CARTESIAN_POINT('Ctrl Pts',(-6.60520032851953,-4.35377469291024,
24.8291736001751));
#240349=CARTESIAN_POINT('Ctrl Pts',(-6.61081954406833,-4.34523767031747,
24.8287610482132));
#240350=CARTESIAN_POINT('Ctrl Pts',(-6.62156871649564,-4.32883782013141,
24.8279686833773));
#240351=CARTESIAN_POINT('Ctrl Pts',(-6.62670125268815,-4.32097670062247,
24.8275889401349));
#240352=CARTESIAN_POINT('Ctrl Pts',(-6.63763962354227,-4.30415789391444,
24.8267766057991));
#240353=CARTESIAN_POINT('Ctrl Pts',(-6.64344134329728,-4.29519755832799,
24.8263439036952));
#240354=CARTESIAN_POINT('Ctrl Pts',(-6.65731368971747,-4.2736773768335,
24.8253048131739));
#240355=CARTESIAN_POINT('Ctrl Pts',(-6.66536691698014,-4.26110639900326,
24.8246979384826));
#240356=CARTESIAN_POINT('Ctrl Pts',(-6.74569384203709,-4.13493225572388,
24.8186082185335));
#240357=CARTESIAN_POINT('Ctrl Pts',(-6.8150904613982,-4.019526196529,24.8130502646201));
#240358=CARTESIAN_POINT('Ctrl Pts',(-7.07042589224615,-3.56926764338862,
24.7915061307935));
#240359=CARTESIAN_POINT('Ctrl Pts',(-7.23490359258804,-3.22285014961678,
24.7752459526445));
#240360=CARTESIAN_POINT('Ctrl Pts',(-7.42031007689021,-2.74581747595993,
24.7537405127815));
#240361=CARTESIAN_POINT('Ctrl Pts',(-7.46403738280445,-2.62462601690647,
24.7483469613483));
#240362=CARTESIAN_POINT('Ctrl Pts',(-7.58670156865326,-2.25675471832648,
24.7321983807278));
#240363=CARTESIAN_POINT('Ctrl Pts',(-7.65650666553869,-2.00721060201868,
24.7215461312734));
#240364=CARTESIAN_POINT('Ctrl Pts',(-7.72318865482372,-1.71406349184627,
24.7093574827083));
#240365=CARTESIAN_POINT('Ctrl Pts',(-7.73210823394862,-1.67336754392676,
24.7076723989871));
#240366=CARTESIAN_POINT('Ctrl Pts',(-7.74597837700718,-1.60760464455309,
24.7049602313704));
#240367=CARTESIAN_POINT('Ctrl Pts',(-7.75112967470828,-1.58258095594426,
24.703930739403));
#240368=CARTESIAN_POINT('Ctrl Pts',(-7.76011158640798,-1.53785307219791,
24.7020949857497));
#240369=CARTESIAN_POINT('Ctrl Pts',(-7.76398859115839,-1.51815844509082,
24.7012881782103));
#240370=CARTESIAN_POINT('Ctrl Pts',(-7.77133790987195,-1.48006041193939,
24.6997303124276));
#240371=CARTESIAN_POINT('Ctrl Pts',(-7.77481991163523,-1.46165901506856,
24.6989791453062));
#240372=CARTESIAN_POINT('Ctrl Pts',(-7.78220196596491,-1.42187412134314,
24.6973577825686));
#240373=CARTESIAN_POINT('Ctrl Pts',(-7.78607930032468,-1.40048655422635,
24.6964878552548));
#240374=CARTESIAN_POINT('Ctrl Pts',(-7.79529299447324,-1.34844222269386,
24.6943749478352));
#240375=CARTESIAN_POINT('Ctrl Pts',(-7.80053672141716,-1.31776939005816,
24.6931330267593));
#240376=CARTESIAN_POINT('Ctrl Pts',(-7.82558409321283,-1.16586599309891,
24.6869982566981));
#240377=CARTESIAN_POINT('Ctrl Pts',(-7.84274340238029,-1.04421566810183,
24.6821349300275));
#240378=CARTESIAN_POINT('Ctrl Pts',(-7.89298455370822,-0.616172009389288,
24.6651523667399));
#240379=CARTESIAN_POINT('Ctrl Pts',(-7.9109944847476,-0.308287032974473,
24.6531273941981));
#240380=CARTESIAN_POINT('Ctrl Pts',(-7.91099999873345,-0.000141560223926238,
24.6412306241627));
#240381=CARTESIAN_POINT('',(-7.911,-2.22599716437344E-13,22.642331508237));
#240382=CARTESIAN_POINT('Ctrl Pts',(-7.911,-2.20934381900406E-13,24.642331508237));
#240383=CARTESIAN_POINT('Ctrl Pts',(-7.91100000000006,2.2016758966665,24.5537440725043));
#240384=CARTESIAN_POINT('Ctrl Pts',(-6.94214576672388,4.38610418338655,
24.4651566367716));
#240385=CARTESIAN_POINT('Ctrl Pts',(-3.67820201488323,7.34180684107613,
24.2879817653061));
#240386=CARTESIAN_POINT('Ctrl Pts',(-1.4086817587179,8.08992666571327,24.1993943295734));
#240387=CARTESIAN_POINT('Ctrl Pts',(2.97309270521222,7.65454228025276,24.022219458108));
#240388=CARTESIAN_POINT('Ctrl Pts',(5.05102072675554,6.47444880834262,23.9336320223752));
#240389=CARTESIAN_POINT('Ctrl Pts',(7.66951518847845,2.93425195367772,23.7564571509098));
#240390=CARTESIAN_POINT('Ctrl Pts',(8.18956872247065,0.601881960099923,
23.6678697151771));
#240391=CARTESIAN_POINT('Ctrl Pts',(7.3230668976138,-3.71537198232373,23.4906948437116));
#240392=CARTESIAN_POINT('Ctrl Pts',(5.94329958850263,-5.66643518936444,
23.4021074079789));
#240393=CARTESIAN_POINT('Ctrl Pts',(2.16154501637943,-7.9220591323297,23.2249325365135));
#240394=CARTESIAN_POINT('Ctrl Pts',(-0.210816529299319,-8.20894963713004,
23.1363451007807));
#240395=CARTESIAN_POINT('Ctrl Pts',(-4.42123908576341,-6.91982244717892,
22.9591702293153));
#240396=CARTESIAN_POINT('Ctrl Pts',(-6.22631625634109,-5.3539035880361,
22.8705827935826));
#240397=CARTESIAN_POINT('Ctrl Pts',(-7.65317280859467,-2.31334857514605,
22.7354407413122));
#240398=CARTESIAN_POINT('Ctrl Pts',(-7.91099999999997,-1.15702837836574,
22.6888861247746));
#240399=CARTESIAN_POINT('Ctrl Pts',(-7.911,-2.22599716437344E-13,22.642331508237));
#240400=CARTESIAN_POINT('',(-7.911,-5.77315972805081E-14,18.642331508237));
#240401=CARTESIAN_POINT('Ctrl Pts',(-7.91099999997837,1.85007747019461E-5,
22.6428089873088));
#240402=CARTESIAN_POINT('Ctrl Pts',(-7.91099947188172,0.225834589107863,
22.6340593417855));
#240403=CARTESIAN_POINT('Ctrl Pts',(-7.90133019881069,0.451545623192688,
22.625271724421));
#240404=CARTESIAN_POINT('Ctrl Pts',(-7.87628419288177,0.743347599373823,
22.6136725448826));
#240405=CARTESIAN_POINT('Ctrl Pts',(-7.86969985014172,0.810087925509054,
22.6110031635888));
#240406=CARTESIAN_POINT('Ctrl Pts',(-7.86039549709614,0.893526189294941,
22.6076401591403));
#240407=CARTESIAN_POINT('Ctrl Pts',(-7.85846939797451,0.910310463447805,
22.6069623552187));
#240408=CARTESIAN_POINT('Ctrl Pts',(-7.85514325884769,0.938497395190295,
22.6058217621311));
#240409=CARTESIAN_POINT('Ctrl Pts',(-7.85377211620916,0.949903428503671,
22.605359576643));
#240410=CARTESIAN_POINT('Ctrl Pts',(-7.85121277146412,0.970809288817946,
22.6045112405228));
#240411=CARTESIAN_POINT('Ctrl Pts',(-7.85003215939754,0.980310029480703,
22.6041252539591));
#240412=CARTESIAN_POINT('Ctrl Pts',(-7.84757168723977,0.999820709126633,
22.6033316286725));
#240413=CARTESIAN_POINT('Ctrl Pts',(-7.84628991462983,1.00983038756246,
22.6029239483633));
#240414=CARTESIAN_POINT('Ctrl Pts',(-7.84339225134556,1.03212034556546,
22.602014913668));
#240415=CARTESIAN_POINT('Ctrl Pts',(-7.84176666681656,1.04439932883301,
22.6015133401986));
#240416=CARTESIAN_POINT('Ctrl Pts',(-7.83679430839989,1.08129228993849,
22.6000038185238));
#240417=CARTESIAN_POINT('Ctrl Pts',(-7.83336045860627,1.10589418857624,
22.5989937899261));
#240418=CARTESIAN_POINT('Ctrl Pts',(-7.79597594242603,1.36482300994179,
22.5883289695019));
#240419=CARTESIAN_POINT('Ctrl Pts',(-7.75163812332933,1.59752424659365,
22.5784506834872));
#240420=CARTESIAN_POINT('Ctrl Pts',(-7.66769492256991,1.95099672648986,
22.5631819610048));
#240421=CARTESIAN_POINT('Ctrl Pts',(-7.63550721297095,2.07339409088313,
22.557844577228));
#240422=CARTESIAN_POINT('Ctrl Pts',(-7.57845711590641,2.27093855724286,
22.5491703269968));
#240423=CARTESIAN_POINT('Ctrl Pts',(-7.55537867926464,2.34657776940649,
22.5458344051522));
#240424=CARTESIAN_POINT('Ctrl Pts',(-7.46888534036507,2.61554315244939,
22.5339289701738));
#240425=CARTESIAN_POINT('Ctrl Pts',(-7.39915136782156,2.80675526995091,
22.5253867440962));
#240426=CARTESIAN_POINT('Ctrl Pts',(-7.22505167866806,3.23238142449122,
22.5062460365987));
#240427=CARTESIAN_POINT('Ctrl Pts',(-7.1164986088984,3.4648398212024,22.4957044439306));
#240428=CARTESIAN_POINT('Ctrl Pts',(-6.98210501527786,3.71956025029167,
22.4840320954564));
#240429=CARTESIAN_POINT('Ctrl Pts',(-6.96719668165485,3.7474110143701,22.4827540877373));
#240430=CARTESIAN_POINT('Ctrl Pts',(-6.94165181214019,3.7944528591276,22.4805922490391));
#240431=CARTESIAN_POINT('Ctrl Pts',(-6.93110154893593,3.8136902998665,22.479707266701));
#240432=CARTESIAN_POINT('Ctrl Pts',(-6.91143514245836,3.84919902275244,
22.478071984102));
#240433=CARTESIAN_POINT('Ctrl Pts',(-6.90234123007919,3.8654824266882,22.4773213916176));
#240434=CARTESIAN_POINT('Ctrl Pts',(-6.88338295794391,3.89914856235341,
22.4757680361489));
#240435=CARTESIAN_POINT('Ctrl Pts',(-6.87351013381267,3.91652638191039,
22.4749653924566));
#240436=CARTESIAN_POINT('Ctrl Pts',(-6.85101900454776,3.95576753807374,
22.4731509608421));
#240437=CARTESIAN_POINT('Ctrl Pts',(-6.83836168591077,3.97760828566071,
22.4721396988799));
#240438=CARTESIAN_POINT('Ctrl Pts',(-6.80544566493161,4.03378477728129,
22.4695348352247));
#240439=CARTESIAN_POINT('Ctrl Pts',(-6.78503152774331,4.06802870150093,
22.4679432850186));
#240440=CARTESIAN_POINT('Ctrl Pts',(-6.62875464993973,4.32572807193166,
22.4559356229943));
#240441=CARTESIAN_POINT('Ctrl Pts',(-6.4821440984346,4.54247980283908,22.4456648460621));
#240442=CARTESIAN_POINT('Ctrl Pts',(-6.28058366354077,4.81078733198935,
22.4325530690247));
#240443=CARTESIAN_POINT('Ctrl Pts',(-6.23527154137811,4.86937314146339,
22.4296652489258));
#240444=CARTESIAN_POINT('Ctrl Pts',(-6.15435604600134,4.97101017366863,
22.4246125997869));
#240445=CARTESIAN_POINT('Ctrl Pts',(-6.11910688717685,5.0143365892881,22.4224447028392));
#240446=CARTESIAN_POINT('Ctrl Pts',(-5.95684678751198,5.20951901160713,
22.4126145385632));
#240447=CARTESIAN_POINT('Ctrl Pts',(-5.82462080235687,5.35694936395049,
22.4050135008768));
#240448=CARTESIAN_POINT('Ctrl Pts',(-5.4896007793828,5.70340642148044,22.3866671704931));
#240449=CARTESIAN_POINT('Ctrl Pts',(-5.28134977784322,5.89677110331032,
22.3760093399635));
#240450=CARTESIAN_POINT('Ctrl Pts',(-4.8877576665812,6.22461666329464,22.3568458554157));
#240451=CARTESIAN_POINT('Ctrl Pts',(-4.70612459444823,6.36305095458173,
22.3483344491076));
#240452=CARTESIAN_POINT('Ctrl Pts',(-4.3415918921577,6.61672811096935,22.3315952822459));
#240453=CARTESIAN_POINT('Ctrl Pts',(-4.15945478890625,6.73271429524361,
22.3233836074929));
#240454=CARTESIAN_POINT('Ctrl Pts',(-3.92005662246139,6.87173911146183,
22.3125749451155));
#240455=CARTESIAN_POINT('Ctrl Pts',(-3.86695199250248,6.90176241592576,
22.3101761715765));
#240456=CARTESIAN_POINT('Ctrl Pts',(-3.78062839310874,6.94925737892598,
22.3062684962585));
#240457=CARTESIAN_POINT('Ctrl Pts',(-3.74762264836752,6.96711228571304,
22.3047724465327));
#240458=CARTESIAN_POINT('Ctrl Pts',(-3.7067609966152,6.98884257757154,22.3029167076623));
#240459=CARTESIAN_POINT('Ctrl Pts',(-3.69902377467732,6.99294078151754,
22.3025651617896));
#240460=CARTESIAN_POINT('Ctrl Pts',(-3.68403311561726,7.00084910081391,
22.3018837199889));
#240461=CARTESIAN_POINT('Ctrl Pts',(-3.67678052949254,7.00466081025467,
22.3015538839924));
#240462=CARTESIAN_POINT('Ctrl Pts',(-3.66357803353426,7.01157343321013,
22.3009531647719));
#240463=CARTESIAN_POINT('Ctrl Pts',(-3.65763007008554,7.01467806012467,
22.3006824227379));
#240464=CARTESIAN_POINT('Ctrl Pts',(-3.64569438681568,7.02088875702022,
22.3001389028311));
#240465=CARTESIAN_POINT('Ctrl Pts',(-3.63970663004246,7.02399474283716,
22.2998661220643));
#240466=CARTESIAN_POINT('Ctrl Pts',(-3.6227321961501,7.03277223491493,22.2990924885493));
#240467=CARTESIAN_POINT('Ctrl Pts',(-3.6117362111439,7.03842563449197,22.2985909293477));
#240468=CARTESIAN_POINT('Ctrl Pts',(-3.56563632572705,7.06199063316919,
22.2964863463025));
#240469=CARTESIAN_POINT('Ctrl Pts',(-3.53041244659525,7.07966538728848,
22.2948738448653));
#240470=CARTESIAN_POINT('Ctrl Pts',(-3.12823238779529,7.27772481163952,
22.2763988287588));
#240471=CARTESIAN_POINT('Ctrl Pts',(-2.74802911571958,7.42962425631084,
22.2580950489523));
#240472=CARTESIAN_POINT('Ctrl Pts',(-2.07436532959066,7.63997019556098,
22.2258840418904));
#240473=CARTESIAN_POINT('Ctrl Pts',(-1.78608933201022,7.71245905865922,
22.2121852835603));
#240474=CARTESIAN_POINT('Ctrl Pts',(-1.4540998467207,7.77632307354195,22.1968332689011));
#240475=CARTESIAN_POINT('Ctrl Pts',(-1.41371932530258,7.78376545192754,
22.194972807624));
#240476=CARTESIAN_POINT('Ctrl Pts',(-1.32481652063159,7.79943614115764,
22.1908930085562));
#240477=CARTESIAN_POINT('Ctrl Pts',(-1.27627155825407,7.80752674731903,
22.1886758531657));
#240478=CARTESIAN_POINT('Ctrl Pts',(-1.16778080995629,7.82456914009742,
22.1837463996782));
#240479=CARTESIAN_POINT('Ctrl Pts',(-1.1078010156543,7.83328611152453,22.1810384719679));
#240480=CARTESIAN_POINT('Ctrl Pts',(-0.927566984344306,7.857368295966,22.1729575392434));
#240481=CARTESIAN_POINT('Ctrl Pts',(-0.8070518028975,7.87065980948529,22.167629173485));
#240482=CARTESIAN_POINT('Ctrl Pts',(-0.510681921319957,7.8964670567616,
22.1547289874667));
#240483=CARTESIAN_POINT('Ctrl Pts',(-0.334619928280042,7.90588530861514,
22.1472410774888));
#240484=CARTESIAN_POINT('Ctrl Pts',(-0.0656134310241799,7.91127205124591,
22.1360805822652));
#240485=CARTESIAN_POINT('Ctrl Pts',(0.0271832380362279,7.91149748277865,
22.1322811667856));
#240486=CARTESIAN_POINT('Ctrl Pts',(0.136364745785925,7.9098416346343,22.1278692412764));
#240487=CARTESIAN_POINT('Ctrl Pts',(0.152764209294816,7.90954190389132,
22.1272080993915));
#240488=CARTESIAN_POINT('Ctrl Pts',(0.177884482337895,7.90900462861615,
22.1261977317544));
#240489=CARTESIAN_POINT('Ctrl Pts',(0.186605981675171,7.90880365875589,
22.1258473769466));
#240490=CARTESIAN_POINT('Ctrl Pts',(0.201811108095771,7.90842812093658,
22.1252373202608));
#240491=CARTESIAN_POINT('Ctrl Pts',(0.208294878119738,7.90826000529718,
22.124977419095));
#240492=CARTESIAN_POINT('Ctrl Pts',(0.222870067641702,7.9078641525774,22.1243937104413));
#240493=CARTESIAN_POINT('Ctrl Pts',(0.230961364495052,7.90763196989324,
22.1240700408404));
#240494=CARTESIAN_POINT('Ctrl Pts',(0.252581737747672,7.90697835323765,
22.1232061672142));
#240495=CARTESIAN_POINT('Ctrl Pts',(0.266110139623721,7.90653461440098,
22.1226666547609));
#240496=CARTESIAN_POINT('Ctrl Pts',(0.324218775260846,7.90447931068766,
22.1203536956783));
#240497=CARTESIAN_POINT('Ctrl Pts',(0.368786477951271,7.90252539401648,
22.1185908841695));
#240498=CARTESIAN_POINT('Ctrl Pts',(1.08739624247348,7.86492795316929,22.0903422464757));
#240499=CARTESIAN_POINT('Ctrl Pts',(1.75415916349144,7.74354869690067,22.0669395413601));
#240500=CARTESIAN_POINT('Ctrl Pts',(2.72994846730285,7.43323781131119,22.0320968713692));
#240501=CARTESIAN_POINT('Ctrl Pts',(3.05505821906778,7.30563109655708,22.0203113192068));
#240502=CARTESIAN_POINT('Ctrl Pts',(3.53012980368479,7.08189040513239,22.0016192066847));
#240503=CARTESIAN_POINT('Ctrl Pts',(3.68702782460995,7.00148615918928,21.9951859512676));
#240504=CARTESIAN_POINT('Ctrl Pts',(3.90745831682518,6.87905893891138,21.9856038899837));
#240505=CARTESIAN_POINT('Ctrl Pts',(3.97327889362922,6.84125256043448,21.9826708224208));
#240506=CARTESIAN_POINT('Ctrl Pts',(4.07265036097292,6.78225724436087,21.978117974155));
#240507=CARTESIAN_POINT('Ctrl Pts',(4.10660392991548,6.76175260951729,21.9765397832609));
#240508=CARTESIAN_POINT('Ctrl Pts',(4.14747804407004,6.73664722596892,21.9746108816709));
#240509=CARTESIAN_POINT('Ctrl Pts',(4.15454790129882,6.73228948486491,21.9742761885484));
#240510=CARTESIAN_POINT('Ctrl Pts',(4.16552421250567,6.72549999694147,21.9737548962195));
#240511=CARTESIAN_POINT('Ctrl Pts',(4.16943544558883,6.72307595068726,21.9735688129392));
#240512=CARTESIAN_POINT('Ctrl Pts',(4.17632080872631,6.71880032270922,21.9732406469143));
#240513=CARTESIAN_POINT('Ctrl Pts',(4.17929583225755,6.71695017253029,21.9730986609444));
#240514=CARTESIAN_POINT('Ctrl Pts',(4.18607532265463,6.7127277983333,21.9727746625463));
#240515=CARTESIAN_POINT('Ctrl Pts',(4.18987900084942,6.71035431698915,21.9725925645437));
#240516=CARTESIAN_POINT('Ctrl Pts',(4.20010062288934,6.70396398281072,21.9721023559091));
#240517=CARTESIAN_POINT('Ctrl Pts',(4.20651480684571,6.69994115677308,21.9717938351828));
#240518=CARTESIAN_POINT('Ctrl Pts',(4.23695296205756,6.680790118873,21.970325400161));
#240519=CARTESIAN_POINT('Ctrl Pts',(4.26090078451377,6.66554209851233,21.9691571149886));
#240520=CARTESIAN_POINT('Ctrl Pts',(4.66035652620445,6.40816893017067,21.9494599959016));
#240521=CARTESIAN_POINT('Ctrl Pts',(5.0147402093208,6.1348074521758,21.9289125924497));
#240522=CARTESIAN_POINT('Ctrl Pts',(5.54324189633102,5.65060343332933,21.8956222157966));
#240523=CARTESIAN_POINT('Ctrl Pts',(5.73289344247054,5.45809382295399,21.8830181441089));
#240524=CARTESIAN_POINT('Ctrl Pts',(6.10438682706551,5.04023178486727,21.8573830384152));
#240525=CARTESIAN_POINT('Ctrl Pts',(6.28446923994954,4.81382821691317,21.8444055708804));
#240526=CARTESIAN_POINT('Ctrl Pts',(6.54119723364208,4.45202674585738,21.8252230986467));
#240527=CARTESIAN_POINT('Ctrl Pts',(6.62691928739897,4.32339541815724,21.818678789976));
#240528=CARTESIAN_POINT('Ctrl Pts',(6.75415067617889,4.11979199745794,21.8087454503479));
#240529=CARTESIAN_POINT('Ctrl Pts',(6.79830100027159,4.04652216335594,21.8052528562462));
#240530=CARTESIAN_POINT('Ctrl Pts',(6.84882584814265,3.9595116851916,21.8011995931593));
#240531=CARTESIAN_POINT('Ctrl Pts',(6.85635904392977,3.94645270434103,21.8005937224651));
#240532=CARTESIAN_POINT('Ctrl Pts',(6.86783791703805,3.92642171947991,21.7996681380012));
#240533=CARTESIAN_POINT('Ctrl Pts',(6.87181038928772,3.91946516097647,21.7993473824943));
#240534=CARTESIAN_POINT('Ctrl Pts',(6.87871617792437,3.90732903342419,21.7987890055021));
#240535=CARTESIAN_POINT('Ctrl Pts',(6.88165422405628,3.9021521718947,21.7985512005224));
#240536=CARTESIAN_POINT('Ctrl Pts',(6.8877813985314,3.89132759775534,21.7980547530893));
#240537=CARTESIAN_POINT('Ctrl Pts',(6.89096943075404,3.88567926773465,21.7977961532129));
#240538=CARTESIAN_POINT('Ctrl Pts',(6.89975692693925,3.87006537608898,21.7970825340427));
#240539=CARTESIAN_POINT('Ctrl Pts',(6.90534175404857,3.86009156981522,21.7966280813417));
#240540=CARTESIAN_POINT('Ctrl Pts',(6.92709495946532,3.82104476219223,21.7948543410736));
#240541=CARTESIAN_POINT('Ctrl Pts',(6.94310162327903,3.79188179376777,21.793541295473));
#240542=CARTESIAN_POINT('Ctrl Pts',(7.20123219617396,3.31447196654534,21.7722341279695));
#240543=CARTESIAN_POINT('Ctrl Pts',(7.39969815673857,2.84394314497516,21.7540460092325));
#240544=CARTESIAN_POINT('Ctrl Pts',(7.64136847332154,2.06984492742794,21.7262883056658));
#240545=CARTESIAN_POINT('Ctrl Pts',(7.71467518660256,1.77723268559261,21.7162270292646));
#240546=CARTESIAN_POINT('Ctrl Pts',(7.8225374645392,1.21131559017786,21.69663899123));
#240547=CARTESIAN_POINT('Ctrl Pts',(7.85987595156819,0.93899572923286,21.6871537086428));
#240548=CARTESIAN_POINT('Ctrl Pts',(7.89638970338853,0.506354469200814,
21.6712640996314));
#240549=CARTESIAN_POINT('Ctrl Pts',(7.90499325211327,0.347046390675704,
21.665237634515));
#240550=CARTESIAN_POINT('Ctrl Pts',(7.90950277392658,0.156932182869372,
21.6577204511803));
#240551=CARTESIAN_POINT('Ctrl Pts',(7.91005177978121,0.126264129222067,
21.656497733352));
#240552=CARTESIAN_POINT('Ctrl Pts',(7.91051053026259,0.0883024688019221,
21.6549708614013));
#240553=CARTESIAN_POINT('Ctrl Pts',(7.91058856414158,0.0810107618625305,
21.6546769684268));
#240554=CARTESIAN_POINT('Ctrl Pts',(7.91069583887694,0.0694992955269612,
21.6542120194351));
#240555=CARTESIAN_POINT('Ctrl Pts',(7.91073178551788,0.0652795888302459,
21.6540413775776));
#240556=CARTESIAN_POINT('Ctrl Pts',(7.91079296536326,0.0573532802561827,
21.6537204561918));
#240557=CARTESIAN_POINT('Ctrl Pts',(7.91081896980937,0.0536466812177394,
21.6535702238721));
#240558=CARTESIAN_POINT('Ctrl Pts',(7.91087138337838,0.0453440202853812,
21.6532333542403));
#240559=CARTESIAN_POINT('Ctrl Pts',(7.9108963922299,0.0407479542872487,
21.6530466317827));
#240560=CARTESIAN_POINT('Ctrl Pts',(7.91094955548323,0.0291145307100258,
21.6525733949361));
#240561=CARTESIAN_POINT('Ctrl Pts',(7.9109723247733,0.0220771669155261,
21.6522865559681));
#240562=CARTESIAN_POINT('Ctrl Pts',(7.91104465223491,-0.0159673076060156,
21.650732863045));
#240563=CARTESIAN_POINT('Ctrl Pts',(7.91092130081699,-0.0469740685472476,
21.6494557316463));
#240564=CARTESIAN_POINT('Ctrl Pts',(7.90594116408264,-0.552187211951711,
21.6284789904422));
#240565=CARTESIAN_POINT('Ctrl Pts',(7.85863612941356,-1.02497058752852,
21.6064852780704));
#240566=CARTESIAN_POINT('Ctrl Pts',(7.67751068385218,-1.96902258567539,
21.5613785362503));
#240567=CARTESIAN_POINT('Ctrl Pts',(7.54172299689951,-2.43797134772273,
21.5383768620033));
#240568=CARTESIAN_POINT('Ctrl Pts',(7.22822485254222,-3.23635152834974,
21.5000003508207));
#240569=CARTESIAN_POINT('Ctrl Pts',(7.06872916756617,-3.57131980832494,
21.4841453801161));
#240570=CARTESIAN_POINT('Ctrl Pts',(6.87625230642662,-3.91171235823119,
21.4683228537066));
#240571=CARTESIAN_POINT('Ctrl Pts',(6.86611562341367,-3.92947777822749,
21.4674978269409));
#240572=CARTESIAN_POINT('Ctrl Pts',(6.85126888633146,-3.95526512048715,
21.466301332907));
#240573=CARTESIAN_POINT('Ctrl Pts',(6.84661344438168,-3.96331829029176,
21.4659278304604));
#240574=CARTESIAN_POINT('Ctrl Pts',(6.83843837022138,-3.97740247107555,
21.4652748740868));
#240575=CARTESIAN_POINT('Ctrl Pts',(6.83492494136836,-3.98343705942763,
21.4649951889962));
#240576=CARTESIAN_POINT('Ctrl Pts',(6.82810266970285,-3.99511924421489,
21.464453915443));
#240577=CARTESIAN_POINT('Ctrl Pts',(6.82479479969096,-4.00076739962065,
21.4641922910071));
#240578=CARTESIAN_POINT('Ctrl Pts',(6.81690574877656,-4.01419962020725,
21.4635702769125));
#240579=CARTESIAN_POINT('Ctrl Pts',(6.81231823452317,-4.02197996649668,
21.4632101244152));
#240580=CARTESIAN_POINT('Ctrl Pts',(6.79599666540415,-4.04955303239049,
21.4619342402075));
#240581=CARTESIAN_POINT('Ctrl Pts',(6.78418954091072,-4.06930248606056,
21.4610212451497));
#240582=CARTESIAN_POINT('Ctrl Pts',(6.62266647098264,-4.33682071272996,
21.4486652021049));
#240583=CARTESIAN_POINT('Ctrl Pts',(6.45954090847352,-4.57625125008697,
21.4377470820495));
#240584=CARTESIAN_POINT('Ctrl Pts',(6.13496480416999,-5.00060190909944,
21.4183060161173));
#240585=CARTESIAN_POINT('Ctrl Pts',(5.97734070090344,-5.1879877640431,21.4096817891106));
#240586=CARTESIAN_POINT('Ctrl Pts',(5.50390402895874,-5.70054194215602,
21.3854245849952));
#240587=CARTESIAN_POINT('Ctrl Pts',(5.16852816703237,-6.00628181767911,
21.3701489956794));
#240588=CARTESIAN_POINT('Ctrl Pts',(4.62554652830653,-6.42195708805594,
21.3454416127073));
#240589=CARTESIAN_POINT('Ctrl Pts',(4.4361893134968,-6.55419258023866,21.3368069465427));
#240590=CARTESIAN_POINT('Ctrl Pts',(4.22056204148704,-6.69114201294729,
21.326699399606));
#240591=CARTESIAN_POINT('Ctrl Pts',(4.19974845360624,-6.7042254057345,21.3257216406511));
#240592=CARTESIAN_POINT('Ctrl Pts',(4.16310891011882,-6.72701939555684,
21.323997103028));
#240593=CARTESIAN_POINT('Ctrl Pts',(4.14730904376409,-6.73677173677074,
21.3232523632811));
#240594=CARTESIAN_POINT('Ctrl Pts',(4.12455559772059,-6.75070573765319,
21.3221784515565));
#240595=CARTESIAN_POINT('Ctrl Pts',(4.11762961466437,-6.75493250823952,
21.3218513737654));
#240596=CARTESIAN_POINT('Ctrl Pts',(4.10560263412475,-6.76224693163935,
21.3212830922317));
#240597=CARTESIAN_POINT('Ctrl Pts',(4.10050461781171,-6.76533949132353,
21.321042111575));
#240598=CARTESIAN_POINT('Ctrl Pts',(4.09069745398288,-6.77127355748216,
21.320578352336));
#240599=CARTESIAN_POINT('Ctrl Pts',(4.08598882880483,-6.77411592320258,
21.3203556123759));
#240600=CARTESIAN_POINT('Ctrl Pts',(4.07489255655459,-6.78079841915755,
21.3198305256301));
#240601=CARTESIAN_POINT('Ctrl Pts',(4.06850244610479,-6.78463443335356,
21.3195279979531));
#240602=CARTESIAN_POINT('Ctrl Pts',(4.04961328853411,-6.79593740371535,
21.3186333273905));
#240603=CARTESIAN_POINT('Ctrl Pts',(4.0370990743449,-6.80337886952804,21.3180400858648));
#240604=CARTESIAN_POINT('Ctrl Pts',(3.92584616496902,-6.86911937608084,
21.3127619211503));
#240605=CARTESIAN_POINT('Ctrl Pts',(3.82587388177438,-6.92529831198529,
21.3079899667837));
#240606=CARTESIAN_POINT('Ctrl Pts',(3.32852948085659,-7.1907221540629,21.2842108497175));
#240607=CARTESIAN_POINT('Ctrl Pts',(2.91506385306577,-7.3680378635069,21.264368070567));
#240608=CARTESIAN_POINT('Ctrl Pts',(1.90821527390292,-7.70173633795492,
21.2179821260291));
#240609=CARTESIAN_POINT('Ctrl Pts',(1.30722648202128,-7.82619369685106,
21.1918798392884));
#240610=CARTESIAN_POINT('Ctrl Pts',(0.659868975158418,-7.88352391502151,
21.1655687150648));
#240611=CARTESIAN_POINT('Ctrl Pts',(0.621844084298277,-7.88661437812317,
21.1640288870407));
#240612=CARTESIAN_POINT('Ctrl Pts',(0.566609848015124,-7.89070157449081,
21.1618002867522));
#240613=CARTESIAN_POINT('Ctrl Pts',(0.54941733552787,-7.89191729883797,
21.1611077483324));
#240614=CARTESIAN_POINT('Ctrl Pts',(0.519366456113566,-7.89394359452179,
21.1598992689248));
#240615=CARTESIAN_POINT('Ctrl Pts',(0.506509844379948,-7.89477895624264,
21.1593828905884));
#240616=CARTESIAN_POINT('Ctrl Pts',(0.481625998817894,-7.89633475535607,
21.1583846913591));
#240617=CARTESIAN_POINT('Ctrl Pts',(0.469599049334774,-7.89705913015734,
21.1579028011264));
#240618=CARTESIAN_POINT('Ctrl Pts',(0.440994627876495,-7.89871637793553,
21.15675803145));
#240619=CARTESIAN_POINT('Ctrl Pts',(0.424415764088776,-7.89962454440719,
21.156095602503));
#240620=CARTESIAN_POINT('Ctrl Pts',(0.374570164154309,-7.90219764570721,
21.1541071703505));
#240621=CARTESIAN_POINT('Ctrl Pts',(0.341295539876163,-7.90370468924481,
21.1527840834318));
#240622=CARTESIAN_POINT('Ctrl Pts',(-0.0430653294796413,-7.9186810113998,
21.137550164931));
#240623=CARTESIAN_POINT('Ctrl Pts',(-0.394673749012077,-7.90895805574895,
21.1241172264983));
#240624=CARTESIAN_POINT('Ctrl Pts',(-1.22661763511753,-7.83031644154327,
21.0929999943611));
#240625=CARTESIAN_POINT('Ctrl Pts',(-1.70352733113975,-7.74057019691383,
21.0757346401214));
#240626=CARTESIAN_POINT('Ctrl Pts',(-2.35957022404099,-7.55351072474762,
21.0505783273413));
#240627=CARTESIAN_POINT('Ctrl Pts',(-2.54780071400087,-7.49211599380507,
21.0431770401856));
#240628=CARTESIAN_POINT('Ctrl Pts',(-2.82831680165654,-7.38882596620705,
21.0316340986691));
#240629=CARTESIAN_POINT('Ctrl Pts',(-2.92243036539303,-7.3521102206016,
21.0276713870739));
#240630=CARTESIAN_POINT('Ctrl Pts',(-3.02777372924851,-7.30867119591772,
21.0231082142334));
#240631=CARTESIAN_POINT('Ctrl Pts',(-3.03972304191331,-7.30370948430901,
21.0225887320002));
#240632=CARTESIAN_POINT('Ctrl Pts',(-3.05762491173799,-7.29622455096867,
21.0218075861669));
#240633=CARTESIAN_POINT('Ctrl Pts',(-3.06358667334252,-7.29372329428451,
21.0215469649109));
#240634=CARTESIAN_POINT('Ctrl Pts',(-3.07382205823133,-7.28941427593686,
21.0210986838954));
#240635=CARTESIAN_POINT('Ctrl Pts',(-3.07809717625586,-7.28761005442125,
21.0209111948495));
#240636=CARTESIAN_POINT('Ctrl Pts',(-3.08688651943401,-7.28389158752044,
21.0205252096201));
#240637=CARTESIAN_POINT('Ctrl Pts',(-3.09140055723503,-7.28197690446732,
21.0203266921194));
#240638=CARTESIAN_POINT('Ctrl Pts',(-3.10224204459045,-7.27736646051384,
21.0198492208686));
#240639=CARTESIAN_POINT('Ctrl Pts',(-3.10856775602569,-7.27466664593997,
21.0195700671702));
#240640=CARTESIAN_POINT('Ctrl Pts',(-3.12788425322536,-7.26639256658187,
21.0187158886257));
#240641=CARTESIAN_POINT('Ctrl Pts',(-3.14086357467296,-7.26079174983371,
21.0181395319606));
#240642=CARTESIAN_POINT('Ctrl Pts',(-3.32727219984936,-7.17975962895686,
21.0098263157074));
#240643=CARTESIAN_POINT('Ctrl Pts',(-3.49793586214657,-7.0981770012961,
21.0017503046371));
#240644=CARTESIAN_POINT('Ctrl Pts',(-4.3628255608543,-6.64596714814462,
20.9588999972478));
#240645=CARTESIAN_POINT('Ctrl Pts',(-5.00188316938379,-6.17936010600693,
20.921150105005));
#240646=CARTESIAN_POINT('Ctrl Pts',(-5.79638767176517,-5.39396087513738,
20.8719180164918));
#240647=CARTESIAN_POINT('Ctrl Pts',(-6.0164388465983,-5.14737023493961,
20.8578863960726));
#240648=CARTESIAN_POINT('Ctrl Pts',(-6.23627549657994,-4.86759127089052,
20.843439056477));
#240649=CARTESIAN_POINT('Ctrl Pts',(-6.25200031230084,-4.84737753430764,
20.8424029459769));
#240650=CARTESIAN_POINT('Ctrl Pts',(-6.27415780221411,-4.81860762444148,
20.8409390696484));
#240651=CARTESIAN_POINT('Ctrl Pts',(-6.28067161431032,-4.81011430630571,
20.8405082368316));
#240652=CARTESIAN_POINT('Ctrl Pts',(-6.29183353018156,-4.79549902624557,
20.8397691288665));
#240653=CARTESIAN_POINT('Ctrl Pts',(-6.29648997761467,-4.78938347226887,
20.8394605394564));
#240654=CARTESIAN_POINT('Ctrl Pts',(-6.30534908190281,-4.77771310077262,
20.838872946654));
#240655=CARTESIAN_POINT('Ctrl Pts',(-6.30955332805746,-4.77215950263993,
20.838593883651));
#240656=CARTESIAN_POINT('Ctrl Pts',(-6.31932595889826,-4.75921485744452,
20.8379447176215));
#240657=CARTESIAN_POINT('Ctrl Pts',(-6.32488872616406,-4.75181957112347,
20.8375748253926));
#240658=CARTESIAN_POINT('Ctrl Pts',(-6.34381227697357,-4.72657001203405,
20.8363152275862));
#240659=CARTESIAN_POINT('Ctrl Pts',(-6.35711059236594,-4.70866894255109,
20.8354278577297));
#240660=CARTESIAN_POINT('Ctrl Pts',(-6.48670944749926,-4.53266412410689,
20.8267578671421));
#240661=CARTESIAN_POINT('Ctrl Pts',(-6.59716769700055,-4.37033501285362,
20.8191948236975));
#240662=CARTESIAN_POINT('Ctrl Pts',(-6.79249251988921,-4.05897749541245,
20.8053948962966));
#240663=CARTESIAN_POINT('Ctrl Pts',(-6.87877337749367,-3.91097596847907,
20.7991151281128));
#240664=CARTESIAN_POINT('Ctrl Pts',(-7.27285164837035,-3.18154810208835,
20.7692686341362));
#240665=CARTESIAN_POINT('Ctrl Pts',(-7.51209847467027,-2.56611210108341,
20.7475807677498));
#240666=CARTESIAN_POINT('Ctrl Pts',(-7.69850281660668,-1.82439868890262,
20.7201608877691));
#240667=CARTESIAN_POINT('Ctrl Pts',(-7.72247993861398,-1.72008104818995,
20.7162714700308));
#240668=CARTESIAN_POINT('Ctrl Pts',(-7.77886662927705,-1.44974476356953,
20.7060467822104));
#240669=CARTESIAN_POINT('Ctrl Pts',(-7.80808139873681,-1.28311773366718,
20.6995979093381));
#240670=CARTESIAN_POINT('Ctrl Pts',(-7.83641435877223,-1.08422341681566,
20.6916404810625));
#240671=CARTESIAN_POINT('Ctrl Pts',(-7.84070546545657,-1.05274317164936,
20.6903741640498));
#240672=CARTESIAN_POINT('Ctrl Pts',(-7.8461316237566,-1.0110612587017,20.6886891386515));
#240673=CARTESIAN_POINT('Ctrl Pts',(-7.84743665606868,-1.00088173822597,
20.688276965953));
#240674=CARTESIAN_POINT('Ctrl Pts',(-7.84954405022219,-0.984186113947172,
20.6875999053313));
#240675=CARTESIAN_POINT('Ctrl Pts',(-7.85035811775608,-0.977671481597511,
20.6873354546936));
#240676=CARTESIAN_POINT('Ctrl Pts',(-7.85191795538473,-0.96506120789022,
20.6868230643658));
#240677=CARTESIAN_POINT('Ctrl Pts',(-7.85266473937148,-0.958965694821149,
20.6865751620137));
#240678=CARTESIAN_POINT('Ctrl Pts',(-7.85436999721802,-0.944911218397947,
20.6860030619439));
#240679=CARTESIAN_POINT('Ctrl Pts',(-7.85532347176574,-0.936951662157876,
20.685678684521));
#240680=CARTESIAN_POINT('Ctrl Pts',(-7.85825297630143,-0.912177502636292,
20.6846679122884));
#240681=CARTESIAN_POINT('Ctrl Pts',(-7.86018712173715,-0.895358052431021,
20.6839800459206));
#240682=CARTESIAN_POINT('Ctrl Pts',(-7.87669600195275,-0.747618598424283,
20.677924197034));
#240683=CARTESIAN_POINT('Ctrl Pts',(-7.88805225089174,-0.616362931133154,
20.6724497875655));
#240684=CARTESIAN_POINT('Ctrl Pts',(-7.89678816775971,-0.474103779083254,
20.6664506830004));
#240685=CARTESIAN_POINT('Ctrl Pts',(-7.89742837317041,-0.463317223575977,
20.6659953998199));
#240686=CARTESIAN_POINT('Ctrl Pts',(-7.89965501296814,-0.424455429701931,
20.6643536841128));
#240687=CARTESIAN_POINT('Ctrl Pts',(-7.90111384649708,-0.396373191349824,
20.6631646787213));
#240688=CARTESIAN_POINT('Ctrl Pts',(-7.90320411514384,-0.351521415326295,
20.6612618393129));
#240689=CARTESIAN_POINT('Ctrl Pts',(-7.90393197432876,-0.334756528885346,
20.6605497382605));
#240690=CARTESIAN_POINT('Ctrl Pts',(-7.90652966255593,-0.270183001643106,
20.6578038828691));
#240691=CARTESIAN_POINT('Ctrl Pts',(-7.90801909469223,-0.222360306165593,
20.6557638993645));
#240692=CARTESIAN_POINT('Ctrl Pts',(-7.91035932368518,-0.116307885784508,
20.6512286090017));
#240693=CARTESIAN_POINT('Ctrl Pts',(-7.91100115241832,-0.058076311635061,
20.6487307575025));
#240694=CARTESIAN_POINT('Ctrl Pts',(-7.91098990207056,0.509701392572241,
20.6243222131824));
#240695=CARTESIAN_POINT('Ctrl Pts',(-7.86174935620109,1.01808176974271,
20.6021719372389));
#240696=CARTESIAN_POINT('Ctrl Pts',(-7.72218697327911,1.73179727208443,
20.5714613976149));
#240697=CARTESIAN_POINT('Ctrl Pts',(-7.67161952798435,1.94359224450184,
20.5623790039317));
#240698=CARTESIAN_POINT('Ctrl Pts',(-7.52853977103367,2.44947207946064,
20.5406577788275));
#240699=CARTESIAN_POINT('Ctrl Pts',(-7.42745184572128,2.74076434054692,
20.5280969872044));
#240700=CARTESIAN_POINT('Ctrl Pts',(-7.28674470831208,3.0807231404329,20.5131880115792));
#240701=CARTESIAN_POINT('Ctrl Pts',(-7.26322761146261,3.13576597123713,
20.5107675700267));
#240702=CARTESIAN_POINT('Ctrl Pts',(-7.22683103870119,3.21834705753255,
20.5071262829839));
#240703=CARTESIAN_POINT('Ctrl Pts',(-7.21441384196527,3.24608650047917,
20.5059014531776));
#240704=CARTESIAN_POINT('Ctrl Pts',(-7.19249609564274,3.29430272263465,
20.5037694715243));
#240705=CARTESIAN_POINT('Ctrl Pts',(-7.18306718945709,3.31481164908821,
20.5028616727524));
#240706=CARTESIAN_POINT('Ctrl Pts',(-7.16311649284448,3.35772178959058,
20.5009602886571));
#240707=CARTESIAN_POINT('Ctrl Pts',(-7.15257709330927,3.38011455939787,
20.4999668817465));
#240708=CARTESIAN_POINT('Ctrl Pts',(-7.12712478262492,3.43354026409209,
20.4975939258901));
#240709=CARTESIAN_POINT('Ctrl Pts',(-7.11211400439904,3.46452605875132,
20.4962153582619));
#240710=CARTESIAN_POINT('Ctrl Pts',(-7.05974677432867,3.57084971029093,
20.4914767851592));
#240711=CARTESIAN_POINT('Ctrl Pts',(-7.02139152913762,3.64568969192213,
20.488127152778));
#240712=CARTESIAN_POINT('Ctrl Pts',(-6.794709943032,4.07114602618178,20.4689938297933));
#240713=CARTESIAN_POINT('Ctrl Pts',(-6.58132920444999,4.4077692635504,20.4535252145148));
#240714=CARTESIAN_POINT('Ctrl Pts',(-6.07770338931803,5.0836360648932,20.4209235739589));
#240715=CARTESIAN_POINT('Ctrl Pts',(-5.78227693877506,5.4172948688147,20.4038682580775));
#240716=CARTESIAN_POINT('Ctrl Pts',(-5.43067096644422,5.75268811631658,
20.3844964289683));
#240717=CARTESIAN_POINT('Ctrl Pts',(-5.40073321443414,5.78080344028513,
20.3828533478669));
#240718=CARTESIAN_POINT('Ctrl Pts',(-5.36003351456923,5.81843346260337,
20.3806268234898));
#240719=CARTESIAN_POINT('Ctrl Pts',(-5.34946244625771,5.82815397619461,
20.3800491689768));
#240720=CARTESIAN_POINT('Ctrl Pts',(-5.33155952207037,5.84452667620866,
20.3790718879354));
#240721=CARTESIAN_POINT('Ctrl Pts',(-5.32424152873898,5.85119399347706,
20.3786727015414));
#240722=CARTESIAN_POINT('Ctrl Pts',(-5.31015726583092,5.86397766060507,
20.3779049480101));
#240723=CARTESIAN_POINT('Ctrl Pts',(-5.30339289395329,5.87009608130744,
20.3775364432053));
#240724=CARTESIAN_POINT('Ctrl Pts',(-5.28745394057272,5.88446293520925,
20.3766686488264));
#240725=CARTESIAN_POINT('Ctrl Pts',(-5.27827062417996,5.89270162371462,
20.3761690657088));
#240726=CARTESIAN_POINT('Ctrl Pts',(-5.25074663988041,5.91727843165131,
20.3746728468169));
#240727=CARTESIAN_POINT('Ctrl Pts',(-5.23234925248312,5.93355252751604,
20.3736741869352));
#240728=CARTESIAN_POINT('Ctrl Pts',(-5.20041874966383,5.96153386469735,
20.3719435995793));
#240729=CARTESIAN_POINT('Ctrl Pts',(-5.18692108728663,5.97328141160708,
20.371212872831));
#240730=CARTESIAN_POINT('Ctrl Pts',(-4.92616107393042,6.19868081592559,
20.3571131048857));
#240731=CARTESIAN_POINT('Ctrl Pts',(-4.6659401344634,6.39685080528621,20.3433501424095));
#240732=CARTESIAN_POINT('Ctrl Pts',(-4.22688785360173,6.69012952596437,
20.3210782471044));
#240733=CARTESIAN_POINT('Ctrl Pts',(-4.05535217828034,6.79547891472674,
20.3125871545781));
#240734=CARTESIAN_POINT('Ctrl Pts',(-3.66934621425892,7.01271999203399,
20.2940113076679));
#240735=CARTESIAN_POINT('Ctrl Pts',(-3.45338060462254,7.1215525131337,20.2839607745937));
#240736=CARTESIAN_POINT('Ctrl Pts',(-3.11605419996019,7.27258412732115,
20.2687891367996));
#240737=CARTESIAN_POINT('Ctrl Pts',(-2.99808990153073,7.32200323538005,
20.2635769678611));
#240738=CARTESIAN_POINT('Ctrl Pts',(-2.84418133791662,7.38213716835213,
20.2568896004129));
#240739=CARTESIAN_POINT('Ctrl Pts',(-2.80928855997919,7.39548608686989,
20.2553808606657));
#240740=CARTESIAN_POINT('Ctrl Pts',(-2.75336477497699,7.41642793229259,
20.2529741741643));
#240741=CARTESIAN_POINT('Ctrl Pts',(-2.73239394819534,7.42417969710052,
20.252074243437));
#240742=CARTESIAN_POINT('Ctrl Pts',(-2.6944823315391,7.43801115243769,20.2504518366645));
#240743=CARTESIAN_POINT('Ctrl Pts',(-2.67755313412428,7.44412212116101,
20.2497289782724));
#240744=CARTESIAN_POINT('Ctrl Pts',(-2.63761052865143,7.45838640624921,
20.2480272157248));
#240745=CARTESIAN_POINT('Ctrl Pts',(-2.61457991838856,7.46649107286388,
20.2470489118075));
#240746=CARTESIAN_POINT('Ctrl Pts',(-2.54709021940113,7.48989071556468,
20.2441903745017));
#240747=CARTESIAN_POINT('Ctrl Pts',(-2.50253174316113,7.50489616354739,
20.2423136242906));
#240748=CARTESIAN_POINT('Ctrl Pts',(-2.11147629759914,7.63271743287569,
20.2259297004352));
#240749=CARTESIAN_POINT('Ctrl Pts',(-1.75769280324902,7.72186717236216,
20.2116741168259));
#240750=CARTESIAN_POINT('Ctrl Pts',(-1.05124290684691,7.84880033087584,
20.183826940435));
#240751=CARTESIAN_POINT('Ctrl Pts',(-0.699659541783445,7.88791894207995,
20.1703455207084));
#240752=CARTESIAN_POINT('Ctrl Pts',(0.129790875696725,7.92429752897928,
20.1390689469837));
#240753=CARTESIAN_POINT('Ctrl Pts',(0.60711348199341,7.90207113504019,20.1215101104165));
#240754=CARTESIAN_POINT('Ctrl Pts',(1.2804445546505,7.80932282080689,20.0955806383408));
#240755=CARTESIAN_POINT('Ctrl Pts',(1.48023232260705,7.77392870705506,20.0877260389873));
#240756=CARTESIAN_POINT('Ctrl Pts',(1.69832461855102,7.72657937933853,20.078815728932));
#240757=CARTESIAN_POINT('Ctrl Pts',(1.7182015154207,7.72218356162564,20.0780005242406));
#240758=CARTESIAN_POINT('Ctrl Pts',(1.74688754589496,7.71572334644354,20.0768192951148));
#240759=CARTESIAN_POINT('Ctrl Pts',(1.75571053092691,7.71372046341466,20.0764553349855));
#240760=CARTESIAN_POINT('Ctrl Pts',(1.77119188624082,7.7101781435857,20.0758155446941));
#240761=CARTESIAN_POINT('Ctrl Pts',(1.77785174240546,7.70864520427608,20.0755399378421));
#240762=CARTESIAN_POINT('Ctrl Pts',(1.79153785927188,7.70547630867441,20.0749727708743));
#240763=CARTESIAN_POINT('Ctrl Pts',(1.79856388391593,7.70383936747289,20.0746811765623));
#240764=CARTESIAN_POINT('Ctrl Pts',(1.81638704340427,7.69966117077797,20.0739403733921));
#240765=CARTESIAN_POINT('Ctrl Pts',(1.82718107198305,7.69710681782101,20.0734906990327));
#240766=CARTESIAN_POINT('Ctrl Pts',(1.87004883197118,7.68686712228251,20.0717006473563));
#240767=CARTESIAN_POINT('Ctrl Pts',(1.90207947157292,7.67900400001702,20.070353777417));
#240768=CARTESIAN_POINT('Ctrl Pts',(2.46169666275869,7.53790878499424,20.046646234895));
#240769=CARTESIAN_POINT('Ctrl Pts',(2.97408131709752,7.35082264186398,20.021718839324));
#240770=CARTESIAN_POINT('Ctrl Pts',(3.63914852300124,7.02700920951749,19.9877996600801));
#240771=CARTESIAN_POINT('Ctrl Pts',(3.81195453103858,6.93478660606003,19.9788308465271));
#240772=CARTESIAN_POINT('Ctrl Pts',(4.40715840068742,6.58816312596132,19.9476401985171));
#240773=CARTESIAN_POINT('Ctrl Pts',(4.80907306980818,6.3007827118657,19.9261110866259));
#240774=CARTESIAN_POINT('Ctrl Pts',(5.20597165233274,5.95674536766719,19.9047430027069));
#240775=CARTESIAN_POINT('Ctrl Pts',(5.23015543593674,5.93552275436501,19.9034401261152));
#240776=CARTESIAN_POINT('Ctrl Pts',(5.26289629957581,5.90643535197804,19.9016749546935));
#240777=CARTESIAN_POINT('Ctrl Pts',(5.27156634752686,5.89869852359713,19.9012073983207));
#240778=CARTESIAN_POINT('Ctrl Pts',(5.28588804470872,5.88586157922251,19.9004348482886));
#240779=CARTESIAN_POINT('Ctrl Pts',(5.29154942121424,5.88077237055003,19.9001294034453));
#240780=CARTESIAN_POINT('Ctrl Pts',(5.30250135960793,5.87089867161536,19.8995384106328));
#240781=CARTESIAN_POINT('Ctrl Pts',(5.30779281242425,5.86611518312908,19.8992528214901));
#240782=CARTESIAN_POINT('Ctrl Pts',(5.32000810743495,5.85504246188589,19.8985934229701));
#240783=CARTESIAN_POINT('Ctrl Pts',(5.32692728560109,5.84874808727013,19.8982198288159));
#240784=CARTESIAN_POINT('Ctrl Pts',(5.34867987139071,5.82888914455127,19.897045036568));
#240785=CARTESIAN_POINT('Ctrl Pts',(5.36347280722148,5.81528025806648,19.8962456988135));
#240786=CARTESIAN_POINT('Ctrl Pts',(5.55471542991089,5.63799450291346,19.8859061386516));
#240787=CARTESIAN_POINT('Ctrl Pts',(5.72366545121628,5.4663983630254,19.8767136597119));
#240788=CARTESIAN_POINT('Ctrl Pts',(6.01433522197778,5.14289878850957,19.8606421727424));
#240789=CARTESIAN_POINT('Ctrl Pts',(6.13877234309855,4.99370752062864,19.8536635454289));
#240790=CARTESIAN_POINT('Ctrl Pts',(6.68840670977723,4.28310191560628,19.8220239499397));
#240791=CARTESIAN_POINT('Ctrl Pts',(7.04287989768205,3.67116140114844,19.7994587090832));
#240792=CARTESIAN_POINT('Ctrl Pts',(7.38858744289925,2.83430188987769,19.7663505689866));
#240793=CARTESIAN_POINT('Ctrl Pts',(7.45834846080899,2.64528243095303,19.7587173697232));
#240794=CARTESIAN_POINT('Ctrl Pts',(7.52510778228723,2.44066901551668,19.7501031695655));
#240795=CARTESIAN_POINT('Ctrl Pts',(7.529364245289,2.42750621741429,19.7495474851352));
#240796=CARTESIAN_POINT('Ctrl Pts',(7.5351873985636,2.40933588313313,19.7487782106013));
#240797=CARTESIAN_POINT('Ctrl Pts',(7.53678368682007,2.40433778555811,19.7485663786761));
#240798=CARTESIAN_POINT('Ctrl Pts',(7.53950948225137,2.39577372866259,19.7482030162123));
#240799=CARTESIAN_POINT('Ctrl Pts',(7.54064143641804,2.39220854425085,19.7480516322639));
#240800=CARTESIAN_POINT('Ctrl Pts',(7.54283997961578,2.38526698285068,19.7477566505204));
#240801=CARTESIAN_POINT('Ctrl Pts',(7.54390683117187,2.38189069020287,19.7476130686374));
#240802=CARTESIAN_POINT('Ctrl Pts',(7.5464548006046,2.37380818194039,19.7472690912954));
#240803=CARTESIAN_POINT('Ctrl Pts',(7.54793378186227,2.36910129936091,19.7470685665204));
#240804=CARTESIAN_POINT('Ctrl Pts',(7.55236531638669,2.3549515945079,19.7464651211991));
#240805=CARTESIAN_POINT('Ctrl Pts',(7.55530451978847,2.34550474263469,19.7460613899193));
#240806=CARTESIAN_POINT('Ctrl Pts',(7.58491040271362,2.24971580938813,19.7419589228398));
#240807=CARTESIAN_POINT('Ctrl Pts',(7.61011251564614,2.16293164540803,19.7381708867654));
#240808=CARTESIAN_POINT('Ctrl Pts',(7.70610953898764,1.80988899206583,19.7225352516025));
#240809=CARTESIAN_POINT('Ctrl Pts',(7.76445621658028,1.54046147382365,19.7100927972623));
#240810=CARTESIAN_POINT('Ctrl Pts',(7.85179929363146,1.00282120593915,19.6850298083011));
#240811=CARTESIAN_POINT('Ctrl Pts',(7.88137679948177,0.735052137332435,
19.6724368488032));
#240812=CARTESIAN_POINT('Ctrl Pts',(7.9327023936629,-0.134201643794408,
19.6320814850932));
#240813=CARTESIAN_POINT('Ctrl Pts',(7.8995584229053,-0.736869550851738,
19.6051076769524));
#240814=CARTESIAN_POINT('Ctrl Pts',(7.79288191539919,-1.36234608977134,
19.5792690619989));
#240815=CARTESIAN_POINT('Ctrl Pts',(7.78717026582562,-1.3946234987114,19.5779411194538));
#240816=CARTESIAN_POINT('Ctrl Pts',(7.77844040197462,-1.44223090068032,
19.575990409465));
#240817=CARTESIAN_POINT('Ctrl Pts',(7.77557715980859,-1.45758872585251,
19.5753623448484));
#240818=CARTESIAN_POINT('Ctrl Pts',(7.77115432439072,-1.48092795160832,
19.5744097190642));
#240819=CARTESIAN_POINT('Ctrl Pts',(7.76962789451794,-1.4889155491938,19.574084021512));
#240820=CARTESIAN_POINT('Ctrl Pts',(7.76686189660701,-1.50326955208913,
19.5734993185415));
#240821=CARTESIAN_POINT('Ctrl Pts',(7.76562681162257,-1.50963680734525,
19.5732401595628));
#240822=CARTESIAN_POINT('Ctrl Pts',(7.76319898613434,-1.52207119880334,
19.5727344614775));
#240823=CARTESIAN_POINT('Ctrl Pts',(7.76200696038873,-1.52813846874612,
19.5724878980501));
#240824=CARTESIAN_POINT('Ctrl Pts',(7.7586895288115,-1.54491977237181,19.571806453356));
#240825=CARTESIAN_POINT('Ctrl Pts',(7.75654904106625,-1.55563083101748,
19.5713720905621));
#240826=CARTESIAN_POINT('Ctrl Pts',(7.74794361033847,-1.59823329491209,
19.5696467546712));
#240827=CARTESIAN_POINT('Ctrl Pts',(7.741304066329,-1.63008933534529,19.5683617908376));
#240828=CARTESIAN_POINT('Ctrl Pts',(7.69805515450783,-1.83136893724368,
19.5602746442576));
#240829=CARTESIAN_POINT('Ctrl Pts',(7.65608133562765,-1.99959713998963,
19.5536597971191));
#240830=CARTESIAN_POINT('Ctrl Pts',(7.55758499850289,-2.34553917490843,
19.5402900474365));
#240831=CARTESIAN_POINT('Ctrl Pts',(7.50023952415913,-2.52290640362542,
19.5335663882337));
#240832=CARTESIAN_POINT('Ctrl Pts',(7.2970620125559,-3.08291992399194,19.5125484767092));
#240833=CARTESIAN_POINT('Ctrl Pts',(7.12777901090042,-3.4563393659593,19.4988903193199));
#240834=CARTESIAN_POINT('Ctrl Pts',(6.72646949039652,-4.18536610419681,
19.4707186353078));
#240835=CARTESIAN_POINT('Ctrl Pts',(6.49323210775315,-4.53878300446091,
19.4562236048039));
#240836=CARTESIAN_POINT('Ctrl Pts',(6.18342529954361,-4.93514221662879,
19.436907695107));
#240837=CARTESIAN_POINT('Ctrl Pts',(6.13298329429413,-4.99768868428522,
19.4337601095561));
#240838=CARTESIAN_POINT('Ctrl Pts',(6.07555114854313,-5.06672366219893,
19.4301593403808));
#240839=CARTESIAN_POINT('Ctrl Pts',(6.06949019508079,-5.07398257761095,
19.4297791355549));
#240840=CARTESIAN_POINT('Ctrl Pts',(6.06036919511765,-5.08486663782468,
19.4292066322581));
#240841=CARTESIAN_POINT('Ctrl Pts',(6.05731886417883,-5.08849994430902,
19.4290151129272));
#240842=CARTESIAN_POINT('Ctrl Pts',(6.05202012415163,-5.09479985699783,
19.4286823220164));
#240843=CARTESIAN_POINT('Ctrl Pts',(6.04977322970132,-5.09746770809901,
19.4285411729235));
#240844=CARTESIAN_POINT('Ctrl Pts',(6.04508707958194,-5.10302434791125,
19.4282467270026));
#240845=CARTESIAN_POINT('Ctrl Pts',(6.04264751654127,-5.10591287487736,
19.4280934055184));
#240846=CARTESIAN_POINT('Ctrl Pts',(6.03688645936826,-5.11272425403975,
19.4277312528581));
#240847=CARTESIAN_POINT('Ctrl Pts',(6.03356321438374,-5.11664561592186,
19.4275222821108));
#240848=CARTESIAN_POINT('Ctrl Pts',(6.02264114149838,-5.12950800419541,
19.4268352830302));
#240849=CARTESIAN_POINT('Ctrl Pts',(6.01502627570537,-5.1384353244905,19.4263559866161));
#240850=CARTESIAN_POINT('Ctrl Pts',(5.72222632904747,-5.48015784994654,
19.4079154140099));
#240851=CARTESIAN_POINT('Ctrl Pts',(5.40992645708177,-5.78866253848166,
19.3878720113857));
#240852=CARTESIAN_POINT('Ctrl Pts',(4.80768315451328,-6.29208633658248,
19.3512012394283));
#240853=CARTESIAN_POINT('Ctrl Pts',(4.52728564901074,-6.49675774905601,
19.3347707410609));
#240854=CARTESIAN_POINT('Ctrl Pts',(3.76992160943709,-6.97667045242813,
19.2932178707207));
#240855=CARTESIAN_POINT('Ctrl Pts',(3.27601230682214,-7.22178302922347,
19.2688527421055));
#240856=CARTESIAN_POINT('Ctrl Pts',(2.72690199471424,-7.42625204076528,
19.2449859721987));
#240857=CARTESIAN_POINT('Ctrl Pts',(2.69312042686586,-7.43856950458513,
19.24352938245));
#240858=CARTESIAN_POINT('Ctrl Pts',(2.64808853795734,-7.4546420898588,19.241603020218));
#240859=CARTESIAN_POINT('Ctrl Pts',(2.63691235046668,-7.45860274115461,
19.2411261774669));
#240860=CARTESIAN_POINT('Ctrl Pts',(2.61869056275803,-7.46501415817808,
19.2403507503374));
#240861=CARTESIAN_POINT('Ctrl Pts',(2.61165034658844,-7.46748010461694,
19.2400516453995));
#240862=CARTESIAN_POINT('Ctrl Pts',(2.59820613460645,-7.47216781323428,
19.2394813990162));
#240863=CARTESIAN_POINT('Ctrl Pts',(2.59180275285883,-7.47439130883709,
19.2392101984106));
#240864=CARTESIAN_POINT('Ctrl Pts',(2.57728878662772,-7.47941021109845,
19.238596403636));
#240865=CARTESIAN_POINT('Ctrl Pts',(2.56917649076423,-7.48220066260464,
19.2382539789761));
#240866=CARTESIAN_POINT('Ctrl Pts',(2.54462077387564,-7.49060264541635,
19.2372194063836));
#240867=CARTESIAN_POINT('Ctrl Pts',(2.52816333949308,-7.49617322427117,
19.2365286543539));
#240868=CARTESIAN_POINT('Ctrl Pts',(2.38525232641287,-7.544022154678,19.2305529327192));
#240869=CARTESIAN_POINT('Ctrl Pts',(2.25776368119933,-7.58315265857015,
19.2253755122488));
#240870=CARTESIAN_POINT('Ctrl Pts',(1.79856115802301,-7.71148892177604,
19.2072180163425));
#240871=CARTESIAN_POINT('Ctrl Pts',(1.46209740235628,-7.78229900855084,
19.1948372757722));
#240872=CARTESIAN_POINT('Ctrl Pts',(0.884241338001069,-7.86509801106841,
19.174360975963));
#240873=CARTESIAN_POINT('Ctrl Pts',(0.644971956958332,-7.8883244275455,
19.1661003967226));
#240874=CARTESIAN_POINT('Ctrl Pts',(-0.108863998888231,-7.92696893060566,
19.1400487451691));
#240875=CARTESIAN_POINT('Ctrl Pts',(-0.62409799557544,-7.9031135359761,
19.1222036195459));
#240876=CARTESIAN_POINT('Ctrl Pts',(-1.16636529533192,-7.82461662109957,
19.1004847108101));
#240877=CARTESIAN_POINT('Ctrl Pts',(-1.19934108394442,-7.81963005435704,
19.0991536354783));
#240878=CARTESIAN_POINT('Ctrl Pts',(-1.24279745333352,-7.8127772764407,
19.0973865960682));
#240879=CARTESIAN_POINT('Ctrl Pts',(-1.25330751389175,-7.81109816577966,
19.0969582339062));
#240880=CARTESIAN_POINT('Ctrl Pts',(-1.26958487790401,-7.80846395980715,
19.0962932922865));
#240881=CARTESIAN_POINT('Ctrl Pts',(-1.27535458897554,-7.80752366925352,
19.0960572996053));
#240882=CARTESIAN_POINT('Ctrl Pts',(-1.28688445695356,-7.80563152345428,
19.0955851191524));
#240883=CARTESIAN_POINT('Ctrl Pts',(-1.29264461309927,-7.80467968525813,
19.0953489321676));
#240884=CARTESIAN_POINT('Ctrl Pts',(-1.30547020447907,-7.80254572963671,
19.0948223921611));
#240885=CARTESIAN_POINT('Ctrl Pts',(-1.3125350937906,-7.80136039066242,
19.0945319151144));
#240886=CARTESIAN_POINT('Ctrl Pts',(-1.33309320821116,-7.79788245753654,
19.0936854021472));
#240887=CARTESIAN_POINT('Ctrl Pts',(-1.34658206838306,-7.79556444739808,
19.0931284037695));
#240888=CARTESIAN_POINT('Ctrl Pts',(-1.44242276225144,-7.77883840907748,
19.0891599073342));
#240889=CARTESIAN_POINT('Ctrl Pts',(-1.52454603434658,-7.76316103261057,
19.0857020721842));
#240890=CARTESIAN_POINT('Ctrl Pts',(-1.78714767343735,-7.70870271666713,
19.0744866456546));
#240891=CARTESIAN_POINT('Ctrl Pts',(-1.96651938767471,-7.66490650605838,
19.0665852701679));
#240892=CARTESIAN_POINT('Ctrl Pts',(-2.88209025194624,-7.40710109747689,
19.025403022942));
#240893=CARTESIAN_POINT('Ctrl Pts',(-3.58598658390007,-7.09313081695239,
18.9913388361158));
#240894=CARTESIAN_POINT('Ctrl Pts',(-4.36463843130316,-6.59983967931645,
18.9531377967241));
#240895=CARTESIAN_POINT('Ctrl Pts',(-4.49312749330956,-6.51304535230898,
18.9467948813139));
#240896=CARTESIAN_POINT('Ctrl Pts',(-4.64271044466376,-6.40546756260444,
18.9393474295766));
#240897=CARTESIAN_POINT('Ctrl Pts',(-4.66634028449643,-6.38827389307354,
18.9381689667992));
#240898=CARTESIAN_POINT('Ctrl Pts',(-4.70326282439339,-6.36109394598825,
18.9363244843165));
#240899=CARTESIAN_POINT('Ctrl Pts',(-4.71662019470146,-6.35119605479172,
18.9356565719948));
#240900=CARTESIAN_POINT('Ctrl Pts',(-4.74023279045556,-6.33358340709557,
18.9344747359603));
#240901=CARTESIAN_POINT('Ctrl Pts',(-4.75050061873216,-6.32588567355723,
18.933960439506));
#240902=CARTESIAN_POINT('Ctrl Pts',(-4.7717976364832,-6.30983832387473,
18.9328929208718));
#240903=CARTESIAN_POINT('Ctrl Pts',(-4.78282375079526,-6.30148469229766,
18.932339791111));
#240904=CARTESIAN_POINT('Ctrl Pts',(-4.81125227344537,-6.27982900612894,
18.9309125160287));
#240905=CARTESIAN_POINT('Ctrl Pts',(-4.8286214787523,-6.26648349600445,
18.9300393679856));
#240906=CARTESIAN_POINT('Ctrl Pts',(-4.90184838607415,-6.20973488010401,
18.9263535163539));
#240907=CARTESIAN_POINT('Ctrl Pts',(-4.95717850641239,-6.16565538576281,
18.9235568028503));
#240908=CARTESIAN_POINT('Ctrl Pts',(-5.32964480475741,-5.86066979694523,
18.9046463678356));
#240909=CARTESIAN_POINT('Ctrl Pts',(-5.62664578650971,-5.57615010463298,
18.8891988399541));
#240910=CARTESIAN_POINT('Ctrl Pts',(-6.30534442883819,-4.81626458508839,
18.8517593036166));
#240911=CARTESIAN_POINT('Ctrl Pts',(-6.65676723491854,-4.31753312438085,
18.8304109926013));
#240912=CARTESIAN_POINT('Ctrl Pts',(-6.95766242595286,-3.76500990253246,
18.805876122935));
#240913=CARTESIAN_POINT('Ctrl Pts',(-6.96767718657558,-3.74644372882379,
18.805050503328));
#240914=CARTESIAN_POINT('Ctrl Pts',(-6.99035917066659,-3.70398849964009,
18.803159395557));
#240915=CARTESIAN_POINT('Ctrl Pts',(-7.00297837366307,-3.68007418613781,
18.8020918923767));
#240916=CARTESIAN_POINT('Ctrl Pts',(-7.02484851386608,-3.63810881640134,
18.8002138855589));
#240917=CARTESIAN_POINT('Ctrl Pts',(-7.03415313349208,-3.62008592259415,
18.7994058204276));
#240918=CARTESIAN_POINT('Ctrl Pts',(-7.05008114190442,-3.58894036751498,
18.7980064651438));
#240919=CARTESIAN_POINT('Ctrl Pts',(-7.0567374837265,-3.57583460896057,
18.7974167391941));
#240920=CARTESIAN_POINT('Ctrl Pts',(-7.06639187030768,-3.55669401855285,
18.7965540609624));
#240921=CARTESIAN_POINT('Ctrl Pts',(-7.06941881737628,-3.55067373754263,
18.7962825217044));
#240922=CARTESIAN_POINT('Ctrl Pts',(-7.0747561871207,-3.5400243868076,18.7958018244254));
#240923=CARTESIAN_POINT('Ctrl Pts',(-7.0770697703803,-3.53539689870533,
18.7955928232146));
#240924=CARTESIAN_POINT('Ctrl Pts',(-7.08185201221599,-3.52580824557546,
18.795159489854));
#240925=CARTESIAN_POINT('Ctrl Pts',(-7.08432000015436,-3.52084675080762,
18.7949351243002));
#240926=CARTESIAN_POINT('Ctrl Pts',(-7.09064142553778,-3.50810498078884,
18.7943585444258));
#240927=CARTESIAN_POINT('Ctrl Pts',(-7.09448726444883,-3.50032096177427,
18.7940059456127));
#240928=CARTESIAN_POINT('Ctrl Pts',(-7.11024318364745,-3.4682981760712,
18.7925538329663));
#240929=CARTESIAN_POINT('Ctrl Pts',(-7.12204181289879,-3.44400504570947,
18.7914485824966));
#240930=CARTESIAN_POINT('Ctrl Pts',(-7.20093438722308,-3.27942772639249,
18.7839332811853));
#240931=CARTESIAN_POINT('Ctrl Pts',(-7.26399947844926,-3.13726111848784,
18.7773026052747));
#240932=CARTESIAN_POINT('Ctrl Pts',(-7.71112719486996,-2.04341882552673,
18.7256981864378));
#240933=CARTESIAN_POINT('Ctrl Pts',(-7.91094841064365,-1.02695608467868,
18.6757941483577));
#240934=CARTESIAN_POINT('Ctrl Pts',(-7.91099999001413,-0.000397487684091757,
18.632833427413));
#240935=CARTESIAN_POINT('',(-7.91112653880827,0.00440551095844195,16.642331508237));
#240936=CARTESIAN_POINT('Ctrl Pts',(-7.911,-5.77315972805081E-14,18.642331508237));
#240937=CARTESIAN_POINT('Ctrl Pts',(-7.91100000000002,2.20167589666668,
18.5537440725043));
#240938=CARTESIAN_POINT('Ctrl Pts',(-6.94214576672377,4.38610418338673,
18.4651566367716));
#240939=CARTESIAN_POINT('Ctrl Pts',(-3.67820201488301,7.34180684107624,
18.2879817653061));
#240940=CARTESIAN_POINT('Ctrl Pts',(-1.40868175871763,8.08992666571332,
18.1993943295734));
#240941=CARTESIAN_POINT('Ctrl Pts',(2.9730927052125,7.65454228025265,18.022219458108));
#240942=CARTESIAN_POINT('Ctrl Pts',(5.0510207267558,6.47444880834242,17.9336320223752));
#240943=CARTESIAN_POINT('Ctrl Pts',(7.66951518847859,2.93425195367738,17.7564571509098));
#240944=CARTESIAN_POINT('Ctrl Pts',(8.18956872247068,0.60188196009954,17.6678697151771));
#240945=CARTESIAN_POINT('Ctrl Pts',(7.32306689761362,-3.71537198232411,
17.4906948437116));
#240946=CARTESIAN_POINT('Ctrl Pts',(5.94329958850233,-5.66643518936477,
17.4021074079789));
#240947=CARTESIAN_POINT('Ctrl Pts',(2.16154501637897,-7.92205913232984,
17.2249325365134));
#240948=CARTESIAN_POINT('Ctrl Pts',(-0.210816529299819,-8.20894963713003,
17.1363451007807));
#240949=CARTESIAN_POINT('Ctrl Pts',(-4.42123908576386,-6.91982244717863,
16.9591702293153));
#240950=CARTESIAN_POINT('Ctrl Pts',(-6.22631625634146,-5.35390358803568,
16.8705827935825));
#240951=CARTESIAN_POINT('Ctrl Pts',(-7.6531728085948,-2.3133485751456,16.7354407413122));
#240952=CARTESIAN_POINT('Ctrl Pts',(-7.91100000000001,-1.15702837836537,
16.6888861247746));
#240953=CARTESIAN_POINT('Ctrl Pts',(-7.911,5.32907051820075E-14,16.642331508237));
#240954=CARTESIAN_POINT('',(-7.91918800173243,0.000313487325539099,14.6423316599192));
#240955=CARTESIAN_POINT('Ctrl Pts',(-7.91117084713064,0.00594812703317959,
16.642331508237));
#240956=CARTESIAN_POINT('Ctrl Pts',(-7.91495777771905,0.699069697383863,
16.6145091754524));
#240957=CARTESIAN_POINT('Ctrl Pts',(-7.5015571643441,4.02599103967887,16.4807172654514));
#240958=CARTESIAN_POINT('Ctrl Pts',(-3.89567832531485,7.80704314161589,
16.2939405668419));
#240959=CARTESIAN_POINT('Ctrl Pts',(1.56115343882902,8.08629267461694,16.0820014124088));
#240960=CARTESIAN_POINT('Ctrl Pts',(5.24511136736693,6.37222732002422,15.9230470465842));
#240961=CARTESIAN_POINT('Ctrl Pts',(7.6385445361554,3.07862117984459,15.7640926807593));
#240962=CARTESIAN_POINT('Ctrl Pts',(8.40705311350932,-2.31605264250739,
15.5521535263265));
#240963=CARTESIAN_POINT('Ctrl Pts',(4.12950229334074,-8.39726041388267,
15.287229583285));
#240964=CARTESIAN_POINT('Ctrl Pts',(-4.85377709130171,-8.00864403078137,
14.9693208516356));
#240965=CARTESIAN_POINT('Ctrl Pts',(-7.87757738652791,-2.77203907481525,
14.7543548828771));
#240966=CARTESIAN_POINT('Ctrl Pts',(-7.92006828996515,-0.0745985010899101,
14.6453584913352));
#240967=CARTESIAN_POINT('Ctrl Pts',(-7.92011057934193,0.000313101301251344,
14.6423316770099));
#240968=CARTESIAN_POINT('',(-7.90467196448321,-0.00677022214583101,12.642331508237));
#240969=CARTESIAN_POINT('Ctrl Pts',(-7.91099999365225,0.000316913346238894,
14.642331508237));
#240970=CARTESIAN_POINT('Ctrl Pts',(-7.91099160947722,0.209608220964732,
14.6338653232035));
#240971=CARTESIAN_POINT('Ctrl Pts',(-7.9026734681258,0.419065023665548,
14.62539913817));
#240972=CARTESIAN_POINT('Ctrl Pts',(-7.88603207588891,0.62802794368667,
14.6169329531365));
#240973=CARTESIAN_POINT('Ctrl Pts',(-7.86941516844141,0.836683412683476,
14.6084792245583));
#240974=CARTESIAN_POINT('Ctrl Pts',(-7.84449946276681,1.0448461810492,14.60002549598));
#240975=CARTESIAN_POINT('Ctrl Pts',(-7.81132342387363,1.25185756683547,
14.5915717674017));
#240976=CARTESIAN_POINT('Ctrl Pts',(-7.77822011466537,1.45841513494589,
14.583136571386));
#240977=CARTESIAN_POINT('Ctrl Pts',(-7.73689265527382,1.66382609268568,
14.5747013753703));
#240978=CARTESIAN_POINT('Ctrl Pts',(-7.68743107903436,1.86743792536636,
14.5662661793546));
#240979=CARTESIAN_POINT('Ctrl Pts',(-7.63803532221137,2.07077880808887,
14.5578422082072));
#240980=CARTESIAN_POINT('Ctrl Pts',(-7.5805271015822,2.27232508058972,14.5494182370598));
#240981=CARTESIAN_POINT('Ctrl Pts',(-7.51504765843897,2.47143272038529,
14.5409942659124));
#240982=CARTESIAN_POINT('Ctrl Pts',(-7.44970173420307,2.67013436047726,
14.5325874720556));
#240983=CARTESIAN_POINT('Ctrl Pts',(-7.37641710833143,2.86640703628315,
14.5241806781988));
#240984=CARTESIAN_POINT('Ctrl Pts',(-7.29538505604854,3.05962054575133,
14.515773884342));
#240985=CARTESIAN_POINT('Ctrl Pts',(-7.2204712854315,3.23824557277003,14.5080018409484));
#240986=CARTESIAN_POINT('Ctrl Pts',(-7.13893640916405,3.41425589335646,
14.5002297975548));
#240987=CARTESIAN_POINT('Ctrl Pts',(-7.05096979243143,3.58716405900532,
14.4924577541612));
#240988=CARTESIAN_POINT('Ctrl Pts',(-6.96161669767182,3.76279750137008,
14.4845632123951));
#240989=CARTESIAN_POINT('Ctrl Pts',(-6.86570200825127,3.93508139648814,
14.476668670629));
#240990=CARTESIAN_POINT('Ctrl Pts',(-6.76351680122221,4.10350599848287,
14.4687741288628));
#240991=CARTESIAN_POINT('Ctrl Pts',(-6.66130856596594,4.27196855626507,
14.4608778080006));
#240992=CARTESIAN_POINT('Ctrl Pts',(-6.55282717441282,4.43656979476182,
14.4529814871384));
#240993=CARTESIAN_POINT('Ctrl Pts',(-6.43840766156614,4.59682801325941,
14.4450851662761));
#240994=CARTESIAN_POINT('Ctrl Pts',(-6.3239434998463,4.75714876784627,14.4371857641053));
#240995=CARTESIAN_POINT('Ctrl Pts',(-6.20353679781398,4.91312284650394,
14.4292863619345));
#240996=CARTESIAN_POINT('Ctrl Pts',(-6.07756374070671,5.06430054179717,
14.4213869597637));
#240997=CARTESIAN_POINT('Ctrl Pts',(-5.95145206467407,5.21564459083414,
14.4134788652053));
#240998=CARTESIAN_POINT('Ctrl Pts',(-5.81976201597311,5.36218144894817,
14.4055707706468));
#240999=CARTESIAN_POINT('Ctrl Pts',(-5.68290844638268,5.50349639684014,
14.3976626760884));
#241000=CARTESIAN_POINT('Ctrl Pts',(-5.54597334162283,5.64489553791941,
14.3897498700137));
#241001=CARTESIAN_POINT('Ctrl Pts',(-5.40386882865687,5.78106632889452,
14.3818370639389));
#241002=CARTESIAN_POINT('Ctrl Pts',(-5.25704413753824,5.91163327143817,
14.3739242578641));
#241003=CARTESIAN_POINT('Ctrl Pts',(-5.11001369598899,6.04238318187674,
14.3660003633052));
#241004=CARTESIAN_POINT('Ctrl Pts',(-4.95825012312907,6.16751333505882,
14.3580764687463));
#241005=CARTESIAN_POINT('Ctrl Pts',(-4.80223411572721,6.28668978857282,
14.3501525741874));
#241006=CARTESIAN_POINT('Ctrl Pts',(-4.69296379485831,6.3701584629246,14.3446028455705));
#241007=CARTESIAN_POINT('Ctrl Pts',(-4.58160814846415,6.45070756604176,
14.3390531169535));
#241008=CARTESIAN_POINT('Ctrl Pts',(-4.4683397720312,6.5282356484493,14.3335033883366));
#241009=CARTESIAN_POINT('Ctrl Pts',(-4.30252118821672,6.64173243577439,
14.3253788952627));
#241010=CARTESIAN_POINT('Ctrl Pts',(-4.13223745152282,6.74900267259293,
14.3172544021888));
#241011=CARTESIAN_POINT('Ctrl Pts',(-3.95798447766342,6.84969195472143,
14.3091299091149));
#241012=CARTESIAN_POINT('Ctrl Pts',(-3.7838854558489,6.95029227813353,14.3010125940094));
#241013=CARTESIAN_POINT('Ctrl Pts',(-3.60582446489278,7.04432307928305,
14.2928952789038));
#241014=CARTESIAN_POINT('Ctrl Pts',(-3.4243263340565,7.13147321090721,14.2847779637982));
#241015=CARTESIAN_POINT('Ctrl Pts',(-3.24296271382359,7.21855875444589,
14.2766666645394));
#241016=CARTESIAN_POINT('Ctrl Pts',(-3.05816732094315,7.2987736578556,14.2685553652807));
#241017=CARTESIAN_POINT('Ctrl Pts',(-2.87049002626376,7.37185241368276,
14.2604440660219));
#241018=CARTESIAN_POINT('Ctrl Pts',(-2.68292513480602,7.44488740136202,
14.2523376247624));
#241019=CARTESIAN_POINT('Ctrl Pts',(-2.49248208156313,7.51079464820408,
14.244231183503));
#241020=CARTESIAN_POINT('Ctrl Pts',(-2.29973171106852,7.56935631722446,
14.2361247422435));
#241021=CARTESIAN_POINT('Ctrl Pts',(-2.10706940378885,7.627891230764,14.2280220046308));
#241022=CARTESIAN_POINT('Ctrl Pts',(-1.91210218797431,7.67908716653114,
14.2199192670181));
#241023=CARTESIAN_POINT('Ctrl Pts',(-1.71541765013888,7.72277562056493,
14.2118165294053));
#241024=CARTESIAN_POINT('Ctrl Pts',(-1.51695690455812,7.76685861385071,
14.2036406180421));
#241025=CARTESIAN_POINT('Ctrl Pts',(-1.31674797921391,7.80329775242719,
14.1954647066788));
#241026=CARTESIAN_POINT('Ctrl Pts',(-1.11540787354316,7.83197205534072,
14.1872887953156));
#241027=CARTESIAN_POINT('Ctrl Pts',(-0.915945814777616,7.86037889199031,
14.1791891466769));
#241028=CARTESIAN_POINT('Ctrl Pts',(-0.715373913618147,7.88116510167342,
14.1710894980383));
#241029=CARTESIAN_POINT('Ctrl Pts',(-0.514300307894198,7.89426476584742,
14.1629898493996));
#241030=CARTESIAN_POINT('Ctrl Pts',(-0.313228068651659,7.90736434099706,
14.1548902558056));
#241031=CARTESIAN_POINT('Ctrl Pts',(-0.111654451680012,7.91277745408288,
14.1467906622115));
#241032=CARTESIAN_POINT('Ctrl Pts',(0.0898090014107483,7.91049020878388,
14.1386910686175));
#241033=CARTESIAN_POINT('Ctrl Pts',(0.291297095913608,7.90820268372717,
14.1305904843454));
#241034=CARTESIAN_POINT('Ctrl Pts',(0.492674678992804,7.89821292611473,
14.1224899000733));
#241035=CARTESIAN_POINT('Ctrl Pts',(0.693331375740398,7.88055915550502,
14.1143893158012));
#241036=CARTESIAN_POINT('Ctrl Pts',(0.897265327583533,7.86261705208298,
14.1061564275417));
#241037=CARTESIAN_POINT('Ctrl Pts',(1.10045429902011,7.83675844239101,14.0979235392822));
#241038=CARTESIAN_POINT('Ctrl Pts',(1.30226408393771,7.80307819105293,14.0896906510227));
#241039=CARTESIAN_POINT('Ctrl Pts',(1.50102036219682,7.76990754271434,14.0815823314461));
#241040=CARTESIAN_POINT('Ctrl Pts',(1.69843858236954,7.72915036219104,14.0734740118696));
#241041=CARTESIAN_POINT('Ctrl Pts',(1.89392397681129,7.68094870247545,14.065365692293));
#241042=CARTESIAN_POINT('Ctrl Pts',(2.09391425501415,7.63163625453585,14.057070519692));
#241043=CARTESIAN_POINT('Ctrl Pts',(2.29188120657217,7.57453217548862,14.048775347091));
#241044=CARTESIAN_POINT('Ctrl Pts',(2.48720496812253,7.50984237161784,14.04048017449));
#241045=CARTESIAN_POINT('Ctrl Pts',(2.68252872967288,7.44515256774706,14.032185001889));
#241046=CARTESIAN_POINT('Ctrl Pts',(2.87520897606093,7.37287718975586,14.023889829288));
#241047=CARTESIAN_POINT('Ctrl Pts',(3.06464797065199,7.2932745605783,14.015594656687));
#241048=CARTESIAN_POINT('Ctrl Pts',(3.24341785300369,7.21815511284434,14.0077666641812));
#241049=CARTESIAN_POINT('Ctrl Pts',(3.41964401130501,7.13636638325002,13.9999386716753));
#241050=CARTESIAN_POINT('Ctrl Pts',(3.5927892581542,7.04810516000519,13.9921106791695));
#241051=CARTESIAN_POINT('Ctrl Pts',(3.76578826356659,6.95991848369906,13.9842892983201));
#241052=CARTESIAN_POINT('Ctrl Pts',(3.93571122723641,6.86527035761309,13.9764679174706));
#241053=CARTESIAN_POINT('Ctrl Pts',(4.10204015953403,6.76440592584227,13.9686465366211));
#241054=CARTESIAN_POINT('Ctrl Pts',(4.26825798031597,6.66360887380953,13.9608303806322));
#241055=CARTESIAN_POINT('Ctrl Pts',(4.43088625131069,6.5566039679859,13.9530142246434));
#241056=CARTESIAN_POINT('Ctrl Pts',(4.58943072520149,6.44368269071162,13.9451980686545));
#241057=CARTESIAN_POINT('Ctrl Pts',(4.74789903371938,6.33081566125173,13.9373856675769));
#241058=CARTESIAN_POINT('Ctrl Pts',(4.90228716674321,6.21203812559488,13.9295732664993));
#241059=CARTESIAN_POINT('Ctrl Pts',(5.05212892981133,6.087685461369,13.9217608654217));
#241060=CARTESIAN_POINT('Ctrl Pts',(5.20192689577287,5.96336914406521,13.9139507478234));
#241061=CARTESIAN_POINT('Ctrl Pts',(5.34718086868082,5.83348116963574,13.9061406302251));
#241062=CARTESIAN_POINT('Ctrl Pts',(5.48745675924078,5.69839796043262,13.8983305126268));
#241063=CARTESIAN_POINT('Ctrl Pts',(5.62774064229124,5.56330705460207,13.8905199500319));
#241064=CARTESIAN_POINT('Ctrl Pts',(5.76304561808925,5.42302056223409,13.882709387437));
#241065=CARTESIAN_POINT('Ctrl Pts',(5.89297326897815,5.27795292240363,13.8748988248421));
#241066=CARTESIAN_POINT('Ctrl Pts',(5.99421601557345,5.16491273274382,13.8688126468488));
#241067=CARTESIAN_POINT('Ctrl Pts',(6.09219438355787,5.04897027525893,13.8627264688555));
#241068=CARTESIAN_POINT('Ctrl Pts',(6.18673635657413,4.93033611980399,13.8566402908622));
#241069=CARTESIAN_POINT('Ctrl Pts',(6.32095478386334,4.76191473763961,13.8479999249761));
#241070=CARTESIAN_POINT('Ctrl Pts',(6.44818247280803,4.58814793997287,13.8393595590899));
#241071=CARTESIAN_POINT('Ctrl Pts',(6.56804077931242,4.40962144875148,13.8307191932037));
#241072=CARTESIAN_POINT('Ctrl Pts',(6.68809846894754,4.23079798044293,13.8220644541526));
#241073=CARTESIAN_POINT('Ctrl Pts',(6.80076214391928,4.04719918287814,13.8134097151016));
#241074=CARTESIAN_POINT('Ctrl Pts',(6.90569788511941,3.85943748744002,13.8047549760505));
#241075=CARTESIAN_POINT('Ctrl Pts',(7.01387917710065,3.66586852261663,13.7958325551328));
#241076=CARTESIAN_POINT('Ctrl Pts',(7.11384676695315,3.46787530176986,13.786910134215));
#241077=CARTESIAN_POINT('Ctrl Pts',(7.20528795746181,3.26615162692362,13.7779877132972));
#241078=CARTESIAN_POINT('Ctrl Pts',(7.29428345054031,3.06982327852086,13.7693039325567));
#241079=CARTESIAN_POINT('Ctrl Pts',(7.37520271079234,2.86996167315181,13.7606201518162));
#241080=CARTESIAN_POINT('Ctrl Pts',(7.44780754301474,2.66722398800941,13.7519363710757));
#241081=CARTESIAN_POINT('Ctrl Pts',(7.52340527036207,2.45612910940026,13.7428946300693));
#241082=CARTESIAN_POINT('Ctrl Pts',(7.58998853841794,2.24191630478465,13.7338528890629));
#241083=CARTESIAN_POINT('Ctrl Pts',(7.64734627763182,2.02534340544778,13.7248111480566));
#241084=CARTESIAN_POINT('Ctrl Pts',(7.7047040168457,1.80877050611091,13.7157694070502));
#241085=CARTESIAN_POINT('Ctrl Pts',(7.75283618695792,1.58983778856473,13.7067276660438));
#241086=CARTESIAN_POINT('Ctrl Pts',(7.79159140450717,1.36931529795366,13.6976859250375));
#241087=CARTESIAN_POINT('Ctrl Pts',(7.82726160143207,1.16634699680898,13.6893639311838));
#241088=CARTESIAN_POINT('Ctrl Pts',(7.85501855400681,0.961859510919619,
13.6810419373302));
#241089=CARTESIAN_POINT('Ctrl Pts',(7.87474800181552,0.756481928338384,
13.6727199434766));
#241090=CARTESIAN_POINT('Ctrl Pts',(7.89445990191067,0.551287012146152,
13.6644053513488));
#241091=CARTESIAN_POINT('Ctrl Pts',(7.90615851249631,0.345203868562909,
13.6560907592211));
#241092=CARTESIAN_POINT('Ctrl Pts',(7.90978105619522,0.13886915804202,13.6477761670933));
#241093=CARTESIAN_POINT('Ctrl Pts',(7.91340059886103,-0.0672946180895682,
13.6394684630443));
#241094=CARTESIAN_POINT('Ctrl Pts',(7.90895741685068,-0.273709253870452,
13.6311607589952));
#241095=CARTESIAN_POINT('Ctrl Pts',(7.89644068938977,-0.479734758954975,
13.6228530549462));
#241096=CARTESIAN_POINT('Ctrl Pts',(7.88393659074577,-0.685552393540713,
13.6145537329981));
#241097=CARTESIAN_POINT('Ctrl Pts',(7.8633752240688,-0.890981390013255,
13.60625441105));
#241098=CARTESIAN_POINT('Ctrl Pts',(7.83479781068352,-1.095383159314,13.5979550891019));
#241099=CARTESIAN_POINT('Ctrl Pts',(7.80623865543539,-1.29965433612594,
13.5896610695987));
#241100=CARTESIAN_POINT('Ctrl Pts',(7.76967370946852,-1.50289930603503,
13.5813670500955));
#241101=CARTESIAN_POINT('Ctrl Pts',(7.72519601193587,-1.70448454882117,
13.5730730305923));
#241102=CARTESIAN_POINT('Ctrl Pts',(7.68075129684107,-1.90592030606487,
13.5647851615194));
#241103=CARTESIAN_POINT('Ctrl Pts',(7.6284056039201,-2.10569850763858,13.5564972924466));
#241104=CARTESIAN_POINT('Ctrl Pts',(7.56830315791786,-2.30319523919501,
13.5482094233737));
#241105=CARTESIAN_POINT('Ctrl Pts',(7.54539245095782,-2.37847985809532,
13.5450501353201));
#241106=CARTESIAN_POINT('Ctrl Pts',(7.52135514613833,-2.45343306631481,
13.5418908472664));
#241107=CARTESIAN_POINT('Ctrl Pts',(7.49620117606039,-2.52802075308548,
13.5387315592127));
#241108=CARTESIAN_POINT('Ctrl Pts',(7.43169130684809,-2.71930832731386,
13.530629249378));
#241109=CARTESIAN_POINT('Ctrl Pts',(7.3598604819201,-2.90811028686713,13.5225269395432));
#241110=CARTESIAN_POINT('Ctrl Pts',(7.28093271431342,-3.09385516946747,
13.5144246297084));
#241111=CARTESIAN_POINT('Ctrl Pts',(7.20198752547956,-3.27964105036152,
13.5063205315021));
#241112=CARTESIAN_POINT('Ctrl Pts',(7.11594239453415,-3.46236821501396,
13.4982164332957));
#241113=CARTESIAN_POINT('Ctrl Pts',(7.02306894780017,-3.64148644847747,
13.4901123350893));
#241114=CARTESIAN_POINT('Ctrl Pts',(6.93016335187538,-3.82066668573718,
13.4820054315579));
#241115=CARTESIAN_POINT('Ctrl Pts',(6.83042487268483,-3.99623521722305,
13.4738985280265));
#241116=CARTESIAN_POINT('Ctrl Pts',(6.72417070117546,-4.16766713899437,
13.4657916244951));
#241117=CARTESIAN_POINT('Ctrl Pts',(6.61782070445251,-4.33925366646526,
13.4576774097613));
#241118=CARTESIAN_POINT('Ctrl Pts',(6.50494344117653,-4.50669585802107,
13.4495631950274));
#241119=CARTESIAN_POINT('Ctrl Pts',(6.38589973895333,-4.66949735239628,
13.4414489802936));
#241120=CARTESIAN_POINT('Ctrl Pts',(6.26679785622839,-4.83237841311937,
13.4333307998809));
#241121=CARTESIAN_POINT('Ctrl Pts',(6.14152371665662,-4.99061399937773,
13.4252126194683));
#241122=CARTESIAN_POINT('Ctrl Pts',(6.01047851030768,-5.14374076690588,
13.4170944390557));
#241123=CARTESIAN_POINT('Ctrl Pts',(5.87929237717569,-5.29703220785743,
13.4089675283042));
#241124=CARTESIAN_POINT('Ctrl Pts',(5.74232298845278,-5.44520361406672,
13.4008406175528));
#241125=CARTESIAN_POINT('Ctrl Pts',(5.60000942884617,-5.58782743083875,
13.3927137068013));
#241126=CARTESIAN_POINT('Ctrl Pts',(5.52449728862179,-5.66350419474794,
13.3884015356635));
#241127=CARTESIAN_POINT('Ctrl Pts',(5.44748114347228,-5.73761973610153,
13.3840893645257));
#241128=CARTESIAN_POINT('Ctrl Pts',(5.36903041219186,-5.81011475213347,
13.3797771933879));
#241129=CARTESIAN_POINT('Ctrl Pts',(5.22352776130406,-5.94457133190829,
13.3717794052043));
#241130=CARTESIAN_POINT('Ctrl Pts',(5.07283573485256,-6.07368435372215,
13.3637816170206));
#241131=CARTESIAN_POINT('Ctrl Pts',(4.91737977091784,-6.19703938897987,
13.355783828837));
#241132=CARTESIAN_POINT('Ctrl Pts',(4.76205073661163,-6.32029370498307,
13.3477925708389));
#241133=CARTESIAN_POINT('Ctrl Pts',(4.60196577737757,-6.43779919678073,
13.3398013128408));
#241134=CARTESIAN_POINT('Ctrl Pts',(4.437585495946,-6.54917979339166,13.3318100548426));
#241135=CARTESIAN_POINT('Ctrl Pts',(4.273311556453,-6.66048833495768,13.3238239666));
#241136=CARTESIAN_POINT('Ctrl Pts',(4.10474810912281,-6.76567969161241,
13.3158378783574));
#241137=CARTESIAN_POINT('Ctrl Pts',(3.93238732758968,-6.86441919653893,
13.3078517901148));
#241138=CARTESIAN_POINT('Ctrl Pts',(3.76010883571297,-6.96311156057955,
13.2998695146447));
#241139=CARTESIAN_POINT('Ctrl Pts',(3.58403691314571,-7.05535804693963,
13.2918872391747));
#241140=CARTESIAN_POINT('Ctrl Pts',(3.40469144528709,-7.14086809585424,
13.2839049637046));
#241141=CARTESIAN_POINT('Ctrl Pts',(3.22540121283494,-7.22635180910302,
13.275925146642));
#241142=CARTESIAN_POINT('Ctrl Pts',(3.04283974672231,-7.30510307728589,
13.2679453295794));
#241143=CARTESIAN_POINT('Ctrl Pts',(2.85755055253053,-7.37687778397694,
13.2599655125168));
#241144=CARTESIAN_POINT('Ctrl Pts',(2.66589388806462,-7.45111903121981,
13.2517114687343));
#241145=CARTESIAN_POINT('Ctrl Pts',(2.47131902410358,-7.51789553407416,
13.2434574249519));
#241146=CARTESIAN_POINT('Ctrl Pts',(2.27444941787763,-7.57699154318626,
13.2352033811695));
#241147=CARTESIAN_POINT('Ctrl Pts',(2.08409473330921,-7.63413191335023,
13.2272224849268));
#241148=CARTESIAN_POINT('Ctrl Pts',(1.89159509497252,-7.68409190491757,
13.2192415886842));
#241149=CARTESIAN_POINT('Ctrl Pts',(1.69752906883348,-7.72672738359943,
13.2112606924416));
#241150=CARTESIAN_POINT('Ctrl Pts',(1.50341995755849,-7.769372327902,13.203278024338));
#241151=CARTESIAN_POINT('Ctrl Pts',(1.30774409210163,-7.80468944529393,
13.1952953562345));
#241152=CARTESIAN_POINT('Ctrl Pts',(1.11109022321741,-7.83258574902763,
13.187312688131));
#241153=CARTESIAN_POINT('Ctrl Pts',(0.914362465654845,-7.86049253422821,
13.1793270207028));
#241154=CARTESIAN_POINT('Ctrl Pts',(0.716656303351637,-7.88097290013038,
13.1713413532747));
#241155=CARTESIAN_POINT('Ctrl Pts',(0.518565978983622,-7.89398570593086,
13.1633556858465));
#241156=CARTESIAN_POINT('Ctrl Pts',(0.320370771139717,-7.90700540166051,
13.1553657902231));
#241157=CARTESIAN_POINT('Ctrl Pts',(0.121791329243065,-7.91254963283518,
13.1473758945998));
#241158=CARTESIAN_POINT('Ctrl Pts',(-0.0765773490314934,-7.91062936242214,
13.1393859989764));
#241159=CARTESIAN_POINT('Ctrl Pts',(-0.275181011409237,-7.90870681729001,
13.131386638661));
#241160=CARTESIAN_POINT('Ctrl Pts',(-0.473573076801867,-7.89930211007153,
13.1233872783456));
#241161=CARTESIAN_POINT('Ctrl Pts',(-0.671161645071544,-7.88247822998484,
13.1153879180301));
#241162=CARTESIAN_POINT('Ctrl Pts',(-0.868888338898598,-7.86564258905674,
13.1073829657105));
#241163=CARTESIAN_POINT('Ctrl Pts',(-1.06581008426671,-7.84137747212006,
13.0993780133909));
#241164=CARTESIAN_POINT('Ctrl Pts',(-1.26134392584015,-7.80979721252391,
13.0913730610712));
#241165=CARTESIAN_POINT('Ctrl Pts',(-1.45713295507633,-7.77817573810493,
13.0833576616338));
#241166=CARTESIAN_POINT('Ctrl Pts',(-1.65153013554003,-7.73922011694579,
13.0753422621964));
#241167=CARTESIAN_POINT('Ctrl Pts',(-1.84396530479523,-7.69309514790448,
13.067326862759));
#241168=CARTESIAN_POINT('Ctrl Pts',(-1.88764740001141,-7.68262494488855,
13.0655073957521));
#241169=CARTESIAN_POINT('Ctrl Pts',(-1.93122847039918,-7.6717855238411,
13.0636879287453));
#241170=CARTESIAN_POINT('Ctrl Pts',(-1.97470198113393,-7.6605791612453,
13.0618684617384));
#241171=CARTESIAN_POINT('Ctrl Pts',(-2.16013496408955,-7.61277926634147,
13.0541076623741));
#241172=CARTESIAN_POINT('Ctrl Pts',(-2.34416056971887,-7.55815743266138,
13.0463468630099));
#241173=CARTESIAN_POINT('Ctrl Pts',(-2.52622540524093,-7.49680640018904,
13.0385860636456));
#241174=CARTESIAN_POINT('Ctrl Pts',(-2.70806921584986,-7.43552984726451,
13.0308346858152));
#241175=CARTESIAN_POINT('Ctrl Pts',(-2.8879566586254,-7.36754046866688,
13.0230833079847));
#241176=CARTESIAN_POINT('Ctrl Pts',(-3.06534398242874,-7.29298205601714,
13.0153319301543));
#241177=CARTESIAN_POINT('Ctrl Pts',(-3.24255196739692,-7.21849902202799,
13.0075883889778));
#241178=CARTESIAN_POINT('Ctrl Pts',(-3.4172645371924,-7.13746031240183,
12.9998448478013));
#241179=CARTESIAN_POINT('Ctrl Pts',(-3.58895248720248,-7.05005964830108,
12.9921013066248));
#241180=CARTESIAN_POINT('Ctrl Pts',(-3.76050165929437,-6.96272963145433,
12.9843640246675));
#241181=CARTESIAN_POINT('Ctrl Pts',(-3.92903076112556,-6.869048060348,12.9766267427103));
#241182=CARTESIAN_POINT('Ctrl Pts',(-4.09402990757578,-6.76925698403267,
12.9688894607531));
#241183=CARTESIAN_POINT('Ctrl Pts',(-4.2589290905073,-6.66952636540659,
12.9611568663712));
#241184=CARTESIAN_POINT('Ctrl Pts',(-4.4203022703938,-6.56369379713786,
12.9534242719893));
#241185=CARTESIAN_POINT('Ctrl Pts',(-4.57766347511734,-6.45204759038374,
12.9456916776074));
#241186=CARTESIAN_POINT('Ctrl Pts',(-4.73496118197615,-6.34044643473193,
12.937962203456));
#241187=CARTESIAN_POINT('Ctrl Pts',(-4.88824984562933,-6.22303652024753,
12.9302327293046));
#241188=CARTESIAN_POINT('Ctrl Pts',(-5.03707177534301,-6.10014991045653,
12.9225032551532));
#241189=CARTESIAN_POINT('Ctrl Pts',(-5.1858913050233,-5.97726528244313,
12.9147739056541));
#241190=CARTESIAN_POINT('Ctrl Pts',(-5.33024396038324,-5.84890435506099,
12.907044556155));
#241191=CARTESIAN_POINT('Ctrl Pts',(-5.46970419884377,-5.71544022601504,
12.8993152066559));
#241192=CARTESIAN_POINT('Ctrl Pts',(-5.60917007550081,-5.58197070118749,
12.8915855446693));
#241193=CARTESIAN_POINT('Ctrl Pts',(-5.74374288107121,-5.44339781157549,
12.8838558826826));
#241194=CARTESIAN_POINT('Ctrl Pts',(-5.87303322717905,-5.30013223537403,
12.876126220696));
#241195=CARTESIAN_POINT('Ctrl Pts',(-6.00235249070338,-5.15683461601961,
12.8683948298729));
#241196=CARTESIAN_POINT('Ctrl Pts',(-6.12638670121882,-5.00884248660251,
12.8606634390499));
#241197=CARTESIAN_POINT('Ctrl Pts',(-6.24478610264365,-4.85660040895159,
12.8529320482268));
#241198=CARTESIAN_POINT('Ctrl Pts',(-6.36323368715811,-4.7042963758044,
12.8451975110847));
#241199=CARTESIAN_POINT('Ctrl Pts',(-6.47604167612806,-4.54773923373394,
12.8374629739425));
#241200=CARTESIAN_POINT('Ctrl Pts',(-6.582903036094,-4.38740340262716,12.8297284368004));
#241201=CARTESIAN_POINT('Ctrl Pts',(-6.68989024165548,-4.22687875155628,
12.8219847910578));
#241202=CARTESIAN_POINT('Ctrl Pts',(-6.79091663303328,-4.06256682320184,
12.8142411453152));
#241203=CARTESIAN_POINT('Ctrl Pts',(-6.88572012340353,-3.89496846998222,
12.8064974995726));
#241204=CARTESIAN_POINT('Ctrl Pts',(-6.98058435577491,-3.72726273401415,
12.7987488923614));
#241205=CARTESIAN_POINT('Ctrl Pts',(-7.06921758044806,-3.55626669639221,
12.7910002851502));
#241206=CARTESIAN_POINT('Ctrl Pts',(-7.15140552479671,-3.38250203546237,
12.783251677939));
#241207=CARTESIAN_POINT('Ctrl Pts',(-7.23371799966124,-3.20847408770819,
12.7754913301002));
#241208=CARTESIAN_POINT('Ctrl Pts',(-7.30956554881387,-3.03166946694644,
12.7677309822614));
#241209=CARTESIAN_POINT('Ctrl Pts',(-7.37878310472328,-2.8526270161818,
12.7599706344225));
#241210=CARTESIAN_POINT('Ctrl Pts',(-7.42638559578358,-2.72949544139617,
12.7546336663113));
#241211=CARTESIAN_POINT('Ctrl Pts',(-7.47085339602555,-2.60530576544274,
12.7492966982001));
#241212=CARTESIAN_POINT('Ctrl Pts',(-7.51214685623806,-2.48023599891473,
12.7439597300889));
#241213=CARTESIAN_POINT('Ctrl Pts',(-7.58953553677097,-2.24584091174236,
12.7339576397326));
#241214=CARTESIAN_POINT('Ctrl Pts',(-7.65597446903994,-2.00774751142973,
12.7239555493762));
#241215=CARTESIAN_POINT('Ctrl Pts',(-7.71116937423448,-1.76685819517815,
12.7139534590199));
#241216=CARTESIAN_POINT('Ctrl Pts',(-7.76593347273457,-1.52784906568836,
12.7040294368742));
#241217=CARTESIAN_POINT('Ctrl Pts',(-7.80962837999544,-1.28608735383261,
12.6941054147285));
#241218=CARTESIAN_POINT('Ctrl Pts',(-7.84201276806946,-1.04247625653326,
12.6841813925827));
#241219=CARTESIAN_POINT('Ctrl Pts',(-7.87386998810044,-0.802830773317237,
12.6744189182582));
#241220=CARTESIAN_POINT('Ctrl Pts',(-7.89478191907505,-0.561395526168362,
12.6646564439336));
#241221=CARTESIAN_POINT('Ctrl Pts',(-7.90456362223255,-0.319053196313435,
12.6548939696091));
#241222=CARTESIAN_POINT('Ctrl Pts',(-7.90875934364808,-0.215103926243778,
12.6507064961259));
#241223=CARTESIAN_POINT('Ctrl Pts',(-7.91090782873707,-0.110988063861366,
12.6465190226428));
#241224=CARTESIAN_POINT('Ctrl Pts',(-7.91099709751604,-0.00677665793934715,
12.6423315491596));
#241225=CARTESIAN_POINT('',(-7.90222559779306,0.00578867911134829,10.6423315007885));
#241226=CARTESIAN_POINT('Ctrl Pts',(-7.90467196448321,-0.00677022214583101,
12.642331508237));
#241227=CARTESIAN_POINT('Ctrl Pts',(-7.88763856955293,1.78596353784846,
12.5702380049711));
#241228=CARTESIAN_POINT('Ctrl Pts',(-6.82905835000328,4.91048047638214,
12.4451597130971));
#241229=CARTESIAN_POINT('Ctrl Pts',(-3.14753813267382,7.60142069635078,
12.2670966326146));
#241230=CARTESIAN_POINT('Ctrl Pts',(2.24296169861674,8.43405333923742,12.0551574781816));
#241231=CARTESIAN_POINT('Ctrl Pts',(7.112990747597,5.05288013614879,11.8432183237487));
#241232=CARTESIAN_POINT('Ctrl Pts',(8.23030514357243,-0.295633148393404,
11.6312791693155));
#241233=CARTESIAN_POINT('Ctrl Pts',(7.10478066087843,-4.19983146691073,
11.4723248034909));
#241234=CARTESIAN_POINT('Ctrl Pts',(4.21961160578687,-7.07249030027441,
11.313370437666));
#241235=CARTESIAN_POINT('Ctrl Pts',(-0.992041909284247,-8.66363251511341,
11.1014312832332));
#241236=CARTESIAN_POINT('Ctrl Pts',(-6.62199532390963,-5.88691039012652,
10.87775164009));
#241237=CARTESIAN_POINT('Ctrl Pts',(-7.89102930427202,-1.61035822570545,
10.7070567855553));
#241238=CARTESIAN_POINT('Ctrl Pts',(-7.90039148196552,0.00578714936241065,
10.642331508237));
#241239=CARTESIAN_POINT('Ctrl Pts',(-7.91099787678106,0.00579599565279081,
10.6423314651635));
#241240=CARTESIAN_POINT('Ctrl Pts',(-7.91084011201517,0.22113030623056,
10.6337190262862));
#241241=CARTESIAN_POINT('Ctrl Pts',(-7.90188645289187,0.436110537192641,
10.625106587409));
#241242=CARTESIAN_POINT('Ctrl Pts',(-7.88424739306299,0.650049263501995,
10.6164941485317));
#241243=CARTESIAN_POINT('Ctrl Pts',(-7.86650936761889,0.865188313290822,
10.6078333887507));
#241244=CARTESIAN_POINT('Ctrl Pts',(-7.83998829271854,1.07927392276559,
10.5991726289697));
#241245=CARTESIAN_POINT('Ctrl Pts',(-7.80484642310435,1.29162429202741,
10.5905118691887));
#241246=CARTESIAN_POINT('Ctrl Pts',(-7.76960354634283,1.50458501313636,
10.581826216064));
#241247=CARTESIAN_POINT('Ctrl Pts',(-7.72569036399297,1.71580030444112,
10.5731405629392));
#241248=CARTESIAN_POINT('Ctrl Pts',(-7.67331901160124,1.92460290610788,
10.5644549098145));
#241249=CARTESIAN_POINT('Ctrl Pts',(-7.62072078907441,2.13431003042467,
10.5557316308656));
#241250=CARTESIAN_POINT('Ctrl Pts',(-7.55959107197527,2.34158331837183,
10.5470083519167));
#241251=CARTESIAN_POINT('Ctrl Pts',(-7.49019186016789,2.54577039378547,
10.5382850729678));
#241252=CARTESIAN_POINT('Ctrl Pts',(-7.43798576035897,2.69937171808185,
10.5317229181592));
#241253=CARTESIAN_POINT('Ctrl Pts',(-7.38110100282061,2.8512270490789,10.5251607633507));
#241254=CARTESIAN_POINT('Ctrl Pts',(-7.31966593697622,3.00106840493015,
10.5185986085422));
#241255=CARTESIAN_POINT('Ctrl Pts',(-7.24557212977723,3.1817846844406,10.510684316818));
#241256=CARTESIAN_POINT('Ctrl Pts',(-7.16467709171961,3.3600106342992,10.5027700250937));
#241257=CARTESIAN_POINT('Ctrl Pts',(-7.0771675753867,3.53519732262503,10.4948557333695));
#241258=CARTESIAN_POINT('Ctrl Pts',(-6.98975853982763,3.71018285689646,
10.4869505290472));
#241259=CARTESIAN_POINT('Ctrl Pts',(-6.89575030608029,3.88213577507176,
10.479045324725));
#241260=CARTESIAN_POINT('Ctrl Pts',(-6.79537842180121,4.05052504059888,
10.4711401204028));
#241261=CARTESIAN_POINT('Ctrl Pts',(-6.69510314731133,4.21875222835326,
10.4632425249855));
#241262=CARTESIAN_POINT('Ctrl Pts',(-6.58847659906755,4.38342230214607,
10.4553449295682));
#241263=CARTESIAN_POINT('Ctrl Pts',(-6.47578128375428,4.54402660258254,
10.4474473341509));
#241264=CARTESIAN_POINT('Ctrl Pts',(-6.3631735186266,4.70450613353527,10.4395558741789));
#241265=CARTESIAN_POINT('Ctrl Pts',(-6.24450657656139,4.86092590298295,
10.4316644142069));
#241266=CARTESIAN_POINT('Ctrl Pts',(-6.12010767000815,5.0128039167224,10.4237729542349));
#241267=CARTESIAN_POINT('Ctrl Pts',(-5.99578231786302,5.16459212824641,
10.4158861603141));
#241268=CARTESIAN_POINT('Ctrl Pts',(-5.86573197233401,5.31184366896547,
10.4079993663934));
#241269=CARTESIAN_POINT('Ctrl Pts',(-5.73032590167918,5.45410726522175,
10.4001125724726));
#241270=CARTESIAN_POINT('Ctrl Pts',(-5.59497476743434,5.59631314286015,
10.3922289783503));
#241271=CARTESIAN_POINT('Ctrl Pts',(-5.45427247593998,5.73353485970938,
10.384345384228));
#241272=CARTESIAN_POINT('Ctrl Pts',(-5.30862732871614,5.86535564862082,
10.3764617901058));
#241273=CARTESIAN_POINT('Ctrl Pts',(-5.16299386279386,5.99716586499746,
10.3685788282781));
#241274=CARTESIAN_POINT('Ctrl Pts',(-5.01241858207212,6.12357578017002,
10.3606958664505));
#241275=CARTESIAN_POINT('Ctrl Pts',(-4.85734564250934,6.24420645952674,
10.3528129046228));
#241276=CARTESIAN_POINT('Ctrl Pts',(-4.70227232770731,6.36483743078073,
10.3449299237203));
#241277=CARTESIAN_POINT('Ctrl Pts',(-4.54270160435299,6.47968892606496,
10.3370469428177));
#241278=CARTESIAN_POINT('Ctrl Pts',(-4.37910968259495,6.58842313363396,
10.3291639619152));
#241279=CARTESIAN_POINT('Ctrl Pts',(-4.21548985849375,6.69717588697919,
10.3212796364864));
#241280=CARTESIAN_POINT('Ctrl Pts',(-4.0478477567119,6.79980908269741,10.3133953110575));
#241281=CARTESIAN_POINT('Ctrl Pts',(-3.87668765577041,6.89602884416802,
10.3055109856287));
#241282=CARTESIAN_POINT('Ctrl Pts',(-3.70546958249056,6.99228119550355,
10.2976239897599));
#241283=CARTESIAN_POINT('Ctrl Pts',(-3.53073143644949,7.08211561553676,
10.2897369938911));
#241284=CARTESIAN_POINT('Ctrl Pts',(-3.35300132737368,7.16528457904013,
10.2818499980222));
#241285=CARTESIAN_POINT('Ctrl Pts',(-3.17509761438337,7.24853478065056,
10.2739552982626));
#241286=CARTESIAN_POINT('Ctrl Pts',(-2.99419641350989,7.32510637492556,
10.2660605985029));
#241287=CARTESIAN_POINT('Ctrl Pts',(-2.81084599246224,7.39479991660755,
10.2581658987433));
#241288=CARTESIAN_POINT('Ctrl Pts',(-2.62739306749653,7.46453242117299,
10.2502667853714));
#241289=CARTESIAN_POINT('Ctrl Pts',(-2.44148851844214,7.52737909640816,
10.2423676719995));
#241290=CARTESIAN_POINT('Ctrl Pts',(-2.25369520558157,7.58319055017996,
10.2344685586277));
#241291=CARTESIAN_POINT('Ctrl Pts',(-2.06567266421524,7.63907012978627,
10.226559803262));
#241292=CARTESIAN_POINT('Ctrl Pts',(-1.87575708710941,7.68789724919696,
10.2186510478964));
#241293=CARTESIAN_POINT('Ctrl Pts',(-1.68452201279013,7.72957350624376,
10.2107422925307));
#241294=CARTESIAN_POINT('Ctrl Pts',(-1.60349896248135,7.74723102792698,
10.2073914873181));
#241295=CARTESIAN_POINT('Ctrl Pts',(-1.52223912846249,7.7636055542267,10.2040406821054));
#241296=CARTESIAN_POINT('Ctrl Pts',(-1.44078636577397,7.77869241249452,
10.2006898768928));
#241297=CARTESIAN_POINT('Ctrl Pts',(-1.23193470200725,7.8173763729428,10.1920981334022));
#241298=CARTESIAN_POINT('Ctrl Pts',(-1.02139613098446,7.84766857101163,
10.1835063899116));
#241299=CARTESIAN_POINT('Ctrl Pts',(-0.809837471830828,7.86943989552107,
10.174914646421));
#241300=CARTESIAN_POINT('Ctrl Pts',(-0.59858373311001,7.89117984092403,
10.1663352862483));
#241301=CARTESIAN_POINT('Ctrl Pts',(-0.386313087132472,7.90442339618755,
10.1577559260757));
#241302=CARTESIAN_POINT('Ctrl Pts',(-0.173700237161343,7.90909281950908,
10.149176565903));
#241303=CARTESIAN_POINT('Ctrl Pts',(0.0481825568613072,7.91396583020996,
10.1402231446668));
#241304=CARTESIAN_POINT('Ctrl Pts',(0.270437816712338,7.90950025771785,
10.1312697234305));
#241305=CARTESIAN_POINT('Ctrl Pts',(0.492290480755137,7.89566786805004,
10.1223163021943));
#241306=CARTESIAN_POINT('Ctrl Pts',(0.704039497636602,7.88246543513847,
10.1137706390052));
#241307=CARTESIAN_POINT('Ctrl Pts',(0.915421462210409,7.86073030452146,
10.1052249758162));
#241308=CARTESIAN_POINT('Ctrl Pts',(1.12575916832216,7.83049087190188,10.0966793126271));
#241309=CARTESIAN_POINT('Ctrl Pts',(1.33577481171214,7.80029774098518,10.0881467342986));
#241310=CARTESIAN_POINT('Ctrl Pts',(1.54474914109195,7.76162631997591,10.07961415597));
#241311=CARTESIAN_POINT('Ctrl Pts',(1.75200864203953,7.71455680633818,10.0710815776415));
#241312=CARTESIAN_POINT('Ctrl Pts',(1.95881897803677,7.66758929996989,10.062567490794));
#241313=CARTESIAN_POINT('Ctrl Pts',(2.16392165896475,7.61226007246776,10.0540534039464));
#241314=CARTESIAN_POINT('Ctrl Pts',(2.36665188143885,7.54870054195303,10.0455393170989));
#241315=CARTESIAN_POINT('Ctrl Pts',(2.39684288358654,7.53923512580117,10.0442713817552));
#241316=CARTESIAN_POINT('Ctrl Pts',(2.42698128175428,7.52958727327394,10.0430034464116));
#241317=CARTESIAN_POINT('Ctrl Pts',(2.45706489385209,7.51975751652935,10.0417355110679));
#241318=CARTESIAN_POINT('Ctrl Pts',(2.64442867903153,7.45853679525852,10.0338386812399));
#241319=CARTESIAN_POINT('Ctrl Pts',(2.82949288590725,7.39031267098654,10.0259418514119));
#241320=CARTESIAN_POINT('Ctrl Pts',(3.0117087418066,7.31529435187168,10.0180450215839));
#241321=CARTESIAN_POINT('Ctrl Pts',(3.1939660984105,7.24025894690509,10.0101463932077));
#241322=CARTESIAN_POINT('Ctrl Pts',(3.37337349464752,7.15842639333845,10.0022477648315));
#241323=CARTESIAN_POINT('Ctrl Pts',(3.54940309944911,7.07005365167911,9.99434913645532));
#241324=CARTESIAN_POINT('Ctrl Pts',(3.72550175846788,6.98164624249607,9.98644740954578));
#241325=CARTESIAN_POINT('Ctrl Pts',(3.89821967970184,6.8866936855725,9.97854568263623));
#241326=CARTESIAN_POINT('Ctrl Pts',(4.06705430413475,6.78549852901163,9.97064395572668));
#241327=CARTESIAN_POINT('Ctrl Pts',(4.23607502340706,6.68419183196272,9.96273351928492));
#241328=CARTESIAN_POINT('Ctrl Pts',(4.40120360083051,6.57662896464247,9.95482308284316));
#241329=CARTESIAN_POINT('Ctrl Pts',(4.56196608780908,6.46315607220497,9.9469126464014));
#241330=CARTESIAN_POINT('Ctrl Pts',(4.72282455024674,6.34961543627114,9.93899748741657));
#241331=CARTESIAN_POINT('Ctrl Pts',(4.87931145338171,6.23015794712718,9.93108232843174));
#241332=CARTESIAN_POINT('Ctrl Pts',(5.03098630054118,6.10516976371394,9.92316716944691));
#241333=CARTESIAN_POINT('Ctrl Pts',(5.18287371041121,5.98000641726247,9.9152409178671));
#241334=CARTESIAN_POINT('Ctrl Pts',(5.32993533367976,5.84929711584608,9.90731466628729));
#241335=CARTESIAN_POINT('Ctrl Pts',(5.47176687964138,5.71346551707978,9.89938841470748));
#241336=CARTESIAN_POINT('Ctrl Pts',(5.57082314764714,5.61859965941869,9.8938526582194));
#241337=CARTESIAN_POINT('Ctrl Pts',(5.66732911631661,5.52123603491172,9.88831690173133));
#241338=CARTESIAN_POINT('Ctrl Pts',(5.76115891386824,5.42152828722275,9.88278114524325));
#241339=CARTESIAN_POINT('Ctrl Pts',(5.89885173923236,5.27520972053894,9.87465756434186));
#241340=CARTESIAN_POINT('Ctrl Pts',(6.03108242737734,5.12352022575209,9.86653398344048));
#241341=CARTESIAN_POINT('Ctrl Pts',(6.15742438184121,4.96689500411549,9.8584104025391));
#241342=CARTESIAN_POINT('Ctrl Pts',(6.28365463989171,4.81040825172748,9.85029400353429));
#241343=CARTESIAN_POINT('Ctrl Pts',(6.40400634340106,4.64899472080601,9.84217760452949));
#241344=CARTESIAN_POINT('Ctrl Pts',(6.51809117228047,4.48312485548187,9.83406120552468));
#241345=CARTESIAN_POINT('Ctrl Pts',(6.63209141237905,4.31737797521915,9.82595082446549));
#241346=CARTESIAN_POINT('Ctrl Pts',(6.73983386163787,4.14718161220173,9.81784044340631));
#241347=CARTESIAN_POINT('Ctrl Pts',(6.84097142903509,3.9730379946743,9.80973006234712));
#241348=CARTESIAN_POINT('Ctrl Pts',(6.94204841315618,3.79899869239925,9.80162453955641));
#241349=CARTESIAN_POINT('Ctrl Pts',(7.03652824432652,3.62101712740149,9.79351901676571));
#241350=CARTESIAN_POINT('Ctrl Pts',(7.12410769532924,3.4396236051857,9.78541349397499));
#241351=CARTESIAN_POINT('Ctrl Pts',(7.21164714563034,3.25831293194962,9.77731167326959));
#241352=CARTESIAN_POINT('Ctrl Pts',(7.29229236202178,3.07359369784467,9.76920985256418));
#241353=CARTESIAN_POINT('Ctrl Pts',(7.36578627721016,2.88602036002218,9.76110803185878));
#241354=CARTESIAN_POINT('Ctrl Pts',(7.43995748519188,2.69671841555783,9.7529315477644));
#241355=CARTESIAN_POINT('Ctrl Pts',(7.50684476678568,2.50450979065043,9.74475506367002));
#241356=CARTESIAN_POINT('Ctrl Pts',(7.5662333607541,2.30998565593202,9.73657857957565));
#241357=CARTESIAN_POINT('Ctrl Pts',(7.6250573061041,2.11731099729274,9.72847983499552));
#241358=CARTESIAN_POINT('Ctrl Pts',(7.67652445379345,1.92236498446628,9.7203810904154));
#241359=CARTESIAN_POINT('Ctrl Pts',(7.72047593411518,1.72573820458037,9.71228234583528));
#241360=CARTESIAN_POINT('Ctrl Pts',(7.76442715590926,1.52911258127578,9.7041836488929));
#241361=CARTESIAN_POINT('Ctrl Pts',(7.80086272862794,1.33080652374314,9.69608495195053));
#241362=CARTESIAN_POINT('Ctrl Pts',(7.82967465811501,1.13142200264603,9.68798625500815));
#241363=CARTESIAN_POINT('Ctrl Pts',(7.8584901442091,0.932012869091566,9.67988655834507));
#241364=CARTESIAN_POINT('Ctrl Pts',(7.87968006490698,0.73152532405803,9.671786861682));
#241365=CARTESIAN_POINT('Ctrl Pts',(7.8931880989192,0.530568219063547,9.66368716501892));
#241366=CARTESIAN_POINT('Ctrl Pts',(7.90692105171448,0.326265029253143,
9.65545260240015));
#241367=CARTESIAN_POINT('Ctrl Pts',(7.91271401193322,0.121476846567367,
9.64721803978139));
#241368=CARTESIAN_POINT('Ctrl Pts',(7.91056295792561,-0.0831546071802162,
9.63898347716262));
#241369=CARTESIAN_POINT('Ctrl Pts',(7.90844510494008,-0.284627621674178,
9.63087601311709));
#241370=CARTESIAN_POINT('Ctrl Pts',(7.89862673624289,-0.485948387733569,
9.62276854907157));
#241371=CARTESIAN_POINT('Ctrl Pts',(7.88115654522144,-0.686507472438068,
9.61466108502604));
#241372=CARTESIAN_POINT('Ctrl Pts',(7.86327554084196,-0.891782724868992,
9.60636297312065));
#241373=CARTESIAN_POINT('Ctrl Pts',(7.83737846417857,-1.09625967758778,
9.59806486121527));
#241374=CARTESIAN_POINT('Ctrl Pts',(7.80357339207048,-1.29929339048948,
9.58976674930988));
#241375=CARTESIAN_POINT('Ctrl Pts',(7.76976831996239,-1.50232710339118,
9.58146863740449));
#241376=CARTESIAN_POINT('Ctrl Pts',(7.72805535156513,-1.70391723110227,
9.5731705254991));
#241377=CARTESIAN_POINT('Ctrl Pts',(7.67859786229843,-1.90343265420819,
9.56487241359372));
#241378=CARTESIAN_POINT('Ctrl Pts',(7.63195627071978,-2.09158852334186,
9.5570467606521));
#241379=CARTESIAN_POINT('Ctrl Pts',(7.57833708343701,-2.27826124570093,
9.54922110771048));
#241380=CARTESIAN_POINT('Ctrl Pts',(7.51785168359855,-2.46288998199562,
9.54139545476887));
#241381=CARTESIAN_POINT('Ctrl Pts',(7.45741739758756,-2.64736269582211,
9.53357641497812));
#241382=CARTESIAN_POINT('Ctrl Pts',(7.39012856107222,-2.82979453024159,
9.52575737518737));
#241383=CARTESIAN_POINT('Ctrl Pts',(7.31614729843773,-3.00963614205476,
9.51793833539662));
#241384=CARTESIAN_POINT('Ctrl Pts',(7.24221547118042,-3.18935758103504,
9.51012452040425));
#241385=CARTESIAN_POINT('Ctrl Pts',(7.16160025724386,-3.36649191982711,
9.50231070541188));
#241386=CARTESIAN_POINT('Ctrl Pts',(7.07451323002585,-3.54050611610674,
9.49449689041951));
#241387=CARTESIAN_POINT('Ctrl Pts',(6.98746798788579,-3.71443681893174,
9.48668682456038));
#241388=CARTESIAN_POINT('Ctrl Pts',(6.89395727496761,-3.88525004675205,
9.47887675870126));
#241389=CARTESIAN_POINT('Ctrl Pts',(6.7942403649099,-4.05243369641367,9.47106669284213));
#241390=CARTESIAN_POINT('Ctrl Pts',(6.69455257874541,-4.21956851745878,
9.46325890803567));
#241391=CARTESIAN_POINT('Ctrl Pts',(6.58866238726719,-4.38307557008177,
9.45545112322922));
#241392=CARTESIAN_POINT('Ctrl Pts',(6.47687457155242,-4.54246813795954,
9.44764333842276));
#241393=CARTESIAN_POINT('Ctrl Pts',(6.36508021315268,-4.70187003471947,
9.43983509664453));
#241394=CARTESIAN_POINT('Ctrl Pts',(6.2473877379407,-4.8571566733063,9.4320268548663));
#241395=CARTESIAN_POINT('Ctrl Pts',(6.12414499222924,-5.00787071659738,
9.42421861308807));
#241396=CARTESIAN_POINT('Ctrl Pts',(6.0278616042375,-5.12561605424163,9.41811842464837));
#241397=CARTESIAN_POINT('Ctrl Pts',(5.92819149177514,-5.24057104731698,
9.41201823620866));
#241398=CARTESIAN_POINT('Ctrl Pts',(5.82531752358805,-5.35253180741395,
9.40591804776896));
#241399=CARTESIAN_POINT('Ctrl Pts',(5.67928539102838,-5.51146286497972,
9.39725867997588));
#241400=CARTESIAN_POINT('Ctrl Pts',(5.52686841486363,-5.66428149419263,
9.38859931218279));
#241401=CARTESIAN_POINT('Ctrl Pts',(5.36858988646197,-5.81052180367463,
9.37993994438971));
#241402=CARTESIAN_POINT('Ctrl Pts',(5.21003743637605,-5.95701520112935,
9.37126559042867));
#241403=CARTESIAN_POINT('Ctrl Pts',(5.04560332164886,-6.09690736730511,
9.36259123646763));
#241404=CARTESIAN_POINT('Ctrl Pts',(4.87584411823539,-6.22977247856367,
9.35391688250659));
#241405=CARTESIAN_POINT('Ctrl Pts',(4.70141911963666,-6.3662893588217,9.34500411579305));
#241406=CARTESIAN_POINT('Ctrl Pts',(4.52137238261631,-6.49538727664552,
9.33609134907952));
#241407=CARTESIAN_POINT('Ctrl Pts',(4.33633789484381,-6.61665282916835,
9.32717858236599));
#241408=CARTESIAN_POINT('Ctrl Pts',(4.15563539520363,-6.73507933832845,
9.31847447945397));
#241409=CARTESIAN_POINT('Ctrl Pts',(3.97017627356648,-6.8460360228435,9.30977037654195));
#241410=CARTESIAN_POINT('Ctrl Pts',(3.7805760327062,-6.94918454647216,9.30106627362992));
#241411=CARTESIAN_POINT('Ctrl Pts',(3.584157850797,-7.05604224552271,9.29204917501564));
#241412=CARTESIAN_POINT('Ctrl Pts',(3.38329546915963,-7.15451973244231,
9.28303207640135));
#241413=CARTESIAN_POINT('Ctrl Pts',(3.17869751905459,-7.24429451929974,
9.27401497778706));
#241414=CARTESIAN_POINT('Ctrl Pts',(2.97409956894955,-7.33406930615716,
9.26499787917277));
#241415=CARTESIAN_POINT('Ctrl Pts',(2.76576630604029,-7.41514131334428,
9.25598078055848));
#241416=CARTESIAN_POINT('Ctrl Pts',(2.55442732361032,-7.48724395544803,
9.2469636819442));
#241417=CARTESIAN_POINT('Ctrl Pts',(2.36035336384111,-7.55345627984745,
9.23868322173954));
#241418=CARTESIAN_POINT('Ctrl Pts',(2.16357684847049,-7.61216197823561,
9.23040276153488));
#241419=CARTESIAN_POINT('Ctrl Pts',(1.96469543193453,-7.66315162708762,
9.22212230133022));
#241420=CARTESIAN_POINT('Ctrl Pts',(1.76598859761605,-7.71409651617212,
9.21384910988465));
#241421=CARTESIAN_POINT('Ctrl Pts',(1.56518083565212,-7.75733879224521,
9.20557591843909));
#241422=CARTESIAN_POINT('Ctrl Pts',(1.36288538465213,-7.792718680172,9.19730272699352));
#241423=CARTESIAN_POINT('Ctrl Pts',(1.16075177834765,-7.82807026273077,
9.18903615444197));
#241424=CARTESIAN_POINT('Ctrl Pts',(0.957133150287012,-7.85557195343149,
9.18076958189042));
#241425=CARTESIAN_POINT('Ctrl Pts',(0.752654151315554,-7.87511477557676,
9.17250300933887));
#241426=CARTESIAN_POINT('Ctrl Pts',(0.548365589235476,-7.8946393969566,
9.16424413567271));
#241427=CARTESIAN_POINT('Ctrl Pts',(0.343218551836084,-7.90621991579081,
9.15598526200656));
#241428=CARTESIAN_POINT('Ctrl Pts',(0.137844450573246,-7.90979898021727,
9.14772638834041));
#241429=CARTESIAN_POINT('Ctrl Pts',(-0.0674099135277758,-7.9133759579784,
9.1394723297609));
#241430=CARTESIAN_POINT('Ctrl Pts',(-0.272890779820393,-7.90896078059047,
9.13121827118139));
#241431=CARTESIAN_POINT('Ctrl Pts',(-0.477963770675786,-7.89654808342996,
9.12296421260188));
#241432=CARTESIAN_POINT('Ctrl Pts',(-0.682906975524917,-7.88414324198163,
9.1147153778273));
#241433=CARTESIAN_POINT('Ctrl Pts',(-0.887442522784967,-7.86375099972519,
9.10646654305271));
#241434=CARTESIAN_POINT('Ctrl Pts',(-1.09093763596683,-7.83541805358406,
9.09821770827812));
#241435=CARTESIAN_POINT('Ctrl Pts',(-1.17488314562582,-7.82373018763599,
9.09481491089189));
#241436=CARTESIAN_POINT('Ctrl Pts',(-1.25865163316916,-7.8106916524491,
9.09141211350566));
#241437=CARTESIAN_POINT('Ctrl Pts',(-1.34219888083408,-7.79630830356828,
9.08800931611943));
#241438=CARTESIAN_POINT('Ctrl Pts',(-1.54246652179313,-7.76183057473867,
9.07985261168873));
#241439=CARTESIAN_POINT('Ctrl Pts',(-1.74137495677086,-7.71963717112491,
9.07169590725802));
#241440=CARTESIAN_POINT('Ctrl Pts',(-1.9383181463002,-7.66986595474285,
9.06353920282732));
#241441=CARTESIAN_POINT('Ctrl Pts',(-2.1353203067587,-7.62007983530735,
9.05538005602508));
#241442=CARTESIAN_POINT('Ctrl Pts',(-2.33035574563551,-7.56271145302439,
9.04722090922285));
#241443=CARTESIAN_POINT('Ctrl Pts',(-2.52283233455093,-7.4979489203211,
9.03906176242061));
#241444=CARTESIAN_POINT('Ctrl Pts',(-2.71538770680269,-7.4331598794153,
9.03089927596647));
#241445=CARTESIAN_POINT('Ctrl Pts',(-2.9053818443482,-7.36097074974645,
9.02273678951233));
#241446=CARTESIAN_POINT('Ctrl Pts',(-3.0922407765744,-7.28161850001018,
9.01457430305819));
#241447=CARTESIAN_POINT('Ctrl Pts',(-3.27927779040433,-7.20219062543906,
9.00640403753424));
#241448=CARTESIAN_POINT('Ctrl Pts',(-3.46317334050545,-7.11558611008798,
8.99823377201029));
#241449=CARTESIAN_POINT('Ctrl Pts',(-3.64337500980557,-7.02208939973882,
8.99006350648634));
#241450=CARTESIAN_POINT('Ctrl Pts',(-3.82366938334809,-6.92854459026975,
8.98188903779225));
#241451=CARTESIAN_POINT('Ctrl Pts',(-4.00026581133523,-6.82810066111308,
8.97371456909816));
#241452=CARTESIAN_POINT('Ctrl Pts',(-4.17263830753271,-6.72108700691417,
8.96554010040408));
#241453=CARTESIAN_POINT('Ctrl Pts',(-4.34519482194472,-6.61395910907426,
8.95735690496316));
#241454=CARTESIAN_POINT('Ctrl Pts',(-4.51351813219441,-6.50024764074212,
8.94917370952225));
#241455=CARTESIAN_POINT('Ctrl Pts',(-4.67711175205704,-6.3803249649818,
8.94099051408134));
#241456=CARTESIAN_POINT('Ctrl Pts',(-4.75664800408561,-6.32202073422253,
8.93701199281911));
#241457=CARTESIAN_POINT('Ctrl Pts',(-4.83506677825874,-6.26224895531807,
8.93303347155689));
#241458=CARTESIAN_POINT('Ctrl Pts',(-4.91231393835858,-6.20105577873704,
8.92905495029467));
#241459=CARTESIAN_POINT('Ctrl Pts',(-5.06467539118251,-6.08035902723515,
8.92120775851674));
#241460=CARTESIAN_POINT('Ctrl Pts',(-5.21276933187155,-5.95389820078589,
8.91336056673882));
#241461=CARTESIAN_POINT('Ctrl Pts',(-5.35612987218644,-5.82200942907791,
8.9055133749609));
#241462=CARTESIAN_POINT('Ctrl Pts',(-5.49936350951701,-5.69023740552595,
8.89767312952995));
#241463=CARTESIAN_POINT('Ctrl Pts',(-5.63787183538287,-5.55304724188308,
8.889832884099));
#241464=CARTESIAN_POINT('Ctrl Pts',(-5.77122058026558,-5.41081639070474,
8.88199263866805));
#241465=CARTESIAN_POINT('Ctrl Pts',(-5.90447698927311,-5.26868402571862,
8.87415782212902));
#241466=CARTESIAN_POINT('Ctrl Pts',(-6.03258069520401,-5.12151818025878,
8.86632300558998));
#241467=CARTESIAN_POINT('Ctrl Pts',(-6.15513282804547,-4.96973448678267,
8.85848818905095));
#241468=CARTESIAN_POINT('Ctrl Pts',(-6.27762371764066,-4.81802664450478,
8.85065728782198));
#241469=CARTESIAN_POINT('Ctrl Pts',(-6.39456834165947,-4.66170582363914,
8.84282638659301));
#241470=CARTESIAN_POINT('Ctrl Pts',(-6.5056066906416,-4.50122234361725,
8.83499548536405));
#241471=CARTESIAN_POINT('Ctrl Pts',(-6.61943505737918,-4.33670645710859,
8.82696782010112));
#241472=CARTESIAN_POINT('Ctrl Pts',(-6.72705619161308,-4.16781625990227,
8.81894015483819));
#241473=CARTESIAN_POINT('Ctrl Pts',(-6.82812775317153,-3.99507101143006,
8.81091248957526));
#241474=CARTESIAN_POINT('Ctrl Pts',(-6.92669905157804,-3.82659905776764,
8.8030834091105));
#241475=CARTESIAN_POINT('Ctrl Pts',(-7.01904081241868,-3.65446084903053,
8.79525432864574));
#241476=CARTESIAN_POINT('Ctrl Pts',(-7.10488071172684,-3.47916528381909,
8.78742524818098));
#241477=CARTESIAN_POINT('Ctrl Pts',(-7.19073027564623,-3.30384998229036,
8.77959528624945));
#241478=CARTESIAN_POINT('Ctrl Pts',(-7.27007636510633,-3.12537693073728,
8.77176532431792));
#241479=CARTESIAN_POINT('Ctrl Pts',(-7.34269374456673,-2.94427742807987,
8.76393536238639));
#241480=CARTESIAN_POINT('Ctrl Pts',(-7.41533197604286,-2.76312592286182,
8.75610315208827));
#241481=CARTESIAN_POINT('Ctrl Pts',(-7.48123751801491,-2.57934678931001,
8.74827094179016));
#241482=CARTESIAN_POINT('Ctrl Pts',(-7.54023412577994,-2.39348915360477,
8.74043873149204));
#241483=CARTESIAN_POINT('Ctrl Pts',(-7.60181734548886,-2.19948288701055,
8.73226313045552));
#241484=CARTESIAN_POINT('Ctrl Pts',(-7.65587202929742,-2.00321216380559,
8.72408752941899));
#241485=CARTESIAN_POINT('Ctrl Pts',(-7.70225654814461,-1.80531578028985,
8.71591192838247));
#241486=CARTESIAN_POINT('Ctrl Pts',(-7.74676446764627,-1.61542577978758,
8.70806709131495));
#241487=CARTESIAN_POINT('Ctrl Pts',(-7.78421063099003,-1.42403942123451,
8.70022225424743));
#241488=CARTESIAN_POINT('Ctrl Pts',(-7.81452279807668,-1.23172823233851,
8.69237741717991));
#241489=CARTESIAN_POINT('Ctrl Pts',(-7.84485569390023,-1.03928553294957,
8.68452721548231));
#241490=CARTESIAN_POINT('Ctrl Pts',(-7.86804482960821,-0.845917089121394,
8.6766770137847));
#241491=CARTESIAN_POINT('Ctrl Pts',(-7.88406999468733,-0.652197300570159,
8.6688268120871));
#241492=CARTESIAN_POINT('Ctrl Pts',(-7.90011556588749,-0.458230833158753,
8.66096661410145));
#241493=CARTESIAN_POINT('Ctrl Pts',(-7.9089789397769,-0.263912475701678,
8.65310641611579));
#241494=CARTESIAN_POINT('Ctrl Pts',(-7.91069193117117,-0.0698152569529835,
8.64524621813014));
#241495=CARTESIAN_POINT('Ctrl Pts',(-7.91090366690793,-0.0458237075776071,
8.64427465177134));
#241496=CARTESIAN_POINT('Ctrl Pts',(-7.91100622103527,-0.0218355284886099,
8.64330308541254));
#241497=CARTESIAN_POINT('Ctrl Pts',(-7.91099970833086,0.00214820601359551,
8.64233151905374));
#241498=CARTESIAN_POINT('Origin',(0.,0.,4.30282021618968));
#241499=CARTESIAN_POINT('',(-6.76699855375495,-0.00289230543239241,137.30282021619));
#241500=CARTESIAN_POINT('Ctrl Pts',(3.09910619832119,6.01563211736948,136.651395695404));
#241501=CARTESIAN_POINT('Ctrl Pts',(2.93375330764808,6.10081787314662,136.660145143307));
#241502=CARTESIAN_POINT('Ctrl Pts',(2.76488627843049,6.17918207037049,136.668894591209));
#241503=CARTESIAN_POINT('Ctrl Pts',(2.59307866646677,6.25045854554007,136.677644039111));
#241504=CARTESIAN_POINT('Ctrl Pts',(2.42127244185344,6.3217344451505,136.686393416362));
#241505=CARTESIAN_POINT('Ctrl Pts',(2.24652594672423,6.38592262741853,136.695142793612));
#241506=CARTESIAN_POINT('Ctrl Pts',(2.06943269687071,6.44280508110578,136.703892170862));
#241507=CARTESIAN_POINT('Ctrl Pts',(1.89234081822012,6.49968709436186,136.712641480368));
#241508=CARTESIAN_POINT('Ctrl Pts',(1.71290249405508,6.54926340459566,136.721390789873));
#241509=CARTESIAN_POINT('Ctrl Pts',(1.53172716624962,6.59136563150406,136.730140099378));
#241510=CARTESIAN_POINT('Ctrl Pts',(1.35055318107239,6.63346754640729,136.738889344046));
#241511=CARTESIAN_POINT('Ctrl Pts',(1.16764249714326,6.66809542395792,136.747638588713));
#241512=CARTESIAN_POINT('Ctrl Pts',(0.983616340613428,6.69513165624682,
136.75638783338));
#241513=CARTESIAN_POINT('Ctrl Pts',(0.799591486713008,6.7221676971597,136.765137016116));
#241514=CARTESIAN_POINT('Ctrl Pts',(0.614451459525972,6.74161215869377,
136.773886198851));
#241515=CARTESIAN_POINT('Ctrl Pts',(0.428825047909639,6.75339900185716,
136.782635381587));
#241516=CARTESIAN_POINT('Ctrl Pts',(0.243199888596407,6.76518576550223,
136.791384505298));
#241517=CARTESIAN_POINT('Ctrl Pts',(0.0570886373912859,6.76931499599835,
136.800133629008));
#241518=CARTESIAN_POINT('Ctrl Pts',(-0.128876626811774,6.76577266947846,
136.808882752719));
#241519=CARTESIAN_POINT('Ctrl Pts',(-0.314840698188627,6.7622303656799,
136.81763182031));
#241520=CARTESIAN_POINT('Ctrl Pts',(-0.500658497951566,6.7510166087922,
136.826380887902));
#241521=CARTESIAN_POINT('Ctrl Pts',(-0.685698951926375,6.73216948296217,
136.835129955493));
#241522=CARTESIAN_POINT('Ctrl Pts',(-0.870738280460203,6.71332247176289,
136.843878969872));
#241523=CARTESIAN_POINT('Ctrl Pts',(-1.05499998761305,6.68684221356179,
136.85262798425));
#241524=CARTESIAN_POINT('Ctrl Pts',(-1.23785829161493,6.65281863948509,
136.861376998629));
#241525=CARTESIAN_POINT('Ctrl Pts',(-1.43007412917463,6.61705395368848,
136.870573732328));
#241526=CARTESIAN_POINT('Ctrl Pts',(-1.62073882535838,6.57295372727778,
136.879770466027));
#241527=CARTESIAN_POINT('Ctrl Pts',(-1.80913696091546,6.5206834347827,136.888967199726));
#241528=CARTESIAN_POINT('Ctrl Pts',(-1.98838356186147,6.47095219815188,
136.89771719744));
#241529=CARTESIAN_POINT('Ctrl Pts',(-2.16557827572571,6.41382586850878,
136.906467195154));
#241530=CARTESIAN_POINT('Ctrl Pts',(-2.3401191862174,6.34949849943263,136.915217192868));
#241531=CARTESIAN_POINT('Ctrl Pts',(-2.51465655691146,6.28517243495532,
136.923967013126));
#241532=CARTESIAN_POINT('Ctrl Pts',(-2.68653996295384,6.21364572242351,
136.932716833384));
#241533=CARTESIAN_POINT('Ctrl Pts',(-2.85518555380051,6.13516132252192,
136.941466653642));
#241534=CARTESIAN_POINT('Ctrl Pts',(-3.02382794858743,6.05667841000479,
136.95021630808));
#241535=CARTESIAN_POINT('Ctrl Pts',(-3.18923239109328,5.97123819492056,
136.958965962517));
#241536=CARTESIAN_POINT('Ctrl Pts',(-3.35083705967737,5.87913088810691,
136.967715616955));
#241537=CARTESIAN_POINT('Ctrl Pts',(-3.51243888042425,5.78702520443087,
136.976465117204));
#241538=CARTESIAN_POINT('Ctrl Pts',(-3.67024081223702,5.68825280605775,
136.985214617453));
#241539=CARTESIAN_POINT('Ctrl Pts',(-3.82370687544401,5.58314917682505,
136.993964117702));
#241540=CARTESIAN_POINT('Ctrl Pts',(-3.97717043817814,5.47804726008022,
137.002713475392));
#241541=CARTESIAN_POINT('Ctrl Pts',(-4.12629803722458,5.36661448084237,
137.011462833083));
#241542=CARTESIAN_POINT('Ctrl Pts',(-4.27058317206905,5.24922931204579,
137.020212190773));
#241543=CARTESIAN_POINT('Ctrl Pts',(-4.41486614774839,5.13184589986788,
137.028961417533));
#241544=CARTESIAN_POINT('Ctrl Pts',(-4.55430658194423,5.00851045723026,
137.037710644293));
#241545=CARTESIAN_POINT('Ctrl Pts',(-4.6884308900186,4.87964187103105,137.046459871053));
#241546=CARTESIAN_POINT('Ctrl Pts',(-4.8225533691786,4.75077504207937,137.055208978509));
#241547=CARTESIAN_POINT('Ctrl Pts',(-4.95135966065167,4.61637541908059,
137.063958085965));
#241548=CARTESIAN_POINT('Ctrl Pts',(-5.07441230869284,4.476899454018,137.072707193421));
#241549=CARTESIAN_POINT('Ctrl Pts',(-5.19746344226446,4.3374252055548,137.081456193198));
#241550=CARTESIAN_POINT('Ctrl Pts',(-5.31476088454787,4.1928749549131,137.090205192974));
#241551=CARTESIAN_POINT('Ctrl Pts',(-5.42590627628865,4.0437396158669,137.09895419275));
#241552=CARTESIAN_POINT('Ctrl Pts',(-5.53706380672674,3.89458798906724,
137.107704148045));
#241553=CARTESIAN_POINT('Ctrl Pts',(-5.64206777071866,3.7408505015528,137.11645410334));
#241554=CARTESIAN_POINT('Ctrl Pts',(-5.74056148164006,3.58304938223163,
137.125204058634));
#241555=CARTESIAN_POINT('Ctrl Pts',(-5.83905138951881,3.42525435593287,
137.133953676075));
#241556=CARTESIAN_POINT('Ctrl Pts',(-5.93103139557648,3.26339625497191,
137.142703293517));
#241557=CARTESIAN_POINT('Ctrl Pts',(-6.01618907820841,3.09802485065015,
137.151452910958));
#241558=CARTESIAN_POINT('Ctrl Pts',(-6.10134392544986,2.93265895249636,
137.160202237074));
#241559=CARTESIAN_POINT('Ctrl Pts',(-6.17967677261841,2.76378023986016,
137.168951563189));
#241560=CARTESIAN_POINT('Ctrl Pts',(-6.25092157009239,2.59196229227081,
137.177700889305));
#241561=CARTESIAN_POINT('Ctrl Pts',(-6.3221643740777,2.42014915229049,137.186449970608));
#241562=CARTESIAN_POINT('Ctrl Pts',(-6.38631941548939,2.24539720662801,
137.19519905191));
#241563=CARTESIAN_POINT('Ctrl Pts',(-6.44316881037556,2.06829994947628,
137.203948133213));
#241564=CARTESIAN_POINT('Ctrl Pts',(-6.50002334524592,1.89118668024382,
137.212698005555));
#241565=CARTESIAN_POINT('Ctrl Pts',(-6.54957082411117,1.71172794807624,
137.221447877897));
#241566=CARTESIAN_POINT('Ctrl Pts',(-6.59164294296104,1.53053334250251,
137.23019775024));
#241567=CARTESIAN_POINT('Ctrl Pts',(-6.6337121408215,1.34935131693519,137.238947015095));
#241568=CARTESIAN_POINT('Ctrl Pts',(-6.66830695239702,1.16643393829691,
137.24769627995));
#241569=CARTESIAN_POINT('Ctrl Pts',(-6.69530988153998,0.982402458340346,
137.256445544804));
#241570=CARTESIAN_POINT('Ctrl Pts',(-6.72231419690491,0.798361530946396,
137.265195258811));
#241571=CARTESIAN_POINT('Ctrl Pts',(-6.74172580829284,0.613206671361794,
137.273944972819));
#241572=CARTESIAN_POINT('Ctrl Pts',(-6.75347878028184,0.427566795112697,
137.282694686826));
#241573=CARTESIAN_POINT('Ctrl Pts',(-6.76248992368205,0.285234494206634,
137.289403196614));
#241574=CARTESIAN_POINT('Ctrl Pts',(-6.76699999999985,0.142617266095565,
137.296111706402));
#241575=CARTESIAN_POINT('Ctrl Pts',(-6.767,6.94095400683209E-12,137.30282021619));
#241576=CARTESIAN_POINT('',(3.93014697525799,-5.50874157615607,137.999994970183));
#241577=CARTESIAN_POINT('Ctrl Pts',(-6.76699661606879,-0.00676743035154104,
137.30282021619));
#241578=CARTESIAN_POINT('Ctrl Pts',(-6.76675997058177,-0.243397750383354,
137.313965237425));
#241579=CARTESIAN_POINT('Ctrl Pts',(-6.75410846046182,-0.479452755848537,
137.32511025866));
#241580=CARTESIAN_POINT('Ctrl Pts',(-6.72924119810341,-0.713864061112333,
137.336255279896));
#241581=CARTESIAN_POINT('Ctrl Pts',(-6.7034162722948,-0.957302783070773,
137.347829507182));
#241582=CARTESIAN_POINT('Ctrl Pts',(-6.66441646993814,-1.19896933863425,
137.359403734469));
#241583=CARTESIAN_POINT('Ctrl Pts',(-6.61251193072666,-1.43769780065132,
137.370977961756));
#241584=CARTESIAN_POINT('Ctrl Pts',(-6.58579060248779,-1.56059922103628,
137.376936568289));
#241585=CARTESIAN_POINT('Ctrl Pts',(-6.55564981007044,-1.68272237431578,
137.382895174822));
#241586=CARTESIAN_POINT('Ctrl Pts',(-6.52213127688092,-1.80391036560347,
137.388853781355));
#241587=CARTESIAN_POINT('Ctrl Pts',(-6.476833696767,-1.96768611059689,137.396906354995));
#241588=CARTESIAN_POINT('Ctrl Pts',(-6.42527716931142,-2.13006556088003,
137.404958928634));
#241589=CARTESIAN_POINT('Ctrl Pts',(-6.36755898385533,-2.29051993816323,
137.413011502274));
#241590=CARTESIAN_POINT('Ctrl Pts',(-6.30991413540764,-2.45077044133083,
137.421053844274));
#241591=CARTESIAN_POINT('Ctrl Pts',(-6.24612333029497,-2.60910039008183,
137.429096186274));
#241592=CARTESIAN_POINT('Ctrl Pts',(-6.17633473175018,-2.76499155177306,
137.437138528274));
#241593=CARTESIAN_POINT('Ctrl Pts',(-6.10661936852886,-2.92071912313737,
137.445172430737));
#241594=CARTESIAN_POINT('Ctrl Pts',(-6.03091888762117,-3.07401266096776,
137.453206333199));
#241595=CARTESIAN_POINT('Ctrl Pts',(-5.94943105221846,-3.22436957480043,
137.461240235661));
#241596=CARTESIAN_POINT('Ctrl Pts',(-5.86801073572888,-3.37460190641353,
137.46926748142));
#241597=CARTESIAN_POINT('Ctrl Pts',(-5.78081278558136,-3.52190212884627,
137.477294727179));
#241598=CARTESIAN_POINT('Ctrl Pts',(-5.6880827714529,-3.66578823516862,
137.485321972938));
#241599=CARTESIAN_POINT('Ctrl Pts',(-5.59540914186583,-3.80958685145666,
137.493344337725));
#241600=CARTESIAN_POINT('Ctrl Pts',(-5.49721034636524,-3.94997516976006,
137.501366702512));
#241601=CARTESIAN_POINT('Ctrl Pts',(-5.39377746694698,-4.08649649908758,
137.509389067299));
#241602=CARTESIAN_POINT('Ctrl Pts',(-5.28774626359827,-4.22644736299833,
137.51761296087));
#241603=CARTESIAN_POINT('Ctrl Pts',(-5.17621473704244,-4.36233404085406,
137.525836854441));
#241604=CARTESIAN_POINT('Ctrl Pts',(-5.05954349078207,-4.49369654793076,
137.534060748012));
#241605=CARTESIAN_POINT('Ctrl Pts',(-4.94577196478572,-4.62179420153317,
137.542080246828));
#241606=CARTESIAN_POINT('Ctrl Pts',(-4.82711344885099,-4.74558962290845,
137.550099745643));
#241607=CARTESIAN_POINT('Ctrl Pts',(-4.70394248253506,-4.86469054730123,
137.558119244459));
#241608=CARTESIAN_POINT('Ctrl Pts',(-4.58075989890919,-4.9838027051234,
137.566139499663));
#241609=CARTESIAN_POINT('Ctrl Pts',(-4.45306428714298,-5.09821922345179,
137.574159754866));
#241610=CARTESIAN_POINT('Ctrl Pts',(-4.32126605820613,-5.20758568380739,
137.582180010069));
#241611=CARTESIAN_POINT('Ctrl Pts',(-4.18942909599465,-5.31698428511949,
137.59020262229));
#241612=CARTESIAN_POINT('Ctrl Pts',(-4.05348740551106,-5.42132963515267,
137.598225234511));
#241613=CARTESIAN_POINT('Ctrl Pts',(-3.91388323497627,-5.52030859852705,
137.606247846732));
#241614=CARTESIAN_POINT('Ctrl Pts',(-3.7681257785839,-5.62365022422875,
137.614624068922));
#241615=CARTESIAN_POINT('Ctrl Pts',(-3.61837602773323,-5.72114139189279,
137.623000291111));
#241616=CARTESIAN_POINT('Ctrl Pts',(-3.46516838418653,-5.81247770483759,
137.6313765133));
#241617=CARTESIAN_POINT('Ctrl Pts',(-3.31817049754964,-5.90011200731284,
137.639413233475));
#241618=CARTESIAN_POINT('Ctrl Pts',(-3.16798987172157,-5.98208046317299,
137.64744995365));
#241619=CARTESIAN_POINT('Ctrl Pts',(-3.01512071593136,-6.05816276344253,
137.655486673825));
#241620=CARTESIAN_POINT('Ctrl Pts',(-2.86213645315186,-6.13430235194969,
137.663529445467));
#241621=CARTESIAN_POINT('Ctrl Pts',(-2.70645996954239,-6.20454680768543,
137.671572217109));
#241622=CARTESIAN_POINT('Ctrl Pts',(-2.54860298262317,-6.26872489721509,
137.679614988751));
#241623=CARTESIAN_POINT('Ctrl Pts',(-2.39052228006946,-6.33299394022295,
137.687669158645));
#241624=CARTESIAN_POINT('Ctrl Pts',(-2.23025525810373,-6.39117933781976,
137.695723328539));
#241625=CARTESIAN_POINT('Ctrl Pts',(-2.06832677251032,-6.44316019994203,
137.703777498433));
#241626=CARTESIAN_POINT('Ctrl Pts',(-2.04832227399967,-6.44958186858851,
137.70477250329));
#241627=CARTESIAN_POINT('Ctrl Pts',(-2.02829242796762,-6.45590890876347,
137.705767508147));
#241628=CARTESIAN_POINT('Ctrl Pts',(-2.00823823124795,-6.46214114721693,
137.706762513004));
#241629=CARTESIAN_POINT('Ctrl Pts',(-1.84137858411901,-6.51399608430093,
137.715041386581));
#241630=CARTESIAN_POINT('Ctrl Pts',(-1.67227889322659,-6.55945574328369,
137.723320260158));
#241631=CARTESIAN_POINT('Ctrl Pts',(-1.50146737897553,-6.59832438652969,
137.731599133736));
#241632=CARTESIAN_POINT('Ctrl Pts',(-1.33086001777546,-6.63714657417144,
137.739868112445));
#241633=CARTESIAN_POINT('Ctrl Pts',(-1.15854525003179,-6.66939335785156,
137.748137091155));
#241634=CARTESIAN_POINT('Ctrl Pts',(-0.985068047904076,-6.69491821764825,
137.756406069864));
#241635=CARTESIAN_POINT('Ctrl Pts',(-0.811764623609784,-6.72041750835126,
137.764666765265));
#241636=CARTESIAN_POINT('Ctrl Pts',(-0.637301432280176,-6.73920823695477,
137.772927460666));
#241637=CARTESIAN_POINT('Ctrl Pts',(-0.462235428407887,-6.75119451717432,
137.781188156067));
#241638=CARTESIAN_POINT('Ctrl Pts',(-0.287310939905778,-6.76317110823181,
137.789442173899));
#241639=CARTESIAN_POINT('Ctrl Pts',(-0.111784961143709,-6.76835418502657,
137.797696191731));
#241640=CARTESIAN_POINT('Ctrl Pts',(0.06377845566846,-6.76669943980022,
137.805950209562));
#241641=CARTESIAN_POINT('Ctrl Pts',(0.239228010772019,-6.7650457677594,
137.814198874248));
#241642=CARTESIAN_POINT('Ctrl Pts',(0.414714602696616,-6.75656311526461,
137.822447538934));
#241643=CARTESIAN_POINT('Ctrl Pts',(0.589672091611263,-6.74125921652437,
137.83069620362));
#241644=CARTESIAN_POINT('Ctrl Pts',(0.764567338287138,-6.7259607622434,
137.838941933791));
#241645=CARTESIAN_POINT('Ctrl Pts',(0.938933504922963,-6.70384592580967,
137.847187663962));
#241646=CARTESIAN_POINT('Ctrl Pts',(1.11220716957069,-6.67497447275685,
137.855433394133));
#241647=CARTESIAN_POINT('Ctrl Pts',(1.285449543949,-6.64610823339617,137.863677635265));
#241648=CARTESIAN_POINT('Ctrl Pts',(1.45759946058247,-6.61048786635831,
137.871921876398));
#241649=CARTESIAN_POINT('Ctrl Pts',(1.62810119702784,-6.56822468344655,
137.880166117531));
#241650=CARTESIAN_POINT('Ctrl Pts',(1.79860200943978,-6.52596172957993,
137.888410313984));
#241651=CARTESIAN_POINT('Ctrl Pts',(1.9674543163267,-6.47705611755172,137.896654510437));
#241652=CARTESIAN_POINT('Ctrl Pts',(2.13411500467748,-6.4216697319942,137.90489870689));
#241653=CARTESIAN_POINT('Ctrl Pts',(2.30086722539536,-6.3662529274637,137.91314743117));
#241654=CARTESIAN_POINT('Ctrl Pts',(2.46542508579837,-6.30434834740739,
137.921396155451));
#241655=CARTESIAN_POINT('Ctrl Pts',(2.62726227747752,-6.23616724642177,
137.929644879731));
#241656=CARTESIAN_POINT('Ctrl Pts',(2.78914341309458,-6.16796763210162,
137.937895843802));
#241657=CARTESIAN_POINT('Ctrl Pts',(2.94830208456367,-6.09348824471639,
137.946146807873));
#241658=CARTESIAN_POINT('Ctrl Pts',(3.10423415084922,-6.01298755500969,
137.954397771944));
#241659=CARTESIAN_POINT('Ctrl Pts',(3.26031933642722,-5.93240781672149,
137.962656838144));
#241660=CARTESIAN_POINT('Ctrl Pts',(3.41317127472098,-5.8457951308704,137.970915904345));
#241661=CARTESIAN_POINT('Ctrl Pts',(3.56231163725544,-5.75345329337733,
137.979174970545));
#241662=CARTESIAN_POINT('Ctrl Pts',(3.68763259641482,-5.67585949215202,
137.986114970424));
#241663=CARTESIAN_POINT('Ctrl Pts',(3.81033325902537,-5.59422126474488,
137.993054970304));
#241664=CARTESIAN_POINT('Ctrl Pts',(3.93014697525799,-5.50874157615607,
137.999994970183));
#241665=CARTESIAN_POINT('',(-3.92888236737319,-5.50964357679733,138.));
#241666=CARTESIAN_POINT('Origin',(0.,0.,138.));
#241667=CARTESIAN_POINT('',(-6.767,6.64344400075779E-12,137.69717978381));
#241668=CARTESIAN_POINT('Ctrl Pts',(-6.76699999999825,4.86320023540543E-6,
137.697286552978));
#241669=CARTESIAN_POINT('Ctrl Pts',(-6.76700012425513,-0.17289492391004,
137.705426224725));
#241670=CARTESIAN_POINT('Ctrl Pts',(-6.76036941594973,-0.345936048758181,
137.713565896472));
#241671=CARTESIAN_POINT('Ctrl Pts',(-6.74710141855822,-0.518566724433509,
137.721705568218));
#241672=CARTESIAN_POINT('Ctrl Pts',(-6.73384006786635,-0.691110919518242,
137.729841162338));
#241673=CARTESIAN_POINT('Ctrl Pts',(-6.71394807658885,-0.863244710707634,
137.737976756457));
#241674=CARTESIAN_POINT('Ctrl Pts',(-6.68747105695194,-1.03441764410229,
137.746112350576));
#241675=CARTESIAN_POINT('Ctrl Pts',(-6.66099847292775,-1.20556190142803,
137.754246581764));
#241676=CARTESIAN_POINT('Ctrl Pts',(-6.62794310576004,-1.37574525885523,
137.762380812953));
#241677=CARTESIAN_POINT('Ctrl Pts',(-6.58840230936357,-1.54442352027313,
137.770515044141));
#241678=CARTESIAN_POINT('Ctrl Pts',(-6.54886654853085,-1.71308030032959,
137.778648239426));
#241679=CARTESIAN_POINT('Ctrl Pts',(-6.50284709023229,-1.88023201037332,
137.786781434712));
#241680=CARTESIAN_POINT('Ctrl Pts',(-6.4504921137362,-2.04534605644792,
137.794914629997));
#241681=CARTESIAN_POINT('Ctrl Pts',(-6.39811630240641,-2.21052581019584,
137.803051061913));
#241682=CARTESIAN_POINT('Ctrl Pts',(-6.33940004546313,-2.3736659301633,
137.81118749383));
#241683=CARTESIAN_POINT('Ctrl Pts',(-6.27454113990482,-2.53424988579301,
137.819323925747));
#241684=CARTESIAN_POINT('Ctrl Pts',(-6.21682352896187,-2.67715273305712,
137.826564495223));
#241685=CARTESIAN_POINT('Ctrl Pts',(-6.15424223112599,-2.81803139624315,
137.833805064699));
#241686=CARTESIAN_POINT('Ctrl Pts',(-6.08696823580425,-2.95653626669962,
137.841045634175));
#241687=CARTESIAN_POINT('Ctrl Pts',(-6.00343429352145,-3.12851739847668,
137.850036230167));
#241688=CARTESIAN_POINT('Ctrl Pts',(-5.91263302428386,-3.29690429134303,
137.859026826159));
#241689=CARTESIAN_POINT('Ctrl Pts',(-5.8148925622811,-3.46111448656758,
137.868017422151));
#241690=CARTESIAN_POINT('Ctrl Pts',(-5.71710988895613,-3.62539559949928,
137.877011900926));
#241691=CARTESIAN_POINT('Ctrl Pts',(-5.61238216277252,-3.78549620326186,
137.8860063797));
#241692=CARTESIAN_POINT('Ctrl Pts',(-5.50108187272786,-3.9408612294199,
137.895000858475));
#241693=CARTESIAN_POINT('Ctrl Pts',(-5.38973960828518,-4.0962848479989,
137.903998729314));
#241694=CARTESIAN_POINT('Ctrl Pts',(-5.27181996794762,-4.24696912163422,
137.912996600154));
#241695=CARTESIAN_POINT('Ctrl Pts',(-5.14773770480197,-4.39238950032442,
137.921994470993));
#241696=CARTESIAN_POINT('Ctrl Pts',(-5.02366300552272,-4.53780101440907,
137.930991793336));
#241697=CARTESIAN_POINT('Ctrl Pts',(-4.89342659445217,-4.67794909155439,
137.939989115679));
#241698=CARTESIAN_POINT('Ctrl Pts',(-4.75748267824785,-4.81234325107548,
137.948986438022));
#241699=CARTESIAN_POINT('Ctrl Pts',(-4.62157878878662,-4.94669784015717,
137.957981111232));
#241700=CARTESIAN_POINT('Ctrl Pts',(-4.47997092572928,-5.07530172645476,
137.966975784442));
#241701=CARTESIAN_POINT('Ctrl Pts',(-4.33314991941424,-5.19770148968565,
137.975970457652));
#241702=CARTESIAN_POINT('Ctrl Pts',(-4.20240432861014,-5.30669971657128,
137.983980305102));
#241703=CARTESIAN_POINT('Ctrl Pts',(-4.06752526370029,-5.4107784463858,
137.991990152551));
#241704=CARTESIAN_POINT('Ctrl Pts',(-3.92888236737319,-5.50964357679733,
138.));
#241705=CARTESIAN_POINT('Ctrl Pts',(3.0991061983214,6.01563211736937,137.045755263024));
#241706=CARTESIAN_POINT('Ctrl Pts',(2.9337533076482,6.10081787314656,137.054504710927));
#241707=CARTESIAN_POINT('Ctrl Pts',(2.76488627843052,6.17918207037047,137.063254158829));
#241708=CARTESIAN_POINT('Ctrl Pts',(2.59307866646672,6.2504585455401,137.072003606731));
#241709=CARTESIAN_POINT('Ctrl Pts',(2.42127244185352,6.32173444515046,137.080752983982));
#241710=CARTESIAN_POINT('Ctrl Pts',(2.24652594672447,6.38592262741844,137.089502361232));
#241711=CARTESIAN_POINT('Ctrl Pts',(2.0694326968711,6.44280508110565,137.098251738482));
#241712=CARTESIAN_POINT('Ctrl Pts',(1.89234081822066,6.4996870943617,137.107001047988));
#241713=CARTESIAN_POINT('Ctrl Pts',(1.71290249405578,6.54926340459548,137.115750357493));
#241714=CARTESIAN_POINT('Ctrl Pts',(1.53172716625048,6.59136563150386,137.124499666998));
#241715=CARTESIAN_POINT('Ctrl Pts',(1.35055318107328,6.63346754640711,137.133248911666));
#241716=CARTESIAN_POINT('Ctrl Pts',(1.16764249714418,6.66809542395776,137.141998156333));
#241717=CARTESIAN_POINT('Ctrl Pts',(0.983616340614383,6.69513165624668,
137.150747401));
#241718=CARTESIAN_POINT('Ctrl Pts',(0.799591486713868,6.7221676971596,137.159496583736));
#241719=CARTESIAN_POINT('Ctrl Pts',(0.614451459526737,6.74161215869371,
137.168245766471));
#241720=CARTESIAN_POINT('Ctrl Pts',(0.428825047910307,6.75339900185712,
137.176994949207));
#241721=CARTESIAN_POINT('Ctrl Pts',(0.243199888596977,6.76518576550221,
137.185744072918));
#241722=CARTESIAN_POINT('Ctrl Pts',(0.0570886373917548,6.76931499599835,
137.194493196628));
#241723=CARTESIAN_POINT('Ctrl Pts',(-0.128876626811405,6.76577266947846,
137.203242320339));
#241724=CARTESIAN_POINT('Ctrl Pts',(-0.314840698188485,6.76223036567992,
137.21199138793));
#241725=CARTESIAN_POINT('Ctrl Pts',(-0.500658497951649,6.7510166087922,
137.220740455522));
#241726=CARTESIAN_POINT('Ctrl Pts',(-0.685698951926683,6.73216948296214,
137.229489523113));
#241727=CARTESIAN_POINT('Ctrl Pts',(-0.870738280460354,6.71332247176287,
137.238238537492));
#241728=CARTESIAN_POINT('Ctrl Pts',(-1.05499998761304,6.68684221356178,
137.24698755187));
#241729=CARTESIAN_POINT('Ctrl Pts',(-1.23785829161477,6.65281863948512,
137.255736566249));
#241730=CARTESIAN_POINT('Ctrl Pts',(-1.43007412917444,6.61705395368852,
137.264933299948));
#241731=CARTESIAN_POINT('Ctrl Pts',(-1.62073882535816,6.57295372727783,
137.274130033647));
#241732=CARTESIAN_POINT('Ctrl Pts',(-1.80913696091522,6.52068343478277,
137.283326767346));
#241733=CARTESIAN_POINT('Ctrl Pts',(-1.9883835618612,6.47095219815196,137.29207676506));
#241734=CARTESIAN_POINT('Ctrl Pts',(-2.16557827572541,6.41382586850888,
137.300826762774));
#241735=CARTESIAN_POINT('Ctrl Pts',(-2.34011918621708,6.34949849943275,
137.309576760487));
#241736=CARTESIAN_POINT('Ctrl Pts',(-2.514656556911,6.2851724349555,137.318326580746));
#241737=CARTESIAN_POINT('Ctrl Pts',(-2.68653996295324,6.21364572242376,
137.327076401004));
#241738=CARTESIAN_POINT('Ctrl Pts',(-2.85518555379978,6.13516132252226,
137.335826221262));
#241739=CARTESIAN_POINT('Ctrl Pts',(-3.02382794858668,6.05667841000517,
137.3445758757));
#241740=CARTESIAN_POINT('Ctrl Pts',(-3.18923239109251,5.97123819492097,
137.353325530137));
#241741=CARTESIAN_POINT('Ctrl Pts',(-3.35083705967659,5.87913088810735,
137.362075184575));
#241742=CARTESIAN_POINT('Ctrl Pts',(-3.51243888042357,5.78702520443129,
137.370824684824));
#241743=CARTESIAN_POINT('Ctrl Pts',(-3.67024081223644,5.68825280605813,
137.379574185073));
#241744=CARTESIAN_POINT('Ctrl Pts',(-3.82370687544351,5.58314917682539,
137.388323685322));
#241745=CARTESIAN_POINT('Ctrl Pts',(-3.97717043817763,5.47804726008059,
137.397073043012));
#241746=CARTESIAN_POINT('Ctrl Pts',(-4.12629803722406,5.36661448084277,
137.405822400703));
#241747=CARTESIAN_POINT('Ctrl Pts',(-4.27058317206852,5.24922931204622,
137.414571758393));
#241748=CARTESIAN_POINT('Ctrl Pts',(-4.41486614774784,5.13184589986834,
137.423320985153));
#241749=CARTESIAN_POINT('Ctrl Pts',(-4.55430658194368,5.00851045723076,
137.432070211913));
#241750=CARTESIAN_POINT('Ctrl Pts',(-4.68843089001804,4.87964187103159,
137.440819438673));
#241751=CARTESIAN_POINT('Ctrl Pts',(-4.82255336917822,4.75077504207976,
137.449568546129));
#241752=CARTESIAN_POINT('Ctrl Pts',(-4.95135966065145,4.61637541908083,
137.458317653585));
#241753=CARTESIAN_POINT('Ctrl Pts',(-5.07441230869278,4.47689945401807,
137.467066761041));
#241754=CARTESIAN_POINT('Ctrl Pts',(-5.1974634422643,4.33742520555499,137.475815760818));
#241755=CARTESIAN_POINT('Ctrl Pts',(-5.31476088454762,4.19287495491342,
137.484564760594));
#241756=CARTESIAN_POINT('Ctrl Pts',(-5.42590627628832,4.04373961586736,
137.49331376037));
#241757=CARTESIAN_POINT('Ctrl Pts',(-5.53706380672648,3.89458798906763,
137.502063715665));
#241758=CARTESIAN_POINT('Ctrl Pts',(-5.64206777071847,3.7408505015531,137.51081367096));
#241759=CARTESIAN_POINT('Ctrl Pts',(-5.74056148163992,3.58304938223186,
137.519563626254));
#241760=CARTESIAN_POINT('Ctrl Pts',(-5.83905138951873,3.42525435593301,
137.528313243695));
#241761=CARTESIAN_POINT('Ctrl Pts',(-5.93103139557645,3.26339625497197,
137.537062861137));
#241762=CARTESIAN_POINT('Ctrl Pts',(-6.01618907820842,3.09802485065013,
137.545812478578));
#241763=CARTESIAN_POINT('Ctrl Pts',(-6.10134392544986,2.93265895249636,
137.554561804694));
#241764=CARTESIAN_POINT('Ctrl Pts',(-6.1796767726184,2.76378023986018,137.563311130809));
#241765=CARTESIAN_POINT('Ctrl Pts',(-6.25092157009236,2.59196229227086,
137.572060456925));
#241766=CARTESIAN_POINT('Ctrl Pts',(-6.32216437407767,2.42014915229057,
137.580809538228));
#241767=CARTESIAN_POINT('Ctrl Pts',(-6.38631941548935,2.24539720662811,
137.58955861953));
#241768=CARTESIAN_POINT('Ctrl Pts',(-6.44316881037552,2.06829994947642,
137.598307700833));
#241769=CARTESIAN_POINT('Ctrl Pts',(-6.50002334524583,1.8911866802441,137.607057573175));
#241770=CARTESIAN_POINT('Ctrl Pts',(-6.54957082411105,1.71172794807668,
137.615807445517));
#241771=CARTESIAN_POINT('Ctrl Pts',(-6.5916429429609,1.53053334250311,137.62455731786));
#241772=CARTESIAN_POINT('Ctrl Pts',(-6.63371214082143,1.34935131693556,
137.633306582715));
#241773=CARTESIAN_POINT('Ctrl Pts',(-6.668306952397,1.16643393829707,137.642055847569));
#241774=CARTESIAN_POINT('Ctrl Pts',(-6.69530988153999,0.98240245834028,
137.650805112424));
#241775=CARTESIAN_POINT('Ctrl Pts',(-6.72231419690491,0.798361530946359,
137.659554826431));
#241776=CARTESIAN_POINT('Ctrl Pts',(-6.74172580829284,0.613206671361785,
137.668304540438));
#241777=CARTESIAN_POINT('Ctrl Pts',(-6.75347878028184,0.427566795112718,
137.677054254445));
#241778=CARTESIAN_POINT('Ctrl Pts',(-6.76248992368206,0.285234494206549,
137.683762764234));
#241779=CARTESIAN_POINT('Ctrl Pts',(-6.76699999999986,0.142617266095373,
137.690471274022));
#241780=CARTESIAN_POINT('Ctrl Pts',(-6.767,6.64344399020961E-12,137.69717978381));
#241781=CARTESIAN_POINT('Origin',(-1.11022302462516E-15,0.,-22.));
#241782=CARTESIAN_POINT('',(6.,0.,-24.));
#241783=CARTESIAN_POINT('',(5.65685424949238,-2.,-22.));
#241784=CARTESIAN_POINT('Ctrl Pts',(6.,9.71445146547012E-16,-24.));
#241785=CARTESIAN_POINT('Ctrl Pts',(6.,-0.253174643734702,-24.));
#241786=CARTESIAN_POINT('Ctrl Pts',(5.98240475886912,-0.521932274441712,
-23.9490088416061));
#241787=CARTESIAN_POINT('Ctrl Pts',(5.9188739106068,-1.01415562391481,-23.7442869722332));
#241788=CARTESIAN_POINT('Ctrl Pts',(5.87374622031366,-1.23776803829002,
-23.5906590864562));
#241789=CARTESIAN_POINT('Ctrl Pts',(5.78813771212597,-1.59074095999941,
-23.2376861647468));
#241790=CARTESIAN_POINT('Ctrl Pts',(5.74186082552466,-1.7443058152527,-23.0141063599154));
#241791=CARTESIAN_POINT('Ctrl Pts',(5.67565356574251,-1.94898067853762,
-22.522003946927));
#241792=CARTESIAN_POINT('Ctrl Pts',(5.65685424949238,-2.,-22.2532921208158));
#241793=CARTESIAN_POINT('Ctrl Pts',(5.65685424949238,-2.,-22.));
#241794=CARTESIAN_POINT('',(6.,0.,-20.));
#241795=CARTESIAN_POINT('Ctrl Pts',(6.,-3.46944695195361E-16,-20.));
#241796=CARTESIAN_POINT('Ctrl Pts',(6.,0.253174643734703,-20.));
#241797=CARTESIAN_POINT('Ctrl Pts',(5.98240475886912,0.521932274441713,
-20.0509911583939));
#241798=CARTESIAN_POINT('Ctrl Pts',(5.9188739106068,1.01415562391481,-20.2557130277668));
#241799=CARTESIAN_POINT('Ctrl Pts',(5.87374622031365,1.23776803829002,-20.4093409135438));
#241800=CARTESIAN_POINT('Ctrl Pts',(5.78813771212597,1.59074095999941,-20.7623138352532));
#241801=CARTESIAN_POINT('Ctrl Pts',(5.74186082552466,1.7443058152527,-20.9858936400846));
#241802=CARTESIAN_POINT('Ctrl Pts',(5.67565356574251,1.94898067853762,-21.477996053073));
#241803=CARTESIAN_POINT('Ctrl Pts',(5.65685424949238,2.,-21.7467078791842));
#241804=CARTESIAN_POINT('Ctrl Pts',(5.65685424949238,2.,-22.2532921208158));
#241805=CARTESIAN_POINT('Ctrl Pts',(5.67565356574251,1.94898067853762,-22.5220039469271));
#241806=CARTESIAN_POINT('Ctrl Pts',(5.74186082552466,1.7443058152527,-23.0141063599154));
#241807=CARTESIAN_POINT('Ctrl Pts',(5.78813771212597,1.59074095999941,-23.2376861647468));
#241808=CARTESIAN_POINT('Ctrl Pts',(5.87374622031365,1.23776803829002,-23.5906590864562));
#241809=CARTESIAN_POINT('Ctrl Pts',(5.9188739106068,1.01415562391481,-23.7442869722332));
#241810=CARTESIAN_POINT('Ctrl Pts',(5.98240475886912,0.521932274441715,
-23.9490088416061));
#241811=CARTESIAN_POINT('Ctrl Pts',(6.,0.253174643734703,-24.));
#241812=CARTESIAN_POINT('Ctrl Pts',(6.,7.11236625150491E-16,-24.));
#241813=CARTESIAN_POINT('Ctrl Pts',(5.65685424949238,-2.,-22.));
#241814=CARTESIAN_POINT('Ctrl Pts',(5.65685424949238,-2.,-21.7467078791842));
#241815=CARTESIAN_POINT('Ctrl Pts',(5.67565356574251,-1.94898067853762,
-21.477996053073));
#241816=CARTESIAN_POINT('Ctrl Pts',(5.74186082552466,-1.7443058152527,-20.9858936400846));
#241817=CARTESIAN_POINT('Ctrl Pts',(5.78813771212597,-1.59074095999941,
-20.7623138352532));
#241818=CARTESIAN_POINT('Ctrl Pts',(5.87374622031365,-1.23776803829002,
-20.4093409135438));
#241819=CARTESIAN_POINT('Ctrl Pts',(5.9188739106068,-1.01415562391481,-20.2557130277668));
#241820=CARTESIAN_POINT('Ctrl Pts',(5.98240475886912,-0.521932274441714,
-20.0509911583939));
#241821=CARTESIAN_POINT('Ctrl Pts',(6.,-0.253174643734704,-20.));
#241822=CARTESIAN_POINT('Ctrl Pts',(6.,-1.04083408558608E-16,-20.));
#241823=CARTESIAN_POINT('',(-5.65685424949238,-2.,-22.));
#241824=CARTESIAN_POINT('',(-1.11022302462516E-15,-2.,-22.));
#241825=CARTESIAN_POINT('',(-6.,0.,-20.));
#241826=CARTESIAN_POINT('Ctrl Pts',(-6.,-1.38777878078145E-16,-20.));
#241827=CARTESIAN_POINT('Ctrl Pts',(-6.,-0.253174643734703,-20.));
#241828=CARTESIAN_POINT('Ctrl Pts',(-5.98240475886912,-0.521932274441714,
-20.0509911583939));
#241829=CARTESIAN_POINT('Ctrl Pts',(-5.9188739106068,-1.01415562391481,
-20.2557130277668));
#241830=CARTESIAN_POINT('Ctrl Pts',(-5.87374622031365,-1.23776803829002,
-20.4093409135438));
#241831=CARTESIAN_POINT('Ctrl Pts',(-5.78813771212597,-1.59074095999941,
-20.7623138352532));
#241832=CARTESIAN_POINT('Ctrl Pts',(-5.74186082552466,-1.7443058152527,
-20.9858936400846));
#241833=CARTESIAN_POINT('Ctrl Pts',(-5.67565356574251,-1.94898067853762,
-21.477996053073));
#241834=CARTESIAN_POINT('Ctrl Pts',(-5.65685424949238,-2.,-21.7467078791842));
#241835=CARTESIAN_POINT('Ctrl Pts',(-5.65685424949238,-2.,-22.));
#241836=CARTESIAN_POINT('',(-6.,0.,-24.));
#241837=CARTESIAN_POINT('Ctrl Pts',(-6.,6.24500451351651E-16,-24.));
#241838=CARTESIAN_POINT('Ctrl Pts',(-6.,0.253174643734704,-24.));
#241839=CARTESIAN_POINT('Ctrl Pts',(-5.98240475886912,0.521932274441715,
-23.9490088416061));
#241840=CARTESIAN_POINT('Ctrl Pts',(-5.9188739106068,1.01415562391481,-23.7442869722332));
#241841=CARTESIAN_POINT('Ctrl Pts',(-5.87374622031365,1.23776803829002,
-23.5906590864562));
#241842=CARTESIAN_POINT('Ctrl Pts',(-5.78813771212597,1.59074095999941,
-23.2376861647468));
#241843=CARTESIAN_POINT('Ctrl Pts',(-5.74186082552466,1.7443058152527,-23.0141063599154));
#241844=CARTESIAN_POINT('Ctrl Pts',(-5.67565356574251,1.94898067853762,
-22.522003946927));
#241845=CARTESIAN_POINT('Ctrl Pts',(-5.65685424949238,2.,-22.2532921208158));
#241846=CARTESIAN_POINT('Ctrl Pts',(-5.65685424949238,2.,-21.7467078791842));
#241847=CARTESIAN_POINT('Ctrl Pts',(-5.67565356574251,1.94898067853762,
-21.477996053073));
#241848=CARTESIAN_POINT('Ctrl Pts',(-5.74186082552466,1.7443058152527,-20.9858936400846));
#241849=CARTESIAN_POINT('Ctrl Pts',(-5.78813771212597,1.59074095999941,
-20.7623138352532));
#241850=CARTESIAN_POINT('Ctrl Pts',(-5.87374622031365,1.23776803829002,
-20.4093409135438));
#241851=CARTESIAN_POINT('Ctrl Pts',(-5.9188739106068,1.01415562391481,-20.2557130277668));
#241852=CARTESIAN_POINT('Ctrl Pts',(-5.98240475886912,0.521932274441713,
-20.0509911583939));
#241853=CARTESIAN_POINT('Ctrl Pts',(-6.,0.253174643734703,-20.));
#241854=CARTESIAN_POINT('Ctrl Pts',(-6.,-2.94902990916057E-16,-20.));
#241855=CARTESIAN_POINT('Ctrl Pts',(-5.65685424949238,-2.,-22.));
#241856=CARTESIAN_POINT('Ctrl Pts',(-5.65685424949238,-2.,-22.2532921208158));
#241857=CARTESIAN_POINT('Ctrl Pts',(-5.67565356574251,-1.94898067853762,
-22.522003946927));
#241858=CARTESIAN_POINT('Ctrl Pts',(-5.74186082552466,-1.7443058152527,
-23.0141063599154));
#241859=CARTESIAN_POINT('Ctrl Pts',(-5.78813771212597,-1.59074095999941,
-23.2376861647468));
#241860=CARTESIAN_POINT('Ctrl Pts',(-5.87374622031365,-1.23776803829002,
-23.5906590864562));
#241861=CARTESIAN_POINT('Ctrl Pts',(-5.9188739106068,-1.01415562391481,
-23.7442869722332));
#241862=CARTESIAN_POINT('Ctrl Pts',(-5.98240475886912,-0.521932274441713,
-23.9490088416061));
#241863=CARTESIAN_POINT('Ctrl Pts',(-6.,-0.253174643734702,-24.));
#241864=CARTESIAN_POINT('Ctrl Pts',(-6.,1.05818132034585E-15,-24.));
#241865=CARTESIAN_POINT('Ctrl Pts',(-2.92234961580469,6.09539287100994,
7.33528614149682));
#241866=CARTESIAN_POINT('Ctrl Pts',(-3.93714486470952,5.60886538126811,
7.38828008561611));
#241867=CARTESIAN_POINT('Ctrl Pts',(-5.71537785310802,4.12322732536813,
7.49425881834364));
#241868=CARTESIAN_POINT('Ctrl Pts',(-6.99675326026537,0.871633769604885,
7.65322233967944));
#241869=CARTESIAN_POINT('Ctrl Pts',(-6.55091532659029,-2.56655158848262,
7.81217670550419));
#241870=CARTESIAN_POINT('Ctrl Pts',(-3.86326988828824,-6.37353479344272,
8.02411585993721));
#241871=CARTESIAN_POINT('Ctrl Pts',(2.36377026589466,-7.63953912008178,
8.28903980297847));
#241872=CARTESIAN_POINT('Ctrl Pts',(7.71195073098936,-2.1230738351773,8.606948534628));
#241873=CARTESIAN_POINT('Ctrl Pts',(6.24580147088772,4.06257053960132,8.87187247766926));
#241874=CARTESIAN_POINT('Ctrl Pts',(2.36304990153233,6.62817509056407,9.08381163210228));
#241875=CARTESIAN_POINT('Ctrl Pts',(-1.10032041202936,6.96614410245639,
9.24276599792703));
#241876=CARTESIAN_POINT('Ctrl Pts',(-4.28427191756992,5.58239383986575,
9.40172036375181));
#241877=CARTESIAN_POINT('Ctrl Pts',(-7.19973962574471,1.93580196426138,
9.61365951818479));
#241878=CARTESIAN_POINT('Ctrl Pts',(-6.77647567883404,-3.11256971208317,
9.82559867261786));
#241879=CARTESIAN_POINT('Ctrl Pts',(-3.29440639851251,-6.21029458306668,
10.0375378270508));
#241880=CARTESIAN_POINT('Ctrl Pts',(1.20026516117126,-7.35377856012818,
10.2494769814839));
#241881=CARTESIAN_POINT('Ctrl Pts',(6.76952833401824,-4.26652457372789,
10.5144009245251));
#241882=CARTESIAN_POINT('Ctrl Pts',(7.2358798186972,3.40243708410996,10.8323096561747));
#241883=CARTESIAN_POINT('Ctrl Pts',(2.10440537187899,7.14786414098517,11.0972335992159));
#241884=CARTESIAN_POINT('Ctrl Pts',(-2.51597475780455,6.57195704382539,
11.3091727536489));
#241885=CARTESIAN_POINT('Ctrl Pts',(-5.36562902415266,4.57639845624688,
11.4681271194737));
#241886=CARTESIAN_POINT('Ctrl Pts',(-6.88511019966572,1.4546699720389,11.6270814852985));
#241887=CARTESIAN_POINT('Ctrl Pts',(-6.72813106585684,-3.21150195768999,
11.8390206397315));
#241888=CARTESIAN_POINT('Ctrl Pts',(-3.12381767200652,-6.77133116212613,
12.0509597941645));
#241889=CARTESIAN_POINT('Ctrl Pts',(1.53599132603708,-6.86015371718211,
12.2628989485975));
#241890=CARTESIAN_POINT('Ctrl Pts',(5.69401924554645,-4.80588969870767,
12.4748381030305));
#241891=CARTESIAN_POINT('Ctrl Pts',(7.91717704197876,1.16114852504975,12.7397620460718));
#241892=CARTESIAN_POINT('Ctrl Pts',(3.2842236423008,7.29029237713238,13.0576707777213));
#241893=CARTESIAN_POINT('Ctrl Pts',(-3.04967515282414,6.79852489801197,
13.3225947207625));
#241894=CARTESIAN_POINT('Ctrl Pts',(-6.18512036033732,3.35634566664468,
13.5345338751956));
#241895=CARTESIAN_POINT('Ctrl Pts',(-7.05217846098628,-0.0127773233050138,
13.6934882410203));
#241896=CARTESIAN_POINT('Ctrl Pts',(-6.176389907705,-3.37239090485859,13.8524426068451));
#241897=CARTESIAN_POINT('Ctrl Pts',(-3.02267724704907,-6.81505045200992,
14.0643817612781));
#241898=CARTESIAN_POINT('Ctrl Pts',(2.0303998283825,-7.17541903106724,14.2763209157112));
#241899=CARTESIAN_POINT('Ctrl Pts',(5.62807325196858,-4.21257292617558,
14.4882600701441));
#241900=CARTESIAN_POINT('Ctrl Pts',(7.45088764127239,0.0519955308776357,
14.7001992245772));
#241901=CARTESIAN_POINT('Ctrl Pts',(5.25932460636586,6.03071000917909,14.9651231676184));
#241902=CARTESIAN_POINT('Ctrl Pts',(-2.24603046352291,7.67397127462124,
15.283031899268));
#241903=CARTESIAN_POINT('Ctrl Pts',(-6.73789351069379,3.1813912437732,15.5479558423092));
#241904=CARTESIAN_POINT('Ctrl Pts',(-6.88130840713808,-1.47253684735641,
15.7598949967422));
#241905=CARTESIAN_POINT('Ctrl Pts',(-5.34900987301425,-4.59581088177074,
15.918849362567));
#241906=CARTESIAN_POINT('Ctrl Pts',(-2.49890939824775,-6.57846977125929,
16.0778037283918));
#241907=CARTESIAN_POINT('Ctrl Pts',(2.1356643282549,-7.14285855133397,16.2897428828248));
#241908=CARTESIAN_POINT('Ctrl Pts',(6.20868011891633,-4.13055116299326,
16.5016820372578));
#241909=CARTESIAN_POINT('Ctrl Pts',(7.01495057508644,0.459834338936403,
16.7136211916908));
#241910=CARTESIAN_POINT('Ctrl Pts',(5.62639274700488,4.88488841563443,16.9255603461238));
#241911=CARTESIAN_POINT('Ctrl Pts',(0.0735112942413086,8.00153451654928,
17.1904842891651));
#241912=CARTESIAN_POINT('Ctrl Pts',(-6.69670162250066,4.36905886279388,
17.5083930208146));
#241913=CARTESIAN_POINT('Ctrl Pts',(-7.18745818769423,-1.96491832076134,
17.7733169638558));
#241914=CARTESIAN_POINT('Ctrl Pts',(-4.26990858085605,-5.5936259145728,
17.9852561182889));
#241915=CARTESIAN_POINT('Ctrl Pts',(-1.07477207623318,-6.96980984437503,
18.1442104841136));
#241916=CARTESIAN_POINT('Ctrl Pts',(2.37970350210302,-6.62252398667525,
18.3031648499384));
#241917=CARTESIAN_POINT('Ctrl Pts',(6.26747184736106,-4.0373613969903,18.5151040043714));
#241918=CARTESIAN_POINT('Ctrl Pts',(7.40267982884013,0.899718334147306,
18.7270431588044));
#241919=CARTESIAN_POINT('Ctrl Pts',(5.03000323061986,4.91121641654369,18.9389823132374));
#241920=CARTESIAN_POINT('Ctrl Pts',(1.09750105770811,7.36979793515926,19.1509214676704));
#241921=CARTESIAN_POINT('Ctrl Pts',(-5.14763615074514,6.12632031397724,
19.4158454107117));
#241922=CARTESIAN_POINT('Ctrl Pts',(-7.92851849591846,-1.03589691921599,
19.7337541423612));
#241923=CARTESIAN_POINT('Ctrl Pts',(-4.18228023263746,-6.16676505655972,
19.9986780854025));
#241924=CARTESIAN_POINT('Ctrl Pts',(0.393876779249377,-7.02606797887813,
20.2106172398355));
#241925=CARTESIAN_POINT('Ctrl Pts',(3.7160685048052,-5.99368160233694,20.3695716056603));
#241926=CARTESIAN_POINT('Ctrl Pts',(6.11448183316621,-3.48337833487705,
20.528525971485));
#241927=CARTESIAN_POINT('Ctrl Pts',(7.38673979810175,1.00874454769807,20.7404651259181));
#241928=CARTESIAN_POINT('Ctrl Pts',(5.03848790433384,5.49752684095302,20.952404280351));
#241929=CARTESIAN_POINT('Ctrl Pts',(0.627321250835717,7.00196024256239,
21.1643434347841));
#241930=CARTESIAN_POINT('Ctrl Pts',(-3.95891838810468,6.31232091809937,
21.3762825892171));
#241931=CARTESIAN_POINT('Ctrl Pts',(-7.8945072103994,1.30641281180972,21.6412065322584));
#241932=CARTESIAN_POINT('Ctrl Pts',(-5.34939273263063,-5.9429357525924,
21.9591152639079));
#241933=CARTESIAN_POINT('Ctrl Pts',(0.833163582985019,-7.40447821599224,
22.2240392069491));
#241934=CARTESIAN_POINT('Ctrl Pts',(4.86834028654934,-5.08134165505618,
22.4359783613822));
#241935=CARTESIAN_POINT('Ctrl Pts',(6.72073378548061,-2.13661453409292,
22.5949327272069));
#241936=CARTESIAN_POINT('Ctrl Pts',(6.91025718008171,1.33009714575273,22.7538870930317));
#241937=CARTESIAN_POINT('Ctrl Pts',(4.95547789167846,5.5699846743467,22.9658262474647));
#241938=CARTESIAN_POINT('Ctrl Pts',(0.252483078837816,7.4528795793316,23.1777654018977));
#241939=CARTESIAN_POINT('Ctrl Pts',(-4.07689061791219,5.72712336865149,
23.3897045563307));
#241940=CARTESIAN_POINT('Ctrl Pts',(-7.11243366736574,2.22074705990363,
23.6016437107637));
#241941=CARTESIAN_POINT('Ctrl Pts',(-6.84678358765764,-4.14143852226377,
23.866567653805));
#241942=CARTESIAN_POINT('Ctrl Pts',(-0.199013732592527,-7.99342739390318,
24.1844763854546));
#241943=CARTESIAN_POINT('Ctrl Pts',(5.4481367907149,-5.08313532347652,24.4494003284958));
#241944=CARTESIAN_POINT('Ctrl Pts',(7.0027744961245,-0.694204233260489,
24.6613394829288));
#241945=CARTESIAN_POINT('Ctrl Pts',(6.4949934177085,2.74744331816343,24.8202938487536));
#241946=CARTESIAN_POINT('Ctrl Pts',(4.38453006323543,5.50424461998147,24.9792482145783));
#241947=CARTESIAN_POINT('Ctrl Pts',(0.142302896148915,7.45394125903327,
25.1911873690113));
#241948=CARTESIAN_POINT('Ctrl Pts',(-4.65488093005226,5.82591153864809,
25.4031265234444));
#241949=CARTESIAN_POINT('Ctrl Pts',(-6.82149347660548,1.69947225302547,
25.6150656778774));
#241950=CARTESIAN_POINT('Ctrl Pts',(-6.84726779860935,-2.93825694432527,
25.8270048323104));
#241951=CARTESIAN_POINT('Ctrl Pts',(-2.5080668857004,-7.59865508012841,
26.0919287753516));
#241952=CARTESIAN_POINT('Ctrl Pts',(5.04702373367946,-6.20177711620133,
26.4098375070012));
#241953=CARTESIAN_POINT('Ctrl Pts',(7.44439418198704,-0.318519183587702,
26.6747614500424));
#241954=CARTESIAN_POINT('Ctrl Pts',(5.77123662450275,4.0266112284459,26.8867006044755));
#241955=CARTESIAN_POINT('Ctrl Pts',(3.14735236276397,6.31090781006993,27.0456549703002));
#241956=CARTESIAN_POINT('Ctrl Pts',(-0.248676851823201,7.03270734037595,
27.204609336125));
#241957=CARTESIAN_POINT('Ctrl Pts',(-4.73927178521599,5.75506675488882,
27.416548490558));
#241958=CARTESIAN_POINT('Ctrl Pts',(-7.32481757918334,1.39864547359366,
27.628487644991));
#241959=CARTESIAN_POINT('Ctrl Pts',(-6.28725926764394,-3.14505168345447,
27.840426799424));
#241960=CARTESIAN_POINT('Ctrl Pts',(-3.29087610852275,-6.68495060678104,
28.052365953857));
#241961=CARTESIAN_POINT('Ctrl Pts',(3.03618386846919,-7.4034820217757,28.3172898968983));
#241962=CARTESIAN_POINT('Ctrl Pts',(7.86714544468835,-1.42916427309168,
28.6351986285478));
#241963=CARTESIAN_POINT('Ctrl Pts',(5.86240940769175,4.59919722818268,28.9001225715891));
#241964=CARTESIAN_POINT('Ctrl Pts',(1.76568091712064,6.81198510420894,29.1120617260221));
#241965=CARTESIAN_POINT('Ctrl Pts',(-1.71310338992859,6.8409546890776,29.2710160918468));
#241966=CARTESIAN_POINT('Ctrl Pts',(-4.76235409461543,5.18081037961341,
29.4299704576716));
#241967=CARTESIAN_POINT('Ctrl Pts',(-7.34285557553195,1.28994666721163,
29.6419096121046));
#241968=CARTESIAN_POINT('Ctrl Pts',(-6.47398806841075,-3.7008972181341,
29.8538487665376));
#241969=CARTESIAN_POINT('Ctrl Pts',(-2.73097441663356,-6.47786677277848,
30.0657879209707));
#241970=CARTESIAN_POINT('Ctrl Pts',(1.84731678194465,-7.21843825795398,
30.2777270754036));
#241971=CARTESIAN_POINT('Ctrl Pts',(7.12105446691572,-3.64973174481743,
30.542651018445));
#241972=CARTESIAN_POINT('Ctrl Pts',(6.90582425186084,4.03039444344759,30.8605597500945));
#241973=CARTESIAN_POINT('Ctrl Pts',(1.46258344691281,7.30625135537594,31.1254836931357));
#241974=CARTESIAN_POINT('Ctrl Pts',(-3.08857164243337,6.32309223170156,
31.3374228475688));
#241975=CARTESIAN_POINT('Ctrl Pts',(-5.75013434350845,4.08281022265331,
31.4963772133934));
#241976=CARTESIAN_POINT('Ctrl Pts',(-6.98694564257054,0.838691421069132,
31.6553315792183));
#241977=CARTESIAN_POINT('Ctrl Pts',(-6.41700301498727,-3.79520259182766,
31.8672707336512));
#241978=CARTESIAN_POINT('Ctrl Pts',(-2.51135435712696,-7.02155688021231,
32.0792098880843));
#241979=CARTESIAN_POINT('Ctrl Pts',(2.13798780902864,-6.6970133133076,32.2911490425173));
#241980=CARTESIAN_POINT('Ctrl Pts',(6.09757350988195,-4.28229231467612,
32.5030881969503));
#241981=CARTESIAN_POINT('Ctrl Pts',(7.78310022106858,1.85830823027581,32.7680121399916));
#241982=CARTESIAN_POINT('Ctrl Pts',(2.625131338256,7.55269312393059,33.085920871641));
#241983=CARTESIAN_POINT('Ctrl Pts',(-3.64025173563295,6.50146341282771,
33.3508448146825));
#241984=CARTESIAN_POINT('Ctrl Pts',(-6.45826320049278,2.79492515001907,
33.5627839691153));
#241985=CARTESIAN_POINT('Ctrl Pts',(-7.02329053943438,-0.637788586672086,
33.7217383349402));
#241986=CARTESIAN_POINT('Ctrl Pts',(-5.85317344787643,-3.90655517061833,
33.8806927007649));
#241987=CARTESIAN_POINT('Ctrl Pts',(-2.40673684018765,-7.05613975127012,
34.092631855198));
#241988=CARTESIAN_POINT('Ctrl Pts',(2.65839357106603,-6.96721647076019,
34.3045710096309));
#241989=CARTESIAN_POINT('Ctrl Pts',(5.97929916872158,-3.69715575018147,
34.516510164064));
#241990=CARTESIAN_POINT('Ctrl Pts',(7.41695445299038,0.712191560617269,
34.728449318497));
#241991=CARTESIAN_POINT('Ctrl Pts',(4.70410047050428,6.47312886425953,34.9933732615382));
#241992=CARTESIAN_POINT('Ctrl Pts',(-2.91736413645297,7.44469438343174,
35.3112819931877));
#241993=CARTESIAN_POINT('Ctrl Pts',(-6.99335390629178,2.57166489816807,
35.576205936229));
#241994=CARTESIAN_POINT('Ctrl Pts',(-6.72370891457839,-2.07665803469601,
35.7881450906621));
#241995=CARTESIAN_POINT('Ctrl Pts',(-4.9206133586103,-5.05182624975003,
35.9470994564868));
#241996=CARTESIAN_POINT('Ctrl Pts',(-1.90599944753247,-6.77406663814406,
36.1060538223116));
#241997=CARTESIAN_POINT('Ctrl Pts',(2.76035781957077,-6.92545414505831,
36.3179929767445));
#241998=CARTESIAN_POINT('Ctrl Pts',(6.55035102549848,-3.56399539447913,
36.5299321311776));
#241999=CARTESIAN_POINT('Ctrl Pts',(6.94658480072917,1.07978645872825,36.7418712856106));
#242000=CARTESIAN_POINT('Ctrl Pts',(5.17128248312963,5.3643515597344,36.9538104400436));
#242001=CARTESIAN_POINT('Ctrl Pts',(-0.635984634104433,7.97655828506829,
37.2187343830848));
#242002=CARTESIAN_POINT('Ctrl Pts',(-7.05759166159136,3.75830918174626,
37.5366431147344));
#242003=CARTESIAN_POINT('Ctrl Pts',(-6.98501212133915,-2.59423685731685,
37.8015670577756));
#242004=CARTESIAN_POINT('Ctrl Pts',(-3.75731894680806,-5.95006928472314,
38.0135062122087));
#242005=CARTESIAN_POINT('Ctrl Pts',(-0.452781167209595,-7.03763976750855,
38.1724605780334));
#242006=CARTESIAN_POINT('Ctrl Pts',(2.95731728034348,-6.38553734742756,
38.3314149438582));
#242007=CARTESIAN_POINT('Ctrl Pts',(6.60065160063017,-3.46596146176918,
38.5433540982912));
#242008=CARTESIAN_POINT('Ctrl Pts',(7.29379945881797,1.55230511938344,38.7552932527242));
#242009=CARTESIAN_POINT('Ctrl Pts',(4.57490663890595,5.3377156570455,38.9672324071572));
#242010=CARTESIAN_POINT('Ctrl Pts',(0.439968219370932,7.43806817276445,
39.1791715615902));
#242011=CARTESIAN_POINT('Ctrl Pts',(-5.67037568507045,5.6459541372624,39.4440955046315));
#242012=CARTESIAN_POINT('Ctrl Pts',(-7.80549854202645,-1.73455483562362,
39.762004236281));
#242013=CARTESIAN_POINT('Ctrl Pts',(-3.61923596515816,-6.51318587448737,
40.0269281793224));
#242014=CARTESIAN_POINT('Ctrl Pts',(1.01507386770645,-6.9635045202935,40.2388673337553));
#242015=CARTESIAN_POINT('Ctrl Pts',(4.23268601565952,-5.64072277065963,
40.3978216995801));
#242016=CARTESIAN_POINT('Ctrl Pts',(6.39916207500406,-2.92771881331523,
40.5567760654049));
#242017=CARTESIAN_POINT('Ctrl Pts',(7.26825875330756,1.65948941013164,40.7687152198378));
#242018=CARTESIAN_POINT('Ctrl Pts',(4.53139098387666,5.92247055546574,40.9806543742709));
#242019=CARTESIAN_POINT('Ctrl Pts',(0.00424177129030791,7.03000435259828,
41.1925935287039));
#242020=CARTESIAN_POINT('Ctrl Pts',(-4.50282233051353,5.93658329652475,
41.4045326831369));
#242021=CARTESIAN_POINT('Ctrl Pts',(-7.97922898576225,0.601550764840454,
41.6694566261781));
#242022=CARTESIAN_POINT('Ctrl Pts',(-4.80159388164659,-6.39368314534717,
41.9873653578277));
#242023=CARTESIAN_POINT('Ctrl Pts',(1.48617170717807,-7.30148977017016,
42.2522893008689));
#242024=CARTESIAN_POINT('Ctrl Pts',(5.29955859651241,-4.62984328494818,
42.464228455302));
#242025=CARTESIAN_POINT('Ctrl Pts',(6.88365916119135,-1.53252107168022,
42.6231828211267));
#242026=CARTESIAN_POINT('Ctrl Pts',(6.76516872873376,1.93734477669137,42.7821371869515));
#242027=CARTESIAN_POINT('Ctrl Pts',(4.44228546067889,5.98728572002473,42.9940763413845));
#242028=CARTESIAN_POINT('Ctrl Pts',(-0.409087847200969,7.44592565517477,
43.2060154958175));
#242029=CARTESIAN_POINT('Ctrl Pts',(-4.56846195731471,5.34323259223688,
43.4179546502505));
#242030=CARTESIAN_POINT('Ctrl Pts',(-7.28127440862704,1.5816046165276,43.6298938046836));
#242031=CARTESIAN_POINT('Ctrl Pts',(-6.45276501179143,-4.73199558669585,
43.8948177477248));
#242032=CARTESIAN_POINT('Ctrl Pts',(0.510257573223466,-7.97960683093662,
44.2127264793743));
#242033=CARTESIAN_POINT('Ctrl Pts',(5.87723216227991,-4.5802403122302,44.4776504224156));
#242034=CARTESIAN_POINT('Ctrl Pts',(7.03674349602929,-0.0707893504553004,
44.6895895768486));
#242035=CARTESIAN_POINT('Ctrl Pts',(6.22591451695742,3.31230625246769,44.8485439426733));
#242036=CARTESIAN_POINT('Ctrl Pts',(3.87941151685467,5.87119911048039,45.0074983084981));
#242037=CARTESIAN_POINT('Ctrl Pts',(-0.518928492009235,7.43721746539336,
45.2194374629312));
#242038=CARTESIAN_POINT('Ctrl Pts',(-5.15293343338446,5.39040246736978,
45.4313766173641));
#242039=CARTESIAN_POINT('Ctrl Pts',(-6.94527669779923,1.08816854447353,
45.6433157717972));
#242040=CARTESIAN_POINT('Ctrl Pts',(-6.55988990217875,-3.53359231491712,
45.8552549262302));
#242041=CARTESIAN_POINT('Ctrl Pts',(-1.82469796774667,-7.79104844397787,
46.1201788692715));
#242042=CARTESIAN_POINT('Ctrl Pts',(5.57684727553539,-5.73003162580412,
46.4380876009209));
#242043=CARTESIAN_POINT('Ctrl Pts',(7.44332668653606,0.34255954900659,46.7030115439622));
#242044=CARTESIAN_POINT('Ctrl Pts',(5.39162868515475,4.52229038015749,46.9149506983953));
#242045=CARTESIAN_POINT('Ctrl Pts',(2.57560536052975,6.56503170665673,47.07390506422));
#242046=CARTESIAN_POINT('Ctrl Pts',(-0.871033878891199,6.98298737603286,
47.2328594300447));
#242047=CARTESIAN_POINT('Ctrl Pts',(-5.2307129054187,5.31235662474358,47.4447985844778));
#242048=CARTESIAN_POINT('Ctrl Pts',(-7.41995642837388,0.743914195422315,
47.6567377389107));
#242049=CARTESIAN_POINT('Ctrl Pts',(-5.98375640066137,-3.68993746935074,
47.8686768933438));
#242050=CARTESIAN_POINT('Ctrl Pts',(-2.68541139296351,-6.95032343328639,
48.0806160477768));
#242051=CARTESIAN_POINT('Ctrl Pts',(3.6804332198673,-7.10523538273054,48.3455399908181));
#242052=CARTESIAN_POINT('Ctrl Pts',(7.96285483987609,-0.726244288393699,
48.6634487224676));
#242053=CARTESIAN_POINT('Ctrl Pts',(5.43169215040701,5.10070383283746,48.9283726655089));
#242054=CARTESIAN_POINT('Ctrl Pts',(1.15495939305906,6.94167407484916,49.140311819942));
#242055=CARTESIAN_POINT('Ctrl Pts',(-2.3127010697674,6.66219168476068,49.2992661857666));
#242056=CARTESIAN_POINT('Ctrl Pts',(-5.20280583031192,4.73831448978248,
49.4582205515914));
#242057=CARTESIAN_POINT('Ctrl Pts',(-7.42828904121764,0.634044420759983,
49.6701597060245));
#242058=CARTESIAN_POINT('Ctrl Pts',(-6.12048357297907,-4.26014583811528,
49.8820988604574));
#242059=CARTESIAN_POINT('Ctrl Pts',(-2.14606795096395,-6.69442839531649,
50.0940380148904));
#242060=CARTESIAN_POINT('Ctrl Pts',(2.47984404763027,-7.02629373682747,
50.3059771693235));
#242061=CARTESIAN_POINT('Ctrl Pts',(7.41651765727688,-3.00420111996666,
50.5709011123647));
#242062=CARTESIAN_POINT('Ctrl Pts',(6.52141556975414,4.62662154643429,50.8888098440143));
#242063=CARTESIAN_POINT('Ctrl Pts',(0.809246122055264,7.40713034319324,
51.1537337870554));
#242064=CARTESIAN_POINT('Ctrl Pts',(-3.63685573074989,6.02445437817901,
51.3656729414886));
#242065=CARTESIAN_POINT('Ctrl Pts',(-6.0893784968316,3.55708501513851,51.5246273073133));
#242066=CARTESIAN_POINT('Ctrl Pts',(-7.03378339253583,0.216110848634113,
51.6835816731381));
#242067=CARTESIAN_POINT('Ctrl Pts',(-6.05536415093935,-4.34902924879671,
51.895520827571));
#242068=CARTESIAN_POINT('Ctrl Pts',(-1.8791229213296,-7.2165129235422,52.1074599820041));
#242069=CARTESIAN_POINT('Ctrl Pts',(2.72315518706222,-6.48115769113438,
52.3193991364371));
#242070=CARTESIAN_POINT('Ctrl Pts',(6.45313109988518,-3.72498713882919,
52.5313382908701));
#242071=CARTESIAN_POINT('Ctrl Pts',(7.58775913309835,2.54084038616979,52.7962622339114));
#242072=CARTESIAN_POINT('Ctrl Pts',(1.94537547108583,7.75564325145627,53.1141709655609));
#242073=CARTESIAN_POINT('Ctrl Pts',(-4.20217428426094,6.1532260231371,53.3790949086021));
#242074=CARTESIAN_POINT('Ctrl Pts',(-6.68057017534676,2.21150453160647,
53.5910340630352));
#242075=CARTESIAN_POINT('Ctrl Pts',(-6.9391191756799,-1.25777953088348,
53.7499884288599));
#242076=CARTESIAN_POINT('Ctrl Pts',(-5.48388405553002,-4.40996920369223,
53.9089427946847));
#242077=CARTESIAN_POINT('Ctrl Pts',(-1.77185193776174,-7.24168703535447,
54.1208819491178));
#242078=CARTESIAN_POINT('Ctrl Pts',(3.26546191579567,-6.70417185084077,
54.3328211035507));
#242079=CARTESIAN_POINT('Ctrl Pts',(6.28345936197013,-3.15263661665029,
54.5447602579837));
#242080=CARTESIAN_POINT('Ctrl Pts',(7.32463911719643,1.36678161371311,54.7566994124168));
#242081=CARTESIAN_POINT('Ctrl Pts',(4.11184826737424,6.86459484281479,55.0216233554581));
#242082=CARTESIAN_POINT('Ctrl Pts',(-3.56573393857394,7.15681699127929,
55.3395320871076));
#242083=CARTESIAN_POINT('Ctrl Pts',(-7.19376650262481,1.94169583427197,
55.6044560301488));
#242084=CARTESIAN_POINT('Ctrl Pts',(-6.51318411840115,-2.66443292294169,
55.8163951845819));
#242085=CARTESIAN_POINT('Ctrl Pts',(-4.4534845077477,-5.4680764462331,55.9753495504066));
#242086=CARTESIAN_POINT('Ctrl Pts',(-1.29808652736431,-6.91634181337834,
56.1343039162313));
#242087=CARTESIAN_POINT('Ctrl Pts',(3.36332330666462,-6.65353640872412,
56.3462430706644));
#242088=CARTESIAN_POINT('Ctrl Pts',(6.84046120552639,-2.96938583293011,
56.5581822250974));
#242089=CARTESIAN_POINT('Ctrl Pts',(6.82353936752462,1.6912390990088,56.7701213795304));
#242090=CARTESIAN_POINT('Ctrl Pts',(4.67546675461387,5.80158950661353,56.9820605339634));
#242091=CARTESIAN_POINT('Ctrl Pts',(-1.34047444450577,7.88879501530715,
57.2469844770046));
#242092=CARTESIAN_POINT('Ctrl Pts',(-7.36292825745679,3.11797617741172,
57.5648932086542));
#242093=CARTESIAN_POINT('Ctrl Pts',(-6.72758391760391,-3.20313500163717,
57.8298171516955));
#242094=CARTESIAN_POINT('Ctrl Pts',(-3.21515378405285,-6.25967701290882,
58.0417563061285));
#242095=CARTESIAN_POINT('Ctrl Pts',(0.172773783780828,-7.05007329764989,
58.2007106719533));
#242096=CARTESIAN_POINT('Ctrl Pts',(3.51165269883899,-6.09828730339489,
58.359665037778));
#242097=CARTESIAN_POINT('Ctrl Pts',(6.88187468914349,-2.86727940220291,
58.5716041922111));
#242098=CARTESIAN_POINT('Ctrl Pts',(7.12750634893194,2.19267302055105,58.783543346644));
#242099=CARTESIAN_POINT('Ctrl Pts',(4.08379892209254,5.7221993633646,58.995482501077));
#242100=CARTESIAN_POINT('Ctrl Pts',(-0.221027804521507,7.44779006728682,
59.2074216555101));
#242101=CARTESIAN_POINT('Ctrl Pts',(-6.14848117016335,5.1211461441805,59.4723455985513));
#242102=CARTESIAN_POINT('Ctrl Pts',(-7.62103803718001,-2.41955929938033,
59.7902543302009));
#242103=CARTESIAN_POINT('Ctrl Pts',(-3.02770308154028,-6.80833850929487,
60.0551782732421));
#242104=CARTESIAN_POINT('Ctrl Pts',(1.62828085824023,-6.84612822022322,
60.2671174276751));
#242105=CARTESIAN_POINT('Ctrl Pts',(4.71598617216184,-5.24336330102886,
60.4260717934999));
#242106=CARTESIAN_POINT('Ctrl Pts',(6.63347166576597,-2.34901391470771,
60.5850261593247));
#242107=CARTESIAN_POINT('Ctrl Pts',(7.0925660109032,2.29717169326795,60.7969653137576));
#242108=CARTESIAN_POINT('Ctrl Pts',(3.98862546939676,6.30079586988792,61.0089044681907));
#242109=CARTESIAN_POINT('Ctrl Pts',(-0.618871097123766,7.00271217138896,
61.2208436226237));
#242110=CARTESIAN_POINT('Ctrl Pts',(-5.01128255547801,5.51411618719717,
61.4327827770568));
#242111=CARTESIAN_POINT('Ctrl Pts',(-8.00114270057177,-0.108046355772149,
61.6977067200978));
#242112=CARTESIAN_POINT('Ctrl Pts',(-4.21599954944376,-6.79410301411839,
62.0156154517476));
#242113=CARTESIAN_POINT('Ctrl Pts',(2.12748151280638,-7.14102805062289,
62.2805393947886));
#242114=CARTESIAN_POINT('Ctrl Pts',(5.68906172348862,-4.14190135896367,
62.4924785492218));
#242115=CARTESIAN_POINT('Ctrl Pts',(6.99240019375371,-0.916364454238048,
62.6514329150465));
#242116=CARTESIAN_POINT('Ctrl Pts',(6.56682862513636,2.52934270515092,62.8103872808712));
#242117=CARTESIAN_POINT('Ctrl Pts',(3.89412582486431,6.35745817662179,63.0223264353044));
#242118=CARTESIAN_POINT('Ctrl Pts',(-1.06743866082989,7.38036153819596,
63.2342655897372));
#242119=CARTESIAN_POINT('Ctrl Pts',(-5.02407290057349,4.91728285538854,
63.4462047441704));
#242120=CARTESIAN_POINT('Ctrl Pts',(-7.39280100026574,0.93001265970799,
63.6581438986033));
#242121=CARTESIAN_POINT('Ctrl Pts',(-6.00795385229093,-5.28530500904657,
63.9230678416446));
#242122=CARTESIAN_POINT('Ctrl Pts',(1.21551241471566,-7.90297523322938,
64.2409765732942));
#242123=CARTESIAN_POINT('Ctrl Pts',(6.26006522526891,-4.04129219216908,
64.5059005163353));
#242124=CARTESIAN_POINT('Ctrl Pts',(7.01532315789409,0.553182746814791,
64.7178396707685));
#242125=CARTESIAN_POINT('Ctrl Pts',(5.90782867371946,3.85109655092691,64.8767940365932));
#242126=CARTESIAN_POINT('Ctrl Pts',(3.34375639684328,6.19193878123707,65.0357484024179));
#242127=CARTESIAN_POINT('Ctrl Pts',(-1.17607516319154,7.36195202496903,
65.247687556851));
#242128=CARTESIAN_POINT('Ctrl Pts',(-5.61042490559491,4.91246314058462,
65.4596267112839));
#242129=CARTESIAN_POINT('Ctrl Pts',(-7.01439055682164,0.468299377290018,
65.671565865717));
#242130=CARTESIAN_POINT('Ctrl Pts',(-6.22087619441535,-4.10111320864855,
65.88350502015));
#242131=CARTESIAN_POINT('Ctrl Pts',(-1.12696604053075,-7.92211499999566,
66.1484289631913));
#242132=CARTESIAN_POINT('Ctrl Pts',(6.06277297200943,-5.2131825077762,66.4663376948408));
#242133=CARTESIAN_POINT('Ctrl Pts',(7.38366945566897,1.00094184309718,66.7312616378821));
#242134=CARTESIAN_POINT('Ctrl Pts',(4.96958083852046,4.98237257263741,66.943200792315));
#242135=CARTESIAN_POINT('Ctrl Pts',(1.98358462215674,6.76747931875516,67.1021551581399));
#242136=CARTESIAN_POINT('Ctrl Pts',(-1.48653460954908,6.87830121153664,
67.2611095239646));
#242137=CARTESIAN_POINT('Ctrl Pts',(-5.68098076067773,4.82783057365139,
67.4730486783976));
#242138=CARTESIAN_POINT('Ctrl Pts',(-7.45668949435264,0.0833272357797441,
67.6849878328307));
#242139=CARTESIAN_POINT('Ctrl Pts',(-5.63315273213393,-4.20577811385,67.8969269872636));
#242140=CARTESIAN_POINT('Ctrl Pts',(-2.05880859419072,-7.16098717781453,
68.1088661416967));
#242141=CARTESIAN_POINT('Ctrl Pts',(4.29571221098905,-6.75106026423516,
68.3737900847379));
#242142=CARTESIAN_POINT('Ctrl Pts',(7.99588512145278,-0.0176077317945067,
68.6916988163875));
#242143=CARTESIAN_POINT('Ctrl Pts',(4.9582195286531,5.56206056255386,68.9566227594286));
#242144=CARTESIAN_POINT('Ctrl Pts',(0.535146807666416,7.01672199441423,
69.1685619138617));
#242145=CARTESIAN_POINT('Ctrl Pts',(-2.89409475134154,6.43098770826065,
69.3275162796864));
#242146=CARTESIAN_POINT('Ctrl Pts',(-5.60230340683511,4.25852102893992,
69.4864706455113));
#242147=CARTESIAN_POINT('Ctrl Pts',(-7.45525241801838,-0.0268482377574512,
69.6984097999442));
#242148=CARTESIAN_POINT('Ctrl Pts',(-5.71879957776433,-4.78586178669096,
69.9103489543773));
#242149=CARTESIAN_POINT('Ctrl Pts',(-1.54427169558857,-6.85829422219245,
70.1222881088102));
#242150=CARTESIAN_POINT('Ctrl Pts',(3.09285805960138,-6.7788444056032,70.3342272632433));
#242151=CARTESIAN_POINT('Ctrl Pts',(7.65358787062285,-2.33501825228283,
70.5991512062845));
#242152=CARTESIAN_POINT('Ctrl Pts',(6.08569908081881,5.18642192048741,70.9170599379341));
#242153=CARTESIAN_POINT('Ctrl Pts',(0.149496258939197,7.44971896383081,
71.1819838809753));
#242154=CARTESIAN_POINT('Ctrl Pts',(-4.1564535195748,5.67837535520366,71.3939230354084));
#242155=CARTESIAN_POINT('Ctrl Pts',(-6.38081912316377,3.00340405698944,
71.5528774012331));
#242156=CARTESIAN_POINT('Ctrl Pts',(-7.02501524399713,-0.408252188217427,
71.7118317670579));
#242157=CARTESIAN_POINT('Ctrl Pts',(-5.64660810487616,-4.86843712768816,
71.9237709214909));
#242158=CARTESIAN_POINT('Ctrl Pts',(-1.23105069577916,-7.35502050892989,
72.1357100759239));
#242159=CARTESIAN_POINT('Ctrl Pts',(3.28566072525786,-6.21387000785308,
72.3476492303569));
#242160=CARTESIAN_POINT('Ctrl Pts',(6.76075871342928,-3.13933136936446,
72.5595883847899));
#242161=CARTESIAN_POINT('Ctrl Pts',(7.32662904256254,3.20541028052231,72.8245123278312));
#242162=CARTESIAN_POINT('Ctrl Pts',(1.26079203493607,7.89410385780598,73.1424210594807));
#242163=CARTESIAN_POINT('Ctrl Pts',(-5.94922018012124,5.33486142538932,
73.4603297911302));
#242164=CARTESIAN_POINT('Ctrl Pts',(-7.7092089677762,-2.11567753454102,
73.7782385227798));
#242165=CARTESIAN_POINT('Ctrl Pts',(-2.39279777489314,-7.62420395766902,
74.0961472544292));
#242166=CARTESIAN_POINT('Ctrl Pts',(5.11354927904136,-6.14476086141691,
74.4140559860789));
#242167=CARTESIAN_POINT('Ctrl Pts',(7.9364501518555,0.983314385591691,74.7319647177282));
#242168=CARTESIAN_POINT('Ctrl Pts',(4.2113156217051,6.1504536875151,74.9968886607696));
#242169=CARTESIAN_POINT('Ctrl Pts',(-0.346322503067723,7.02052758700276,
75.2088278152026));
#242170=CARTESIAN_POINT('Ctrl Pts',(-4.8128110953465,5.69637269346616,75.4207669696356));
#242171=CARTESIAN_POINT('Ctrl Pts',(-7.34061996470585,1.3042858927657,75.6327061240687));
#242172=CARTESIAN_POINT('Ctrl Pts',(-6.2493396542438,-3.23469672666109,
75.8446452785016));
#242173=CARTESIAN_POINT('Ctrl Pts',(-3.95397872191655,-5.839635337819,76.0035996443264));
#242174=CARTESIAN_POINT('Ctrl Pts',(-0.675821523237244,-7.00452124014909,
76.1625540101512));
#242175=CARTESIAN_POINT('Ctrl Pts',(3.93109667452361,-6.32986103378635,
76.3744931645842));
#242176=CARTESIAN_POINT('Ctrl Pts',(7.88051160939144,-1.35360349210481,
76.6394171076255));
#242177=CARTESIAN_POINT('Ctrl Pts',(5.38962152202552,5.91453272720326,76.9573258392749));
#242178=CARTESIAN_POINT('Ctrl Pts',(-0.800496012063925,7.4079490135184,
77.2222497823163));
#242179=CARTESIAN_POINT('Ctrl Pts',(-4.82861356016322,5.1093508192883,77.4341889367493));
#242180=CARTESIAN_POINT('Ctrl Pts',(-7.36055018309903,1.19642912620305,
77.6461280911822));
#242181=CARTESIAN_POINT('Ctrl Pts',(-6.42463045389124,-3.78227880717078,
77.8580672456154));
#242182=CARTESIAN_POINT('Ctrl Pts',(-2.64387061986552,-6.52156062316159,
78.0700064000482));
#242183=CARTESIAN_POINT('Ctrl Pts',(0.793861069575679,-7.00736554888885,
78.2289607658731));
#242184=CARTESIAN_POINT('Ctrl Pts',(4.04171201133761,-5.76067128640936,
78.3879151316978));
#242185=CARTESIAN_POINT('Ctrl Pts',(7.10270483729022,-2.25211957723571,
78.5998542861308));
#242186=CARTESIAN_POINT('Ctrl Pts',(6.86684019138204,4.09646124035234,78.864778229172));
#242187=CARTESIAN_POINT('Ctrl Pts',(0.248045042783987,7.9980267408734,79.1826869608217));
#242188=CARTESIAN_POINT('Ctrl Pts',(-5.42557734563471,5.10700897344742,
79.4476109038628));
#242189=CARTESIAN_POINT('Ctrl Pts',(-6.99080999885538,0.741319638476606,
79.659550058296));
#242190=CARTESIAN_POINT('Ctrl Pts',(-6.3696296295627,-3.87775450816691,
79.8714892127287));
#242191=CARTESIAN_POINT('Ctrl Pts',(-2.4209356389253,-7.05128081154447,
80.083428367162));
#242192=CARTESIAN_POINT('Ctrl Pts',(2.23257239746651,-6.67356225655268,
80.2953675215949));
#242193=CARTESIAN_POINT('Ctrl Pts',(5.16003344080966,-4.80701978077493,
80.4543218874197));
#242194=CARTESIAN_POINT('Ctrl Pts',(6.8165859479432,-1.74783471113904,80.6132762532443));
#242195=CARTESIAN_POINT('Ctrl Pts',(6.86027898238168,2.90809757190748,80.8252154076776));
#242196=CARTESIAN_POINT('Ctrl Pts',(2.55255244952595,7.57753020198079,81.0901393507185));
#242197=CARTESIAN_POINT('Ctrl Pts',(-5.01276718579973,6.23715669761748,
81.4080480823685));
#242198=CARTESIAN_POINT('Ctrl Pts',(-7.44278175877897,0.351325870925839,
81.6729720254094));
#242199=CARTESIAN_POINT('Ctrl Pts',(-5.79278720436264,-3.98303848780944,
81.8849111798426));
#242200=CARTESIAN_POINT('Ctrl Pts',(-2.31706440085395,-7.08804446171282,
82.0968503342754));
#242201=CARTESIAN_POINT('Ctrl Pts',(2.74641161828516,-6.9309965827701,82.3087894887087));
#242202=CARTESIAN_POINT('Ctrl Pts',(6.03590165419069,-3.61783138536833,
82.5207286431415));
#242203=CARTESIAN_POINT('Ctrl Pts',(7.0459703068444,-0.296119431394292,
82.6796830089663));
#242204=CARTESIAN_POINT('Ctrl Pts',(6.31498177687263,3.10512082193679,82.8386373747911));
#242205=CARTESIAN_POINT('Ctrl Pts',(3.32037324809578,6.67050078333239,83.050576529224));
#242206=CARTESIAN_POINT('Ctrl Pts',(-2.98865185291137,7.41636353406801,
83.3155004722653));
#242207=CARTESIAN_POINT('Ctrl Pts',(-7.86412952468985,1.47831841928965,
83.633409203915));
#242208=CARTESIAN_POINT('Ctrl Pts',(-5.88251902724038,-4.57322643993298,
83.8983331469561));
#242209=CARTESIAN_POINT('Ctrl Pts',(-1.81038802006712,-6.79289882207679,
84.1102723013891));
#242210=CARTESIAN_POINT('Ctrl Pts',(2.84922712524779,-6.89137624265787,
84.3222114558222));
#242211=CARTESIAN_POINT('Ctrl Pts',(6.59366141269033,-3.47924123655858,
84.5341506102552));
#242212=CARTESIAN_POINT('Ctrl Pts',(6.93799848399193,1.17685587398636,84.7460897646883));
#242213=CARTESIAN_POINT('Ctrl Pts',(5.54517247875604,4.35711446526757,84.905044130513));
#242214=CARTESIAN_POINT('Ctrl Pts',(2.77800178948208,6.46556078145453,85.0639984963377));
#242215=CARTESIAN_POINT('Ctrl Pts',(-1.8155118597288,7.22664347358443,85.2759376507708));
#242216=CARTESIAN_POINT('Ctrl Pts',(-7.09332286364526,3.69042798594542,
85.540861593812));
#242217=CARTESIAN_POINT('Ctrl Pts',(-6.93549859986734,-3.99109229424056,
85.8587703254616));
#242218=CARTESIAN_POINT('Ctrl Pts',(-1.49474916635836,-7.29959965384536,
86.1236942685027));
#242219=CARTESIAN_POINT('Ctrl Pts',(3.04219705054772,-6.33766647085607,
86.3356334229359));
#242220=CARTESIAN_POINT('Ctrl Pts',(6.64600161752001,-3.38228092107058,
86.5475725773687));
#242221=CARTESIAN_POINT('Ctrl Pts',(7.2715845009025,1.6448553898765,86.7595117318021));
#242222=CARTESIAN_POINT('Ctrl Pts',(4.50525864164091,5.40587248128648,86.9714508862347));
#242223=CARTESIAN_POINT('Ctrl Pts',(1.37901740415747,6.91604621743004,87.1304052520598));
#242224=CARTESIAN_POINT('Ctrl Pts',(-2.09425987377605,6.71824722246359,
87.2893596178843));
#242225=CARTESIAN_POINT('Ctrl Pts',(-6.07874824292151,4.3092086287733,87.5012987723175));
#242226=CARTESIAN_POINT('Ctrl Pts',(-7.78849857574283,-1.80935842303686,
87.7662227153585));
#242227=CARTESIAN_POINT('Ctrl Pts',(-2.67323260379538,-7.54213404653577,
88.0841314470083));
#242228=CARTESIAN_POINT('Ctrl Pts',(3.61149077593769,-6.51732802243875,
88.3490553900493));
#242229=CARTESIAN_POINT('Ctrl Pts',(6.43251165346284,-2.83615461818277,
88.5609945444826));
#242230=CARTESIAN_POINT('Ctrl Pts',(7.2482914225384,1.75255047946504,88.7729336989153));
#242231=CARTESIAN_POINT('Ctrl Pts',(4.45432858118756,5.97833148112297,88.9848728533486));
#242232=CARTESIAN_POINT('Ctrl Pts',(-0.0929907162208757,7.0364881467041,
89.1968120077815));
#242233=CARTESIAN_POINT('Ctrl Pts',(-3.44997981742828,6.15069293185211,
89.3557663736062));
#242234=CARTESIAN_POINT('Ctrl Pts',(-5.95988905589371,3.74172321297108,
89.5147207394312));
#242235=CARTESIAN_POINT('Ctrl Pts',(-7.42015744381375,-0.679501814664077,
89.7266598938637));
#242236=CARTESIAN_POINT('Ctrl Pts',(-4.74003399571024,-6.43945383451685,
89.9915838369055));
#242237=CARTESIAN_POINT('Ctrl Pts',(2.87395643469399,-7.46795373187258,
90.3094925685547));
#242238=CARTESIAN_POINT('Ctrl Pts',(6.98182202518171,-2.60242029377199,
90.5744165115962));
#242239=CARTESIAN_POINT('Ctrl Pts',(6.73095821900039,2.0285908025635,90.7863556660291));
#242240=CARTESIAN_POINT('Ctrl Pts',(4.36659833218498,6.04499633866525,90.9982948204622));
#242241=CARTESIAN_POINT('Ctrl Pts',(-0.50395667669231,7.43824697596069,
91.2102339748951));
#242242=CARTESIAN_POINT('Ctrl Pts',(-4.64654291086805,5.28492683861115,
91.4221731293282));
#242243=CARTESIAN_POINT('Ctrl Pts',(-6.62070062977333,2.42893133981105,
91.5811274951529));
#242244=CARTESIAN_POINT('Ctrl Pts',(-6.96082222641317,-1.0333073566566,
91.7400818609777));
#242245=CARTESIAN_POINT('Ctrl Pts',(-5.19497417370953,-5.3416011215372,
91.9520210154106));
#242246=CARTESIAN_POINT('Ctrl Pts',(0.586787841480146,-7.97434436154179,
92.216944958452));
#242247=CARTESIAN_POINT('Ctrl Pts',(7.03974198416446,-3.80420705618134,
92.5348536901015));
#242248=CARTESIAN_POINT('Ctrl Pts',(6.99625226324018,2.56337364538507,92.7997776331427));
#242249=CARTESIAN_POINT('Ctrl Pts',(3.79408463287575,5.91826841134726,93.0117167875758));
#242250=CARTESIAN_POINT('Ctrl Pts',(-0.613955443182657,7.43183829499158,
93.2236559420087));
#242251=CARTESIAN_POINT('Ctrl Pts',(-5.22000878757889,5.3228750375121,93.4355950964418));
#242252=CARTESIAN_POINT('Ctrl Pts',(-6.96667552007488,0.993098640619434,
93.6475342508748));
#242253=CARTESIAN_POINT('Ctrl Pts',(-6.60909799444585,-2.46032680398553,
93.8064886166995));
#242254=CARTESIAN_POINT('Ctrl Pts',(-4.61594820447646,-5.31166568362871,
93.9654429825243));
#242255=CARTESIAN_POINT('Ctrl Pts',(-0.472760899151676,-7.4361923280231,
94.1773821369574));
#242256=CARTESIAN_POINT('Ctrl Pts',(5.63156268528228,-5.67626547028052,
94.4423060799985));
#242257=CARTESIAN_POINT('Ctrl Pts',(7.82178656201855,1.68807982872061,94.7602148116482));
#242258=CARTESIAN_POINT('Ctrl Pts',(3.64784541378302,6.4970496391739,95.0251387546894));
#242259=CARTESIAN_POINT('Ctrl Pts',(-0.966463691743675,6.96325549744629,
95.2370779091224));
#242260=CARTESIAN_POINT('Ctrl Pts',(-5.29940377398743,5.24647323154949,
95.4490170635554));
#242261=CARTESIAN_POINT('Ctrl Pts',(-7.42699769040191,0.648995927672792,
95.6609562179884));
#242262=CARTESIAN_POINT('Ctrl Pts',(-5.93818747723761,-3.77607497240045,
95.8728953724214));
#242263=CARTESIAN_POINT('Ctrl Pts',(-3.42074886478076,-6.16699776931195,
96.0318497382463));
#242264=CARTESIAN_POINT('Ctrl Pts',(-0.0523603294637201,-7.03690475684776,
96.1908041040708));
#242265=CARTESIAN_POINT('Ctrl Pts',(4.47669087758938,-5.95648369372606,
96.4027432585041));
#242266=CARTESIAN_POINT('Ctrl Pts',(7.96945573777992,-0.649817829033016,
96.6676672015452));
#242267=CARTESIAN_POINT('Ctrl Pts',(4.84419055635731,6.3689698055185,96.9855759331948));
#242268=CARTESIAN_POINT('Ctrl Pts',(-1.45394444495315,7.30783659695112,
97.2504998762359));
#242269=CARTESIAN_POINT('Ctrl Pts',(-5.26246902619562,4.66126580860892,
97.4624390306691));
#242270=CARTESIAN_POINT('Ctrl Pts',(-7.43762669290687,0.53932449052114,
97.6743781851019));
#242271=CARTESIAN_POINT('Ctrl Pts',(-6.06410627124071,-4.33683127853385,
97.8863173395352));
#242272=CARTESIAN_POINT('Ctrl Pts',(-2.05543456090541,-6.73023041788661,
98.098256493968));
#242273=CARTESIAN_POINT('Ctrl Pts',(1.41182644723664,-6.90942330194649,
98.2572108597928));
#242274=CARTESIAN_POINT('Ctrl Pts',(4.53639519977446,-5.37976660762449,
98.4161652256177));
#242275=CARTESIAN_POINT('Ctrl Pts',(7.27436459572607,-1.61371587820268,
98.6281043800504));
#242276=CARTESIAN_POINT('Ctrl Pts',(6.47672915079787,4.68897296586018,98.8930283230921));
#242277=CARTESIAN_POINT('Ctrl Pts',(-0.461826873943633,7.98853393736367,
99.2109370547412));
#242278=CARTESIAN_POINT('Ctrl Pts',(-5.85687752741677,4.60601951858521,
99.4758609977827));
#242279=CARTESIAN_POINT('Ctrl Pts',(-7.02900210216742,0.118779787425345,
99.6878001522157));
#242280=CARTESIAN_POINT('Ctrl Pts',(-6.00086032543074,-4.42705738428912,
99.8997393066486));
#242281=CARTESIAN_POINT('Ctrl Pts',(-1.78642551855117,-7.23810571033889,
100.111678461082));
#242282=CARTESIAN_POINT('Ctrl Pts',(2.81528895915896,-6.44941553851574,
100.323617615515));
#242283=CARTESIAN_POINT('Ctrl Pts',(5.56578953098327,-4.33074718488558,
100.48257198134));
#242284=CARTESIAN_POINT('Ctrl Pts',(6.94467503324845,-1.13677563468953,
100.641526347164));
#242285=CARTESIAN_POINT('Ctrl Pts',(6.57552301821642,3.50470487259935,100.853465501597));
#242286=CARTESIAN_POINT('Ctrl Pts',(1.87088082740638,7.77394963303761,101.118389444639));
#242287=CARTESIAN_POINT('Ctrl Pts',(-5.54586137949077,5.76830825193848,
101.436298176288));
#242288=CARTESIAN_POINT('Ctrl Pts',(-7.44462839157768,-0.309739064478167,
101.701222119329));
#242289=CARTESIAN_POINT('Ctrl Pts',(-5.41695646656369,-4.48079924003838,
101.913161273763));
#242290=CARTESIAN_POINT('Ctrl Pts',(-1.67970458774967,-7.26551816644961,
102.125100428195));
#242291=CARTESIAN_POINT('Ctrl Pts',(3.34992324121293,-6.66029313809475,
102.337039582629));
#242292=CARTESIAN_POINT('Ctrl Pts',(6.33280825391566,-3.06860755574061,
102.548978737061));
#242293=CARTESIAN_POINT('Ctrl Pts',(7.04448552145472,0.329557310058005,
102.707933102886));
#242294=CARTESIAN_POINT('Ctrl Pts',(6.01490902677195,3.65262091664403,102.866887468711));
#242295=CARTESIAN_POINT('Ctrl Pts',(2.71607318310361,6.93854492463233,103.078826623144));
#242296=CARTESIAN_POINT('Ctrl Pts',(-3.63423001483137,7.12227914130449,
103.343750566185));
#242297=CARTESIAN_POINT('Ctrl Pts',(-7.96420750968263,0.775472290042344,
103.661659297835));
#242298=CARTESIAN_POINT('Ctrl Pts',(-5.45402451437071,-5.07661765089621,
103.926583240876));
#242299=CARTESIAN_POINT('Ctrl Pts',(-1.20118223144524,-6.92662547255407,
104.138522395309));
#242300=CARTESIAN_POINT('Ctrl Pts',(3.44882239259403,-6.61171580102016,
104.350461549742));
#242301=CARTESIAN_POINT('Ctrl Pts',(6.87608904987469,-2.88112647857823,
104.562400704175));
#242302=CARTESIAN_POINT('Ctrl Pts',(6.80638321060322,1.78716543790136,104.774339858608));
#242303=CARTESIAN_POINT('Ctrl Pts',(5.13716049914964,4.83145591810317,104.933294224433));
#242304=CARTESIAN_POINT('Ctrl Pts',(2.19400096420631,6.68633905288312,105.092248590258));
#242305=CARTESIAN_POINT('Ctrl Pts',(-2.44889156040358,7.03728565090971,
105.304187744691));
#242306=CARTESIAN_POINT('Ctrl Pts',(-7.3925022614039,3.04719515005204,105.569111687732));
#242307=CARTESIAN_POINT('Ctrl Pts',(-6.55445662757077,-4.59010423053793,
105.887020419382));
#242308=CARTESIAN_POINT('Ctrl Pts',(-0.84187481190605,-7.40335579165466,
106.151944362423));
#242309=CARTESIAN_POINT('Ctrl Pts',(3.59195542694403,-6.04308161462527,
106.363883516856));
#242310=CARTESIAN_POINT('Ctrl Pts',(6.91962929457424,-2.7799086594323,106.575822671289));
#242311=CARTESIAN_POINT('Ctrl Pts',(7.09717573846594,2.28289004218361,106.787761825722));
#242312=CARTESIAN_POINT('Ctrl Pts',(4.00838403999365,5.78391477287955,106.999700980155));
#242313=CARTESIAN_POINT('Ctrl Pts',(0.760594345871106,7.01105416635946,
107.15865534598));
#242314=CARTESIAN_POINT('Ctrl Pts',(-2.68148139540731,6.50618380366963,
107.317609711804));
#242315=CARTESIAN_POINT('Ctrl Pts',(-6.436765619817,3.75346607319929,107.529548866237));
#242316=CARTESIAN_POINT('Ctrl Pts',(-7.59747484998492,-2.49256170860609,
107.794472809279));
#242317=CARTESIAN_POINT('Ctrl Pts',(-1.99422331481243,-7.74938913080039,
108.112381540928));
#242318=CARTESIAN_POINT('Ctrl Pts',(4.1749326607475,-6.17157738791076,108.377305483969));
#242319=CARTESIAN_POINT('Ctrl Pts',(6.65857430471428,-2.25485419013588,
108.589244638402));
#242320=CARTESIAN_POINT('Ctrl Pts',(7.06442890749218,2.38809671916914,108.801183792835));
#242321=CARTESIAN_POINT('Ctrl Pts',(3.90691519543565,6.34960660695168,109.013122947268));
#242322=CARTESIAN_POINT('Ctrl Pts',(-0.716295588026219,7.00055235982021,
109.225062101702));
#242323=CARTESIAN_POINT('Ctrl Pts',(-3.98156109415913,5.82070060526018,
109.384016467526));
#242324=CARTESIAN_POINT('Ctrl Pts',(-6.26807582664584,3.19874906681764,
109.542970833351));
#242325=CARTESIAN_POINT('Ctrl Pts',(-7.3307269191519,-1.33450441885264,
109.754909987784));
#242326=CARTESIAN_POINT('Ctrl Pts',(-4.15062511488581,-6.83423727441782,
110.019833930825));
#242327=CARTESIAN_POINT('Ctrl Pts',(3.52455864249324,-7.18383218801323,
110.337742662475));
#242328=CARTESIAN_POINT('Ctrl Pts',(7.18500597614252,-1.9733522999061,110.602666605516));
#242329=CARTESIAN_POINT('Ctrl Pts',(6.52466527420378,2.61719740366944,110.814605759949));
#242330=CARTESIAN_POINT('Ctrl Pts',(3.81362146703718,6.40823322260278,111.026544914382));
#242331=CARTESIAN_POINT('Ctrl Pts',(-1.16125352223572,7.36430449292163,
111.238484068815));
#242332=CARTESIAN_POINT('Ctrl Pts',(-5.09667868721811,4.85228596346781,
111.450423223248));
#242333=CARTESIAN_POINT('Ctrl Pts',(-6.80992886475379,1.83255372079252,
111.609377589073));
#242334=CARTESIAN_POINT('Ctrl Pts',(-6.84184037924238,-1.64620484327354,
111.768331954898));
#242335=CARTESIAN_POINT('Ctrl Pts',(-4.70108165962939,-5.78102849297703,
111.98027110933));
#242336=CARTESIAN_POINT('Ctrl Pts',(1.2912750482904,-7.89095030506626,112.245195052372));
#242337=CARTESIAN_POINT('Ctrl Pts',(7.34921693556565,-3.16527549573553,
112.563103784021));
#242338=CARTESIAN_POINT('Ctrl Pts',(6.74151534594509,3.17338951550774,112.828027727063));
#242339=CARTESIAN_POINT('Ctrl Pts',(3.25459340362493,6.23125998231941,113.039966881496));
#242340=CARTESIAN_POINT('Ctrl Pts',(-1.27025133821028,7.34817142334694,
113.251906035929));
#242341=CARTESIAN_POINT('Ctrl Pts',(-5.67125105544294,4.83925633475936,
113.463845190362));
#242342=CARTESIAN_POINT('Ctrl Pts',(-7.02727875005749,0.371706982716854,
113.675784344795));
#242343=CARTESIAN_POINT('Ctrl Pts',(-6.36501824456443,-3.03643327424791,
113.83473871062));
#242344=CARTESIAN_POINT('Ctrl Pts',(-4.12698786823344,-5.69988958634311,
113.993693076444));
#242345=CARTESIAN_POINT('Ctrl Pts',(0.188197924330976,-7.4488281459833,
114.205632230877));
#242346=CARTESIAN_POINT('Ctrl Pts',(6.11250753694742,-5.15477832482867,
114.470556173918));
#242347=CARTESIAN_POINT('Ctrl Pts',(7.64138120966544,2.37471087471314,114.788464905568));
#242348=CARTESIAN_POINT('Ctrl Pts',(3.0576301475705,6.79480154658071,115.053388848609));
#242349=CARTESIAN_POINT('Ctrl Pts',(-1.57983992658859,6.85018868327952,
115.265328003042));
#242350=CARTESIAN_POINT('Ctrl Pts',(-5.74356178094228,4.75611814378246,
115.477267157475));
#242351=CARTESIAN_POINT('Ctrl Pts',(-7.45529008054121,-0.0118415520598074,
115.689206311908));
#242352=CARTESIAN_POINT('Ctrl Pts',(-5.58012845229728,-4.28753765789555,
115.901145466341));
#242353=CARTESIAN_POINT('Ctrl Pts',(-2.86068114714526,-6.44592023352485,
116.060099832166));
#242354=CARTESIAN_POINT('Ctrl Pts',(0.571553529458742,-7.01385034941665,
116.219054197991));
#242355=CARTESIAN_POINT('Ctrl Pts',(4.98701779701701,-5.53625439257915,
116.430993352424));
#242356=CARTESIAN_POINT('Ctrl Pts',(7.99568601189068,0.0591030169962317,
116.695917295465));
#242357=CARTESIAN_POINT('Ctrl Pts',(4.26061901329965,6.77326244533743,117.013826027115));
#242358=CARTESIAN_POINT('Ctrl Pts',(-2.09594363167219,7.15020632356861,
117.278749970156));
#242359=CARTESIAN_POINT('Ctrl Pts',(-5.65490322588073,4.17648760277076,
117.490689124589));
#242360=CARTESIAN_POINT('Ctrl Pts',(-7.45615665129927,-0.122023442024885,
117.702628279022));
#242361=CARTESIAN_POINT('Ctrl Pts',(-5.65584968870064,-4.85724764719652,
117.914567433455));
#242362=CARTESIAN_POINT('Ctrl Pts',(-1.45081887747908,-6.88592312596942,
118.126506587888));
#242363=CARTESIAN_POINT('Ctrl Pts',(2.018678504524,-6.75709415192438,118.285460953713));
#242364=CARTESIAN_POINT('Ctrl Pts',(4.9953704984076,-4.95651528240232,118.444415319538));
#242365=CARTESIAN_POINT('Ctrl Pts',(7.38876452641094,-0.962609983517036,
118.65635447397));
#242366=CARTESIAN_POINT('Ctrl Pts',(6.03563693453518,5.24457574660108,118.921278417012));
#242367=CARTESIAN_POINT('Ctrl Pts',(-1.16806356881025,7.91615980315751,
119.239187148661));
#242368=CARTESIAN_POINT('Ctrl Pts',(-6.24207561025776,4.06877404786426,
119.504111091703));
#242369=CARTESIAN_POINT('Ctrl Pts',(-7.01186580799012,-0.504695037535718,
119.716050246136));
#242370=CARTESIAN_POINT('Ctrl Pts',(-5.58485557652853,-4.94151291796711,
119.927989400569));
#242371=CARTESIAN_POINT('Ctrl Pts',(-1.13785365035902,-7.36795626193152,
120.139928555001));
#242372=CARTESIAN_POINT('Ctrl Pts',(3.37584513009584,-6.17450260098888,
120.351867709435));
#242373=CARTESIAN_POINT('Ctrl Pts',(5.92773481558134,-3.82038535212645,
120.510822075259));
#242374=CARTESIAN_POINT('Ctrl Pts',(7.01809949255712,-0.516768491317174,
120.669776441084));
#242375=CARTESIAN_POINT('Ctrl Pts',(6.23900818738519,4.07372508214002,120.881715595517));
#242376=CARTESIAN_POINT('Ctrl Pts',(1.17448267020993,7.90917684874589,121.146639538559));
#242377=CARTESIAN_POINT('Ctrl Pts',(-6.03530163148667,5.25405488616963,
121.464548270208));
#242378=CARTESIAN_POINT('Ctrl Pts',(-7.38787504286815,-0.968365905902512,
121.729472213249));
#242379=CARTESIAN_POINT('Ctrl Pts',(-4.99848645493423,-4.94328962837636,
121.941411367682));
#242380=CARTESIAN_POINT('Ctrl Pts',(-1.02912307268412,-7.38580174594381,
122.153350522115));
#242381=CARTESIAN_POINT('Ctrl Pts',(3.92706612823956,-6.33716356359886,
122.365289676548));
#242382=CARTESIAN_POINT('Ctrl Pts',(6.57986650300704,-2.49522935110501,
122.577228830981));
#242383=CARTESIAN_POINT('Ctrl Pts',(6.98755045709731,0.952639959332536,
122.736183196806));
#242384=CARTESIAN_POINT('Ctrl Pts',(5.66749025225642,4.1713696074104,122.895137562631));
#242385=CARTESIAN_POINT('Ctrl Pts',(2.09039369796188,7.15197269252594,123.107076717064));
#242386=CARTESIAN_POINT('Ctrl Pts',(-4.2512015357783,6.77213212138965,123.372000660105));
#242387=CARTESIAN_POINT('Ctrl Pts',(-8.00159567484203,0.0665220734654481,
123.689909391754));
#242388=CARTESIAN_POINT('Ctrl Pts',(-4.98259894856729,-5.54004854622093,
123.954833334796));
#242389=CARTESIAN_POINT('Ctrl Pts',(-0.582521403186913,-7.00582957293448,
124.166772489229));
#242390=CARTESIAN_POINT('Ctrl Pts',(4.02127044483243,-6.28001160338379,
124.378711643662));
#242391=CARTESIAN_POINT('Ctrl Pts',(7.1043919316239,-2.26033309254376,124.590650798095));
#242392=CARTESIAN_POINT('Ctrl Pts',(6.62119186744593,2.38340742771311,124.802589952528));
#242393=CARTESIAN_POINT('Ctrl Pts',(4.68871164421649,5.26776683234803,124.961544318353));
#242394=CARTESIAN_POINT('Ctrl Pts',(1.5927301814374,6.85448617550486,125.120498684177));
#242395=CARTESIAN_POINT('Ctrl Pts',(-3.06299494632564,6.79253422265207,
125.33243783861));
#242396=CARTESIAN_POINT('Ctrl Pts',(-7.63349198563593,2.37997648572275,
125.597361781652));
#242397=CARTESIAN_POINT('Ctrl Pts',(-6.12182161169902,-5.15298541473229,
125.915270513301));
#242398=CARTESIAN_POINT('Ctrl Pts',(-0.182373686338716,-7.44883682297308,
126.180194456342));
#242399=CARTESIAN_POINT('Ctrl Pts',(4.11343992445248,-5.70092897500878,
126.392133610776));
#242400=CARTESIAN_POINT('Ctrl Pts',(7.13878949156039,-2.15565450021674,
126.604072765208));
#242401=CARTESIAN_POINT('Ctrl Pts',(6.86690194892787,2.90295505152627,126.816011919642));
#242402=CARTESIAN_POINT('Ctrl Pts',(3.4799576646154,6.11642929857729,127.027951074075));
#242403=CARTESIAN_POINT('Ctrl Pts',(0.136184311171292,7.05087498938877,
127.186905439899));
#242404=CARTESIAN_POINT('Ctrl Pts',(-3.24759578423723,6.24290731816938,
127.345859805724));
#242405=CARTESIAN_POINT('Ctrl Pts',(-6.74411635140901,3.16817831660003,
127.557798960157));
#242406=CARTESIAN_POINT('Ctrl Pts',(-7.34664802028274,-3.15614493226094,
127.822722903198));
#242407=CARTESIAN_POINT('Ctrl Pts',(-1.29951660707707,-7.89564532624417,
128.140631634848));
#242408=CARTESIAN_POINT('Ctrl Pts',(4.70551179355111,-5.77724752260976,
128.405555577889));
#242409=CARTESIAN_POINT('Ctrl Pts',(6.83222435584126,-1.65580480178665,
128.617494732322));
#242410=CARTESIAN_POINT('Ctrl Pts',(6.82495913021777,3.00484518735816,128.829433886755));
#242411=CARTESIAN_POINT('Ctrl Pts',(3.32874874236082,6.67090115483483,129.041373041188));
#242412=CARTESIAN_POINT('Ctrl Pts',(-1.3339621786439,6.90951211142804,129.253312195621));
#242413=CARTESIAN_POINT('Ctrl Pts',(-4.4818017325012,5.44489095512069,129.412266561446));
#242414=CARTESIAN_POINT('Ctrl Pts',(-6.52692378448263,2.63059614394271,
129.571220927271));
#242415=CARTESIAN_POINT('Ctrl Pts',(-7.18359298217773,-1.97900254517614,
129.783160081704));
#242416=CARTESIAN_POINT('Ctrl Pts',(-3.528544817525,-7.17522539280143,130.048084024745));
#242417=CARTESIAN_POINT('Ctrl Pts',(4.14741748141174,-6.84316350563237,
130.365992756394));
#242418=CARTESIAN_POINT('Ctrl Pts',(7.33163354923769,-1.32875117226272,
130.630916699436));
#242419=CARTESIAN_POINT('Ctrl Pts',(6.26701378668714,3.18520287977783,130.842855853869));
#242420=CARTESIAN_POINT('Ctrl Pts',(3.23062589135893,6.72102805265527,131.054795008302));
#242421=CARTESIAN_POINT('Ctrl Pts',(-1.809409625499,7.23239429306926,131.266734162735));
#242422=CARTESIAN_POINT('Ctrl Pts',(-5.50669623769313,4.38145058775621,
131.478673317168));
#242423=CARTESIAN_POINT('Ctrl Pts',(-6.94555312241035,1.22175125511097,
131.637627682993));
#242424=CARTESIAN_POINT('Ctrl Pts',(-6.66900335975431,-2.24614431714648,
131.796582048817));
#242425=CARTESIAN_POINT('Ctrl Pts',(-4.17018484809034,-6.17495082242762,
132.00852120325));
#242426=CARTESIAN_POINT('Ctrl Pts',(1.98559807003753,-7.74544305904998,
132.273445146292));
#242427=CARTESIAN_POINT('Ctrl Pts',(7.60084290492707,-2.50142866096168,
132.591353877941));
#242428=CARTESIAN_POINT('Ctrl Pts',(6.43371300725464,3.75842625377709,132.856277820982));
#242429=CARTESIAN_POINT('Ctrl Pts',(2.68948376270878,6.49520249623938,133.068216975416));
#242430=CARTESIAN_POINT('Ctrl Pts',(-1.91654836717798,7.20666392385459,
133.280156129848));
#242431=CARTESIAN_POINT('Ctrl Pts',(-6.0778526942598,4.31754549373526,133.492095284281));
#242432=CARTESIAN_POINT('Ctrl Pts',(-7.03256675939648,-0.252610300115997,
133.704034438715));
#242433=CARTESIAN_POINT('Ctrl Pts',(-6.07083740358252,-3.58863913962263,
133.862988804539));
#242434=CARTESIAN_POINT('Ctrl Pts',(-3.60554071796445,-6.04324618883724,
134.021943170364));
#242435=CARTESIAN_POINT('Ctrl Pts',(0.847672210623471,-7.40283294222638,
134.233882324797));
#242436=CARTESIAN_POINT('Ctrl Pts',(6.54534463423149,-4.59271145197401,
134.498806267838));
#242437=CARTESIAN_POINT('Ctrl Pts',(7.40081577286274,3.04264222337198,134.816714999488));
#242438=CARTESIAN_POINT('Ctrl Pts',(2.44336599080527,7.0390807783047,135.081638942529));
#242439=CARTESIAN_POINT('Ctrl Pts',(-2.18080593719544,6.68318470426492,
135.293578096962));
#242440=CARTESIAN_POINT('Ctrl Pts',(-6.14244425541415,4.22836746363605,
135.505517251395));
#242441=CARTESIAN_POINT('Ctrl Pts',(-7.42503155180524,-0.672671077163957,
135.717456405828));
#242442=CARTESIAN_POINT('Ctrl Pts',(-5.17798142336632,-4.76514587670965,
135.929395560261));
#242443=CARTESIAN_POINT('Ctrl Pts',(-2.27843768804545,-6.67432321415518,
136.088349926086));
#242444=CARTESIAN_POINT('Ctrl Pts',(1.19159215245574,-6.93518694849042,
136.247304291911));
#242445=CARTESIAN_POINT('Ctrl Pts',(5.45674202613881,-5.07331073985723,
136.459243446344));
#242446=CARTESIAN_POINT('Ctrl Pts',(7.96176695298124,0.769346198559143,
136.724167389385));
#242447=CARTESIAN_POINT('Ctrl Pts',(3.63863730986622,7.12111552809232,137.042076121035));
#242448=CARTESIAN_POINT('Ctrl Pts',(-2.7132561331389,6.94154457948401,137.307000064076));
#242449=CARTESIAN_POINT('Ctrl Pts',(-6.01384419569356,3.65176076193676,
137.518939218509));
#242450=CARTESIAN_POINT('Ctrl Pts',(-7.04258940770208,0.340934081417236,
137.677893584334));
#242451=CARTESIAN_POINT('Ctrl Pts',(-6.33771717830036,-3.08215861357682,
137.83685466469));
#242452=CARTESIAN_POINT('Ctrl Pts',(-4.84060268287388,-4.85066217551467,
137.942830956438));
#242453=CARTESIAN_POINT('Ctrl Pts',(-3.92431279643241,-5.50397225712299,
137.995822459578));
#242454=CARTESIAN_POINT('Ctrl Pts',(-3.09240756406622,6.45009718150145,
7.56239467184173));
#242455=CARTESIAN_POINT('Ctrl Pts',(-4.16625597930013,5.93525758761204,
7.61538861596101));
#242456=CARTESIAN_POINT('Ctrl Pts',(-6.04796825433211,4.36316698740353,
7.72136734868855));
#242457=CARTESIAN_POINT('Ctrl Pts',(-7.40390971324263,0.922356054745332,
7.88033087002435));
#242458=CARTESIAN_POINT('Ctrl Pts',(-6.93212749013402,-2.71590486739369,
8.03928523584911));
#242459=CARTESIAN_POINT('Ctrl Pts',(-4.08808205560294,-6.74442479383243,
8.25122439028213));
#242460=CARTESIAN_POINT('Ctrl Pts',(2.50132325387603,-8.0841006952593,8.51614833332338));
#242461=CARTESIAN_POINT('Ctrl Pts',(8.16072609698623,-2.24662016873822,
8.8340570649729));
#242462=CARTESIAN_POINT('Ctrl Pts',(6.60925838844497,4.29898044993359,9.09898100801417));
#242463=CARTESIAN_POINT('Ctrl Pts',(2.50056096992704,7.01388316961167,9.31092016244718));
#242464=CARTESIAN_POINT('Ctrl Pts',(-1.16435047560862,7.37151934125338,
9.46987452827195));
#242465=CARTESIAN_POINT('Ctrl Pts',(-4.53358311844593,5.90724560902383,
9.6288288940967));
#242466=CARTESIAN_POINT('Ctrl Pts',(-7.61870830154839,2.04845053597936,
9.84076804852971));
#242467=CARTESIAN_POINT('Ctrl Pts',(-7.17081369511765,-3.29369698590258,
10.0527072029627));
#242468=CARTESIAN_POINT('Ctrl Pts',(-3.48611514884083,-6.57168527676829,
10.2646463573957));
#242469=CARTESIAN_POINT('Ctrl Pts',(1.2701112294088,-7.78171110014282,10.4765855118288));
#242470=CARTESIAN_POINT('Ctrl Pts',(7.16346206903531,-4.51480301765152,
10.74150945487));
#242471=CARTESIAN_POINT('Ctrl Pts',(7.65695157177441,3.60043237751478,11.0594181865195));
#242472=CARTESIAN_POINT('Ctrl Pts',(2.22686534652227,7.5638140682943,11.3243421295608));
#242473=CARTESIAN_POINT('Ctrl Pts',(-2.66238485975687,6.95439367115044,
11.5362812839938));
#242474=CARTESIAN_POINT('Ctrl Pts',(-5.67786677217702,4.84270914258127,
11.6952356498186));
#242475=CARTESIAN_POINT('Ctrl Pts',(-7.285769897525,1.53932041547079,11.8541900156433));
#242476=CARTESIAN_POINT('Ctrl Pts',(-7.11965580283671,-3.39838631636118,
12.0661291700763));
#242477=CARTESIAN_POINT('Ctrl Pts',(-3.30559948933912,-7.16536980767384,
12.2780683245094));
#242478=CARTESIAN_POINT('Ctrl Pts',(1.62537403782534,-7.25936114246434,
12.4900074789424));
#242479=CARTESIAN_POINT('Ctrl Pts',(6.02536674244457,-5.08555498492485,
12.7019466333754));
#242480=CARTESIAN_POINT('Ctrl Pts',(8.37789497815503,1.22871831024241,12.9668705764166));
#242481=CARTESIAN_POINT('Ctrl Pts',(3.47533983566063,7.71453051659892,13.2847793080662));
#242482=CARTESIAN_POINT('Ctrl Pts',(-3.22714245398094,7.19414600682971,
13.5497032511075));
#242483=CARTESIAN_POINT('Ctrl Pts',(-6.54504611067856,3.55165879914496,
13.7616424055404));
#242484=CARTESIAN_POINT('Ctrl Pts',(-7.46256022823305,-0.0135208638365823,
13.9205967713652));
#242485=CARTESIAN_POINT('Ctrl Pts',(-6.53580761381524,-3.56863774504305,
14.07955113719));
#242486=CARTESIAN_POINT('Ctrl Pts',(-3.19857348071929,-7.21163321914283,
14.291490291623));
#242487=CARTESIAN_POINT('Ctrl Pts',(2.14855325776632,-7.59297243800312,
14.503429446056));
#242488=CARTESIAN_POINT('Ctrl Pts',(5.95558320653318,-4.45771180512786,
14.715368600489));
#242489=CARTESIAN_POINT('Ctrl Pts',(7.88447117219099,0.0550212651201416,
14.927307754922));
#242490=CARTESIAN_POINT('Ctrl Pts',(5.56537626663262,6.38165028175068,15.1922316979633));
#242491=CARTESIAN_POINT('Ctrl Pts',(-2.37673191358021,8.12053653256265,
15.5101404296128));
#242492=CARTESIAN_POINT('Ctrl Pts',(-7.12998634579964,3.36652339380924,
15.7750643726541));
#242493=CARTESIAN_POINT('Ctrl Pts',(-7.2817468703326,-1.55822700354007,
15.9870035270871));
#242494=CARTESIAN_POINT('Ctrl Pts',(-5.66028051609993,-4.86325121982078,
16.1459578929119));
#242495=CARTESIAN_POINT('Ctrl Pts',(-2.64432642941238,-6.96128538851076,
16.3049122587366));
#242496=CARTESIAN_POINT('Ctrl Pts',(2.25994333028622,-7.55851719237741,
16.5168514131696));
#242497=CARTESIAN_POINT('Ctrl Pts',(6.56997686340006,-4.37091701523981,
16.7287905676027));
#242498=CARTESIAN_POINT('Ctrl Pts',(7.42316596981569,0.486593109960187,
16.9407297220357));
#242499=CARTESIAN_POINT('Ctrl Pts',(5.95380490929089,5.16915081085088,17.1526688764687));
#242500=CARTESIAN_POINT('Ctrl Pts',(0.0777890780505113,8.4671613996115,
17.4175928195099));
#242501=CARTESIAN_POINT('Ctrl Pts',(-7.08639741108168,4.62330400239646,
17.7355015511595));
#242502=CARTESIAN_POINT('Ctrl Pts',(-7.60571217961958,-2.07926123727055,
18.0004254942007));
#242503=CARTESIAN_POINT('Ctrl Pts',(-4.5183839475935,-5.91913130284974,
18.2123646486338));
#242504=CARTESIAN_POINT('Ctrl Pts',(-1.13731542598947,-7.37539840075269,
18.3713190144585));
#242505=CARTESIAN_POINT('Ctrl Pts',(2.51818368012486,-7.0079032155646,18.5302733802833));
#242506=CARTESIAN_POINT('Ctrl Pts',(6.63218981176315,-4.27230433189676,
18.7422125347163));
#242507=CARTESIAN_POINT('Ctrl Pts',(7.8334580411794,0.952074921836845,18.9541516891493));
#242508=CARTESIAN_POINT('Ctrl Pts',(5.32271017592142,5.19701089600908,19.1660908435823));
#242509=CARTESIAN_POINT('Ctrl Pts',(1.16136705686085,7.79866267782204,19.3780299980154));
#242510=CARTESIAN_POINT('Ctrl Pts',(-5.44718841425855,6.4828243603618,19.6429539410565));
#242511=CARTESIAN_POINT('Ctrl Pts',(-8.38989641623108,-1.09617803812816,
19.9608626727062));
#242512=CARTESIAN_POINT('Ctrl Pts',(-4.42565631316116,-6.52562267142425,
20.2257866157473));
#242513=CARTESIAN_POINT('Ctrl Pts',(0.416797334882363,-7.43493031977308,
20.4377257701804));
#242514=CARTESIAN_POINT('Ctrl Pts',(3.93231470002717,-6.34246711051537,
20.5966801360051));
#242515=CARTESIAN_POINT('Ctrl Pts',(6.4702969723287,-3.68608377759403,20.7556345018299));
#242516=CARTESIAN_POINT('Ctrl Pts',(7.81659042501185,1.06744561042331,20.9675736562629));
#242517=CARTESIAN_POINT('Ctrl Pts',(5.33168859145039,5.81744001288424,21.1795128106959));
#242518=CARTESIAN_POINT('Ctrl Pts',(0.663826453443777,7.40941970128585,
21.391451965129));
#242519=CARTESIAN_POINT('Ctrl Pts',(-4.18929655188581,6.67964874851767,
21.603391119562));
#242520=CARTESIAN_POINT('Ctrl Pts',(-8.35390593924179,1.38243584517833,
21.8683150626032));
#242521=CARTESIAN_POINT('Ctrl Pts',(-5.66068565515894,-6.28876824822158,
22.1862237942527));
#242522=CARTESIAN_POINT('Ctrl Pts',(0.88164720339901,-7.83536108043323,
22.4511477372941));
#242523=CARTESIAN_POINT('Ctrl Pts',(5.151639709757,-5.37703609613148,22.663086891727));
#242524=CARTESIAN_POINT('Ctrl Pts',(7.11182805845451,-2.26094883068994,
22.8220412575518));
#242525=CARTESIAN_POINT('Ctrl Pts',(7.31238023601108,1.40749842257895,22.9809956233766));
#242526=CARTESIAN_POINT('Ctrl Pts',(5.24384804368006,5.89411432688507,23.1929347778096));
#242527=CARTESIAN_POINT('Ctrl Pts',(0.267175624221262,7.8865790255047,23.4048739322426));
#242528=CARTESIAN_POINT('Ctrl Pts',(-4.31413384508076,6.06039726724439,
23.6168130866756));
#242529=CARTESIAN_POINT('Ctrl Pts',(-7.52632181752917,2.34997721312367,
23.8287522411086));
#242530=CARTESIAN_POINT('Ctrl Pts',(-7.24521297571152,-4.38243793388043,
24.0936761841499));
#242531=CARTESIAN_POINT('Ctrl Pts',(-0.210594779177801,-8.45858250567698,
24.4115849157994));
#242532=CARTESIAN_POINT('Ctrl Pts',(5.76517584705003,-5.37893414206013,
24.6765088588406));
#242533=CARTESIAN_POINT('Ctrl Pts',(7.4102813380527,-0.73460150364279,24.8884480132737));
#242534=CARTESIAN_POINT('Ctrl Pts',(6.87295136244285,2.90732308447373,25.0474023790985));
#242535=CARTESIAN_POINT('Ctrl Pts',(4.63967550600167,5.82454871424181,25.2063567449232));
#242536=CARTESIAN_POINT('Ctrl Pts',(0.150583814495755,7.88770248668208,
25.4182958993562));
#242537=CARTESIAN_POINT('Ctrl Pts',(-4.92575868406381,6.16493413801628,
25.6302350537893));
#242538=CARTESIAN_POINT('Ctrl Pts',(-7.21845117750304,1.79836827932979,
25.8421742082222));
#242539=CARTESIAN_POINT('Ctrl Pts',(-7.24572536396301,-3.10924057500208,
26.0541133626553));
#242540=CARTESIAN_POINT('Ctrl Pts',(-2.65401681119048,-8.04083752314715,
26.3190373056965));
#242541=CARTESIAN_POINT('Ctrl Pts',(5.3407211394704,-6.56267215978184,26.6369460373461));
#242542=CARTESIAN_POINT('Ctrl Pts',(7.87759984423547,-0.337054515071836,
26.9018699803873));
#242543=CARTESIAN_POINT('Ctrl Pts',(6.10707757042656,4.26092858741369,27.1138091348203));
#242544=CARTESIAN_POINT('Ctrl Pts',(3.33050371548742,6.67815340862603,27.2727635006451));
#242545=CARTESIAN_POINT('Ctrl Pts',(-0.263147904490414,7.4419560403116,
27.4317178664699));
#242546=CARTESIAN_POINT('Ctrl Pts',(-5.01506042860352,6.08996674055397,
27.6436570209029));
#242547=CARTESIAN_POINT('Ctrl Pts',(-7.75106481605285,1.48003572830395,
27.8555961753358));
#242548=CARTESIAN_POINT('Ctrl Pts',(-6.65312870553,-3.32806915459214,28.0675353297689));
#242549=CARTESIAN_POINT('Ctrl Pts',(-3.482379423516,-7.07396257792533,28.2794744842018));
#242550=CARTESIAN_POINT('Ctrl Pts',(3.21286608213192,-7.8343069154852,28.5443984272432));
#242551=CARTESIAN_POINT('Ctrl Pts',(8.32495193223544,-1.51233048383331,
28.8623071588927));
#242552=CARTESIAN_POINT('Ctrl Pts',(6.20355589829181,4.86683462517456,29.1272311019339));
#242553=CARTESIAN_POINT('Ctrl Pts',(1.86842977113328,7.20838949201477,29.339170256367));
#242554=CARTESIAN_POINT('Ctrl Pts',(-1.81279264205507,7.23904488070974,
29.4981246221917));
#242555=CARTESIAN_POINT('Ctrl Pts',(-5.03948594832806,5.48229312442995,
29.6570789880165));
#242556=CARTESIAN_POINT('Ctrl Pts',(-7.7701524830614,1.36501149942906,29.8690181424494));
#242557=CARTESIAN_POINT('Ctrl Pts',(-6.85072366569395,-3.9162605628341,
30.0809572968826));
#242558=CARTESIAN_POINT('Ctrl Pts',(-2.88989582135995,-6.85482808039567,
30.2928964513155));
#242559=CARTESIAN_POINT('Ctrl Pts',(1.95481620639003,-7.63849504827036,
30.5048356057486));
#242560=CARTESIAN_POINT('Ctrl Pts',(7.53544428035591,-3.86211765814873,
30.7697595487898));
#242561=CARTESIAN_POINT('Ctrl Pts',(7.3076893459521,4.26493195601293,31.0876682804394));
#242562=CARTESIAN_POINT('Ctrl Pts',(1.54769439284355,7.73141818286851,31.3525922234805));
#242563=CARTESIAN_POINT('Ctrl Pts',(-3.26830241582556,6.6910468685367,31.5645313779137));
#242564=CARTESIAN_POINT('Ctrl Pts',(-6.08474730131315,4.32039792463397,
31.7234857437383));
#242565=CARTESIAN_POINT('Ctrl Pts',(-7.39353136871431,0.887496718532063,
31.8824401095632));
#242566=CARTESIAN_POINT('Ctrl Pts',(-6.79042252674316,-4.01605377353168,
32.0943792639961));
#242567=CARTESIAN_POINT('Ctrl Pts',(-2.65749558780613,-7.43015671035946,
32.3063184184292));
#242568=CARTESIAN_POINT('Ctrl Pts',(2.26240201951379,-7.08672723986146,
32.5182575728622));
#242569=CARTESIAN_POINT('Ctrl Pts',(6.45240471654349,-4.53148831810734,
32.7301967272952));
#242570=CARTESIAN_POINT('Ctrl Pts',(8.23601593229881,1.9664472712618,32.9951206703364));
#242571=CARTESIAN_POINT('Ctrl Pts',(2.77789350157973,7.99220093968132,33.313029401986));
#242572=CARTESIAN_POINT('Ctrl Pts',(-3.85208598639099,6.87979786080079,
33.5779533450272));
#242573=CARTESIAN_POINT('Ctrl Pts',(-6.8340837331447,2.95756798850223,33.7898924994603));
#242574=CARTESIAN_POINT('Ctrl Pts',(-7.43199125502254,-0.674902906563349,
33.948846865285));
#242575=CARTESIAN_POINT('Ctrl Pts',(-6.19378247767171,-4.13388620366533,
34.1078012311098));
#242576=CARTESIAN_POINT('Ctrl Pts',(-2.54679014757844,-7.46675203470667,
34.3197403855428));
#242577=CARTESIAN_POINT('Ctrl Pts',(2.81309133683725,-7.37265411302604,
34.5316795399758));
#242578=CARTESIAN_POINT('Ctrl Pts',(6.32724773147186,-3.91230137063581,
34.7436186944088));
#242579=CARTESIAN_POINT('Ctrl Pts',(7.84856333708846,0.753635553120347,
34.9555578488418));
#242580=CARTESIAN_POINT('Ctrl Pts',(4.97784241777191,6.84981446256493,35.2204817918832));
#242581=CARTESIAN_POINT('Ctrl Pts',(-3.08713196871166,7.87791751506195,
35.5383905235326));
#242582=CARTESIAN_POINT('Ctrl Pts',(-7.40031254338871,2.72131573180937,
35.8033144665739));
#242583=CARTESIAN_POINT('Ctrl Pts',(-7.11497631685437,-2.19750333079328,
36.0152536210069));
#242584=CARTESIAN_POINT('Ctrl Pts',(-5.206954666791,-5.34580312450827,36.1742079868317));
#242585=CARTESIAN_POINT('Ctrl Pts',(-2.01691374528798,-7.16826446705451,
36.3331623526564));
#242586=CARTESIAN_POINT('Ctrl Pts',(2.92098910910757,-7.32846154578664,
36.5451015070894));
#242587=CARTESIAN_POINT('Ctrl Pts',(6.93153035112154,-3.77139212111251,
36.7570406615225));
#242588=CARTESIAN_POINT('Ctrl Pts',(7.35082184076201,1.14262160642573,36.9689798159554));
#242589=CARTESIAN_POINT('Ctrl Pts',(5.47221077870483,5.67651496929609,37.1809189703885));
#242590=CARTESIAN_POINT('Ctrl Pts',(-0.67299397803026,8.44073174631607,
37.4458429134297));
#242591=CARTESIAN_POINT('Ctrl Pts',(-7.46828843488125,3.97701345481512,
37.7637516450793));
#242592=CARTESIAN_POINT('Ctrl Pts',(-7.39148533163188,-2.74520120288113,
38.0286755881206));
#242593=CARTESIAN_POINT('Ctrl Pts',(-3.97596559592911,-6.29631689626835,
38.2406147425535));
#242594=CARTESIAN_POINT('Ctrl Pts',(-0.479129498664982,-7.4471754962219,
38.3995691083783));
#242595=CARTESIAN_POINT('Ctrl Pts',(3.12941007387295,-6.7571258028181,38.558523474203));
#242596=CARTESIAN_POINT('Ctrl Pts',(6.98475802729447,-3.66765337835299,
38.7704626286361));
#242597=CARTESIAN_POINT('Ctrl Pts',(7.71824168307701,1.64263716666871,38.9824017830691));
#242598=CARTESIAN_POINT('Ctrl Pts',(4.84113051310985,5.64832906487674,39.1943409375021));
#242599=CARTESIAN_POINT('Ctrl Pts',(0.46557093722521,7.87090571062995,39.4062800919351));
#242600=CARTESIAN_POINT('Ctrl Pts',(-6.00034731120954,5.97450461984868,
39.6712040349764));
#242601=CARTESIAN_POINT('Ctrl Pts',(-8.25971766079083,-1.83549239453124,
39.9891127666259));
#242602=CARTESIAN_POINT('Ctrl Pts',(-3.82984726203311,-6.89220247827404,
40.2540367096672));
#242603=CARTESIAN_POINT('Ctrl Pts',(1.07414324747652,-7.36872615600191,
40.4659758641002));
#242604=CARTESIAN_POINT('Ctrl Pts',(4.47899531950356,-5.96896882852342,
40.624930229925));
#242605=CARTESIAN_POINT('Ctrl Pts',(6.77154338324349,-3.09808920698211,
40.7838845957497));
#242606=CARTESIAN_POINT('Ctrl Pts',(7.69121470776753,1.75605874691569,40.9958237501828));
#242607=CARTESIAN_POINT('Ctrl Pts',(4.79508258645515,6.26711213628601,41.2077629046157));
#242608=CARTESIAN_POINT('Ctrl Pts',(0.00448860928583322,7.43909575973327,
41.4197020590487));
#242609=CARTESIAN_POINT('Ctrl Pts',(-4.76485146035186,6.28204612877034,
41.6316412134818));
#242610=CARTESIAN_POINT('Ctrl Pts',(-8.4435578609544,0.636556326217869,
41.896565156523));
#242611=CARTESIAN_POINT('Ctrl Pts',(-5.08100918482557,-6.7657456226258,
42.2144738881726));
#242612=CARTESIAN_POINT('Ctrl Pts',(1.57265530582791,-7.72637951055219,
42.4793978312138));
#242613=CARTESIAN_POINT('Ctrl Pts',(5.60795156111167,-4.89926404335092,
42.6913369856469));
#242614=CARTESIAN_POINT('Ctrl Pts',(7.28423441993201,-1.62170184173807,
42.8502913514716));
#242615=CARTESIAN_POINT('Ctrl Pts',(7.15884876873537,2.05008312805698,43.0092457172964));
#242616=CARTESIAN_POINT('Ctrl Pts',(4.70079181698436,6.335699037752,43.2211848717293));
#242617=CARTESIAN_POINT('Ctrl Pts',(-0.43289356831613,7.87922043721453,
43.4331240261624));
#242618=CARTESIAN_POINT('Ctrl Pts',(-4.83431080133031,5.6541670426541,43.6450631805954));
#242619=CARTESIAN_POINT('Ctrl Pts',(-7.70498777268218,1.67364166595904,
43.8570023350284));
#242620=CARTESIAN_POINT('Ctrl Pts',(-6.82826559275586,-5.00736081209647,
44.1219262780697));
#242621=CARTESIAN_POINT('Ctrl Pts',(0.539950583094435,-8.44395769377002,
44.4398350097192));
#242622=CARTESIAN_POINT('Ctrl Pts',(6.21924122155443,-4.84677456460966,
44.7047589527604));
#242623=CARTESIAN_POINT('Ctrl Pts',(7.44622706873499,-0.0749087383720799,
44.9166981071936));
#242624=CARTESIAN_POINT('Ctrl Pts',(6.58821416894859,3.50505663464716,45.0756524730181));
#242625=CARTESIAN_POINT('Ctrl Pts',(4.10516300101935,6.21285709320837,45.2346068388431));
#242626=CARTESIAN_POINT('Ctrl Pts',(-0.549126081705336,7.87000549872679,
45.4465459932759));
#242627=CARTESIAN_POINT('Ctrl Pts',(-5.45279395741946,5.70408183651311,
45.6584851477091));
#242628=CARTESIAN_POINT('Ctrl Pts',(-7.34943761644713,1.1514914641658,45.8704243021421));
#242629=CARTESIAN_POINT('Ctrl Pts',(-6.94162431600446,-3.73921981951735,
46.082363456575));
#242630=CARTESIAN_POINT('Ctrl Pts',(-1.93088115367067,-8.24442667977177,
46.3472873996164));
#242631=CARTESIAN_POINT('Ctrl Pts',(5.90137627792282,-6.06347476227379,
46.6651961312657));
#242632=CARTESIAN_POINT('Ctrl Pts',(7.87647022887751,0.362493842202579,
46.9301200743072));
#242633=CARTESIAN_POINT('Ctrl Pts',(5.7053794106066,4.78545239860063,47.1420592287401));
#242634=CARTESIAN_POINT('Ctrl Pts',(2.7254854983381,6.94706533338848,47.3010135945649));
#242635=CARTESIAN_POINT('Ctrl Pts',(-0.921721255073133,7.38934276194536,
47.4599679603896));
#242636=CARTESIAN_POINT('Ctrl Pts',(-5.53509958791175,5.62149433473857,
47.6719071148227));
#242637=CARTESIAN_POINT('Ctrl Pts',(-7.85174000401877,0.78720419777877,
47.8838462692556));
#242638=CARTESIAN_POINT('Ctrl Pts',(-6.331964339536,-3.90466304217649,48.0957854236888));
#242639=CARTESIAN_POINT('Ctrl Pts',(-2.84168138518263,-7.35477803256649,
48.3077245781216));
#242640=CARTESIAN_POINT('Ctrl Pts',(3.89460571952277,-7.51870464888691,
48.572648521163));
#242641=CARTESIAN_POINT('Ctrl Pts',(8.42623086752431,-0.768506040016876,
48.8905572528124));
#242642=CARTESIAN_POINT('Ctrl Pts',(5.74777425697222,5.39752500160179,49.1554811958538));
#242643=CARTESIAN_POINT('Ctrl Pts',(1.22216901905492,7.34562534894807,49.3674203502868));
#242644=CARTESIAN_POINT('Ctrl Pts',(-2.44728222896209,7.04987926420199,
49.5263747161115));
#242645=CARTESIAN_POINT('Ctrl Pts',(-5.50556853875714,5.01404742604368,
49.6853290819364));
#242646=CARTESIAN_POINT('Ctrl Pts',(-7.86055750992125,0.670940859405257,
49.8972682363692));
#242647=CARTESIAN_POINT('Ctrl Pts',(-6.47664796657427,-4.50805308939218,
50.1092073908024));
#242648=CARTESIAN_POINT('Ctrl Pts',(-2.27095236266987,-7.08399189981036,
50.3211465452353));
#242649=CARTESIAN_POINT('Ctrl Pts',(2.62415162413245,-7.43516921507365,
50.5330856996684));
#242650=CARTESIAN_POINT('Ctrl Pts',(7.84810112327243,-3.17902218718639,
50.7980096427096));
#242651=CARTESIAN_POINT('Ctrl Pts',(6.90091107759898,4.89585482479138,51.1159183743592));
#242652=CARTESIAN_POINT('Ctrl Pts',(0.856337932839807,7.83816754074625,
51.3808423174003));
#242653=CARTESIAN_POINT('Ctrl Pts',(-3.84849236051841,6.3750306218306,51.5927814718335));
#242654=CARTESIAN_POINT('Ctrl Pts',(-6.44373281766883,3.76407961160719,
51.7517358376581));
#242655=CARTESIAN_POINT('Ctrl Pts',(-7.44309471031215,0.228686813986007,
51.910690203483));
#242656=CARTESIAN_POINT('Ctrl Pts',(-6.40773910221589,-4.60210882113104,
52.122629357916));
#242657=CARTESIAN_POINT('Ctrl Pts',(-1.98847321494345,-7.63645767441696,
52.334568512349));
#242658=CARTESIAN_POINT('Ctrl Pts',(2.88162157363182,-6.85831050452472,
52.546507666782));
#242659=CARTESIAN_POINT('Ctrl Pts',(6.82865298432106,-3.94175232896983,
52.7584468212151));
#242660=CARTESIAN_POINT('Ctrl Pts',(8.02930751700683,2.68869747369813,53.0233707642562));
#242661=CARTESIAN_POINT('Ctrl Pts',(2.05858114621105,8.20696118126715,53.3412794959059));
#242662=CARTESIAN_POINT('Ctrl Pts',(-4.44670804338187,6.51129577188378,
53.606203438947));
#242663=CARTESIAN_POINT('Ctrl Pts',(-7.06932723955645,2.34019684178733,
53.8181425933801));
#242664=CARTESIAN_POINT('Ctrl Pts',(-7.34292177457965,-1.33097248672672,
53.9770969592048));
#242665=CARTESIAN_POINT('Ctrl Pts',(-5.80300332378635,-4.66659500596445,
54.1360513250296));
#242666=CARTESIAN_POINT('Ctrl Pts',(-1.87495989703104,-7.66309672313511,
54.3479904794625));
#242667=CARTESIAN_POINT('Ctrl Pts',(3.45548632304764,-7.09430234843002,
54.5599296338957));
#242668=CARTESIAN_POINT('Ctrl Pts',(6.64910767499218,-3.33609547172361,
54.7718687883286));
#242669=CARTESIAN_POINT('Ctrl Pts',(7.75087596897043,1.44631764037241,54.9838079427617));
#242670=CARTESIAN_POINT('Ctrl Pts',(4.35112575701066,7.26406070696073,55.2487318858029));
#242671=CARTESIAN_POINT('Ctrl Pts',(-3.77323183491082,7.57328790462749,
55.5666406174525));
#242672=CARTESIAN_POINT('Ctrl Pts',(-7.61238758926359,2.05468738324218,
55.8315645604936));
#242673=CARTESIAN_POINT('Ctrl Pts',(-6.89220061999691,-2.81948213187466,
56.0435037149268));
#242674=CARTESIAN_POINT('Ctrl Pts',(-4.71264256122068,-5.78627583495556,
56.2024580807514));
#242675=CARTESIAN_POINT('Ctrl Pts',(-1.37362503593767,-7.31881894749509,
56.3614124465763));
#242676=CARTESIAN_POINT('Ctrl Pts',(3.55904248337716,-7.04072031862616,
56.5733516010092));
#242677=CARTESIAN_POINT('Ctrl Pts',(7.23852268026616,-3.14218092206377,
56.7852907554423));
#242678=CARTESIAN_POINT('Ctrl Pts',(7.220616123312,1.78965601998303,56.9972299098752));
#242679=CARTESIAN_POINT('Ctrl Pts',(4.9475424430092,6.13919675347174,57.2091690643084));
#242680=CARTESIAN_POINT('Ctrl Pts',(-1.41847959915863,8.34786133896,57.4740930073495));
#242681=CARTESIAN_POINT('Ctrl Pts',(-7.79139323847274,3.29941806533262,
57.7920017389992));
#242682=CARTESIAN_POINT('Ctrl Pts',(-7.1190768148242,-3.38953246874281,
58.0569256820402));
#242683=CARTESIAN_POINT('Ctrl Pts',(-3.40225065052701,-6.62394137875892,
58.2688648364734));
#242684=CARTESIAN_POINT('Ctrl Pts',(0.182827870063121,-7.4603325608144,
58.4278192022981));
#242685=CARTESIAN_POINT('Ctrl Pts',(3.71600348895036,-6.45316004726959,
58.5867735681229));
#242686=CARTESIAN_POINT('Ctrl Pts',(7.28234610553302,-3.0341326936749,58.7987127225559));
#242687=CARTESIAN_POINT('Ctrl Pts',(7.54227161156929,2.32026948370767,59.0106518769889));
#242688=CARTESIAN_POINT('Ctrl Pts',(4.32144415866702,6.05518672326604,59.2225910314219));
#242689=CARTESIAN_POINT('Ctrl Pts',(-0.233889898346162,7.88119334356588,
59.434530185855));
#242690=CARTESIAN_POINT('Ctrl Pts',(-6.50627480548557,5.41915689597893,
59.6994541288961));
#242691=CARTESIAN_POINT('Ctrl Pts',(-8.06452299367309,-2.56035877385966,
60.0173628605457));
#242692=CARTESIAN_POINT('Ctrl Pts',(-3.20389177956769,-7.20453069372653,
60.282286803587));
#242693=CARTESIAN_POINT('Ctrl Pts',(1.72303410078483,-7.24451947100556,
60.49422595802));
#242694=CARTESIAN_POINT('Ctrl Pts',(4.99041977453763,-5.54848613785086,
60.6531803238448));
#242695=CARTESIAN_POINT('Ctrl Pts',(7.01948796416786,-2.48570819817419,
60.8121346896695));
#242696=CARTESIAN_POINT('Ctrl Pts',(7.50529801846231,2.43084916390639,61.0240738441026));
#242697=CARTESIAN_POINT('Ctrl Pts',(4.22073235354174,6.66745303241609,61.2360129985355));
#242698=CARTESIAN_POINT('Ctrl Pts',(-0.654884566712431,7.41021538650372,
61.4479521529686));
#242699=CARTESIAN_POINT('Ctrl Pts',(-5.30290010354056,5.8349947296536,61.6598913074015));
#242700=CARTESIAN_POINT('Ctrl Pts',(-8.46674678300096,-0.114333810730216,
61.9248152504429));
#242701=CARTESIAN_POINT('Ctrl Pts',(-4.46133783113658,-7.18946680379233,
62.2427239820923));
#242702=CARTESIAN_POINT('Ctrl Pts',(2.25128433881871,-7.556580170806,62.5076479251336));
#242703=CARTESIAN_POINT('Ctrl Pts',(6.02012073128016,-4.38292770406461,
62.7195870795667));
#242704=CARTESIAN_POINT('Ctrl Pts',(7.39930333222143,-0.969689716247477,
62.8785414453915));
#242705=CARTESIAN_POINT('Ctrl Pts',(6.94896681850422,2.67653071734569,63.0374958112161));
#242706=CARTESIAN_POINT('Ctrl Pts',(4.1207335669581,6.72741264333794,63.2494349656491));
#242707=CARTESIAN_POINT('Ctrl Pts',(-1.12955526302388,7.80984100014096,
63.4613741200822));
#242708=CARTESIAN_POINT('Ctrl Pts',(-5.31643474693376,5.20343035426541,
63.6733132745152));
#242709=CARTESIAN_POINT('Ctrl Pts',(-7.82300434185401,0.984132140796148,
63.8852524289482));
#242710=CARTESIAN_POINT('Ctrl Pts',(-6.35756989406835,-5.59286852605801,
64.1501763719894));
#242711=CARTESIAN_POINT('Ctrl Pts',(1.28624575415458,-8.36286673493512,
64.468085103639));
#242712=CARTESIAN_POINT('Ctrl Pts',(6.62435218204968,-4.27646386868794,
64.7330090466803));
#242713=CARTESIAN_POINT('Ctrl Pts',(7.42356023403596,0.585373666898152,
64.9449482011133));
#242714=CARTESIAN_POINT('Ctrl Pts',(6.25161821125358,4.07520032498098,65.1039025669381));
#242715=CARTESIAN_POINT('Ctrl Pts',(3.53833693205918,6.55226131047918,65.2628569327628));
#242716=CARTESIAN_POINT('Ctrl Pts',(-1.24451356227045,7.79036019687026,
65.4747960871958));
#242717=CARTESIAN_POINT('Ctrl Pts',(-5.93690786408821,5.19833016966197,
65.6867352416289));
#242718=CARTESIAN_POINT('Ctrl Pts',(-7.42257336285703,0.495550747503218,
65.8986743960618));
#242719=CARTESIAN_POINT('Ctrl Pts',(-6.58288265534216,-4.33976600161993,
66.110613550495));
#242720=CARTESIAN_POINT('Ctrl Pts',(-1.19254667180593,-8.38312028680404,
66.375537493536));
#242721=CARTESIAN_POINT('Ctrl Pts',(6.4155790588712,-5.51654905789318,66.6934462251858));
#242722=CARTESIAN_POINT('Ctrl Pts',(7.81334141260345,1.05918884928924,66.9583701682268));
#242723=CARTESIAN_POINT('Ctrl Pts',(5.25877167200093,5.27230778524644,67.17030932266));
#242724=CARTESIAN_POINT('Ctrl Pts',(2.09901377177692,7.16129381706967,67.3292636884847));
#242725=CARTESIAN_POINT('Ctrl Pts',(-1.57303932628563,7.27856467940848,
67.4882180543094));
#242726=CARTESIAN_POINT('Ctrl Pts',(-6.01156951947919,5.10877264761354,
67.7001572087426));
#242727=CARTESIAN_POINT('Ctrl Pts',(-7.89061064785605,0.0881762308052003,
67.9120963631754));
#242728=CARTESIAN_POINT('Ctrl Pts',(-5.96095827281491,-4.45052158773688,
68.1240355176085));
#242729=CARTESIAN_POINT('Ctrl Pts',(-2.17861519210624,-7.57770076348474,
68.3359746720415));
#242730=CARTESIAN_POINT('Ctrl Pts',(4.54568914768806,-7.14391930167323,
68.6008986150827));
#242731=CARTESIAN_POINT('Ctrl Pts',(8.46118325379544,-0.0186323644137214,
68.9188073467324));
#242732=CARTESIAN_POINT('Ctrl Pts',(5.2467492225371,5.88572909360765,69.1837312897735));
#242733=CARTESIAN_POINT('Ctrl Pts',(0.566288176802008,7.42504047192828,
69.3956704442066));
#242734=CARTESIAN_POINT('Ctrl Pts',(-3.06250848692811,6.80522102006031,
69.5546248100314));
#242735=CARTESIAN_POINT('Ctrl Pts',(-5.92831375746228,4.50633372899844,
69.7135791758561));
#242736=CARTESIAN_POINT('Ctrl Pts',(-7.88908994489078,-0.0284105957327118,
69.9255183302893));
#242737=CARTESIAN_POINT('Ctrl Pts',(-6.05158909666752,-5.06436160468178,
70.137457484722));
#242738=CARTESIAN_POINT('Ctrl Pts',(-1.63413626028271,-7.25739343937373,
70.3493966391552));
#242739=CARTESIAN_POINT('Ctrl Pts',(3.2728382690313,-7.17332026330462,70.5613357935883));
#242740=CARTESIAN_POINT('Ctrl Pts',(8.09896697347761,-2.47089809738648,
70.8262597366294));
#242741=CARTESIAN_POINT('Ctrl Pts',(6.43983928834939,5.48823121320375,71.1441684682791));
#242742=CARTESIAN_POINT('Ctrl Pts',(0.158195774879766,7.88323448684002,
71.4090924113202));
#242743=CARTESIAN_POINT('Ctrl Pts',(-4.39832668689196,6.00881249973269,
71.6210315657532));
#242744=CARTESIAN_POINT('Ctrl Pts',(-6.75213301471285,3.17817874136241,
71.779985931578));
#242745=CARTESIAN_POINT('Ctrl Pts',(-7.43381632393515,-0.43200928049931,
71.9389402974028));
#242746=CARTESIAN_POINT('Ctrl Pts',(-5.97519664327555,-5.15174218629462,
72.1508794518358));
#242747=CARTESIAN_POINT('Ctrl Pts',(-1.30268824194961,-7.78302532067559,
72.3628186062687));
#242748=CARTESIAN_POINT('Ctrl Pts',(3.47686054563489,-6.57546876338237,
72.5747577607018));
#242749=CARTESIAN_POINT('Ctrl Pts',(7.15418212494621,-3.32201596284964,
72.7866969151348));
#242750=CARTESIAN_POINT('Ctrl Pts',(7.75298169246792,3.39194015110797,73.051620858176));
#242751=CARTESIAN_POINT('Ctrl Pts',(1.33416029501156,8.35347911467427,73.3695295898257));
#242752=CARTESIAN_POINT('Ctrl Pts',(-6.29541838040319,5.6453087392055,73.6874383214751));
#242753=CARTESIAN_POINT('Ctrl Pts',(-8.1578247845443,-2.23879346110978,
74.0053470531247));
#242754=CARTESIAN_POINT('Ctrl Pts',(-2.53203993743254,-8.06787314603517,
74.3232557847741));
#242755=CARTESIAN_POINT('Ctrl Pts',(5.41111795255811,-6.50233800379432,
74.6411645164237));
#242756=CARTESIAN_POINT('Ctrl Pts',(8.39828963266304,1.04053561128162,74.9590732480732));
#242757=CARTESIAN_POINT('Ctrl Pts',(4.4563813353463,6.50836210795808,75.2239971911145));
#242758=CARTESIAN_POINT('Ctrl Pts',(-0.366475770832498,7.42906752031522,
75.4359363455475));
#242759=CARTESIAN_POINT('Ctrl Pts',(-5.09287915284989,6.02785714267165,
75.6478754999804));
#242760=CARTESIAN_POINT('Ctrl Pts',(-7.76778677712684,1.38018515603965,
75.8598146544136));
#242761=CARTESIAN_POINT('Ctrl Pts',(-6.6130024664685,-3.42293083992707,
76.0717538088464));
#242762=CARTESIAN_POINT('Ctrl Pts',(-4.18406943566272,-6.17945655523008,
76.2307081746713));
#242763=CARTESIAN_POINT('Ctrl Pts',(-0.715149063313115,-7.41212972895188,
76.3896625404961));
#242764=CARTESIAN_POINT('Ctrl Pts',(4.15985583163179,-6.69820956209441,
76.601601694929));
#242765=CARTESIAN_POINT('Ctrl Pts',(8.33909590344503,-1.43237265489772,
76.8665256379704));
#242766=CARTESIAN_POINT('Ctrl Pts',(5.70325544624252,6.25871238834748,77.1844343696198));
#242767=CARTESIAN_POINT('Ctrl Pts',(-0.847078634713838,7.8390338512972,
77.4493583126611));
#242768=CARTESIAN_POINT('Ctrl Pts',(-5.10960119783234,5.40667517520201,
77.6612974670941));
#242769=CARTESIAN_POINT('Ctrl Pts',(-7.78887677874035,1.26605196713225,
77.8732366215271));
#242770=CARTESIAN_POINT('Ctrl Pts',(-6.79849382308411,-4.00237792543563,
78.0851757759601));
#242771=CARTESIAN_POINT('Ctrl Pts',(-2.79772326318019,-6.90106457198351,
78.2971149303932));
#242772=CARTESIAN_POINT('Ctrl Pts',(0.840057590336768,-7.4151395542697,
78.4560692962179));
#242773=CARTESIAN_POINT('Ctrl Pts',(4.27690811805749,-6.09589741208402,
78.6150236620428));
#242774=CARTESIAN_POINT('Ctrl Pts',(7.51602684544494,-2.38317536620462,
78.8269628164757));
#242775=CARTESIAN_POINT('Ctrl Pts',(7.2664367172965,4.33484332506232,79.0918867595171));
#242776=CARTESIAN_POINT('Ctrl Pts',(0.262479329093425,8.463449498758,79.4097954911665));
#242777=CARTESIAN_POINT('Ctrl Pts',(-5.74130361826883,5.40419705220362,
79.6747194342077));
#242778=CARTESIAN_POINT('Ctrl Pts',(-7.39762060038627,0.784458657860876,
79.8866585886409));
#242779=CARTESIAN_POINT('Ctrl Pts',(-6.74029237988116,-4.10340956735422,
80.0985977430736));
#242780=CARTESIAN_POINT('Ctrl Pts',(-2.56181520562744,-7.46161034259711,
80.3105368975069));
#242781=CARTESIAN_POINT('Ctrl Pts',(2.36249069307547,-7.06191151456218,
80.5224760519397));
#242782=CARTESIAN_POINT('Ctrl Pts',(5.46030712988442,-5.08675082895186,
80.6814304177646));
#242783=CARTESIAN_POINT('Ctrl Pts',(7.21325806895984,-1.84954505519482,
80.8403847835894));
#242784=CARTESIAN_POINT('Ctrl Pts',(7.25949369712115,3.07732616240482,81.0523239380222));
#242785=CARTESIAN_POINT('Ctrl Pts',(2.70109108776638,8.01848334190188,81.3172478810638));
#242786=CARTESIAN_POINT('Ctrl Pts',(-5.30447112776438,6.60011055681453,
81.635156612713));
#242787=CARTESIAN_POINT('Ctrl Pts',(-7.87589359057637,0.371770295664173,
81.9000805557545));
#242788=CARTESIAN_POINT('Ctrl Pts',(-6.12988222590252,-4.21482025321488,
82.1120197101873));
#242789=CARTESIAN_POINT('Ctrl Pts',(-2.45189947187555,-7.50051335038523,
82.3239588646206));
#242790=CARTESIAN_POINT('Ctrl Pts',(2.90623134771161,-7.33432651013266,
82.5358980190533));
#242791=CARTESIAN_POINT('Ctrl Pts',(6.38714403999805,-3.82836094665771,
82.7478371734866));
#242792=CARTESIAN_POINT('Ctrl Pts',(7.45599080795447,-0.313351272057573,
82.906791539311));
#242793=CARTESIAN_POINT('Ctrl Pts',(6.6824644485123,3.28581462846386,83.0657459051361));
#242794=CARTESIAN_POINT('Ctrl Pts',(3.51359306648352,7.05867188748558,83.2776850595689));
#242795=CARTESIAN_POINT('Ctrl Pts',(-3.16256807410052,7.84793803129486,
83.5426090026103));
#242796=CARTESIAN_POINT('Ctrl Pts',(-8.32176050922241,1.5643450178527,83.8605177342598));
#242797=CARTESIAN_POINT('Ctrl Pts',(-6.22483574080837,-4.83935253966577,
84.1254416773011));
#242798=CARTESIAN_POINT('Ctrl Pts',(-1.91573847867857,-7.18819253716854,
84.337380831734));
#242799=CARTESIAN_POINT('Ctrl Pts',(3.01502991504078,-7.29240057533304,
84.5493199861671));
#242800=CARTESIAN_POINT('Ctrl Pts',(6.97736106495208,-3.68170593242992,
84.7612591406));
#242801=CARTESIAN_POINT('Ctrl Pts',(7.34173586737877,1.2453397043426,84.9731982950332));
#242802=CARTESIAN_POINT('Ctrl Pts',(5.86785825508849,4.61066453412179,85.1321526608577));
#242803=CARTESIAN_POINT('Ctrl Pts',(2.93965982041344,6.84180597638467,85.2911070266827));
#242804=CARTESIAN_POINT('Ctrl Pts',(-1.92116048583458,7.64717774343563,
85.5030461811155));
#242805=CARTESIAN_POINT('Ctrl Pts',(-7.50609891412956,3.90518210300933,
85.7679701241569));
#242806=CARTESIAN_POINT('Ctrl Pts',(-7.33909050950137,-4.22334272834674,
86.0858788558065));
#242807=CARTESIAN_POINT('Ctrl Pts',(-1.58173190621261,-7.72437940420364,
86.3508027988476));
#242808=CARTESIAN_POINT('Ctrl Pts',(3.21922918449413,-6.70646921470574,
86.5627419532807));
#242809=CARTESIAN_POINT('Ctrl Pts',(7.03274706135878,-3.57910328303859,
86.7746811077136));
#242810=CARTESIAN_POINT('Ctrl Pts',(7.69473398792592,1.74057314085235,86.9866202621468));
#242811=CARTESIAN_POINT('Ctrl Pts',(4.76742954577874,5.72045208454751,87.1985594165797));
#242812=CARTESIAN_POINT('Ctrl Pts',(1.45926545835945,7.31850615016874,87.3575137824045));
#242813=CARTESIAN_POINT('Ctrl Pts',(-2.21612945958299,7.10919679686913,
87.5164681482293));
#242814=CARTESIAN_POINT('Ctrl Pts',(-6.43248396591558,4.5599709516912,87.7284073026623));
#242815=CARTESIAN_POINT('Ctrl Pts',(-8.24172842909861,-1.91464896713466,
87.9933312457035));
#242816=CARTESIAN_POINT('Ctrl Pts',(-2.82879388550048,-7.98102740636118,
88.3112399773531));
#242817=CARTESIAN_POINT('Ctrl Pts',(3.82165136322666,-6.89658566691984,
88.5761639203943));
#242818=CARTESIAN_POINT('Ctrl Pts',(6.80683364698421,-3.00119669005193,
88.7881030748274));
#242819=CARTESIAN_POINT('Ctrl Pts',(7.67008543412729,1.85453524444709,89.0000422292602));
#242820=CARTESIAN_POINT('Ctrl Pts',(4.71353575314952,6.3262237320047,89.2119813836935));
#242821=CARTESIAN_POINT('Ctrl Pts',(-0.098402050417027,7.44595686007123,
89.4239205381264));
#242822=CARTESIAN_POINT('Ctrl Pts',(-3.65074172699665,6.50861527444854,
89.582874903951));
#242823=CARTESIAN_POINT('Ctrl Pts',(-6.30670810150985,3.95946231205651,
89.7418292697761));
#242824=CARTESIAN_POINT('Ctrl Pts',(-7.85195271698889,-0.719043518989206,
89.9537684242088));
#242825=CARTESIAN_POINT('Ctrl Pts',(-5.01586699380124,-6.81417980881466,
90.2186923672503));
#242826=CARTESIAN_POINT('Ctrl Pts',(3.04119827736541,-7.90253037611894,
90.5366010988996));
#242827=CARTESIAN_POINT('Ctrl Pts',(7.38810959676663,-2.75386085149218,
90.8015250419411));
#242828=CARTESIAN_POINT('Ctrl Pts',(7.12264747423663,2.14663896075815,91.0134641963739));
#242829=CARTESIAN_POINT('Ctrl Pts',(4.62070028810255,6.3967679641548,91.2254033508071));
#242830=CARTESIAN_POINT('Ctrl Pts',(-0.533283023543019,7.87109491877717,
91.43734250524));
#242831=CARTESIAN_POINT('Ctrl Pts',(-4.91693545721402,5.59246834905301,
91.649281659673));
#242832=CARTESIAN_POINT('Ctrl Pts',(-7.00597375351663,2.57027619392447,
91.8082360254978));
#242833=CARTESIAN_POINT('Ctrl Pts',(-7.36588777354428,-1.09343778323085,
91.9671903913226));
#242834=CARTESIAN_POINT('Ctrl Pts',(-5.49728114084035,-5.65244063308855,
92.1791295457554));
#242835=CARTESIAN_POINT('Ctrl Pts',(0.620934315895268,-8.43838898971278,
92.4440534887969));
#242836=CARTESIAN_POINT('Ctrl Pts',(7.44940004548645,-4.02558222745956,
92.7619622204463));
#242837=CARTESIAN_POINT('Ctrl Pts',(7.40337956209903,2.71254199280134,93.0268861634876));
#242838=CARTESIAN_POINT('Ctrl Pts',(4.01487075809005,6.26266546016378,93.2388253179207));
#242839=CARTESIAN_POINT('Ctrl Pts',(-0.649682860062558,7.86431330257443,
93.4507644723536));
#242840=CARTESIAN_POINT('Ctrl Pts',(-5.52377257392429,5.63262483706841,
93.6627036267866));
#242841=CARTESIAN_POINT('Ctrl Pts',(-7.3720816832314,1.05088923361697,93.8746427812198));
#242842=CARTESIAN_POINT('Ctrl Pts',(-6.9936959353334,-2.60349862917581,
94.0335971470443));
#242843=CARTESIAN_POINT('Ctrl Pts',(-4.8845603776014,-5.62076318624192,
94.1925515128693));
#242844=CARTESIAN_POINT('Ctrl Pts',(-0.500271895129622,-7.86892070635947,
94.4044906673021));
#242845=CARTESIAN_POINT('Ctrl Pts',(5.95927569764219,-6.00657983596767,
94.6694146103437));
#242846=CARTESIAN_POINT('Ctrl Pts',(8.27695351647176,1.78631290481188,94.9873233419929));
#242847=CARTESIAN_POINT('Ctrl Pts',(3.86012155736479,6.87512723995585,95.2522472850343));
#242848=CARTESIAN_POINT('Ctrl Pts',(-1.02270433851611,7.36846264196782,
95.4641864394672));
#242849=CARTESIAN_POINT('Ctrl Pts',(-5.60778772912366,5.55177704206492,
95.6761255939003));
#242850=CARTESIAN_POINT('Ctrl Pts',(-7.85919101256279,0.686762427372801,
95.8880647483333));
#242851=CARTESIAN_POINT('Ctrl Pts',(-6.28374366028536,-3.99581307588229,
96.1000039027662));
#242852=CARTESIAN_POINT('Ctrl Pts',(-3.61980976095626,-6.52586892624304,
96.2589582685911));
#242853=CARTESIAN_POINT('Ctrl Pts',(-0.0554072921370151,-7.44639771367499,
96.4179126344158));
#242854=CARTESIAN_POINT('Ctrl Pts',(4.73719936073806,-6.30310457383125,
96.6298517888488));
#242855=CARTESIAN_POINT('Ctrl Pts',(8.43321588618773,-0.687632156979905,
96.8947757318901));
#242856=CARTESIAN_POINT('Ctrl Pts',(5.12608465367676,6.73959415922588,97.2126844635397));
#242857=CARTESIAN_POINT('Ctrl Pts',(-1.53855266836986,7.73309567313556,
97.4776084065809));
#242858=CARTESIAN_POINT('Ctrl Pts',(-5.5687036671652,4.93251511273872,97.689547561014));
#242859=CARTESIAN_POINT('Ctrl Pts',(-7.87043854008896,0.570708968205702,
97.9014867154469));
#242860=CARTESIAN_POINT('Ctrl Pts',(-6.41698994571513,-4.58920102416412,
98.11342586988));
#242861=CARTESIAN_POINT('Ctrl Pts',(-2.17504481640704,-7.12187732077639,
98.325365024313));
#242862=CARTESIAN_POINT('Ctrl Pts',(1.49398373177941,-7.31149783267407,
98.4843193901377));
#242863=CARTESIAN_POINT('Ctrl Pts',(4.80037800867734,-5.69282705270879,
98.6432737559625));
#242864=CARTESIAN_POINT('Ctrl Pts',(7.69767586257887,-1.70762155254026,
98.8552129103956));
#242865=CARTESIAN_POINT('Ctrl Pts',(6.85362425769077,4.96183461037897,99.1201368534366));
#242866=CARTESIAN_POINT('Ctrl Pts',(-0.48870159495969,8.45340428814426,
99.4380455850865));
#242867=CARTESIAN_POINT('Ctrl Pts',(-6.1977021057436,4.87405391965216,99.7029695281274));
#242868=CARTESIAN_POINT('Ctrl Pts',(-7.43803518614661,0.125691844365409,
99.9149086825606));
#242869=CARTESIAN_POINT('Ctrl Pts',(-6.35006357928672,-4.68467758535475,
100.126847836994));
#242870=CARTESIAN_POINT('Ctrl Pts',(-1.89038154652329,-7.65930699294415,
100.338786991427));
#242871=CARTESIAN_POINT('Ctrl Pts',(2.97911681246191,-6.82472120626732,
100.55072614586));
#242872=CARTESIAN_POINT('Ctrl Pts',(5.88967505890723,-4.58276288373128,
100.709680511685));
#242873=CARTESIAN_POINT('Ctrl Pts',(7.34880093971353,-1.20292710781303,
100.868634877509));
#242874=CARTESIAN_POINT('Ctrl Pts',(6.9581671574302,3.70865135342868,101.080574031942));
#242875=CARTESIAN_POINT('Ctrl Pts',(1.97975149545645,8.22633285143508,101.345497974984));
#242876=CARTESIAN_POINT('Ctrl Pts',(-5.86858724447197,6.10397878942532,
101.663406706633));
#242877=CARTESIAN_POINT('Ctrl Pts',(-7.87784768299701,-0.327763461531114,
101.928330649674));
#242878=CARTESIAN_POINT('Ctrl Pts',(-5.73218107129307,-4.7415467978292,
102.140269804107));
#242879=CARTESIAN_POINT('Ctrl Pts',(-1.7774502901569,-7.68831464013599,
102.35220895854));
#242880=CARTESIAN_POINT('Ctrl Pts',(3.54486263865986,-7.04787023693198,
102.564148112973));
#242881=CARTESIAN_POINT('Ctrl Pts',(6.70132828744226,-3.2471765750409,102.776087267406));
#242882=CARTESIAN_POINT('Ctrl Pts',(7.45441961963896,0.348734974387096,
102.935041633231));
#242883=CARTESIAN_POINT('Ctrl Pts',(6.36492980544189,3.86517495723589,103.093995999056));
#242884=CARTESIAN_POINT('Ctrl Pts',(2.87412745229389,7.34231410660148,103.305935153489));
#242885=CARTESIAN_POINT('Ctrl Pts',(-3.84571384841862,7.5367402212391,103.57085909653));
#242886=CARTESIAN_POINT('Ctrl Pts',(-8.42766225216046,0.820598727297953,
103.88876782818));
#242887=CARTESIAN_POINT('Ctrl Pts',(-5.77140619028756,-5.37203719178541,
104.153691771221));
#242888=CARTESIAN_POINT('Ctrl Pts',(-1.27108166601713,-7.32970103540452,
104.365630925654));
#242889=CARTESIAN_POINT('Ctrl Pts',(3.64951694906699,-6.99646607782685,
104.577570080087));
#242890=CARTESIAN_POINT('Ctrl Pts',(7.27622378719676,-3.04878556186414,
104.78950923452));
#242891=CARTESIAN_POINT('Ctrl Pts',(7.20246161190543,1.89116452340786,105.001448388953));
#242892=CARTESIAN_POINT('Ctrl Pts',(5.4361031614677,5.11260895882911,105.160402754778));
#242893=CARTESIAN_POINT('Ctrl Pts',(2.32167470332257,7.07543182075821,105.319357120603));
#242894=CARTESIAN_POINT('Ctrl Pts',(-2.59139794363207,7.44680077279955,
105.531296275036));
#242895=CARTESIAN_POINT('Ctrl Pts',(-7.82268821872125,3.22451813439498,
105.796220218077));
#242896=CARTESIAN_POINT('Ctrl Pts',(-6.93587486720317,-4.85721248600803,
106.114128949726));
#242897=CARTESIAN_POINT('Ctrl Pts',(-0.890865357879725,-7.83417333975615,
106.379052892768));
#242898=CARTESIAN_POINT('Ctrl Pts',(3.80097920933104,-6.39474181811339,
106.590992047201));
#242899=CARTESIAN_POINT('Ctrl Pts',(7.32229773444863,-2.94167765531786,
106.802931201634));
#242900=CARTESIAN_POINT('Ctrl Pts',(7.51017599620535,2.41573643215052,107.014870356067));
#242901=CARTESIAN_POINT('Ctrl Pts',(4.2416407187964,6.12049348812788,107.2268095105));
#242902=CARTESIAN_POINT('Ctrl Pts',(0.804855002849698,7.41904282049959,
107.385763876324));
#242903=CARTESIAN_POINT('Ctrl Pts',(-2.83752269243022,6.88479294156259,
107.544718242149));
#242904=CARTESIAN_POINT('Ctrl Pts',(-6.81133516099195,3.97188851513535,
107.756657396582));
#242905=CARTESIAN_POINT('Ctrl Pts',(-8.03958861281681,-2.63760935375736,
108.021581339624));
#242906=CARTESIAN_POINT('Ctrl Pts',(-2.11027155334492,-8.20034311958203,
108.339490071273));
#242907=CARTESIAN_POINT('Ctrl Pts',(4.41788116991169,-6.5307150429149,108.604414014314));
#242908=CARTESIAN_POINT('Ctrl Pts',(7.04605138085898,-2.3860691122409,108.816353168747));
#242909=CARTESIAN_POINT('Ctrl Pts',(7.47552355515081,2.52706531694266,109.02829232318));
#242910=CARTESIAN_POINT('Ctrl Pts',(4.13426717911749,6.71910417356882,109.240231477613));
#242911=CARTESIAN_POINT('Ctrl Pts',(-0.757978402905966,7.40792989075192,
109.452170632047));
#242912=CARTESIAN_POINT('Ctrl Pts',(-4.21325688678036,6.15941996895951,
109.611124997871));
#242913=CARTESIAN_POINT('Ctrl Pts',(-6.63282893793018,3.38489130673388,
109.770079363696));
#242914=CARTESIAN_POINT('Ctrl Pts',(-7.75731803350436,-1.41216216458898,
109.982018518129));
#242915=CARTESIAN_POINT('Ctrl Pts',(-4.39215911452095,-7.23193656492455,
110.24694246117));
#242916=CARTESIAN_POINT('Ctrl Pts',(3.72966045783671,-7.60187517504613,
110.56485119282));
#242917=CARTESIAN_POINT('Ctrl Pts',(7.60311726848728,-2.08818600820106,
110.829775135861));
#242918=CARTESIAN_POINT('Ctrl Pts',(6.9043498894944,2.76949787389946,111.041714290294));
#242919=CARTESIAN_POINT('Ctrl Pts',(4.03554448357857,6.78114240086186,111.253653444727));
#242920=CARTESIAN_POINT('Ctrl Pts',(-1.22882941744544,7.79284956010438,
111.46559259916));
#242921=CARTESIAN_POINT('Ctrl Pts',(-5.39326562391045,5.134651150323,111.677531753593));
#242922=CARTESIAN_POINT('Ctrl Pts',(-7.20621359546558,1.93919405025541,
111.836486119418));
#242923=CARTESIAN_POINT('Ctrl Pts',(-7.2399821111322,-1.742001121909,111.995440485243));
#242924=CARTESIAN_POINT('Ctrl Pts',(-4.97464793565611,-6.11743924925306,
112.207379639676));
#242925=CARTESIAN_POINT('Ctrl Pts',(1.36641718192386,-8.3501420497681,112.472303582717));
#242926=CARTESIAN_POINT('Ctrl Pts',(7.77688402461956,-3.34946983496645,
112.790212314366));
#242927=CARTESIAN_POINT('Ctrl Pts',(7.13381894360561,3.35805602738686,113.055136257408));
#242928=CARTESIAN_POINT('Ctrl Pts',(3.44398534826098,6.59387069869117,113.26707541184));
#242929=CARTESIAN_POINT('Ctrl Pts',(-1.34417005593833,7.77577767174627,
113.479014566274));
#242930=CARTESIAN_POINT('Ctrl Pts',(-6.00127362130826,5.12086329887732,
113.690953720707));
#242931=CARTESIAN_POINT('Ctrl Pts',(-7.43621154838904,0.393337429153544,
113.90289287514));
#242932=CARTESIAN_POINT('Ctrl Pts',(-6.73541264825281,-3.21313000138109,
114.061847240965));
#242933=CARTESIAN_POINT('Ctrl Pts',(-4.36714636452488,-6.03157869127675,
114.220801606789));
#242934=CARTESIAN_POINT('Ctrl Pts',(0.199149575258351,-7.88229183034368,
114.432740761222));
#242935=CARTESIAN_POINT('Ctrl Pts',(6.46820778747301,-5.45474620715169,
114.697664704263));
#242936=CARTESIAN_POINT('Ctrl Pts',(8.08604998008524,2.5129005207721,115.015573435913));
#242937=CARTESIAN_POINT('Ctrl Pts',(3.23556036735803,7.1902059853941,115.280497378954));
#242938=CARTESIAN_POINT('Ctrl Pts',(-1.67177428483406,7.24881622133312,
115.492436533387));
#242939=CARTESIAN_POINT('Ctrl Pts',(-6.07779226688301,5.03288711380715,
115.70437568782));
#242940=CARTESIAN_POINT('Ctrl Pts',(-7.88912979907862,-0.012530638005558,
115.916314842253));
#242941=CARTESIAN_POINT('Ctrl Pts',(-5.90484839357282,-4.5370388993801,
116.128253996686));
#242942=CARTESIAN_POINT('Ctrl Pts',(-3.02715047165072,-6.82102250179571,
116.287208362511));
#242943=CARTESIAN_POINT('Ctrl Pts',(0.604813485768121,-7.42200171959558,
116.446162728336));
#242944=CARTESIAN_POINT('Ctrl Pts',(5.2772233254442,-5.85842120587252,116.658101882769));
#242945=CARTESIAN_POINT('Ctrl Pts',(8.46097255761023,0.0625423514801803,
116.92302582581));
#242946=CARTESIAN_POINT('Ctrl Pts',(4.50855379967994,7.16741347650078,117.24093455746));
#242947=CARTESIAN_POINT('Ctrl Pts',(-2.21791119905249,7.56629254763077,
117.505858500501));
#242948=CARTESIAN_POINT('Ctrl Pts',(-5.98397447560684,4.41952659742876,
117.717797654934));
#242949=CARTESIAN_POINT('Ctrl Pts',(-7.89004679749403,-0.1291242543574,
117.929736809367));
#242950=CARTESIAN_POINT('Ctrl Pts',(-5.98497601517829,-5.13990156533564,
118.1416759638));
#242951=CARTESIAN_POINT('Ctrl Pts',(-1.53524521725277,-7.28663012979732,
118.353615118233));
#242952=CARTESIAN_POINT('Ctrl Pts',(2.13614984430581,-7.15030431455134,
118.512569484058));
#242953=CARTESIAN_POINT('Ctrl Pts',(5.28606208889017,-5.24494580245065,
118.671523849883));
#242954=CARTESIAN_POINT('Ctrl Pts',(7.81873297671236,-1.01862637453541,
118.883463004315));
#242955=CARTESIAN_POINT('Ctrl Pts',(6.38686391572332,5.54976913829684,119.148386947357));
#242956=CARTESIAN_POINT('Ctrl Pts',(-1.23603575560048,8.37681854397064,
119.466295679006));
#242957=CARTESIAN_POINT('Ctrl Pts',(-6.60531571179499,4.3055449539786,119.731219622048));
#242958=CARTESIAN_POINT('Ctrl Pts',(-7.41990169334089,-0.534064351226985,
119.943158776481));
#242959=CARTESIAN_POINT('Ctrl Pts',(-5.90985059955452,-5.22907041745032,
120.155097930914));
#242960=CARTESIAN_POINT('Ctrl Pts',(-1.20406785558409,-7.79671383358068,
120.367037085347));
#242961=CARTESIAN_POINT('Ctrl Pts',(3.57229297924018,-6.53381048057249,
120.57897623978));
#242962=CARTESIAN_POINT('Ctrl Pts',(6.27268273526995,-4.04270197401007,
120.737930605604));
#242963=CARTESIAN_POINT('Ctrl Pts',(7.42649812971622,-0.546840385823883,
120.896884971429));
#242964=CARTESIAN_POINT('Ctrl Pts',(6.60206978884195,4.31078409982334,121.108824125862));
#242965=CARTESIAN_POINT('Ctrl Pts',(1.2428283986206,8.36942923609148,121.373748068903));
#242966=CARTESIAN_POINT('Ctrl Pts',(-6.38650910065396,5.55979988983391,
121.691656800553));
#242967=CARTESIAN_POINT('Ctrl Pts',(-7.81779173216678,-1.02471724669847,
121.956580743594));
#242968=CARTESIAN_POINT('Ctrl Pts',(-5.28935936977621,-5.23095051854392,
122.168519898027));
#242969=CARTESIAN_POINT('Ctrl Pts',(-1.08901000657497,-7.81559778553687,
122.38045905246));
#242970=CARTESIAN_POINT('Ctrl Pts',(4.15559073899923,-6.70593704216965,
122.592398206893));
#242971=CARTESIAN_POINT('Ctrl Pts',(6.96276339914931,-2.64043223223665,
122.804337361326));
#242972=CARTESIAN_POINT('Ctrl Pts',(7.39417137872784,1.00807617272766,122.963291727151));
#242973=CARTESIAN_POINT('Ctrl Pts',(5.99729396871652,4.41411077466833,123.122246092976));
#242974=CARTESIAN_POINT('Ctrl Pts',(2.21203830249847,7.56816170548093,123.334185247409));
#242975=CARTESIAN_POINT('Ctrl Pts',(-4.49858829844026,7.1662173765172,123.59910919045));
#242976=CARTESIAN_POINT('Ctrl Pts',(-8.46722611683975,0.0703931391534947,
123.917017922099));
#242977=CARTESIAN_POINT('Ctrl Pts',(-5.27254733448871,-5.86243614965592,
124.181941865141));
#242978=CARTESIAN_POINT('Ctrl Pts',(-0.616419604178061,-7.41351419649813,
124.393881019574));
#242979=CARTESIAN_POINT('Ctrl Pts',(4.25527701186128,-6.64545928375415,
124.605820174007));
#242980=CARTESIAN_POINT('Ctrl Pts',(7.51781211550661,-2.39186684402398,
124.81775932844));
#242981=CARTESIAN_POINT('Ctrl Pts',(7.00649357738897,2.52210314530843,125.029698482873));
#242982=CARTESIAN_POINT('Ctrl Pts',(4.9615580818537,5.57430976430365,125.188652848697));
#242983=CARTESIAN_POINT('Ctrl Pts',(1.68541465194798,7.25336379407827,125.347607214523));
#242984=CARTESIAN_POINT('Ctrl Pts',(-3.24123735554682,7.18780672090154,
125.559546368955));
#242985=CARTESIAN_POINT('Ctrl Pts',(-8.07770166476711,2.51847254926066,
125.824470311997));
#242986=CARTESIAN_POINT('Ctrl Pts',(-6.47806386870863,-5.45284896367621,
126.142379043646));
#242987=CARTESIAN_POINT('Ctrl Pts',(-0.192986412053176,-7.88230101226661,
126.407302986687));
#242988=CARTESIAN_POINT('Ctrl Pts',(4.35281003611391,-6.03267856425323,
126.619242141121));
#242989=CARTESIAN_POINT('Ctrl Pts',(7.55421134507096,-2.28109677429749,
126.831181295553));
#242990=CARTESIAN_POINT('Ctrl Pts',(7.26650206864976,3.07188438745797,127.043120449986));
#242991=CARTESIAN_POINT('Ctrl Pts',(3.6824640510103,6.47235776503311,127.25505960442));
#242992=CARTESIAN_POINT('Ctrl Pts',(0.144109175608007,7.46118090475793,
127.414013970244));
#242993=CARTESIAN_POINT('Ctrl Pts',(-3.4365805220192,6.60619581861787,127.572968336069));
#242994=CARTESIAN_POINT('Ctrl Pts',(-7.13657130729556,3.35254157735825,
127.784907490502));
#242995=CARTESIAN_POINT('Ctrl Pts',(-7.7741656185088,-3.33980794393267,
128.049831433543));
#242996=CARTESIAN_POINT('Ctrl Pts',(-1.37513833513254,-8.35511028454946,
128.367740165193));
#242997=CARTESIAN_POINT('Ctrl Pts',(4.97933586881002,-6.11343825590796,
128.632664108234));
#242998=CARTESIAN_POINT('Ctrl Pts',(7.22980651019096,-1.75215972311049,
128.844603262667));
#242999=CARTESIAN_POINT('Ctrl Pts',(7.22211850511719,3.17970373427608,129.0565424171));
#243000=CARTESIAN_POINT('Ctrl Pts',(3.52245594917145,7.05909555748589,129.268481571533));
#243001=CARTESIAN_POINT('Ctrl Pts',(-1.41158837023047,7.31159181017459,
129.480420725966));
#243002=CARTESIAN_POINT('Ctrl Pts',(-4.74260762753219,5.7617411291468,129.639375091791));
#243003=CARTESIAN_POINT('Ctrl Pts',(-6.90673982745152,2.78367631632252,
129.798329457616));
#243004=CARTESIAN_POINT('Ctrl Pts',(-7.6016220492973,-2.094165053665,130.010268612049));
#243005=CARTESIAN_POINT('Ctrl Pts',(-3.7338785971554,-7.5927675315013,130.27519255509));
#243006=CARTESIAN_POINT('Ctrl Pts',(4.38876482180459,-7.24138223315527,
130.59310128674));
#243007=CARTESIAN_POINT('Ctrl Pts',(7.75827742238802,-1.40607412393191,
130.858025229781));
#243008=CARTESIAN_POINT('Ctrl Pts',(6.63170509553124,3.37055683729277,131.069964384214));
#243009=CARTESIAN_POINT('Ctrl Pts',(3.4186231137691,7.11213944968299,131.281903538646));
#243010=CARTESIAN_POINT('Ctrl Pts',(-1.91470314918058,7.65326321574815,
131.49384269308));
#243011=CARTESIAN_POINT('Ctrl Pts',(-5.82714299697742,4.6364168290748,131.705781847513));
#243012=CARTESIAN_POINT('Ctrl Pts',(-7.34973012681403,1.29284764638627,
131.864736213338));
#243013=CARTESIAN_POINT('Ctrl Pts',(-7.05708732553743,-2.37685239259637,
132.023690579162));
#243014=CARTESIAN_POINT('Ctrl Pts',(-4.41285707159829,-6.53428478500254,
132.235629733595));
#243015=CARTESIAN_POINT('Ctrl Pts',(2.10114438661684,-8.19616741724167,
132.500553676637));
#243016=CARTESIAN_POINT('Ctrl Pts',(8.04315266228028,-2.6469922935616,132.818462408286));
#243017=CARTESIAN_POINT('Ctrl Pts',(6.80810491019363,3.9771373395256,133.083386351327));
#243018=CARTESIAN_POINT('Ctrl Pts',(2.84599073507557,6.87317260771338,133.29532550576));
#243019=CARTESIAN_POINT('Ctrl Pts',(-2.02807652975791,7.62603553978654,
133.507264660194));
#243020=CARTESIAN_POINT('Ctrl Pts',(-6.43153630330859,4.56879295715197,
133.719203814626));
#243021=CARTESIAN_POINT('Ctrl Pts',(-7.4418072786159,-0.267310248786153,
133.93114296906));
#243022=CARTESIAN_POINT('Ctrl Pts',(-6.42411277744482,-3.79746993996031,
134.090097334884));
#243023=CARTESIAN_POINT('Ctrl Pts',(-3.81535505829936,-6.39491596926097,
134.249051700709));
#243024=CARTESIAN_POINT('Ctrl Pts',(0.897000119973648,-7.83362006457017,
134.460990855142));
#243025=CARTESIAN_POINT('Ctrl Pts',(6.92623262694139,-4.85997142739007,
134.725914798183));
#243026=CARTESIAN_POINT('Ctrl Pts',(7.83148551168685,3.21970026290371,135.043823529833));
#243027=CARTESIAN_POINT('Ctrl Pts',(2.58555082899131,7.44870036260414,135.308747472874));
#243028=CARTESIAN_POINT('Ctrl Pts',(-2.30771182868448,7.07209391365953,
135.520686627307));
#243029=CARTESIAN_POINT('Ctrl Pts',(-6.49988658939628,4.47442546144379,
135.73262578174));
#243030=CARTESIAN_POINT('Ctrl Pts',(-7.85711046003902,-0.711815285858144,
135.944564936173));
#243031=CARTESIAN_POINT('Ctrl Pts',(-5.47929954500003,-5.04244019035943,
136.156504090606));
#243032=CARTESIAN_POINT('Ctrl Pts',(-2.41102498573675,-7.06271675396063,
136.315458456431));
#243033=CARTESIAN_POINT('Ctrl Pts',(1.26093351925047,-7.33876072244591,
136.474412822256));
#243034=CARTESIAN_POINT('Ctrl Pts',(5.77428184003987,-5.36853784432293,
136.686351976689));
#243035=CARTESIAN_POINT('Ctrl Pts',(8.42507967409952,0.814116145085501,
136.95127591973));
#243036=CARTESIAN_POINT('Ctrl Pts',(3.85037761363912,7.53550889481658,137.269184651379));
#243037=CARTESIAN_POINT('Ctrl Pts',(-2.87114647199993,7.34548831796273,
137.534108594421));
#243038=CARTESIAN_POINT('Ctrl Pts',(-6.3638030095027,3.86426474823463,137.746047748854));
#243039=CARTESIAN_POINT('Ctrl Pts',(-7.45241316685895,0.360773785080116,
137.905002114679));
#243040=CARTESIAN_POINT('Ctrl Pts',(-6.70652287292767,-3.26151619872227,
138.063963195035));
#243041=CARTESIAN_POINT('Ctrl Pts',(-5.12228799394831,-5.13293287057993,
138.169939486783));
#243042=CARTESIAN_POINT('Ctrl Pts',(-4.15267718476094,-5.82426050198983,
138.222930989923));
#243043=CARTESIAN_POINT('Ctrl Pts',(-3.26246551232774,6.80480149199297,
7.78950320218665));
#243044=CARTESIAN_POINT('Ctrl Pts',(-4.39536709389074,6.26164979395597,
7.84249714630593));
#243045=CARTESIAN_POINT('Ctrl Pts',(-6.38055865555621,4.60310664943894,
7.94847587903347));
#243046=CARTESIAN_POINT('Ctrl Pts',(-7.81106616621988,0.973078339885786,
8.10743940036926));
#243047=CARTESIAN_POINT('Ctrl Pts',(-7.31333965367775,-2.86525814630475,
8.26639376619402));
#243048=CARTESIAN_POINT('Ctrl Pts',(-4.31289422291763,-7.11531479422214,
8.47833292062704));
#243049=CARTESIAN_POINT('Ctrl Pts',(2.63887624185738,-8.52866227043683,
8.74325686366829));
#243050=CARTESIAN_POINT('Ctrl Pts',(8.60950146298311,-2.37016650229916,
9.06116559531783));
#243051=CARTESIAN_POINT('Ctrl Pts',(6.97271530600223,4.53539036026586,9.32608953835907));
#243052=CARTESIAN_POINT('Ctrl Pts',(2.63807203832175,7.39959124865925,9.53802869279212));
#243053=CARTESIAN_POINT('Ctrl Pts',(-1.22838053918788,7.77689458005039,
9.69698305861685));
#243054=CARTESIAN_POINT('Ctrl Pts',(-4.78289431932195,6.23209737818189,
9.85593742444163));
#243055=CARTESIAN_POINT('Ctrl Pts',(-8.03767697735206,2.16109910769733,
10.0678765788747));
#243056=CARTESIAN_POINT('Ctrl Pts',(-7.56515171140129,-3.47482425972199,
10.2798157333077));
#243057=CARTESIAN_POINT('Ctrl Pts',(-3.67782389916916,-6.93307597046991,
10.4917548877407));
#243058=CARTESIAN_POINT('Ctrl Pts',(1.33995729764632,-8.20964364015745,
10.7036940421737));
#243059=CARTESIAN_POINT('Ctrl Pts',(7.55739580405241,-4.76308146157516,
10.968617985215));
#243060=CARTESIAN_POINT('Ctrl Pts',(8.07802332485162,3.7984276709196,11.2865267168645));
#243061=CARTESIAN_POINT('Ctrl Pts',(2.34932532116556,7.97976399560343,11.5514506599058));
#243062=CARTESIAN_POINT('Ctrl Pts',(-2.80879496170917,7.33683029847549,
11.7633898143388));
#243063=CARTESIAN_POINT('Ctrl Pts',(-5.9901045202014,5.10901982891564,11.9223441801636));
#243064=CARTESIAN_POINT('Ctrl Pts',(-7.68642959538423,1.62397085890266,
12.0812985459883));
#243065=CARTESIAN_POINT('Ctrl Pts',(-7.51118053981663,-3.58527067503237,
12.2932377004213));
#243066=CARTESIAN_POINT('Ctrl Pts',(-3.48738130667171,-7.55940845322157,
12.5051768548543));
#243067=CARTESIAN_POINT('Ctrl Pts',(1.7147567496136,-7.65856856774657,12.7171160092874));
#243068=CARTESIAN_POINT('Ctrl Pts',(6.35671423934268,-5.36522027114204,
12.9290551637204));
#243069=CARTESIAN_POINT('Ctrl Pts',(8.83861291433131,1.29628809543511,13.1939791067616));
#243070=CARTESIAN_POINT('Ctrl Pts',(3.66645602902048,8.13876865606542,13.5118878384111));
#243071=CARTESIAN_POINT('Ctrl Pts',(-3.40460975513775,7.58976711564749,
13.7768117814524));
#243072=CARTESIAN_POINT('Ctrl Pts',(-6.90497186101978,3.7469719316452,13.9887509358854));
#243073=CARTESIAN_POINT('Ctrl Pts',(-7.87294199547984,-0.0142644043681365,
14.1477053017102));
#243074=CARTESIAN_POINT('Ctrl Pts',(-6.89522531992549,-3.7648845852275,
14.3066596675349));
#243075=CARTESIAN_POINT('Ctrl Pts',(-3.37446971438952,-7.60821598627574,
14.518598821968));
#243076=CARTESIAN_POINT('Ctrl Pts',(2.26670668715013,-8.01052584493903,
14.730537976401));
#243077=CARTESIAN_POINT('Ctrl Pts',(6.28309316109777,-4.70285068408011,
14.942477130834));
#243078=CARTESIAN_POINT('Ctrl Pts',(8.31805470310959,0.0580469993626351,
15.154416285267));
#243079=CARTESIAN_POINT('Ctrl Pts',(5.87142792689939,6.73259055432228,15.4193402283083));
#243080=CARTESIAN_POINT('Ctrl Pts',(-2.50743336363754,8.56710179050404,
15.7372489599578));
#243081=CARTESIAN_POINT('Ctrl Pts',(-7.52207918090548,3.5516555438453,16.002172902999));
#243082=CARTESIAN_POINT('Ctrl Pts',(-7.68218533352712,-1.64391715972375,
16.2141120574321));
#243083=CARTESIAN_POINT('Ctrl Pts',(-5.97155115918559,-5.13069155787081,
16.3730664232568));
#243084=CARTESIAN_POINT('Ctrl Pts',(-2.78974346057701,-7.34410100576223,
16.5320207890816));
#243085=CARTESIAN_POINT('Ctrl Pts',(2.38422233231754,-7.97417583342083,
16.7439599435146));
#243086=CARTESIAN_POINT('Ctrl Pts',(6.93127360788379,-4.61128286748637,
16.9558990979476));
#243087=CARTESIAN_POINT('Ctrl Pts',(7.83138136454493,0.513351880983981,
17.1678382523807));
#243088=CARTESIAN_POINT('Ctrl Pts',(6.28121707157689,5.45341320606732,17.3797774068136));
#243089=CARTESIAN_POINT('Ctrl Pts',(0.082066861859703,8.93278828267373,
17.6447013498549));
#243090=CARTESIAN_POINT('Ctrl Pts',(-7.47609319966269,4.87754914199904,
17.9626100815045));
#243091=CARTESIAN_POINT('Ctrl Pts',(-8.02396617154493,-2.19360415377977,
18.2275340245457));
#243092=CARTESIAN_POINT('Ctrl Pts',(-4.76685931433096,-6.24463669112668,
18.4394731789787));
#243093=CARTESIAN_POINT('Ctrl Pts',(-1.19985877574573,-7.78098695713035,
18.5984275448035));
#243094=CARTESIAN_POINT('Ctrl Pts',(2.6566638581467,-7.39328244445395,18.7573819106283));
#243095=CARTESIAN_POINT('Ctrl Pts',(6.99690777616525,-4.50724726680322,
18.9693210650612));
#243096=CARTESIAN_POINT('Ctrl Pts',(8.26423625351865,1.00443150952637,19.1812602194943));
#243097=CARTESIAN_POINT('Ctrl Pts',(5.61541712122299,5.48280537547449,19.3931993739273));
#243098=CARTESIAN_POINT('Ctrl Pts',(1.22523305601358,8.2275274204848,19.6051385283603));
#243099=CARTESIAN_POINT('Ctrl Pts',(-5.74674067777189,6.83932840674638,
19.8700624714015));
#243100=CARTESIAN_POINT('Ctrl Pts',(-8.85127433654376,-1.15645915704036,
20.1879712030511));
#243101=CARTESIAN_POINT('Ctrl Pts',(-4.66903239368483,-6.88448028628875,
20.4528951460923));
#243102=CARTESIAN_POINT('Ctrl Pts',(0.43971789051534,-7.84379266066805,
20.6648343005254));
#243103=CARTESIAN_POINT('Ctrl Pts',(4.14856089524914,-6.69125261869378,
20.8237886663501));
#243104=CARTESIAN_POINT('Ctrl Pts',(6.82611211149119,-3.88878922031102,
20.9827430321749));
#243105=CARTESIAN_POINT('Ctrl Pts',(8.24644105192192,1.12614667314857,21.1946821866079));
#243106=CARTESIAN_POINT('Ctrl Pts',(5.62488927856695,6.13735318481544,21.4066213410409));
#243107=CARTESIAN_POINT('Ctrl Pts',(0.700331656051833,7.8168791600093,21.6185604954739));
#243108=CARTESIAN_POINT('Ctrl Pts',(-4.41967471566694,7.04697657893599,
21.830499649907));
#243109=CARTESIAN_POINT('Ctrl Pts',(-8.81330466808416,1.45845887854694,
22.0954235929482));
#243110=CARTESIAN_POINT('Ctrl Pts',(-5.97197857768723,-6.63460074385073,
22.4133323245977));
#243111=CARTESIAN_POINT('Ctrl Pts',(0.930130823812995,-8.26624394487423,
22.678256267639));
#243112=CARTESIAN_POINT('Ctrl Pts',(5.43493913296469,-5.67273053720678,
22.890195422072));
#243113=CARTESIAN_POINT('Ctrl Pts',(7.50292233142839,-2.38528312728696,
23.0491497878967));
#243114=CARTESIAN_POINT('Ctrl Pts',(7.71450329194046,1.4848996994052,23.2081041537216));
#243115=CARTESIAN_POINT('Ctrl Pts',(5.53221819568165,6.21824397942342,23.4200433081545));
#243116=CARTESIAN_POINT('Ctrl Pts',(0.281868169604722,8.32027847167783,
23.6319824625876));
#243117=CARTESIAN_POINT('Ctrl Pts',(-4.55137707224933,6.39367116583729,
23.8439216170206));
#243118=CARTESIAN_POINT('Ctrl Pts',(-7.9402099676926,2.47920736634371,24.0558607714536));
#243119=CARTESIAN_POINT('Ctrl Pts',(-7.6436423637654,-4.6234373454971,24.3207847144949));
#243120=CARTESIAN_POINT('Ctrl Pts',(-0.222175825763065,-8.9237376174508,
24.6386934461444));
#243121=CARTESIAN_POINT('Ctrl Pts',(6.08221490338514,-5.67473296064375,
24.9036173891856));
#243122=CARTESIAN_POINT('Ctrl Pts',(7.81778817998088,-0.774998774025085,
25.1155565436187));
#243123=CARTESIAN_POINT('Ctrl Pts',(7.25090930717722,3.06720285078402,25.2745109094434));
#243124=CARTESIAN_POINT('Ctrl Pts',(4.8948209487679,6.14485280850215,25.4334652752682));
#243125=CARTESIAN_POINT('Ctrl Pts',(0.158864732842611,8.32146371433087,
25.6454044297012));
#243126=CARTESIAN_POINT('Ctrl Pts',(-5.19663643807538,6.50395673738447,
25.8573435841342));
#243127=CARTESIAN_POINT('Ctrl Pts',(-7.6154088784006,1.89726430563413,26.0692827385672));
#243128=CARTESIAN_POINT('Ctrl Pts',(-7.64418292931668,-3.28022420567889,
26.2812218930003));
#243129=CARTESIAN_POINT('Ctrl Pts',(-2.79996673668053,-8.48301996616586,
26.5461458360415));
#243130=CARTESIAN_POINT('Ctrl Pts',(5.63441854526134,-6.92356720336237,
26.8640545676911));
#243131=CARTESIAN_POINT('Ctrl Pts',(8.31080550648391,-0.355589846555956,
27.1289785107322));
#243132=CARTESIAN_POINT('Ctrl Pts',(6.44291851635036,4.49524594638147,27.3409176651653));
#243133=CARTESIAN_POINT('Ctrl Pts',(3.51365506821086,7.04539900718213,27.49987203099));
#243134=CARTESIAN_POINT('Ctrl Pts',(-0.277618957157626,7.85120474024724,
27.6588263968148));
#243135=CARTESIAN_POINT('Ctrl Pts',(-5.29084907199106,6.42486672621914,
27.8707655512479));
#243136=CARTESIAN_POINT('Ctrl Pts',(-8.17731205292236,1.56142598301422,
28.0827047056808));
#243137=CARTESIAN_POINT('Ctrl Pts',(-7.01899814341604,-3.51108662572979,
28.2946438601139));
#243138=CARTESIAN_POINT('Ctrl Pts',(-3.67388273850926,-7.46297454906964,
28.5065830145468));
#243139=CARTESIAN_POINT('Ctrl Pts',(3.38954829579464,-8.26513180919469,
28.7715069575882));
#243140=CARTESIAN_POINT('Ctrl Pts',(8.78275841978252,-1.59549669457496,
29.0894156892376));
#243141=CARTESIAN_POINT('Ctrl Pts',(6.54470238889186,5.13447202216646,29.3543396322789));
#243142=CARTESIAN_POINT('Ctrl Pts',(1.97117862514593,7.6047938798206,29.566278786712));
#243143=CARTESIAN_POINT('Ctrl Pts',(-1.91248189418154,7.6371350723419,29.7252331525367));
#243144=CARTESIAN_POINT('Ctrl Pts',(-5.3166178020407,5.78377586924648,29.8841875183615));
#243145=CARTESIAN_POINT('Ctrl Pts',(-8.19744939059084,1.4400763316465,30.0961266727944));
#243146=CARTESIAN_POINT('Ctrl Pts',(-7.22745926297717,-4.13162390753411,
30.3080658272275));
#243147=CARTESIAN_POINT('Ctrl Pts',(-3.04881722608634,-7.23178938801285,
30.5200049816605));
#243148=CARTESIAN_POINT('Ctrl Pts',(2.0623156308354,-8.05855183858673,30.7319441360935));
#243149=CARTESIAN_POINT('Ctrl Pts',(7.9498340937961,-4.07450357148001,30.9968680791348));
#243150=CARTESIAN_POINT('Ctrl Pts',(7.70955444004336,4.49946946857826,31.3147768107843));
#243151=CARTESIAN_POINT('Ctrl Pts',(1.63280533877429,8.15658501036109,31.5797007538256));
#243152=CARTESIAN_POINT('Ctrl Pts',(-3.44803318921775,7.05900150537185,
31.7916399082586));
#243153=CARTESIAN_POINT('Ctrl Pts',(-6.41936025911783,4.55798562661464,
31.9505942740834));
#243154=CARTESIAN_POINT('Ctrl Pts',(-7.8001170948581,0.936302015994993,
32.1095486399081));
#243155=CARTESIAN_POINT('Ctrl Pts',(-7.16384203849904,-4.23690495523571,
32.3214877943411));
#243156=CARTESIAN_POINT('Ctrl Pts',(-2.80363681848531,-7.83875654050661,
32.5334269487741));
#243157=CARTESIAN_POINT('Ctrl Pts',(2.38681622999895,-7.47644116641532,
32.7453661032072));
#243158=CARTESIAN_POINT('Ctrl Pts',(6.80723592320504,-4.78068432153856,
32.9573052576402));
#243159=CARTESIAN_POINT('Ctrl Pts',(8.68893164352905,2.07458631224778,33.2222292006814));
#243160=CARTESIAN_POINT('Ctrl Pts',(2.93065566490345,8.43170875543204,33.540137932331));
#243161=CARTESIAN_POINT('Ctrl Pts',(-4.06392023714902,7.25813230877389,
33.8050618753722));
#243162=CARTESIAN_POINT('Ctrl Pts',(-7.20990426579662,3.12021082698539,
34.0170010298053));
#243163=CARTESIAN_POINT('Ctrl Pts',(-7.84069197061069,-0.712017226454603,
34.17595539563));
#243164=CARTESIAN_POINT('Ctrl Pts',(-6.53439150746701,-4.36121723671235,
34.3349097614548));
#243165=CARTESIAN_POINT('Ctrl Pts',(-2.68684345496923,-7.8773643181432,
34.5468489158878));
#243166=CARTESIAN_POINT('Ctrl Pts',(2.96778910260848,-7.7780917552919,34.7587880703208));
#243167=CARTESIAN_POINT('Ctrl Pts',(6.67519629422216,-4.12744699109014,
34.9707272247538));
#243168=CARTESIAN_POINT('Ctrl Pts',(8.28017222118654,0.795079545623429,
35.1826663791868));
#243169=CARTESIAN_POINT('Ctrl Pts',(5.25158436503955,7.2265000608703,35.4475903222281));
#243170=CARTESIAN_POINT('Ctrl Pts',(-3.25689980097036,8.31114064669219,
35.7654990538776));
#243171=CARTESIAN_POINT('Ctrl Pts',(-7.80727118048563,2.87096656545065,
36.0304229969189));
#243172=CARTESIAN_POINT('Ctrl Pts',(-7.50624371913036,-2.31834862689053,
36.2423621513519));
#243173=CARTESIAN_POINT('Ctrl Pts',(-5.49329597497169,-5.63977999926653,
36.4013165171766));
#243174=CARTESIAN_POINT('Ctrl Pts',(-2.12782804304351,-7.56246229596497,
36.5602708830014));
#243175=CARTESIAN_POINT('Ctrl Pts',(3.08162039864436,-7.73146894651498,
36.7722100374344));
#243176=CARTESIAN_POINT('Ctrl Pts',(7.31270967674463,-3.97878884774588,
36.9841491918675));
#243177=CARTESIAN_POINT('Ctrl Pts',(7.75505888079484,1.20545675412319,37.1960883463004));
#243178=CARTESIAN_POINT('Ctrl Pts',(5.77313907428006,5.9886783788578,37.4080275007335));
#243179=CARTESIAN_POINT('Ctrl Pts',(-0.710003321956093,8.90490520756383,
37.6729514437747));
#243180=CARTESIAN_POINT('Ctrl Pts',(-7.87898520817115,4.19571772788399,
37.9908601754243));
#243181=CARTESIAN_POINT('Ctrl Pts',(-7.7979585419246,-2.89616554844543,
38.2557841184655));
#243182=CARTESIAN_POINT('Ctrl Pts',(-4.19461224505018,-6.64256450781354,
38.4677232728986));
#243183=CARTESIAN_POINT('Ctrl Pts',(-0.505477830120367,-7.85671122493527,
38.6266776387233));
#243184=CARTESIAN_POINT('Ctrl Pts',(3.30150286740242,-7.12871425820865,
38.7856320045481));
#243185=CARTESIAN_POINT('Ctrl Pts',(7.36886445395877,-3.86934529493679,
38.9975711589811));
#243186=CARTESIAN_POINT('Ctrl Pts',(8.14268390733605,1.73296921395396,39.209510313414));
#243187=CARTESIAN_POINT('Ctrl Pts',(5.10735438731375,5.95894247270799,39.4214494678471));
#243188=CARTESIAN_POINT('Ctrl Pts',(0.491173655079499,8.30374324849543,
39.6333886222801));
#243189=CARTESIAN_POINT('Ctrl Pts',(-6.33031893734865,6.30305510243496,
39.8983125653214));
#243190=CARTESIAN_POINT('Ctrl Pts',(-8.71393677955521,-1.93642995343888,
40.2162212969708));
#243191=CARTESIAN_POINT('Ctrl Pts',(-4.04045855890807,-7.2712190820607,
40.4811452400122));
#243192=CARTESIAN_POINT('Ctrl Pts',(1.13321262724659,-7.77394779171034,
40.6930843944451));
#243193=CARTESIAN_POINT('Ctrl Pts',(4.72530462334761,-6.29721488638721,
40.85203876027));
#243194=CARTESIAN_POINT('Ctrl Pts',(7.14392469148291,-3.26845960064897,
41.0109931260947));
#243195=CARTESIAN_POINT('Ctrl Pts',(8.11417066222751,1.85262808369974,41.2229322805278));
#243196=CARTESIAN_POINT('Ctrl Pts',(5.05877418903363,6.61175371710629,41.4348714349606));
#243197=CARTESIAN_POINT('Ctrl Pts',(0.00473544728136623,7.84818716686823,
41.6468105893938));
#243198=CARTESIAN_POINT('Ctrl Pts',(-5.02688059019021,6.62750896101593,
41.8587497438267));
#243199=CARTESIAN_POINT('Ctrl Pts',(-8.90788673614655,0.671561887595279,
42.123673686868));
#243200=CARTESIAN_POINT('Ctrl Pts',(-5.36042448800456,-7.13780809990443,
42.4415824185176));
#243201=CARTESIAN_POINT('Ctrl Pts',(1.65913890447776,-8.15126925093418,
42.7065063615587));
#243202=CARTESIAN_POINT('Ctrl Pts',(5.91634452571092,-5.16868480175369,
42.9184455159919));
#243203=CARTESIAN_POINT('Ctrl Pts',(7.68480967867267,-1.71088261179591,
43.0773998818165));
#243204=CARTESIAN_POINT('Ctrl Pts',(7.55252880873698,2.16282147942261,43.2363542476413));
#243205=CARTESIAN_POINT('Ctrl Pts',(4.95929817328987,6.68411235547928,43.4482934020744));
#243206=CARTESIAN_POINT('Ctrl Pts',(-0.456699289431316,8.3125152192543,
43.6602325565073));
#243207=CARTESIAN_POINT('Ctrl Pts',(-5.10015964534588,5.96510149307131,
43.8721717109404));
#243208=CARTESIAN_POINT('Ctrl Pts',(-8.12870113673735,1.76567871539049,
44.0841108653733));
#243209=CARTESIAN_POINT('Ctrl Pts',(-7.20376617372028,-5.2827260374971,
44.3490348084147));
#243210=CARTESIAN_POINT('Ctrl Pts',(0.569643592965396,-8.9083085566034,
44.6669435400641));
#243211=CARTESIAN_POINT('Ctrl Pts',(6.56125028082896,-5.11330881698911,
44.9318674831055));
#243212=CARTESIAN_POINT('Ctrl Pts',(7.85571064144068,-0.079028126288852,
45.1438066375384));
#243213=CARTESIAN_POINT('Ctrl Pts',(6.95051382093977,3.69780701682662,45.3027610033632));
#243214=CARTESIAN_POINT('Ctrl Pts',(4.33091448518403,6.55451507593636,45.461715369188));
#243215=CARTESIAN_POINT('Ctrl Pts',(-0.579323671401443,8.30279353206021,
45.673654523621));
#243216=CARTESIAN_POINT('Ctrl Pts',(-5.75265448145445,6.01776120565647,
45.8855936780539));
#243217=CARTESIAN_POINT('Ctrl Pts',(-7.75359853509504,1.21481438385805,
46.0975328324871));
#243218=CARTESIAN_POINT('Ctrl Pts',(-7.32335872983018,-3.94484732411758,
46.3094719869199));
#243219=CARTESIAN_POINT('Ctrl Pts',(-2.03706433959468,-8.69780491556567,
46.5743959299614));
#243220=CARTESIAN_POINT('Ctrl Pts',(6.22590528031026,-6.39691789874345,
46.8923046616107));
#243221=CARTESIAN_POINT('Ctrl Pts',(8.30961377121896,0.382428135398561,
47.1572286046521));
#243222=CARTESIAN_POINT('Ctrl Pts',(6.01913013605845,5.04861441704378,47.3691677590852));
#243223=CARTESIAN_POINT('Ctrl Pts',(2.87536563614646,7.32909896012022,47.5281221249098));
#243224=CARTESIAN_POINT('Ctrl Pts',(-0.972408631255065,7.79569814785787,
47.6870764907346));
#243225=CARTESIAN_POINT('Ctrl Pts',(-5.83948627040479,5.93063204473356,
47.8990156451677));
#243226=CARTESIAN_POINT('Ctrl Pts',(-8.28352357966365,0.830494200135225,
48.1109547996006));
#243227=CARTESIAN_POINT('Ctrl Pts',(-6.68017227841064,-4.11938861500226,
48.3228939540337));
#243228=CARTESIAN_POINT('Ctrl Pts',(-2.99795137740172,-7.75923263184659,
48.5348331084667));
#243229=CARTESIAN_POINT('Ctrl Pts',(4.10877821917824,-7.93217391504327,
48.799757051508));
#243230=CARTESIAN_POINT('Ctrl Pts',(8.88960689517256,-0.810767791640073,
49.1176657831574));
#243231=CARTESIAN_POINT('Ctrl Pts',(6.06385636353744,5.69434617036614,49.3825897261988));
#243232=CARTESIAN_POINT('Ctrl Pts',(1.28937864505078,7.74957662304695,49.5945288806317));
#243233=CARTESIAN_POINT('Ctrl Pts',(-2.5818633881568,7.43756684364333,49.7534832464565));
#243234=CARTESIAN_POINT('Ctrl Pts',(-5.80833124720238,5.28978036230487,
49.9124376122813));
#243235=CARTESIAN_POINT('Ctrl Pts',(-8.29282597862484,0.707837298050547,
50.1243767667142));
#243236=CARTESIAN_POINT('Ctrl Pts',(-6.83281236016946,-4.75596034066911,
50.3363159211473));
#243237=CARTESIAN_POINT('Ctrl Pts',(-2.3958367743758,-7.47355540430421,
50.5482550755803));
#243238=CARTESIAN_POINT('Ctrl Pts',(2.76845920063465,-7.84404469331985,
50.7601942300133));
#243239=CARTESIAN_POINT('Ctrl Pts',(8.27968458926794,-3.35384325440609,
51.0251181730547));
#243240=CARTESIAN_POINT('Ctrl Pts',(7.28040658544384,5.16508810314844,51.3430269047041));
#243241=CARTESIAN_POINT('Ctrl Pts',(0.903429743624333,8.26920473829927,
51.6079508477454));
#243242=CARTESIAN_POINT('Ctrl Pts',(-4.06012899028692,6.72560686548218,
51.8198900021784));
#243243=CARTESIAN_POINT('Ctrl Pts',(-6.79808713850607,3.97107420807589,
51.9788443680031));
#243244=CARTESIAN_POINT('Ctrl Pts',(-7.85240602808846,0.241262779337893,
52.1377987338279));
#243245=CARTESIAN_POINT('Ctrl Pts',(-6.76011405349243,-4.85518839346535,
52.3497378882609));
#243246=CARTESIAN_POINT('Ctrl Pts',(-2.09782350855731,-8.05640242529173,
52.561677042694));
#243247=CARTESIAN_POINT('Ctrl Pts',(3.04008796020144,-7.23546331791505,
52.7736161971269));
#243248=CARTESIAN_POINT('Ctrl Pts',(7.20417486875693,-4.15851751911049,
52.98555535156));
#243249=CARTESIAN_POINT('Ctrl Pts',(8.47085590091533,2.83655456122647,53.2504792946012));
#243250=CARTESIAN_POINT('Ctrl Pts',(2.17178682133626,8.658279111078,53.5683880262508));
#243251=CARTESIAN_POINT('Ctrl Pts',(-4.69124180250278,6.86936552063046,
53.8333119692919));
#243252=CARTESIAN_POINT('Ctrl Pts',(-7.45808430376615,2.4688891519682,54.0452511237251));
#243253=CARTESIAN_POINT('Ctrl Pts',(-7.74672437347938,-1.40416544256998,
54.2042054895497));
#243254=CARTESIAN_POINT('Ctrl Pts',(-6.12212259204269,-4.92322080823666,
54.3631598553746));
#243255=CARTESIAN_POINT('Ctrl Pts',(-1.97806785630035,-8.08450641091576,
54.5750990098075));
#243256=CARTESIAN_POINT('Ctrl Pts',(3.64551073029963,-7.48443284601927,
54.7870381642407));
#243257=CARTESIAN_POINT('Ctrl Pts',(7.01475598801421,-3.51955432679692,
54.9989773186736));
#243258=CARTESIAN_POINT('Ctrl Pts',(8.17711282074447,1.52585366703169,55.2109164731066));
#243259=CARTESIAN_POINT('Ctrl Pts',(4.59040324664707,7.66352657110666,55.475840416148));
#243260=CARTESIAN_POINT('Ctrl Pts',(-3.98072973124768,7.98975881797569,
55.7937491477973));
#243261=CARTESIAN_POINT('Ctrl Pts',(-8.03100867590238,2.16767893221239,
56.0586730908387));
#243262=CARTESIAN_POINT('Ctrl Pts',(-7.27121712159267,-2.97453134080762,
56.2706122452717));
#243263=CARTESIAN_POINT('Ctrl Pts',(-4.97180061469368,-6.10447522367803,
56.4295666110964));
#243264=CARTESIAN_POINT('Ctrl Pts',(-1.44916354451103,-7.72129608161182,
56.5885209769212));
#243265=CARTESIAN_POINT('Ctrl Pts',(3.75476166008969,-7.42790422852821,
56.8004601313542));
#243266=CARTESIAN_POINT('Ctrl Pts',(7.63658415500593,-3.31497601119741,
57.0123992857873));
#243267=CARTESIAN_POINT('Ctrl Pts',(7.61769287909937,1.88807294095723,57.2243384402202));
#243268=CARTESIAN_POINT('Ctrl Pts',(5.21961813140454,6.47680400032997,57.4362775946533));
#243269=CARTESIAN_POINT('Ctrl Pts',(-1.49648475381148,8.80692766261284,
57.7012015376945));
#243270=CARTESIAN_POINT('Ctrl Pts',(-8.21985821948872,3.48085995325354,
58.0191102693441));
#243271=CARTESIAN_POINT('Ctrl Pts',(-7.51056971204447,-3.57592993584844,
58.2840342123853));
#243272=CARTESIAN_POINT('Ctrl Pts',(-3.58934751700118,-6.98820574460903,
58.4959733668183));
#243273=CARTESIAN_POINT('Ctrl Pts',(0.192881956345414,-7.87059182397891,
58.6549277326431));
#243274=CARTESIAN_POINT('Ctrl Pts',(3.92035427906174,-6.8080327911443,58.8138820984678));
#243275=CARTESIAN_POINT('Ctrl Pts',(7.68281752192254,-3.20098598514689,
59.0258212529009));
#243276=CARTESIAN_POINT('Ctrl Pts',(7.95703687420663,2.44786594686428,59.2377604073338));
#243277=CARTESIAN_POINT('Ctrl Pts',(4.55908939524148,6.3881740831675,59.4496995617669));
#243278=CARTESIAN_POINT('Ctrl Pts',(-0.246751992170809,8.31459661984495,
59.6616387161999));
#243279=CARTESIAN_POINT('Ctrl Pts',(-6.86406844080779,5.71716764777737,
59.9265626592412));
#243280=CARTESIAN_POINT('Ctrl Pts',(-8.50800795016616,-2.70115824833899,
60.2444713908907));
#243281=CARTESIAN_POINT('Ctrl Pts',(-3.38008047759511,-7.60072287815818,
60.509395333932));
#243282=CARTESIAN_POINT('Ctrl Pts',(1.81778734332943,-7.64291072178791,
60.721334488365));
#243283=CARTESIAN_POINT('Ctrl Pts',(5.26485337691342,-5.85360897467286,
60.8802888541898));
#243284=CARTESIAN_POINT('Ctrl Pts',(7.40550426256974,-2.62240248164066,
61.0392432200145));
#243285=CARTESIAN_POINT('Ctrl Pts',(7.91803002602142,2.56452663454484,61.2511823744476));
#243286=CARTESIAN_POINT('Ctrl Pts',(4.45283923768672,7.03411019494427,61.4631215288804));
#243287=CARTESIAN_POINT('Ctrl Pts',(-0.690898036301095,7.81771860161846,
61.6750606833136));
#243288=CARTESIAN_POINT('Ctrl Pts',(-5.59451765160311,6.15587327211004,
61.8869998377465));
#243289=CARTESIAN_POINT('Ctrl Pts',(-8.93235086543013,-0.120621265688294,
62.1519237807879));
#243290=CARTESIAN_POINT('Ctrl Pts',(-4.70667611282939,-7.58483059346624,
62.4698325124373));
#243291=CARTESIAN_POINT('Ctrl Pts',(2.37508716483103,-7.97213229098914,
62.7347564554786));
#243292=CARTESIAN_POINT('Ctrl Pts',(6.35117973907172,-4.62395404916552,
62.9466956099116));
#243293=CARTESIAN_POINT('Ctrl Pts',(7.80620647068915,-1.02301497825693,
63.1056499757364));
#243294=CARTESIAN_POINT('Ctrl Pts',(7.33110501187211,2.82371872954047,63.2646043415611));
#243295=CARTESIAN_POINT('Ctrl Pts',(4.34734130905187,7.09736711005406,63.4765434959941));
#243296=CARTESIAN_POINT('Ctrl Pts',(-1.19167186521786,8.23932046208598,
63.6884826504273));
#243297=CARTESIAN_POINT('Ctrl Pts',(-5.60879659329404,5.48957785314227,
63.9004218048601));
#243298=CARTESIAN_POINT('Ctrl Pts',(-8.2532076834423,1.03825162188433,64.1123609592932));
#243299=CARTESIAN_POINT('Ctrl Pts',(-6.70718593584579,-5.90043204306947,
64.3772849023344));
#243300=CARTESIAN_POINT('Ctrl Pts',(1.3569790935935,-8.82275823664084,64.695193633984));
#243301=CARTESIAN_POINT('Ctrl Pts',(6.98863913883046,-4.51163554520679,
64.9601175770253));
#243302=CARTESIAN_POINT('Ctrl Pts',(7.83179731017781,0.617564586981519,
65.1720567314582));
#243303=CARTESIAN_POINT('Ctrl Pts',(6.5954077487877,4.29930409903505,65.3310110972831));
#243304=CARTESIAN_POINT('Ctrl Pts',(3.73291746727506,6.91258383972131,65.4899654631077));
#243305=CARTESIAN_POINT('Ctrl Pts',(-1.31295196134937,8.21876836877148,
65.7019046175408));
#243306=CARTESIAN_POINT('Ctrl Pts',(-6.2633908225815,5.48419719873932,65.9138437719738));
#243307=CARTESIAN_POINT('Ctrl Pts',(-7.83075616889244,0.522802117716418,
66.1257829264069));
#243308=CARTESIAN_POINT('Ctrl Pts',(-6.94488911626896,-4.5784187945913,
66.3377220808398));
#243309=CARTESIAN_POINT('Ctrl Pts',(-1.25812730308113,-8.84412557361244,
66.6026460238811));
#243310=CARTESIAN_POINT('Ctrl Pts',(6.768385145733,-5.81991560801015,66.9205547555308));
#243311=CARTESIAN_POINT('Ctrl Pts',(8.24301336953791,1.11743585548131,67.1854786985716));
#243312=CARTESIAN_POINT('Ctrl Pts',(5.54796250548142,5.56224299785549,67.397417853005));
#243313=CARTESIAN_POINT('Ctrl Pts',(2.21444292139709,7.55510831538417,67.5563722188296));
#243314=CARTESIAN_POINT('Ctrl Pts',(-1.65954404302216,7.67882814728032,
67.7153265846545));
#243315=CARTESIAN_POINT('Ctrl Pts',(-6.34215827828067,5.38971472157569,
67.9272657390875));
#243316=CARTESIAN_POINT('Ctrl Pts',(-8.32453180135945,0.0930252258306557,
68.1392048935204));
#243317=CARTESIAN_POINT('Ctrl Pts',(-6.28876381349589,-4.69526506162374,
68.3511440479535));
#243318=CARTESIAN_POINT('Ctrl Pts',(-2.29842179002175,-7.99441434915497,
68.5630832023865));
#243319=CARTESIAN_POINT('Ctrl Pts',(4.79566608438709,-7.5367783391113,68.8280071454277));
#243320=CARTESIAN_POINT('Ctrl Pts',(8.92648138613808,-0.0196569970329377,
69.1459158770774));
#243321=CARTESIAN_POINT('Ctrl Pts',(5.53527891642114,6.20939762466144,69.4108398201185));
#243322=CARTESIAN_POINT('Ctrl Pts',(0.5974295459376,7.83335894944233,69.6227789745516));
#243323=CARTESIAN_POINT('Ctrl Pts',(-3.23092222251469,7.17945433185997,
69.7817333403763));
#243324=CARTESIAN_POINT('Ctrl Pts',(-6.25432410808943,4.75414642905697,
69.9406877062012));
#243325=CARTESIAN_POINT('Ctrl Pts',(-8.32292747176321,-0.0299729537079767,
70.152626860634));
#243326=CARTESIAN_POINT('Ctrl Pts',(-6.38437861557071,-5.3428614226726,
70.3645660150671));
#243327=CARTESIAN_POINT('Ctrl Pts',(-1.72400082497685,-7.65649265655503,
70.5765051695001));
#243328=CARTESIAN_POINT('Ctrl Pts',(3.45281847846123,-7.56779612100605,
70.7884443239331));
#243329=CARTESIAN_POINT('Ctrl Pts',(8.54434607633237,-2.60677794249014,
71.0533682669744));
#243330=CARTESIAN_POINT('Ctrl Pts',(6.79397949587998,5.7900405059201,71.371276998624));
#243331=CARTESIAN_POINT('Ctrl Pts',(0.166895290820339,8.31675000984924,
71.6362009416652));
#243332=CARTESIAN_POINT('Ctrl Pts',(-4.64019985420912,6.3392496442617,71.8481400960982));
#243333=CARTESIAN_POINT('Ctrl Pts',(-7.12344690626189,3.3529534257354,72.0070944619229));
#243334=CARTESIAN_POINT('Ctrl Pts',(-7.84261740387319,-0.455766372781194,
72.1660488277477));
#243335=CARTESIAN_POINT('Ctrl Pts',(-6.30378518167492,-5.43504724490109,
72.3779879821807));
#243336=CARTESIAN_POINT('Ctrl Pts',(-1.37432578812005,-8.21103013242127,
72.5899271366136));
#243337=CARTESIAN_POINT('Ctrl Pts',(3.66806036601191,-6.93706751891167,
72.8018662910468));
#243338=CARTESIAN_POINT('Ctrl Pts',(7.54760553646316,-3.50470055633481,
73.0138054454797));
#243339=CARTESIAN_POINT('Ctrl Pts',(8.17933434237327,3.57847002169365,73.2787293885211));
#243340=CARTESIAN_POINT('Ctrl Pts',(1.40752855508706,8.81285437154256,73.5966381201706));
#243341=CARTESIAN_POINT('Ctrl Pts',(-6.64161658068516,5.95575605302166,
73.9145468518201));
#243342=CARTESIAN_POINT('Ctrl Pts',(-8.60644060131243,-2.36190938767852,
74.2324555834696));
#243343=CARTESIAN_POINT('Ctrl Pts',(-2.67128209997195,-8.51154233440134,
74.5503643151191));
#243344=CARTESIAN_POINT('Ctrl Pts',(5.70868662607485,-6.85991514617173,
74.8682730467687));
#243345=CARTESIAN_POINT('Ctrl Pts',(8.8601291134706,1.09775683697152,75.1861817784181));
#243346=CARTESIAN_POINT('Ctrl Pts',(4.7014470489875,6.86627052840108,75.4511057214595));
#243347=CARTESIAN_POINT('Ctrl Pts',(-0.386629038597262,7.83760745362767,
75.6630448758923));
#243348=CARTESIAN_POINT('Ctrl Pts',(-5.37294721035328,6.35934159187716,
75.8749840303256));
#243349=CARTESIAN_POINT('Ctrl Pts',(-8.19495358954785,1.45608441931355,
76.0869231847584));
#243350=CARTESIAN_POINT('Ctrl Pts',(-6.97666527869318,-3.61116495319303,
76.2988623391915));
#243351=CARTESIAN_POINT('Ctrl Pts',(-4.41416014940891,-6.51927777264119,
76.4578167050163));
#243352=CARTESIAN_POINT('Ctrl Pts',(-0.754476603388974,-7.81973821775469,
76.616771070841));
#243353=CARTESIAN_POINT('Ctrl Pts',(4.38861498873997,-7.06655809040249,
76.828710225274));
#243354=CARTESIAN_POINT('Ctrl Pts',(8.79768019749863,-1.51114181769062,
77.0936341683152));
#243355=CARTESIAN_POINT('Ctrl Pts',(6.01688937045951,6.60289204949171,77.4115428999649));
#243356=CARTESIAN_POINT('Ctrl Pts',(-0.893661257363742,8.27011868907599,
77.6764668430059));
#243357=CARTESIAN_POINT('Ctrl Pts',(-5.39058883550149,5.70399953111573,
77.8884059974392));
#243358=CARTESIAN_POINT('Ctrl Pts',(-8.21720337438167,1.33567480806146,
78.100345151872));
#243359=CARTESIAN_POINT('Ctrl Pts',(-7.172357192277,-4.22247704370048,78.3122843063052));
#243360=CARTESIAN_POINT('Ctrl Pts',(-2.95157590649486,-7.28056852080544,
78.5242234607381));
#243361=CARTESIAN_POINT('Ctrl Pts',(0.886254111097857,-7.82291355965053,
78.6831778265629));
#243362=CARTESIAN_POINT('Ctrl Pts',(4.51210422477735,-6.4311235377587,78.8421321923876));
#243363=CARTESIAN_POINT('Ctrl Pts',(7.92934885359968,-2.51423115517351,
79.0540713468206));
#243364=CARTESIAN_POINT('Ctrl Pts',(7.66603324321095,4.57322540977227,79.318995289862));
#243365=CARTESIAN_POINT('Ctrl Pts',(0.276913615402863,8.92887225664263,
79.6369040215116));
#243366=CARTESIAN_POINT('Ctrl Pts',(-6.05702989090295,5.7013851309598,79.9018279645525));
#243367=CARTESIAN_POINT('Ctrl Pts',(-7.80443120191717,0.827597677245151,
80.113767118986));
#243368=CARTESIAN_POINT('Ctrl Pts',(-7.11095513019963,-4.32906462654154,
80.3257062734185));
#243369=CARTESIAN_POINT('Ctrl Pts',(-2.70269477232959,-7.87193987364972,
80.537645427852));
#243370=CARTESIAN_POINT('Ctrl Pts',(2.49240898868442,-7.45026077257168,
80.7495845822845));
#243371=CARTESIAN_POINT('Ctrl Pts',(5.7605808189592,-5.3664818771288,80.9085389481096));
#243372=CARTESIAN_POINT('Ctrl Pts',(7.60993018997647,-1.95125539925059,
81.0674933139342));
#243373=CARTESIAN_POINT('Ctrl Pts',(7.65870841186064,3.24655475290215,81.2794324683674));
#243374=CARTESIAN_POINT('Ctrl Pts',(2.8496297260068,8.45943648182299,81.5443564114084));
#243375=CARTESIAN_POINT('Ctrl Pts',(-5.59617506972902,6.96306441601157,
81.8622651430582));
#243376=CARTESIAN_POINT('Ctrl Pts',(-8.30900542237379,0.392214720402506,
82.1271890860993));
#243377=CARTESIAN_POINT('Ctrl Pts',(-6.46697724744239,-4.44660201862032,
82.3391282405323));
#243378=CARTESIAN_POINT('Ctrl Pts',(-2.58673454289715,-7.91298223905764,
82.5510673949653));
#243379=CARTESIAN_POINT('Ctrl Pts',(3.06605107713806,-7.73765643749523,
82.7630065493983));
#243380=CARTESIAN_POINT('Ctrl Pts',(6.73838642580539,-4.03889050794708,
82.9749457038315));
#243381=CARTESIAN_POINT('Ctrl Pts',(7.86601130906456,-0.330583112720854,
83.1339000696561));
#243382=CARTESIAN_POINT('Ctrl Pts',(7.04994712015195,3.46650843499095,83.292854435481));
#243383=CARTESIAN_POINT('Ctrl Pts',(3.70681288487125,7.44684299163876,83.5047935899139));
#243384=CARTESIAN_POINT('Ctrl Pts',(-3.33648429528967,8.27951252852172,
83.7697175329551));
#243385=CARTESIAN_POINT('Ctrl Pts',(-8.77939149375497,1.65037161641574,
84.0876262646048));
#243386=CARTESIAN_POINT('Ctrl Pts',(-6.56715245437637,-5.10547863939855,
84.352550207646));
#243387=CARTESIAN_POINT('Ctrl Pts',(-2.02108893729002,-7.58348625226029,
84.564489362079));
#243388=CARTESIAN_POINT('Ctrl Pts',(3.18083270483377,-7.6934249080082,84.776428516512));
#243389=CARTESIAN_POINT('Ctrl Pts',(7.36106071721383,-3.88417062830127,
84.988367670945));
#243390=CARTESIAN_POINT('Ctrl Pts',(7.74547325076561,1.31382353469886,85.2003068253781));
#243391=CARTESIAN_POINT('Ctrl Pts',(6.19054403142093,4.86421460297602,85.3592611912026));
#243392=CARTESIAN_POINT('Ctrl Pts',(3.10131785134482,7.21805117131482,85.5182155570277));
#243393=CARTESIAN_POINT('Ctrl Pts',(-2.02680911194038,8.06771201328684,
85.7301547114604));
#243394=CARTESIAN_POINT('Ctrl Pts',(-7.91887496461385,4.11993622007326,
85.9950786545018));
#243395=CARTESIAN_POINT('Ctrl Pts',(-7.7426824191354,-4.45559316245293,
86.3129873861515));
#243396=CARTESIAN_POINT('Ctrl Pts',(-1.66871464606686,-8.1491591545619,
86.5779113291926));
#243397=CARTESIAN_POINT('Ctrl Pts',(3.39626131844057,-7.07527195855542,
86.7898504836257));
#243398=CARTESIAN_POINT('Ctrl Pts',(7.41949250519753,-3.77592564500659,
87.0017896380585));
#243399=CARTESIAN_POINT('Ctrl Pts',(8.11788347494936,1.83629089182822,87.2137287924919));
#243400=CARTESIAN_POINT('Ctrl Pts',(5.02960044991658,6.03503168780853,87.4256679469244));
#243401=CARTESIAN_POINT('Ctrl Pts',(1.53951351256144,7.72096608290747,87.5846223127496));
#243402=CARTESIAN_POINT('Ctrl Pts',(-2.33799904538993,7.50014637127467,
87.7435766785741));
#243403=CARTESIAN_POINT('Ctrl Pts',(-6.78621968890966,4.8107332746091,87.9555158330073));
#243404=CARTESIAN_POINT('Ctrl Pts',(-8.69495828245439,-2.01993951123245,
88.2204397760485));
#243405=CARTESIAN_POINT('Ctrl Pts',(-2.98435516720558,-8.41992076618659,
88.538348507698));
#243406=CARTESIAN_POINT('Ctrl Pts',(4.03181195051564,-7.2758433114009,88.8032724507394));
#243407=CARTESIAN_POINT('Ctrl Pts',(7.18115564050557,-3.16623876192109,
89.0152116051722));
#243408=CARTESIAN_POINT('Ctrl Pts',(8.0918794457162,1.95652000942912,89.2271507596054));
#243409=CARTESIAN_POINT('Ctrl Pts',(4.97274292511143,6.67411598288644,89.4390899140382));
#243410=CARTESIAN_POINT('Ctrl Pts',(-0.103813384613165,7.85542557343836,
89.6510290684714));
#243411=CARTESIAN_POINT('Ctrl Pts',(-3.85150363656501,6.86653761704497,
89.809983434296));
#243412=CARTESIAN_POINT('Ctrl Pts',(-6.653527147126,4.17720141114196,89.9689378001209));
#243413=CARTESIAN_POINT('Ctrl Pts',(-8.28374799016402,-0.758585223314343,
90.1808769545537));
#243414=CARTESIAN_POINT('Ctrl Pts',(-5.29169999189226,-7.18890578311246,
90.4458008975953));
#243415=CARTESIAN_POINT('Ctrl Pts',(3.20844012003686,-8.3371070203653,90.7637096292446));
#243416=CARTESIAN_POINT('Ctrl Pts',(7.79439716835156,-2.90530140921238,
91.0286335722861));
#243417=CARTESIAN_POINT('Ctrl Pts',(7.51433672947288,2.2646871189528,91.2405727267189));
#243418=CARTESIAN_POINT('Ctrl Pts',(4.87480224402012,6.74853958964436,91.452511881152));
#243419=CARTESIAN_POINT('Ctrl Pts',(-0.562609370393717,8.30394286159366,
91.664451035585));
#243420=CARTESIAN_POINT('Ctrl Pts',(-5.18732800355999,5.90000985949486,
91.876390190018));
#243421=CARTESIAN_POINT('Ctrl Pts',(-7.39124687725992,2.7116210480379,92.0353445558428));
#243422=CARTESIAN_POINT('Ctrl Pts',(-7.7709533206754,-1.15356820980508,
92.1942989216675));
#243423=CARTESIAN_POINT('Ctrl Pts',(-5.79958810797117,-5.96328014463993,
92.4062380761006));
#243424=CARTESIAN_POINT('Ctrl Pts',(0.65508079031038,-8.90243361788374,
92.6711620191416));
#243425=CARTESIAN_POINT('Ctrl Pts',(7.85905810680846,-4.24695739873778,
92.9890707507916));
#243426=CARTESIAN_POINT('Ctrl Pts',(7.81050686095784,2.8617103402176,93.2539946938323));
#243427=CARTESIAN_POINT('Ctrl Pts',(4.23565688330435,6.60706250898031,93.4659338482658));
#243428=CARTESIAN_POINT('Ctrl Pts',(-0.685410276942486,8.29678831015729,
93.6778730026984));
#243429=CARTESIAN_POINT('Ctrl Pts',(-5.82753636026967,5.94237463662472,
93.8898121571318));
#243430=CARTESIAN_POINT('Ctrl Pts',(-7.77748784638796,1.1086798266145,94.1017513115646));
#243431=CARTESIAN_POINT('Ctrl Pts',(-7.37829387622094,-2.74667045436609,
94.2607056773893));
#243432=CARTESIAN_POINT('Ctrl Pts',(-5.15317255072635,-5.92986068885513,
94.4196600432142));
#243433=CARTESIAN_POINT('Ctrl Pts',(-0.527782891107564,-8.30164908469586,
94.6315991976472));
#243434=CARTESIAN_POINT('Ctrl Pts',(6.28698871000212,-6.33689420165481,
94.8965231406882));
#243435=CARTESIAN_POINT('Ctrl Pts',(8.73212047092496,1.88454598090315,95.2144318723381));
#243436=CARTESIAN_POINT('Ctrl Pts',(4.07239770094658,7.25320484073779,95.4793558153791));
#243437=CARTESIAN_POINT('Ctrl Pts',(-1.07894498528856,7.77366978648934,
95.6912949698123));
#243438=CARTESIAN_POINT('Ctrl Pts',(-5.91617168425987,5.85708085258035,
95.903234124245));
#243439=CARTESIAN_POINT('Ctrl Pts',(-8.29138433472371,0.724528927072806,
96.1151732786783));
#243440=CARTESIAN_POINT('Ctrl Pts',(-6.62929984333307,-4.21555117936412,
96.3271124331113));
#243441=CARTESIAN_POINT('Ctrl Pts',(-3.81887065713178,-6.88474008317412,
96.4860667989358));
#243442=CARTESIAN_POINT('Ctrl Pts',(-0.0584542548102956,-7.85589067050221,
96.6450211647609));
#243443=CARTESIAN_POINT('Ctrl Pts',(4.99770784388671,-6.64972545393648,
96.8569603191938));
#243444=CARTESIAN_POINT('Ctrl Pts',(8.89697603459555,-0.725446484926773,
97.1218842622352));
#243445=CARTESIAN_POINT('Ctrl Pts',(5.40797875099621,7.11021851293324,97.4397929938846));
#243446=CARTESIAN_POINT('Ctrl Pts',(-1.62316089178656,8.15835474932004,
97.7047169369258));
#243447=CARTESIAN_POINT('Ctrl Pts',(-5.87493830813479,5.20376441686851,
97.916656091359));
#243448=CARTESIAN_POINT('Ctrl Pts',(-8.30325038727105,0.602093445890282,
98.1285952457918));
#243449=CARTESIAN_POINT('Ctrl Pts',(-6.76987362018956,-4.84157076979441,
98.340534400225));
#243450=CARTESIAN_POINT('Ctrl Pts',(-2.29465507190867,-7.51352422366614,
98.5524735546578));
#243451=CARTESIAN_POINT('Ctrl Pts',(1.57614101632218,-7.71357236340167,
98.7114279204827));
#243452=CARTESIAN_POINT('Ctrl Pts',(5.06436081758022,-6.00588749779308,
98.8703822863075));
#243453=CARTESIAN_POINT('Ctrl Pts',(8.12098712943168,-1.80152722687786,
99.0823214407404));
#243454=CARTESIAN_POINT('Ctrl Pts',(7.23051936458366,5.23469625489779,99.3472453837818));
#243455=CARTESIAN_POINT('Ctrl Pts',(-0.515576315975734,8.91827463892484,
99.6651541154311));
#243456=CARTESIAN_POINT('Ctrl Pts',(-6.53852668407044,5.14208832071911,
99.9300780584726));
#243457=CARTESIAN_POINT('Ctrl Pts',(-7.8470682701258,0.132603901305477,
100.142017212906));
#243458=CARTESIAN_POINT('Ctrl Pts',(-6.69926683314272,-4.94229778642039,
100.353956367339));
#243459=CARTESIAN_POINT('Ctrl Pts',(-1.99433757449542,-8.08050827554942,
100.565895521772));
#243460=CARTESIAN_POINT('Ctrl Pts',(3.14294466576488,-7.2000268740189,100.777834676205));
#243461=CARTESIAN_POINT('Ctrl Pts',(6.21356058683115,-4.83477858257698,
100.93678904203));
#243462=CARTESIAN_POINT('Ctrl Pts',(7.75292684617862,-1.26907858093652,
101.095743407854));
#243463=CARTESIAN_POINT('Ctrl Pts',(7.34081129664397,3.912597834258,101.307682562287));
#243464=CARTESIAN_POINT('Ctrl Pts',(2.08862216350653,8.67871606983256,101.572606505329));
#243465=CARTESIAN_POINT('Ctrl Pts',(-6.19131310945317,6.43964932691215,
101.890515236978));
#243466=CARTESIAN_POINT('Ctrl Pts',(-8.31106697441633,-0.345787858584055,
102.155439180019));
#243467=CARTESIAN_POINT('Ctrl Pts',(-6.04740567602245,-5.00229435562004,
102.367378334452));
#243468=CARTESIAN_POINT('Ctrl Pts',(-1.87519599256411,-8.11111111382233,
102.579317488886));
#243469=CARTESIAN_POINT('Ctrl Pts',(3.73980203610677,-7.43544733576923,
102.791256643318));
#243470=CARTESIAN_POINT('Ctrl Pts',(7.06984832096886,-3.42574559434119,
103.003195797751));
#243471=CARTESIAN_POINT('Ctrl Pts',(7.86435371782322,0.36791263871619,103.162150163576));
#243472=CARTESIAN_POINT('Ctrl Pts',(6.71495058411182,4.07772899782774,103.321104529401));
#243473=CARTESIAN_POINT('Ctrl Pts',(3.0321817214842,7.74608328857064,103.533043683834));
#243474=CARTESIAN_POINT('Ctrl Pts',(-4.05719768200587,7.95120130117371,
103.797967626875));
#243475=CARTESIAN_POINT('Ctrl Pts',(-8.89111699463826,0.865725164553574,
104.115876358525));
#243476=CARTESIAN_POINT('Ctrl Pts',(-6.08878786620442,-5.66745673267461,
104.380800301566));
#243477=CARTESIAN_POINT('Ctrl Pts',(-1.34098110058904,-7.73277659825497,
104.592739455999));
#243478=CARTESIAN_POINT('Ctrl Pts',(3.85021150553996,-7.38121635463353,
104.804678610432));
#243479=CARTESIAN_POINT('Ctrl Pts',(7.67635852451879,-3.21644464515006,
105.016617764865));
#243480=CARTESIAN_POINT('Ctrl Pts',(7.59854001320767,1.99516360891437,105.228556919298));
#243481=CARTESIAN_POINT('Ctrl Pts',(5.73504582378576,5.39376199955503,105.387511285123));
#243482=CARTESIAN_POINT('Ctrl Pts',(2.44934844243884,7.46452458863333,105.546465650948));
#243483=CARTESIAN_POINT('Ctrl Pts',(-2.73390432686058,7.85631589468939,
105.758404805381));
#243484=CARTESIAN_POINT('Ctrl Pts',(-8.25287417603857,3.40184111873792,
106.023328748422));
#243485=CARTESIAN_POINT('Ctrl Pts',(-7.31729310683559,-5.12432074147813,
106.341237480071));
#243486=CARTESIAN_POINT('Ctrl Pts',(-0.939855903853375,-8.26499088785765,
106.606161423113));
#243487=CARTESIAN_POINT('Ctrl Pts',(4.01000299171803,-6.7464020216015,106.818100577546));
#243488=CARTESIAN_POINT('Ctrl Pts',(7.72496617432305,-3.10344665120341,
107.030039731979));
#243489=CARTESIAN_POINT('Ctrl Pts',(7.92317625394474,2.54858282211741,107.241978886412));
#243490=CARTESIAN_POINT('Ctrl Pts',(4.47489739759916,6.45707220337623,107.453918040845));
#243491=CARTESIAN_POINT('Ctrl Pts',(0.849115659828287,7.82703147463972,
107.612872406669));
#243492=CARTESIAN_POINT('Ctrl Pts',(-2.99356398945314,7.26340207945554,
107.771826772494));
#243493=CARTESIAN_POINT('Ctrl Pts',(-7.18590470216688,4.19031095707143,
107.983765926927));
#243494=CARTESIAN_POINT('Ctrl Pts',(-8.48170237564872,-2.78265699890864,
108.248689869968));
#243495=CARTESIAN_POINT('Ctrl Pts',(-2.22631979187741,-8.65129710836367,
108.566598601618));
#243496=CARTESIAN_POINT('Ctrl Pts',(4.6608296790759,-6.88985269791904,108.831522544659));
#243497=CARTESIAN_POINT('Ctrl Pts',(7.4335284570037,-2.51728403434591,109.043461699092));
#243498=CARTESIAN_POINT('Ctrl Pts',(7.88661820280942,2.66603391471617,109.255400853525));
#243499=CARTESIAN_POINT('Ctrl Pts',(4.36161916279933,7.08860174018598,109.467340007958));
#243500=CARTESIAN_POINT('Ctrl Pts',(-0.799661217785712,7.81530742168362,
109.679279162391));
#243501=CARTESIAN_POINT('Ctrl Pts',(-4.44495267940158,6.49813933265885,
109.838233528216));
#243502=CARTESIAN_POINT('Ctrl Pts',(-6.99758204921451,3.5710335466501,109.997187894041));
#243503=CARTESIAN_POINT('Ctrl Pts',(-8.18390914785682,-1.48981991032531,
110.209127048474));
#243504=CARTESIAN_POINT('Ctrl Pts',(-4.63369311415609,-7.62963585543128,
110.474050991515));
#243505=CARTESIAN_POINT('Ctrl Pts',(3.93476227318016,-8.01991816207902,
110.791959723165));
#243506=CARTESIAN_POINT('Ctrl Pts',(8.02122856083205,-2.20301971649602,
111.056883666206));
#243507=CARTESIAN_POINT('Ctrl Pts',(7.28403450478502,2.92179834412948,111.268822820639));
#243508=CARTESIAN_POINT('Ctrl Pts',(4.25746750011996,7.15405157912097,111.480761975072));
#243509=CARTESIAN_POINT('Ctrl Pts',(-1.29640531265514,8.22139462728711,
111.692701129505));
#243510=CARTESIAN_POINT('Ctrl Pts',(-5.68985256060279,5.41701633717821,
111.904640283938));
#243511=CARTESIAN_POINT('Ctrl Pts',(-7.60249832617733,2.04583437971828,
112.063594649763));
#243512=CARTESIAN_POINT('Ctrl Pts',(-7.63812384302203,-1.83779740054446,
112.222549015588));
#243513=CARTESIAN_POINT('Ctrl Pts',(-5.24821421168279,-6.45385000552909,
112.43448817002));
#243514=CARTESIAN_POINT('Ctrl Pts',(1.44155931555731,-8.80933379446994,
112.699412113062));
#243515=CARTESIAN_POINT('Ctrl Pts',(8.20455111367348,-3.53366417419736,
113.017320844711));
#243516=CARTESIAN_POINT('Ctrl Pts',(7.52612254126613,3.54272253926597,113.282244787752));
#243517=CARTESIAN_POINT('Ctrl Pts',(3.63337729289704,6.95648141506293,113.494183942186));
#243518=CARTESIAN_POINT('Ctrl Pts',(-1.41808877366636,8.20338392014562,
113.706123096618));
#243519=CARTESIAN_POINT('Ctrl Pts',(-6.3312961871736,5.40247026299526,113.918062251052));
#243520=CARTESIAN_POINT('Ctrl Pts',(-7.84514434672058,0.414967875590241,
114.130001405485));
#243521=CARTESIAN_POINT('Ctrl Pts',(-7.10580705194119,-3.3898267285143,
114.28895577131));
#243522=CARTESIAN_POINT('Ctrl Pts',(-4.60730486081632,-6.36326779621038,
114.447910137134));
#243523=CARTESIAN_POINT('Ctrl Pts',(0.210101226185732,-8.31575551470409,
114.659849291567));
#243524=CARTESIAN_POINT('Ctrl Pts',(6.82390803799858,-5.75471408947469,
114.924773234609));
#243525=CARTESIAN_POINT('Ctrl Pts',(8.53071875050506,2.65109016683102,115.242681966258));
#243526=CARTESIAN_POINT('Ctrl Pts',(3.41349058714555,7.58561042420752,115.507605909299));
#243527=CARTESIAN_POINT('Ctrl Pts',(-1.76370864307955,7.64744375938669,
115.719545063732));
#243528=CARTESIAN_POINT('Ctrl Pts',(-6.41202275282373,5.30965608383186,
115.931484218165));
#243529=CARTESIAN_POINT('Ctrl Pts',(-8.32296951761604,-0.0132197239513161,
116.143423372598));
#243530=CARTESIAN_POINT('Ctrl Pts',(-6.22956833484834,-4.78654014086465,
116.355362527031));
#243531=CARTESIAN_POINT('Ctrl Pts',(-3.19361979615618,-7.19612477006659,
116.514316892856));
#243532=CARTESIAN_POINT('Ctrl Pts',(0.638073442077508,-7.83015308977449,
116.673271258681));
#243533=CARTESIAN_POINT('Ctrl Pts',(5.56742885387138,-6.18058801916594,
116.885210413114));
#243534=CARTESIAN_POINT('Ctrl Pts',(8.92625910332977,0.065981685964151,
117.150134356155));
#243535=CARTESIAN_POINT('Ctrl Pts',(4.75648858606023,7.5615645076641,117.468043087805));
#243536=CARTESIAN_POINT('Ctrl Pts',(-2.3398787664328,7.98237877169294,117.732967030846));
#243537=CARTESIAN_POINT('Ctrl Pts',(-6.31304572533293,4.66256559208677,
117.944906185279));
#243538=CARTESIAN_POINT('Ctrl Pts',(-8.32393694368881,-0.136225066689908,
118.156845339712));
#243539=CARTESIAN_POINT('Ctrl Pts',(-6.31410234165591,-5.42255548347479,
118.368784494145));
#243540=CARTESIAN_POINT('Ctrl Pts',(-1.61967155702648,-7.68733713362521,
118.580723648578));
#243541=CARTESIAN_POINT('Ctrl Pts',(2.25362118408763,-7.5435144771783,118.739678014403));
#243542=CARTESIAN_POINT('Ctrl Pts',(5.57675367937275,-5.53337632249897,
118.898632380228));
#243543=CARTESIAN_POINT('Ctrl Pts',(8.24870142701377,-1.0746427655538,119.11057153466));
#243544=CARTESIAN_POINT('Ctrl Pts',(6.73809089691147,5.85496252999263,119.375495477702));
#243545=CARTESIAN_POINT('Ctrl Pts',(-1.30400794239072,8.83747728478373,
119.693404209351));
#243546=CARTESIAN_POINT('Ctrl Pts',(-6.96855581333222,4.54231586009295,
119.958328152393));
#243547=CARTESIAN_POINT('Ctrl Pts',(-7.82793757869164,-0.56343366491826,
120.170267306826));
#243548=CARTESIAN_POINT('Ctrl Pts',(-6.23484562258053,-5.51662791693352,
120.382206461258));
#243549=CARTESIAN_POINT('Ctrl Pts',(-1.27028206080914,-8.22547140522983,
120.594145615692));
#243550=CARTESIAN_POINT('Ctrl Pts',(3.76874082838451,-6.89311836015612,
120.806084770125));
#243551=CARTESIAN_POINT('Ctrl Pts',(6.61763065495857,-4.26501859589367,
120.965039135949));
#243552=CARTESIAN_POINT('Ctrl Pts',(7.83489676687533,-0.576912280330592,
121.123993501774));
#243553=CARTESIAN_POINT('Ctrl Pts',(6.96513139029871,4.54784311750666,121.335932656207));
#243554=CARTESIAN_POINT('Ctrl Pts',(1.31117412703128,8.82968162343708,121.600856599248));
#243555=CARTESIAN_POINT('Ctrl Pts',(-6.73771656982127,5.86554489349819,
121.918765330898));
#243556=CARTESIAN_POINT('Ctrl Pts',(-8.24770842146538,-1.08106858749443,
122.183689273939));
#243557=CARTESIAN_POINT('Ctrl Pts',(-5.58023228461821,-5.5186114087115,
122.395628428372));
#243558=CARTESIAN_POINT('Ctrl Pts',(-1.14889694046579,-8.2453938251299,
122.607567582805));
#243559=CARTESIAN_POINT('Ctrl Pts',(4.3841153497589,-7.07471052074045,122.819506737238));
#243560=CARTESIAN_POINT('Ctrl Pts',(7.34566029529158,-2.78563511336829,
123.031445891671));
#243561=CARTESIAN_POINT('Ctrl Pts',(7.80079230035837,1.06351238612278,123.190400257496));
#243562=CARTESIAN_POINT('Ctrl Pts',(6.32709768517662,4.65685194192624,123.349354623321));
#243563=CARTESIAN_POINT('Ctrl Pts',(2.33368290703505,7.98435071843594,123.561293777754));
#243564=CARTESIAN_POINT('Ctrl Pts',(-4.74597506110222,7.56030263164477,
123.826217720795));
#243565=CARTESIAN_POINT('Ctrl Pts',(-8.9328565588375,0.0742642048415293,
124.144126452445));
#243566=CARTESIAN_POINT('Ctrl Pts',(-5.5624957204101,-6.1848237530909,124.409050395486));
#243567=CARTESIAN_POINT('Ctrl Pts',(-0.650317805169212,-7.82119882006179,
124.620989549919));
#243568=CARTESIAN_POINT('Ctrl Pts',(4.48928357889013,-7.0109069641245,124.832928704352));
#243569=CARTESIAN_POINT('Ctrl Pts',(7.9312322993893,-2.52340059550421,125.044867858785));
#243570=CARTESIAN_POINT('Ctrl Pts',(7.39179528733201,2.66079886290376,125.256807013218));
#243571=CARTESIAN_POINT('Ctrl Pts',(5.2344045194909,5.88085269625925,125.415761379043));
#243572=CARTESIAN_POINT('Ctrl Pts',(1.77809912245857,7.65224141265171,125.574715744867));
#243573=CARTESIAN_POINT('Ctrl Pts',(-3.41947976476801,7.58307921915096,
125.7866548993));
#243574=CARTESIAN_POINT('Ctrl Pts',(-8.52191134389828,2.65696861279858,
126.051578842342));
#243575=CARTESIAN_POINT('Ctrl Pts',(-6.83430612571826,-5.75271251262015,
126.369487573991));
#243576=CARTESIAN_POINT('Ctrl Pts',(-0.203599137767642,-8.31576520156013,
126.634411517033));
#243577=CARTESIAN_POINT('Ctrl Pts',(4.59218014777536,-6.36442815349768,
126.846350671465));
#243578=CARTESIAN_POINT('Ctrl Pts',(7.9696331985815,-2.40653904837824,127.058289825898));
#243579=CARTESIAN_POINT('Ctrl Pts',(7.66610218837164,3.24081372338967,127.270228980331));
#243580=CARTESIAN_POINT('Ctrl Pts',(3.88497043740519,6.82828623148893,127.482168134765));
#243581=CARTESIAN_POINT('Ctrl Pts',(0.152034040044715,7.87148682012707,
127.641122500589));
#243582=CARTESIAN_POINT('Ctrl Pts',(-3.62556525980116,6.96948431906636,
127.800076866414));
#243583=CARTESIAN_POINT('Ctrl Pts',(-7.52902626318211,3.5369048381165,128.012016020847));
#243584=CARTESIAN_POINT('Ctrl Pts',(-8.20168321673487,-3.52347095560442,
128.276939963888));
#243585=CARTESIAN_POINT('Ctrl Pts',(-1.45076006318804,-8.81457524285472,
128.594848695538));
#243586=CARTESIAN_POINT('Ctrl Pts',(5.25315994406895,-6.44962898920616,
128.859772638579));
#243587=CARTESIAN_POINT('Ctrl Pts',(7.62738866454065,-1.84851464443432,
129.071711793012));
#243588=CARTESIAN_POINT('Ctrl Pts',(7.61927788001662,3.354562281194,129.283650947445));
#243589=CARTESIAN_POINT('Ctrl Pts',(3.71616315598209,7.44728996013693,129.495590101878));
#243590=CARTESIAN_POINT('Ctrl Pts',(-1.48921456181703,7.71367150892115,
129.707529256311));
#243591=CARTESIAN_POINT('Ctrl Pts',(-5.00341352256318,6.07859130317289,
129.866483622136));
#243592=CARTESIAN_POINT('Ctrl Pts',(-7.28655587042038,2.93675648870235,
130.025437987961));
#243593=CARTESIAN_POINT('Ctrl Pts',(-8.01965111641687,-2.20932756215386,
130.237377142394));
#243594=CARTESIAN_POINT('Ctrl Pts',(-3.93921237678579,-8.01030967020114,
130.502301085435));
#243595=CARTESIAN_POINT('Ctrl Pts',(4.63011216219744,-7.63960096067819,
130.820209817085));
#243596=CARTESIAN_POINT('Ctrl Pts',(8.18492129553836,-1.48339707560108,
131.085133760126));
#243597=CARTESIAN_POINT('Ctrl Pts',(6.99639640437534,3.5559107948077,131.297072914559));
#243598=CARTESIAN_POINT('Ctrl Pts',(3.60662033617928,7.50325084671076,131.509012068992));
#243599=CARTESIAN_POINT('Ctrl Pts',(-2.01999667286217,8.07413213842702,
131.720951223425));
#243600=CARTESIAN_POINT('Ctrl Pts',(-6.14758975626172,4.89138307039339,
131.932890377858));
#243601=CARTESIAN_POINT('Ctrl Pts',(-7.75390713121773,1.36394403766155,
132.091844743683));
#243602=CARTESIAN_POINT('Ctrl Pts',(-7.44517129132054,-2.50756046804626,
132.250799109507));
#243603=CARTESIAN_POINT('Ctrl Pts',(-4.65552929510624,-6.89361874757744,
132.46273826394));
#243604=CARTESIAN_POINT('Ctrl Pts',(2.21669070319618,-8.64689177543339,
132.727662206981));
#243605=CARTESIAN_POINT('Ctrl Pts',(8.48546241963345,-2.79255592616151,
133.045570938631));
#243606=CARTESIAN_POINT('Ctrl Pts',(7.18249681313266,4.19584842527409,133.310494881672));
#243607=CARTESIAN_POINT('Ctrl Pts',(3.00249770744235,7.25114271918739,133.522434036105));
#243608=CARTESIAN_POINT('Ctrl Pts',(-2.13960469233783,8.04540715571849,
133.734373190538));
#243609=CARTESIAN_POINT('Ctrl Pts',(-6.78521991235738,4.82004042056871,
133.946312344972));
#243610=CARTESIAN_POINT('Ctrl Pts',(-7.85104779783532,-0.282010197456314,
134.158251499404));
#243611=CARTESIAN_POINT('Ctrl Pts',(-6.7773881513071,-4.00630074029798,
134.317205865229));
#243612=CARTESIAN_POINT('Ctrl Pts',(-4.02516939863429,-6.74658574968469,
134.476160231054));
#243613=CARTESIAN_POINT('Ctrl Pts',(0.946328029323823,-8.26440718691397,
134.688099385487));
#243614=CARTESIAN_POINT('Ctrl Pts',(7.3071206196513,-5.12723140280613,134.953023328528));
#243615=CARTESIAN_POINT('Ctrl Pts',(8.26215525051097,3.39675830243544,135.270932060178));
#243616=CARTESIAN_POINT('Ctrl Pts',(2.72773566717734,7.85831994690357,135.535856003219));
#243617=CARTESIAN_POINT('Ctrl Pts',(-2.43461772017353,7.46100312305416,
135.747795157652));
#243618=CARTESIAN_POINT('Ctrl Pts',(-6.85732892337842,4.72048345925153,
135.959734312085));
#243619=CARTESIAN_POINT('Ctrl Pts',(-8.28918936827278,-0.750959494552329,
136.171673466518));
#243620=CARTESIAN_POINT('Ctrl Pts',(-5.78061766663374,-5.31973450400921,
136.383612620951));
#243621=CARTESIAN_POINT('Ctrl Pts',(-2.54361228342804,-7.45111029376608,
136.542566986776));
#243622=CARTESIAN_POINT('Ctrl Pts',(1.33027488604519,-7.74233449640139,
136.701521352601));
#243623=CARTESIAN_POINT('Ctrl Pts',(6.09182165394096,-5.66376494878866,
136.913460507034));
#243624=CARTESIAN_POINT('Ctrl Pts',(8.88839239521778,0.858886091611861,
137.178384450075));
#243625=CARTESIAN_POINT('Ctrl Pts',(4.06211791741203,7.94990226154086,137.496293181724));
#243626=CARTESIAN_POINT('Ctrl Pts',(-3.02903681086098,7.74943205644144,
137.761217124766));
#243627=CARTESIAN_POINT('Ctrl Pts',(-6.71376182331183,4.07676873453249,
137.973156279199));
#243628=CARTESIAN_POINT('Ctrl Pts',(-7.86223692601581,0.380613488742994,
138.132110645024));
#243629=CARTESIAN_POINT('Ctrl Pts',(-7.07532856755501,-3.44087378386772,
138.291071725379));
#243630=CARTESIAN_POINT('Ctrl Pts',(-5.40397330502272,-5.41520356564519,
138.397048017128));
#243631=CARTESIAN_POINT('Ctrl Pts',(-4.38104157308948,-6.14454874685667,
138.450039520268));
#243632=CARTESIAN_POINT('Ctrl Pts',(-3.43252346058927,7.15950580248449,
8.01661173253155));
#243633=CARTESIAN_POINT('Ctrl Pts',(-4.62447820848135,6.58804200029991,
8.06960567665085));
#243634=CARTESIAN_POINT('Ctrl Pts',(-6.71314905678031,4.84304631147434,
8.17558440937839));
#243635=CARTESIAN_POINT('Ctrl Pts',(-8.21822261919714,1.02380062502623,
8.33454793071417));
#243636=CARTESIAN_POINT('Ctrl Pts',(-7.69455181722148,-3.01461142521582,
8.49350229653894));
#243637=CARTESIAN_POINT('Ctrl Pts',(-4.53770639023232,-7.48620479461186,
8.70544145097195));
#243638=CARTESIAN_POINT('Ctrl Pts',(2.77642922983875,-8.97322384561435,
8.97036539401322));
#243639=CARTESIAN_POINT('Ctrl Pts',(9.05827682897998,-2.49371283586009,
9.28827412566274));
#243640=CARTESIAN_POINT('Ctrl Pts',(7.3361722235595,4.77180027059814,9.553198068704));
#243641=CARTESIAN_POINT('Ctrl Pts',(2.77558310671645,7.78529932770683,9.76513722313702));
#243642=CARTESIAN_POINT('Ctrl Pts',(-1.29241060276714,8.18226981884739,
9.92409158896177));
#243643=CARTESIAN_POINT('Ctrl Pts',(-5.03220552019797,6.55694914733997,
10.0830459547865));
#243644=CARTESIAN_POINT('Ctrl Pts',(-8.45664565315574,2.2737476794153,10.2949851092195));
#243645=CARTESIAN_POINT('Ctrl Pts',(-7.95948972768491,-3.65595153354138,
10.5069242636526));
#243646=CARTESIAN_POINT('Ctrl Pts',(-3.8695326494975,-7.29446666417152,
10.7188634180856));
#243647=CARTESIAN_POINT('Ctrl Pts',(1.40980336588385,-8.6375761801721,10.9308025725186));
#243648=CARTESIAN_POINT('Ctrl Pts',(7.9513295390695,-5.01135990549878,11.1957265155599));
#243649=CARTESIAN_POINT('Ctrl Pts',(8.49909507792882,3.99642296432439,11.5136352472094));
#243650=CARTESIAN_POINT('Ctrl Pts',(2.47178529580885,8.39571392291258,11.7785591902507));
#243651=CARTESIAN_POINT('Ctrl Pts',(-2.95520506366149,7.71926692580053,
11.9904983446837));
#243652=CARTESIAN_POINT('Ctrl Pts',(-6.30234226822578,5.37533051525002,
12.1494527105084));
#243653=CARTESIAN_POINT('Ctrl Pts',(-8.08708929324349,1.70862130233454,
12.3084070763332));
#243654=CARTESIAN_POINT('Ctrl Pts',(-7.90270527679653,-3.77215503370355,
12.5203462307662));
#243655=CARTESIAN_POINT('Ctrl Pts',(-3.66916312400431,-7.9534470987693,
12.7322853851992));
#243656=CARTESIAN_POINT('Ctrl Pts',(1.80413946140186,-8.0577759930288,12.9442245396322));
#243657=CARTESIAN_POINT('Ctrl Pts',(6.68806173624078,-5.64488555735922,
13.1561636940653));
#243658=CARTESIAN_POINT('Ctrl Pts',(9.2993308505076,1.36385788062776,13.4210876371065));
#243659=CARTESIAN_POINT('Ctrl Pts',(3.85757222238032,8.56300679553197,13.738996368756));
#243660=CARTESIAN_POINT('Ctrl Pts',(-3.58207705629457,7.98538822446524,
14.0039203117973));
#243661=CARTESIAN_POINT('Ctrl Pts',(-7.26489761136101,3.94228506414547,
14.2158594662303));
#243662=CARTESIAN_POINT('Ctrl Pts',(-8.28332376272661,-0.015007944899706,
14.374813832055));
#243663=CARTESIAN_POINT('Ctrl Pts',(-7.25464302603574,-3.96113142541196,
14.5337681978798));
#243664=CARTESIAN_POINT('Ctrl Pts',(-3.55036594805974,-8.00479875340866,
14.7457073523128));
#243665=CARTESIAN_POINT('Ctrl Pts',(2.38486011653395,-8.42807925187489,
14.9576465067459));
#243666=CARTESIAN_POINT('Ctrl Pts',(6.61060311566235,-4.94798956303239,
15.1695856611789));
#243667=CARTESIAN_POINT('Ctrl Pts',(8.7516382340282,0.0610727336051463,
15.3815248156119));
#243668=CARTESIAN_POINT('Ctrl Pts',(6.17747958716616,7.08353082689385,15.6464487586532));
#243669=CARTESIAN_POINT('Ctrl Pts',(-2.63813481369485,9.01366704844546,
15.9643574903027));
#243670=CARTESIAN_POINT('Ctrl Pts',(-7.91417201601133,3.73678769388132,
16.2292814333439));
#243671=CARTESIAN_POINT('Ctrl Pts',(-8.08262379672163,-1.72960731590742,
16.441220587777));
#243672=CARTESIAN_POINT('Ctrl Pts',(-6.28282180227127,-5.39813189592084,
16.6001749536017));
#243673=CARTESIAN_POINT('Ctrl Pts',(-2.93516049174163,-7.72691662301371,
16.7591293194265));
#243674=CARTESIAN_POINT('Ctrl Pts',(2.50850133434887,-8.38983447446427,
16.9710684738595));
#243675=CARTESIAN_POINT('Ctrl Pts',(7.29257035236751,-4.85164871973294,
17.1830076282925));
#243676=CARTESIAN_POINT('Ctrl Pts',(8.23959675927419,0.540110652007771,
17.3949467827255));
#243677=CARTESIAN_POINT('Ctrl Pts',(6.60862923386289,5.73767560128377,17.6068859371585));
#243678=CARTESIAN_POINT('Ctrl Pts',(0.0863446456689102,9.39841516573596,
17.8718098801998));
#243679=CARTESIAN_POINT('Ctrl Pts',(-7.86578898824371,5.13179428160162,
18.1897186118493));
#243680=CARTESIAN_POINT('Ctrl Pts',(-8.44222016347028,-2.30794707028898,
18.4546425548906));
#243681=CARTESIAN_POINT('Ctrl Pts',(-5.01533468106842,-6.57014207940362,
18.6665817093236));
#243682=CARTESIAN_POINT('Ctrl Pts',(-1.262402125502,-8.18657551350801,18.8255360751483));
#243683=CARTESIAN_POINT('Ctrl Pts',(2.79514403616855,-7.77866167334332,
18.9844904409731));
#243684=CARTESIAN_POINT('Ctrl Pts',(7.36162574056733,-4.74219020170966,
19.1964295954061));
#243685=CARTESIAN_POINT('Ctrl Pts',(8.69501446585794,1.05678809721589,19.4083687498392));
#243686=CARTESIAN_POINT('Ctrl Pts',(5.90812406652453,5.76859985493989,19.6203079042721));
#243687=CARTESIAN_POINT('Ctrl Pts',(1.28909905516634,8.65639216314757,19.8322470587052));
#243688=CARTESIAN_POINT('Ctrl Pts',(-6.04629294128532,7.19583245313094,
20.0971710017464));
#243689=CARTESIAN_POINT('Ctrl Pts',(-9.31265225685634,-1.21674027595255,
20.415079733396));
#243690=CARTESIAN_POINT('Ctrl Pts',(-4.91240847420854,-7.24333790115327,
20.6800036764372));
#243691=CARTESIAN_POINT('Ctrl Pts',(0.462638446148335,-8.252655001563,20.8919428308703));
#243692=CARTESIAN_POINT('Ctrl Pts',(4.3648070904711,-7.04003812687221,21.050897196695));
#243693=CARTESIAN_POINT('Ctrl Pts',(7.18192725065368,-4.09149466302802,
21.2098515625198));
#243694=CARTESIAN_POINT('Ctrl Pts',(8.67629167883199,1.18484773587382,21.4217907169528));
#243695=CARTESIAN_POINT('Ctrl Pts',(5.91808996568352,6.45726635674664,21.6337298713858));
#243696=CARTESIAN_POINT('Ctrl Pts',(0.736836858659884,8.22433861873278,
21.8456690258188));
#243697=CARTESIAN_POINT('Ctrl Pts',(-4.65005287944806,7.41430440935427,
22.0576081802518));
#243698=CARTESIAN_POINT('Ctrl Pts',(-9.27270339692655,1.53448191191556,
22.3225321232931));
#243699=CARTESIAN_POINT('Ctrl Pts',(-6.28327150021554,-6.98043323947992,
22.6404408549426));
#243700=CARTESIAN_POINT('Ctrl Pts',(0.978614444226989,-8.69712680931522,
22.9053647979839));
#243701=CARTESIAN_POINT('Ctrl Pts',(5.71823855617235,-5.96842497828208,
23.1173039524169));
#243702=CARTESIAN_POINT('Ctrl Pts',(7.89401660440229,-2.50961742388398,
23.2762583182416));
#243703=CARTESIAN_POINT('Ctrl Pts',(8.11662634786984,1.56230097623142,23.4352126840664));
#243704=CARTESIAN_POINT('Ctrl Pts',(5.82058834768326,6.54237363196179,23.6471518384994));
#243705=CARTESIAN_POINT('Ctrl Pts',(0.296560714988169,8.75397791785091,
23.8590909929324));
#243706=CARTESIAN_POINT('Ctrl Pts',(-4.7886202994179,6.72694506443021,24.0710301473655));
#243707=CARTESIAN_POINT('Ctrl Pts',(-8.35409811785603,2.60843751956376,
24.2829693017985));
#243708=CARTESIAN_POINT('Ctrl Pts',(-8.04207175181927,-4.86443675711376,
24.5478932448397));
#243709=CARTESIAN_POINT('Ctrl Pts',(-0.233756872348344,-9.3888927292246,
24.8658019764893));
#243710=CARTESIAN_POINT('Ctrl Pts',(6.39925395972027,-5.97053177922736,
25.1307259195305));
#243711=CARTESIAN_POINT('Ctrl Pts',(8.22529502190908,-0.815396044407385,
25.3426650739636));
#243712=CARTESIAN_POINT('Ctrl Pts',(7.62886725191158,3.22708261709433,25.5016194397883));
#243713=CARTESIAN_POINT('Ctrl Pts',(5.14996639153414,6.46515690276247,25.6605738056131));
#243714=CARTESIAN_POINT('Ctrl Pts',(0.167145651189453,8.75522494197968,
25.872512960046));
#243715=CARTESIAN_POINT('Ctrl Pts',(-5.46751419208695,6.84297933675263,
26.0844521144791));
#243716=CARTESIAN_POINT('Ctrl Pts',(-8.01236657929817,1.99616033193848,
26.296391268912));
#243717=CARTESIAN_POINT('Ctrl Pts',(-8.04264049467031,-3.4512078363557,
26.5083304233452));
#243718=CARTESIAN_POINT('Ctrl Pts',(-2.94591666217063,-8.92520240918457,
26.7732543663863));
#243719=CARTESIAN_POINT('Ctrl Pts',(5.9281159510523,-7.28446224694289,27.091163098036));
#243720=CARTESIAN_POINT('Ctrl Pts',(8.74401116873232,-0.374125178040082,
27.3560870410771));
#243721=CARTESIAN_POINT('Ctrl Pts',(6.77875946227417,4.72956330534926,27.5680261955102));
#243722=CARTESIAN_POINT('Ctrl Pts',(3.6968064209343,7.41264460573822,27.7269805613349));
#243723=CARTESIAN_POINT('Ctrl Pts',(-0.292090009824848,8.26045344018289,
27.8859349271598));
#243724=CARTESIAN_POINT('Ctrl Pts',(-5.56663771537859,6.7597667118843,28.0978740815927));
#243725=CARTESIAN_POINT('Ctrl Pts',(-8.6035592897919,1.6428162377245,28.3098132360258));
#243726=CARTESIAN_POINT('Ctrl Pts',(-7.38486758130208,-3.69410409686745,
28.5217523904587));
#243727=CARTESIAN_POINT('Ctrl Pts',(-3.86538605350254,-7.85198652021393,
28.7336915448917));
#243728=CARTESIAN_POINT('Ctrl Pts',(3.56623050945739,-8.69595670290421,
28.998615487933));
#243729=CARTESIAN_POINT('Ctrl Pts',(9.24056490732958,-1.67866290531658,
29.3165242195825));
#243730=CARTESIAN_POINT('Ctrl Pts',(6.88584887949192,5.40210941915832,29.5814481626238));
#243731=CARTESIAN_POINT('Ctrl Pts',(2.07392747915858,8.00119826762644,29.7933873170568));
#243732=CARTESIAN_POINT('Ctrl Pts',(-2.01217114630803,8.03522526397403,
29.9523416828816));
#243733=CARTESIAN_POINT('Ctrl Pts',(-5.59374965575332,6.08525861406302,
30.1112960487063));
#243734=CARTESIAN_POINT('Ctrl Pts',(-8.62474629812029,1.51514116386394,
30.3232352031394));
#243735=CARTESIAN_POINT('Ctrl Pts',(-7.60419486026038,-4.34698725223412,
30.5351743575724));
#243736=CARTESIAN_POINT('Ctrl Pts',(-3.20773863081272,-7.60875069563005,
30.7471135120054));
#243737=CARTESIAN_POINT('Ctrl Pts',(2.16981505528078,-8.4786086289031,30.9590526664384));
#243738=CARTESIAN_POINT('Ctrl Pts',(8.36422390723629,-4.28688948481131,
31.2239766094797));
#243739=CARTESIAN_POINT('Ctrl Pts',(8.11141953413463,4.7340069811436,31.5418853411291));
#243740=CARTESIAN_POINT('Ctrl Pts',(1.71791628470502,8.58175183785365,31.8068092841705));
#243741=CARTESIAN_POINT('Ctrl Pts',(-3.62776396260994,7.42695614220699,
32.0187484386034));
#243742=CARTESIAN_POINT('Ctrl Pts',(-6.7539732169225,4.79557332859529,32.1777028044282));
#243743=CARTESIAN_POINT('Ctrl Pts',(-8.2067028210019,0.985107313457929,
32.336657170253));
#243744=CARTESIAN_POINT('Ctrl Pts',(-7.53726155025489,-4.45775613693974,
32.548596324686));
#243745=CARTESIAN_POINT('Ctrl Pts',(-2.9497780491645,-8.24735637065377,
32.760535479119));
#243746=CARTESIAN_POINT('Ctrl Pts',(2.51123044048412,-7.86615509296918,
32.9724746335521));
#243747=CARTESIAN_POINT('Ctrl Pts',(7.16206712986657,-5.02988032496978,
33.184413787985));
#243748=CARTESIAN_POINT('Ctrl Pts',(9.14184735475931,2.18272535323379,33.4493377310263));
#243749=CARTESIAN_POINT('Ctrl Pts',(3.08341782822716,8.87121657118275,33.7672464626758));
#243750=CARTESIAN_POINT('Ctrl Pts',(-4.27575448790704,7.636466756747,34.0321704057171));
#243751=CARTESIAN_POINT('Ctrl Pts',(-7.58572479844854,3.28285366546854,
34.2441095601501));
#243752=CARTESIAN_POINT('Ctrl Pts',(-8.24939268619883,-0.749131546345857,
34.4030639259749));
#243753=CARTESIAN_POINT('Ctrl Pts',(-6.87500053726231,-4.58854826975936,
34.5620182917996));
#243754=CARTESIAN_POINT('Ctrl Pts',(-2.82689676236,-8.28797660157973,34.7739574462327));
#243755=CARTESIAN_POINT('Ctrl Pts',(3.12248686837969,-8.18352939755775,
34.9858966006656));
#243756=CARTESIAN_POINT('Ctrl Pts',(7.02314485697244,-4.34259261154448,
35.1978357550987));
#243757=CARTESIAN_POINT('Ctrl Pts',(8.71178110528462,0.836523538126509,
35.4097749095317));
#243758=CARTESIAN_POINT('Ctrl Pts',(5.52532631230719,7.60318565917569,35.674698852573));
#243759=CARTESIAN_POINT('Ctrl Pts',(-3.42666763322906,8.74436377832241,
35.9926075842225));
#243760=CARTESIAN_POINT('Ctrl Pts',(-8.21422981758254,3.02061739909196,
36.2575315272637));
#243761=CARTESIAN_POINT('Ctrl Pts',(-7.89751112140635,-2.43919392298781,
36.4694706816968));
#243762=CARTESIAN_POINT('Ctrl Pts',(-5.77963728315236,-5.93375687402476,
36.6284250475215));
#243763=CARTESIAN_POINT('Ctrl Pts',(-2.23874234079903,-7.95666012487542,
36.7873794133463));
#243764=CARTESIAN_POINT('Ctrl Pts',(3.24225168818117,-8.13447634724329,
36.9993185677793));
#243765=CARTESIAN_POINT('Ctrl Pts',(7.69388900236769,-4.18618557437927,
37.2112577222123));
#243766=CARTESIAN_POINT('Ctrl Pts',(8.15929592082769,1.26829190182066,37.4231968766453));
#243767=CARTESIAN_POINT('Ctrl Pts',(6.07406736985527,6.30084178841948,37.6351360310783));
#243768=CARTESIAN_POINT('Ctrl Pts',(-0.747012665881907,9.36907866881162,
37.9000599741196));
#243769=CARTESIAN_POINT('Ctrl Pts',(-8.28968198146107,4.41442200095284,
38.2179687057692));
#243770=CARTESIAN_POINT('Ctrl Pts',(-8.20443175221731,-3.04712989400972,
38.4828926488103));
#243771=CARTESIAN_POINT('Ctrl Pts',(-4.41325889417126,-6.98881211935876,
38.6948318032434));
#243772=CARTESIAN_POINT('Ctrl Pts',(-0.531826161575748,-8.26624695364861,
38.8537861690681));
#243773=CARTESIAN_POINT('Ctrl Pts',(3.4735956609319,-7.50030271359922,39.012740534893));
#243774=CARTESIAN_POINT('Ctrl Pts',(7.75297088062306,-4.07103721152057,
39.2246796893259));
#243775=CARTESIAN_POINT('Ctrl Pts',(8.56712613159509,1.82330126123921,39.436618843759));
#243776=CARTESIAN_POINT('Ctrl Pts',(5.37357826151764,6.26955588053925,39.6485579981919));
#243777=CARTESIAN_POINT('Ctrl Pts',(0.516776372933795,8.73658078636091,
39.860497152625));
#243778=CARTESIAN_POINT('Ctrl Pts',(-6.66029056348775,6.63160558502124,
40.1254210956662));
#243779=CARTESIAN_POINT('Ctrl Pts',(-9.16815589831957,-2.03736751234651,
40.4433298273158));
#243780=CARTESIAN_POINT('Ctrl Pts',(-4.25106985578304,-7.65023568584735,
40.708253770357));
#243781=CARTESIAN_POINT('Ctrl Pts',(1.19228200701667,-8.17916942741876,
40.9201929247901));
#243782=CARTESIAN_POINT('Ctrl Pts',(4.97161392719165,-6.62546094425101,
41.0791472906148));
#243783=CARTESIAN_POINT('Ctrl Pts',(7.51630599972235,-3.43882999431583,
41.2381016564396));
#243784=CARTESIAN_POINT('Ctrl Pts',(8.5371266166875,1.94919742048378,41.4500408108726));
#243785=CARTESIAN_POINT('Ctrl Pts',(5.32246579161211,6.95639529792656,41.6619799653056));
#243786=CARTESIAN_POINT('Ctrl Pts',(0.00498228527689334,8.2572785740032,
41.8739191197386));
#243787=CARTESIAN_POINT('Ctrl Pts',(-5.28890972002855,6.97297179326152,
42.0858582741717));
#243788=CARTESIAN_POINT('Ctrl Pts',(-9.37221561133872,0.706567448972694,
42.3507822172128));
#243789=CARTESIAN_POINT('Ctrl Pts',(-5.63983979118354,-7.50987057718307,
42.6686909488625));
#243790=CARTESIAN_POINT('Ctrl Pts',(1.7456225031276,-8.5761589913162,42.9336148919036));
#243791=CARTESIAN_POINT('Ctrl Pts',(6.22473749031018,-5.43810556015643,
43.1455540463367));
#243792=CARTESIAN_POINT('Ctrl Pts',(8.08538493741333,-1.80006338185378,
43.3045084121615));
#243793=CARTESIAN_POINT('Ctrl Pts',(7.94620884873859,2.27555983078824,43.4634627779862));
#243794=CARTESIAN_POINT('Ctrl Pts',(5.21780452959536,7.03252567320655,43.6754019324192));
#243795=CARTESIAN_POINT('Ctrl Pts',(-0.48050501054649,8.74581000129407,
43.8873410868522));
#243796=CARTESIAN_POINT('Ctrl Pts',(-5.36600848936145,6.27603594348851,
44.0992802412853));
#243797=CARTESIAN_POINT('Ctrl Pts',(-8.5524145007925,1.85771576482195,44.3112193957182));
#243798=CARTESIAN_POINT('Ctrl Pts',(-7.57926675468472,-5.55809126289773,
44.5761433387595));
#243799=CARTESIAN_POINT('Ctrl Pts',(0.599336602836362,-9.3726594194368,
44.8940520704091));
#243800=CARTESIAN_POINT('Ctrl Pts',(6.90325934010349,-5.37984306936858,
45.1589760134503));
#243801=CARTESIAN_POINT('Ctrl Pts',(8.2651942141464,-0.083147514205629,
45.3709151678833));
#243802=CARTESIAN_POINT('Ctrl Pts',(7.31281347293094,3.89055739900608,45.5298695337081));
#243803=CARTESIAN_POINT('Ctrl Pts',(4.55666596934872,6.89617305866435,45.6888238995329));
#243804=CARTESIAN_POINT('Ctrl Pts',(-0.609521261097548,8.73558156539363,
45.9007630539659));
#243805=CARTESIAN_POINT('Ctrl Pts',(-6.05251500548945,6.3314405747998,46.1127022083988));
#243806=CARTESIAN_POINT('Ctrl Pts',(-8.15775945374294,1.2781373035503,46.324641362832));
#243807=CARTESIAN_POINT('Ctrl Pts',(-7.70509314365592,-4.15047482871782,
46.5365805172648));
#243808=CARTESIAN_POINT('Ctrl Pts',(-2.14324752551869,-9.15118315135956,
46.8015044603062));
#243809=CARTESIAN_POINT('Ctrl Pts',(6.55043428269769,-6.73036103521313,
47.1194131919557));
#243810=CARTESIAN_POINT('Ctrl Pts',(8.7427573135604,0.402362428594548,47.3843371349969));
#243811=CARTESIAN_POINT('Ctrl Pts',(6.3328808615103,5.31177643548693,47.59627628943));
#243812=CARTESIAN_POINT('Ctrl Pts',(3.02524577395481,7.71113258685195,47.7552306552547));
#243813=CARTESIAN_POINT('Ctrl Pts',(-1.023096007437,8.20205353377038,47.9141850210795));
#243814=CARTESIAN_POINT('Ctrl Pts',(-6.14387295289784,6.23976975472853,
48.1261241755125));
#243815=CARTESIAN_POINT('Ctrl Pts',(-8.71530715530853,0.873784202491687,
48.3380633299456));
#243816=CARTESIAN_POINT('Ctrl Pts',(-7.02838021728527,-4.33411418782803,
48.5500024843785));
#243817=CARTESIAN_POINT('Ctrl Pts',(-3.15422136962083,-8.16368723112667,
48.7619416388116));
#243818=CARTESIAN_POINT('Ctrl Pts',(4.32295071883371,-8.34564318119966,
49.0268655818528));
#243819=CARTESIAN_POINT('Ctrl Pts',(9.35298292282078,-0.853029543263231,
49.3447743135024));
#243820=CARTESIAN_POINT('Ctrl Pts',(6.37993847010265,5.99116733913045,49.6096982565436));
#243821=CARTESIAN_POINT('Ctrl Pts',(1.35658827104663,8.15352789714588,49.8216374109767));
#243822=CARTESIAN_POINT('Ctrl Pts',(-2.71644454735151,7.82525442308462,
49.9805917768014));
#243823=CARTESIAN_POINT('Ctrl Pts',(-6.11109395564759,5.56551329856609,
50.1395461426262));
#243824=CARTESIAN_POINT('Ctrl Pts',(-8.72509444732845,0.744733736695816,
50.3514852970592));
#243825=CARTESIAN_POINT('Ctrl Pts',(-7.18897675376466,-5.00386759194602,
50.5634244514922));
#243826=CARTESIAN_POINT('Ctrl Pts',(-2.52072118608171,-7.86311890879807,
50.7753636059252));
#243827=CARTESIAN_POINT('Ctrl Pts',(2.91276677713683,-8.25292017156604,
50.9873027603582));
#243828=CARTESIAN_POINT('Ctrl Pts',(8.7112680552635,-3.52866432162581,51.2522267033995));
#243829=CARTESIAN_POINT('Ctrl Pts',(7.65990209328867,5.43432138150552,51.570135435049));
#243830=CARTESIAN_POINT('Ctrl Pts',(0.950521554408865,8.70024193585228,
51.8350593780902));
#243831=CARTESIAN_POINT('Ctrl Pts',(-4.27176562005544,7.07618310913376,
52.0469985325234));
#243832=CARTESIAN_POINT('Ctrl Pts',(-7.15244145934331,4.17806880454457,
52.2059528983479));
#243833=CARTESIAN_POINT('Ctrl Pts',(-8.26171734586479,0.253838744689786,
52.3649072641729));
#243834=CARTESIAN_POINT('Ctrl Pts',(-7.11248900476896,-5.10826796579968,
52.5768464186057));
#243835=CARTESIAN_POINT('Ctrl Pts',(-2.20717380217117,-8.47634717616648,
52.7887855730389));
#243836=CARTESIAN_POINT('Ctrl Pts',(3.19855434677107,-7.61261613130539,
53.0007247274718));
#243837=CARTESIAN_POINT('Ctrl Pts',(7.5796967531928,-4.37528270925114,53.2126638819049));
#243838=CARTESIAN_POINT('Ctrl Pts',(8.91240428482381,2.98441164875481,53.4775878249461));
#243839=CARTESIAN_POINT('Ctrl Pts',(2.28499249646148,9.10959704088886,53.7954965565956));
#243840=CARTESIAN_POINT('Ctrl Pts',(-4.93577556162372,7.22743526937714,
54.0604204996369));
#243841=CARTESIAN_POINT('Ctrl Pts',(-7.84684136797584,2.59758146214908,
54.2723596540699));
#243842=CARTESIAN_POINT('Ctrl Pts',(-8.15052697237911,-1.47735839841323,
54.4313140198947));
#243843=CARTESIAN_POINT('Ctrl Pts',(-6.44124186029901,-5.17984661050887,
54.5902683857195));
#243844=CARTESIAN_POINT('Ctrl Pts',(-2.08117581556965,-8.5059160986964,
54.8022075401524));
#243845=CARTESIAN_POINT('Ctrl Pts',(3.83553513755162,-7.87456334360853,
55.0141466945856));
#243846=CARTESIAN_POINT('Ctrl Pts',(7.38040430103625,-3.70301318187023,
55.2260858490184));
#243847=CARTESIAN_POINT('Ctrl Pts',(8.6033496725185,1.60538969369099,55.4380250034515));
#243848=CARTESIAN_POINT('Ctrl Pts',(4.82968073628349,8.06299243525258,55.7029489464928));
#243849=CARTESIAN_POINT('Ctrl Pts',(-4.18822762758455,8.40622973132391,
56.0208576781423));
#243850=CARTESIAN_POINT('Ctrl Pts',(-8.44962976254117,2.2806704811826,56.2857816211834));
#243851=CARTESIAN_POINT('Ctrl Pts',(-7.65023362318843,-3.12958054974059,
56.4977207756167));
#243852=CARTESIAN_POINT('Ctrl Pts',(-5.23095866816667,-6.42267461240047,
56.6566751414413));
#243853=CARTESIAN_POINT('Ctrl Pts',(-1.52470205308439,-8.12377321572858,
56.8156295072661));
#243854=CARTESIAN_POINT('Ctrl Pts',(3.95048083680223,-7.81508813843023,
57.027568661699));
#243855=CARTESIAN_POINT('Ctrl Pts',(8.0346456297457,-3.48777110033108,57.2395078161322));
#243856=CARTESIAN_POINT('Ctrl Pts',(8.01476963488675,1.98648986193146,57.4514469705651));
#243857=CARTESIAN_POINT('Ctrl Pts',(5.49169381979988,6.81441124718818,57.6633861249983));
#243858=CARTESIAN_POINT('Ctrl Pts',(-1.57448990846434,9.2659939862657,57.9283100680393));
#243859=CARTESIAN_POINT('Ctrl Pts',(-8.64832320050468,3.66230184117443,
58.246218799689));
#243860=CARTESIAN_POINT('Ctrl Pts',(-7.90206260926476,-3.76232740295407,
58.5111427427301));
#243861=CARTESIAN_POINT('Ctrl Pts',(-3.77644438347535,-7.35247011045913,
58.7230818971633));
#243862=CARTESIAN_POINT('Ctrl Pts',(0.202936042627704,-8.28085108714341,
58.8820362629879));
#243863=CARTESIAN_POINT('Ctrl Pts',(4.12470506917314,-7.16290553501901,
59.0409906288128));
#243864=CARTESIAN_POINT('Ctrl Pts',(8.08328893831205,-3.36783927661889,
59.2529297832456));
#243865=CARTESIAN_POINT('Ctrl Pts',(8.37180213684398,2.5754624100209,59.4648689376788));
#243866=CARTESIAN_POINT('Ctrl Pts',(4.79673463181595,6.72116144306895,59.6768080921117));
#243867=CARTESIAN_POINT('Ctrl Pts',(-0.259614085995455,8.747999896124,59.8887472465449));
#243868=CARTESIAN_POINT('Ctrl Pts',(-7.22186207613001,6.01517839957581,
60.1536711895859));
#243869=CARTESIAN_POINT('Ctrl Pts',(-8.95149290665923,-2.84195772281832,
60.4715799212356));
#243870=CARTESIAN_POINT('Ctrl Pts',(-3.55626917562253,-7.99691506258984,
60.7365038642768));
#243871=CARTESIAN_POINT('Ctrl Pts',(1.91254058587403,-8.04130197257024,
60.9484430187099));
#243872=CARTESIAN_POINT('Ctrl Pts',(5.53928697928919,-6.15873181149487,
61.1073973845346));
#243873=CARTESIAN_POINT('Ctrl Pts',(7.79152056097164,-2.75909676510714,
61.2663517503593));
#243874=CARTESIAN_POINT('Ctrl Pts',(8.33076203358052,2.6982041051833,61.4782909047926));
#243875=CARTESIAN_POINT('Ctrl Pts',(4.68494612183171,7.40076735747243,61.6902300592252));
#243876=CARTESIAN_POINT('Ctrl Pts',(-0.726911505889756,8.22522181673321,
61.9021692136586));
#243877=CARTESIAN_POINT('Ctrl Pts',(-5.88613519966566,6.47675181456649,
62.1141083680913));
#243878=CARTESIAN_POINT('Ctrl Pts',(-9.39795494785929,-0.126908720646365,
62.3790323111328));
#243879=CARTESIAN_POINT('Ctrl Pts',(-4.95201439452223,-7.98019438314016,
62.6969410427822));
#243880=CARTESIAN_POINT('Ctrl Pts',(2.49888999084336,-8.38768441117226,
62.9618649858234));
#243881=CARTESIAN_POINT('Ctrl Pts',(6.68223874686327,-4.86498039426644,
63.1738041402566));
#243882=CARTESIAN_POINT('Ctrl Pts',(8.21310960915687,-1.07634024026636,
63.3327585060813));
#243883=CARTESIAN_POINT('Ctrl Pts',(7.71324320523999,2.97090674173524,63.491712871906));
#243884=CARTESIAN_POINT('Ctrl Pts',(4.57394905114565,7.46732157677019,63.703652026339));
#243885=CARTESIAN_POINT('Ctrl Pts',(-1.25378846741183,8.66879992403101,
63.9155911807722));
#243886=CARTESIAN_POINT('Ctrl Pts',(-5.9011584396543,5.77572535201913,64.127530335205));
#243887=CARTESIAN_POINT('Ctrl Pts',(-8.68341102503059,1.09237110297249,
64.3394694896381));
#243888=CARTESIAN_POINT('Ctrl Pts',(-7.05680197762321,-6.20799556008093,
64.6043934326793));
#243889=CARTESIAN_POINT('Ctrl Pts',(1.42771243303241,-9.28264973834655,
64.9223021643289));
#243890=CARTESIAN_POINT('Ctrl Pts',(7.35292609561125,-4.74680722172566,
65.1872261073701));
#243891=CARTESIAN_POINT('Ctrl Pts',(8.24003438631967,0.649755507064886,
65.3991652618031));
#243892=CARTESIAN_POINT('Ctrl Pts',(6.93919728632182,4.52340787308913,65.5581196276279));
#243893=CARTESIAN_POINT('Ctrl Pts',(3.92749800249095,7.27290636896342,65.7170739934526));
#243894=CARTESIAN_POINT('Ctrl Pts',(-1.38139036042829,8.64717654067271,
65.9290131478857));
#243895=CARTESIAN_POINT('Ctrl Pts',(-6.58987378107479,5.77006422781667,
66.1409523023186));
#243896=CARTESIAN_POINT('Ctrl Pts',(-8.23893897492785,0.550053487929615,
66.3528914567518));
#243897=CARTESIAN_POINT('Ctrl Pts',(-7.30689557719576,-4.81707158756267,
66.5648306111847));
#243898=CARTESIAN_POINT('Ctrl Pts',(-1.32370793435634,-9.30513086042084,
66.829754554226));
#243899=CARTESIAN_POINT('Ctrl Pts',(7.12119123259477,-6.12328215812712,
67.1476632858755));
#243900=CARTESIAN_POINT('Ctrl Pts',(8.67268532647238,1.17568286167335,67.4125872289168));
#243901=CARTESIAN_POINT('Ctrl Pts',(5.83715333896189,5.85217821046453,67.6245263833497));
#243902=CARTESIAN_POINT('Ctrl Pts',(2.32987207101727,7.94892281369866,67.7834807491746));
#243903=CARTESIAN_POINT('Ctrl Pts',(-1.74604875975871,8.07909161515217,
67.9424351149993));
#243904=CARTESIAN_POINT('Ctrl Pts',(-6.67274703708215,5.67065679553783,
68.1543742694324));
#243905=CARTESIAN_POINT('Ctrl Pts',(-8.75845295486286,0.0978742208561194,
68.3663134238653));
#243906=CARTESIAN_POINT('Ctrl Pts',(-6.61656935417688,-4.94000853551062,
68.5782525782984));
#243907=CARTESIAN_POINT('Ctrl Pts',(-2.41822838793727,-8.41112793482519,
68.7901917327313));
#243908=CARTESIAN_POINT('Ctrl Pts',(5.0456430210861,-7.92963737654938,69.0551156757727));
#243909=CARTESIAN_POINT('Ctrl Pts',(9.39177951848075,-0.0206816296521539,
69.3730244074221));
#243910=CARTESIAN_POINT('Ctrl Pts',(5.82380861030514,6.53306615571522,69.6379483504635));
#243911=CARTESIAN_POINT('Ctrl Pts',(0.628570915073197,8.24167742695639,
69.8498875048964));
#243912=CARTESIAN_POINT('Ctrl Pts',(-3.39933595810127,7.55368764365964,
70.0088418707212));
#243913=CARTESIAN_POINT('Ctrl Pts',(-6.58033445871659,5.0019591291155,70.1677962365461));
#243914=CARTESIAN_POINT('Ctrl Pts',(-8.75676499863564,-0.031535311683235,
70.3797353909789));
#243915=CARTESIAN_POINT('Ctrl Pts',(-6.7171681344739,-5.62136124066343,
70.5916745454121));
#243916=CARTESIAN_POINT('Ctrl Pts',(-1.813865389671,-8.05559187373631,70.8036136998449));
#243917=CARTESIAN_POINT('Ctrl Pts',(3.63279868789117,-7.96227197870748,
71.0155528542781));
#243918=CARTESIAN_POINT('Ctrl Pts',(8.98972517918711,-2.74265778759378,
71.2804767973192));
#243919=CARTESIAN_POINT('Ctrl Pts',(7.14811970341057,6.09184979863643,71.5983855289689));
#243920=CARTESIAN_POINT('Ctrl Pts',(0.175594806760906,8.75026553285845,
71.86330947201));
#243921=CARTESIAN_POINT('Ctrl Pts',(-4.88207302152628,6.66968678879071,
72.0752486264431));
#243922=CARTESIAN_POINT('Ctrl Pts',(-7.49476079781095,3.52772811010838,
72.2342029922678));
#243923=CARTESIAN_POINT('Ctrl Pts',(-8.25141848381123,-0.479523465063083,
72.3931573580926));
#243924=CARTESIAN_POINT('Ctrl Pts',(-6.6323737200743,-5.71835230350754,
72.6050965125256));
#243925=CARTESIAN_POINT('Ctrl Pts',(-1.4459633342905,-8.63903494416697,
72.8170356669587));
#243926=CARTESIAN_POINT('Ctrl Pts',(3.85926018638893,-7.29866627444097,
73.0289748213916));
#243927=CARTESIAN_POINT('Ctrl Pts',(7.94102894798011,-3.68738514981999,
73.2409139758247));
#243928=CARTESIAN_POINT('Ctrl Pts',(8.60568699227863,3.76499989227933,73.5058379188659));
#243929=CARTESIAN_POINT('Ctrl Pts',(1.48089681516255,9.27222962841085,73.8237466505155));
#243930=CARTESIAN_POINT('Ctrl Pts',(-6.98781478096711,6.26620336683783,
74.141655382165));
#243931=CARTESIAN_POINT('Ctrl Pts',(-9.05505641808052,-2.48502531424726,
74.4595641138145));
#243932=CARTESIAN_POINT('Ctrl Pts',(-2.81052426251138,-8.95521152276751,
74.7774728454639));
#243933=CARTESIAN_POINT('Ctrl Pts',(6.00625529959161,-7.21749228854913,
75.0953815771136));
#243934=CARTESIAN_POINT('Ctrl Pts',(9.32196859427813,1.15497806266144,75.4132903087629));
#243935=CARTESIAN_POINT('Ctrl Pts',(4.94651276262872,7.22417894884408,75.6782142518044));
#243936=CARTESIAN_POINT('Ctrl Pts',(-0.40678230636204,8.24614738694012,
75.8901534062373));
#243937=CARTESIAN_POINT('Ctrl Pts',(-5.65301526785667,6.69082604108267,
76.1020925606704));
#243938=CARTESIAN_POINT('Ctrl Pts',(-8.62212040196883,1.5319836825875,76.3140317151032));
#243939=CARTESIAN_POINT('Ctrl Pts',(-7.34032809091788,-3.79939906645903,
76.5259708695365));
#243940=CARTESIAN_POINT('Ctrl Pts',(-4.64425086315509,-6.85909899005226,
76.6849252353611));
#243941=CARTESIAN_POINT('Ctrl Pts',(-0.793804143464836,-8.2273467065575,
76.8438796011859));
#243942=CARTESIAN_POINT('Ctrl Pts',(4.61737414584813,-7.43490661871054,
77.0558187556188));
#243943=CARTESIAN_POINT('Ctrl Pts',(9.25626449155225,-1.58991098048353,
77.3207426986603));
#243944=CARTESIAN_POINT('Ctrl Pts',(6.33052329467649,6.94707171063594,77.6386514303096));
#243945=CARTESIAN_POINT('Ctrl Pts',(-0.940243880013648,8.7012035268548,
77.903575373351));
#243946=CARTESIAN_POINT('Ctrl Pts',(-5.67157647317062,6.00132388702944,
78.1155145277839));
#243947=CARTESIAN_POINT('Ctrl Pts',(-8.64552997002301,1.40529764899067,
78.327453682217));
#243948=CARTESIAN_POINT('Ctrl Pts',(-7.54622056146987,-4.44257616196536,
78.53939283665));
#243949=CARTESIAN_POINT('Ctrl Pts',(-3.10542854980952,-7.66007246962735,
78.751331991083));
#243950=CARTESIAN_POINT('Ctrl Pts',(0.932450631858945,-8.23068756503138,
78.9102863569078));
#243951=CARTESIAN_POINT('Ctrl Pts',(4.74730033149722,-6.76634966343337,
79.0692407227326));
#243952=CARTESIAN_POINT('Ctrl Pts',(8.34267086175441,-2.64528694414241,
79.2811798771655));
#243953=CARTESIAN_POINT('Ctrl Pts',(8.0656297691254,4.81160749448224,79.5461038202069));
#243954=CARTESIAN_POINT('Ctrl Pts',(0.291347901712305,9.39429501452725,
79.8640125518562));
#243955=CARTESIAN_POINT('Ctrl Pts',(-6.37275616353708,5.99857320971597,
80.1289364948976));
#243956=CARTESIAN_POINT('Ctrl Pts',(-8.21124180344807,0.87073669662942,
80.3408756493307));
#243957=CARTESIAN_POINT('Ctrl Pts',(-7.48161788051808,-4.55471968572886,
80.5528148037635));
#243958=CARTESIAN_POINT('Ctrl Pts',(-2.84357433903173,-8.28226940470237,
80.7647539581967));
#243959=CARTESIAN_POINT('Ctrl Pts',(2.62232728429337,-7.83861003058117,
80.9766931126296));
#243960=CARTESIAN_POINT('Ctrl Pts',(6.06085450803398,-5.64621292530574,
81.1356474784545));
#243961=CARTESIAN_POINT('Ctrl Pts',(8.0066023109931,-2.05296574330638,81.2946018442791));
#243962=CARTESIAN_POINT('Ctrl Pts',(8.05792312660012,3.41578334339948,81.5065409987122));
#243963=CARTESIAN_POINT('Ctrl Pts',(2.99816836424723,8.90038962174408,81.7714649417535));
#243964=CARTESIAN_POINT('Ctrl Pts',(-5.88787901169365,7.32601827520863,
82.089373673403));
#243965=CARTESIAN_POINT('Ctrl Pts',(-8.74211725417119,0.412659145140834,
82.3542976164443));
#243966=CARTESIAN_POINT('Ctrl Pts',(-6.80407226898225,-4.67838378402576,
82.5662367708773));
#243967=CARTESIAN_POINT('Ctrl Pts',(-2.72156961391875,-8.32545112773004,
82.7781759253103));
#243968=CARTESIAN_POINT('Ctrl Pts',(3.22587080656452,-8.14098636485779,
82.9901150797432));
#243969=CARTESIAN_POINT('Ctrl Pts',(7.08962881161275,-4.24942006923645,
83.2020542341765));
#243970=CARTESIAN_POINT('Ctrl Pts',(8.27603181017464,-0.347814953384133,
83.3610086000008));
#243971=CARTESIAN_POINT('Ctrl Pts',(7.41742979179161,3.64720224151801,83.519962965826));
#243972=CARTESIAN_POINT('Ctrl Pts',(3.90003270325899,7.83501409579196,83.7319021202586));
#243973=CARTESIAN_POINT('Ctrl Pts',(-3.51040051647884,8.71108702574855,
83.9968260633002));
#243974=CARTESIAN_POINT('Ctrl Pts',(-9.23702247828752,1.7363982149788,84.3147347949496));
#243975=CARTESIAN_POINT('Ctrl Pts',(-6.90946916794436,-5.37160473913135,
84.5796587379909));
#243976=CARTESIAN_POINT('Ctrl Pts',(-2.12643939590146,-7.97877996735202,
84.7915978924239));
#243977=CARTESIAN_POINT('Ctrl Pts',(3.34663549462676,-8.09444924068338,
85.0035370468568));
#243978=CARTESIAN_POINT('Ctrl Pts',(7.74476036947559,-4.08663532417261,
85.21547620129));
#243979=CARTESIAN_POINT('Ctrl Pts',(8.14921063415244,1.38230736505511,85.4274153557229));
#243980=CARTESIAN_POINT('Ctrl Pts',(6.51322980775338,5.11776467183024,85.5863697215476));
#243981=CARTESIAN_POINT('Ctrl Pts',(3.26297588227619,7.59429636624497,85.7453240873726));
#243982=CARTESIAN_POINT('Ctrl Pts',(-2.13245773804618,8.48824628313803,
85.9572632418053));
#243983=CARTESIAN_POINT('Ctrl Pts',(-8.33165101509813,4.33469033713718,
86.2221871848468));
#243984=CARTESIAN_POINT('Ctrl Pts',(-8.14627432876946,-4.68784359655912,
86.5400959164963));
#243985=CARTESIAN_POINT('Ctrl Pts',(-1.7556973859211,-8.57393890492018,
86.8050198595376));
#243986=CARTESIAN_POINT('Ctrl Pts',(3.57329345238697,-7.44407470240509,
87.0169590139705));
#243987=CARTESIAN_POINT('Ctrl Pts',(7.8062379490363,-3.97274800697461,87.2288981684036));
#243988=CARTESIAN_POINT('Ctrl Pts',(8.54103296197277,1.93200864280407,87.4408373228366));
#243989=CARTESIAN_POINT('Ctrl Pts',(5.29177135405442,6.34961129106956,87.6527764772695));
#243990=CARTESIAN_POINT('Ctrl Pts',(1.61976156676342,8.12342601564617,87.8117308430944));
#243991=CARTESIAN_POINT('Ctrl Pts',(-2.45986863119688,7.89109594568021,
87.9706852089191));
#243992=CARTESIAN_POINT('Ctrl Pts',(-7.13995541190373,5.061495597527,88.1826243633521));
#243993=CARTESIAN_POINT('Ctrl Pts',(-9.14818813581019,-2.12523005533024,
88.4475483063934));
#243994=CARTESIAN_POINT('Ctrl Pts',(-3.13991644891066,-8.858814126012,88.7654570380429));
#243995=CARTESIAN_POINT('Ctrl Pts',(4.2419725378046,-7.65510095588199,89.0303809810843));
#243996=CARTESIAN_POINT('Ctrl Pts',(7.55547763402694,-3.33128083379027,
89.2423201355171));
#243997=CARTESIAN_POINT('Ctrl Pts',(8.51367345730509,2.05850477441118,89.4542592899503));
#243998=CARTESIAN_POINT('Ctrl Pts',(5.23195009707337,7.02200823376817,89.6661984443832));
#243999=CARTESIAN_POINT('Ctrl Pts',(-0.109224718809311,8.26489428680549,
89.8781375988163));
#244000=CARTESIAN_POINT('Ctrl Pts',(-4.05226554613339,7.22445995964139,
90.0370919646409));
#244001=CARTESIAN_POINT('Ctrl Pts',(-7.00034619274214,4.39494051022739,
90.1960463304658));
#244002=CARTESIAN_POINT('Ctrl Pts',(-8.71554326333916,-0.798126927639463,
90.4079854848986));
#244003=CARTESIAN_POINT('Ctrl Pts',(-5.56753298998327,-7.56363175741028,
90.6729094279402));
#244004=CARTESIAN_POINT('Ctrl Pts',(3.37568196270829,-8.77168366461165,
90.9908181595894));
#244005=CARTESIAN_POINT('Ctrl Pts',(8.20068473993648,-3.05674196693257,
91.2557421026311));
#244006=CARTESIAN_POINT('Ctrl Pts',(7.90602598470913,2.38273527714745,91.4676812570636));
#244007=CARTESIAN_POINT('Ctrl Pts',(5.12890419993768,7.10031121513393,91.6796204114972));
#244008=CARTESIAN_POINT('Ctrl Pts',(-0.591935717244415,8.73679080441012,
91.8915595659297));
#244009=CARTESIAN_POINT('Ctrl Pts',(-5.45772054990596,6.20755136993672,
92.103498720363));
#244010=CARTESIAN_POINT('Ctrl Pts',(-7.77652000100319,2.85296590215134,
92.2624530861876));
#244011=CARTESIAN_POINT('Ctrl Pts',(-8.17601886780652,-1.21369863637932,
92.4214074520124));
#244012=CARTESIAN_POINT('Ctrl Pts',(-6.10189507510199,-6.27411965619128,
92.6333466064455));
#244013=CARTESIAN_POINT('Ctrl Pts',(0.689227264725502,-9.36647824605471,
92.8982705494865));
#244014=CARTESIAN_POINT('Ctrl Pts',(8.26871616813045,-4.46833257001599,
93.2161792811364));
#244015=CARTESIAN_POINT('Ctrl Pts',(8.21763415981667,3.01087868763386,93.4811032241773));
#244016=CARTESIAN_POINT('Ctrl Pts',(4.45644300851865,6.95145955779684,93.6930423786106));
#244017=CARTESIAN_POINT('Ctrl Pts',(-0.721137693822396,8.72926331774012,
93.9049815330433));
#244018=CARTESIAN_POINT('Ctrl Pts',(-6.13130014661506,6.25212443618104,
94.1169206874767));
#244019=CARTESIAN_POINT('Ctrl Pts',(-8.1828940095445,1.16647041961204,94.3288598419095));
#244020=CARTESIAN_POINT('Ctrl Pts',(-7.76289181710849,-2.88984227955638,
94.4878142077343));
#244021=CARTESIAN_POINT('Ctrl Pts',(-5.42178472385128,-6.23895819146835,
94.6467685735592));
#244022=CARTESIAN_POINT('Ctrl Pts',(-0.555293887085499,-8.73437746303224,
94.8587077279919));
#244023=CARTESIAN_POINT('Ctrl Pts',(6.61470172236203,-6.66720856734195,
95.1236316710334));
#244024=CARTESIAN_POINT('Ctrl Pts',(9.18728742537818,1.98277905699441,95.4415404026827));
#244025=CARTESIAN_POINT('Ctrl Pts',(4.28467384452833,7.63128244151975,95.7064643457242));
#244026=CARTESIAN_POINT('Ctrl Pts',(-1.13518563206099,8.17887693101086,
95.9184035001571));
#244027=CARTESIAN_POINT('Ctrl Pts',(-6.22455563939611,6.1623846630958,96.1303426545902));
#244028=CARTESIAN_POINT('Ctrl Pts',(-8.72357765688459,0.762295426772799,
96.3422818090232));
#244029=CARTESIAN_POINT('Ctrl Pts',(-6.97485602638083,-4.43528928284595,
96.5542209634562));
#244030=CARTESIAN_POINT('Ctrl Pts',(-4.01793155330728,-7.24361124010522,
96.7131753292809));
#244031=CARTESIAN_POINT('Ctrl Pts',(-0.0615012174835848,-8.26538362732942,
96.8721296951056));
#244032=CARTESIAN_POINT('Ctrl Pts',(5.25821632703537,-6.99634633404169,
97.0840688495389));
#244033=CARTESIAN_POINT('Ctrl Pts',(9.36073618300337,-0.763260812873669,
97.3489927925797));
#244034=CARTESIAN_POINT('Ctrl Pts',(5.68987284831566,7.48084286664063,97.6669015242299));
#244035=CARTESIAN_POINT('Ctrl Pts',(-1.70776911520327,8.58361382550448,
97.9318254672705));
#244036=CARTESIAN_POINT('Ctrl Pts',(-6.18117294910438,5.47501372099833,
98.1437646217039));
#244037=CARTESIAN_POINT('Ctrl Pts',(-8.73606223445313,0.633477923574835,
98.3557037761367));
#244038=CARTESIAN_POINT('Ctrl Pts',(-7.12275729466399,-5.09394051542466,
98.5676429305698));
#244039=CARTESIAN_POINT('Ctrl Pts',(-2.41426532741029,-7.90517112655593,
98.7795820850029));
#244040=CARTESIAN_POINT('Ctrl Pts',(1.65829830086496,-8.11564689412926,
98.9385364508275));
#244041=CARTESIAN_POINT('Ctrl Pts',(5.32834362648309,-6.31894794287737,
99.0974908166525));
#244042=CARTESIAN_POINT('Ctrl Pts',(8.5442983962845,-1.89543290121545,99.3094299710852));
#244043=CARTESIAN_POINT('Ctrl Pts',(7.60741447147656,5.50755789941659,99.5743539141267));
#244044=CARTESIAN_POINT('Ctrl Pts',(-0.542451036991783,9.38314498970543,
99.8922626457761));
#244045=CARTESIAN_POINT('Ctrl Pts',(-6.87935126239726,5.41012272178607,
100.157186588818));
#244046=CARTESIAN_POINT('Ctrl Pts',(-8.256101354105,0.139515958245546,100.369125743251));
#244047=CARTESIAN_POINT('Ctrl Pts',(-7.04847008699869,-5.19991798748602,
100.581064897684));
#244048=CARTESIAN_POINT('Ctrl Pts',(-2.09829360246755,-8.50170955815468,
100.793004052116));
#244049=CARTESIAN_POINT('Ctrl Pts',(3.30677251906783,-7.57533254177048,
101.00494320655));
#244050=CARTESIAN_POINT('Ctrl Pts',(6.5374461147551,-5.08679428142266,101.163897572374));
#244051=CARTESIAN_POINT('Ctrl Pts',(8.1570527526437,-1.33523005406003,101.322851938199));
#244052=CARTESIAN_POINT('Ctrl Pts',(7.72345543585777,4.11654431508733,101.534791092632));
#244053=CARTESIAN_POINT('Ctrl Pts',(2.19749283155659,9.13109928823001,101.799715035674));
#244054=CARTESIAN_POINT('Ctrl Pts',(-6.51403897443435,6.775319864399,102.117623767323));
#244055=CARTESIAN_POINT('Ctrl Pts',(-8.74428626583565,-0.363812255637007,
102.382547710364));
#244056=CARTESIAN_POINT('Ctrl Pts',(-6.36263028075182,-5.26304191341087,
102.594486864797));
#244057=CARTESIAN_POINT('Ctrl Pts',(-1.97294169497133,-8.53390758750871,
102.80642601923));
#244058=CARTESIAN_POINT('Ctrl Pts',(3.93474143355371,-7.82302443460647,
103.018365173664));
#244059=CARTESIAN_POINT('Ctrl Pts',(7.43836835449544,-3.60431461364149,
103.230304328096));
#244060=CARTESIAN_POINT('Ctrl Pts',(8.2742878160075,0.387090303045284,103.389258693921));
#244061=CARTESIAN_POINT('Ctrl Pts',(7.06497136278176,4.2902830384196,103.548213059746));
#244062=CARTESIAN_POINT('Ctrl Pts',(3.1902359906745,8.14985247053979,103.760152214179));
#244063=CARTESIAN_POINT('Ctrl Pts',(-4.26868151559312,8.36566238110832,
104.02507615722));
#244064=CARTESIAN_POINT('Ctrl Pts',(-9.35457173711607,0.910851601809192,
104.34298488887));
#244065=CARTESIAN_POINT('Ctrl Pts',(-6.40616954212128,-5.96287627356382,
104.607908831911));
#244066=CARTESIAN_POINT('Ctrl Pts',(-1.41088053516091,-8.1358521611054,
104.819847986344));
#244067=CARTESIAN_POINT('Ctrl Pts',(4.05090606201291,-7.76596663144024,
105.031787140777));
#244068=CARTESIAN_POINT('Ctrl Pts',(8.07649326184086,-3.38410372843594,
105.24372629521));
#244069=CARTESIAN_POINT('Ctrl Pts',(7.9946184145099,2.09916269442086,105.455665449643));
#244070=CARTESIAN_POINT('Ctrl Pts',(6.03398848610383,5.67491504028099,105.614619815468));
#244071=CARTESIAN_POINT('Ctrl Pts',(2.57702218155512,7.8536173565084,105.773574181293));
#244072=CARTESIAN_POINT('Ctrl Pts',(-2.8764107100891,8.26583101657924,105.985513335726));
#244073=CARTESIAN_POINT('Ctrl Pts',(-8.6830601333559,3.57916410308085,106.250437278767));
#244074=CARTESIAN_POINT('Ctrl Pts',(-7.698711346468,-5.39142899694823,106.568346010416));
#244075=CARTESIAN_POINT('Ctrl Pts',(-0.988846449827039,-8.69580843595914,
106.833269953458));
#244076=CARTESIAN_POINT('Ctrl Pts',(4.21902677410503,-7.09806222508963,
107.045209107891));
#244077=CARTESIAN_POINT('Ctrl Pts',(8.12763461419744,-3.26521564708898,
107.257148262323));
#244078=CARTESIAN_POINT('Ctrl Pts',(8.33617651168416,2.68142921208433,107.469087416757));
#244079=CARTESIAN_POINT('Ctrl Pts',(4.70815407640191,6.79365091862457,107.68102657119));
#244080=CARTESIAN_POINT('Ctrl Pts',(0.893376316806882,8.23502012877987,
107.839980937014));
#244081=CARTESIAN_POINT('Ctrl Pts',(-3.14960528647604,7.64201121734848,
107.998935302839));
#244082=CARTESIAN_POINT('Ctrl Pts',(-7.56047424334183,4.40873339900752,
108.210874457272));
#244083=CARTESIAN_POINT('Ctrl Pts',(-8.92381613848062,-2.92770464405993,
108.475798400314));
#244084=CARTESIAN_POINT('Ctrl Pts',(-2.34236803040989,-9.10225109714528,
108.793707131963));
#244085=CARTESIAN_POINT('Ctrl Pts',(4.90377818824009,-7.2489903529232,109.058631075004));
#244086=CARTESIAN_POINT('Ctrl Pts',(7.82100553314839,-2.64849895645091,
109.270570229437));
#244087=CARTESIAN_POINT('Ctrl Pts',(8.29771285046806,2.80500251248967,109.482509383871));
#244088=CARTESIAN_POINT('Ctrl Pts',(4.58897114648115,7.45809930680315,109.694448538303));
#244089=CARTESIAN_POINT('Ctrl Pts',(-0.841344032665456,8.22268495261532,
109.906387692737));
#244090=CARTESIAN_POINT('Ctrl Pts',(-4.6766484720228,6.83685869635818,110.065342058561));
#244091=CARTESIAN_POINT('Ctrl Pts',(-7.36233516049885,3.75717578656633,
110.224296424386));
#244092=CARTESIAN_POINT('Ctrl Pts',(-8.61050026220927,-1.56747765606163,
110.436235578819));
#244093=CARTESIAN_POINT('Ctrl Pts',(-4.87522711379125,-8.02733514593802,
110.70115952186));
#244094=CARTESIAN_POINT('Ctrl Pts',(4.13986408852363,-8.43796114911191,
111.01906825351));
#244095=CARTESIAN_POINT('Ctrl Pts',(8.4393398531768,-2.31785342479099,111.283992196551));
#244096=CARTESIAN_POINT('Ctrl Pts',(7.66371912007564,3.07409881435952,111.495931350984));
#244097=CARTESIAN_POINT('Ctrl Pts',(4.47939051666135,7.52696075738007,111.707870505417));
#244098=CARTESIAN_POINT('Ctrl Pts',(-1.36398120786484,8.64993969446986,
111.91980965985));
#244099=CARTESIAN_POINT('Ctrl Pts',(-5.98643949729513,5.69938152403339,
112.131748814283));
#244100=CARTESIAN_POINT('Ctrl Pts',(-7.99878305688911,2.15247470918116,
112.290703180108));
#244101=CARTESIAN_POINT('Ctrl Pts',(-8.03626557491185,-1.93359367917992,
112.449657545933));
#244102=CARTESIAN_POINT('Ctrl Pts',(-5.5217804877095,-6.79026076180513,
112.661596700365));
#244103=CARTESIAN_POINT('Ctrl Pts',(1.51670144919076,-9.26852553917179,
112.926520643407));
#244104=CARTESIAN_POINT('Ctrl Pts',(8.6322182027274,-3.71785851342826,113.244429375056));
#244105=CARTESIAN_POINT('Ctrl Pts',(7.91842613892663,3.72738905114509,113.509353318098));
#244106=CARTESIAN_POINT('Ctrl Pts',(3.8227692375331,7.31909213143469,113.721292472531));
#244107=CARTESIAN_POINT('Ctrl Pts',(-1.49200749139442,8.63099016854494,
113.933231626964));
#244108=CARTESIAN_POINT('Ctrl Pts',(-6.66131875303892,5.68407722711321,
114.145170781397));
#244109=CARTESIAN_POINT('Ctrl Pts',(-8.25407714505212,0.43659832202693,
114.35710993583));
#244110=CARTESIAN_POINT('Ctrl Pts',(-7.47620145562958,-3.56652345564748,
114.516064301654));
#244111=CARTESIAN_POINT('Ctrl Pts',(-4.84746335710774,-6.694956901144,114.675018667479));
#244112=CARTESIAN_POINT('Ctrl Pts',(0.221052877113095,-8.74921919906447,
114.886957821912));
#244113=CARTESIAN_POINT('Ctrl Pts',(7.17960828852418,-6.05468197179771,
115.151881764953));
#244114=CARTESIAN_POINT('Ctrl Pts',(8.97538752092487,2.78927981288996,115.469790496603));
#244115=CARTESIAN_POINT('Ctrl Pts',(3.59142080693308,7.98101486302093,115.734714439644));
#244116=CARTESIAN_POINT('Ctrl Pts',(-1.85564300132502,8.04607129744028,
115.946653594077));
#244117=CARTESIAN_POINT('Ctrl Pts',(-6.74625323876447,5.58642505385656,
116.15859274851));
#244118=CARTESIAN_POINT('Ctrl Pts',(-8.75680923615344,-0.0139088098970721,
116.370531902943));
#244119=CARTESIAN_POINT('Ctrl Pts',(-6.55428827612388,-5.03604138234919,
116.582471057376));
#244120=CARTESIAN_POINT('Ctrl Pts',(-3.36008912066162,-7.57122703833746,
116.741425423201));
#244121=CARTESIAN_POINT('Ctrl Pts',(0.671333398386882,-8.23830445995342,
116.900379789026));
#244122=CARTESIAN_POINT('Ctrl Pts',(5.85763438229858,-6.50275483245934,
117.112318943459));
#244123=CARTESIAN_POINT('Ctrl Pts',(9.39154564904932,0.069421020448106,
117.3772428865));
#244124=CARTESIAN_POINT('Ctrl Pts',(5.00442337244051,7.95571553882744,117.69515161815));
#244125=CARTESIAN_POINT('Ctrl Pts',(-2.4618463338131,8.39846499575511,117.960075561191));
#244126=CARTESIAN_POINT('Ctrl Pts',(-6.64211697505903,4.90560458674478,
118.172014715624));
#244127=CARTESIAN_POINT('Ctrl Pts',(-8.75782708988359,-0.143325879022417,
118.383953870057));
#244128=CARTESIAN_POINT('Ctrl Pts',(-6.64322866813353,-5.70520940161391,
118.59589302449));
#244129=CARTESIAN_POINT('Ctrl Pts',(-1.70409789680017,-8.0880441374531,
118.807832178923));
#244130=CARTESIAN_POINT('Ctrl Pts',(2.37109252386944,-7.93672463980526,
118.966786544748));
#244131=CARTESIAN_POINT('Ctrl Pts',(5.86744526985531,-5.82180684254729,
119.125740910572));
#244132=CARTESIAN_POINT('Ctrl Pts',(8.67866987731518,-1.13065915657217,
119.337680065005));
#244133=CARTESIAN_POINT('Ctrl Pts',(7.08931787809962,6.1601559216884,119.602604008047));
#244134=CARTESIAN_POINT('Ctrl Pts',(-1.37198012918096,9.29813602559685,
119.920512739696));
#244135=CARTESIAN_POINT('Ctrl Pts',(-7.33179591486946,4.77908676620727,
120.185436682737));
#244136=CARTESIAN_POINT('Ctrl Pts',(-8.2359734640424,-0.592802978609528,
120.397375837171));
#244137=CARTESIAN_POINT('Ctrl Pts',(-6.55984064560654,-5.80418541641674,
120.609314991604));
#244138=CARTESIAN_POINT('Ctrl Pts',(-1.33649626603419,-8.65422897687898,
120.821254146037));
#244139=CARTESIAN_POINT('Ctrl Pts',(3.96518867752886,-7.25242623973973,
121.03319330047));
#244140=CARTESIAN_POINT('Ctrl Pts',(6.9625785746472,-4.4873352177773,121.192147666294));
#244141=CARTESIAN_POINT('Ctrl Pts',(8.24329540403443,-0.606984174837291,
121.351102032119));
#244142=CARTESIAN_POINT('Ctrl Pts',(7.32819299175547,4.78490213518995,121.563041186552));
#244143=CARTESIAN_POINT('Ctrl Pts',(1.37951985544195,9.28993401078269,121.827965129593));
#244144=CARTESIAN_POINT('Ctrl Pts',(-7.08892403898856,6.17128989716245,
122.145873861243));
#244145=CARTESIAN_POINT('Ctrl Pts',(-8.67762511076401,-1.13741992829038,
122.410797804284));
#244146=CARTESIAN_POINT('Ctrl Pts',(-5.87110519946018,-5.80627229887907,
122.622736958717));
#244147=CARTESIAN_POINT('Ctrl Pts',(-1.20878387435662,-8.67518986472293,
122.83467611315));
#244148=CARTESIAN_POINT('Ctrl Pts',(4.61263996051857,-7.44348399931125,
123.046615267583));
#244149=CARTESIAN_POINT('Ctrl Pts',(7.72855719143385,-2.93083799449995,
123.258554422016));
#244150=CARTESIAN_POINT('Ctrl Pts',(8.20741322198891,1.11894859951792,123.417508787841));
#244151=CARTESIAN_POINT('Ctrl Pts',(6.65690140163672,4.89959310918416,123.576463153666));
#244152=CARTESIAN_POINT('Ctrl Pts',(2.45532751157165,8.40053973139096,123.788402308099));
#244153=CARTESIAN_POINT('Ctrl Pts',(-4.99336182376418,7.9543878867723,124.05332625114));
#244154=CARTESIAN_POINT('Ctrl Pts',(-9.39848700083521,0.0781352705295933,
124.37123498279));
#244155=CARTESIAN_POINT('Ctrl Pts',(-5.85244410633151,-6.5072113565259,
124.636158925831));
#244156=CARTESIAN_POINT('Ctrl Pts',(-0.684216006160355,-8.22888344362542,
124.848098080264));
#244157=CARTESIAN_POINT('Ctrl Pts',(4.72329014591897,-7.37635464449487,
125.060037234697));
#244158=CARTESIAN_POINT('Ctrl Pts',(8.34465248327202,-2.65493434698441,
125.27197638913));
#244159=CARTESIAN_POINT('Ctrl Pts',(7.77709699727505,2.79949458049909,125.483915543563));
#244160=CARTESIAN_POINT('Ctrl Pts',(5.50725095712811,6.18739562821485,125.642869909388));
#244161=CARTESIAN_POINT('Ctrl Pts',(1.87078359296915,8.05111903122513,125.801824275212));
#244162=CARTESIAN_POINT('Ctrl Pts',(-3.59772217398919,7.97835171740039,
126.013763429645));
#244163=CARTESIAN_POINT('Ctrl Pts',(-8.96612102302944,2.7954646763365,126.278687372687));
#244164=CARTESIAN_POINT('Ctrl Pts',(-7.19054838272788,-6.05257606156408,
126.596596104336));
#244165=CARTESIAN_POINT('Ctrl Pts',(-0.214211863482096,-8.74922939085366,
126.861520047377));
#244166=CARTESIAN_POINT('Ctrl Pts',(4.8315502594368,-6.69617774274212,127.073459201811));
#244167=CARTESIAN_POINT('Ctrl Pts',(8.38505505209209,-2.53198132245899,
127.285398356243));
#244168=CARTESIAN_POINT('Ctrl Pts',(8.06570230809352,3.40974305932135,127.497337510677));
#244169=CARTESIAN_POINT('Ctrl Pts',(4.08747682380009,7.18421469794477,127.709276665109));
#244170=CARTESIAN_POINT('Ctrl Pts',(0.159958904481424,8.28179273549621,
127.868231030934));
#244171=CARTESIAN_POINT('Ctrl Pts',(-3.81454999758313,7.33277281951486,
128.027185396759));
#244172=CARTESIAN_POINT('Ctrl Pts',(-7.92148121906867,3.72126809887472,
128.239124551192));
#244173=CARTESIAN_POINT('Ctrl Pts',(-8.62920081496092,-3.70713396727616,
128.504048494233));
#244174=CARTESIAN_POINT('Ctrl Pts',(-1.52638179124352,-9.27404020116001,
128.821957225883));
#244175=CARTESIAN_POINT('Ctrl Pts',(5.52698401932788,-6.78581972250434,
129.086881168924));
#244176=CARTESIAN_POINT('Ctrl Pts',(8.02497081889033,-1.94486956575818,
129.298820323357));
#244177=CARTESIAN_POINT('Ctrl Pts',(8.01643725491605,3.52942082811193,129.51075947779));
#244178=CARTESIAN_POINT('Ctrl Pts',(3.90987036279272,7.83548436278796,129.722698632223));
#244179=CARTESIAN_POINT('Ctrl Pts',(-1.5668407534036,8.11575120766773,129.934637786656));
#244180=CARTESIAN_POINT('Ctrl Pts',(-5.26421941759418,6.39544147719898,
130.093592152481));
#244181=CARTESIAN_POINT('Ctrl Pts',(-7.66637191338927,3.08983666108217,
130.252546518306));
#244182=CARTESIAN_POINT('Ctrl Pts',(-8.43768018353644,-2.32449007064272,
130.464485672739));
#244183=CARTESIAN_POINT('Ctrl Pts',(-4.14454615641619,-8.42785180890101,
130.72940961578));
#244184=CARTESIAN_POINT('Ctrl Pts',(4.87145950259031,-8.0378196882011,131.047318347429));
#244185=CARTESIAN_POINT('Ctrl Pts',(8.61156516868868,-1.56072002727027,
131.312242290471));
#244186=CARTESIAN_POINT('Ctrl Pts',(7.36108771321945,3.74126475232265,131.524181444904));
#244187=CARTESIAN_POINT('Ctrl Pts',(3.79461755858945,7.89436224373846,131.736120599337));
#244188=CARTESIAN_POINT('Ctrl Pts',(-2.12529019654376,8.49500106110592,
131.94805975377));
#244189=CARTESIAN_POINT('Ctrl Pts',(-6.46803651554601,5.14634931171196,
132.159998908203));
#244190=CARTESIAN_POINT('Ctrl Pts',(-8.15808413562142,1.43504042893685,
132.318953274028));
#244191=CARTESIAN_POINT('Ctrl Pts',(-7.83325525710364,-2.63826854349615,
132.477907639852));
#244192=CARTESIAN_POINT('Ctrl Pts',(-4.8982015186142,-7.25295271015235,
132.689846794285));
#244193=CARTESIAN_POINT('Ctrl Pts',(2.33223701977551,-9.09761613362508,
132.954770737327));
#244194=CARTESIAN_POINT('Ctrl Pts',(8.92777217698664,-2.93811955876141,
133.272679468976));
#244195=CARTESIAN_POINT('Ctrl Pts',(7.55688871607167,4.41455951102258,133.537603412017));
#244196=CARTESIAN_POINT('Ctrl Pts',(3.15900467980914,7.6291128306614,133.74954256645));
#244197=CARTESIAN_POINT('Ctrl Pts',(-2.25113285491774,8.46477877165042,
133.961481720883));
#244198=CARTESIAN_POINT('Ctrl Pts',(-7.13890352140618,5.07128788398544,
134.173420875317));
#244199=CARTESIAN_POINT('Ctrl Pts',(-8.26028831705473,-0.296710146126478,
134.385360029749));
#244200=CARTESIAN_POINT('Ctrl Pts',(-7.13066352516941,-4.21513154063565,
134.544314395574));
#244201=CARTESIAN_POINT('Ctrl Pts',(-4.2349837389692,-7.09825553010841,
134.703268761399));
#244202=CARTESIAN_POINT('Ctrl Pts',(0.995655938673994,-8.69519430925777,
134.915207915832));
#244203=CARTESIAN_POINT('Ctrl Pts',(7.68800861236119,-5.3944913782222,135.180131858873));
#244204=CARTESIAN_POINT('Ctrl Pts',(8.6928249893351,3.5738163419672,135.498040590523));
#244205=CARTESIAN_POINT('Ctrl Pts',(2.86992050536337,8.26793953120299,135.762964533564));
#244206=CARTESIAN_POINT('Ctrl Pts',(-2.56152361166258,7.8499123324488,135.974903687997));
#244207=CARTESIAN_POINT('Ctrl Pts',(-7.21477125736058,4.96654145705927,
136.18684284243));
#244208=CARTESIAN_POINT('Ctrl Pts',(-8.72126827650654,-0.790103703246512,
136.398781996863));
#244209=CARTESIAN_POINT('Ctrl Pts',(-6.08193578826746,-5.59702881765901,
136.610721151296));
#244210=CARTESIAN_POINT('Ctrl Pts',(-2.67619958111933,-7.83950383357153,
136.769675517121));
#244211=CARTESIAN_POINT('Ctrl Pts',(1.3996162528399,-8.14590827035688,136.928629882946));
#244212=CARTESIAN_POINT('Ctrl Pts',(6.40936146784205,-5.95899205325436,
137.140569037379));
#244213=CARTESIAN_POINT('Ctrl Pts',(9.35170511633603,0.903656038138216,
137.40549298042));
#244214=CARTESIAN_POINT('Ctrl Pts',(4.27385822118494,8.36429562826514,137.723401712069));
#244215=CARTESIAN_POINT('Ctrl Pts',(-3.18692714972201,8.15337579492017,
137.988325655111));
#244216=CARTESIAN_POINT('Ctrl Pts',(-7.06372063712096,4.28927272083034,
138.200264809544));
#244217=CARTESIAN_POINT('Ctrl Pts',(-8.27206068517265,0.40045319240588,
138.359219175368));
#244218=CARTESIAN_POINT('Ctrl Pts',(-7.44413426218233,-3.62023136901316,
138.518180255724));
#244219=CARTESIAN_POINT('Ctrl Pts',(-5.68565861609716,-5.69747426071045,
138.624156547473));
#244220=CARTESIAN_POINT('Ctrl Pts',(-4.60940596141801,-6.46483699172352,
138.677148050613));
#244221=CARTESIAN_POINT('Ctrl Pts',(-3.42490370648437,7.13754033682952,
138.));
#244222=CARTESIAN_POINT('Ctrl Pts',(-3.60315378289199,7.03782110867972,
138.));
#244223=CARTESIAN_POINT('Ctrl Pts',(-3.77697596682028,6.93110617027609,
138.));
#244224=CARTESIAN_POINT('Ctrl Pts',(-3.94592285661015,6.81740720159191,
138.));
#244225=CARTESIAN_POINT('Ctrl Pts',(-4.11538230205325,6.70336328989492,
138.));
#244226=CARTESIAN_POINT('Ctrl Pts',(-4.27993741495876,6.5822926792708,138.));
#244227=CARTESIAN_POINT('Ctrl Pts',(-4.43932721728487,6.45467407365266,
138.));
#244228=CARTESIAN_POINT('Ctrl Pts',(-4.59985158806564,6.32614705330504,
138.));
#244229=CARTESIAN_POINT('Ctrl Pts',(-4.75513728704195,6.19097784029614,
138.));
#244230=CARTESIAN_POINT('Ctrl Pts',(-4.90487911920266,6.04961867430912,
138.));
#244231=CARTESIAN_POINT('Ctrl Pts',(-5.05399550788871,5.90884993897649,
138.));
#244232=CARTESIAN_POINT('Ctrl Pts',(-5.19761460421856,5.76194216159953,
138.));
#244233=CARTESIAN_POINT('Ctrl Pts',(-5.33539102092455,5.60931572741658,
138.));
#244234=CARTESIAN_POINT('Ctrl Pts',(-5.44873023956294,5.48376041680946,
138.));
#244235=CARTESIAN_POINT('Ctrl Pts',(-5.55811488447614,5.35433451946705,
138.));
#244236=CARTESIAN_POINT('Ctrl Pts',(-5.66332759072228,5.2212635732539,138.));
#244237=CARTESIAN_POINT('Ctrl Pts',(-5.67874041195431,5.20176974234377,
138.));
#244238=CARTESIAN_POINT('Ctrl Pts',(-5.69406497234922,5.18219598688969,
138.));
#244239=CARTESIAN_POINT('Ctrl Pts',(-5.70929635822883,5.1625484140524,138.));
#244240=CARTESIAN_POINT('Ctrl Pts',(-5.83335269592323,5.00252319047495,
138.));
#244241=CARTESIAN_POINT('Ctrl Pts',(-5.95094323302251,4.83797793878056,
138.));
#244242=CARTESIAN_POINT('Ctrl Pts',(-6.06181278565512,4.66936481397146,
138.));
#244243=CARTESIAN_POINT('Ctrl Pts',(-6.17280782281805,4.50056084922218,
138.));
#244244=CARTESIAN_POINT('Ctrl Pts',(-6.27706702203869,4.32767912330544,
138.));
#244245=CARTESIAN_POINT('Ctrl Pts',(-6.3742898456234,4.15114664381216,138.));
#244246=CARTESIAN_POINT('Ctrl Pts',(-6.41202336569123,4.08263195135644,
138.));
#244247=CARTESIAN_POINT('Ctrl Pts',(-6.44869647661346,4.01356710710628,
138.));
#244248=CARTESIAN_POINT('Ctrl Pts',(-6.48428962272322,3.9439763260544,138.));
#244249=CARTESIAN_POINT('Ctrl Pts',(-6.57620068165998,3.76427424636205,
138.));
#244250=CARTESIAN_POINT('Ctrl Pts',(-6.66091404102716,3.58106572388496,
138.));
#244251=CARTESIAN_POINT('Ctrl Pts',(-6.73826053739278,3.39476139218723,
138.));
#244252=CARTESIAN_POINT('Ctrl Pts',(-6.81486615435339,3.2102416150447,138.));
#244253=CARTESIAN_POINT('Ctrl Pts',(-6.88424542684704,3.0226844125455,138.));
#244254=CARTESIAN_POINT('Ctrl Pts',(-6.94618315954604,2.83248581782527,
138.));
#244255=CARTESIAN_POINT('Ctrl Pts',(-6.96453053523597,2.77614463578707,
138.));
#244256=CARTESIAN_POINT('Ctrl Pts',(-6.98222458498384,2.71957169207803,
138.));
#244257=CARTESIAN_POINT('Ctrl Pts',(-6.99925883342174,2.66277735691564,
138.));
#244258=CARTESIAN_POINT('Ctrl Pts',(-7.00951057192051,2.62859676630024,
138.));
#244259=CARTESIAN_POINT('Ctrl Pts',(-7.01952332218084,2.59433598864154,
138.));
#244260=CARTESIAN_POINT('Ctrl Pts',(-7.02929560087802,2.55999729648689,
138.));
#244261=CARTESIAN_POINT('Ctrl Pts',(-7.03613199613462,2.53597496971556,
138.));
#244262=CARTESIAN_POINT('Ctrl Pts',(-7.04284847966699,2.51192225244768,
138.));
#244263=CARTESIAN_POINT('Ctrl Pts',(-7.04944318094255,2.48784598206391,
138.));
#244264=CARTESIAN_POINT('Ctrl Pts',(-7.10167376413709,2.29715991597125,
138.));
#244265=CARTESIAN_POINT('Ctrl Pts',(-7.14630341841885,2.1048780735385,138.));
#244266=CARTESIAN_POINT('Ctrl Pts',(-7.18322675984256,1.91140034900355,
138.));
#244267=CARTESIAN_POINT('Ctrl Pts',(-7.22000686923813,1.71867315802871,
138.));
#244268=CARTESIAN_POINT('Ctrl Pts',(-7.24914041866994,1.524758701822,138.));
#244269=CARTESIAN_POINT('Ctrl Pts',(-7.27047217192691,1.33004595658973,
138.));
#244270=CARTESIAN_POINT('Ctrl Pts',(-7.29148754274809,1.13822109834324,
138.));
#244271=CARTESIAN_POINT('Ctrl Pts',(-7.30493081407415,0.945620872512938,
138.));
#244272=CARTESIAN_POINT('Ctrl Pts',(-7.3106035273759,0.752620165465328,
138.));
#244273=CARTESIAN_POINT('Ctrl Pts',(-7.31455505027739,0.618178907228735,
138.));
#244274=CARTESIAN_POINT('Ctrl Pts',(-7.31473503652726,0.483543379414253,
138.));
#244275=CARTESIAN_POINT('Ctrl Pts',(-7.3110617236461,0.348843391340057,
138.));
#244276=CARTESIAN_POINT('Ctrl Pts',(-7.30698329038145,0.199287682397503,
138.));
#244277=CARTESIAN_POINT('Ctrl Pts',(-7.29815477473225,0.0496521820743232,
138.));
#244278=CARTESIAN_POINT('Ctrl Pts',(-7.28460785612623,-0.099828577738282,
138.));
#244279=CARTESIAN_POINT('Ctrl Pts',(-7.27923431788771,-0.159121809072706,
138.));
#244280=CARTESIAN_POINT('Ctrl Pts',(-7.27311821566584,-0.218390598344035,
138.));
#244281=CARTESIAN_POINT('Ctrl Pts',(-7.26626087139555,-0.27761989288037,
138.));
#244282=CARTESIAN_POINT('Ctrl Pts',(-7.26368656164304,-0.299855111727345,
138.));
#244283=CARTESIAN_POINT('Ctrl Pts',(-7.26100889000677,-0.3220751844165,
138.));
#244284=CARTESIAN_POINT('Ctrl Pts',(-7.25822828218742,-0.344278585099771,
138.));
#244285=CARTESIAN_POINT('Ctrl Pts',(-7.23431083840358,-0.535261500402182,
138.));
#244286=CARTESIAN_POINT('Ctrl Pts',(-7.20277958541697,-0.725030926027641,
138.));
#244287=CARTESIAN_POINT('Ctrl Pts',(-7.163817492447,-0.913118345634504,
138.));
#244288=CARTESIAN_POINT('Ctrl Pts',(-7.12463947625704,-1.10224812303549,
138.));
#244289=CARTESIAN_POINT('Ctrl Pts',(-7.07794778369885,-1.28967793268298,
138.));
#244290=CARTESIAN_POINT('Ctrl Pts',(-7.0238779237268,-1.47491810765451,
138.));
#244291=CARTESIAN_POINT('Ctrl Pts',(-6.97016135742329,-1.65894791919977,
138.));
#244292=CARTESIAN_POINT('Ctrl Pts',(-6.90916240290187,-1.84081728860338,
138.));
#244293=CARTESIAN_POINT('Ctrl Pts',(-6.84096862416969,-2.02002252000683,
138.));
#244294=CARTESIAN_POINT('Ctrl Pts',(-6.77414302540993,-2.19563233533101,
138.));
#244295=CARTESIAN_POINT('Ctrl Pts',(-6.70040803332846,-2.36868437319925,
138.));
#244296=CARTESIAN_POINT('Ctrl Pts',(-6.61980768402212,-2.53867320106378,
138.));
#244297=CARTESIAN_POINT('Ctrl Pts',(-6.57470303536745,-2.63380041108253,
138.));
#244298=CARTESIAN_POINT('Ctrl Pts',(-6.52744775912282,-2.72796772928592,
138.));
#244299=CARTESIAN_POINT('Ctrl Pts',(-6.47804480086152,-2.82108121632785,
138.));
#244300=CARTESIAN_POINT('Ctrl Pts',(-6.46323930063093,-2.84898626093223,
138.));
#244301=CARTESIAN_POINT('Ctrl Pts',(-6.44824088784976,-2.87679662862212,
138.));
#244302=CARTESIAN_POINT('Ctrl Pts',(-6.43304958529191,-2.90450971444846,
138.));
#244303=CARTESIAN_POINT('Ctrl Pts',(-6.42219754347207,-2.92430680328918,
138.));
#244304=CARTESIAN_POINT('Ctrl Pts',(-6.41124835080748,-2.9440518496595,
138.));
#244305=CARTESIAN_POINT('Ctrl Pts',(-6.4002062787239,-2.96373661052125,
138.));
#244306=CARTESIAN_POINT('Ctrl Pts',(-6.37888604171424,-3.00174431087616,
138.));
#244307=CARTESIAN_POINT('Ctrl Pts',(-6.35721514239056,-3.03953534017548,
138.));
#244308=CARTESIAN_POINT('Ctrl Pts',(-6.33519494702275,-3.07710388684579,
138.));
#244309=CARTESIAN_POINT('Ctrl Pts',(-6.23932871838984,-3.2406607865165,
138.));
#244310=CARTESIAN_POINT('Ctrl Pts',(-6.13684529840294,-3.40000354179732,
138.));
#244311=CARTESIAN_POINT('Ctrl Pts',(-6.02808002948692,-3.55482687716532,
138.));
#244312=CARTESIAN_POINT('Ctrl Pts',(-5.91930392863085,-3.70966563139914,
138.));
#244313=CARTESIAN_POINT('Ctrl Pts',(-5.80424417060215,-3.85998451885378,
138.));
#244314=CARTESIAN_POINT('Ctrl Pts',(-5.68320070145349,-4.0054404017757,
138.));
#244315=CARTESIAN_POINT('Ctrl Pts',(-5.57833647525666,-4.13145396298363,
138.));
#244316=CARTESIAN_POINT('Ctrl Pts',(-5.46898049117472,-4.25381724526501,
138.));
#244317=CARTESIAN_POINT('Ctrl Pts',(-5.35531105443876,-4.37228026380955,
138.));
#244318=CARTESIAN_POINT('Ctrl Pts',(-5.33628706891599,-4.39210651451059,
138.));
#244319=CARTESIAN_POINT('Ctrl Pts',(-5.31714211142194,-4.41182350054872,
138.));
#244320=CARTESIAN_POINT('Ctrl Pts',(-5.29788733618046,-4.43141968005266,
138.));
#244321=CARTESIAN_POINT('Ctrl Pts',(-5.1670532765616,-4.56457354372363,
138.));
#244322=CARTESIAN_POINT('Ctrl Pts',(-5.0310357855152,-4.69227461210752,
138.));
#244323=CARTESIAN_POINT('Ctrl Pts',(-4.89014018822931,-4.8142080523858,
138.));
#244324=CARTESIAN_POINT('Ctrl Pts',(-4.75091868359083,-4.93469270448491,
138.));
#244325=CARTESIAN_POINT('Ctrl Pts',(-4.60693372766405,-5.04954629887319,
138.));
#244326=CARTESIAN_POINT('Ctrl Pts',(-4.4584541052344,-5.15842196959294,
138.));
#244327=CARTESIAN_POINT('Ctrl Pts',(-4.31052817018024,-5.26689163790383,
138.));
#244328=CARTESIAN_POINT('Ctrl Pts',(-4.15814051823896,-5.36942825198228,
138.));
#244329=CARTESIAN_POINT('Ctrl Pts',(-4.0015392161787,-5.46564050896491,
138.));
#244330=CARTESIAN_POINT('Ctrl Pts',(-3.97741995172579,-5.48045883320132,
138.));
#244331=CARTESIAN_POINT('Ctrl Pts',(-3.95320070856606,-5.49512703602489,
138.));
#244332=CARTESIAN_POINT('Ctrl Pts',(-3.92888236737319,-5.50964357679733,
138.));
#244333=CARTESIAN_POINT('Ctrl Pts',(-3.93307528793382,-5.51266228421142,
8.));
#244334=CARTESIAN_POINT('Ctrl Pts',(-4.08477702892364,-5.42354303040725,
8.));
#244335=CARTESIAN_POINT('Ctrl Pts',(-4.2326033773089,-5.32840285450346,
8.));
#244336=CARTESIAN_POINT('Ctrl Pts',(-4.37614884580116,-5.22732383700667,
8.));
#244337=CARTESIAN_POINT('Ctrl Pts',(-4.52451204222272,-5.12285236685515,
8.));
#244338=CARTESIAN_POINT('Ctrl Pts',(-4.66830321494952,-5.01203736235522,
8.));
#244339=CARTESIAN_POINT('Ctrl Pts',(-4.80734470112666,-4.89535635028057,
8.));
#244340=CARTESIAN_POINT('Ctrl Pts',(-4.90085472814102,-4.81688448629847,
8.));
#244341=CARTESIAN_POINT('Ctrl Pts',(-4.9922160791375,-4.73575833801607,
8.));
#244342=CARTESIAN_POINT('Ctrl Pts',(-5.08136863104384,-4.65211150438784,
8.));
#244343=CARTESIAN_POINT('Ctrl Pts',(-5.16684420744904,-4.57191457041387,
8.));
#244344=CARTESIAN_POINT('Ctrl Pts',(-5.25028943769945,-4.48940047532547,
8.));
#244345=CARTESIAN_POINT('Ctrl Pts',(-5.33164630104632,-4.4046799163009,
8.));
#244346=CARTESIAN_POINT('Ctrl Pts',(-5.36052043404078,-4.3746119836397,
8.));
#244347=CARTESIAN_POINT('Ctrl Pts',(-5.38911990294402,-4.34427800399018,
8.));
#244348=CARTESIAN_POINT('Ctrl Pts',(-5.41743426293231,-4.31369271508244,
8.));
#244349=CARTESIAN_POINT('Ctrl Pts',(-5.54469908345851,-4.17622072895257,
8.));
#244350=CARTESIAN_POINT('Ctrl Pts',(-5.66626061200855,-4.03361876143901,
8.));
#244351=CARTESIAN_POINT('Ctrl Pts',(-5.78192961588972,-3.88639015566724,
8.));
#244352=CARTESIAN_POINT('Ctrl Pts',(-5.89884602501638,-3.73757379752478,
8.));
#244353=CARTESIAN_POINT('Ctrl Pts',(-6.00974262846789,-3.58402994987003,
8.));
#244354=CARTESIAN_POINT('Ctrl Pts',(-6.11439363561345,-3.42623394506887,
8.));
#244355=CARTESIAN_POINT('Ctrl Pts',(-6.20326627145087,-3.29222905344095,
8.));
#244356=CARTESIAN_POINT('Ctrl Pts',(-6.2876342928174,-3.15515659780525,
7.99999999999999));
#244357=CARTESIAN_POINT('Ctrl Pts',(-6.36733843599083,-3.01528734055045,
8.));
#244358=CARTESIAN_POINT('Ctrl Pts',(-6.38616415319831,-2.98225092640356,
8.));
#244359=CARTESIAN_POINT('Ctrl Pts',(-6.40473029313281,-2.94905712598991,
8.));
#244360=CARTESIAN_POINT('Ctrl Pts',(-6.42303229992168,-2.91571354682276,
8.));
#244361=CARTESIAN_POINT('Ctrl Pts',(-6.4370381909391,-2.890196862159,8.));
#244362=CARTESIAN_POINT('Ctrl Pts',(-6.45088590547151,-2.86459878170226,
8.));
#244363=CARTESIAN_POINT('Ctrl Pts',(-6.46457090104649,-2.83892831167736,
8.));
#244364=CARTESIAN_POINT('Ctrl Pts',(-6.50871475005265,-2.75612277867679,
8.));
#244365=CARTESIAN_POINT('Ctrl Pts',(-6.55117967921877,-2.67253853642597,
8.));
#244366=CARTESIAN_POINT('Ctrl Pts',(-6.59194388268187,-2.58823590697107,
8.));
#244367=CARTESIAN_POINT('Ctrl Pts',(-6.67487547307193,-2.41672878697819,
8.));
#244368=CARTESIAN_POINT('Ctrl Pts',(-6.75077053581255,-2.24225053131111,
8.));
#244369=CARTESIAN_POINT('Ctrl Pts',(-6.81961261254839,-2.06524773591551,
8.));
#244370=CARTESIAN_POINT('Ctrl Pts',(-6.88950151585512,-1.88555340014043,
8.));
#244371=CARTESIAN_POINT('Ctrl Pts',(-6.9521216439269,-1.70325663984402,
8.));
#244372=CARTESIAN_POINT('Ctrl Pts',(-7.00741369037057,-1.51879182789295,
8.));
#244373=CARTESIAN_POINT('Ctrl Pts',(-7.0628309406438,-1.3339093120882,8.));
#244374=CARTESIAN_POINT('Ctrl Pts',(-7.11088715402154,-1.14684829515692,
8.));
#244375=CARTESIAN_POINT('Ctrl Pts',(-7.15147618870233,-0.958022046524551,
8.));
#244376=CARTESIAN_POINT('Ctrl Pts',(-7.19180261574612,-0.770417487822679,
8.));
#244377=CARTESIAN_POINT('Ctrl Pts',(-7.2247583831861,-0.581069823050405,
8.));
#244378=CARTESIAN_POINT('Ctrl Pts',(-7.25019015456882,-0.390370100156946,
8.));
#244379=CARTESIAN_POINT('Ctrl Pts',(-7.25461100843692,-0.357220399536,8.));
#244380=CARTESIAN_POINT('Ctrl Pts',(-7.25880438016642,-0.324029821772479,
8.));
#244381=CARTESIAN_POINT('Ctrl Pts',(-7.26276930380526,-0.290800398970626,
8.));
#244382=CARTESIAN_POINT('Ctrl Pts',(-7.26536291111864,-0.269063770009185,
8.));
#244383=CARTESIAN_POINT('Ctrl Pts',(-7.2678582400438,-0.247314718960559,
8.));
#244384=CARTESIAN_POINT('Ctrl Pts',(-7.27025432548459,-0.225561724677436,
8.));
#244385=CARTESIAN_POINT('Ctrl Pts',(-7.29190456618673,-0.029008816252474,
8.));
#244386=CARTESIAN_POINT('Ctrl Pts',(-7.30547920730303,0.168056767898447,
8.));
#244387=CARTESIAN_POINT('Ctrl Pts',(-7.31093639138176,0.365179631119353,
8.));
#244388=CARTESIAN_POINT('Ctrl Pts',(-7.31601373382377,0.548581961934194,
8.));
#244389=CARTESIAN_POINT('Ctrl Pts',(-7.31406402678812,0.732034590064997,
8.));
#244390=CARTESIAN_POINT('Ctrl Pts',(-7.30501644905688,0.915186995232694,
8.));
#244391=CARTESIAN_POINT('Ctrl Pts',(-7.29543570235443,1.10913247478293,
8.));
#244392=CARTESIAN_POINT('Ctrl Pts',(-7.27789678584438,1.30274173829146,
8.));
#244393=CARTESIAN_POINT('Ctrl Pts',(-7.25262567498423,1.49556132410732,
8.));
#244394=CARTESIAN_POINT('Ctrl Pts',(-7.22706505774481,1.69058985516706,
8.));
#244395=CARTESIAN_POINT('Ctrl Pts',(-7.19359401339139,1.88481121070243,
8.));
#244396=CARTESIAN_POINT('Ctrl Pts',(-7.15239307289344,2.07775770668224,
8.00000000000001));
#244397=CARTESIAN_POINT('Ctrl Pts',(-7.12126212790101,2.22354580472647,
8.00000000000001));
#244398=CARTESIAN_POINT('Ctrl Pts',(-7.08571697074218,2.36860617775617,
8.));
#244399=CARTESIAN_POINT('Ctrl Pts',(-7.04581601192821,2.51273388279635,
8.));
#244400=CARTESIAN_POINT('Ctrl Pts',(-7.03758572487512,2.54246280210164,
8.));
#244401=CARTESIAN_POINT('Ctrl Pts',(-7.0291688248226,2.5721560492647,8.));
#244402=CARTESIAN_POINT('Ctrl Pts',(-7.02057375510083,2.60178484484585,
8.));
#244403=CARTESIAN_POINT('Ctrl Pts',(-6.96487859664556,2.79377636069724,
8.));
#244404=CARTESIAN_POINT('Ctrl Pts',(-6.90165155752994,2.98326793251129,
8.));
#244405=CARTESIAN_POINT('Ctrl Pts',(-6.83116652485267,3.16979076589306,
8.));
#244406=CARTESIAN_POINT('Ctrl Pts',(-6.7599815615844,3.35816580863119,8.));
#244407=CARTESIAN_POINT('Ctrl Pts',(-6.68139363798646,3.54351357239222,
8.));
#244408=CARTESIAN_POINT('Ctrl Pts',(-6.59563147485587,3.72535328419925,
8.));
#244409=CARTESIAN_POINT('Ctrl Pts',(-6.50963684921469,3.90768588138123,
8.00000000000001));
#244410=CARTESIAN_POINT('Ctrl Pts',(-6.41642887221547,4.08649212780057,
8.00000000000001));
#244411=CARTESIAN_POINT('Ctrl Pts',(-6.31618684025996,4.26127846250173,
8.00000000000001));
#244412=CARTESIAN_POINT('Ctrl Pts',(-6.27693611103826,4.32971772855785,
8.00000000000001));
#244413=CARTESIAN_POINT('Ctrl Pts',(-6.23660638793653,4.39754050986302,
8.));
#244414=CARTESIAN_POINT('Ctrl Pts',(-6.19520638596164,4.46471642251084,
8.));
#244415=CARTESIAN_POINT('Ctrl Pts',(-6.08977872012769,4.63578403924718,
8.));
#244416=CARTESIAN_POINT('Ctrl Pts',(-5.97741342575072,4.80265872580366,
8.00000000000001));
#244417=CARTESIAN_POINT('Ctrl Pts',(-5.85843694593526,4.96505810776332,
8.));
#244418=CARTESIAN_POINT('Ctrl Pts',(-5.83953977033486,4.99085219448575,
8.));
#244419=CARTESIAN_POINT('Ctrl Pts',(-5.82047572315112,5.0165333219891,8.));
#244420=CARTESIAN_POINT('Ctrl Pts',(-5.80124601398966,5.04210028898929,
8.));
#244421=CARTESIAN_POINT('Ctrl Pts',(-5.78077292230514,5.06932040215351,
8.));
#244422=CARTESIAN_POINT('Ctrl Pts',(-5.76011205307566,5.09641111474705,
8.00000000000001));
#244423=CARTESIAN_POINT('Ctrl Pts',(-5.73926483449688,5.12337095070669,
8.));
#244424=CARTESIAN_POINT('Ctrl Pts',(-5.71429336715346,5.15566430728594,
8.));
#244425=CARTESIAN_POINT('Ctrl Pts',(-5.68904997949879,5.18777534729725,
8.));
#244426=CARTESIAN_POINT('Ctrl Pts',(-5.66356734128388,5.21966427514444,
8.));
#244427=CARTESIAN_POINT('Ctrl Pts',(-5.53736200954869,5.37759740136523,
8.00000000000001));
#244428=CARTESIAN_POINT('Ctrl Pts',(-5.40516318792086,5.5302553487043,8.));
#244429=CARTESIAN_POINT('Ctrl Pts',(-5.26739364824614,5.67740877299484,
8.));
#244430=CARTESIAN_POINT('Ctrl Pts',(-5.12711751743733,5.82723951964233,
8.));
#244431=CARTESIAN_POINT('Ctrl Pts',(-4.98106582098125,5.971364160092,8.));
#244432=CARTESIAN_POINT('Ctrl Pts',(-4.82963500543593,6.10951954978689,
8.));
#244433=CARTESIAN_POINT('Ctrl Pts',(-4.67771471353531,6.24812150510563,
8.));
#244434=CARTESIAN_POINT('Ctrl Pts',(-4.52038003859389,6.38071607588409,
8.));
#244435=CARTESIAN_POINT('Ctrl Pts',(-4.35798729149729,6.50700863540348,
8.));
#244436=CARTESIAN_POINT('Ctrl Pts',(-4.19674147632236,6.63240922794422,
8.));
#244437=CARTESIAN_POINT('Ctrl Pts',(-4.03050829304627,6.75159697672051,
8.));
#244438=CARTESIAN_POINT('Ctrl Pts',(-3.85960026731181,6.86424773665911,
8.));
#244439=CARTESIAN_POINT('Ctrl Pts',(-3.71651503581681,6.95855963333356,
8.));
#244440=CARTESIAN_POINT('Ctrl Pts',(-3.57015237858456,7.04828919588474,
8.));
#244441=CARTESIAN_POINT('Ctrl Pts',(-3.42067962509762,7.13322310757501,
7.99999999999999));
#244442=CARTESIAN_POINT('Ctrl Pts',(4.60640650704272,-6.46396313977181,
7.32419035487299));
#244443=CARTESIAN_POINT('Ctrl Pts',(5.68304415359234,-5.69672795305586,
7.3772077233627));
#244444=CARTESIAN_POINT('Ctrl Pts',(7.44170011697942,-3.61976711392297,
7.48320988046067));
#244445=CARTESIAN_POINT('Ctrl Pts',(8.2695054703986,0.400329493614926,7.64219682616689));
#244446=CARTESIAN_POINT('Ctrl Pts',(7.06153867496872,4.28794777733252,7.80115119199166));
#244447=CARTESIAN_POINT('Ctrl Pts',(3.18594271746802,8.15085724155371,8.01309034642465));
#244448=CARTESIAN_POINT('Ctrl Pts',(-4.27253803917999,8.36171192239284,
8.27801428946594));
#244449=CARTESIAN_POINT('Ctrl Pts',(-9.34881640263045,0.90337690149306,
8.59592302111545));
#244450=CARTESIAN_POINT('Ctrl Pts',(-6.40738163527747,-5.9571513384547,
8.86084696415672));
#244451=CARTESIAN_POINT('Ctrl Pts',(-1.39918391556983,-8.14339202368617,
9.07278611858973));
#244452=CARTESIAN_POINT('Ctrl Pts',(2.67537291108373,-7.83708223431333,
9.2317404844145));
#244453=CARTESIAN_POINT('Ctrl Pts',(6.08005709651601,-5.59529991221756,
9.39069485023925));
#244454=CARTESIAN_POINT('Ctrl Pts',(8.71857430285288,-0.789859642577828,
9.60263400467228));
#244455=CARTESIAN_POINT('Ctrl Pts',(7.21254263612409,4.96500730727687,9.81457315910527));
#244456=CARTESIAN_POINT('Ctrl Pts',(2.56073236468874,7.84748751803708,10.0265123135383));
#244457=CARTESIAN_POINT('Ctrl Pts',(-2.86903399551457,8.2653855894407,10.2384514679713));
#244458=CARTESIAN_POINT('Ctrl Pts',(-8.69013980172793,3.57271240080031,
10.5033754110126));
#244459=CARTESIAN_POINT('Ctrl Pts',(-7.68563380952286,-5.39282503599071,
10.8212841426621));
#244460=CARTESIAN_POINT('Ctrl Pts',(-0.995348383535201,-8.69250838977446,
11.0862080857034));
#244461=CARTESIAN_POINT('Ctrl Pts',(4.2336755651751,-7.09606290023127,11.2981472401364));
#244462=CARTESIAN_POINT('Ctrl Pts',(7.12846088456057,-4.21382949912462,
11.4571016059612));
#244463=CARTESIAN_POINT('Ctrl Pts',(8.25773673872998,-0.296618493249961,
11.6160559717859));
#244464=CARTESIAN_POINT('Ctrl Pts',(7.13669833548613,5.06972137834538,11.8279951262189));
#244465=CARTESIAN_POINT('Ctrl Pts',(2.25043748671926,8.46216402683687,12.0399342806519));
#244466=CARTESIAN_POINT('Ctrl Pts',(-3.15802887272445,7.6267562205539,12.251873435085));
#244467=CARTESIAN_POINT('Ctrl Pts',(-7.55455441577774,4.41319586680862,
12.4638125895179));
#244468=CARTESIAN_POINT('Ctrl Pts',(-8.92501441489603,-2.93721198242924,
12.7287365325592));
#244469=CARTESIAN_POINT('Ctrl Pts',(-2.3315165987433,-9.0948059072455,13.0466452642087));
#244470=CARTESIAN_POINT('Ctrl Pts',(4.89668847883403,-7.25071229477944,
13.31156920725));
#244471=CARTESIAN_POINT('Ctrl Pts',(7.83083558801256,-2.63745359024292,
13.523508361683));
#244472=CARTESIAN_POINT('Ctrl Pts',(8.1555641278621,1.43459714924663,13.6824627275078));
#244473=CARTESIAN_POINT('Ctrl Pts',(6.46603855843502,5.1447596198217,13.8414170933326));
#244474=CARTESIAN_POINT('Ctrl Pts',(2.12463370076545,8.49237698071761,14.0533562477656));
#244475=CARTESIAN_POINT('Ctrl Pts',(-3.7934454125899,7.89192369888149,14.2652954021985));
#244476=CARTESIAN_POINT('Ctrl Pts',(-7.35881389526889,3.74010908684348,
14.4772345566316));
#244477=CARTESIAN_POINT('Ctrl Pts',(-8.60890508199618,-1.56023792552856,
14.6891737110646));
#244478=CARTESIAN_POINT('Ctrl Pts',(-4.86995472333722,-8.03533682977006,
14.9540976541059));
#244479=CARTESIAN_POINT('Ctrl Pts',(4.1432659185206,-8.42524847071499,15.2720063857554));
#244480=CARTESIAN_POINT('Ctrl Pts',(8.43507380939552,-2.32377204262004,
15.5369303287966));
#244481=CARTESIAN_POINT('Ctrl Pts',(7.66400379406276,3.08888221979113,15.7488694832297));
#244482=CARTESIAN_POINT('Ctrl Pts',(5.26259331597973,6.39346594447912,15.9078238490544));
#244483=CARTESIAN_POINT('Ctrl Pts',(1.56635676098601,8.1132442764234,16.0667782148792));
#244484=CARTESIAN_POINT('Ctrl Pts',(-3.90866261554707,7.83306400513209,
16.2787173693122));
#244485=CARTESIAN_POINT('Ctrl Pts',(-8.01396100145449,3.5283306005865,16.4906565237452));
#244486=CARTESIAN_POINT('Ctrl Pts',(-8.02249192943588,-1.94426880137432,
16.7025956781782));
#244487=CARTESIAN_POINT('Ctrl Pts',(-5.52527675051475,-6.78372360311353,
16.9145348326112));
#244488=CARTESIAN_POINT('Ctrl Pts',(1.52591029648008,-9.27117547791387,
17.1794587756525));
#244489=CARTESIAN_POINT('Ctrl Pts',(8.62653528067062,-3.70598884469431,
17.4973675073021));
#244490=CARTESIAN_POINT('Ctrl Pts',(7.91903429724152,3.72011861030341,17.7622914503433));
#244491=CARTESIAN_POINT('Ctrl Pts',(3.81337169451136,7.33050774795007,17.9742306047763));
#244492=CARTESIAN_POINT('Ctrl Pts',(-0.159909493655665,8.27923451452099,
18.1331849706011));
#244493=CARTESIAN_POINT('Ctrl Pts',(-4.08621421445045,7.18199551553807,
18.2921393364258));
#244494=CARTESIAN_POINT('Ctrl Pts',(-8.06321083680452,3.4086897999003,18.5040784908588));
#244495=CARTESIAN_POINT('Ctrl Pts',(-8.38246493369623,-2.53119920101162,
18.7160176452919));
#244496=CARTESIAN_POINT('Ctrl Pts',(-4.83005780802961,-6.69410931349035,
18.9279567997249));
#244497=CARTESIAN_POINT('Ctrl Pts',(0.214145694079805,-8.74652678009534,
19.1398959541579));
#244498=CARTESIAN_POINT('Ctrl Pts',(7.18832724386593,-6.05070643894309,
19.4048198971992));
#244499=CARTESIAN_POINT('Ctrl Pts',(8.96335141509527,2.79460116567021,19.7227286288486));
#244500=CARTESIAN_POINT('Ctrl Pts',(3.59661084838262,7.97588722844733,19.98765257189));
#244501=CARTESIAN_POINT('Ctrl Pts',(-1.87020571352034,8.04863206466617,
20.1995917263229));
#244502=CARTESIAN_POINT('Ctrl Pts',(-5.50554978380011,6.18548436023368,
20.3585460921477));
#244503=CARTESIAN_POINT('Ctrl Pts',(-7.77469467530229,2.79862982500579,
20.5175004579725));
#244504=CARTESIAN_POINT('Ctrl Pts',(-8.34207484510865,-2.65411424571596,
20.7294396124055));
#244505=CARTESIAN_POINT('Ctrl Pts',(-4.72183113573663,-7.37407611063491,
20.9413787668385));
#244506=CARTESIAN_POINT('Ctrl Pts',(0.684004653885784,-8.22634156617198,
21.1533179212715));
#244507=CARTESIAN_POINT('Ctrl Pts',(5.85063630387345,-6.50520129842388,
21.3652570757045));
#244508=CARTESIAN_POINT('Ctrl Pts',(9.39558383634547,0.0781111347793227,
21.6301810187458));
#244509=CARTESIAN_POINT('Ctrl Pts',(4.99181938924929,7.95193080017495,21.9480897503953));
#244510=CARTESIAN_POINT('Ctrl Pts',(-2.45456906825707,8.39794482982405,
22.2130136934366));
#244511=CARTESIAN_POINT('Ctrl Pts',(-6.65484510472912,4.89807963954436,
22.4249528478696));
#244512=CARTESIAN_POINT('Ctrl Pts',(-8.20487797662277,1.11860295964548,
22.5839072136944));
#244513=CARTESIAN_POINT('Ctrl Pts',(-7.72616986326117,-2.92993266742093,
22.7428615795191));
#244514=CARTESIAN_POINT('Ctrl Pts',(-4.61121512984712,-7.44118472939463,
22.9548007339522));
#244515=CARTESIAN_POINT('Ctrl Pts',(1.20841048463845,-8.67251012455243,
23.1667398883851));
#244516=CARTESIAN_POINT('Ctrl Pts',(5.86929163264628,-5.80447875875298,
23.3786790428182));
#244517=CARTESIAN_POINT('Ctrl Pts',(8.67494461835349,-1.13706858267993,
23.5906181972512));
#244518=CARTESIAN_POINT('Ctrl Pts',(7.08673429158096,6.16938360419446,23.8555421402925));
#244519=CARTESIAN_POINT('Ctrl Pts',(-1.37909372589059,9.28706437798646,
24.173450871942));
#244520=CARTESIAN_POINT('Ctrl Pts',(-7.3259293348859,4.78342409324861,24.4383748149832));
#244521=CARTESIAN_POINT('Ctrl Pts',(-8.24074907476951,-0.606796679244106,
24.6503139694162));
#244522=CARTESIAN_POINT('Ctrl Pts',(-6.96042785497538,-4.48594909336698,
24.809268335241));
#244523=CARTESIAN_POINT('Ctrl Pts',(-3.96396384261985,-7.2501859869929,
24.9682227010657));
#244524=CARTESIAN_POINT('Ctrl Pts',(1.33608342634073,-8.65155571146394,
25.1801618554988));
#244525=CARTESIAN_POINT('Ctrl Pts',(6.55781433047578,-5.80239252092228,
25.3921010099317));
#244526=CARTESIAN_POINT('Ctrl Pts',(8.23342939650299,-0.592619863543954,
25.6040401643649));
#244527=CARTESIAN_POINT('Ctrl Pts',(7.32953114506682,4.77761052061731,25.8159793187978));
#244528=CARTESIAN_POINT('Ctrl Pts',(1.37155632862688,9.29526385922294,26.0809032618391));
#244529=CARTESIAN_POINT('Ctrl Pts',(-7.08712800903743,6.15825306797093,
26.3988119934886));
#244530=CARTESIAN_POINT('Ctrl Pts',(-8.67598906217926,-1.13030989934556,
26.6637359365299));
#244531=CARTESIAN_POINT('Ctrl Pts',(-5.86563283358155,-5.82000850384829,
26.8756750909629));
#244532=CARTESIAN_POINT('Ctrl Pts',(-2.37036010048857,-7.93427300933166,
27.0346294567876));
#244533=CARTESIAN_POINT('Ctrl Pts',(1.70357150606366,-8.08554576483948,
27.1935838226124));
#244534=CARTESIAN_POINT('Ctrl Pts',(6.64117659469234,-5.70344707951407,
27.4055229770454));
#244535=CARTESIAN_POINT('Ctrl Pts',(8.75512182332181,-0.14328160608686,
27.6174621314784));
#244536=CARTESIAN_POINT('Ctrl Pts',(6.64006524501561,4.9040892601789,27.8294012859115));
#244537=CARTESIAN_POINT('Ctrl Pts',(2.46108587685203,8.39587073506834,28.0413404403444));
#244538=CARTESIAN_POINT('Ctrl Pts',(-5.00287752104787,7.95325804212126,
28.3062643833857));
#244539=CARTESIAN_POINT('Ctrl Pts',(-9.38864462872237,0.0693995765018132,
28.6241731150352));
#244540=CARTESIAN_POINT('Ctrl Pts',(-5.85582497657862,-6.50074615096535,
28.8890970580765));
#244541=CARTESIAN_POINT('Ctrl Pts',(-0.671126025509802,-8.2357596723763,
29.1010362125095));
#244542=CARTESIAN_POINT('Ctrl Pts',(3.359051199195,-7.56888830897797,29.2599905783343));
#244543=CARTESIAN_POINT('Ctrl Pts',(6.55226367610338,-5.03448576424663,
29.4189449441591));
#244544=CARTESIAN_POINT('Ctrl Pts',(8.75410428400366,-0.0139045135065831,
29.630884098592));
#244545=CARTESIAN_POINT('Ctrl Pts',(6.74416934134095,5.58469942388712,29.842823253025));
#244546=CARTESIAN_POINT('Ctrl Pts',(1.85506979875823,8.04358589011153,30.0547624074581));
#244547=CARTESIAN_POINT('Ctrl Pts',(-3.59031142780148,7.97854955142952,
30.266701561891));
#244548=CARTESIAN_POINT('Ctrl Pts',(-8.97261505059773,2.78841821270769,
30.5316255049324));
#244549=CARTESIAN_POINT('Ctrl Pts',(-7.17739052902341,-6.05281169866873,
30.8495342365819));
#244550=CARTESIAN_POINT('Ctrl Pts',(-0.220984594540438,-8.74651659145448,
31.1144581796232));
#244551=CARTESIAN_POINT('Ctrl Pts',(4.84596599019363,-6.69288884900557,
31.3263973340562));
#244552=CARTESIAN_POINT('Ctrl Pts',(7.47389207938856,-3.56542176723172,
31.4853516998809));
#244553=CARTESIAN_POINT('Ctrl Pts',(8.25152748533976,0.436463458113405,
31.6443060657057));
#244554=CARTESIAN_POINT('Ctrl Pts',(6.65926109162368,5.6823214326799,31.8562452201387));
#244555=CARTESIAN_POINT('Ctrl Pts',(1.49154661474766,8.62832408152842,32.0681843745717));
#244556=CARTESIAN_POINT('Ctrl Pts',(-3.82158839556387,7.3168312857929,32.2801235290048));
#244557=CARTESIAN_POINT('Ctrl Pts',(-7.91598016080529,3.7262376718286,32.4920626834377));
#244558=CARTESIAN_POINT('Ctrl Pts',(-8.6295517363744,-3.71671007806775,
32.7569866264791));
#244559=CARTESIAN_POINT('Ctrl Pts',(-1.51623294465423,-9.26566251938852,
33.0748953581285));
#244560=CARTESIAN_POINT('Ctrl Pts',(5.52007482625293,-6.78816327058959,
33.3398193011698));
#244561=CARTESIAN_POINT('Ctrl Pts',(8.03378319654136,-1.93299639788226,
33.5517584556028));
#244562=CARTESIAN_POINT('Ctrl Pts',(7.996312256756,2.15180981618979,33.7107128214276));
#244563=CARTESIAN_POINT('Ctrl Pts',(5.98459030406109,5.6976210021485,33.8696671872523));
#244564=CARTESIAN_POINT('Ctrl Pts',(1.36355987815356,8.64726775400164,34.0816063416853));
#244565=CARTESIAN_POINT('Ctrl Pts',(-4.47800684634566,7.524635701742,34.2935454961184));
#244566=CARTESIAN_POINT('Ctrl Pts',(-7.66135182018962,3.07314923444068,
34.5054846505514));
#244567=CARTESIAN_POINT('Ctrl Pts',(-8.43673296636848,-2.31713744680997,
34.7174238049844));
#244568=CARTESIAN_POINT('Ctrl Pts',(-4.13858529690325,-8.43535468818172,
34.9823477480256));
#244569=CARTESIAN_POINT('Ctrl Pts',(4.87372117073586,-8.02485552614977,
35.3002564796752));
#244570=CARTESIAN_POINT('Ctrl Pts',(8.60784050446359,-1.56699346690693,
35.5651804227164));
#244571=CARTESIAN_POINT('Ctrl Pts',(7.36006095721478,3.75601520621774,35.7771195771495));
#244572=CARTESIAN_POINT('Ctrl Pts',(4.67520386931402,6.83474681118095,35.9360739429742));
#244573=CARTESIAN_POINT('Ctrl Pts',(0.841084144012684,8.22014498985731,
36.095028308799));
#244574=CARTESIAN_POINT('Ctrl Pts',(-4.58755362703686,7.45579552226102,
36.306967463232));
#244575=CARTESIAN_POINT('Ctrl Pts',(-8.29514971181719,2.80413605561278,
36.518906617665));
#244576=CARTESIAN_POINT('Ctrl Pts',(-7.81858964795988,-2.64768084305508,
36.730845772098));
#244577=CARTESIAN_POINT('Ctrl Pts',(-4.90226342584214,-7.24675116151151,
36.942784926531));
#244578=CARTESIAN_POINT('Ctrl Pts',(2.3416444799405,-9.09943943903892,37.2077088695723));
#244579=CARTESIAN_POINT('Ctrl Pts',(8.92105959839902,-2.926800284862,37.5256176012218));
#244580=CARTESIAN_POINT('Ctrl Pts',(7.55813883548847,4.40737155446349,37.7905415442631));
#244581=CARTESIAN_POINT('Ctrl Pts',(3.14863238283442,7.63965062296849,38.0024806986961));
#244582=CARTESIAN_POINT('Ctrl Pts',(-0.893100355538415,8.23247635572276,
38.1614350645209));
#244583=CARTESIAN_POINT('Ctrl Pts',(-4.70669974170726,6.79155238019986,
38.3203894303456));
#244584=CARTESIAN_POINT('Ctrl Pts',(-8.33360149172359,2.68060092662989,
38.5323285847787));
#244585=CARTESIAN_POINT('Ctrl Pts',(-8.12512401220396,-3.26420703175445,
38.7442677392116));
#244586=CARTESIAN_POINT('Ctrl Pts',(-4.21772352936819,-7.09586965492464,
38.9562068936447));
#244587=CARTESIAN_POINT('Ctrl Pts',(0.988540998120691,-8.69312232677373,
39.1681460480777));
#244588=CARTESIAN_POINT('Ctrl Pts',(7.6963332375881,-5.38976360067576,39.4330699911189));
#244589=CARTESIAN_POINT('Ctrl Pts',(8.68037796208286,3.57805851000828,39.7509787227685));
#244590=CARTESIAN_POINT('Ctrl Pts',(2.87552219543382,8.26327772613146,40.0159026658097));
#244591=CARTESIAN_POINT('Ctrl Pts',(-2.57622614712117,7.8511913976253,40.2278418202428));
#244592=CARTESIAN_POINT('Ctrl Pts',(-6.03212460513054,5.67316207601861,
40.3867961860675));
#244593=CARTESIAN_POINT('Ctrl Pts',(-7.99214890082263,2.09851426934996,
40.5457505518923));
#244594=CARTESIAN_POINT('Ctrl Pts',(-8.07399845725793,-3.38305838892906,
40.7576897063253));
#244595=CARTESIAN_POINT('Ctrl Pts',(-4.04965474926068,-7.76356774760414,
40.9696288607583));
#244596=CARTESIAN_POINT('Ctrl Pts',(1.41044471838918,-8.13333902073644,
41.1815680151913));
#244597=CARTESIAN_POINT('Ctrl Pts',(6.40419069553413,-5.96103435893907,
41.3935071696244));
#244598=CARTESIAN_POINT('Ctrl Pts',(9.35168213791974,0.910570242477697,
41.6584311126656));
#244599=CARTESIAN_POINT('Ctrl Pts',(4.26736293265541,8.36307825305098,41.9763398443152));
#244600=CARTESIAN_POINT('Ctrl Pts',(-3.1892505363311,8.14733500551711,42.2412637873563));
#244601=CARTESIAN_POINT('Ctrl Pts',(-7.06278901428503,4.28895778283618,
42.4532029417895));
#244602=CARTESIAN_POINT('Ctrl Pts',(-8.27173191327942,0.386970732009184,
42.6121573076141));
#244603=CARTESIAN_POINT('Ctrl Pts',(-7.4360706647855,-3.60320125165142,
42.771111673439));
#244604=CARTESIAN_POINT('Ctrl Pts',(-3.93352600370737,-7.82060792578586,
42.9830508278718));
#244605=CARTESIAN_POINT('Ctrl Pts',(1.9723322591907,-8.53127148901054,43.194989982305));
#244606=CARTESIAN_POINT('Ctrl Pts',(6.36066488331213,-5.26141617552407,
43.4069291367379));
#244607=CARTESIAN_POINT('Ctrl Pts',(8.7415851819939,-0.363699875120048,
43.618868291171));
#244608=CARTESIAN_POINT('Ctrl Pts',(6.51202680730175,6.77322698838271,43.8837922342122));
#244609=CARTESIAN_POINT('Ctrl Pts',(-2.19681403260211,9.12827871900386,
44.2017009658618));
#244610=CARTESIAN_POINT('Ctrl Pts',(-7.72106968360267,4.11527272687538,
44.466624908903));
#244611=CARTESIAN_POINT('Ctrl Pts',(-8.15453306347553,-1.33481760549541,
44.6785640633361));
#244612=CARTESIAN_POINT('Ctrl Pts',(-6.53542671722701,-5.0852229859026,
44.8375184291608));
#244613=CARTESIAN_POINT('Ctrl Pts',(-3.30575106693872,-7.5729925442337,
44.9964727949856));
#244614=CARTESIAN_POINT('Ctrl Pts',(2.09764544585784,-8.49908340553139,
45.2084119494186));
#244615=CARTESIAN_POINT('Ctrl Pts',(7.04629283569648,-5.1983117483911,45.4203511038516));
#244616=CARTESIAN_POINT('Ctrl Pts',(8.2535510691205,0.139472862184186,45.6322902582846));
#244617=CARTESIAN_POINT('Ctrl Pts',(6.87722625139314,5.40845155107887,45.8442294127176));
#244618=CARTESIAN_POINT('Ctrl Pts',(0.542283475490215,9.38024656431713,
46.1091533557589));
#244619=CARTESIAN_POINT('Ctrl Pts',(-7.60506456392797,5.50585663127388,
46.4270620874084));
#244620=CARTESIAN_POINT('Ctrl Pts',(-8.54165908809657,-1.89484740766892,
46.6919860304496));
#244621=CARTESIAN_POINT('Ctrl Pts',(-5.32669771709283,-6.31699603878098,
46.9039251848827));
#244622=CARTESIAN_POINT('Ctrl Pts',(-1.65778605748533,-8.11313999510693,
47.0628795507074));
#244623=CARTESIAN_POINT('Ctrl Pts',(2.41351956808077,-7.90272924286775,
47.2218339165322));
#244624=CARTESIAN_POINT('Ctrl Pts',(7.12055709626584,-5.09236701245357,
47.4337730709653));
#244625=CARTESIAN_POINT('Ctrl Pts',(8.73336369099004,0.633282244141819,
47.6457122253982));
#244626=CARTESIAN_POINT('Ctrl Pts',(6.17926360329026,5.47332250565583,47.8576513798313));
#244627=CARTESIAN_POINT('Ctrl Pts',(1.70724159043718,8.5809623728985,48.0695905342643));
#244628=CARTESIAN_POINT('Ctrl Pts',(-5.68811526363237,7.478532056681,48.3345144773055));
#244629=CARTESIAN_POINT('Ctrl Pts',(-9.35784467962813,-0.763025043894934,
48.6524232089551));
#244630=CARTESIAN_POINT('Ctrl Pts',(-5.25659207975775,-6.99418518361079,
48.9173471519963));
#244631=CARTESIAN_POINT('Ctrl Pts',(0.0614822199421796,-8.26283047507858,
49.1292863064293));
#244632=CARTESIAN_POINT('Ctrl Pts',(4.01669042628314,-7.24137371028467,
49.2882406722541));
#244633=CARTESIAN_POINT('Ctrl Pts',(6.97270151424152,-4.43391923526801,
49.4471950380788));
#244634=CARTESIAN_POINT('Ctrl Pts',(8.7208829698701,0.762059955998786,49.6591341925119));
#244635=CARTESIAN_POINT('Ctrl Pts',(6.22263289279893,6.16048112092758,49.8710733469448));
#244636=CARTESIAN_POINT('Ctrl Pts',(1.13483497661836,8.17635050041949,50.083012501378));
#244637=CARTESIAN_POINT('Ctrl Pts',(-4.28335032160907,7.62892516122616,
50.2949516558109));
#244638=CARTESIAN_POINT('Ctrl Pts',(-9.18444949980501,1.98216658248081,
50.5598755988522));
#244639=CARTESIAN_POINT('Ctrl Pts',(-6.61265846080802,-6.6651490865816,
50.8777843305017));
#244640=CARTESIAN_POINT('Ctrl Pts',(0.555122358467198,-8.73167943998994,
51.1427082735429));
#244641=CARTESIAN_POINT('Ctrl Pts',(5.42010995078664,-6.23703099596596,
51.354647427976));
#244642=CARTESIAN_POINT('Ctrl Pts',(7.76049388307317,-2.88894961592975,
51.5136017938007));
#244643=CARTESIAN_POINT('Ctrl Pts',(8.18036633808948,1.16611010039288,51.6725561596255));
#244644=CARTESIAN_POINT('Ctrl Pts',(6.12940620636044,6.25019317366569,51.8844953140585));
#244645=CARTESIAN_POINT('Ctrl Pts',(0.720914936547745,8.72656687444214,
52.0964344684915));
#244646=CARTESIAN_POINT('Ctrl Pts',(-4.45506642661906,6.94931227275606,
52.3083736229245));
#244647=CARTESIAN_POINT('Ctrl Pts',(-8.21509575723348,3.00994863622323,
52.5203127773576));
#244648=CARTESIAN_POINT('Ctrl Pts',(-8.26616198646753,-4.46695231546649,
52.7852367203988));
#244649=CARTESIAN_POINT('Ctrl Pts',(-0.689014364486892,-9.36358496897353,
53.1031454520484));
#244650=CARTESIAN_POINT('Ctrl Pts',(6.10001021798649,-6.27218159941767,
53.3680693950896));
#244651=CARTESIAN_POINT('Ctrl Pts',(8.17349332006236,-1.2133237285046,53.5800085495226));
#244652=CARTESIAN_POINT('Ctrl Pts',(7.77411785726235,2.85208462952825,53.7389629153473));
#244653=CARTESIAN_POINT('Ctrl Pts',(5.45603467637146,6.20563387590808,53.8979172811722));
#244654=CARTESIAN_POINT('Ctrl Pts',(0.59175287007345,8.734092035894,54.1098564356051));
#244655=CARTESIAN_POINT('Ctrl Pts',(-5.12731989678988,7.09811795026197,
54.3217955900382));
#244656=CARTESIAN_POINT('Ctrl Pts',(-7.90358383695811,2.38199925735514,
54.5337347444712));
#244657=CARTESIAN_POINT('Ctrl Pts',(-8.19815157297799,-3.05579774849325,
54.7456738989042));
#244658=CARTESIAN_POINT('Ctrl Pts',(-3.37463922465833,-8.76897411779567,
55.0105978419453));
#244659=CARTESIAN_POINT('Ctrl Pts',(5.56581319571568,-7.56129537421026,
55.3285065735951));
#244660=CARTESIAN_POINT('Ctrl Pts',(8.71285105812484,-0.797880388621073,
55.5934305166362));
#244661=CARTESIAN_POINT('Ctrl Pts',(6.99818380676628,4.39358292626538,55.8053696710693));
#244662=CARTESIAN_POINT('Ctrl Pts',(4.05101381344076,7.22222834559451,55.964324036894));
#244663=CARTESIAN_POINT('Ctrl Pts',(0.109190979620403,8.26234128571045,
56.1232784027188));
#244664=CARTESIAN_POINT('Ctrl Pts',(-5.2303339633563,7.01983915645279,56.3352175571518));
#244665=CARTESIAN_POINT('Ctrl Pts',(-8.51104360906945,2.05786890845034,
56.5471567115849));
#244666=CARTESIAN_POINT('Ctrl Pts',(-7.55314376961135,-3.33025181111693,
56.7590958660178));
#244667=CARTESIAN_POINT('Ctrl Pts',(-4.24066220519041,-7.65273631812093,
56.9710350204508));
#244668=CARTESIAN_POINT('Ctrl Pts',(3.13894653812266,-8.85607766485711,
57.2359589634921));
#244669=CARTESIAN_POINT('Ctrl Pts',(9.14536228789039,-2.12457357813009,
57.5538676951416));
#244670=CARTESIAN_POINT('Ctrl Pts',(7.13774990105824,5.0599321166944,57.8187916381829));
#244671=CARTESIAN_POINT('Ctrl Pts',(2.45910878514273,7.8886584097735,58.0307307926159));
#244672=CARTESIAN_POINT('Ctrl Pts',(-1.61926122726644,8.12091671367639,
58.1896851584407));
#244673=CARTESIAN_POINT('Ctrl Pts',(-5.29013674173023,6.34764991515613,
58.3486395242654));
#244674=CARTESIAN_POINT('Ctrl Pts',(-8.53839466246798,1.93141185111956,
58.5605786786985));
#244675=CARTESIAN_POINT('Ctrl Pts',(-7.80382662551038,-3.97152083701247,
58.7725178331314));
#244676=CARTESIAN_POINT('Ctrl Pts',(-3.57218967273978,-7.44177525002184,
58.9844569875644));
#244677=CARTESIAN_POINT('Ctrl Pts',(1.75515505625667,-8.57129044086796,
59.1963961419975));
#244678=CARTESIAN_POINT('Ctrl Pts',(8.1437579690245,-4.68639553571003,59.4613200850388));
#244679=CARTESIAN_POINT('Ctrl Pts',(8.32907739304941,4.33335136427322,59.7792288166883));
#244680=CARTESIAN_POINT('Ctrl Pts',(2.13179902823639,8.4856242892802,60.0441527597295));
#244681=CARTESIAN_POINT('Ctrl Pts',(-3.26196795879774,7.59195051083932,
60.2560919141626));
#244682=CARTESIAN_POINT('Ctrl Pts',(-6.51121789057064,5.11618380964859,
60.4150462799873));
#244683=CARTESIAN_POINT('Ctrl Pts',(-8.14669336739134,1.38188037444908,
60.5740006458121));
#244684=CARTESIAN_POINT('Ctrl Pts',(-7.7423680361898,-4.08537297475924,
60.785939800245));
#244685=CARTESIAN_POINT('Ctrl Pts',(-3.34560172894389,-8.09194888955291,
60.9978789546782));
#244686=CARTESIAN_POINT('Ctrl Pts',(2.12578254514033,-7.97631534611332,
61.209818109111));
#244687=CARTESIAN_POINT('Ctrl Pts',(6.90733485360991,-5.36994546651301,
61.4217572635443));
#244688=CARTESIAN_POINT('Ctrl Pts',(9.23416918970506,1.7358618467706,61.6866812065853));
#244689=CARTESIAN_POINT('Ctrl Pts',(3.50931616427147,8.70839619705249,62.004589938235));
#244690=CARTESIAN_POINT('Ctrl Pts',(-3.89882799483674,7.83259388340096,
62.269513881276));
#244691=CARTESIAN_POINT('Ctrl Pts',(-7.41513856994077,3.64607563166662,
62.4814530357093));
#244692=CARTESIAN_POINT('Ctrl Pts',(-8.27347536873333,-0.347707514385417,
62.6404074015339));
#244693=CARTESIAN_POINT('Ctrl Pts',(-7.08743884650086,-4.2481074361057,
62.7993617673587));
#244694=CARTESIAN_POINT('Ctrl Pts',(-3.22487434473777,-8.13847163854236,
63.0113009217918));
#244695=CARTESIAN_POINT('Ctrl Pts',(2.72072892922625,-8.32287942082066,
63.2232400762246));
#244696=CARTESIAN_POINT('Ctrl Pts',(6.80197051142163,-4.67693864526975,
63.4351792306578));
#244697=CARTESIAN_POINT('Ctrl Pts',(8.73941684035996,0.412531675932698,
63.6471183850907));
#244698=CARTESIAN_POINT('Ctrl Pts',(5.88606026343599,7.32375529017553,63.912042328132));
#244699=CARTESIAN_POINT('Ctrl Pts',(-2.99724223890796,8.89764031791383,
64.2299510597815));
#244700=CARTESIAN_POINT('Ctrl Pts',(-8.05543405846353,3.41472821837216,
64.4948750028228));
#244701=CARTESIAN_POINT('Ctrl Pts',(-8.00412909525724,-2.05233158863933,
64.7068141572559));
#244702=CARTESIAN_POINT('Ctrl Pts',(-6.05898232879026,-5.64446882638074,
64.8657685230806));
#244703=CARTESIAN_POINT('Ctrl Pts',(-2.62151725419616,-7.83618870864836,
65.0247228889054));
#244704=CARTESIAN_POINT('Ctrl Pts',(2.84269596503497,-8.2797110336745,65.2366620433383));
#244705=CARTESIAN_POINT('Ctrl Pts',(7.47930683576014,-4.55331275184693,
65.4486011977714));
#244706=CARTESIAN_POINT('Ctrl Pts',(8.20870537006574,0.870467734972957,
65.6605403522044));
#244707=CARTESIAN_POINT('Ctrl Pts',(6.37078765082055,5.99672025367893,65.8724795066374));
#244708=CARTESIAN_POINT('Ctrl Pts',(-0.291257931997344,9.39139317630174,
66.1374034496787));
#244709=CARTESIAN_POINT('Ctrl Pts',(-8.06313827302813,4.81012114802201,
66.4553121813282));
#244710=CARTESIAN_POINT('Ctrl Pts',(-8.34009391566828,-2.64446972925217,
66.7202361243695));
#244711=CARTESIAN_POINT('Ctrl Pts',(-4.74583379392158,-6.76425968799533,
66.9321752788024));
#244712=CARTESIAN_POINT('Ctrl Pts',(-0.932162842170672,-8.22814484734424,
67.0911296446274));
#244713=CARTESIAN_POINT('Ctrl Pts',(3.10446974242751,-7.6577068235964,67.2500840104519));
#244714=CARTESIAN_POINT('Ctrl Pts',(7.54388852932836,-4.44120266009448,
67.4620231648852));
#244715=CARTESIAN_POINT('Ctrl Pts',(8.6428613613827,1.40486124923329,67.6739623193179));
#244716=CARTESIAN_POINT('Ctrl Pts',(5.66982223737212,5.99947279384697,67.885901473751));
#244717=CARTESIAN_POINT('Ctrl Pts',(0.939958826895868,8.69850944202151,
68.0978406281841));
#244718=CARTESIAN_POINT('Ctrl Pts',(-6.32857928004383,6.94493921256201,
68.3627645712253));
#244719=CARTESIAN_POINT('Ctrl Pts',(-9.25338504462195,-1.58944354354721,
68.6806733028749));
#244720=CARTESIAN_POINT('Ctrl Pts',(-4.6159820866088,-7.43256989263452,
68.9455972459161));
#244721=CARTESIAN_POINT('Ctrl Pts',(0.793606342692045,-8.22486083743239,
69.1575364003492));
#244722=CARTESIAN_POINT('Ctrl Pts',(4.6427128645978,-6.85685909553858,69.3164907661738));
#244723=CARTESIAN_POINT('Ctrl Pts',(7.3382534308987,-3.798451248715,69.4754451319988));
#244724=CARTESIAN_POINT('Ctrl Pts',(8.61901727285212,1.53202566838775,69.6873842864315));
#244725=CARTESIAN_POINT('Ctrl Pts',(5.65211232994788,6.68777139916866,69.8993234408648));
#244726=CARTESIAN_POINT('Ctrl Pts',(0.405670874433816,8.24475487152382,
70.1112625952976));
#244727=CARTESIAN_POINT('Ctrl Pts',(-4.94268127029696,7.21925138814969,
70.3232017497307));
#244728=CARTESIAN_POINT('Ctrl Pts',(-9.32397158221413,1.16030971141512,
70.588125692772));
#244729=CARTESIAN_POINT('Ctrl Pts',(-5.99590603536385,-7.22501731502557,
70.9060344244214));
#244730=CARTESIAN_POINT('Ctrl Pts',(1.32691188893416,-8.64811949535424,
71.1709583674628));
#244731=CARTESIAN_POINT('Ctrl Pts',(5.95151754507708,-5.73206742692903,
71.3828975218956));
#244732=CARTESIAN_POINT('Ctrl Pts',(7.9861670350496,-2.18976184285739,71.5418518877206));
#244733=CARTESIAN_POINT('Ctrl Pts',(8.04452003161391,1.88662359923558,71.7008062535452));
#244734=CARTESIAN_POINT('Ctrl Pts',(5.55197452254941,6.76876230204749,71.9127454079784));
#244735=CARTESIAN_POINT('Ctrl Pts',(-0.056676988297962,8.75631944978158,
72.1246845624112));
#244736=CARTESIAN_POINT('Ctrl Pts',(-5.05197385037126,6.52685787508822,
72.3366237168444));
#244737=CARTESIAN_POINT('Ctrl Pts',(-8.45305692825313,2.27051267268757,
72.5485628712773));
#244738=CARTESIAN_POINT('Ctrl Pts',(-7.83028221592002,-5.18317005046361,
72.8134868143186));
#244739=CARTESIAN_POINT('Ctrl Pts',(0.130805184506471,-9.38593239092925,
73.1313955459682));
#244740=CARTESIAN_POINT('Ctrl Pts',(7.95627519325664,-4.97374396463105,
73.4493042776175));
#244741=CARTESIAN_POINT('Ctrl Pts',(8.49225628872148,3.99956479643668,73.7672130092672));
#244742=CARTESIAN_POINT('Ctrl Pts',(1.23306637670374,9.30161229503668,74.0851217409166));
#244743=CARTESIAN_POINT('Ctrl Pts',(-7.1526073352008,6.07890164024892,74.4030304725663));
#244744=CARTESIAN_POINT('Ctrl Pts',(-8.98311340169015,-2.735369255759,74.7209392042156));
#244745=CARTESIAN_POINT('Ctrl Pts',(-3.63348368341516,-7.96286352711625,
74.9858631472571));
#244746=CARTESIAN_POINT('Ctrl Pts',(1.81407828852932,-8.05179690935647,
75.19780230169));
#244747=CARTESIAN_POINT('Ctrl Pts',(6.71443182649054,-5.62074264088269,
75.409741456123));
#244748=CARTESIAN_POINT('Ctrl Pts',(8.75440499161001,-0.0309425844198426,
75.6216806105561));
#244749=CARTESIAN_POINT('Ctrl Pts',(6.57815063855531,5.00015852955729,75.833619764989));
#244750=CARTESIAN_POINT('Ctrl Pts',(3.39836701499377,7.55149140710295,75.9925741308139));
#244751=CARTESIAN_POINT('Ctrl Pts',(-0.62841393059698,8.23906875854624,
76.1515284966386));
#244752=CARTESIAN_POINT('Ctrl Pts',(-5.82198280292298,6.53109349262364,
76.3634676510716));
#244753=CARTESIAN_POINT('Ctrl Pts',(-9.3888942806352,-0.0207020382397817,
76.6283915941129));
#244754=CARTESIAN_POINT('Ctrl Pts',(-5.0440754447665,-7.92717273684912,
76.9463003257624));
#244755=CARTESIAN_POINT('Ctrl Pts',(2.41747718053897,-8.40853690166243,
77.2112242688036));
#244756=CARTESIAN_POINT('Ctrl Pts',(6.61452732186301,-4.93847952898536,
77.4231634232367));
#244757=CARTESIAN_POINT('Ctrl Pts',(8.75574595011106,0.0978413767321471,
77.6351025776695));
#244758=CARTESIAN_POINT('Ctrl Pts',(6.67068665116703,5.6689065083369,77.8470417321028));
#244759=CARTESIAN_POINT('Ctrl Pts',(1.74550905742564,8.07659541114981,78.0589808865355));
#244760=CARTESIAN_POINT('Ctrl Pts',(-2.32915219108236,7.94646773541228,
78.2179352523606));
#244761=CARTESIAN_POINT('Ctrl Pts',(-5.83535034661537,5.85037034336685,
78.3768896181851));
#244762=CARTESIAN_POINT('Ctrl Pts',(-8.6700062972319,1.17531980275567,78.5888287726184));
#244763=CARTESIAN_POINT('Ctrl Pts',(-7.11899155498003,-6.12139075719558,
78.8537527156595));
#244764=CARTESIAN_POINT('Ctrl Pts',(1.3232990659429,-9.30225649786416,79.171661447309));
#244765=CARTESIAN_POINT('Ctrl Pts',(7.3046384891676,-4.8155836252492,79.4365853903503));
#244766=CARTESIAN_POINT('Ctrl Pts',(8.23639399556954,0.549883585184681,
79.6485245447833));
#244767=CARTESIAN_POINT('Ctrl Pts',(6.5878381851895,5.76828186615729,79.8604636992164));
#244768=CARTESIAN_POINT('Ctrl Pts',(1.38096365496417,8.64450545691486,80.0724028536493));
#244769=CARTESIAN_POINT('Ctrl Pts',(-3.92628481094429,7.27065978857151,
80.2843420080824));
#244770=CARTESIAN_POINT('Ctrl Pts',(-6.93705378861793,4.52201060669062,
80.4432963739071));
#244771=CARTESIAN_POINT('Ctrl Pts',(-8.23748906457628,0.649554799191576,
80.6022507397318));
#244772=CARTESIAN_POINT('Ctrl Pts',(-7.35065479861294,-4.74534094694224,
80.8141898941649));
#244773=CARTESIAN_POINT('Ctrl Pts',(-1.42727141702365,-9.27978235578654,
81.0791138372061));
#244774=CARTESIAN_POINT('Ctrl Pts',(7.05462215267386,-6.20607792875995,
81.3970225688557));
#244775=CARTESIAN_POINT('Ctrl Pts',(8.68072874534535,1.0920336727712,81.6619465118969));
#244776=CARTESIAN_POINT('Ctrl Pts',(5.89933558949375,5.77394124777071,81.87388566633));
#244777=CARTESIAN_POINT('Ctrl Pts',(1.2534011759003,8.66612215767996,82.085824820763));
#244778=CARTESIAN_POINT('Ctrl Pts',(-4.57253617197667,7.46501494350422,
82.2977639751959));
#244779=CARTESIAN_POINT('Ctrl Pts',(-7.71086060751405,2.96998903753608,
82.509703129629));
#244780=CARTESIAN_POINT('Ctrl Pts',(-8.21057260419263,-1.07600776198775,
82.6686574954537));
#244781=CARTESIAN_POINT('Ctrl Pts',(-6.68017462332549,-4.86347761639228,
82.8276118612785));
#244782=CARTESIAN_POINT('Ctrl Pts',(-2.49811809120793,-8.38509348057498,
83.0395510157114));
#244783=CARTESIAN_POINT('Ctrl Pts',(4.95048473210504,-7.97772932499307,
83.3044749587528));
#244784=CARTESIAN_POINT('Ctrl Pts',(9.39505194771926,-0.126869518922279,
83.6223836904022));
#244785=CARTESIAN_POINT('Ctrl Pts',(5.88431699012904,6.47475116532634,83.8873076334436));
#244786=CARTESIAN_POINT('Ctrl Pts',(0.726686965102308,8.22268107034541,
84.0992467878765));
#244787=CARTESIAN_POINT('Ctrl Pts',(-4.68349895600442,7.39848128259805,
84.3111859423098));
#244788=CARTESIAN_POINT('Ctrl Pts',(-8.32818868613579,2.69737063801516,
84.5231250967425));
#244789=CARTESIAN_POINT('Ctrl Pts',(-7.78911378360293,-2.75824448837895,
84.7350642511757));
#244790=CARTESIAN_POINT('Ctrl Pts',(-5.53757591012922,-6.15682939768139,
84.8940186170005));
#244791=CARTESIAN_POINT('Ctrl Pts',(-1.91194980781425,-8.03881803847154,
85.0529729828251));
#244792=CARTESIAN_POINT('Ctrl Pts',(3.55517065472387,-7.99444483947463,
85.2649121372583));
#244793=CARTESIAN_POINT('Ctrl Pts',(8.94872781730662,-2.84107985058827,
85.5298360802993));
#244794=CARTESIAN_POINT('Ctrl Pts',(7.21963126456139,6.01332032898139,85.8477448119492));
#244795=CARTESIAN_POINT('Ctrl Pts',(0.259533891981588,8.74529766515297,
86.1126687549902));
#244796=CARTESIAN_POINT('Ctrl Pts',(-4.79525293485256,6.71908529642643,
86.3246079094232));
#244797=CARTESIAN_POINT('Ctrl Pts',(-8.36921611223426,2.57466685739491,
86.5365470638563));
#244798=CARTESIAN_POINT('Ctrl Pts',(-8.08079203456533,-3.36679896115177,
86.7484862182892));
#244799=CARTESIAN_POINT('Ctrl Pts',(-4.12343096012912,-7.16069293494938,
86.9604253727224));
#244800=CARTESIAN_POINT('Ctrl Pts',(-0.20287335629181,-8.27829315704055,
87.119379738547));
#244801=CARTESIAN_POINT('Ctrl Pts',(3.77527785111434,-7.35019895445982,
87.2783341043719));
#244802=CARTESIAN_POINT('Ctrl Pts',(7.89962168578836,-3.76116523128593,
87.4902732588048));
#244803=CARTESIAN_POINT('Ctrl Pts',(8.64565175936641,3.6611705671027,87.7551972018461));
#244804=CARTESIAN_POINT('Ctrl Pts',(1.57400355324675,9.26313174847145,88.0731059334957));
#244805=CARTESIAN_POINT('Ctrl Pts',(-5.48999745202445,6.81230629596051,
88.3380298765369));
#244806=CARTESIAN_POINT('Ctrl Pts',(-8.01229389654767,1.98587624116183,
88.54996903097));
#244807=CARTESIAN_POINT('Ctrl Pts',(-8.0321637517713,-3.48669373828258,
88.7619081854028));
#244808=CARTESIAN_POINT('Ctrl Pts',(-3.94926054510204,-7.8126740811074,
88.9738473398362));
#244809=CARTESIAN_POINT('Ctrl Pts',(1.52423107718599,-8.12126380650983,
89.1857864942687));
#244810=CARTESIAN_POINT('Ctrl Pts',(5.22934284069866,-6.42069066744618,
89.3447408600939));
#244811=CARTESIAN_POINT('Ctrl Pts',(7.64787048893159,-3.12861383168092,
89.5036952259183));
#244812=CARTESIAN_POINT('Ctrl Pts',(8.44701969721102,2.27996598890042,89.7156343803516));
#244813=CARTESIAN_POINT('Ctrl Pts',(4.18693389661271,8.40363307213325,89.9805583233925));
#244814=CARTESIAN_POINT('Ctrl Pts',(-4.82818886236687,8.06050180103496,
90.2984670550424));
#244815=CARTESIAN_POINT('Ctrl Pts',(-8.60069212356836,1.60489379362226,
90.5633909980834));
#244816=CARTESIAN_POINT('Ctrl Pts',(-7.37812451624919,-3.70186933218736,
90.7753301525166));
#244817=CARTESIAN_POINT('Ctrl Pts',(-3.83435035223363,-7.87213091457285,
90.9872693069495));
#244818=CARTESIAN_POINT('Ctrl Pts',(2.08053294659223,-8.50328864668548,
91.1992084613827));
#244819=CARTESIAN_POINT('Ctrl Pts',(6.43925217997725,-5.17824657140275,
91.4111476158157));
#244820=CARTESIAN_POINT('Ctrl Pts',(8.14800929900498,-1.47690204682834,
91.5701019816404));
#244821=CARTESIAN_POINT('Ctrl Pts',(7.84441750217561,2.5967790770139,91.7290563474652));
#244822=CARTESIAN_POINT('Ctrl Pts',(4.93425091533369,7.22520273626573,91.940995501898));
#244823=CARTESIAN_POINT('Ctrl Pts',(-2.2842866691219,9.10678311364272,92.2059194449396));
#244824=CARTESIAN_POINT('Ctrl Pts',(-8.90965126982931,2.98348977293375,
92.5238281765888));
#244825=CARTESIAN_POINT('Ctrl Pts',(-7.57735540756411,-4.37393119752425,
92.7887521196303));
#244826=CARTESIAN_POINT('Ctrl Pts',(-3.19756632291204,-7.61026461697919,
93.0006912740631));
#244827=CARTESIAN_POINT('Ctrl Pts',(2.20649201279304,-8.47372885790721,
93.2126304284962));
#244828=CARTESIAN_POINT('Ctrl Pts',(7.11029197821448,-5.10669003712246,
93.4245695829292));
#244829=CARTESIAN_POINT('Ctrl Pts',(8.25916532611732,0.253760334661598,
93.6365087373623));
#244830=CARTESIAN_POINT('Ctrl Pts',(7.15023209159534,4.17677821160243,93.7954631031868));
#244831=CARTESIAN_POINT('Ctrl Pts',(4.27044608444791,7.07399729736161,93.954417469012));
#244832=CARTESIAN_POINT('Ctrl Pts',(-0.950227941146778,8.69755445717221,
94.1663566234446));
#244833=CARTESIAN_POINT('Ctrl Pts',(-7.65753597247037,5.43264273590476,
94.4312805664861));
#244834=CARTESIAN_POINT('Ctrl Pts',(-8.7085771706482,-3.5275743277836,94.7491892981357));
#244835=CARTESIAN_POINT('Ctrl Pts',(-2.91186703220212,-8.25037086923931,
95.0141132411768));
#244836=CARTESIAN_POINT('Ctrl Pts',(2.51994254285583,-7.8606900149142,95.22605239561));
#244837=CARTESIAN_POINT('Ctrl Pts',(7.1867561003735,-5.00232191223157,95.4379915500428));
#244838=CARTESIAN_POINT('Ctrl Pts',(8.72239929178196,0.744503690674433,
95.6499307044759));
#244839=CARTESIAN_POINT('Ctrl Pts',(6.10920625702525,5.56379412817455,95.8618698589088));
#244840=CARTESIAN_POINT('Ctrl Pts',(2.71560544576572,7.82283722542689,96.0208242247336));
#244841=CARTESIAN_POINT('Ctrl Pts',(-1.35616922499205,8.15100929679513,
96.1797785905584));
#244842=CARTESIAN_POINT('Ctrl Pts',(-6.37796772621453,5.98931668548074,
96.3917177449913));
#244843=CARTESIAN_POINT('Ctrl Pts',(-9.35009381440451,-0.85276604499158,
96.6566416880326));
#244844=CARTESIAN_POINT('Ctrl Pts',(-4.32161537230249,-8.34306523701283,
96.9745504196823));
#244845=CARTESIAN_POINT('Ctrl Pts',(3.15324704008515,-8.16116549258814,
97.2394743627233));
#244846=CARTESIAN_POINT('Ctrl Pts',(7.02620917168331,-4.33277539293464,
97.4514135171566));
#244847=CARTESIAN_POINT('Ctrl Pts',(8.71261502302726,0.873514293167906,
97.6633526715894));
#244848=CARTESIAN_POINT('Ctrl Pts',(6.14197512894139,6.23784230853676,97.8752918260226));
#244849=CARTESIAN_POINT('Ctrl Pts',(1.0227799761445,8.19951994399571,98.0872309804555));
#244850=CARTESIAN_POINT('Ctrl Pts',(-3.02431128459427,7.70875064108789,
98.2461853462802));
#244851=CARTESIAN_POINT('Ctrl Pts',(-6.33092465357644,5.31013564365306,
98.405139712105));
#244852=CARTESIAN_POINT('Ctrl Pts',(-8.7400567020074,0.402238140045645,
98.6170788665382));
#244853=CARTESIAN_POINT('Ctrl Pts',(-6.54841087316406,-6.72828204684399,
98.8820028095792));
#244854=CARTESIAN_POINT('Ctrl Pts',(2.142585482776,-9.14835637828844,99.1999115412288));
#244855=CARTESIAN_POINT('Ctrl Pts',(7.70271306345742,-4.14919275947252,
99.4648354842702));
#244856=CARTESIAN_POINT('Ctrl Pts',(8.15523954627708,1.27774249076433,99.6767746387031));
#244857=CARTESIAN_POINT('Ctrl Pts',(6.05064540172951,6.32948481176616,99.8887137931363));
#244858=CARTESIAN_POINT('Ctrl Pts',(0.609332981805773,8.73288317040774,
100.100652947569));
#244859=CARTESIAN_POINT('Ctrl Pts',(-4.55525842887585,6.89404285145814,
100.312592102002));
#244860=CARTESIAN_POINT('Ctrl Pts',(-7.3105545667479,3.88935561747675,100.471546467826));
#244861=CARTESIAN_POINT('Ctrl Pts',(-8.26264112040473,-0.0831218301869292,
100.630500833652));
#244862=CARTESIAN_POINT('Ctrl Pts',(-6.90112694396627,-5.37818125195461,
100.842439988084));
#244863=CARTESIAN_POINT('Ctrl Pts',(-0.599151469554942,-9.36976423300961,
101.107363931126));
#244864=CARTESIAN_POINT('Ctrl Pts',(7.57692554188092,-5.55637438515131,
101.425272662775));
#244865=CARTESIAN_POINT('Ctrl Pts',(8.54977268556443,1.85714192198488,101.690196605817));
#244866=CARTESIAN_POINT('Ctrl Pts',(5.36435094540862,6.2740972947795,101.902135760249));
#244867=CARTESIAN_POINT('Ctrl Pts',(0.480356583988195,8.74310844677501,
102.114074914683));
#244868=CARTESIAN_POINT('Ctrl Pts',(-5.21619276540107,7.03035334708608,
102.326014069115));
#244869=CARTESIAN_POINT('Ctrl Pts',(-7.9437542886209,2.27485691717137,102.537953223549));
#244870=CARTESIAN_POINT('Ctrl Pts',(-8.08288738621888,-1.79950734766523,
102.696907589373));
#244871=CARTESIAN_POINT('Ctrl Pts',(-6.22281468754034,-5.43642574563372,
102.855861955198));
#244872=CARTESIAN_POINT('Ctrl Pts',(-1.7450832855641,-8.57350984148596,
103.067801109631));
#244873=CARTESIAN_POINT('Ctrl Pts',(5.63809766156071,-7.50755080065118,
103.332725052672));
#244874=CARTESIAN_POINT('Ctrl Pts',(9.36932056200261,0.706349192403,103.650633784322));
#244875=CARTESIAN_POINT('Ctrl Pts',(5.28727599165471,6.97081786315566,103.915557727363));
#244876=CARTESIAN_POINT('Ctrl Pts',(-0.00498074626342562,8.25472792537904,
104.127496881796));
#244877=CARTESIAN_POINT('Ctrl Pts',(-5.32082169786743,6.95424648825107,
104.339436036229));
#244878=CARTESIAN_POINT('Ctrl Pts',(-8.53448952384093,1.94859531923814,
104.551375190662));
#244879=CARTESIAN_POINT('Ctrl Pts',(-7.51398423530762,-3.43776775002822,
104.763314345095));
#244880=CARTESIAN_POINT('Ctrl Pts',(-4.97007821053796,-6.62341435920571,
104.92226871092));
#244881=CARTESIAN_POINT('Ctrl Pts',(-1.19191371467555,-8.17664290647606,
105.081223076745));
#244882=CARTESIAN_POINT('Ctrl Pts',(4.24975671303451,-7.64787255095371,
105.293162231178));
#244883=CARTESIAN_POINT('Ctrl Pts',(9.16532388241747,-2.03673817562357,
105.558086174219));
#244884=CARTESIAN_POINT('Ctrl Pts',(6.65823321967812,6.6295571019147,105.875994905869));
#244885=CARTESIAN_POINT('Ctrl Pts',(-0.51661674225922,8.73388208271878,
106.14091884891));
#244886=CARTESIAN_POINT('Ctrl Pts',(-5.37191837928407,6.26761923350293,
106.352858003343));
#244887=CARTESIAN_POINT('Ctrl Pts',(-8.56447977198818,1.82273804894021,
106.564797157776));
#244888=CARTESIAN_POINT('Ctrl Pts',(-7.75057601113544,-4.06977968031675,
106.776736312209));
#244889=CARTESIAN_POINT('Ctrl Pts',(-3.47252267763465,-7.49798589255131,
106.988675466642));
#244890=CARTESIAN_POINT('Ctrl Pts',(0.531661882066579,-8.26369353471885,
107.147629832466));
#244891=CARTESIAN_POINT('Ctrl Pts',(4.41189565171434,-6.98665329622418,
107.306584198291));
#244892=CARTESIAN_POINT('Ctrl Pts',(8.20189742781796,-3.04618864471102,
107.518523352724));
#244893=CARTESIAN_POINT('Ctrl Pts',(8.28712132352169,4.41305839921567,107.783447295766));
#244894=CARTESIAN_POINT('Ctrl Pts',(0.74678191590698,9.36618458846757,108.101356027415));
#244895=CARTESIAN_POINT('Ctrl Pts',(-6.07219110863386,6.29889547725997,
108.366279970456));
#244896=CARTESIAN_POINT('Ctrl Pts',(-8.15677553875159,1.26790013025069,
108.578219124889));
#244897=CARTESIAN_POINT('Ctrl Pts',(-7.69151238309534,-4.18489247419079,
108.790158279322));
#244898=CARTESIAN_POINT('Ctrl Pts',(-3.24125016634453,-8.13196363185907,
109.002097433755));
#244899=CARTESIAN_POINT('Ctrl Pts',(2.23805079999365,-7.95420233639011,
109.214036588188));
#244900=CARTESIAN_POINT('Ctrl Pts',(5.77785197050303,-5.931923954296,109.372990954013));
#244901=CARTESIAN_POINT('Ctrl Pts',(7.89507160387075,-2.43844046328999,
109.531945319838));
#244902=CARTESIAN_POINT('Ctrl Pts',(8.21169246659059,3.01968433942239,109.743884474271));
#244903=CARTESIAN_POINT('Ctrl Pts',(3.4256091458593,8.74166267053705,110.008808417312));
#244904=CARTESIAN_POINT('Ctrl Pts',(-5.52361955555509,7.60083705789452,
110.326717148962));
#244905=CARTESIAN_POINT('Ctrl Pts',(-8.7090900621896,0.836265138511122,
110.591641092003));
#244906=CARTESIAN_POINT('Ctrl Pts',(-7.02097542855796,-4.34125119769074,
110.803580246436));
#244907=CARTESIAN_POINT('Ctrl Pts',(-3.12152234153726,-8.18100152983312,
111.015519400869));
#244908=CARTESIAN_POINT('Ctrl Pts',(2.82602354241485,-8.28541647042698,
111.227458555302));
#244909=CARTESIAN_POINT('Ctrl Pts',(6.87287687018398,-4.58713088094033,
111.439397709735));
#244910=CARTESIAN_POINT('Ctrl Pts',(8.24684447350177,-0.748900141855164,
111.59835207556));
#244911=CARTESIAN_POINT('Ctrl Pts',(7.58338159077484,3.2818396018016,111.757306441385));
#244912=CARTESIAN_POINT('Ctrl Pts',(4.27443372015049,7.63410787503385,111.969245595818));
#244913=CARTESIAN_POINT('Ctrl Pts',(-3.08246536969312,8.86847627895,112.234169538859));
#244914=CARTESIAN_POINT('Ctrl Pts',(-9.13902346548749,2.1820511159092,112.552078270508));
#244915=CARTESIAN_POINT('Ctrl Pts',(-7.15985478877821,-5.02832660999927,
112.81700221355));
#244916=CARTESIAN_POINT('Ctrl Pts',(-2.51045472892191,-7.86372526121687,
113.028941367983));
#244917=CARTESIAN_POINT('Ctrl Pts',(2.94886687155791,-8.24480878696875,
113.240880522416));
#244918=CARTESIAN_POINT('Ctrl Pts',(7.53493331273293,-4.45637914941877,
113.452819676849));
#244919=CARTESIAN_POINT('Ctrl Pts',(8.20416779507647,0.984803016758322,
113.664758831282));
#244920=CARTESIAN_POINT('Ctrl Pts',(6.75188693482159,4.79409199035459,113.823713197106));
#244921=CARTESIAN_POINT('Ctrl Pts',(3.62664335718611,7.42466197769528,113.982667562931));
#244922=CARTESIAN_POINT('Ctrl Pts',(-1.71738562550865,8.5791009604101,114.194606717364));
#244923=CARTESIAN_POINT('Ctrl Pts',(-8.10891394093082,4.73254466056412,
114.459530660406));
#244924=CARTESIAN_POINT('Ctrl Pts',(-8.36164022351918,-4.28556527748645,
114.777439392055));
#244925=CARTESIAN_POINT('Ctrl Pts',(-2.16914480590855,-8.47598961208767,
115.042363335096));
#244926=CARTESIAN_POINT('Ctrl Pts',(3.20674776995516,-7.60640037532565,
115.254302489529));
#244927=CARTESIAN_POINT('Ctrl Pts',(7.60184594723935,-4.34564448088987,
115.466241643962));
#244928=CARTESIAN_POINT('Ctrl Pts',(8.62208213981668,1.51467314129497,115.678180798395));
#244929=CARTESIAN_POINT('Ctrl Pts',(5.59202176323629,6.0833788958997,115.890119952828));
#244930=CARTESIAN_POINT('Ctrl Pts',(2.01154959266723,8.03274320695225,116.049074318653));
#244931=CARTESIAN_POINT('Ctrl Pts',(-2.07328684917035,7.9987267214422,116.208028684478));
#244932=CARTESIAN_POINT('Ctrl Pts',(-6.88372186139305,5.40044072373649,
116.419967838911));
#244933=CARTESIAN_POINT('Ctrl Pts',(-9.23771052450177,-1.67814437137133,
116.684891781952));
#244934=CARTESIAN_POINT('Ctrl Pts',(-3.56512891153324,-8.69327054791941,
117.002800513602));
#244935=CARTESIAN_POINT('Ctrl Pts',(3.86419204732527,-7.84956106509181,
117.267724456643));
#244936=CARTESIAN_POINT('Ctrl Pts',(7.38258641782075,-3.69296299917493,
117.479663611076));
#244937=CARTESIAN_POINT('Ctrl Pts',(8.60090167609176,1.64230877670762,117.691602765509));
#244938=CARTESIAN_POINT('Ctrl Pts',(5.56491819765861,6.75767864018963,117.903541919942));
#244939=CARTESIAN_POINT('Ctrl Pts',(0.291999784095893,8.25790181085207,
118.115481074375));
#244940=CARTESIAN_POINT('Ctrl Pts',(-3.69566448850107,7.41035486201767,
118.2744354402));
#244941=CARTESIAN_POINT('Ctrl Pts',(-6.77666552377574,4.72810235740781,
118.433389806024));
#244942=CARTESIAN_POINT('Ctrl Pts',(-8.74131016986724,-0.374009611892281,
118.645328960458));
#244943=CARTESIAN_POINT('Ctrl Pts',(-5.92628477378799,-7.28221209836851,
118.910252903499));
#244944=CARTESIAN_POINT('Ctrl Pts',(2.94500667733487,-8.92244544088817,
119.228161635148));
#244945=CARTESIAN_POINT('Ctrl Pts',(8.04015614710591,-3.45014176859058,
119.49308557819));
#244946=CARTESIAN_POINT('Ctrl Pts',(8.00989158325591,1.99554372398919,119.705024732623));
#244947=CARTESIAN_POINT('Ctrl Pts',(5.46582529332645,6.84086556092725,119.916963887056));
#244948=CARTESIAN_POINT('Ctrl Pts',(-0.167094020397713,8.75252047921361,
120.128903041489));
#244949=CARTESIAN_POINT('Ctrl Pts',(-5.14837558233741,6.46315983515627,
120.340842195922));
#244950=CARTESIAN_POINT('Ctrl Pts',(-7.62651071766266,3.22608578093847,
120.499796561746));
#244951=CARTESIAN_POINT('Ctrl Pts',(-8.22275425290849,-0.815144171010343,
120.658750927571));
#244952=CARTESIAN_POINT('Ctrl Pts',(-6.39727724933591,-5.96868749983967,
120.870690082004));
#244953=CARTESIAN_POINT('Ctrl Pts',(0.233684665549838,-9.38599252837668,
121.135614025046));
#244954=CARTESIAN_POINT('Ctrl Pts',(8.03958757993772,-4.86293414716715,
121.453522756695));
#244955=CARTESIAN_POINT('Ctrl Pts',(8.35151756196486,2.60763178102463,121.718446699736));
#244956=CARTESIAN_POINT('Ctrl Pts',(4.78714110894806,6.72486713124396,121.930385854169));
#244957=CARTESIAN_POINT('Ctrl Pts',(-0.296469108270646,8.75127384028694,
122.142325008602));
#244958=CARTESIAN_POINT('Ctrl Pts',(-5.81879038537252,6.54035271233923,
122.354264163035));
#244959=CARTESIAN_POINT('Ctrl Pts',(-8.11411914629701,1.56181838613904,
122.566203317468));
#244960=CARTESIAN_POINT('Ctrl Pts',(-7.89157816631291,-2.5088422105765,
122.725157683293));
#244961=CARTESIAN_POINT('Ctrl Pts',(-5.71647220940666,-5.96658134967907,
122.884112049118));
#244962=CARTESIAN_POINT('Ctrl Pts',(-0.978312153156251,-8.69444029288825,
123.096051203551));
#244963=CARTESIAN_POINT('Ctrl Pts',(6.28133061646463,-6.97827700455636,
123.360975146592));
#244964=CARTESIAN_POINT('Ctrl Pts',(9.26983908661552,1.53400791504753,123.678883878242));
#244965=CARTESIAN_POINT('Ctrl Pts',(4.64861649203921,7.41201415292483,123.943807821283));
#244966=CARTESIAN_POINT('Ctrl Pts',(-0.736609251960068,8.22179814516222,
124.155746975716));
#244967=CARTESIAN_POINT('Ctrl Pts',(-5.91626188541497,6.45527172650657,
124.367686130149));
#244968=CARTESIAN_POINT('Ctrl Pts',(-8.67361159831449,1.18448173995706,
124.579625284582));
#244969=CARTESIAN_POINT('Ctrl Pts',(-7.17970877483334,-4.09023081257849,
124.791564439015));
#244970=CARTESIAN_POINT('Ctrl Pts',(-4.3634588146324,-7.03786348017661,
124.95051880484));
#244971=CARTESIAN_POINT('Ctrl Pts',(-0.462495538518424,-8.25010578114652,
125.109473170664));
#244972=CARTESIAN_POINT('Ctrl Pts',(4.91089104594106,-7.24110045576698,
125.321412325098));
#244973=CARTESIAN_POINT('Ctrl Pts',(9.30977560646184,-1.21636442852571,
125.586336268139));
#244974=CARTESIAN_POINT('Ctrl Pts',(6.04442525950268,7.19360968203438,125.904244999789));
#244975=CARTESIAN_POINT('Ctrl Pts',(-1.28870085632782,8.65371822953107,
126.169168942829));
#244976=CARTESIAN_POINT('Ctrl Pts',(-5.90629906469245,5.76681795171991,
126.381108097263));
#244977=CARTESIAN_POINT('Ctrl Pts',(-8.69232860192757,1.05646165853806,
126.593047251695));
#244978=CARTESIAN_POINT('Ctrl Pts',(-7.35935175642168,-4.74072535335686,
126.804986406129));
#244979=CARTESIAN_POINT('Ctrl Pts',(-2.79428062454671,-7.77625886804627,
127.016925560562));
#244980=CARTESIAN_POINT('Ctrl Pts',(1.26201217326531,-8.18404670484764,
127.175879926386));
#244981=CARTESIAN_POINT('Ctrl Pts',(5.01378545920402,-6.56811258219065,
127.334834292211));
#244982=CARTESIAN_POINT('Ctrl Pts',(8.4396123869428,-2.30723415235086,127.546773446644));
#244983=CARTESIAN_POINT('Ctrl Pts',(7.86335926958056,5.13020908571511,127.811697389686));
#244984=CARTESIAN_POINT('Ctrl Pts',(-0.0863179740656035,9.3955120234359,
128.129606121335));
#244985=CARTESIAN_POINT('Ctrl Pts',(-6.60658784808237,5.73590325047324,
128.394530064376));
#244986=CARTESIAN_POINT('Ctrl Pts',(-8.23705157250959,0.539943813445461,
128.606469218809));
#244987=CARTESIAN_POINT('Ctrl Pts',(-7.29031769922452,-4.85015005997164,
128.818408373242));
#244988=CARTESIAN_POINT('Ctrl Pts',(-2.5077264657993,-8.38724287971926,
129.030347527675));
#244989=CARTESIAN_POINT('Ctrl Pts',(2.93425382945483,-7.72452980160819,
129.242286682108));
#244990=CARTESIAN_POINT('Ctrl Pts',(6.28088105743071,-5.39646442914402,
129.401241047933));
#244991=CARTESIAN_POINT('Ctrl Pts',(8.08012709843497,-1.72907304538782,
129.560195413758));
#244992=CARTESIAN_POINT('Ctrl Pts',(7.91172735197586,3.73563341135219,129.772134568191));
#244993=CARTESIAN_POINT('Ctrl Pts',(2.63731990175192,9.0108827536864,130.037058511232));
#244994=CARTESIAN_POINT('Ctrl Pts',(-6.17557138222025,7.0813427454344,130.354967242881));
#244995=CARTESIAN_POINT('Ctrl Pts',(-8.74893487918551,0.0610538684213404,
130.619891185923));
#244996=CARTESIAN_POINT('Ctrl Pts',(-6.60856112015652,-4.94646114387313,
130.831830340356));
#244997=CARTESIAN_POINT('Ctrl Pts',(-2.38412344038647,-8.42547584343258,
131.043769494789));
#244998=CARTESIAN_POINT('Ctrl Pts',(3.54926925064944,-8.00232609504537,
131.255708649222));
#244999=CARTESIAN_POINT('Ctrl Pts',(7.25240208852943,-3.95990784377751,
131.467647803655));
#245000=CARTESIAN_POINT('Ctrl Pts',(8.28076506882167,-0.0150033089913116,
131.62660216948));
#245001=CARTESIAN_POINT('Ctrl Pts',(7.26265350624478,3.94106730409408,131.785556535304));
#245002=CARTESIAN_POINT('Ctrl Pts',(3.58097056341955,7.98292156195555,131.997495689737));
#245003=CARTESIAN_POINT('Ctrl Pts',(-3.85638062987201,8.56036170837607,
132.262419632779));
#245004=CARTESIAN_POINT('Ctrl Pts',(-9.29645831505568,1.36343658901342,
132.580328364428));
#245005=CARTESIAN_POINT('Ctrl Pts',(-6.6859958139991,-5.64314186911429,
132.845252307469));
#245006=CARTESIAN_POINT('Ctrl Pts',(-1.80358216812555,-8.05528697015432,
133.057191461902));
#245007=CARTESIAN_POINT('Ctrl Pts',(3.66802973050227,-7.95099030277828,
133.269130616335));
#245008=CARTESIAN_POINT('Ctrl Pts',(7.90026415480175,-3.77098982631053,
133.481069770768));
#245009=CARTESIAN_POINT('Ctrl Pts',(8.08459121557868,1.70809351433024,133.693008925202));
#245010=CARTESIAN_POINT('Ctrl Pts',(6.3003954935726,5.37367009175038,133.851963291026));
#245011=CARTESIAN_POINT('Ctrl Pts',(2.95429220966773,7.71688246736308,134.010917656851));
#245012=CARTESIAN_POINT('Ctrl Pts',(-2.47102176873227,8.39312051202395,
134.222856811284));
#245013=CARTESIAN_POINT('Ctrl Pts',(-8.49646973291041,3.99518848123922,
134.487780754325));
#245014=CARTESIAN_POINT('Ctrl Pts',(-7.94887339718645,-5.00981191143028,
134.805689485975));
#245015=CARTESIAN_POINT('Ctrl Pts',(-1.4093678818468,-8.63490805875611,
135.070613429016));
#245016=CARTESIAN_POINT('Ctrl Pts',(3.86833736244917,-7.29221342526346,
135.282552583449));
#245017=CARTESIAN_POINT('Ctrl Pts',(7.95703106514325,-3.65482222106151,
135.494491737882));
#245018=CARTESIAN_POINT('Ctrl Pts',(8.45403342063807,2.2730453255652,135.706430892315));
#245019=CARTESIAN_POINT('Ctrl Pts',(5.03065108698298,6.55492372538339,135.918370046748));
#245020=CARTESIAN_POINT('Ctrl Pts',(1.292011381003,8.17974234020297,136.077324412573));
#245021=CARTESIAN_POINT('Ctrl Pts',(-2.77472573740587,7.78289447205871,
136.236278778398));
#245022=CARTESIAN_POINT('Ctrl Pts',(-7.33390610192825,4.7703262757849,136.448217932831));
#245023=CARTESIAN_POINT('Ctrl Pts',(-9.05547875439378,-2.49294253543202,
136.713141875872));
#245024=CARTESIAN_POINT('Ctrl Pts',(-2.77557159916479,-8.97045204363947,
137.031050607521));
#245025=CARTESIAN_POINT('Ctrl Pts',(4.53630470631618,-7.48389232836955,
137.295974550563));
#245026=CARTESIAN_POINT('Ctrl Pts',(7.69217499320704,-3.01368022077503,
137.507913704996));
#245027=CARTESIAN_POINT('Ctrl Pts',(8.21568403484059,1.02348437607822,137.666868070821));
#245028=CARTESIAN_POINT('Ctrl Pts',(6.71054899145757,4.84288607544307,137.825887206215));
#245029=CARTESIAN_POINT('Ctrl Pts',(4.62085797159542,6.58783761712044,137.931921553001));
#245030=CARTESIAN_POINT('Ctrl Pts',(3.42771117511922,7.15909185610951,137.984971111179));
#245031=CARTESIAN_POINT('Ctrl Pts',(4.3786726516329,-6.14439445976196,7.5507492878767));
#245032=CARTESIAN_POINT('Ctrl Pts',(5.4020829415103,-5.4150902343734,7.60376665636641));
#245033=CARTESIAN_POINT('Ctrl Pts',(7.07379358162461,-3.44081123600024,
7.70976881346437));
#245034=CARTESIAN_POINT('Ctrl Pts',(7.86067347517091,0.380537801570955,
7.8687557591706));
#245035=CARTESIAN_POINT('Ctrl Pts',(6.71242675331904,4.07595804571959,8.02771012499535));
#245036=CARTESIAN_POINT('Ctrl Pts',(3.02843446954156,7.74789103749108,8.23964927942837));
#245037=CARTESIAN_POINT('Ctrl Pts',(-4.06131014199803,7.94832137794174,
8.50457322246963));
#245038=CARTESIAN_POINT('Ctrl Pts',(-8.88662488748039,0.858715297192927,
8.82248195411916));
#245039=CARTESIAN_POINT('Ctrl Pts',(-6.09061026031311,-5.66263867668864,
9.08740589716043));
#245040=CARTESIAN_POINT('Ctrl Pts',(-1.3300103532646,-7.74079488884142,
9.29934505159343));
#245041=CARTESIAN_POINT('Ctrl Pts',(2.54310647155665,-7.44962859780676,
9.45829941741821));
#245042=CARTESIAN_POINT('Ctrl Pts',(5.77946815770139,-5.31867664433347,
9.61725378324296));
#245043=CARTESIAN_POINT('Ctrl Pts',(8.28754101548936,-0.750810161955585,
9.82919293767598));
#245044=CARTESIAN_POINT('Ctrl Pts',(6.85596530424556,4.71954476407852,10.041132092109));
#245045=CARTESIAN_POINT('Ctrl Pts',(2.43413358249498,7.45951945984923,10.253071246542));
#245046=CARTESIAN_POINT('Ctrl Pts',(-2.72719324131664,7.85675727497228,
10.465010400975));
#245047=CARTESIAN_POINT('Ctrl Pts',(-8.26051227361675,3.39608283759135,
10.7299343440162));
#245048=CARTESIAN_POINT('Ctrl Pts',(-7.30566755686335,-5.12621182347484,
11.0478430756658));
#245049=CARTESIAN_POINT('Ctrl Pts',(-0.946139846574816,-8.26276376220919,
11.312767018707));
#245050=CARTESIAN_POINT('Ctrl Pts',(4.0243689706447,-6.74524415246625,11.5247061731401));
#245051=CARTESIAN_POINT('Ctrl Pts',(6.77604042885482,-4.00550406444893,
11.6836605389648));
#245052=CARTESIAN_POINT('Ctrl Pts',(7.84948657201265,-0.281954118113144,
11.8426149047896));
#245053=CARTESIAN_POINT('Ctrl Pts',(6.78387063251435,4.81908192792366,12.0545540592226));
#245054=CARTESIAN_POINT('Ctrl Pts',(2.13917921968976,8.04380728042435,12.2664932136556));
#245055=CARTESIAN_POINT('Ctrl Pts',(-3.00190064357618,7.24970078792561,
12.4784323680886));
#245056=CARTESIAN_POINT('Ctrl Pts',(-7.18106853250261,4.19501405678216,
12.6903715225216));
#245057=CARTESIAN_POINT('Ctrl Pts',(-8.48377503682947,-2.79200061042099,
12.9552954655629));
#245058=CARTESIAN_POINT('Ctrl Pts',(-2.2162499015533,-8.64517229147749,
13.2732041972124));
#245059=CARTESIAN_POINT('Ctrl Pts',(4.6546035164407,-6.89224791200518,13.5381281402537));
#245060=CARTESIAN_POINT('Ctrl Pts',(7.44369077636594,-2.50706182528472,
13.7500672946867));
#245061=CARTESIAN_POINT('Ctrl Pts',(7.75236522237301,1.3636728095776,13.9090216605115));
#245062=CARTESIAN_POINT('Ctrl Pts',(6.1463672728273,4.8904103908539,14.0679760263362));
#245063=CARTESIAN_POINT('Ctrl Pts',(2.0195949849537,8.07252655100552,14.2799151807692));
#245064=CARTESIAN_POINT('Ctrl Pts',(-3.60590313906814,7.50175878230377,
14.4918543352022));
#245065=CARTESIAN_POINT('Ctrl Pts',(-6.99500513087751,3.555203681579,14.7037934896353));
#245066=CARTESIAN_POINT('Ctrl Pts',(-8.18329367705831,-1.48310209359639,
14.9157326440683));
#245067=CARTESIAN_POINT('Ctrl Pts',(-4.6291914378742,-7.63808178227025,
15.1806565871096));
#245068=CARTESIAN_POINT('Ctrl Pts',(3.93842904184229,-8.00871677424294,
15.4985653187591));
#245069=CARTESIAN_POINT('Ctrl Pts',(8.01805636285859,-2.20888822471383,
15.7634892618003));
#245070=CARTESIAN_POINT('Ctrl Pts',(7.28510689705072,2.93617249785386,15.9754284162333));
#245071=CARTESIAN_POINT('Ctrl Pts',(5.00241856512635,6.07738254047629,16.1343827820581));
#245072=CARTESIAN_POINT('Ctrl Pts',(1.48891842297151,7.71213760116044,16.2933371478829));
#245073=CARTESIAN_POINT('Ctrl Pts',(-3.71542417565377,7.44580902387277,
16.5052763023159));
#245074=CARTESIAN_POINT('Ctrl Pts',(-7.61776274296967,3.35389520727049,
16.7172154567489));
#245075=CARTESIAN_POINT('Ctrl Pts',(-7.62587191461766,-1.84814705670977,
16.9291546111819));
#245076=CARTESIAN_POINT('Ctrl Pts',(-5.2521153231257,-6.44834644354046,
17.1410937656149));
#245077=CARTESIAN_POINT('Ctrl Pts',(1.45047157124013,-8.81282241408086,
17.4060177086562));
#245078=CARTESIAN_POINT('Ctrl Pts',(8.20005226505081,-3.52277029322367,
17.7239264403057));
#245079=CARTESIAN_POINT('Ctrl Pts',(7.52752907318606,3.53620150433122,17.988850383347));
#245080=CARTESIAN_POINT('Ctrl Pts',(3.62484429538331,6.96809839719076,18.20078953778));
#245081=CARTESIAN_POINT('Ctrl Pts',(-0.152003807205115,7.86992152988776,
18.3597439036047));
#245082=CARTESIAN_POINT('Ctrl Pts',(-3.88419788878212,6.82692838766171,
18.5186982694295));
#245083=CARTESIAN_POINT('Ctrl Pts',(-7.66457774004274,3.24016926901836,
18.7306374238625));
#245084=CARTESIAN_POINT('Ctrl Pts',(-7.96804839137267,-2.40606049430473,
18.9425765782956));
#245085=CARTESIAN_POINT('Ctrl Pts',(-4.59126696645052,-6.3631625505062,
19.1545157327285));
#245086=CARTESIAN_POINT('Ctrl Pts',(0.203558650913005,-8.31411156401997,
19.3664548871616));
#245087=CARTESIAN_POINT('Ctrl Pts',(6.83294708480065,-5.75156855278744,
19.6313788302028));
#245088=CARTESIAN_POINT('Ctrl Pts',(8.52021671301704,2.65644025937182,19.9492875618523));
#245089=CARTESIAN_POINT('Ctrl Pts',(3.41879978163113,7.58157128041503,20.2142115048936));
#245090=CARTESIAN_POINT('Ctrl Pts',(-1.77774553726379,7.65071972061739,
20.4261506593266));
#245091=CARTESIAN_POINT('Ctrl Pts',(-5.23336362817136,5.87968325501715,
20.5851050251514));
#245092=CARTESIAN_POINT('Ctrl Pts',(-7.39032538650155,2.66026974780967,
20.7440593909761));
#245093=CARTESIAN_POINT('Ctrl Pts',(-7.92965512841919,-2.52289880284267,
20.9559985454091));
#245094=CARTESIAN_POINT('Ctrl Pts',(-4.48839085913739,-7.00951280511866,
21.1679376998422));
#245095=CARTESIAN_POINT('Ctrl Pts',(0.650188485748879,-7.81964352987934,
21.3798768542752));
#245096=CARTESIAN_POINT('Ctrl Pts',(5.56138958627605,-6.18359386546308,
21.5918160087082));
#245097=CARTESIAN_POINT('Ctrl Pts',(8.93108020914646,0.0742494369790274,
21.8567399517494));
#245098=CARTESIAN_POINT('Ctrl Pts',(4.74503129677803,7.55879922216376,22.174648683399));
#245099=CARTESIAN_POINT('Ctrl Pts',(-2.33321884082268,7.982762984564,22.4395726264402));
#245100=CARTESIAN_POINT('Ctrl Pts',(-6.3258395055626,4.65592590024462,22.6515117808733));
#245101=CARTESIAN_POINT('Ctrl Pts',(-7.79924106812923,1.06330090059327,
22.810466146698));
#245102=CARTESIAN_POINT('Ctrl Pts',(-7.34419956866848,-2.78508117387092,
22.9694205125228));
#245103=CARTESIAN_POINT('Ctrl Pts',(-4.38324354331086,-7.07330367403193,
23.1813596669558));
#245104=CARTESIAN_POINT('Ctrl Pts',(1.14866847572867,-8.24375418134102,
23.3932988213888));
#245105=CARTESIAN_POINT('Ctrl Pts',(5.57912262346678,-5.51751400122422,
23.6052379758219));
#245106=CARTESIAN_POINT('Ctrl Pts',(8.24606831740575,-1.08085361081387,
23.8171771302548));
#245107=CARTESIAN_POINT('Ctrl Pts',(6.73637673629011,5.86437849630028,24.0821010732962));
#245108=CARTESIAN_POINT('Ctrl Pts',(-1.3109133925462,8.82792579067301,24.4000098049456));
#245109=CARTESIAN_POINT('Ctrl Pts',(-6.96374633402792,4.54693875285423,
24.6649337479869));
#245110=CARTESIAN_POINT('Ctrl Pts',(-7.83333875277766,-0.57679755801928,
24.8768729024199));
#245111=CARTESIAN_POINT('Ctrl Pts',(-6.61631470119941,-4.26417047251733,
25.0358272682447));
#245112=CARTESIAN_POINT('Ctrl Pts',(-3.7679913926847,-6.89174762408888,
25.1947816340694));
#245113=CARTESIAN_POINT('Ctrl Pts',(1.27002945794566,-8.22383572312823,
25.4067207885025));
#245114=CARTESIAN_POINT('Ctrl Pts',(6.23360578781741,-5.51553090387492,
25.6186599429354));
#245115=CARTESIAN_POINT('Ctrl Pts',(7.82638094846845,-0.563321622906876,
25.8305990973685));
#245116=CARTESIAN_POINT('Ctrl Pts',(6.96717007609529,4.54141259456727,26.0425382518014));
#245117=CARTESIAN_POINT('Ctrl Pts',(1.30374863294259,8.83571990180765,26.3074621948428));
#245118=CARTESIAN_POINT('Ctrl Pts',(-6.73675098894321,5.85379823715844,
26.6253709264922));
#245119=CARTESIAN_POINT('Ctrl Pts',(-8.24706112548936,-1.07442906668484,
26.8902948695336));
#245120=CARTESIAN_POINT('Ctrl Pts',(-5.57564470996179,-5.53227597892406,
27.1022340239665));
#245121=CARTESIAN_POINT('Ctrl Pts',(-2.25317303860719,-7.54201440611787,
27.2611883897913));
#245122=CARTESIAN_POINT('Ctrl Pts',(1.61934947606041,-7.68580846260585,
27.4201427556161));
#245123=CARTESIAN_POINT('Ctrl Pts',(6.31284674624026,-5.42147717725839,
27.632081910049));
#245124=CARTESIAN_POINT('Ctrl Pts',(8.32228168115093,-0.136197977555209,
27.8440210644821));
#245125=CARTESIAN_POINT('Ctrl Pts',(6.31179034003158,4.66163841421322,28.0559602189151));
#245126=CARTESIAN_POINT('Ctrl Pts',(2.33941346813801,7.98079142995397,28.2678993733482));
#245127=CARTESIAN_POINT('Ctrl Pts',(-4.75554273106144,7.56006084725168,
28.5328233163894));
#245128=CARTESIAN_POINT('Ctrl Pts',(-8.92448406558058,0.0659685651278762,
28.850732048039));
#245129=CARTESIAN_POINT('Ctrl Pts',(-5.56632173875549,-6.17935897383808,
29.1156559910802));
#245130=CARTESIAN_POINT('Ctrl Pts',(-0.637946557518925,-7.82859601898417,
29.3275951455132));
#245131=CARTESIAN_POINT('Ctrl Pts',(3.19298472656766,-7.19469377943924,
29.486549511338));
#245132=CARTESIAN_POINT('Ctrl Pts',(6.22832954950417,-4.78558830994203,
29.6455038771627));
#245133=CARTESIAN_POINT('Ctrl Pts',(8.32131444745636,-0.0132170951335337,
29.8574430315957));
#245134=CARTESIAN_POINT('Ctrl Pts',(6.41074768537356,5.30860022830765,30.0693821860288));
#245135=CARTESIAN_POINT('Ctrl Pts',(1.76335791951407,7.64592302139324,30.2813213404618));
#245136=CARTESIAN_POINT('Ctrl Pts',(-3.41281179499102,7.584101982127,30.4932604948948));
#245137=CARTESIAN_POINT('Ctrl Pts',(-8.52902236822057,2.65056298236675,
30.758184437936));
#245138=CARTESIAN_POINT('Ctrl Pts',(-6.82255106480021,-5.75356973161703,
31.0760931695856));
#245139=CARTESIAN_POINT('Ctrl Pts',(-0.210059446353434,-8.31410187909029,
31.3410171126268));
#245140=CARTESIAN_POINT('Ctrl Pts',(4.60638867185572,-6.36200242396248,
31.5529562670599));
#245141=CARTESIAN_POINT('Ctrl Pts',(7.10439402150931,-3.38915264205359,
31.7119106328846));
#245142=CARTESIAN_POINT('Ctrl Pts',(7.84358429483301,0.414885356851344,
31.8708649987094));
#245143=CARTESIAN_POINT('Ctrl Pts',(6.33003717266334,5.40139595083994,32.0828041531424));
#245144=CARTESIAN_POINT('Ctrl Pts',(1.41780677859154,8.20175263026691,32.2947433075754));
#245145=CARTESIAN_POINT('Ctrl Pts',(-3.63265477501151,6.95509807888935,
32.5066824620084));
#245146=CARTESIAN_POINT('Ctrl Pts',(-7.5246259286918,3.5420180485976,32.7186216164415));
#245147=CARTESIAN_POINT('Ctrl Pts',(-8.20291959169172,-3.53296148483668,
32.9835455594827));
#245148=CARTESIAN_POINT('Ctrl Pts',(-1.44127265323067,-8.80758200798813,
33.3014542911322));
#245149=CARTESIAN_POINT('Ctrl Pts',(5.24717057422674,-6.45256662049017,
33.5663782341735));
#245150=CARTESIAN_POINT('Ctrl Pts',(7.63660495834726,-1.83743194400528,
33.7783173886065));
#245151=CARTESIAN_POINT('Ctrl Pts',(7.60098652584082,2.0454275538338,33.9372717544313));
#245152=CARTESIAN_POINT('Ctrl Pts',(5.68872110083175,5.41593913245269,34.096226120256));
#245153=CARTESIAN_POINT('Ctrl Pts',(1.29614751503337,8.21975975587624,34.3081652746891));
#245154=CARTESIAN_POINT('Ctrl Pts',(-4.25662087832244,7.15262895498851,
34.520104429122));
#245155=CARTESIAN_POINT('Ctrl Pts',(-7.28258603280336,2.92121732779361,
34.7320435835551));
#245156=CARTESIAN_POINT('Ctrl Pts',(-8.0196334935899,-2.20258163340734,
34.943982737988));
#245157=CARTESIAN_POINT('Ctrl Pts',(-3.93397982316526,-8.01832335541715,
35.2089066810293));
#245158=CARTESIAN_POINT('Ctrl Pts',(4.63277167774011,-7.62811865864157,
35.5268154126789));
#245159=CARTESIAN_POINT('Ctrl Pts',(8.18228173064822,-1.489523651103,35.7917393557201));
#245160=CARTESIAN_POINT('Ctrl Pts',(6.99619053994434,3.57032342617563,36.0036785101531));
#245161=CARTESIAN_POINT('Ctrl Pts',(4.44406877510223,6.4968471404334,36.1626328759779));
#245162=CARTESIAN_POINT('Ctrl Pts',(0.79950220057253,7.81375330303946,36.3215872418026));
#245163=CARTESIAN_POINT('Ctrl Pts',(-4.36075182984694,7.08719213112898,
36.5335263962357));
#245164=CARTESIAN_POINT('Ctrl Pts',(-7.88504990360797,2.66550375860217,
36.7454655506687));
#245165=CARTESIAN_POINT('Ctrl Pts',(-7.43205025729338,-2.51678345799743,
36.9574047051017));
#245166=CARTESIAN_POINT('Ctrl Pts',(-4.65990284639874,-6.88848261124738,
37.1693438595348));
#245167=CARTESIAN_POINT('Ctrl Pts',(2.2258770754351,-8.64957674838206,37.4342678025759));
#245168=CARTESIAN_POINT('Ctrl Pts',(8.48001574055104,-2.78210365162642,
37.7521765342255));
#245169=CARTESIAN_POINT('Ctrl Pts',(7.18447574385862,4.18947768973679,38.0171004772667));
#245170=CARTESIAN_POINT('Ctrl Pts',(2.99296870210795,7.2619577103497,38.2290396316998));
#245171=CARTESIAN_POINT('Ctrl Pts',(-0.848946808315632,7.82547502460054,
38.3879939975245));
#245172=CARTESIAN_POINT('Ctrl Pts',(-4.47400753862085,6.45578817758485,
38.5469483633493));
#245173=CARTESIAN_POINT('Ctrl Pts',(-7.92160068496547,2.54807602182595,
38.7588875177823));
#245174=CARTESIAN_POINT('Ctrl Pts',(-7.7234300205534,-3.10282951306144,
38.9708266722154));
#245175=CARTESIAN_POINT('Ctrl Pts',(-4.0092055796552,-6.74506046091847,
39.1827658266483));
#245176=CARTESIAN_POINT('Ctrl Pts',(0.939669008123714,-8.26334734708059,
39.3947049810814));
#245177=CARTESIAN_POINT('Ctrl Pts',(7.3158380211903,-5.12330174094849,39.6596289241226));
#245178=CARTESIAN_POINT('Ctrl Pts',(8.25123304473913,3.40116464314677,39.9775376557722));
#245179=CARTESIAN_POINT('Ctrl Pts',(2.73336067432644,7.85475362127551,40.2424615988134));
#245180=CARTESIAN_POINT('Ctrl Pts',(-2.4488613754721,7.46304022516467,40.4544007532464));
#245181=CARTESIAN_POINT('Ctrl Pts',(-5.73390537707544,5.39268941908779,
40.6133551190712));
#245182=CARTESIAN_POINT('Ctrl Pts',(-7.59702900000426,1.99476685920308,
40.7723094848959));
#245183=CARTESIAN_POINT('Ctrl Pts',(-7.67483203665867,-3.2158050367097,
40.984248639329));
#245184=CARTESIAN_POINT('Ctrl Pts',(-3.84944586892954,-7.3797485574843,
41.1961877937619));
#245185=CARTESIAN_POINT('Ctrl Pts',(1.3407144388163,-7.73123889133776,41.4081269481951));
#245186=CARTESIAN_POINT('Ctrl Pts',(6.08757707586265,-5.66632972644233,
41.6200661026279));
#245187=CARTESIAN_POINT('Ctrl Pts',(8.88934894509868,0.865553010145839,
41.8849900456693));
#245188=CARTESIAN_POINT('Ctrl Pts',(4.05639088500875,7.94962015925316,42.2028987773188));
#245189=CARTESIAN_POINT('Ctrl Pts',(-3.03157875478146,7.74454293554194,
42.4678227203601));
#245190=CARTESIAN_POINT('Ctrl Pts',(-6.71361527772728,4.07691811806076,
42.6797618747931));
#245191=CARTESIAN_POINT('Ctrl Pts',(-7.86278984604215,0.36783947718078,
42.8387162406178));
#245192=CARTESIAN_POINT('Ctrl Pts',(-7.06844244113665,-3.42506436520817,
42.9976706064427));
#245193=CARTESIAN_POINT('Ctrl Pts',(-3.73905835505177,-7.43396875447881,
43.2096097608755));
#245194=CARTESIAN_POINT('Ctrl Pts',(1.87482309910048,-8.10949817291979,
43.4215489153087));
#245195=CARTESIAN_POINT('Ctrl Pts',(6.04620311476629,-5.00129962073608,
43.6334880697416));
#245196=CARTESIAN_POINT('Ctrl Pts',(8.30941427114553,-0.345719096687952,
43.8454272241747));
#245197=CARTESIAN_POINT('Ctrl Pts',(6.19008193137986,6.43836876575923,44.1103511672159));
#245198=CARTESIAN_POINT('Ctrl Pts',(-2.08820682902614,8.67699025743347,
44.4282598988655));
#245199=CARTESIAN_POINT('Ctrl Pts',(-7.33935153427196,3.91181979176889,
44.6931838419066));
#245200=CARTESIAN_POINT('Ctrl Pts',(-7.75138513226923,-1.26882621739172,
44.9051229963398));
#245201=CARTESIAN_POINT('Ctrl Pts',(-6.21232498471946,-4.83381715916377,
45.0640773621644));
#245202=CARTESIAN_POINT('Ctrl Pts',(-3.1423196732166,-7.19859510743567,
45.2230317279893));
#245203=CARTESIAN_POINT('Ctrl Pts',(1.99394098904562,-8.07890142019655,
45.4349708824222));
#245204=CARTESIAN_POINT('Ctrl Pts',(6.69793464556163,-4.9413149821981,45.6469100368553));
#245205=CARTESIAN_POINT('Ctrl Pts',(7.84550783565501,0.132577532259812,
45.8588491912883));
#245206=CARTESIAN_POINT('Ctrl Pts',(6.5372264605892,5.14106578700417,46.0707883457213));
#245207=CARTESIAN_POINT('Ctrl Pts',(0.515473790672442,8.9165011889322,46.3357122887626));
#245208=CARTESIAN_POINT('Ctrl Pts',(-7.22908153439403,5.23365530556507,
46.653621020412));
#245209=CARTESIAN_POINT('Ctrl Pts',(-8.11937222462681,-1.80116898287009,
46.9185449634533));
#245210=CARTESIAN_POINT('Ctrl Pts',(-5.06335374042494,-6.00469319266439,
47.1304841178864));
#245211=CARTESIAN_POINT('Ctrl Pts',(-1.57582759165378,-7.71203847535647,
47.2894384837111));
#245212=CARTESIAN_POINT('Ctrl Pts',(2.29419876660426,-7.51203011633953,
47.448392849536));
#245213=CARTESIAN_POINT('Ctrl Pts',(6.76852739204454,-4.84060799571636,
47.6603320039688));
#245214=CARTESIAN_POINT('Ctrl Pts',(8.30159923837348,0.601973716159747,
47.8722711584019));
#245215=CARTESIAN_POINT('Ctrl Pts',(5.87377004300275,5.2027296185087,48.0842103128349));
#245216=CARTESIAN_POINT('Ctrl Pts',(1.62283811694658,8.15673241374986,48.2961494672681));
#245217=CARTESIAN_POINT('Ctrl Pts',(-5.40690334344646,7.10880460525727,
48.5610734103091));
#245218=CARTESIAN_POINT('Ctrl Pts',(-8.89520681995229,-0.725302225738014,
48.8789821419588));
#245219=CARTESIAN_POINT('Ctrl Pts',(-4.99671402105694,-6.64840311794251,
49.1439060849999));
#245220=CARTESIAN_POINT('Ctrl Pts',(0.0584426308466855,-7.8543284816466,
49.3558452394331));
#245221=CARTESIAN_POINT('Ctrl Pts',(3.81811125282832,-6.88337101317528,
49.5147996052577));
#245222=CARTESIAN_POINT('Ctrl Pts',(6.62798156908878,-4.21471289286708,
49.6737539710826));
#245223=CARTESIAN_POINT('Ctrl Pts',(8.28973554545862,0.724384850345556,
49.8856931255155));
#245224=CARTESIAN_POINT('Ctrl Pts',(5.91499521963495,5.85591613850521,50.0976322799486));
#245225=CARTESIAN_POINT('Ctrl Pts',(1.0787304308988,7.77212394772737,50.3095714343816));
#245226=CARTESIAN_POINT('Ctrl Pts',(-4.07158788133815,7.25176249941163,
50.5215105888146));
#245227=CARTESIAN_POINT('Ctrl Pts',(-8.73038403875477,1.88417122814108,
50.7864345318559));
#245228=CARTESIAN_POINT('Ctrl Pts',(-6.2857385062876,-6.3356340739471,51.1043432635053));
#245229=CARTESIAN_POINT('Ctrl Pts',(0.527677938456462,-8.29999825422641,
51.3692672065466));
#245230=CARTESIAN_POINT('Ctrl Pts',(5.1521478128489,-5.92868150209316,51.5812063609797));
#245231=CARTESIAN_POINT('Ctrl Pts',(7.37682666022324,-2.74612426321454,
51.7401607268044));
#245232=CARTESIAN_POINT('Ctrl Pts',(7.77594124838299,1.10845935928047,51.8991150926292));
#245233=CARTESIAN_POINT('Ctrl Pts',(5.82637752128669,5.94119296139214,52.1110542470622));
#245234=CARTESIAN_POINT('Ctrl Pts',(0.685273979183349,8.29513844628072,
52.3229934014952));
#245235=CARTESIAN_POINT('Ctrl Pts',(-4.23481459867255,6.60574865675754,
52.5349325559282));
#245236=CARTESIAN_POINT('Ctrl Pts',(-7.80895369693254,2.86114127272587,
52.7468717103612));
#245237=CARTESIAN_POINT('Ctrl Pts',(-7.85749528809018,-4.24611286693366,
53.0117956534025));
#245238=CARTESIAN_POINT('Ctrl Pts',(-0.654950523743482,-8.90066331796877,
53.3297043850521));
#245239=CARTESIAN_POINT('Ctrl Pts',(5.7984348266577,-5.96209431222774,53.5946283280932));
#245240=CARTESIAN_POINT('Ctrl Pts',(7.76940802209826,-1.15333881615956,
53.8065674825263));
#245241=CARTESIAN_POINT('Ctrl Pts',(7.38977708548394,2.71108182666114,53.965521848351));
#245242=CARTESIAN_POINT('Ctrl Pts',(5.18629647367542,5.89883660874095,54.1244762141758));
#245243=CARTESIAN_POINT('Ctrl Pts',(0.562497492298242,8.30229157499353,
54.3364153686088));
#245244=CARTESIAN_POINT('Ctrl Pts',(-4.87383286167256,6.74719760389385,
54.5483545230418));
#245245=CARTESIAN_POINT('Ctrl Pts',(-7.51284246057468,2.264236772948,54.7602936774749));
#245246=CARTESIAN_POINT('Ctrl Pts',(-7.79284720783111,-2.90472367338639,
54.9722328319079));
#245247=CARTESIAN_POINT('Ctrl Pts',(-3.20780210334241,-8.33544913888216,
55.2371567749491));
#245248=CARTESIAN_POINT('Ctrl Pts',(5.29064770703959,-7.18747622802216,
55.5550655065987));
#245249=CARTESIAN_POINT('Ctrl Pts',(8.28210071942974,-0.758434374298012,
55.8199894496399));
#245250=CARTESIAN_POINT('Ctrl Pts',(6.65220405514383,4.17637075071561,56.031928604073));
#245251=CARTESIAN_POINT('Ctrl Pts',(3.85073774300707,6.86517216671053,56.1908829698977));
#245252=CARTESIAN_POINT('Ctrl Pts',(0.103792740727409,7.85386347706992,
56.3498373357225));
#245253=CARTESIAN_POINT('Ctrl Pts',(-4.97175406669828,6.67278879669655,
56.5617764901554));
#245254=CARTESIAN_POINT('Ctrl Pts',(-8.09027032914091,1.9561309442193,56.7737156445885));
#245255=CARTESIAN_POINT('Ctrl Pts',(-7.17972762657543,-3.16560913720782,
56.9856547990215));
#245256=CARTESIAN_POINT('Ctrl Pts',(-4.03101020161681,-7.27439646828475,
57.1975939534545));
#245257=CARTESIAN_POINT('Ctrl Pts',(2.98376171108668,-8.41824641671605,
57.4625178964958));
#245258=CARTESIAN_POINT('Ctrl Pts',(8.69322924019813,-2.01953783469166,
57.7804266281453));
#245259=CARTESIAN_POINT('Ctrl Pts',(6.78487021025572,4.80977663274288,58.0453505711865));
#245260=CARTESIAN_POINT('Ctrl Pts',(2.33753412088888,7.49865492421042,58.2572897256197));
#245261=CARTESIAN_POINT('Ctrl Pts',(-1.53920737148137,7.71943072457896,
58.4162440914443));
#245262=CARTESIAN_POINT('Ctrl Pts',(-5.02860028505904,6.03383158719109,
58.5751984572691));
#245263=CARTESIAN_POINT('Ctrl Pts',(-8.11626918732383,1.83592573486714,
58.7871376117021));
#245264=CARTESIAN_POINT('Ctrl Pts',(-7.41801709661686,-3.77517478056459,
58.9990767661352));
#245265=CARTESIAN_POINT('Ctrl Pts',(-3.39558595242505,-7.07386500020164,
59.2110159205681));
#245266=CARTESIAN_POINT('Ctrl Pts',(1.66838281260135,-8.14753864758852,
59.4229550750012));
#245267=CARTESIAN_POINT('Ctrl Pts',(7.74114274238885,-4.45470714223283,
59.6878790180424));
#245268=CARTESIAN_POINT('Ctrl Pts',(7.91730025097074,4.11911694715805,60.0057877496919));
#245269=CARTESIAN_POINT('Ctrl Pts',(2.02640606933998,8.06610770254379,60.2707116927332));
#245270=CARTESIAN_POINT('Ctrl Pts',(-3.10070113652638,7.21661582049712,
60.4826508471663));
#245271=CARTESIAN_POINT('Ctrl Pts',(-6.18931300628282,4.86324732604201,
60.6416052129909));
#245272=CARTESIAN_POINT('Ctrl Pts',(-7.74393301904625,1.31356227336414,
60.8005595788158));
#245273=CARTESIAN_POINT('Ctrl Pts',(-7.35959692812879,-3.88339823872434,
61.0124987332486));
#245274=CARTESIAN_POINT('Ctrl Pts',(-3.18020017803199,-7.69189502639994,
61.2244378876819));
#245275=CARTESIAN_POINT('Ctrl Pts',(2.02068703217843,-7.58197823258349,
61.4363770421147));
#245276=CARTESIAN_POINT('Ctrl Pts',(6.56584653849631,-5.10446338572904,
61.6483161965479));
#245277=CARTESIAN_POINT('Ctrl Pts',(8.77764566147108,1.65004343056681,61.9132401395891));
#245278=CARTESIAN_POINT('Ctrl Pts',(3.33582081627798,8.27786610003282,62.2311488712386));
#245279=CARTESIAN_POINT('Ctrl Pts',(-3.70607576389775,7.44536214425762,
62.4960728142798));
#245280=CARTESIAN_POINT('Ctrl Pts',(-7.04854519778669,3.46581909993344,
62.7080119687128));
#245281=CARTESIAN_POINT('Ctrl Pts',(-7.86444710766331,-0.330517374373583,
62.8669663345378));
#245282=CARTESIAN_POINT('Ctrl Pts',(-6.73704645906731,-4.0380873514387,
63.0259207003624));
#245283=CARTESIAN_POINT('Ctrl Pts',(-3.06544137532573,-7.73611776018765,
63.2378598547954));
#245284=CARTESIAN_POINT('Ctrl Pts',(2.58622015592732,-7.9114086972287,63.4497990092285));
#245285=CARTESIAN_POINT('Ctrl Pts',(6.46569125196403,-4.44571778632658,
63.6617381636614));
#245286=CARTESIAN_POINT('Ctrl Pts',(8.30735312908238,0.39213672622584,63.8736773180945));
#245287=CARTESIAN_POINT('Ctrl Pts',(5.59506223820433,6.96167977083983,64.1386012611357));
#245288=CARTESIAN_POINT('Ctrl Pts',(-2.84906306070886,8.45775427430321,
64.4565099927852));
#245289=CARTESIAN_POINT('Ctrl Pts',(-7.65718543400385,3.24590915710281,
64.7214339358265));
#245290=CARTESIAN_POINT('Ctrl Pts',(-7.60841691152547,-1.95086738122589,
64.9333730902595));
#245291=CARTESIAN_POINT('Ctrl Pts',(-5.75943529500526,-5.36541472084175,
65.0923274560842));
#245292=CARTESIAN_POINT('Ctrl Pts',(-2.49191335788211,-7.44877924671545,
65.2512818219091));
#245293=CARTESIAN_POINT('Ctrl Pts',(2.70215732371306,-7.8703744906464,65.4632209763419));
#245294=CARTESIAN_POINT('Ctrl Pts',(7.10954108041586,-4.32820377236875,
65.6751601307752));
#245295=CARTESIAN_POINT('Ctrl Pts',(7.80287924095887,0.827433110696188,
65.887099285208));
#245296=CARTESIAN_POINT('Ctrl Pts',(6.05582542777371,5.70025136386296,66.0990384396412));
#245297=CARTESIAN_POINT('Ctrl Pts',(-0.276858574999038,8.92709672907416,
66.3639623826822));
#245298=CARTESIAN_POINT('Ctrl Pts',(-7.66450876371097,4.57231594512697,
66.681871114332));
#245299=CARTESIAN_POINT('Ctrl Pts',(-7.92777213317072,-2.51373109686328,
66.9467950573731));
#245300=CARTESIAN_POINT('Ctrl Pts',(-4.51120686176332,-6.42984479530528,
67.1587342118062));
#245301=CARTESIAN_POINT('Ctrl Pts',(-0.886078103971636,-7.8213576595246,
67.3176885776309));
#245302=CARTESIAN_POINT('Ctrl Pts',(2.95098939665996,-7.27912123939608,
67.4766429434557));
#245303=CARTESIAN_POINT('Ctrl Pts',(7.17092995154372,-4.2216362360521,67.6885820978886));
#245304=CARTESIAN_POINT('Ctrl Pts',(8.21557120872505,1.33540700803337,67.9005212523217));
#245305=CARTESIAN_POINT('Ctrl Pts',(5.38951469707404,5.70286782255762,68.1124604067547));
#245306=CARTESIAN_POINT('Ctrl Pts',(0.893488666859789,8.26846813139917,
68.3243995611877));
#245307=CARTESIAN_POINT('Ctrl Pts',(-6.01570377578533,6.60159179412591,
68.589323504229));
#245308=CARTESIAN_POINT('Ctrl Pts',(-8.79591151323072,-1.51086382949544,
68.9072322358786));
#245309=CARTESIAN_POINT('Ctrl Pts',(-4.38777482885245,-7.06511474193006,
69.1721561789197));
#245310=CARTESIAN_POINT('Ctrl Pts',(0.75437163081327,-7.81823600615633,
69.3840953333529));
#245311=CARTESIAN_POINT('Ctrl Pts',(4.41318407711473,-6.51786622649009,
69.5430496991776));
#245312=CARTESIAN_POINT('Ctrl Pts',(6.97546114514699,-3.61066149413494,
69.7020040650023));
#245313=CARTESIAN_POINT('Ctrl Pts',(8.19290593630667,1.4562846082975,69.9139432194354));
#245314=CARTESIAN_POINT('Ctrl Pts',(5.37268034101302,6.35713797319922,70.1258823738682));
#245315=CARTESIAN_POINT('Ctrl Pts',(0.385615112503278,7.83714650892533,
70.3378215283014));
#245316=CARTESIAN_POINT('Ctrl Pts',(-4.69832249301022,6.86234238559436,
70.5497606827343));
#245317=CARTESIAN_POINT('Ctrl Pts',(-8.86300835786554,1.10294573286832,
70.8146846257757));
#245318=CARTESIAN_POINT('Ctrl Pts',(-5.69947739928546,-6.86782325365974,
71.1325933574252));
#245319=CARTESIAN_POINT('Ctrl Pts',(1.26131134764555,-8.22056938840904,
71.3975173004663));
#245320=CARTESIAN_POINT('Ctrl Pts',(5.65728340963835,-5.44868257745799,
71.6094564548995));
#245321=CARTESIAN_POINT('Ctrl Pts',(7.59134286873771,-2.08150328900666,
71.7684108207242));
#245322=CARTESIAN_POINT('Ctrl Pts',(7.64681098033558,1.79335174723873,71.927365186549));
#245323=CARTESIAN_POINT('Ctrl Pts',(5.27749319719932,6.4341248068459,72.139304340982));
#245324=CARTESIAN_POINT('Ctrl Pts',(-0.0538749626755808,8.32342009874787,
72.351243495415));
#245325=CARTESIAN_POINT('Ctrl Pts',(-4.80221181121656,6.20417977333355,
72.563182649848));
#245326=CARTESIAN_POINT('Ctrl Pts',(-8.03515042318792,2.15826191845753,
72.775121804281));
#245327=CARTESIAN_POINT('Ctrl Pts',(-7.44316476216323,-4.92692186719272,
73.0400457473223));
#245328=CARTESIAN_POINT('Ctrl Pts',(0.124338371616316,-8.92190591677168,
73.3579544789718));
#245329=CARTESIAN_POINT('Ctrl Pts',(7.56292883494232,-4.72784949414696,
73.6758632106214));
#245330=CARTESIAN_POINT('Ctrl Pts',(8.07241182584164,3.8018322885345,73.9937719422708));
#245331=CARTESIAN_POINT('Ctrl Pts',(1.1721054173287,8.84175448043975,74.3116806739204));
#245332=CARTESIAN_POINT('Ctrl Pts',(-6.79899311505185,5.77836982546636,
74.6295894055698));
#245333=CARTESIAN_POINT('Ctrl Pts',(-8.53900169652047,-2.60013668658995,
74.9474981372195));
#245334=CARTESIAN_POINT('Ctrl Pts',(-3.45384967879028,-7.56919145141941,
75.2124220802606));
#245335=CARTESIAN_POINT('Ctrl Pts',(1.72439296830596,-7.65372810011474,
75.4243612346938));
#245336=CARTESIAN_POINT('Ctrl Pts',(6.38248034882689,-5.34286152250664,
75.6363003891266));
#245337=CARTESIAN_POINT('Ctrl Pts',(8.32160028852796,-0.0294128292769415,
75.8482395435598));
#245338=CARTESIAN_POINT('Ctrl Pts',(6.25293669920985,4.75295816244786,76.0601786979928));
#245339=CARTESIAN_POINT('Ctrl Pts',(3.23035682717462,7.1781569544004,76.2191330638176));
#245340=CARTESIAN_POINT('Ctrl Pts',(-0.597346084762983,7.83174150887795,
76.3780874296422));
#245341=CARTESIAN_POINT('Ctrl Pts',(-5.5341526716022,6.20820598826635,76.5900265840752));
#245342=CARTESIAN_POINT('Ctrl Pts',(-8.92472137507585,-0.0196785603991093,
76.8549505271166));
#245343=CARTESIAN_POINT('Ctrl Pts',(-4.79470389098473,-7.53526516049846,
77.1728592587661));
#245344=CARTESIAN_POINT('Ctrl Pts',(2.29796072061545,-7.99283140019599,
77.4377832018074));
#245345=CARTESIAN_POINT('Ctrl Pts',(6.28751497364375,-4.69432847951197,
77.6497223562402));
#245346=CARTESIAN_POINT('Ctrl Pts',(8.32287495204422,0.0930042452481067,
77.8616615106735));
#245347=CARTESIAN_POINT('Ctrl Pts',(6.34089786961344,5.3886442403136,78.0736006651065));
#245348=CARTESIAN_POINT('Ctrl Pts',(1.65921369754144,7.67730060102996,78.2855398195393));
#245349=CARTESIAN_POINT('Ctrl Pts',(-2.2140023866738,7.55360624316107,78.4444941853642));
#245350=CARTESIAN_POINT('Ctrl Pts',(-5.54685934390654,5.56113677446008,
78.6034485511889));
#245351=CARTESIAN_POINT('Ctrl Pts',(-8.24137413950221,1.11721374771911,
78.8153877056219));
#245352=CARTESIAN_POINT('Ctrl Pts',(-6.76703924878134,-5.8187583439523,
79.0803116486632));
#245353=CARTESIAN_POINT('Ctrl Pts',(1.25787713722511,-8.84236683484207,
79.3982203803127));
#245354=CARTESIAN_POINT('Ctrl Pts',(6.94350807591193,-4.57750836564132,
79.663144323354));
#245355=CARTESIAN_POINT('Ctrl Pts',(7.82919898218652,0.522698162297944,
79.875083477787));
#245356=CARTESIAN_POINT('Ctrl Pts',(6.26214530801236,5.4831066289172,80.08702263222));
#245357=CARTESIAN_POINT('Ctrl Pts',(1.31269087512095,8.21713402263037,80.298961786653));
#245358=CARTESIAN_POINT('Ctrl Pts',(-3.73217515603941,6.91120923150708,
80.510900941086));
#245359=CARTESIAN_POINT('Ctrl Pts',(-6.59409621375978,4.29844915850133,
80.6698553069108));
#245360=CARTESIAN_POINT('Ctrl Pts',(-7.83023991261764,0.617441780400932,
80.8288096727356));
#245361=CARTESIAN_POINT('Ctrl Pts',(-6.98724940777033,-4.51073838040169,
81.0407488271686));
#245362=CARTESIAN_POINT('Ctrl Pts',(-1.35670925061133,-8.82100378077065,
81.3056727702099));
#245363=CARTESIAN_POINT('Ctrl Pts',(6.70585217355222,-5.89925870828381,
81.6235815018593));
#245364=CARTESIAN_POINT('Ctrl Pts',(8.25156648580112,1.03804515956493,81.8885054449006));
#245365=CARTESIAN_POINT('Ctrl Pts',(5.60768125197603,5.48848621915918,82.1004445993336));
#245366=CARTESIAN_POINT('Ctrl Pts',(1.19143489443458,8.23768202600654,82.3123837537668));
#245367=CARTESIAN_POINT('Ctrl Pts',(-4.34647681532778,7.09595575796037,
82.5243229081995));
#245368=CARTESIAN_POINT('Ctrl Pts',(-7.32964717965211,2.82315721689529,
82.7362620626329));
#245369=CARTESIAN_POINT('Ctrl Pts',(-7.80465416182032,-1.02281154586677,
82.8952164284572));
#245370=CARTESIAN_POINT('Ctrl Pts',(-6.34991677060407,-4.62303454941871,
83.0541707942825));
#245371=CARTESIAN_POINT('Ctrl Pts',(-2.37461486514492,-7.97054698682075,
83.266109948715));
#245372=CARTESIAN_POINT('Ctrl Pts',(4.7057401633254,-7.58332230646015,83.5310338917566));
#245373=CARTESIAN_POINT('Ctrl Pts',(8.93057461629925,-0.120597279459235,
83.8489426234059));
#245374=CARTESIAN_POINT('Ctrl Pts',(5.59340514972506,6.15464914145068,84.1138665664474));
#245375=CARTESIAN_POINT('Ctrl Pts',(0.690760647269976,7.81616400349735,
84.3258057208802));
#245376=CARTESIAN_POINT('Ctrl Pts',(-4.45195376509949,7.03271142184339,
84.5377448753135));
#245377=CARTESIAN_POINT('Ctrl Pts',(-7.91645548039882,2.56401666373547,
84.7496840297463));
#245378=CARTESIAN_POINT('Ctrl Pts',(-7.40403163563121,-2.62188100188642,
84.9616231841794));
#245379=CARTESIAN_POINT('Ctrl Pts',(-5.26380643066461,-5.85244495100042,
85.1205775500041));
#245380=CARTESIAN_POINT('Ctrl Pts',(-1.81742586590513,-7.64139088521482,
85.279531915829));
#245381=CARTESIAN_POINT('Ctrl Pts',(3.37940832923157,-7.59921143087983,
85.4914710702619));
#245382=CARTESIAN_POINT('Ctrl Pts',(8.50631608405412,-2.70062110755077,
85.756395013303));
#245383=CARTESIAN_POINT('Ctrl Pts',(6.86270348148387,5.71603075624413,86.0743037449527));
#245384=CARTESIAN_POINT('Ctrl Pts',(0.246702924124477,8.31294321468396,
86.3392276879939));
#245385=CARTESIAN_POINT('Ctrl Pts',(-4.5581827942018,6.38690375816221,86.5511668424269));
#245386=CARTESIAN_POINT('Ctrl Pts',(-7.95545457184888,2.44737917470092,
86.7631059968599));
#245387=CARTESIAN_POINT('Ctrl Pts',(-7.6812897496541,-3.20034945074897,
86.975045151293));
#245388=CARTESIAN_POINT('Ctrl Pts',(-3.91957469415952,-6.8066789748294,
87.186984305726));
#245389=CARTESIAN_POINT('Ctrl Pts',(-0.192843600664311,-7.86902671171469,
87.3459386715508));
#245390=CARTESIAN_POINT('Ctrl Pts',(3.58863375468831,-6.98681609987104,
87.5048930373757));
#245391=CARTESIAN_POINT('Ctrl Pts',(7.50907619223898,-3.57521884169963,
87.7168321918084));
#245392=CARTESIAN_POINT('Ctrl Pts',(8.21822365360159,3.48016776431378,87.9817561348498));
#245393=CARTESIAN_POINT('Ctrl Pts',(1.49618716924779,8.80517635460401,88.2996648664993));
#245394=CARTESIAN_POINT('Ctrl Pts',(-5.21858018044238,6.47551605075817,
88.5645888095405));
#245395=CARTESIAN_POINT('Ctrl Pts',(-7.61617805723871,1.88769748683935,
88.7765279639737));
#245396=CARTESIAN_POINT('Ctrl Pts',(-7.63506557650729,-3.31431680922974,
88.9884671184066));
#245397=CARTESIAN_POINT('Ctrl Pts',(-3.75401500422844,-7.42642714722755,
89.2004062728397));
#245398=CARTESIAN_POINT('Ctrl Pts',(1.44887537003911,-7.71976065766127,
89.4123454272726));
#245399=CARTESIAN_POINT('Ctrl Pts',(4.97081194366405,-6.10326131381598,
89.5712997930973));
#245400=CARTESIAN_POINT('Ctrl Pts',(7.26977119842067,-2.97393983821432,
89.7302541589222));
#245401=CARTESIAN_POINT('Ctrl Pts',(8.02941166382867,2.16724787684003,89.942193313355));
#245402=CARTESIAN_POINT('Ctrl Pts',(3.97993814034131,7.98817000867177,90.2071172563967));
#245403=CARTESIAN_POINT('Ctrl Pts',(-4.58949041866838,7.66200263495448,
90.5250259880459));
#245404=CARTESIAN_POINT('Ctrl Pts',(-8.17548675502426,1.52555024229132,
90.7899499310872));
#245405=CARTESIAN_POINT('Ctrl Pts',(-7.01336106360832,-3.51885444325954,
91.0018890855202));
#245406=CARTESIAN_POINT('Ctrl Pts',(-3.64478579961144,-7.4829445236792,
91.2138282399533));
#245407=CARTESIAN_POINT('Ctrl Pts',(1.97767450617641,-8.08289876051093,
91.4257673943862));
#245408=CARTESIAN_POINT('Ctrl Pts',(6.12090517289929,-4.92224179758123,
91.6377065488193));
#245409=CARTESIAN_POINT('Ctrl Pts',(7.74518389296699,-1.40388621623011,
91.7966609146438));
#245410=CARTESIAN_POINT('Ctrl Pts',(7.45660122098534,2.46839819921847,91.955615280469));
#245411=CARTESIAN_POINT('Ctrl Pts',(4.69030892220141,6.86799950795086,92.1675544349015));
#245412=CARTESIAN_POINT('Ctrl Pts',(-2.17135494908673,8.65655736268543,
92.4324783779433));
#245413=CARTESIAN_POINT('Ctrl Pts',(-8.46917142270095,2.83599049610602,
92.7503871095924));
#245414=CARTESIAN_POINT('Ctrl Pts',(-7.20274227732176,-4.15769057408234,
93.0153110526339));
#245415=CARTESIAN_POINT('Ctrl Pts',(-3.03948342129891,-7.23402450459174,
93.2272502070669));
#245416=CARTESIAN_POINT('Ctrl Pts',(2.09740634433605,-8.05480036352543,
93.4391893614998));
#245417=CARTESIAN_POINT('Ctrl Pts',(6.75876976609282,-4.85422291144522,
93.6511285159329));
#245418=CARTESIAN_POINT('Ctrl Pts',(7.85084453217398,0.241214802851541,
93.8630676703659));
#245419=CARTESIAN_POINT('Ctrl Pts',(6.79673529994191,3.97028453722395,94.0220220361907));
#245420=CARTESIAN_POINT('Ctrl Pts',(4.05932161038303,6.72426944003453,94.1809764020154));
#245421=CARTESIAN_POINT('Ctrl Pts',(-0.903250091444178,8.26756035957407,
94.3929155564486));
#245422=CARTESIAN_POINT('Ctrl Pts',(-7.27895883489408,5.16406099579625,
94.6578394994895));
#245423=CARTESIAN_POINT('Ctrl Pts',(-8.27803812656465,-3.35317632346431,
94.9757482311394));
#245424=CARTESIAN_POINT('Ctrl Pts',(-2.76790867666667,-7.84248486010434,
95.2406721741806));
#245425=CARTESIAN_POINT('Ctrl Pts',(2.39536034850992,-7.47206924500643,
95.4526113286135));
#245426=CARTESIAN_POINT('Ctrl Pts',(6.83145361629515,-4.75501459071554,
95.6645504830465));
#245427=CARTESIAN_POINT('Ctrl Pts',(8.29117690268064,0.707696540548531,
95.8764896374795));
#245428=CARTESIAN_POINT('Ctrl Pts',(5.80717622726645,5.28872845918113,96.0884287919126));
#245429=CARTESIAN_POINT('Ctrl Pts',(2.5813499698349,7.43608784087639,96.2473831577373));
#245430=CARTESIAN_POINT('Ctrl Pts',(-1.28912224472129,7.74803557534874,
96.406337523562));
#245431=CARTESIAN_POINT('Ctrl Pts',(-6.06265053096723,5.6932138170156,96.6182766779951));
#245432=CARTESIAN_POINT('Ctrl Pts',(-8.88783914592498,-0.81060656581987,
96.8832006210364));
#245433=CARTESIAN_POINT('Ctrl Pts',(-4.10796116509668,-7.93059655682706,
97.2011093526859));
#245434=CARTESIAN_POINT('Ctrl Pts',(2.99735521759814,-7.75768966399591,
97.4660332957272));
#245435=CARTESIAN_POINT('Ctrl Pts',(6.67884388789089,-4.11856945098259,
97.67797245016));
#245436=CARTESIAN_POINT('Ctrl Pts',(8.2818763535548,0.830329051605735,97.8899116045933));
#245437=CARTESIAN_POINT('Ctrl Pts',(5.83832505511409,5.92945270458212,98.1018507590259));
#245438=CARTESIAN_POINT('Ctrl Pts',(0.972215262230236,7.79414792862997,
98.3137899134594));
#245439=CARTESIAN_POINT('Ctrl Pts',(-2.87479385321957,7.3276415268139,98.4727442792838));
#245440=CARTESIAN_POINT('Ctrl Pts',(-6.01793319755471,5.04761047115112,
98.631698645109));
#245441=CARTESIAN_POINT('Ctrl Pts',(-8.30796135692593,0.382352087374534,
98.8436377995414));
#245442=CARTESIAN_POINT('Ctrl Pts',(-6.2246672233863,-6.39564583497924,
99.1085617425833));
#245443=CARTESIAN_POINT('Ctrl Pts',(2.03665925768212,-8.69607530724048,
99.4264704742322));
#245444=CARTESIAN_POINT('Ctrl Pts',(7.32190243800059,-3.94406286863336,
99.6913944172741));
#245445=CARTESIAN_POINT('Ctrl Pts',(7.75205668761658,1.21457281105868,99.9033335717067));
#245446=CARTESIAN_POINT('Ctrl Pts',(5.75151053316249,6.01656453937227,100.11527272614));
#245447=CARTESIAN_POINT('Ctrl Pts',(0.579208469572439,8.30114247401078,
100.327211880573));
#245448=CARTESIAN_POINT('Ctrl Pts',(-4.33005325803172,6.55321167307216,
100.539151035006));
#245449=CARTESIAN_POINT('Ctrl Pts',(-6.94913167145573,3.69707168672269,
100.69810540083));
#245450=CARTESIAN_POINT('Ctrl Pts',(-7.85414848838492,-0.0790124110920571,
100.857059766655));
#245451=CARTESIAN_POINT('Ctrl Pts',(-6.55994553863086,-5.11229200624264,
101.068998921088));
#245452=CARTESIAN_POINT('Ctrl Pts',(-0.569530316075434,-8.9065370884232,
101.33392286413));
#245453=CARTESIAN_POINT('Ctrl Pts',(7.20233366355529,-5.28167553716792,
101.651831595779));
#245454=CARTESIAN_POINT('Ctrl Pts',(8.12708469795813,1.76532760006358,101.91675553882));
#245455=CARTESIAN_POINT('Ctrl Pts',(5.09914544938941,5.96391529847259,102.128694693253));
#245456=CARTESIAN_POINT('Ctrl Pts',(0.456608472163056,8.31086222799173,
102.340633847686));
#245457=CARTESIAN_POINT('Ctrl Pts',(-4.95831198844199,6.68278318145386,
102.55257300212));
#245458=CARTESIAN_POINT('Ctrl Pts',(-7.5510269451248,2.16239138998465,102.764512156552));
#245459=CARTESIAN_POINT('Ctrl Pts',(-7.68328151025241,-1.71054239298817,
102.923466522377));
#245460=CARTESIAN_POINT('Ctrl Pts',(-5.91516802671592,-5.1676569791757,
103.082420888202));
#245461=CARTESIAN_POINT('Ctrl Pts',(-1.65880897520462,-8.14964832435577,
103.294360042635));
#245462=CARTESIAN_POINT('Ctrl Pts',(5.35935853689139,-7.13638870588163,
103.559283985677));
#245463=CARTESIAN_POINT('Ctrl Pts',(8.90611535184792,0.671428343666077,
103.877192717326));
#245464=CARTESIAN_POINT('Ctrl Pts',(5.02588096619366,6.62619104289825,104.142116660367));
#245465=CARTESIAN_POINT('Ctrl Pts',(-0.00473450560939821,7.84662650989841,
104.3540558148));
#245466=CARTESIAN_POINT('Ctrl Pts',(-5.05776822281027,6.61043893201059,
104.565994969233));
#245467=CARTESIAN_POINT('Ctrl Pts',(-8.11255711291596,1.85225967799525,
104.777934123666));
#245468=CARTESIAN_POINT('Ctrl Pts',(-7.14250408114055,-3.26780964873582,
104.989873278099));
#245469=CARTESIAN_POINT('Ctrl Pts',(-4.72436496945928,-6.29596264913808,
105.148827643924));
#245470=CARTESIAN_POINT('Ctrl Pts',(-1.13298728142614,-7.77240189766538,
105.307782009749));
#245471=CARTESIAN_POINT('Ctrl Pts',(4.03965509058027,-7.26977315849979,
105.519721164181));
#245472=CARTESIAN_POINT('Ctrl Pts',(8.71220396331585,-1.93604488325272,
105.784645107223));
#245473=CARTESIAN_POINT('Ctrl Pts',(6.32906011717109,6.30180170382518,106.102553838872));
#245474=CARTESIAN_POINT('Ctrl Pts',(-0.49107598238367,8.30209200158962,
106.367477781914));
#245475=CARTESIAN_POINT('Ctrl Pts',(-5.10633876063979,5.9577575028673,106.579416936347));
#245476=CARTESIAN_POINT('Ctrl Pts',(-8.14106468800239,1.73262460310113,
106.79135609078));
#245477=CARTESIAN_POINT('Ctrl Pts',(-7.36739911305641,-3.8685758534616,
107.003295245213));
#245478=CARTESIAN_POINT('Ctrl Pts',(-3.30084634464836,-7.12729667254717,
107.215234399646));
#245479=CARTESIAN_POINT('Ctrl Pts',(0.505377312957478,-7.85514887290774,
107.37418876547));
#245480=CARTESIAN_POINT('Ctrl Pts',(4.1937781223789,-6.64124359581554,107.533143131295));
#245481=CARTESIAN_POINT('Ctrl Pts',(7.7964078732041,-2.89558962933918,107.745082285728));
#245482=CARTESIAN_POINT('Ctrl Pts',(7.87741842683513,4.19488338538094,108.01000622877));
#245483=CARTESIAN_POINT('Ctrl Pts',(0.70986213373019,8.90313441615905,108.327914960419));
#245484=CARTESIAN_POINT('Ctrl Pts',(-5.77199105250775,5.98748749586195,
108.59283890346));
#245485=CARTESIAN_POINT('Ctrl Pts',(-7.75351674291794,1.20521704214434,
108.804778057893));
#245486=CARTESIAN_POINT('Ctrl Pts',(-7.31125550254137,-3.97799764279321,
109.016717212326));
#245487=CARTESIAN_POINT('Ctrl Pts',(-3.08100760077888,-7.72993149963135,
109.228656366759));
#245488=CARTESIAN_POINT('Ctrl Pts',(2.12740491224856,-7.56095845702261,
109.440595521192));
#245489=CARTESIAN_POINT('Ctrl Pts',(5.49220360160253,-5.63865849671179,
109.599549887017));
#245490=CARTESIAN_POINT('Ctrl Pts',(7.50475105957328,-2.3178876099886,109.758504252842));
#245491=CARTESIAN_POINT('Ctrl Pts',(7.80571865989455,2.87039565730397,109.970443407275));
#245492=CARTESIAN_POINT('Ctrl Pts',(3.2562521477919,8.30948792877077,110.235367350316));
#245493=CARTESIAN_POINT('Ctrl Pts',(-5.25054005740826,7.22506302994313,
110.553276081966));
#245494=CARTESIAN_POINT('Ctrl Pts',(-8.27852566151433,0.794921439503049,
110.818200025007));
#245495=CARTESIAN_POINT('Ctrl Pts',(-6.67386889320644,-4.12662622461439,
111.03013917944));
#245496=CARTESIAN_POINT('Ctrl Pts',(-2.96719894074821,-7.77654503719568,
111.242078333873));
#245497=CARTESIAN_POINT('Ctrl Pts',(2.6863091607575,-7.87579785913017,111.454017488306));
#245498=CARTESIAN_POINT('Ctrl Pts',(6.53309210628831,-4.36034998368643,
111.665956642739));
#245499=CARTESIAN_POINT('Ctrl Pts',(7.83913280410349,-0.711875637752233,
111.824911008564));
#245500=CARTESIAN_POINT('Ctrl Pts',(7.20847053503805,3.11959035518978,111.983865374389));
#245501=CARTESIAN_POINT('Ctrl Pts',(4.06311210333432,7.25668898759164,112.195804528821));
#245502=CARTESIAN_POINT('Ctrl Pts',(-2.93007288723742,8.4300320618526,112.460728471863));
#245503=CARTESIAN_POINT('Ctrl Pts',(-8.68720379970417,2.07417376887848,
112.778637203512));
#245504=CARTESIAN_POINT('Ctrl Pts',(-6.80588226535307,-4.77973365507787,
113.043561146554));
#245505=CARTESIAN_POINT('Ctrl Pts',(-2.38634159792211,-7.47495443326655,
113.255500300987));
#245506=CARTESIAN_POINT('Ctrl Pts',(2.80307929924439,-7.83719775887135,
113.46743945542));
#245507=CARTESIAN_POINT('Ctrl Pts',(7.16241746747704,-4.23606242241895,
113.679378609853));
#245508=CARTESIAN_POINT('Ctrl Pts',(7.79856599689762,0.936115826975124,
113.891317764286));
#245509=CARTESIAN_POINT('Ctrl Pts',(6.4180837325631,4.55707924506528,114.05027213011));
#245510=CARTESIAN_POINT('Ctrl Pts',(3.44734752807005,7.05759778249045,114.209226495935));
#245511=CARTESIAN_POINT('Ctrl Pts',(-1.63248064607929,8.15496302671398,
114.421165650368));
#245512=CARTESIAN_POINT('Ctrl Pts',(-7.70802135098465,4.4985747233042,114.686089593409));
#245513=CARTESIAN_POINT('Ctrl Pts',(-7.94825322375326,-4.07369333310623,
115.003998325059));
#245514=CARTESIAN_POINT('Ctrl Pts',(-2.06190552756128,-8.05694934939675,
115.2689222681));
#245515=CARTESIAN_POINT('Ctrl Pts',(3.0482109513173,-7.23035130527238,115.480861422533));
#245516=CARTESIAN_POINT('Ctrl Pts',(7.22602204130568,-4.13080231045666,
115.692800576966));
#245517=CARTESIAN_POINT('Ctrl Pts',(8.19581928082761,1.43978996421828,115.904739731399));
#245518=CARTESIAN_POINT('Ctrl Pts',(5.31556056214004,5.78262573228654,116.116678885832));
#245519=CARTESIAN_POINT('Ctrl Pts',(1.91210158620413,7.63561638428962,116.275633251657));
#245520=CARTESIAN_POINT('Ctrl Pts',(-1.9707866449849,7.6032816230003,116.434587617482));
#245521=CARTESIAN_POINT('Ctrl Pts',(-6.54340093733515,5.13345100299747,
116.646526771915));
#245522=CARTESIAN_POINT('Ctrl Pts',(-8.78101191796645,-1.59517942091727,
116.911450714956));
#245523=CARTESIAN_POINT('Ctrl Pts',(-3.38887426470333,-8.26348824039407,
117.229359446606));
#245524=CARTESIAN_POINT('Ctrl Pts',(3.67315216588268,-7.46149049383586,
117.494283389647));
#245525=CARTESIAN_POINT('Ctrl Pts',(7.01760237543226,-3.5103884260452,117.70622254408));
#245526=CARTESIAN_POINT('Ctrl Pts',(8.17568594758414,1.56111548451284,117.918161698513));
#245527=CARTESIAN_POINT('Ctrl Pts',(5.2897969563499,6.4235891046705,118.130100852946));
#245528=CARTESIAN_POINT('Ctrl Pts',(0.277563751038976,7.84964348321566,
118.342040007379));
#245529=CARTESIAN_POINT('Ctrl Pts',(-3.51295635777461,7.04399798923642,
118.500994373204));
#245530=CARTESIAN_POINT('Ctrl Pts',(-6.44163730509991,4.49435204097877,
118.659948739028));
#245531=CARTESIAN_POINT('Ctrl Pts',(-8.30915285520757,-0.355519135476897,
118.871887893461));
#245532=CARTESIAN_POINT('Ctrl Pts',(-5.63329810886282,-6.92219041236727,
119.136811836503));
#245533=CARTESIAN_POINT('Ctrl Pts',(2.7994099472563,-8.48133306905832,119.454720568152));
#245534=CARTESIAN_POINT('Ctrl Pts',(7.64266283975747,-3.27957191430878,
119.719644511194));
#245535=CARTESIAN_POINT('Ctrl Pts',(7.61389451072705,1.89688702375895,119.931583665626));
#245536=CARTESIAN_POINT('Ctrl Pts',(5.19560305715608,6.50266338833404,120.14352282006));
#245537=CARTESIAN_POINT('Ctrl Pts',(-0.158833141679201,8.31980894360886,
120.355461974492));
#245538=CARTESIAN_POINT('Ctrl Pts',(-4.89384758558535,6.14363086932643,
120.567401128926));
#245539=CARTESIAN_POINT('Ctrl Pts',(-7.24946742233022,3.06659291993062,
120.72635549475));
#245540=CARTESIAN_POINT('Ctrl Pts',(-7.8162335680239,-0.77484466107856,
120.885309860575));
#245541=CARTESIAN_POINT('Ctrl Pts',(-6.0810054201158,-5.67360450749057,
121.097249015008));
#245542=CARTESIAN_POINT('Ctrl Pts',(0.222131644826142,-8.92196308111358,
121.362172958049));
#245543=CARTESIAN_POINT('Ctrl Pts',(7.64212238170054,-4.62251794850072,
121.680081689699));
#245544=CARTESIAN_POINT('Ctrl Pts',(7.93863101146212,2.47871436175757,121.94500563274));
#245545=CARTESIAN_POINT('Ctrl Pts',(4.55047200485095,6.39239974770443,122.156944787173));
#245546=CARTESIAN_POINT('Ctrl Pts',(-0.281812118503283,8.31862393664814,
122.368883941606));
#245547=CARTESIAN_POINT('Ctrl Pts',(-5.53111808240576,6.21700744599316,
122.580823096039));
#245548=CARTESIAN_POINT('Ctrl Pts',(-7.71296921877461,1.48460441859632,
122.792762250472));
#245549=CARTESIAN_POINT('Ctrl Pts',(-7.50143033234909,-2.38480880007381,
122.951716616297));
#245550=CARTESIAN_POINT('Ctrl Pts',(-5.43385836418954,-5.67160248224722,
123.110670982122));
#245551=CARTESIAN_POINT('Ctrl Pts',(-0.929945861972466,-8.26460015491946,
123.322610136555));
#245552=CARTESIAN_POINT('Ctrl Pts',(5.97079101554063,-6.63328141549309,
123.587534079596));
#245553=CARTESIAN_POINT('Ctrl Pts',(8.81155209197163,1.458168855644,123.905442811246));
#245554=CARTESIAN_POINT('Ctrl Pts',(4.41879583803649,7.04557524727988,124.170366754287));
#245555=CARTESIAN_POINT('Ctrl Pts',(-0.700192391089372,7.8153247288161,
124.38230590872));
#245556=CARTESIAN_POINT('Ctrl Pts',(-5.62377073711546,6.13613273698301,
124.594245063153));
#245557=CARTESIAN_POINT('Ctrl Pts',(-8.24480119988584,1.12592273243385,
124.806184217586));
#245558=CARTESIAN_POINT('Ctrl Pts',(-6.82475470000086,-3.88801591229979,
125.018123372019));
#245559=CARTESIAN_POINT('Ctrl Pts',(-4.14773593015482,-6.68992202478464,
125.177077737843));
#245560=CARTESIAN_POINT('Ctrl Pts',(-0.439630450095629,-7.84223287757092,
125.336032103669));
#245561=CARTESIAN_POINT('Ctrl Pts',(4.66810392984963,-6.88311126795273,
125.547971258101));
#245562=CARTESIAN_POINT('Ctrl Pts',(8.84951420994463,-1.15622918851469,
125.812895201143));
#245563=CARTESIAN_POINT('Ctrl Pts',(5.74559790547405,6.83796836711839,126.130803932792));
#245564=CARTESIAN_POINT('Ctrl Pts',(-1.22498941140125,8.22589132953309,
126.395727875834));
#245565=CARTESIAN_POINT('Ctrl Pts',(-5.61430046336432,5.48171508822294,
126.607667030266));
#245566=CARTESIAN_POINT('Ctrl Pts',(-8.26259286280484,1.00423177256909,
126.8196061847));
#245567=CARTESIAN_POINT('Ctrl Pts',(-6.99551640097889,-4.50635097486713,
127.031545339132));
#245568=CARTESIAN_POINT('Ctrl Pts',(-2.65613556532327,-7.39181224789329,
127.243484493566));
#245569=CARTESIAN_POINT('Ctrl Pts',(1.19962017695458,-7.77943966330736,
127.40243885939));
#245570=CARTESIAN_POINT('Ctrl Pts',(4.76591139705247,-6.24339490935429,
127.561393225215));
#245571=CARTESIAN_POINT('Ctrl Pts',(8.02237055991287,-2.19316794303078,
127.773332379648));
#245572=CARTESIAN_POINT('Ctrl Pts',(7.47460653571026,4.87657921341394,128.038256322689));
#245573=CARTESIAN_POINT('Ctrl Pts',(-0.0820505423925757,8.93101194655986,
128.356165054339));
#245574=CARTESIAN_POINT('Ctrl Pts',(-6.27996801558465,5.45232876361717,
128.62108899738));
#245575=CARTESIAN_POINT('Ctrl Pts',(-7.82982404950507,0.513249798023501,
128.833028151813));
#245576=CARTESIAN_POINT('Ctrl Pts',(-6.92989528442777,-4.61036588747517,
129.044967306246));
#245577=CARTESIAN_POINT('Ctrl Pts',(-2.38374821605209,-7.9725901228827,
129.256906460679));
#245578=CARTESIAN_POINT('Ctrl Pts',(2.78918870410998,-7.34264058921324,
129.468845615112));
#245579=CARTESIAN_POINT('Ctrl Pts',(5.97036368203372,-5.12967129046876,
129.627799980937));
#245580=CARTESIAN_POINT('Ctrl Pts',(7.68065768697234,-1.64359025738219,
129.786754346762));
#245581=CARTESIAN_POINT('Ctrl Pts',(7.52058337237721,3.55094927679636,129.998693501194));
#245582=CARTESIAN_POINT('Ctrl Pts',(2.50693474615304,8.56539817324321,130.263617444236));
#245583=CARTESIAN_POINT('Ctrl Pts',(-5.87026035982546,6.73125174012964,
130.581526175885));
#245584=CARTESIAN_POINT('Ctrl Pts',(-8.316400610289,0.0580354563857965,
130.846450118927));
#245585=CARTESIAN_POINT('Ctrl Pts',(-6.28184373203611,-4.70191549528422,
131.05838927336));
#245586=CARTESIAN_POINT('Ctrl Pts',(-2.26625593954398,-8.00893290599279,
131.270328427793));
#245587=CARTESIAN_POINT('Ctrl Pts',(3.37379868175747,-7.60670304895033,
131.482267582226));
#245588=CARTESIAN_POINT('Ctrl Pts',(6.89385416487644,-3.76413591636517,
131.694206736659));
#245589=CARTESIAN_POINT('Ctrl Pts',(7.87137641587059,-0.014261567811148,
131.853161102484));
#245590=CARTESIAN_POINT('Ctrl Pts',(6.90359876781664,3.74622682481395,132.012115468308));
#245591=CARTESIAN_POINT('Ctrl Pts',(3.40393272898892,7.58825784698442,132.224054622741));
#245592=CARTESIAN_POINT('Ctrl Pts',(-3.66572693323746,8.13715021530282,
132.488978565783));
#245593=CARTESIAN_POINT('Ctrl Pts',(-8.8368553055286,1.29603032112415,132.806887297432));
#245594=CARTESIAN_POINT('Ctrl Pts',(-6.35545017030808,-5.36415336635995,
133.071811240473));
#245595=CARTESIAN_POINT('Ctrl Pts',(-1.7144157604137,-7.65704561752096,
133.283750394906));
#245596=CARTESIAN_POINT('Ctrl Pts',(3.48668782092298,-7.5579052215536,133.49568954934));
#245597=CARTESIAN_POINT('Ctrl Pts',(7.50968689854422,-3.58455772342483,
133.707628703772));
#245598=CARTESIAN_POINT('Ctrl Pts',(7.68490110483432,1.62364792299449,133.919567858206));
#245599=CARTESIAN_POINT('Ctrl Pts',(5.98891335360918,5.10800387105895,134.07852222403));
#245600=CARTESIAN_POINT('Ctrl Pts',(2.8082364167446,7.3353713277473,134.237476589855));
#245601=CARTESIAN_POINT('Ctrl Pts',(-2.34885814436791,7.97817717382807,
134.449415744288));
#245602=CARTESIAN_POINT('Ctrl Pts',(-8.07641696364469,3.79767233182262,
134.714339687329));
#245603=CARTESIAN_POINT('Ctrl Pts',(-7.55589297261149,-4.76213429554381,
135.032248418979));
#245604=CARTESIAN_POINT('Ctrl Pts',(-1.33969083946443,-8.20801110549739,
135.29717236202));
#245605=CARTESIAN_POINT('Ctrl Pts',(3.67709254282027,-6.93169728860364,
135.509111516453));
#245606=CARTESIAN_POINT('Ctrl Pts',(7.56364733765227,-3.47413327101668,
135.721050670886));
#245607=CARTESIAN_POINT('Ctrl Pts',(8.03607863924848,2.16066936076013,135.932989825319));
#245608=CARTESIAN_POINT('Ctrl Pts',(4.78194321339305,6.23085808992206,136.144928979752));
#245609=CARTESIAN_POINT('Ctrl Pts',(1.22813626868337,7.77534810001959,136.303883345577));
#245610=CARTESIAN_POINT('Ctrl Pts',(-2.63754744258561,7.39811979755767,
136.462837711402));
#245611=CARTESIAN_POINT('Ctrl Pts',(-6.97132874162559,4.53448847191684,
136.674776865835));
#245612=CARTESIAN_POINT('Ctrl Pts',(-8.60778941430539,-2.36969518111316,
136.939700808876));
#245613=CARTESIAN_POINT('Ctrl Pts',(-2.63835148620368,-8.52696629709462,
137.257609540525));
#245614=CARTESIAN_POINT('Ctrl Pts',(4.31203657919717,-7.11389987312211,
137.522533483567));
#245615=CARTESIAN_POINT('Ctrl Pts',(7.31188535419881,-2.86468837331265,
137.734472637999));
#245616=CARTESIAN_POINT('Ctrl Pts',(7.80951289097387,0.972884837682936,
137.893427003825));
#245617=CARTESIAN_POINT('Ctrl Pts',(6.37878947535717,4.60346102348882,138.052446139219));
#245618=CARTESIAN_POINT('Ctrl Pts',(4.39240965737021,6.26214476802734,138.158480486005));
#245619=CARTESIAN_POINT('Ctrl Pts',(3.2582502558657,6.80515705093528,138.211530044183));
#245620=CARTESIAN_POINT('Ctrl Pts',(4.1509387962231,-5.82482577975211,7.77730822088039));
#245621=CARTESIAN_POINT('Ctrl Pts',(5.12112172942826,-5.13345251569094,
7.83032558937012));
#245622=CARTESIAN_POINT('Ctrl Pts',(6.70588704626977,-3.2618553580775,7.93632774646809));
#245623=CARTESIAN_POINT('Ctrl Pts',(7.45184147994325,0.360746109526988,
8.09531469217431));
#245624=CARTESIAN_POINT('Ctrl Pts',(6.36331483166936,3.86396831410664,8.25426905799906));
#245625=CARTESIAN_POINT('Ctrl Pts',(2.87092622161512,7.34492483342846,8.46620821243209));
#245626=CARTESIAN_POINT('Ctrl Pts',(-3.85008224481605,7.53493083349062,
8.73113215547334));
#245627=CARTESIAN_POINT('Ctrl Pts',(-8.42443337233034,0.814053692892807,
9.04904088712287));
#245628=CARTESIAN_POINT('Ctrl Pts',(-5.77383888534872,-5.36812601492259,
9.31396483016413));
#245629=CARTESIAN_POINT('Ctrl Pts',(-1.26083679095937,-7.33819775399668,
9.52590398459714));
#245630=CARTESIAN_POINT('Ctrl Pts',(2.41084003202958,-7.06217496130019,
9.6848583504219));
#245631=CARTESIAN_POINT('Ctrl Pts',(5.47887921888675,-5.04205337644938,
9.84381271624667));
#245632=CARTESIAN_POINT('Ctrl Pts',(7.85650772812585,-0.711760681333348,
10.0557518706797));
#245633=CARTESIAN_POINT('Ctrl Pts',(6.49938797236703,4.47408222088017,10.2676910251127));
#245634=CARTESIAN_POINT('Ctrl Pts',(2.30753480030124,7.07155140166136,10.4796301795457));
#245635=CARTESIAN_POINT('Ctrl Pts',(-2.58535248711871,7.44812896050389,
10.6915693339788));
#245636=CARTESIAN_POINT('Ctrl Pts',(-7.83088474550556,3.21945327438235,
10.95649327702));
#245637=CARTESIAN_POINT('Ctrl Pts',(-6.92570130420384,-4.85959861095894,
11.2744020086696));
#245638=CARTESIAN_POINT('Ctrl Pts',(-0.896931309614421,-7.83301913464394,
11.5393259517108));
#245639=CARTESIAN_POINT('Ctrl Pts',(3.81506237611427,-6.39442540470123,
11.7512651061438));
#245640=CARTESIAN_POINT('Ctrl Pts',(6.42361997314908,-3.79717862977323,
11.9102194719686));
#245641=CARTESIAN_POINT('Ctrl Pts',(7.44123640529532,-0.267289742976332,
12.0691738377934));
#245642=CARTESIAN_POINT('Ctrl Pts',(6.4310429295426,4.56844247750195,12.2811129922264));
#245643=CARTESIAN_POINT('Ctrl Pts',(2.02792095266024,7.62545053401183,12.4930521466594));
#245644=CARTESIAN_POINT('Ctrl Pts',(-2.8457724144279,6.87264535529731,12.7049913010924));
#245645=CARTESIAN_POINT('Ctrl Pts',(-6.8075826492275,3.97683224675571,12.9169304555254));
#245646=CARTESIAN_POINT('Ctrl Pts',(-8.0425356587629,-2.64678923841271,
13.1818543985667));
#245647=CARTESIAN_POINT('Ctrl Pts',(-2.1009832043633,-8.1955386757095,13.4997631302162));
#245648=CARTESIAN_POINT('Ctrl Pts',(4.4125185540474,-6.53378352923089,13.7646870732574));
#245649=CARTESIAN_POINT('Ctrl Pts',(7.05654596471932,-2.37667006032655,
13.9766262276905));
#245650=CARTESIAN_POINT('Ctrl Pts',(7.34916631688393,1.29274846990858,14.1355805935152));
#245651=CARTESIAN_POINT('Ctrl Pts',(5.82669598721959,4.6360611618861,14.29453495934));
#245652=CARTESIAN_POINT('Ctrl Pts',(1.91455626914196,7.65267612129344,14.506474113773));
#245653=CARTESIAN_POINT('Ctrl Pts',(-3.41836086554637,7.11159386572605,
14.718413268206));
#245654=CARTESIAN_POINT('Ctrl Pts',(-6.63119636648613,3.37029827631453,
14.930352422639));
#245655=CARTESIAN_POINT('Ctrl Pts',(-7.75768227212046,-1.40596626166421,
15.1422915770721));
#245656=CARTESIAN_POINT('Ctrl Pts',(-4.38842815241116,-7.24082673477043,
15.4072155201133));
#245657=CARTESIAN_POINT('Ctrl Pts',(3.73359216516395,-7.5921850777709,15.7251242517628));
#245658=CARTESIAN_POINT('Ctrl Pts',(7.60103891632166,-2.09400440680762,
15.9900481948041));
#245659=CARTESIAN_POINT('Ctrl Pts',(6.90621000003866,2.78346277591659,16.2019873492371));
#245660=CARTESIAN_POINT('Ctrl Pts',(4.74224381427298,5.76129913647346,16.3609417150619));
#245661=CARTESIAN_POINT('Ctrl Pts',(1.41148008495701,7.31103092589749,16.5198960808866));
#245662=CARTESIAN_POINT('Ctrl Pts',(-3.52218573576049,7.05855404261346,
16.7318352353197));
#245663=CARTESIAN_POINT('Ctrl Pts',(-7.22156448448482,3.17945981395448,
16.9437743897527));
#245664=CARTESIAN_POINT('Ctrl Pts',(-7.22925189979947,-1.75202531204523,
17.1557135441857));
#245665=CARTESIAN_POINT('Ctrl Pts',(-4.97895389573663,-6.11296928396743,
17.3676526986187));
#245666=CARTESIAN_POINT('Ctrl Pts',(1.37503284600016,-8.35446935024785,
17.6325766416599));
#245667=CARTESIAN_POINT('Ctrl Pts',(7.77356924943103,-3.33955174175305,
17.9504853733095));
#245668=CARTESIAN_POINT('Ctrl Pts',(7.13602384913055,3.35228439835905,18.2154093163507));
#245669=CARTESIAN_POINT('Ctrl Pts',(3.4363168962553,6.60568904643142,18.4273484707838));
#245670=CARTESIAN_POINT('Ctrl Pts',(-0.144098120754572,7.46060854525456,
18.5863028366085));
#245671=CARTESIAN_POINT('Ctrl Pts',(-3.68218156311378,6.47186125978534,
18.7452572024333));
#245672=CARTESIAN_POINT('Ctrl Pts',(-7.26594464328095,3.07164873813643,
18.9571963568663));
#245673=CARTESIAN_POINT('Ctrl Pts',(-7.5536318490491,-2.28092178759782,
19.1691355112993));
#245674=CARTESIAN_POINT('Ctrl Pts',(-4.35247612487143,-6.03221578752203,
19.3810746657323));
#245675=CARTESIAN_POINT('Ctrl Pts',(0.192971607746215,-7.88169634794461,
19.5930138201653));
#245676=CARTESIAN_POINT('Ctrl Pts',(6.47756692573537,-5.4524306666318,19.8579377632066));
#245677=CARTESIAN_POINT('Ctrl Pts',(8.07708201093883,2.51827935307344,20.1758464948561));
#245678=CARTESIAN_POINT('Ctrl Pts',(3.24098871487961,7.18725533238272,20.4407704378974));
#245679=CARTESIAN_POINT('Ctrl Pts',(-1.68528536100722,7.25280737656864,
20.6527095923304));
#245680=CARTESIAN_POINT('Ctrl Pts',(-4.96117747254263,5.57388214980061,
20.8116639581552));
#245681=CARTESIAN_POINT('Ctrl Pts',(-7.00595609770081,2.52190967061355,
20.9706183239799));
#245682=CARTESIAN_POINT('Ctrl Pts',(-7.51723541172976,-2.39168335996942,
21.182557478413));
#245683=CARTESIAN_POINT('Ctrl Pts',(-4.25495058253814,-6.64494949960238,
21.3944966328459));
#245684=CARTESIAN_POINT('Ctrl Pts',(0.616372317611963,-7.4129454935867,
21.606435787279));
#245685=CARTESIAN_POINT('Ctrl Pts',(5.27214286867867,-5.86198643250225,
21.818374941712));
#245686=CARTESIAN_POINT('Ctrl Pts',(8.46657658194745,0.0703877391787107,
22.0832988847532));
#245687=CARTESIAN_POINT('Ctrl Pts',(4.4982432043068,7.16566764415259,22.4012076164028));
#245688=CARTESIAN_POINT('Ctrl Pts',(-2.21186861338831,7.56758113930394,
22.666131559444));
#245689=CARTESIAN_POINT('Ctrl Pts',(-5.99683390639607,4.41377216094488,
22.8780707138771));
#245690=CARTESIAN_POINT('Ctrl Pts',(-7.3936041596357,1.00799884154107,23.0370250797018));
#245691=CARTESIAN_POINT('Ctrl Pts',(-6.96222927407579,-2.6402296803209,
23.1959794455266));
#245692=CARTESIAN_POINT('Ctrl Pts',(-4.15527195677464,-6.70542261866923,
23.4079185999596));
#245693=CARTESIAN_POINT('Ctrl Pts',(1.08892646681892,-7.8149982381296,23.6198577543926));
#245694=CARTESIAN_POINT('Ctrl Pts',(5.28895361428727,-5.23054924369547,
23.8317969088256));
#245695=CARTESIAN_POINT('Ctrl Pts',(7.81719201645802,-1.02463863894781,
24.0437360632586));
#245696=CARTESIAN_POINT('Ctrl Pts',(6.38601918099923,5.55937338840611,24.3086600063));
#245697=CARTESIAN_POINT('Ctrl Pts',(-1.24273305920179,8.36878720335955,
24.6265687379494));
#245698=CARTESIAN_POINT('Ctrl Pts',(-6.60156333316999,4.31045341245984,
24.8914926809907));
#245699=CARTESIAN_POINT('Ctrl Pts',(-7.42592843078579,-0.546798436794452,
25.1034318354237));
#245700=CARTESIAN_POINT('Ctrl Pts',(-6.27220154742346,-4.04239185166769,
25.2623862012485));
#245701=CARTESIAN_POINT('Ctrl Pts',(-3.57201894274956,-6.53330926118485,
25.4213405670732));
#245702=CARTESIAN_POINT('Ctrl Pts',(1.20397548955058,-7.79611573479253,
25.6332797215063));
#245703=CARTESIAN_POINT('Ctrl Pts',(5.90939724515907,-5.22866928682757,
25.8452188759392));
#245704=CARTESIAN_POINT('Ctrl Pts',(7.41933250043391,-0.534023382269806,
26.0571580303723));
#245705=CARTESIAN_POINT('Ctrl Pts',(6.60480900712377,4.30521466851727,26.2690971848052));
#245706=CARTESIAN_POINT('Ctrl Pts',(1.2359409372583,8.37617594439235,26.5340211278465));
#245707=CARTESIAN_POINT('Ctrl Pts',(-6.38637396884901,5.54934340634596,
26.8519298594961));
#245708=CARTESIAN_POINT('Ctrl Pts',(-7.81813318879946,-1.01854823402413,
27.1168538025373));
#245709=CARTESIAN_POINT('Ctrl Pts',(-5.28565658634204,-5.24454345399983,
27.3287929569704));
#245710=CARTESIAN_POINT('Ctrl Pts',(-2.13598597672581,-7.14975580290411,
27.4877473227951));
#245711=CARTESIAN_POINT('Ctrl Pts',(1.53512744605716,-7.28607116037218,
27.6467016886199));
#245712=CARTESIAN_POINT('Ctrl Pts',(5.98451689778819,-5.13950727500275,
27.8586408430529));
#245713=CARTESIAN_POINT('Ctrl Pts',(7.88944153898006,-0.129114349023541,
28.0705799974859));
#245714=CARTESIAN_POINT('Ctrl Pts',(5.98351543504755,4.41918756824753,28.2825191519189));
#245715=CARTESIAN_POINT('Ctrl Pts',(2.21774105942401,7.56571212483959,28.4944583063519));
#245716=CARTESIAN_POINT('Ctrl Pts',(-4.50820794107503,7.1668636523821,28.7593822493932));
#245717=CARTESIAN_POINT('Ctrl Pts',(-8.46032350243878,0.0625375537539325,
29.0772909810427));
#245718=CARTESIAN_POINT('Ctrl Pts',(-5.27681850093237,-5.8579717967108,
29.342214924084));
#245719=CARTESIAN_POINT('Ctrl Pts',(-0.60476708952805,-7.42143236559205,
29.554154078517));
#245720=CARTESIAN_POINT('Ctrl Pts',(3.02691825394032,-6.8204992499005,29.7131084443417));
#245721=CARTESIAN_POINT('Ctrl Pts',(5.90439542290494,-4.53669085563746,
29.8720628101665));
#245722=CARTESIAN_POINT('Ctrl Pts',(7.88852461090912,-0.0125296767604765,
30.0840019645995));
#245723=CARTESIAN_POINT('Ctrl Pts',(6.07732602940615,5.03250103272817,30.2959411190325));
#245724=CARTESIAN_POINT('Ctrl Pts',(1.67164604026992,7.24826015267495,30.5078802734656));
#245725=CARTESIAN_POINT('Ctrl Pts',(-3.23531216218057,7.18965441282447,
30.7198194278986));
#245726=CARTESIAN_POINT('Ctrl Pts',(-8.08542968584339,2.51270775202584,
30.9847433709398));
#245727=CARTESIAN_POINT('Ctrl Pts',(-6.46771160057704,-5.45432776456534,
31.3026521025894));
#245728=CARTESIAN_POINT('Ctrl Pts',(-0.199134298166419,-7.8816871667261,
31.5675760456306));
#245729=CARTESIAN_POINT('Ctrl Pts',(4.3668113535178,-6.0311159989194,31.7795152000637));
#245730=CARTESIAN_POINT('Ctrl Pts',(6.73489596363007,-3.21288351687546,
31.9384695658883));
#245731=CARTESIAN_POINT('Ctrl Pts',(7.43564110432626,0.393307255589283,
32.0974239317132));
#245732=CARTESIAN_POINT('Ctrl Pts',(6.000813253703,5.12047046899997,32.3093630861461));
#245733=CARTESIAN_POINT('Ctrl Pts',(1.34406694243543,7.77518117900539,32.5213022405792));
#245734=CARTESIAN_POINT('Ctrl Pts',(-3.44372115445915,6.5933648719858,32.7332413950122));
#245735=CARTESIAN_POINT('Ctrl Pts',(-7.13327169657829,3.35779842536662,
32.9451805494452));
#245736=CARTESIAN_POINT('Ctrl Pts',(-7.77628744700907,-3.34921289160561,
33.2101044924865));
#245737=CARTESIAN_POINT('Ctrl Pts',(-1.36631236180715,-8.34950149658773,
33.528013224136));
#245738=CARTESIAN_POINT('Ctrl Pts',(4.97426632220056,-6.11696997039077,
33.7929371671773));
#245739=CARTESIAN_POINT('Ctrl Pts',(7.23942672015315,-1.74186749012833,
34.0048763216103));
#245740=CARTESIAN_POINT('Ctrl Pts',(7.20566079492565,1.93904529147781,34.163830687435));
#245741=CARTESIAN_POINT('Ctrl Pts',(5.39285189760239,5.13425726275685,34.3227850532598));
#245742=CARTESIAN_POINT('Ctrl Pts',(1.22873515191321,7.79225175775088,34.5347242076927));
#245743=CARTESIAN_POINT('Ctrl Pts',(-4.03523491029923,6.78062220823502,
34.7466633621258));
#245744=CARTESIAN_POINT('Ctrl Pts',(-6.90382024541709,2.76928542114653,
34.9586025165588));
#245745=CARTESIAN_POINT('Ctrl Pts',(-7.60253402081132,-2.08802582000469,
35.1705416709919));
#245746=CARTESIAN_POINT('Ctrl Pts',(-3.72937434942724,-7.60129202265261,
35.4354656140331));
#245747=CARTESIAN_POINT('Ctrl Pts',(4.39182218474434,-7.23138179113334,
35.7533743456827));
#245748=CARTESIAN_POINT('Ctrl Pts',(7.75672295683287,-1.4120538352991,36.0182982887239));
#245749=CARTESIAN_POINT('Ctrl Pts',(6.63232012267388,3.38463164613355,36.2302374431569));
#245750=CARTESIAN_POINT('Ctrl Pts',(4.21293368089045,6.15894746968582,36.3891918089817));
#245751=CARTESIAN_POINT('Ctrl Pts',(0.75792025713238,7.40736161622165,36.5481461748064));
#245752=CARTESIAN_POINT('Ctrl Pts',(-4.13395003265704,6.71858873999691,
36.7600853292395));
#245753=CARTESIAN_POINT('Ctrl Pts',(-7.47495009539872,2.52687146159157,
36.9720244836724));
#245754=CARTESIAN_POINT('Ctrl Pts',(-7.0455108666269,-2.38588607293978,
37.1839636381055));
#245755=CARTESIAN_POINT('Ctrl Pts',(-4.41754226695533,-6.53021406098323,
37.3959027925385));
#245756=CARTESIAN_POINT('Ctrl Pts',(2.1101096709297,-8.19971405772523,37.6608267355797));
#245757=CARTESIAN_POINT('Ctrl Pts',(8.03897188270305,-2.63740701839083,
37.9787354672293));
#245758=CARTESIAN_POINT('Ctrl Pts',(6.81081265222878,3.97158382501008,38.2436594102705));
#245759=CARTESIAN_POINT('Ctrl Pts',(2.83730502138147,6.88426479773092,38.4555985647036));
#245760=CARTESIAN_POINT('Ctrl Pts',(-0.804793261092854,7.41847369347833,
38.6145529305283));
#245761=CARTESIAN_POINT('Ctrl Pts',(-4.24131533553443,6.12002397496985,
38.7735072963531));
#245762=CARTESIAN_POINT('Ctrl Pts',(-7.50959987820737,2.415551117022,38.9854464507861));
#245763=CARTESIAN_POINT('Ctrl Pts',(-7.32173602890284,-2.94145199436841,
39.1973856052191));
#245764=CARTESIAN_POINT('Ctrl Pts',(-3.80068762994222,-6.39425126691233,
39.4093247596522));
#245765=CARTESIAN_POINT('Ctrl Pts',(0.890797018126755,-7.83357236738745,
39.6212639140849));
#245766=CARTESIAN_POINT('Ctrl Pts',(6.93534280479247,-4.85683988122124,
39.8861878571265));
#245767=CARTESIAN_POINT('Ctrl Pts',(7.82208812739543,3.22427077628526,40.2040965887758));
#245768=CARTESIAN_POINT('Ctrl Pts',(2.59119915321904,7.44622951641959,40.4690205318172));
#245769=CARTESIAN_POINT('Ctrl Pts',(-2.32149660382302,7.07488905270405,
40.6809596862502));
#245770=CARTESIAN_POINT('Ctrl Pts',(-5.43568614902035,5.11221676215697,
40.839914052075));
#245771=CARTESIAN_POINT('Ctrl Pts',(-7.20190909918588,1.89101944905621,
40.9988684178997));
#245772=CARTESIAN_POINT('Ctrl Pts',(-7.27566561605945,-3.04855168449034,
41.2108075723328));
#245773=CARTESIAN_POINT('Ctrl Pts',(-3.64923698859839,-6.99592936736449,
41.4227467267657));
#245774=CARTESIAN_POINT('Ctrl Pts',(1.27098415924342,-7.32913876193906,
41.6346858811988));
#245775=CARTESIAN_POINT('Ctrl Pts',(5.77096345619118,-5.3716250939456,41.8466250356318));
#245776=CARTESIAN_POINT('Ctrl Pts',(8.42701575227761,0.820535777813988,
42.111548978673));
#245777=CARTESIAN_POINT('Ctrl Pts',(3.84541883736212,7.53616206545534,42.4294577103226));
#245778=CARTESIAN_POINT('Ctrl Pts',(-2.87390697323184,7.34175086556677,
42.6943816533638));
#245779=CARTESIAN_POINT('Ctrl Pts',(-6.36444154116952,3.86487845328535,
42.9063208077969));
#245780=CARTESIAN_POINT('Ctrl Pts',(-7.45384777880487,0.348708222352379,
43.0652751736216));
#245781=CARTESIAN_POINT('Ctrl Pts',(-6.70081421748781,-3.24692747876492,
43.2242295394464));
#245782=CARTESIAN_POINT('Ctrl Pts',(-3.54459070639618,-7.04732958317178,
43.4361686938793));
#245783=CARTESIAN_POINT('Ctrl Pts',(1.77731393901028,-7.68772485682904,
43.6481078483124));
#245784=CARTESIAN_POINT('Ctrl Pts',(5.73174134622043,-4.74118306594809,
43.8600470027454));
#245785=CARTESIAN_POINT('Ctrl Pts',(7.8772433602972,-0.327738318255859,
44.0719861571785));
#245786=CARTESIAN_POINT('Ctrl Pts',(5.86813705545796,6.10351054313575,44.3369101002196));
#245787=CARTESIAN_POINT('Ctrl Pts',(-1.97959962545018,8.22570179586308,
44.6548188318693));
#245788=CARTESIAN_POINT('Ctrl Pts',(-6.95763338494124,3.7083668566624,44.9197427749104));
#245789=CARTESIAN_POINT('Ctrl Pts',(-7.34823720106293,-1.20283482928803,
45.1316819293436));
#245790=CARTESIAN_POINT('Ctrl Pts',(-5.8892232522119,-4.58241133242498,
45.2906362951682));
#245791=CARTESIAN_POINT('Ctrl Pts',(-2.97888827949449,-6.8241976706376,
45.4495906609931));
#245792=CARTESIAN_POINT('Ctrl Pts',(1.89023653223341,-7.65871943486173,
45.661529815426));
#245793=CARTESIAN_POINT('Ctrl Pts',(6.34957645542678,-4.68431821600511,
45.8734689698591));
#245794=CARTESIAN_POINT('Ctrl Pts',(7.43746460218952,0.125682202335439,
46.085408124292));
#245795=CARTESIAN_POINT('Ctrl Pts',(6.19722666978529,4.87368002292947,46.2973472787251));
#245796=CARTESIAN_POINT('Ctrl Pts',(0.488664105854659,8.4527558135473,46.5622712217663));
#245797=CARTESIAN_POINT('Ctrl Pts',(-6.85309850486006,4.96145397985629,
46.8801799534159));
#245798=CARTESIAN_POINT('Ctrl Pts',(-7.69708536115706,-1.70749055807123,
47.1451038964571));
#245799=CARTESIAN_POINT('Ctrl Pts',(-4.80000976375706,-5.69239034654781,
47.3570430508902));
#245800=CARTESIAN_POINT('Ctrl Pts',(-1.49386912582224,-7.31093695560598,
47.5159974167149));
#245801=CARTESIAN_POINT('Ctrl Pts',(2.17487796512775,-7.12133098981132,
47.6749517825397));
#245802=CARTESIAN_POINT('Ctrl Pts',(6.41649768782323,-4.58884897897914,
47.8868909369727));
#245803=CARTESIAN_POINT('Ctrl Pts',(7.86983478575692,0.570665188177667,
48.0988300914057));
#245804=CARTESIAN_POINT('Ctrl Pts',(5.56827648271525,4.93213673136158,48.3107692458386));
#245805=CARTESIAN_POINT('Ctrl Pts',(1.538434643456,7.73250245460126,48.5227084002718));
#245806=CARTESIAN_POINT('Ctrl Pts',(-5.12569142326057,6.73907715383353,
48.7876323433129));
#245807=CARTESIAN_POINT('Ctrl Pts',(-8.43256896027644,-0.687579407581075,
49.1055410749626));
#245808=CARTESIAN_POINT('Ctrl Pts',(-4.73683596235613,-6.30262105227425,
49.3704650180036));
#245809=CARTESIAN_POINT('Ctrl Pts',(0.0554030417511936,-7.44582648821461,
49.5824041724369));
#245810=CARTESIAN_POINT('Ctrl Pts',(3.6195320793735,-6.52536831606588,49.7413585382614));
#245811=CARTESIAN_POINT('Ctrl Pts',(6.28326162393605,-3.99550655046614,
49.9003129040864));
#245812=CARTESIAN_POINT('Ctrl Pts',(7.85858812104716,0.686709744692324,
50.1122520585192));
#245813=CARTESIAN_POINT('Ctrl Pts',(5.60735754647097,5.55135115608286,50.3241912129523));
#245814=CARTESIAN_POINT('Ctrl Pts',(1.02262588517924,7.36789739503524,50.5361303673853));
#245815=CARTESIAN_POINT('Ctrl Pts',(-3.85982544106722,6.87459983759712,
50.7480695218184));
#245816=CARTESIAN_POINT('Ctrl Pts',(-8.27631857770454,1.78617587380135,
51.0129934648596));
#245817=CARTESIAN_POINT('Ctrl Pts',(-5.95881855176718,-6.00611906131259,
51.3309021965091));
#245818=CARTESIAN_POINT('Ctrl Pts',(0.500233518445705,-7.86831706846291,
51.5958261395504));
#245819=CARTESIAN_POINT('Ctrl Pts',(4.88418567491117,-5.62033200822035,
51.8077652939834));
#245820=CARTESIAN_POINT('Ctrl Pts',(6.9931594373733,-2.60329891049933,51.9667196598082));
#245821=CARTESIAN_POINT('Ctrl Pts',(7.37151615867653,1.05080861816805,52.1256740256329));
#245822=CARTESIAN_POINT('Ctrl Pts',(5.52334883621293,5.63219274911859,52.337613180066));
#245823=CARTESIAN_POINT('Ctrl Pts',(0.649633021818951,7.8637100181193,52.549552334499));
#245824=CARTESIAN_POINT('Ctrl Pts',(-4.01456277072602,6.26218504075905,
52.761491488932));
#245825=CARTESIAN_POINT('Ctrl Pts',(-7.40281163663164,2.7123339092285,52.973430643365));
#245826=CARTESIAN_POINT('Ctrl Pts',(-7.44882858971283,-4.02527341840082,
53.2383545864063));
#245827=CARTESIAN_POINT('Ctrl Pts',(-0.620886683000079,-8.43774166696402,
53.5562633180558));
#245828=CARTESIAN_POINT('Ctrl Pts',(5.49685943532892,-5.65200702503782,
53.8211872610971));
#245829=CARTESIAN_POINT('Ctrl Pts',(7.36532272413416,-1.09335390381452,
54.03312641553));
#245830=CARTESIAN_POINT('Ctrl Pts',(7.00543631370554,2.57007902379404,54.1920807813549));
#245831=CARTESIAN_POINT('Ctrl Pts',(4.91655827097942,5.59203934157381,54.3510351471795));
#245832=CARTESIAN_POINT('Ctrl Pts',(0.533242114523018,7.87049111409306,
54.5629743016127));
#245833=CARTESIAN_POINT('Ctrl Pts',(-4.62034582655523,6.39627725752574,
54.7749134560455));
#245834=CARTESIAN_POINT('Ctrl Pts',(-7.12210108419128,2.14647428854086,
54.9868526104786));
#245835=CARTESIAN_POINT('Ctrl Pts',(-7.38754284268422,-2.7536495982795,
55.1987917649117));
#245836=CARTESIAN_POINT('Ctrl Pts',(-3.0409649820265,-7.90192415996867,
55.4637157079528));
#245837=CARTESIAN_POINT('Ctrl Pts',(5.01548221836353,-6.81365708183404,
55.7816244396025));
#245838=CARTESIAN_POINT('Ctrl Pts',(7.85135038073463,-0.718988359974968,
56.0465483826436));
#245839=CARTESIAN_POINT('Ctrl Pts',(6.30622430352142,3.95915857516586,56.2584875370768));
#245840=CARTESIAN_POINT('Ctrl Pts',(3.65046167257338,6.50811598782652,56.4174419029014));
#245841=CARTESIAN_POINT('Ctrl Pts',(0.0983945018344138,7.44538566842941,
56.5763962687262));
#245842=CARTESIAN_POINT('Ctrl Pts',(-4.71317417004024,6.32573843694028,
56.7883354231592));
#245843=CARTESIAN_POINT('Ctrl Pts',(-7.66949704921241,1.85439297998827,
57.0002745775923));
#245844=CARTESIAN_POINT('Ctrl Pts',(-6.80631148353952,-3.00096646329874,
57.2122137320253));
#245845=CARTESIAN_POINT('Ctrl Pts',(-3.82135819804321,-6.89605661844852,
57.4241528864583));
#245846=CARTESIAN_POINT('Ctrl Pts',(2.8285768840507,-7.98041516857501,57.6890768294995));
#245847=CARTESIAN_POINT('Ctrl Pts',(8.24109619250587,-1.9145020912532,58.0069855611492));
#245848=CARTESIAN_POINT('Ctrl Pts',(6.43199051945318,4.55962114879134,58.2719095041902));
#245849=CARTESIAN_POINT('Ctrl Pts',(2.21595945663504,7.10865143864736,58.4838486586235));
#245850=CARTESIAN_POINT('Ctrl Pts',(-1.45915351569631,7.31794473548151,
58.6428030244481));
#245851=CARTESIAN_POINT('Ctrl Pts',(-4.76706382838783,5.72001325922605,
58.8017573902729));
#245852=CARTESIAN_POINT('Ctrl Pts',(-7.69414371217973,1.7404396186147,59.0136965447059));
#245853=CARTESIAN_POINT('Ctrl Pts',(-7.03220756772331,-3.5788287241167,
59.2256356991389));
#245854=CARTESIAN_POINT('Ctrl Pts',(-3.21898223211034,-6.70595475038146,
59.4375748535719));
#245855=CARTESIAN_POINT('Ctrl Pts',(1.58161056894603,-7.7237868543091,59.6495140080049));
#245856=CARTESIAN_POINT('Ctrl Pts',(7.33852751575318,-4.22301874875562,
59.9144379510463));
#245857=CARTESIAN_POINT('Ctrl Pts',(7.50552310889206,3.90488253004291,60.2323466826956));
#245858=CARTESIAN_POINT('Ctrl Pts',(1.92101311044358,7.64659111580737,60.497270625737));
#245859=CARTESIAN_POINT('Ctrl Pts',(-2.93943431425503,6.84128113015493,
60.70920978017));
#245860=CARTESIAN_POINT('Ctrl Pts',(-5.867408121995,4.61031084243544,60.8681641459948));
#245861=CARTESIAN_POINT('Ctrl Pts',(-7.34117267070119,1.24524417227922,
61.0271185118195));
#245862=CARTESIAN_POINT('Ctrl Pts',(-6.97682582006776,-3.68142350268944,
61.2390576662526));
#245863=CARTESIAN_POINT('Ctrl Pts',(-3.01479862712008,-7.29184116324697,
61.4509968206856));
#245864=CARTESIAN_POINT('Ctrl Pts',(1.91559151921653,-7.18764111905368,
61.6629359751185));
#245865=CARTESIAN_POINT('Ctrl Pts',(6.22435822338273,-4.83898130494505,
61.8748751295516));
#245866=CARTESIAN_POINT('Ctrl Pts',(8.3211221332371,1.56422501436302,62.1397990725929));
#245867=CARTESIAN_POINT('Ctrl Pts',(3.16232546828451,7.84733600301313,62.4577078042424));
#245868=CARTESIAN_POINT('Ctrl Pts',(-3.51332353295876,7.05813040511431,
62.7226317472836));
#245869=CARTESIAN_POINT('Ctrl Pts',(-6.68195182563262,3.28556256820024,
62.9345709017167));
#245870=CARTESIAN_POINT('Ctrl Pts',(-7.45541884659326,-0.313327234361745,
63.0935252675414));
#245871=CARTESIAN_POINT('Ctrl Pts',(-6.38665407163377,-3.82806726677171,
63.2524796333662));
#245872=CARTESIAN_POINT('Ctrl Pts',(-2.90600840591369,-7.33376388183294,
63.4644187877991));
#245873=CARTESIAN_POINT('Ctrl Pts',(2.45171138262837,-7.49993797363672,
63.6763579422323));
#245874=CARTESIAN_POINT('Ctrl Pts',(6.12941199250644,-4.21449692738344,
63.8882970966652));
#245875=CARTESIAN_POINT('Ctrl Pts',(7.87528941780481,0.371741776518995,
64.1002362510983));
#245876=CARTESIAN_POINT('Ctrl Pts',(5.30406421297267,6.59960425150415,64.3651601941394));
#245877=CARTESIAN_POINT('Ctrl Pts',(-2.70088388250976,8.01786823069259,
64.6830689257891));
#245878=CARTESIAN_POINT('Ctrl Pts',(-7.25893680954418,3.07709009583346,
64.9479928688302));
#245879=CARTESIAN_POINT('Ctrl Pts',(-7.21270472779369,-1.84940317381245,
65.1599320232634));
#245880=CARTESIAN_POINT('Ctrl Pts',(-5.45988826122027,-5.08636061530274,
65.318886389088));
#245881=CARTESIAN_POINT('Ctrl Pts',(-2.36230946156806,-7.06136978478256,
65.4778407549128));
#245882=CARTESIAN_POINT('Ctrl Pts',(2.56161868239115,-7.46103794761829,
65.6897799093458));
#245883=CARTESIAN_POINT('Ctrl Pts',(6.73977532507158,-4.10309479289059,
65.9017190637788));
#245884=CARTESIAN_POINT('Ctrl Pts',(7.39705311185201,0.784398486419424,
66.1136582182119));
#245885=CARTESIAN_POINT('Ctrl Pts',(5.74086320472686,5.403782474047,66.3255973726448));
#245886=CARTESIAN_POINT('Ctrl Pts',(-0.262459218000729,8.46280028184657,
66.5905213156862));
#245887=CARTESIAN_POINT('Ctrl Pts',(-7.2658792543938,4.33451074223193,66.9084300473356));
#245888=CARTESIAN_POINT('Ctrl Pts',(-7.51545035067317,-2.38299246447439,
67.1733539903769));
#245889=CARTESIAN_POINT('Ctrl Pts',(-4.27657992960506,-6.09542990261524,
67.3852931448099));
#245890=CARTESIAN_POINT('Ctrl Pts',(-0.839993365772602,-7.41457047170496,
67.5442475106347));
#245891=CARTESIAN_POINT('Ctrl Pts',(2.79750905089242,-6.90053565519577,
67.7032018764595));
#245892=CARTESIAN_POINT('Ctrl Pts',(6.79797137375908,-4.00206981200973,
67.9151410308924));
#245893=CARTESIAN_POINT('Ctrl Pts',(7.78828105606738,1.26595276683344,68.1270801853255));
#245894=CARTESIAN_POINT('Ctrl Pts',(5.10920715677595,5.40626285126827,68.3390193397585));
#245895=CARTESIAN_POINT('Ctrl Pts',(0.847018506823715,7.83842682077682,
68.5509584941915));
#245896=CARTESIAN_POINT('Ctrl Pts',(-5.70282827152682,6.25824437568983,
68.8158824372328));
#245897=CARTESIAN_POINT('Ctrl Pts',(-8.3384379818395,-1.43228411544367,
69.1337911688823));
#245898=CARTESIAN_POINT('Ctrl Pts',(-4.15956757109609,-6.69765959122558,
69.3987151119235));
#245899=CARTESIAN_POINT('Ctrl Pts',(0.715136918934491,-7.41161117488028,
69.6106542663566));
#245900=CARTESIAN_POINT('Ctrl Pts',(4.18365528963165,-6.1788733574416,69.7696086321812));
#245901=CARTESIAN_POINT('Ctrl Pts',(6.61266885939531,-3.42287173955488,
69.9285629980062));
#245902=CARTESIAN_POINT('Ctrl Pts',(7.76679459976119,1.38054354820726,70.140502152439));
#245903=CARTESIAN_POINT('Ctrl Pts',(5.09324835207816,6.02650454722979,70.3524413068722));
#245904=CARTESIAN_POINT('Ctrl Pts',(0.36555935057273,7.42953814632684,70.5643804613051));
#245905=CARTESIAN_POINT('Ctrl Pts',(-4.45396371572346,6.50543338303905,
70.7763196157382));
#245906=CARTESIAN_POINT('Ctrl Pts',(-8.40204513351695,1.04558175432152,
71.0412435587793));
#245907=CARTESIAN_POINT('Ctrl Pts',(-5.40304876320707,-6.5106291922939,
71.3591522904291));
#245908=CARTESIAN_POINT('Ctrl Pts',(1.19571080635691,-7.79301928146387,
71.62407623347));
#245909=CARTESIAN_POINT('Ctrl Pts',(5.36304927419964,-5.16529772798693,
71.8360153879034));
#245910=CARTESIAN_POINT('Ctrl Pts',(7.19651870242583,-1.97324473515594,
71.9949697537278));
#245911=CARTESIAN_POINT('Ctrl Pts',(7.24910192905725,1.70007989524192,72.1539241195528));
#245912=CARTESIAN_POINT('Ctrl Pts',(5.00301187184924,6.0994873116443,72.3658632739857));
#245913=CARTESIAN_POINT('Ctrl Pts',(-0.0510729370531945,7.89052074771417,
72.5778024284188));
#245914=CARTESIAN_POINT('Ctrl Pts',(-4.55244977206186,5.88150167157887,
72.7897415828518));
#245915=CARTESIAN_POINT('Ctrl Pts',(-7.61724391812272,2.04601116422751,
73.0016807372848));
#245916=CARTESIAN_POINT('Ctrl Pts',(-7.05604730840642,-4.67067368392185,
73.266604680326));
#245917=CARTESIAN_POINT('Ctrl Pts',(0.117871558726145,-8.45787944261411,
73.5845134119757));
#245918=CARTESIAN_POINT('Ctrl Pts',(7.16958247662802,-4.48195502366287,
73.902422143625));
#245919=CARTESIAN_POINT('Ctrl Pts',(7.65256736296178,3.60409978063233,74.2203308752747));
#245920=CARTESIAN_POINT('Ctrl Pts',(1.11114445795367,8.38189666584284,74.5382396069241));
#245921=CARTESIAN_POINT('Ctrl Pts',(-6.4453788949029,5.47783801068378,74.8561483385738));
#245922=CARTESIAN_POINT('Ctrl Pts',(-8.0948899913508,-2.46490411742087,
75.174057070223));
#245923=CARTESIAN_POINT('Ctrl Pts',(-3.27421567416541,-7.1755193757226,
75.4389810132645));
#245924=CARTESIAN_POINT('Ctrl Pts',(1.6347076480826,-7.25565929087297,75.6509201676975));
#245925=CARTESIAN_POINT('Ctrl Pts',(6.05052887116323,-5.06498040413063,
75.8628593221304));
#245926=CARTESIAN_POINT('Ctrl Pts',(7.88879558544593,-0.0278830741340137,
76.0747984765636));
#245927=CARTESIAN_POINT('Ctrl Pts',(5.92772275986439,4.50575779533842,76.2867376309964));
#245928=CARTESIAN_POINT('Ctrl Pts',(3.06234663935547,6.80482250169787,76.4456919968214));
#245929=CARTESIAN_POINT('Ctrl Pts',(-0.566278238928978,7.42441425920965,
76.604646362646));
#245930=CARTESIAN_POINT('Ctrl Pts',(-5.24632254028144,5.88531848390908,
76.8165855170791));
#245931=CARTESIAN_POINT('Ctrl Pts',(-8.46054846951648,-0.0186550825584463,
77.0815094601202));
#245932=CARTESIAN_POINT('Ctrl Pts',(-4.54533233720298,-7.14335758414781,
77.39941819177));
#245933=CARTESIAN_POINT('Ctrl Pts',(2.17844426069194,-7.57712589872956,
77.664342134811));
#245934=CARTESIAN_POINT('Ctrl Pts',(5.96050262542447,-4.45017743003856,
77.8762812892441));
#245935=CARTESIAN_POINT('Ctrl Pts',(7.89000395397738,0.0881671137640604,
78.0882204436772));
#245936=CARTESIAN_POINT('Ctrl Pts',(6.01110908805987,5.10838197229029,78.30015959811));
#245937=CARTESIAN_POINT('Ctrl Pts',(1.57291833765724,7.27800579091012,78.5120987525432));
#245938=CARTESIAN_POINT('Ctrl Pts',(-2.09885258226522,7.16074475090987,
78.6710531183679));
#245939=CARTESIAN_POINT('Ctrl Pts',(-5.25836834119772,5.27190320555331,
78.8300074841926));
#245940=CARTESIAN_POINT('Ctrl Pts',(-7.81274198177251,1.05910769268254,
79.0419466386258));
#245941=CARTESIAN_POINT('Ctrl Pts',(-6.41508694258267,-5.51612593070902,
79.3068705816669));
#245942=CARTESIAN_POINT('Ctrl Pts',(1.19245520850734,-8.38247717181995,
79.6247793133165));
#245943=CARTESIAN_POINT('Ctrl Pts',(6.58237766265624,-4.33943310603345,
79.8897032563578));
#245944=CARTESIAN_POINT('Ctrl Pts',(7.42200396880351,0.495512739411206,
80.1016424107907));
#245945=CARTESIAN_POINT('Ctrl Pts',(5.93645243083523,5.19793139167711,80.3135815652239));
#245946=CARTESIAN_POINT('Ctrl Pts',(1.24441809527773,7.78976258834587,80.5255207196566));
#245947=CARTESIAN_POINT('Ctrl Pts',(-3.53806550113452,6.55175867444267,
80.73745987409));
#245948=CARTESIAN_POINT('Ctrl Pts',(-6.25113863890163,4.07488771031202,
80.8964142399143));
#245949=CARTESIAN_POINT('Ctrl Pts',(-7.42299076065899,0.585328761610284,
81.0553686057394));
#245950=CARTESIAN_POINT('Ctrl Pts',(-6.62384401692773,-4.27613581386113,
81.2673077601722));
#245951=CARTESIAN_POINT('Ctrl Pts',(-1.286147084199,-8.36222520575478,81.5322317032136));
#245952=CARTESIAN_POINT('Ctrl Pts',(6.35708219443056,-5.59243948780764,
81.8501404348632));
#245953=CARTESIAN_POINT('Ctrl Pts',(7.8224042262569,0.984056646358646,82.1150643779043));
#245954=CARTESIAN_POINT('Ctrl Pts',(5.31602691445828,5.20303119054768,82.3270035323375));
#245955=CARTESIAN_POINT('Ctrl Pts',(1.12946861296887,7.8092418943331,82.5389426867703));
#245956=CARTESIAN_POINT('Ctrl Pts',(-4.12041745867891,6.72689657241653,
82.7508818412035));
#245957=CARTESIAN_POINT('Ctrl Pts',(-6.94843375179018,2.67632539625451,
82.9628209956364));
#245958=CARTESIAN_POINT('Ctrl Pts',(-7.39873571944801,-0.969615329745792,
83.1217753614612));
#245959=CARTESIAN_POINT('Ctrl Pts',(-6.01965891788265,-4.38259148244517,
83.280729727286));
#245960=CARTESIAN_POINT('Ctrl Pts',(-2.25111163908191,-7.55600049306653,
83.4926688817188));
#245961=CARTESIAN_POINT('Ctrl Pts',(4.46099559454575,-7.18891528792723,
83.7575928247604));
#245962=CARTESIAN_POINT('Ctrl Pts',(8.46609728487924,-0.114325039996204,
84.0755015564097));
#245963=CARTESIAN_POINT('Ctrl Pts',(5.3024933093211,5.83454711757506,84.340425499451));
#245964=CARTESIAN_POINT('Ctrl Pts',(0.654834329437635,7.40964693664927,
84.552364653884));
#245965=CARTESIAN_POINT('Ctrl Pts',(-4.22040857419456,6.66694156108873,
84.7643038083171));
#245966=CARTESIAN_POINT('Ctrl Pts',(-7.50472227466187,2.43066268945576,
84.9762429627499));
#245967=CARTESIAN_POINT('Ctrl Pts',(-7.01894948765949,-2.4855175153939,
85.1881821171831));
#245968=CARTESIAN_POINT('Ctrl Pts',(-4.99003695120001,-5.54806050431944,
85.3471364830078));
#245969=CARTESIAN_POINT('Ctrl Pts',(-1.72290192399602,-7.24396373195811,
85.5060908488326));
#245970=CARTESIAN_POINT('Ctrl Pts',(3.20364600373927,-7.20397802228505,
85.7180300032656));
#245971=CARTESIAN_POINT('Ctrl Pts',(8.06390435080163,-2.56016236451326,
85.9829539463069));
#245972=CARTESIAN_POINT('Ctrl Pts',(6.50577569840637,5.41874118350685,86.3008626779564));
#245973=CARTESIAN_POINT('Ctrl Pts',(0.233871956267354,7.88058876421495,
86.5657866209976));
#245974=CARTESIAN_POINT('Ctrl Pts',(-4.32111265355103,6.05472221989799,
86.7777257754307));
#245975=CARTESIAN_POINT('Ctrl Pts',(-7.54169303146352,2.32009149200691,
86.9896649298636));
#245976=CARTESIAN_POINT('Ctrl Pts',(-7.28178746474286,-3.03389994034617,
87.2016040842967));
#245977=CARTESIAN_POINT('Ctrl Pts',(-3.71571842818992,-6.45266501470942,
87.4135432387298));
#245978=CARTESIAN_POINT('Ctrl Pts',(-0.182813845036814,-7.45976026638884,
87.5724976045544));
#245979=CARTESIAN_POINT('Ctrl Pts',(3.40198965826229,-6.62343324528226,
87.7314519703793));
#245980=CARTESIAN_POINT('Ctrl Pts',(7.11853069868959,-3.38927245211331,
87.9433911248123));
#245981=CARTESIAN_POINT('Ctrl Pts',(7.79079554783678,3.29916496152483,88.2083150678536));
#245982=CARTESIAN_POINT('Ctrl Pts',(1.41837078524883,8.34722096073662,88.5262237995031));
#245983=CARTESIAN_POINT('Ctrl Pts',(-4.94716290886032,6.1387258055558,88.7911477425443));
#245984=CARTESIAN_POINT('Ctrl Pts',(-7.22006221792976,1.78951873251688,
89.0030868969774));
#245985=CARTESIAN_POINT('Ctrl Pts',(-7.23796740124329,-3.14193988017693,
89.2150260514101));
#245986=CARTESIAN_POINT('Ctrl Pts',(-3.55876946335482,-7.04018021334767,
89.4269652058435));
#245987=CARTESIAN_POINT('Ctrl Pts',(1.37351966289223,-7.31825750881274,
89.6389043602761));
#245988=CARTESIAN_POINT('Ctrl Pts',(4.71228104662943,-5.78583196018578,
89.7978587261012));
#245989=CARTESIAN_POINT('Ctrl Pts',(6.89167190790973,-2.81926584474774,
89.9568130919259));
#245990=CARTESIAN_POINT('Ctrl Pts',(7.61180363044634,2.05452976477962,90.1687522463588));
#245991=CARTESIAN_POINT('Ctrl Pts',(3.77294238406992,7.57270694521032,90.4336761894001));
#245992=CARTESIAN_POINT('Ctrl Pts',(-4.35079197496986,7.26350346887399,
90.7515849210497));
#245993=CARTESIAN_POINT('Ctrl Pts',(-7.75028138648021,1.44620669096039,
91.016508864091));
#245994=CARTESIAN_POINT('Ctrl Pts',(-6.64859761096745,-3.33583955433172,
91.2284480185239));
#245995=CARTESIAN_POINT('Ctrl Pts',(-3.45522124698925,-7.09375813278554,
91.4403871729571));
#245996=CARTESIAN_POINT('Ctrl Pts',(1.8748160657606,-7.66250887433638,91.6523263273899));
#245997=CARTESIAN_POINT('Ctrl Pts',(5.80255816582133,-4.66623702375972,
91.8642654818231));
#245998=CARTESIAN_POINT('Ctrl Pts',(7.34235848692903,-1.33087038563187,
92.0232198476477));
#245999=CARTESIAN_POINT('Ctrl Pts',(7.06878493979507,2.34001732142302,92.1821742134726));
#246000=CARTESIAN_POINT('Ctrl Pts',(4.44636692906912,6.51079627963601,92.3941133679054));
#246001=CARTESIAN_POINT('Ctrl Pts',(-2.05842322905156,8.20633161172813,
92.6590373109469));
#246002=CARTESIAN_POINT('Ctrl Pts',(-8.02869157557259,2.6884912192783,92.9769460425962));
#246003=CARTESIAN_POINT('Ctrl Pts',(-6.82812914707941,-3.94144995064046,
93.2418699856376));
#246004=CARTESIAN_POINT('Ctrl Pts',(-2.88140051968578,-6.85778439220427,
93.4538091400705));
#246005=CARTESIAN_POINT('Ctrl Pts',(1.98832067587906,-7.63587186914367,
93.6657482945037));
#246006=CARTESIAN_POINT('Ctrl Pts',(6.40724755397117,-4.601755785768,93.8776874489367));
#246007=CARTESIAN_POINT('Ctrl Pts',(7.44252373823067,0.228669271041487,
94.0896266033697));
#246008=CARTESIAN_POINT('Ctrl Pts',(6.44323850828845,3.76379086284547,94.2485809691943));
#246009=CARTESIAN_POINT('Ctrl Pts',(3.84819713631814,6.37454158270743,94.4075353350193));
#246010=CARTESIAN_POINT('Ctrl Pts',(-0.85627224174157,7.83756626197594,
94.6194744894521));
#246011=CARTESIAN_POINT('Ctrl Pts',(-6.90038169731781,4.89547925568775,
94.8843984324935));
#246012=CARTESIAN_POINT('Ctrl Pts',(-7.84749908248109,-3.17877831914504,
95.2023071641429));
#246013=CARTESIAN_POINT('Ctrl Pts',(-2.62395032113123,-7.43459885096939,
95.4672311071843));
#246014=CARTESIAN_POINT('Ctrl Pts',(2.27077815416402,-7.08344847509866,
95.6791702616173));
#246015=CARTESIAN_POINT('Ctrl Pts',(6.47615113221677,-4.50770726919954,
95.8911094160503));
#246016=CARTESIAN_POINT('Ctrl Pts',(7.85995451357935,0.670889390422631,
96.1030485704833));
#246017=CARTESIAN_POINT('Ctrl Pts',(5.50514619750763,5.01366279018771,96.3149877249164));
#246018=CARTESIAN_POINT('Ctrl Pts',(2.4470944939041,7.04933845632589,96.473942090741));
#246019=CARTESIAN_POINT('Ctrl Pts',(-1.22207526445053,7.34506185390236,
96.6328964565659));
#246020=CARTESIAN_POINT('Ctrl Pts',(-5.74733333571994,5.39711094855044,
96.844835610999));
#246021=CARTESIAN_POINT('Ctrl Pts',(-8.42558447744543,-0.768447086648144,
97.10975955404));
#246022=CARTESIAN_POINT('Ctrl Pts',(-3.89430695789088,-7.51812787664129,
97.4276682856896));
#246023=CARTESIAN_POINT('Ctrl Pts',(2.84146339511113,-7.35421383540367,
97.692592228731));
#246024=CARTESIAN_POINT('Ctrl Pts',(6.33147860409847,-3.90436350903053,
97.9045313831638));
#246025=CARTESIAN_POINT('Ctrl Pts',(7.85113768408234,0.78714381004357,98.1164705375972));
#246026=CARTESIAN_POINT('Ctrl Pts',(5.53467498128681,5.62106310062747,98.3284096920297));
#246027=CARTESIAN_POINT('Ctrl Pts',(0.921650548315969,7.38877591326425,
98.540348846463));
#246028=CARTESIAN_POINT('Ctrl Pts',(-2.72527642184487,6.94653241253989,
98.6993032122876));
#246029=CARTESIAN_POINT('Ctrl Pts',(-5.70494174153298,4.7850852986492,98.8582575781126));
#246030=CARTESIAN_POINT('Ctrl Pts',(-7.87586601184446,0.362466034703414,
99.0701967325454));
#246031=CARTESIAN_POINT('Ctrl Pts',(-5.90092357360854,-6.06300962311448,
99.3351206755868));
#246032=CARTESIAN_POINT('Ctrl Pts',(1.93073303258823,-8.24379423619251,
99.6530294072363));
#246033=CARTESIAN_POINT('Ctrl Pts',(6.94109181254378,-3.73893297779421,
99.9179533502775));
#246034=CARTESIAN_POINT('Ctrl Pts',(7.34887382895609,1.15140313135301,100.129892504711));
#246035=CARTESIAN_POINT('Ctrl Pts',(5.45237566459545,5.70364426697838,100.341831659144));
#246036=CARTESIAN_POINT('Ctrl Pts',(0.549083957339117,7.86940177761382,
100.553770813577));
#246037=CARTESIAN_POINT('Ctrl Pts',(-4.1048480871876,6.21238049468619,100.76570996801));
#246038=CARTESIAN_POINT('Ctrl Pts',(-6.58770877616357,3.50478775596863,
100.924664333834));
#246039=CARTESIAN_POINT('Ctrl Pts',(-7.4456558563651,-0.0749029919971758,
101.083618699659));
#246040=CARTESIAN_POINT('Ctrl Pts',(-6.21876413329544,-4.84640276053068,
101.295557854092));
#246041=CARTESIAN_POINT('Ctrl Pts',(-0.539909162595909,-8.44330994383676,
101.560481797134));
#246042=CARTESIAN_POINT('Ctrl Pts',(6.82774178522963,-5.00697668918455,
101.878390528783));
#246043=CARTESIAN_POINT('Ctrl Pts',(7.70439671035187,1.67351327814228,102.143314471825));
#246044=CARTESIAN_POINT('Ctrl Pts',(4.83393995337018,5.65373330216565,102.355253626257));
#246045=CARTESIAN_POINT('Ctrl Pts',(0.432860360337941,7.87861600920848,
102.567192780691));
#246046=CARTESIAN_POINT('Ctrl Pts',(-4.70043121148294,6.33521301582163,
102.779131935123));
#246047=CARTESIAN_POINT('Ctrl Pts',(-7.15829960162867,2.04992586279794,
102.991071089556));
#246048=CARTESIAN_POINT('Ctrl Pts',(-7.28367563428598,-1.6215774383111,
103.150025455381));
#246049=CARTESIAN_POINT('Ctrl Pts',(-5.6075213658915,-4.89888821271768,
103.308979821206));
#246050=CARTESIAN_POINT('Ctrl Pts',(-1.57253466484514,-7.72578680722558,
103.520918975639));
#246051=CARTESIAN_POINT('Ctrl Pts',(5.08061941222205,-6.76522661111206,
103.78584291868));
#246052=CARTESIAN_POINT('Ctrl Pts',(8.44291014169328,0.63650749492915,104.10375165033));
#246053=CARTESIAN_POINT('Ctrl Pts',(4.7644859407326,6.28156422264086,104.368675593371));
#246054=CARTESIAN_POINT('Ctrl Pts',(-0.00448826495536526,7.43852509441779,
104.580614747804));
#246055=CARTESIAN_POINT('Ctrl Pts',(-4.79471474775313,6.26663137577012,
104.792553902237));
#246056=CARTESIAN_POINT('Ctrl Pts',(-7.69062470199101,1.75592403675235,
105.00449305667));
#246057=CARTESIAN_POINT('Ctrl Pts',(-6.7710239269735,-3.0978515474434,105.216432211103));
#246058=CARTESIAN_POINT('Ctrl Pts',(-4.47865172838059,-5.96851093907047,
105.375386576928));
#246059=CARTESIAN_POINT('Ctrl Pts',(-1.07406084817673,-7.36816088885468,
105.534340942753));
#246060=CARTESIAN_POINT('Ctrl Pts',(3.82955346812604,-6.89167376604588,
105.746280097186));
#246061=CARTESIAN_POINT('Ctrl Pts',(8.25908404421422,-1.83535159088185,
106.011204040227));
#246062=CARTESIAN_POINT('Ctrl Pts',(5.99988701466406,5.97404630573564,106.329112771877));
#246063=CARTESIAN_POINT('Ctrl Pts',(-0.465535222508124,7.87030192046052,
106.594036714917));
#246064=CARTESIAN_POINT('Ctrl Pts',(-4.84075914199551,5.64789577223166,
106.805975869351));
#246065=CARTESIAN_POINT('Ctrl Pts',(-7.7176496040166,1.64251115726207,107.017915023784));
#246066=CARTESIAN_POINT('Ctrl Pts',(-6.98422221497737,-3.66737202660644,
107.229854178217));
#246067=CARTESIAN_POINT('Ctrl Pts',(-3.12917001166206,-6.75660745254302,
107.44179333265));
#246068=CARTESIAN_POINT('Ctrl Pts',(0.47909274384839,-7.44660421109663,
107.600747698475));
#246069=CARTESIAN_POINT('Ctrl Pts',(3.97566059304344,-6.29583389540692,
107.759702064299));
#246070=CARTESIAN_POINT('Ctrl Pts',(7.39091831859026,-2.74499061396732,
107.971641218732));
#246071=CARTESIAN_POINT('Ctrl Pts',(7.46771553014855,3.97670837154622,108.236565161774));
#246072=CARTESIAN_POINT('Ctrl Pts',(0.672942351553414,8.44008424385051,
108.554473893423));
#246073=CARTESIAN_POINT('Ctrl Pts',(-5.47179099638164,5.67607951446395,
108.819397836464));
#246074=CARTESIAN_POINT('Ctrl Pts',(-7.35025794708428,1.14253395403798,
109.031336990897));
#246075=CARTESIAN_POINT('Ctrl Pts',(-6.93099862198739,-3.77110281139561,
109.24327614533));
#246076=CARTESIAN_POINT('Ctrl Pts',(-2.92076503521324,-7.32789936740364,
109.455215299763));
#246077=CARTESIAN_POINT('Ctrl Pts',(2.01675902450346,-7.1677145776551,109.667154454196));
#246078=CARTESIAN_POINT('Ctrl Pts',(5.20655523270202,-5.34539303912755,
109.826108820021));
#246079=CARTESIAN_POINT('Ctrl Pts',(7.11443051527581,-2.19733475668721,
109.985063185846));
#246080=CARTESIAN_POINT('Ctrl Pts',(7.39974485319851,2.72110697518556,110.197002340279));
#246081=CARTESIAN_POINT('Ctrl Pts',(3.08689514972448,7.87731318700451,110.46192628332));
#246082=CARTESIAN_POINT('Ctrl Pts',(-4.97746055926141,6.84928900199175,
110.77983501497));
#246083=CARTESIAN_POINT('Ctrl Pts',(-7.84796126083906,0.753577740494986,
111.044758958011));
#246084=CARTESIAN_POINT('Ctrl Pts',(-6.32676235785494,-3.91200125153804,
111.256698112444));
#246085=CARTESIAN_POINT('Ctrl Pts',(-2.81287553995915,-7.37208854455821,
111.468637266877));
#246086=CARTESIAN_POINT('Ctrl Pts',(2.54659477910015,-7.46617924783338,
111.68057642131));
#246087=CARTESIAN_POINT('Ctrl Pts',(6.19330734239266,-4.13356908643254,
111.892515575743));
#246088=CARTESIAN_POINT('Ctrl Pts',(7.4314211347052,-0.674851133649304,
112.051469941568));
#246089=CARTESIAN_POINT('Ctrl Pts',(6.83355947930127,2.95734110857797,112.210424307393));
#246090=CARTESIAN_POINT('Ctrl Pts',(3.85179048651812,6.87927010014943,112.422363461825));
#246091=CARTESIAN_POINT('Ctrl Pts',(-2.7776804047817,7.99158784475522,112.687287404867));
#246092=CARTESIAN_POINT('Ctrl Pts',(-8.23538413392086,1.96629642184775,
113.005196136516));
#246093=CARTESIAN_POINT('Ctrl Pts',(-6.45190974192794,-4.53114070015648,
113.270120079558));
#246094=CARTESIAN_POINT('Ctrl Pts',(-2.26222846692231,-7.08618360531622,
113.482059233991));
#246095=CARTESIAN_POINT('Ctrl Pts',(2.65729172693086,-7.42958673077397,
113.693998388424));
#246096=CARTESIAN_POINT('Ctrl Pts',(6.78990162222115,-4.01574569541913,
113.905937542857));
#246097=CARTESIAN_POINT('Ctrl Pts',(7.39296419871876,0.887428637191924,
114.11787669729));
#246098=CARTESIAN_POINT('Ctrl Pts',(6.08428053030461,4.32006649977597,114.276831063114));
#246099=CARTESIAN_POINT('Ctrl Pts',(3.26805169895397,6.69053358728565,114.435785428939));
#246100=CARTESIAN_POINT('Ctrl Pts',(-1.54757566664994,7.73082509301787,
114.647724583372));
#246101=CARTESIAN_POINT('Ctrl Pts',(-7.30712876103848,4.26460478604429,
114.912648526414));
#246102=CARTESIAN_POINT('Ctrl Pts',(-7.53486622398735,-3.86182138872599,
115.230557258063));
#246103=CARTESIAN_POINT('Ctrl Pts',(-1.954666249214,-7.63790908670584,115.495481201104));
#246104=CARTESIAN_POINT('Ctrl Pts',(2.88967413267942,-6.85430223521909,
115.707420355537));
#246105=CARTESIAN_POINT('Ctrl Pts',(6.85019813537203,-3.91596014002346,
115.91935950997));
#246106=CARTESIAN_POINT('Ctrl Pts',(7.76955642183854,1.36490678714159,116.131298664403));
#246107=CARTESIAN_POINT('Ctrl Pts',(5.0390993610438,5.48187256867338,116.343237818836));
#246108=CARTESIAN_POINT('Ctrl Pts',(1.81265357974105,7.23848956162698,116.502192184661));
#246109=CARTESIAN_POINT('Ctrl Pts',(-1.86828644079946,7.20783652455841,
116.661146550486));
#246110=CARTESIAN_POINT('Ctrl Pts',(-6.20308001327729,4.86646128225844,
116.873085704919));
#246111=CARTESIAN_POINT('Ctrl Pts',(-8.32431331143111,-1.51221447046321,
117.13800964796));
#246112=CARTESIAN_POINT('Ctrl Pts',(-3.21261961787344,-7.83370593286875,
117.45591837961));
#246113=CARTESIAN_POINT('Ctrl Pts',(3.48211228444008,-7.07341992257992,
117.720842322651));
#246114=CARTESIAN_POINT('Ctrl Pts',(6.65261833304377,-3.32781385291546,
117.932781477084));
#246115=CARTESIAN_POINT('Ctrl Pts',(7.75047021907653,1.47992219231806,118.144720631517));
#246116=CARTESIAN_POINT('Ctrl Pts',(5.01467571504118,6.08949956915138,118.35665978595));
#246117=CARTESIAN_POINT('Ctrl Pts',(0.263127717982059,7.44138515557925,
118.568598940383));
#246118=CARTESIAN_POINT('Ctrl Pts',(-3.33024822704816,6.67764111645518,
118.727553306208));
#246119=CARTESIAN_POINT('Ctrl Pts',(-6.10660908642409,4.26060172454973,
118.886507672032));
#246120=CARTESIAN_POINT('Ctrl Pts',(-7.87699554054792,-0.337028659061501,
119.098446826465));
#246121=CARTESIAN_POINT('Ctrl Pts',(-5.34031144393764,-6.56216872636603,
119.363370769507));
#246122=CARTESIAN_POINT('Ctrl Pts',(2.65381321717774,-8.04022069722845,
119.681279501156));
#246123=CARTESIAN_POINT('Ctrl Pts',(7.24516953240903,-3.10900206002699,
119.946203444198));
#246124=CARTESIAN_POINT('Ctrl Pts',(7.21789743819818,1.7982303235287,120.158142598631));
#246125=CARTESIAN_POINT('Ctrl Pts',(4.92538082098571,6.16446121574084,120.370081753063));
#246126=CARTESIAN_POINT('Ctrl Pts',(-0.150572262960701,7.88709740800408,
120.582020907497));
#246127=CARTESIAN_POINT('Ctrl Pts',(-4.63931958883328,5.82410190349662,
120.79396006193));
#246128=CARTESIAN_POINT('Ctrl Pts',(-6.8724241269978,2.90710005892275,120.952914427754));
#246129=CARTESIAN_POINT('Ctrl Pts',(-7.40971288313931,-0.734545151146761,
121.111868793579));
#246130=CARTESIAN_POINT('Ctrl Pts',(-5.76473359089571,-5.3785215151415,
121.323807948012));
#246131=CARTESIAN_POINT('Ctrl Pts',(0.210578624102449,-8.45793363385046,
121.588731891054));
#246132=CARTESIAN_POINT('Ctrl Pts',(7.24465718346336,-4.38210174983432,
121.906640622703));
#246133=CARTESIAN_POINT('Ctrl Pts',(7.52574446095941,2.34979694249055,122.171564565744));
#246134=CARTESIAN_POINT('Ctrl Pts',(4.31380290075385,6.05993236416489,122.383503720177));
#246135=CARTESIAN_POINT('Ctrl Pts',(-0.267155128735916,7.88597403300938,
122.59544287461));
#246136=CARTESIAN_POINT('Ctrl Pts',(-5.24344577943899,5.89366217964708,
122.807382029043));
#246137=CARTESIAN_POINT('Ctrl Pts',(-7.31181929125222,1.40739045105361,
123.019321183476));
#246138=CARTESIAN_POINT('Ctrl Pts',(-7.11128249838525,-2.2607753895711,
123.178275549301));
#246139=CARTESIAN_POINT('Ctrl Pts',(-5.15124451897244,-5.37662361481536,
123.337229915126));
#246140=CARTESIAN_POINT('Ctrl Pts',(-0.881579570788664,-7.83476001695065,
123.549169069559));
#246141=CARTESIAN_POINT('Ctrl Pts',(5.66025141461661,-6.28828582642984,
123.8140930126));
#246142=CARTESIAN_POINT('Ctrl Pts',(8.35326509732775,1.38232979624049,124.13200174425));
#246143=CARTESIAN_POINT('Ctrl Pts',(4.18897518403377,6.67913634163493,124.396925687291));
#246144=CARTESIAN_POINT('Ctrl Pts',(-0.663775530218678,7.40885131246999,
124.608864841724));
#246145=CARTESIAN_POINT('Ctrl Pts',(-5.33127958881593,5.81699374745947,
124.820803996157));
#246146=CARTESIAN_POINT('Ctrl Pts',(-7.81599080145722,1.06736372491064,
125.03274315059));
#246147=CARTESIAN_POINT('Ctrl Pts',(-6.4698006251684,-3.68580101202109,
125.244682305023));
#246148=CARTESIAN_POINT('Ctrl Pts',(-3.93201304567724,-6.34198056939268,
125.403636670848));
#246149=CARTESIAN_POINT('Ctrl Pts',(-0.416765361672836,-7.43435997399531,
125.562591036672));
#246150=CARTESIAN_POINT('Ctrl Pts',(4.42531681375818,-6.52512208013845,
125.774530191105));
#246151=CARTESIAN_POINT('Ctrl Pts',(8.38925281342742,-1.09609394850368,
126.039454134147));
#246152=CARTESIAN_POINT('Ctrl Pts',(5.44677055144542,6.48232705220241,126.357362865796));
#246153=CARTESIAN_POINT('Ctrl Pts',(-1.16127796647469,7.79806442953511,
126.622286808837));
#246154=CARTESIAN_POINT('Ctrl Pts',(-5.32230186203618,5.19661222472599,
126.834225963271));
#246155=CARTESIAN_POINT('Ctrl Pts',(-7.83285712368212,0.952001886600132,
127.046165117703));
#246156=CARTESIAN_POINT('Ctrl Pts',(-6.63168104553608,-4.27197659637739,
127.258104272137));
#246157=CARTESIAN_POINT('Ctrl Pts',(-2.51799050609984,-7.00736562774031,
127.470043426569));
#246158=CARTESIAN_POINT('Ctrl Pts',(1.13722818064386,-7.37483262176709,
127.628997792394));
#246159=CARTESIAN_POINT('Ctrl Pts',(4.5180373349009,-5.91867723651794,127.787952158219));
#246160=CARTESIAN_POINT('Ctrl Pts',(7.60512873288296,-2.07910173371068,
127.999891312652));
#246161=CARTESIAN_POINT('Ctrl Pts',(7.08585380183994,4.62294934111277,128.264815255693));
#246162=CARTESIAN_POINT('Ctrl Pts',(-0.0777831107195537,8.46651186968383,
128.582723987343));
#246163=CARTESIAN_POINT('Ctrl Pts',(-5.95334818308693,5.16875427676112,
128.847647930384));
#246164=CARTESIAN_POINT('Ctrl Pts',(-7.42259652650057,0.486555782601546,
129.059587084817));
#246165=CARTESIAN_POINT('Ctrl Pts',(-6.56947286963103,-4.37058171497872,
129.27152623925));
#246166=CARTESIAN_POINT('Ctrl Pts',(-2.25976996630488,-7.55793736604614,
129.483465393683));
#246167=CARTESIAN_POINT('Ctrl Pts',(2.64412357876513,-6.9607513768183,129.695404548116));
#246168=CARTESIAN_POINT('Ctrl Pts',(5.65984630663675,-4.86287815179347,
129.854358913941));
#246169=CARTESIAN_POINT('Ctrl Pts',(7.28118827550971,-1.55810746937658,
130.013313279766));
#246170=CARTESIAN_POINT('Ctrl Pts',(7.12943939277857,3.36626514224055,130.225252434199));
#246171=CARTESIAN_POINT('Ctrl Pts',(2.37654959055416,8.11991359279997,130.49017637724));
#246172=CARTESIAN_POINT('Ctrl Pts',(-5.56494933743067,6.38116073482492,
130.808085108889));
#246173=CARTESIAN_POINT('Ctrl Pts',(-7.88386634139248,0.0550170443502282,
131.073009051931));
#246174=CARTESIAN_POINT('Ctrl Pts',(-5.95512634391571,-4.45736984669529,
131.284948206364));
#246175=CARTESIAN_POINT('Ctrl Pts',(-2.14838843870147,-7.59238996855304,
131.496887360797));
#246176=CARTESIAN_POINT('Ctrl Pts',(3.19832811286549,-7.21108000285525,
131.70882651523));
#246177=CARTESIAN_POINT('Ctrl Pts',(6.53530624122347,-3.56836398895286,
131.920765669663));
#246178=CARTESIAN_POINT('Ctrl Pts',(7.4619877629195,-0.0135198266309791,
132.079720035487));
#246179=CARTESIAN_POINT('Ctrl Pts',(6.5445440293885,3.55138634553384,132.238674401312));
#246180=CARTESIAN_POINT('Ctrl Pts',(3.2268948945583,7.19359413201327,132.450613555745));
#246181=CARTESIAN_POINT('Ctrl Pts',(-3.47507323660292,7.71393872222958,
132.715537498787));
#246182=CARTESIAN_POINT('Ctrl Pts',(-8.37725229600153,1.22862405323487,
133.033446230436));
#246183=CARTESIAN_POINT('Ctrl Pts',(-6.02490452661707,-5.08516486360561,
133.298370173477));
#246184=CARTESIAN_POINT('Ctrl Pts',(-1.62524935270184,-7.25880426488761,
133.51030932791));
#246185=CARTESIAN_POINT('Ctrl Pts',(3.30534591134366,-7.16482014032892,
133.722248482344));
#246186=CARTESIAN_POINT('Ctrl Pts',(7.11910964228672,-3.39812562053916,
133.934187636776));
#246187=CARTESIAN_POINT('Ctrl Pts',(7.28521099408995,1.53920233165873,134.146126791209));
#246188=CARTESIAN_POINT('Ctrl Pts',(5.67743121364578,4.84233765036753,134.305081157034));
#246189=CARTESIAN_POINT('Ctrl Pts',(2.66218062382144,6.95386018813151,134.464035522859));
#246190=CARTESIAN_POINT('Ctrl Pts',(-2.22669452000353,7.56323383563218,
134.675974677292));
#246191=CARTESIAN_POINT('Ctrl Pts',(-7.65636419437899,3.60015618240601,
134.940898620333));
#246192=CARTESIAN_POINT('Ctrl Pts',(-7.16291254803651,-4.51445667965736,
135.258807351983));
#246193=CARTESIAN_POINT('Ctrl Pts',(-1.27001379708206,-7.78111415223867,
135.523731295024));
#246194=CARTESIAN_POINT('Ctrl Pts',(3.48584772319138,-6.57118115194385,
135.735670449457));
#246195=CARTESIAN_POINT('Ctrl Pts',(7.17026361016127,-3.29344432097186,
135.94760960389));
#246196=CARTESIAN_POINT('Ctrl Pts',(7.61812385785892,2.04829339595507,136.159548758323));
#246197=CARTESIAN_POINT('Ctrl Pts',(4.53323533980309,5.90679245446073,136.371487912756));
#246198=CARTESIAN_POINT('Ctrl Pts',(1.16426115636376,7.37095385983623,136.530442278581));
#246199=CARTESIAN_POINT('Ctrl Pts',(-2.50036914776536,7.01334512305659,
136.689396644406));
#246200=CARTESIAN_POINT('Ctrl Pts',(-6.6087513813229,4.29865066804881,136.901335798838));
#246201=CARTESIAN_POINT('Ctrl Pts',(-8.16010007421704,-2.24644782679431,
137.16625974188));
#246202=CARTESIAN_POINT('Ctrl Pts',(-2.50113137324256,-8.08348055054976,
137.484168473529));
#246203=CARTESIAN_POINT('Ctrl Pts',(4.08776845207816,-6.74390741787467,
137.749092416571));
#246204=CARTESIAN_POINT('Ctrl Pts',(6.93159571519058,-2.71569652585027,
137.961031571004));
#246205=CARTESIAN_POINT('Ctrl Pts',(7.40334174710716,0.922285299287664,
138.119985936828));
#246206=CARTESIAN_POINT('Ctrl Pts',(6.04702995925678,4.36403597153456,138.279005072222));
#246207=CARTESIAN_POINT('Ctrl Pts',(4.16396134314499,5.93645191893425,138.385039419009));
#246208=CARTESIAN_POINT('Ctrl Pts',(3.08878933661219,6.45122224576104,138.438088977186));
#246209=CARTESIAN_POINT('Ctrl Pts',(3.92320494081329,-5.50525709974226,
8.0038671538841));
#246210=CARTESIAN_POINT('Ctrl Pts',(4.84016051734621,-4.85181479700849,
8.05688452237381));
#246211=CARTESIAN_POINT('Ctrl Pts',(6.33798051091494,-3.08289948015477,
8.16288667947178));
#246212=CARTESIAN_POINT('Ctrl Pts',(7.04300948471557,0.34095441748302,8.32187362517801));
#246213=CARTESIAN_POINT('Ctrl Pts',(6.01420291001966,3.65197858249371,8.48082799100276));
#246214=CARTESIAN_POINT('Ctrl Pts',(2.71341797368867,6.94195862936583,8.6927671454358));
#246215=CARTESIAN_POINT('Ctrl Pts',(-3.63885434763407,7.12154028903951,
8.95769108847704));
#246216=CARTESIAN_POINT('Ctrl Pts',(-7.96224185718031,0.769392088592678,
9.2755998201266));
#246217=CARTESIAN_POINT('Ctrl Pts',(-5.45706751038434,-5.07361335315654,
9.54052376316782));
#246218=CARTESIAN_POINT('Ctrl Pts',(-1.19166322865416,-6.93560061915194,
9.75246291760087));
#246219=CARTESIAN_POINT('Ctrl Pts',(2.27857359250251,-6.67472132479364,
9.9114172834256));
#246220=CARTESIAN_POINT('Ctrl Pts',(5.17829028007211,-4.76543010856528,
10.0703716492504));
#246221=CARTESIAN_POINT('Ctrl Pts',(7.42547444076233,-0.672711200711117,
10.2823108036834));
#246222=CARTESIAN_POINT('Ctrl Pts',(6.1428106404885,4.22861967768184,10.4942499581164));
#246223=CARTESIAN_POINT('Ctrl Pts',(2.18093601810749,6.6835833434735,10.7061891125494));
#246224=CARTESIAN_POINT('Ctrl Pts',(-2.44351173292077,7.03950064603549,
10.9181282669824));
#246225=CARTESIAN_POINT('Ctrl Pts',(-7.40125721739437,3.04282371117337,
11.1830522100237));
#246226=CARTESIAN_POINT('Ctrl Pts',(-6.54573505154432,-4.59298539844305,
11.5009609416732));
#246227=CARTESIAN_POINT('Ctrl Pts',(-0.847722772654031,-7.40327450707869,
11.7658848847145));
#246228=CARTESIAN_POINT('Ctrl Pts',(3.60575578158385,-6.0436066569362,11.9778240391475));
#246229=CARTESIAN_POINT('Ctrl Pts',(6.07119951744335,-3.58885319509753,
12.1367784049723));
#246230=CARTESIAN_POINT('Ctrl Pts',(7.03298623857799,-0.252625367839518,
12.295732770797));
#246231=CARTESIAN_POINT('Ctrl Pts',(6.07821522657084,4.31780302708026,12.5076719252301));
#246232=CARTESIAN_POINT('Ctrl Pts',(1.91666268563073,7.20709378759929,12.719611079663));
#246233=CARTESIAN_POINT('Ctrl Pts',(-2.68964418527962,6.49558992266904,
12.9315502340961));
#246234=CARTESIAN_POINT('Ctrl Pts',(-6.4340967659524,3.75865043672924,13.1434893885291));
#246235=CARTESIAN_POINT('Ctrl Pts',(-7.60129628069631,-2.50157786640446,
13.4084133315703));
#246236=CARTESIAN_POINT('Ctrl Pts',(-1.98571650717331,-7.74590505994148,
13.7263220632199));
#246237=CARTESIAN_POINT('Ctrl Pts',(4.17043359165409,-6.17531914645662,
13.9912460062611));
#246238=CARTESIAN_POINT('Ctrl Pts',(6.6694011530727,-2.24627829536837,14.2031851606941));
#246239=CARTESIAN_POINT('Ctrl Pts',(6.94596741139484,1.22182413023957,14.3621395265189));
#246240=CARTESIAN_POINT('Ctrl Pts',(5.50702470161187,4.3817119329183,14.5210938923437));
#246241=CARTESIAN_POINT('Ctrl Pts',(1.80951755333021,7.23282569158136,14.7330330467767));
#246242=CARTESIAN_POINT('Ctrl Pts',(-3.2308185920246,6.72142894914833,14.9449722012097));
#246243=CARTESIAN_POINT('Ctrl Pts',(-6.26738760209476,3.18539287105005,
15.1569113556427));
#246244=CARTESIAN_POINT('Ctrl Pts',(-7.33207086718258,-1.32883042973204,
15.3688505100757));
#246245=CARTESIAN_POINT('Ctrl Pts',(-4.14766486694815,-6.84357168727062,
15.633774453117));
#246246=CARTESIAN_POINT('Ctrl Pts',(3.52875528848565,-7.17565338129885,
15.9516831847665));
#246247=CARTESIAN_POINT('Ctrl Pts',(7.18402146978472,-1.97912058890141,
16.2166071278078));
#246248=CARTESIAN_POINT('Ctrl Pts',(6.52731310302662,2.63075305397933,16.4285462822408));
#246249=CARTESIAN_POINT('Ctrl Pts',(4.4820690634196,5.44521573247064,16.5875006480655));
#246250=CARTESIAN_POINT('Ctrl Pts',(1.33404174694253,6.90992425063454,16.7464550138903));
#246251=CARTESIAN_POINT('Ctrl Pts',(-3.32894729586721,6.67129906135416,
16.9583941683233));
#246252=CARTESIAN_POINT('Ctrl Pts',(-6.82536622599997,3.00502442063848,
17.1703333227564));
#246253=CARTESIAN_POINT('Ctrl Pts',(-6.83263188498128,-1.65590356738068,
17.3822724771893));
#246254=CARTESIAN_POINT('Ctrl Pts',(-4.70579246834758,-5.77759212439439,
17.5942116316224));
#246255=CARTESIAN_POINT('Ctrl Pts',(1.29959412076021,-7.89611628641483,
17.8591355746636));
#246256=CARTESIAN_POINT('Ctrl Pts',(7.34708623381123,-3.15633319028242,
18.1770443063132));
#246257=CARTESIAN_POINT('Ctrl Pts',(6.74451862507508,3.16836729238686,18.4419682493544));
#246258=CARTESIAN_POINT('Ctrl Pts',(3.24778949712727,6.24327969567209,18.6539074037875));
#246259=CARTESIAN_POINT('Ctrl Pts',(-0.136192434304023,7.05129556062135,
18.8128617696122));
#246260=CARTESIAN_POINT('Ctrl Pts',(-3.48016523744545,6.11679413190897,
18.971816135437));
#246261=CARTESIAN_POINT('Ctrl Pts',(-6.86731154651915,2.90312820725449,
19.1837552898699));
#246262=CARTESIAN_POINT('Ctrl Pts',(-7.13921530672556,-2.15578308089093,
19.395694444303));
#246263=CARTESIAN_POINT('Ctrl Pts',(-4.11368528329232,-5.70126902453786,
19.607633598736));
#246264=CARTESIAN_POINT('Ctrl Pts',(0.182384564579414,-7.44928113186926,
19.819572753169));
#246265=CARTESIAN_POINT('Ctrl Pts',(6.12218676667009,-5.15329278047616,
20.0844966962103));
#246266=CARTESIAN_POINT('Ctrl Pts',(7.63394730886059,2.38011844677504,20.4024054278598));
#246267=CARTESIAN_POINT('Ctrl Pts',(3.06317764812811,6.79293938435044,20.6673293709011));
#246268=CARTESIAN_POINT('Ctrl Pts',(-1.59282518475065,6.85489503251987,
20.8792685253341));
#246269=CARTESIAN_POINT('Ctrl Pts',(-4.6889913169139,5.26808104458408,21.0382228911588));
#246270=CARTESIAN_POINT('Ctrl Pts',(-6.62158680890006,2.38354959341743,
21.1971772569836));
#246271=CARTESIAN_POINT('Ctrl Pts',(-7.10481569504033,-2.26046791709614,
21.4091164114166));
#246272=CARTESIAN_POINT('Ctrl Pts',(-4.02151030593889,-6.2803861940861,
21.6210555658497));
#246273=CARTESIAN_POINT('Ctrl Pts',(0.582556149475053,-7.00624745729406,
21.8329947202826));
#246274=CARTESIAN_POINT('Ctrl Pts',(4.98289615108128,-5.54037899954143,
22.0449338747157));
#246275=CARTESIAN_POINT('Ctrl Pts',(8.00207295474845,0.0665260413783972,
22.3098578177569));
#246276=CARTESIAN_POINT('Ctrl Pts',(4.25145511183555,6.77253606614142,22.6277665494065));
#246277=CARTESIAN_POINT('Ctrl Pts',(-2.09051838595393,7.15239929404389,
22.8926904924477));
#246278=CARTESIAN_POINT('Ctrl Pts',(-5.66782830722953,4.17161842164514,
23.1046296468807));
#246279=CARTESIAN_POINT('Ctrl Pts',(-6.98796725114217,0.952696782488859,
23.2635840127055));
#246280=CARTESIAN_POINT('Ctrl Pts',(-6.58025897948308,-2.49537818677088,
23.4225383785302));
#246281=CARTESIAN_POINT('Ctrl Pts',(-3.92730037023841,-6.33754156330653,
23.6344775329633));
#246282=CARTESIAN_POINT('Ctrl Pts',(1.02918445790915,-7.38624229491818,
23.8464166873963));
#246283=CARTESIAN_POINT('Ctrl Pts',(4.99878460510776,-4.94358448616671,
24.0583558418293));
#246284=CARTESIAN_POINT('Ctrl Pts',(7.38831571551028,-0.968423667081756,
24.2702949962623));
#246285=CARTESIAN_POINT('Ctrl Pts',(6.03566162570836,5.25436828051194,24.5352189393036));
#246286=CARTESIAN_POINT('Ctrl Pts',(-1.17455272585738,7.90964861604609,
24.8531276709531));
#246287=CARTESIAN_POINT('Ctrl Pts',(-6.23938033231202,4.07396807206546,
25.1180516139943));
#246288=CARTESIAN_POINT('Ctrl Pts',(-7.01851810879394,-0.516799315569627,
25.3299907684274));
#246289=CARTESIAN_POINT('Ctrl Pts',(-5.9280883936475,-3.82061323081804,
25.4889451342521));
#246290=CARTESIAN_POINT('Ctrl Pts',(-3.37604649281442,-6.17487089828082,
25.6478995000769));
#246291=CARTESIAN_POINT('Ctrl Pts',(1.13792152115551,-7.36839574645685,
25.8598386545099));
#246292=CARTESIAN_POINT('Ctrl Pts',(5.5851887025007,-4.94180766978019,26.0717778089429));
#246293=CARTESIAN_POINT('Ctrl Pts',(7.01228405239937,-0.504725141632746,
26.283716963376));
#246294=CARTESIAN_POINT('Ctrl Pts',(6.24244793815225,4.06901674246726,26.4956561178089));
#246295=CARTESIAN_POINT('Ctrl Pts',(1.16813324157401,7.91663198697703,26.7605800608503));
#246296=CARTESIAN_POINT('Ctrl Pts',(-6.03599694875479,5.24488857553349,
27.0784887924997));
#246297=CARTESIAN_POINT('Ctrl Pts',(-7.38920525210955,-0.962667401363433,
27.3434127355411));
#246298=CARTESIAN_POINT('Ctrl Pts',(-4.9956684627223,-4.95681092907559,
27.555351889974));
#246299=CARTESIAN_POINT('Ctrl Pts',(-2.01879891484442,-6.75749719969035,
27.7143062557988));
#246300=CARTESIAN_POINT('Ctrl Pts',(1.45090541605391,-6.88633385813854,
27.8732606216235));
#246301=CARTESIAN_POINT('Ctrl Pts',(5.65618704933612,-4.85753737274708,
28.0851997760566));
#246302=CARTESIAN_POINT('Ctrl Pts',(7.45660139680916,-0.122030720491899,
28.2971389304895));
#246303=CARTESIAN_POINT('Ctrl Pts',(5.65524053006352,4.17673672228185,28.5090780849226));
#246304=CARTESIAN_POINT('Ctrl Pts',(2.09606865070999,7.15063281972518,28.7210172393556));
#246305=CARTESIAN_POINT('Ctrl Pts',(-4.2608731510886,6.77366645751254,28.9859411823969));
#246306=CARTESIAN_POINT('Ctrl Pts',(-7.996162939297,0.0591065423799839,
29.3038499140464));
#246307=CARTESIAN_POINT('Ctrl Pts',(-4.98731526310924,-5.53658461958353,
29.5687738570877));
#246308=CARTESIAN_POINT('Ctrl Pts',(-0.571587621537175,-7.01426871219993,
29.7807130115207));
#246309=CARTESIAN_POINT('Ctrl Pts',(2.86085178131299,-6.44630472036177,
29.9396673773454));
#246310=CARTESIAN_POINT('Ctrl Pts',(5.58046129630571,-4.28779340133288,
30.0986217431702));
#246311=CARTESIAN_POINT('Ctrl Pts',(7.45573477436185,-0.0118422583874216,
30.3105608976032));
#246312=CARTESIAN_POINT('Ctrl Pts',(5.74390437343873,4.7564018371487,30.5225000520362));
#246313=CARTESIAN_POINT('Ctrl Pts',(1.57993416102576,6.85059728395666,30.7344392064692));
#246314=CARTESIAN_POINT('Ctrl Pts',(-3.05781252937014,6.79520684352195,
30.9463783609023));
#246315=CARTESIAN_POINT('Ctrl Pts',(-7.64183700346619,2.37485252168492,
31.2113023039435));
#246316=CARTESIAN_POINT('Ctrl Pts',(-6.11287213635388,-5.15508579751365,
31.529211035593));
#246317=CARTESIAN_POINT('Ctrl Pts',(-0.188209149979401,-7.4492724543619,
31.7941349786343));
#246318=CARTESIAN_POINT('Ctrl Pts',(4.12723403517989,-5.70022957387632,
32.0060741330673));
#246319=CARTESIAN_POINT('Ctrl Pts',(6.3653979057508,-3.03661439169733,32.1650284988921));
#246320=CARTESIAN_POINT('Ctrl Pts',(7.02769791381951,0.37172915432722,32.3239828647168));
#246321=CARTESIAN_POINT('Ctrl Pts',(5.67158933474266,4.83954498716,32.5359220191499));
#246322=CARTESIAN_POINT('Ctrl Pts',(1.27032710627931,7.34860972774388,32.7478611735828));
#246323=CARTESIAN_POINT('Ctrl Pts',(-3.25478753390679,6.23163166508225,
32.9598003280159));
#246324=CARTESIAN_POINT('Ctrl Pts',(-6.7419174644648,3.17357880213563,33.1717394824488));
#246325=CARTESIAN_POINT('Ctrl Pts',(-7.3496553023264,-3.16546429837453,
33.4366634254902));
#246326=CARTESIAN_POINT('Ctrl Pts',(-1.2913520703836,-7.89142098518733,
33.7545721571396));
#246327=CARTESIAN_POINT('Ctrl Pts',(4.70136207017436,-5.78137332029135,
34.019496100181));
#246328=CARTESIAN_POINT('Ctrl Pts',(6.84224848195906,-1.64630303625135,
34.2314352546139));
#246329=CARTESIAN_POINT('Ctrl Pts',(6.81033506401044,1.83266302912182,34.3903896204387));
#246330=CARTESIAN_POINT('Ctrl Pts',(5.09698269437306,4.85257539306103,34.5493439862634));
#246331=CARTESIAN_POINT('Ctrl Pts',(1.16132278879302,7.36474375962547,34.7612831406965));
#246332=CARTESIAN_POINT('Ctrl Pts',(-3.81384894227602,6.40861546148153,
34.9732222951295));
#246333=CARTESIAN_POINT('Ctrl Pts',(-6.52505445803083,2.61735351449946,
35.1851614495625));
#246334=CARTESIAN_POINT('Ctrl Pts',(-7.18543454803273,-1.97347000660205,
35.3971006039956));
#246335=CARTESIAN_POINT('Ctrl Pts',(-3.52476887568925,-7.18426068988804,
35.6620245470368));
#246336=CARTESIAN_POINT('Ctrl Pts',(4.15087269174857,-6.83464492362513,
35.9799332786863));
#246337=CARTESIAN_POINT('Ctrl Pts',(7.33116418301752,-1.33458401949517,
36.2448572217275));
#246338=CARTESIAN_POINT('Ctrl Pts',(6.26844970540344,3.19893986609144,36.4567963761606));
#246339=CARTESIAN_POINT('Ctrl Pts',(3.98179858667866,5.82104779893825,36.6157507419853));
#246340=CARTESIAN_POINT('Ctrl Pts',(0.716338313692228,7.0009699294038,36.7747051078101));
#246341=CARTESIAN_POINT('Ctrl Pts',(-3.90714823546713,6.34998534886486,
36.9866442622431));
#246342=CARTESIAN_POINT('Ctrl Pts',(-7.0648502871895,2.38823916458096,37.1985834166761));
#246343=CARTESIAN_POINT('Ctrl Pts',(-6.65897147596041,-2.25498868788211,
37.4105225711092));
#246344=CARTESIAN_POINT('Ctrl Pts',(-4.17518168751194,-6.17194551071909,
37.6224617255421));
#246345=CARTESIAN_POINT('Ctrl Pts',(1.9943422664243,-7.74985136706838,37.8873856685834));
#246346=CARTESIAN_POINT('Ctrl Pts',(7.59792802485505,-2.49271038515526,
38.205294400233));
#246347=CARTESIAN_POINT('Ctrl Pts',(6.43714956059893,3.75368996028338,38.4702183432742));
#246348=CARTESIAN_POINT('Ctrl Pts',(2.68164134065499,6.50657188511213,38.6821574977073));
#246349=CARTESIAN_POINT('Ctrl Pts',(-0.760639713870074,7.01147236235613,
38.841111863532));
#246350=CARTESIAN_POINT('Ctrl Pts',(-4.00862313244799,5.78425977235483,
39.0000662293568));
#246351=CARTESIAN_POINT('Ctrl Pts',(-7.09759907144927,2.28302621221805,
39.2120053837898));
#246352=CARTESIAN_POINT('Ctrl Pts',(-6.92004203725226,-2.78007447567538,
39.4239445382228));
#246353=CARTESIAN_POINT('Ctrl Pts',(-3.59216968022922,-6.04344207290618,
39.6358836926558));
#246354=CARTESIAN_POINT('Ctrl Pts',(0.84192502812979,-7.40379738769429,
39.8478228470888));
#246355=CARTESIAN_POINT('Ctrl Pts',(6.55484758839465,-4.59037802149398,
40.1127467901301));
#246356=CARTESIAN_POINT('Ctrl Pts',(7.39294321005172,3.04737690942376,40.4306555217796));
#246357=CARTESIAN_POINT('Ctrl Pts',(2.44903763211165,7.03770541156364,40.6955794648208));
#246358=CARTESIAN_POINT('Ctrl Pts',(-2.19413183217394,6.68673788024343,
40.9075186192539));
#246359=CARTESIAN_POINT('Ctrl Pts',(-5.13746692096526,4.83174410522615,
41.0664729850786));
#246360=CARTESIAN_POINT('Ctrl Pts',(-6.80678919836751,1.78727203890934,
41.2254273509034));
#246361=CARTESIAN_POINT('Ctrl Pts',(-6.8764991954602,-2.88129833227098,
41.4373665053365));
#246362=CARTESIAN_POINT('Ctrl Pts',(-3.44902810826724,-6.61211017724467,
41.6493056597694));
#246363=CARTESIAN_POINT('Ctrl Pts',(1.20125387967055,-6.92703863254039,
41.8612448142025));
#246364=CARTESIAN_POINT('Ctrl Pts',(5.4543498365197,-5.07692046144884,42.0731839686354));
#246365=CARTESIAN_POINT('Ctrl Pts',(7.96468255945656,0.775518545482133,
42.3381079116768));
#246366=CARTESIAN_POINT('Ctrl Pts',(3.63444678971545,7.12270397165751,42.6560166433262));
#246367=CARTESIAN_POINT('Ctrl Pts',(-2.71623519168221,6.93895879559161,
42.9209405863675));
#246368=CARTESIAN_POINT('Ctrl Pts',(-6.01526780461176,3.65283878850994,
43.1328797408005));
#246369=CARTESIAN_POINT('Ctrl Pts',(-7.0449057115676,0.329576967523976,
43.2918341066252));
#246370=CARTESIAN_POINT('Ctrl Pts',(-6.33318599383895,-3.06879059232167,
43.4507884724501));
#246371=CARTESIAN_POINT('Ctrl Pts',(-3.35012305774061,-6.66069041186473,
43.6627276268829));
#246372=CARTESIAN_POINT('Ctrl Pts',(1.67980477892008,-7.26595154073829,
43.8746667813162));
#246373=CARTESIAN_POINT('Ctrl Pts',(5.41727957767459,-4.48106651116011,
44.086605935749));
#246374=CARTESIAN_POINT('Ctrl Pts',(7.44507244944886,-0.309757539823755,
44.2985450901822));
#246375=CARTESIAN_POINT('Ctrl Pts',(5.54619217953605,5.76865232051224,44.5634690332233));
#246376=CARTESIAN_POINT('Ctrl Pts',(-1.8709924218742,7.77441333429271,44.8813777648729));
#246377=CARTESIAN_POINT('Ctrl Pts',(-6.57591523561052,3.50491392155589,
45.1463017079142));
#246378=CARTESIAN_POINT('Ctrl Pts',(-6.94508926985662,-1.13684344118434,
45.3582408623472));
#246379=CARTESIAN_POINT('Ctrl Pts',(-5.56612151970435,-4.33100550568619,
45.5171952281719));
#246380=CARTESIAN_POINT('Ctrl Pts',(-2.81545688577237,-6.44980023383955,
45.6761495939967));
#246381=CARTESIAN_POINT('Ctrl Pts',(1.78653207542118,-7.23853744952694,
45.8880887484297));
#246382=CARTESIAN_POINT('Ctrl Pts',(6.00121826529194,-4.4273214498121,46.1000279028627));
#246383=CARTESIAN_POINT('Ctrl Pts',(7.02942136872401,0.118786872411061,
46.3119670572958));
#246384=CARTESIAN_POINT('Ctrl Pts',(5.85722687898137,4.60629425885479,46.5239062117287));
#246385=CARTESIAN_POINT('Ctrl Pts',(0.461854421036876,7.98901043816237,
46.78883015477));
#246386=CARTESIAN_POINT('Ctrl Pts',(-6.47711547532611,4.68925265414749,
47.1067388864195));
#246387=CARTESIAN_POINT('Ctrl Pts',(-7.27479849768731,-1.61381213327239,
47.3716628294608));
#246388=CARTESIAN_POINT('Ctrl Pts',(-4.53666578708917,-5.38008750043123,
47.5836019838938));
#246389=CARTESIAN_POINT('Ctrl Pts',(-1.41191065999068,-6.90983543585552,
47.7425563497185));
#246390=CARTESIAN_POINT('Ctrl Pts',(2.05555716365124,-6.7306318632831,47.9015107155433));
#246391=CARTESIAN_POINT('Ctrl Pts',(6.06446798360192,-4.33708996224195,
48.1134498699764));
#246392=CARTESIAN_POINT('Ctrl Pts',(7.43807033314036,0.5393566601956,48.3253890244092));
#246393=CARTESIAN_POINT('Ctrl Pts',(5.26278292242774,4.66154384421445,48.5373281788424));
#246394=CARTESIAN_POINT('Ctrl Pts',(1.45403116996541,7.30827249545264,48.7492673332753));
#246395=CARTESIAN_POINT('Ctrl Pts',(-4.84447950307468,6.3693497024098,49.0141912763167));
#246396=CARTESIAN_POINT('Ctrl Pts',(-7.96993110060059,-0.649856589424143,
49.3321000079661));
#246397=CARTESIAN_POINT('Ctrl Pts',(-4.4769579036553,-5.95683898660598,
49.5970239510075));
#246398=CARTESIAN_POINT('Ctrl Pts',(0.0523634526556974,-7.03732449478264,
49.8089631054405));
#246399=CARTESIAN_POINT('Ctrl Pts',(3.42095290591867,-6.16736561895647,
49.9679174712652));
#246400=CARTESIAN_POINT('Ctrl Pts',(5.9385416787833,-3.77630020806522,50.12687183709));
#246401=CARTESIAN_POINT('Ctrl Pts',(7.42744069663569,0.6490346390391,50.338810991523));
#246402=CARTESIAN_POINT('Ctrl Pts',(5.29971987330698,5.24678617366048,50.550750145956));
#246403=CARTESIAN_POINT('Ctrl Pts',(0.966521339459677,6.96367084234314,
50.762689300389));
#246404=CARTESIAN_POINT('Ctrl Pts',(-3.64806300079631,6.49743717578258,
50.974628454822));
#246405=CARTESIAN_POINT('Ctrl Pts',(-7.8222531166543,1.68818051946163,51.2395523978633));
#246406=CARTESIAN_POINT('Ctrl Pts',(-5.63189859724677,-5.67660404867808,
51.5574611295129));
#246407=CARTESIAN_POINT('Ctrl Pts',(0.472789098434964,-7.4366358826994,
51.822385072554));
#246408=CARTESIAN_POINT('Ctrl Pts',(4.61622353697344,-5.31198251434755,
52.0343242269871));
#246409=CARTESIAN_POINT('Ctrl Pts',(6.60949221452337,-2.46047355778412,
52.1932785928118));
#246410=CARTESIAN_POINT('Ctrl Pts',(6.96709106897004,0.993157877055618,
52.3522329586366));
#246411=CARTESIAN_POINT('Ctrl Pts',(5.22032015113918,5.32319253684505,52.5641721130696));
#246412=CARTESIAN_POINT('Ctrl Pts',(0.613992064454545,7.43228158995788,
52.7761112675027));
#246413=CARTESIAN_POINT('Ctrl Pts',(-3.7943109427795,5.91862142476055,52.9880504219356));
#246414=CARTESIAN_POINT('Ctrl Pts',(-6.99666957633073,2.56352654573113,
53.1999895763688));
#246415=CARTESIAN_POINT('Ctrl Pts',(-7.04016189133548,-3.80443396986798,
53.4649135194098));
#246416=CARTESIAN_POINT('Ctrl Pts',(-0.586822842256673,-7.97482001595928,
53.7828222510596));
#246417=CARTESIAN_POINT('Ctrl Pts',(5.19528404400013,-5.34191973784788,
54.0477461941006));
#246418=CARTESIAN_POINT('Ctrl Pts',(6.96123742617008,-1.03336899146948,
54.2596853485338));
#246419=CARTESIAN_POINT('Ctrl Pts',(6.62109554192712,2.42907622092694,54.4186397143584));
#246420=CARTESIAN_POINT('Ctrl Pts',(4.6468200682834,5.28524207440665,54.5775940801833));
#246421=CARTESIAN_POINT('Ctrl Pts',(0.503986736747804,7.43869065319261,
54.7895332346163));
#246422=CARTESIAN_POINT('Ctrl Pts',(-4.36685879143792,6.04535691115763,
55.0014723890493));
#246423=CARTESIAN_POINT('Ctrl Pts',(-6.73135970780785,2.02871180413373,
55.2134115434823));
#246424=CARTESIAN_POINT('Ctrl Pts',(-6.98223847753735,-2.60257552317263,
55.4253506979153));
#246425=CARTESIAN_POINT('Ctrl Pts',(-2.87412786071058,-7.46839918105518,
55.6902746409566));
#246426=CARTESIAN_POINT('Ctrl Pts',(4.74031672968744,-6.43983793564593,
56.0081833726062));
#246427=CARTESIAN_POINT('Ctrl Pts',(7.42060004203954,-0.679542345651922,
56.2731073156473));
#246428=CARTESIAN_POINT('Ctrl Pts',(5.96024455189898,3.7419463996161,56.4850464700805));
#246429=CARTESIAN_POINT('Ctrl Pts',(3.45018560213969,6.15105980894251,56.6440008359051));
#246430=CARTESIAN_POINT('Ctrl Pts',(0.0929962629414194,7.03690785978889,
56.80295520173));
#246431=CARTESIAN_POINT('Ctrl Pts',(-4.45459427338222,5.97868807718401,
57.0148943561628));
#246432=CARTESIAN_POINT('Ctrl Pts',(-7.24872376928388,1.75265501575725,
57.226833510596));
#246433=CARTESIAN_POINT('Ctrl Pts',(-6.43289534050361,-2.83632378938966,
57.438772665029));
#246434=CARTESIAN_POINT('Ctrl Pts',(-3.61170619446961,-6.51771676861232,
57.6507118194619));
#246435=CARTESIAN_POINT('Ctrl Pts',(2.67339205701473,-7.54258392043396,
57.9156357625032));
#246436=CARTESIAN_POINT('Ctrl Pts',(7.78896314481361,-1.80946634781474,
58.2335444941528));
#246437=CARTESIAN_POINT('Ctrl Pts',(6.07911082865066,4.30946566483981,58.498468437194));
#246438=CARTESIAN_POINT('Ctrl Pts',(2.09438479238119,6.71864795308429,58.7104075916271));
#246439=CARTESIAN_POINT('Ctrl Pts',(-1.37909965991125,6.91645874638408,
58.8693619574518));
#246440=CARTESIAN_POINT('Ctrl Pts',(-4.50552737171663,5.40619493126099,
59.0283163232766));
#246441=CARTESIAN_POINT('Ctrl Pts',(-7.2720182370356,1.64495350236227,59.2402554777095));
#246442=CARTESIAN_POINT('Ctrl Pts',(-6.64639803882978,-3.38248266766881,
59.4521946321427));
#246443=CARTESIAN_POINT('Ctrl Pts',(-3.04237851179562,-6.33804450056128,
59.6641337865756));
#246444=CARTESIAN_POINT('Ctrl Pts',(1.4948383252907,-7.30003506102965,59.8760729410086));
#246445=CARTESIAN_POINT('Ctrl Pts',(6.93591228911752,-3.99133035527843,
60.1409968840499));
#246446=CARTESIAN_POINT('Ctrl Pts',(7.09374596681339,3.69064811292774,60.4589056156994));
#246447=CARTESIAN_POINT('Ctrl Pts',(1.81562015154718,7.22707452907096,60.7238295587406));
#246448=CARTESIAN_POINT('Ctrl Pts',(-2.77816749198367,6.46594643981271,
60.9357687131737));
#246449=CARTESIAN_POINT('Ctrl Pts',(-5.5455032377072,4.35737435882887,61.0947230789984));
#246450=CARTESIAN_POINT('Ctrl Pts',(-6.93841232235609,1.17692607119428,
61.2536774448232));
#246451=CARTESIAN_POINT('Ctrl Pts',(-6.59405471200675,-3.47944876665455,
61.4656165992562));
#246452=CARTESIAN_POINT('Ctrl Pts',(-2.84939707620817,-6.89178730009399,
61.6775557536893));
#246453=CARTESIAN_POINT('Ctrl Pts',(1.81049600625463,-6.79330400552387,
61.8894949081222));
#246454=CARTESIAN_POINT('Ctrl Pts',(5.88286990826912,-4.57349922416107,
62.1014340625553));
#246455=CARTESIAN_POINT('Ctrl Pts',(7.86459860500312,1.47840659815924,62.3663580055965));
#246456=CARTESIAN_POINT('Ctrl Pts',(2.98883012029103,7.41680590599346,62.6842667372461));
#246457=CARTESIAN_POINT('Ctrl Pts',(-3.32057130201977,6.67089866597099,
62.9491906802873));
#246458=CARTESIAN_POINT('Ctrl Pts',(-6.31535845347854,3.10530603646705,
63.1611298347204));
#246459=CARTESIAN_POINT('Ctrl Pts',(-7.04639058552322,-0.296137094349907,
63.3200842005451));
#246460=CARTESIAN_POINT('Ctrl Pts',(-6.03626168420024,-3.61804718210473,
63.4790385663698));
#246461=CARTESIAN_POINT('Ctrl Pts',(-2.74657543650164,-6.93141000347823,
63.6909777208029));
#246462=CARTESIAN_POINT('Ctrl Pts',(2.31720260932942,-7.08846725004475,
63.9029168752358));
#246463=CARTESIAN_POINT('Ctrl Pts',(5.79313273304886,-3.98327606844028,
64.1148560296689));
#246464=CARTESIAN_POINT('Ctrl Pts',(7.44322570652722,0.351346826812141,
64.3267951841019));
#246465=CARTESIAN_POINT('Ctrl Pts',(5.01306618774103,6.23752873216845,64.5917191271432));
#246466=CARTESIAN_POINT('Ctrl Pts',(-2.55270470431066,7.57798218708196,
64.9096278587927));
#246467=CARTESIAN_POINT('Ctrl Pts',(-6.8606881850845,2.9082710345641,65.1745518018339));
#246468=CARTESIAN_POINT('Ctrl Pts',(-6.81699254406192,-1.74793896639902,
65.386490956267));
#246469=CARTESIAN_POINT('Ctrl Pts',(-5.16034122743529,-4.80730650976375,
65.5454453220917));
#246470=CARTESIAN_POINT('Ctrl Pts',(-2.232705565254,-6.67396032284963,65.7043996879165));
#246471=CARTESIAN_POINT('Ctrl Pts',(2.42108004106924,-7.05170140459022,
65.9163388423495));
#246472=CARTESIAN_POINT('Ctrl Pts',(6.3700095697273,-3.87798581341241,66.1282779967825));
#246473=CARTESIAN_POINT('Ctrl Pts',(6.99122698274514,0.74136386214266,66.3402171512155));
#246474=CARTESIAN_POINT('Ctrl Pts',(5.42590098168002,5.10731358423102,66.5521563056486));
#246475=CARTESIAN_POINT('Ctrl Pts',(-0.248059861002422,7.998503834619,66.8170802486897));
#246476=CARTESIAN_POINT('Ctrl Pts',(-6.86724974507664,4.09670553933687,
67.1349889803395));
#246477=CARTESIAN_POINT('Ctrl Pts',(-7.10312856817561,-2.2522538320855,
67.3999129233804));
#246478=CARTESIAN_POINT('Ctrl Pts',(-4.0419529974468,-5.76101500992519,
67.6118520778137));
#246479=CARTESIAN_POINT('Ctrl Pts',(-0.793908627573567,-7.00778328388534,
67.7708064436383));
#246480=CARTESIAN_POINT('Ctrl Pts',(2.64402870512488,-6.52195007099546,
67.9297608094632));
#246481=CARTESIAN_POINT('Ctrl Pts',(6.42501279597442,-3.78250338796736,
68.141699963896));
#246482=CARTESIAN_POINT('Ctrl Pts',(7.36099090340974,1.19649852563351,68.3536391183292));
#246483=CARTESIAN_POINT('Ctrl Pts',(4.82889961647785,5.10965787997891,68.5655782727621));
#246484=CARTESIAN_POINT('Ctrl Pts',(0.800548346787644,7.40838551015447,
68.7775174271952));
#246485=CARTESIAN_POINT('Ctrl Pts',(-5.38995276726831,5.91489695725373,
69.0424413702364));
#246486=CARTESIAN_POINT('Ctrl Pts',(-7.88096445044827,-1.3537044013919,
69.3603501018861));
#246487=CARTESIAN_POINT('Ctrl Pts',(-3.93136031333972,-6.33020444052113,
69.6252740449271));
#246488=CARTESIAN_POINT('Ctrl Pts',(0.675902207055709,-7.00498634360421,
69.8372131993604));
#246489=CARTESIAN_POINT('Ctrl Pts',(3.95412650214858,-5.83988048839313,
69.9961675651849));
#246490=CARTESIAN_POINT('Ctrl Pts',(6.24987657364358,-3.23508198497481,
70.1551219310099));
#246491=CARTESIAN_POINT('Ctrl Pts',(7.34068326321575,1.304802488117,70.3670610854427));
#246492=CARTESIAN_POINT('Ctrl Pts',(4.81381636314329,5.69587112126037,70.5790002398758));
#246493=CARTESIAN_POINT('Ctrl Pts',(0.345503588642198,7.02192978372834,
70.7909393943088));
#246494=CARTESIAN_POINT('Ctrl Pts',(-4.20960493843672,6.14852438048371,
71.0028785487418));
#246495=CARTESIAN_POINT('Ctrl Pts',(-7.94108190916835,0.988217775774724,
71.2678024917831));
#246496=CARTESIAN_POINT('Ctrl Pts',(-5.1066201271287,-6.15343513092807,
71.5857112234327));
#246497=CARTESIAN_POINT('Ctrl Pts',(1.13011026506829,-7.36546917451868,
71.8506351664738));
#246498=CARTESIAN_POINT('Ctrl Pts',(5.06881513876091,-4.88191287851589,
72.0625743209069));
#246499=CARTESIAN_POINT('Ctrl Pts',(6.80169453611394,-1.86498618130522,
72.2215286867317));
#246500=CARTESIAN_POINT('Ctrl Pts',(6.85139287777893,1.60680804324508,72.3804830525564));
#246501=CARTESIAN_POINT('Ctrl Pts',(4.72853054649915,5.76484981644271,72.5924222069894));
#246502=CARTESIAN_POINT('Ctrl Pts',(-0.0482709114308084,7.45762139668047,
72.8043613614224));
#246503=CARTESIAN_POINT('Ctrl Pts',(-4.30268773290715,5.55882356982419,
73.0163005158555));
#246504=CARTESIAN_POINT('Ctrl Pts',(-7.19933741305753,1.93376040999748,
73.2282396702885));
#246505=CARTESIAN_POINT('Ctrl Pts',(-6.66892985464963,-4.41442550065097,
73.4931636133297));
#246506=CARTESIAN_POINT('Ctrl Pts',(0.11140474583598,-7.99385296845655,
73.8110723449793));
#246507=CARTESIAN_POINT('Ctrl Pts',(6.77623611831373,-4.23606055317877,
74.1289810766287));
#246508=CARTESIAN_POINT('Ctrl Pts',(7.23272290008192,3.40636727273015,74.4468898082783));
#246509=CARTESIAN_POINT('Ctrl Pts',(1.05018349857864,7.92203885124593,74.7647985399278));
#246510=CARTESIAN_POINT('Ctrl Pts',(-6.09176467475394,5.17730619590121,
75.0827072715773));
#246511=CARTESIAN_POINT('Ctrl Pts',(-7.65077828618112,-2.32967154825181,
75.4006160032269));
#246512=CARTESIAN_POINT('Ctrl Pts',(-3.09458166954053,-6.78184730002577,
75.6655399462681));
#246513=CARTESIAN_POINT('Ctrl Pts',(1.54502232785923,-6.85759048163122,
75.8774791007012));
#246514=CARTESIAN_POINT('Ctrl Pts',(5.71857739349959,-4.7870992857546,76.0894182551341));
#246515=CARTESIAN_POINT('Ctrl Pts',(7.45599088236389,-0.0263533189910901,
76.3013574095672));
#246516=CARTESIAN_POINT('Ctrl Pts',(5.60250882051894,4.25855742822898,76.5132965640002));
#246517=CARTESIAN_POINT('Ctrl Pts',(2.89433645153631,6.43148804899533,76.6722509298249));
#246518=CARTESIAN_POINT('Ctrl Pts',(-0.535210393094977,7.01708700954135,
76.8312052956498));
#246519=CARTESIAN_POINT('Ctrl Pts',(-4.95849240896067,5.5624309795518,77.0431444500826));
#246520=CARTESIAN_POINT('Ctrl Pts',(-7.99637556395713,-0.0176316047177856,
77.3080683931241));
#246521=CARTESIAN_POINT('Ctrl Pts',(-4.29596078342121,-6.75145000779716,
77.6259771247734));
#246522=CARTESIAN_POINT('Ctrl Pts',(2.05892780076842,-7.16142039726313,
77.8909010678148));
#246523=CARTESIAN_POINT('Ctrl Pts',(5.63349027720521,-4.20602638056516,
78.1028402222478));
#246524=CARTESIAN_POINT('Ctrl Pts',(7.45713295591053,0.0833299822800066,
78.3147793766808));
#246525=CARTESIAN_POINT('Ctrl Pts',(5.68132030650631,4.82811970426699,78.5267185311138));
#246526=CARTESIAN_POINT('Ctrl Pts',(1.48662297777303,6.87871098079028,78.7386576855468));
#246527=CARTESIAN_POINT('Ctrl Pts',(-1.98370277785666,6.76788325865866,
78.8976120513716));
#246528=CARTESIAN_POINT('Ctrl Pts',(-4.96987733848888,4.98266963664653,
79.0565664171964));
#246529=CARTESIAN_POINT('Ctrl Pts',(-7.38410982404283,1.00100163764598,
79.2685055716293));
#246530=CARTESIAN_POINT('Ctrl Pts',(-6.06313463638398,-5.21349351746575,
79.5334295146707));
#246531=CARTESIAN_POINT('Ctrl Pts',(1.12703327978956,-7.92258750879785,
79.85133824632));
#246532=CARTESIAN_POINT('Ctrl Pts',(6.22124724940058,-4.1013578464256,80.1162621893616));
#246533=CARTESIAN_POINT('Ctrl Pts',(7.01480895542049,0.468327316524474,
80.3282013437944));
#246534=CARTESIAN_POINT('Ctrl Pts',(5.6107595536581,4.91275615443702,80.5401404982275));
#246535=CARTESIAN_POINT('Ctrl Pts',(1.1761453154345,7.3623911540614,80.7520796526603));
#246536=CARTESIAN_POINT('Ctrl Pts',(-3.34395584622964,6.19230811737825,
80.9640188070936));
#246537=CARTESIAN_POINT('Ctrl Pts',(-5.90818106404349,3.85132626212272,
81.1229731729182));
#246538=CARTESIAN_POINT('Ctrl Pts',(-7.01574160870034,0.553215742819636,
81.2819275387429));
#246539=CARTESIAN_POINT('Ctrl Pts',(-6.26043862608513,-4.04153324732057,
81.4938666931761));
#246540=CARTESIAN_POINT('Ctrl Pts',(-1.21558491778668,-7.90344663073891,
81.7587906362172));
#246541=CARTESIAN_POINT('Ctrl Pts',(6.0083122153089,-5.28562026733149,82.0766993678669));
#246542=CARTESIAN_POINT('Ctrl Pts',(7.39324196671269,0.930068133152367,
82.341623310908));
#246543=CARTESIAN_POINT('Ctrl Pts',(5.02437257694055,4.91757616193617,82.5535624653411));
#246544=CARTESIAN_POINT('Ctrl Pts',(1.06750233150316,7.38080176265968,82.7655016197742));
#246545=CARTESIAN_POINT('Ctrl Pts',(-3.89435810203002,6.35783738687267,
82.9774407742069));
#246546=CARTESIAN_POINT('Ctrl Pts',(-6.56722032392826,2.52949357561374,
83.1893799286403));
#246547=CARTESIAN_POINT('Ctrl Pts',(-6.9928172770757,-0.91641911362483,
83.3483342944647));
#246548=CARTESIAN_POINT('Ctrl Pts',(-5.68940106516124,-4.1421484154716,
83.5072886602898));
#246549=CARTESIAN_POINT('Ctrl Pts',(-2.1276084130189,-7.14145399931232,
83.7192278147225));
#246550=CARTESIAN_POINT('Ctrl Pts',(4.21625102576613,-6.7945082693943,83.984151757764));
#246551=CARTESIAN_POINT('Ctrl Pts',(8.00161995345922,-0.108052800533174,
84.3020604894134));
#246552=CARTESIAN_POINT('Ctrl Pts',(5.01158146891714,5.51444509369941,84.5669844324547));
#246553=CARTESIAN_POINT('Ctrl Pts',(0.618908011605294,7.00312986980119,
84.7789235868877));
#246554=CARTESIAN_POINT('Ctrl Pts',(-3.98886338328963,6.30117170033406,
84.9908627413207));
#246555=CARTESIAN_POINT('Ctrl Pts',(-7.09298906892491,2.29730871517607,
85.2028018957538));
#246556=CARTESIAN_POINT('Ctrl Pts',(-6.63386733968778,-2.34915402890138,
85.4147410501868));
#246557=CARTESIAN_POINT('Ctrl Pts',(-4.71626747173541,-5.24367605763847,
85.5736954160115));
#246558=CARTESIAN_POINT('Ctrl Pts',(-1.62837798208691,-6.84653657870138,
85.7326497818363));
#246559=CARTESIAN_POINT('Ctrl Pts',(3.02788367824696,-6.80874461369026,
85.9445889362693));
#246560=CARTESIAN_POINT('Ctrl Pts',(7.62149261754915,-2.41970362147575,
86.2095128793105));
#246561=CARTESIAN_POINT('Ctrl Pts',(6.14884791532884,5.1214516107696,86.5274216109601));
#246562=CARTESIAN_POINT('Ctrl Pts',(0.221040988410256,7.44823431374593,
86.7923455540014));
#246563=CARTESIAN_POINT('Ctrl Pts',(-4.08404251290028,5.72254068163378,
87.0042847084344));
#246564=CARTESIAN_POINT('Ctrl Pts',(-7.12793149107813,2.19280380931291,
87.2162238628674));
#246565=CARTESIAN_POINT('Ctrl Pts',(-6.88228517983163,-2.86745042994337,
87.4281630173003));
#246566=CARTESIAN_POINT('Ctrl Pts',(-3.51186216222031,-6.09865105458944,
87.6401021717336));
#246567=CARTESIAN_POINT('Ctrl Pts',(-0.172784089409316,-7.05049382106299,
87.799056537558));
#246568=CARTESIAN_POINT('Ctrl Pts',(3.21534556183627,-6.26005039069349,
87.9580109033831));
#246569=CARTESIAN_POINT('Ctrl Pts',(6.72798520514021,-3.20332606252702,
88.1699500578158));
#246570=CARTESIAN_POINT('Ctrl Pts',(7.36336744207196,3.1181621587359,88.4348740008574));
#246571=CARTESIAN_POINT('Ctrl Pts',(1.34055440124988,7.88926556686919,88.7527827325067));
#246572=CARTESIAN_POINT('Ctrl Pts',(-4.67574563727826,5.80193556035346,
89.017706675548));
#246573=CARTESIAN_POINT('Ctrl Pts',(-6.82394637862079,1.69133997819441,
89.229645829981));
#246574=CARTESIAN_POINT('Ctrl Pts',(-6.8408692259793,-2.9695629511241,89.4415849844141));
#246575=CARTESIAN_POINT('Ctrl Pts',(-3.3635239224812,-6.65393327946781,
89.653524138847));
#246576=CARTESIAN_POINT('Ctrl Pts',(1.29816395574534,-6.91675435996419,
89.8654632932801));
#246577=CARTESIAN_POINT('Ctrl Pts',(4.45375014959483,-5.46840260655559,
90.0244176591047));
#246578=CARTESIAN_POINT('Ctrl Pts',(6.51357261739879,-2.66459185128115,
90.1833720249296));
#246579=CARTESIAN_POINT('Ctrl Pts',(7.19419559706401,1.94181165271923,90.3953111793625));
#246580=CARTESIAN_POINT('Ctrl Pts',(3.56594662779852,7.15724388174885,90.6602351224039));
#246581=CARTESIAN_POINT('Ctrl Pts',(-4.11209353127135,6.86500430279352,
90.9781438540534));
#246582=CARTESIAN_POINT('Ctrl Pts',(-7.32507601793611,1.36686313962944,
91.2430677970946));
#246583=CARTESIAN_POINT('Ctrl Pts',(-6.28383415832657,-3.1528246654039,
91.4550069515277));
#246584=CARTESIAN_POINT('Ctrl Pts',(-3.26565669436706,-6.70457174189187,
91.6669461059606));
#246585=CARTESIAN_POINT('Ctrl Pts',(1.77195762534478,-7.24211898816184,
91.8788852603937));
#246586=CARTESIAN_POINT('Ctrl Pts',(5.48421115874337,-4.41023224993819,
92.0908244148267));
#246587=CARTESIAN_POINT('Ctrl Pts',(6.93953308089106,-1.25785455503364,
92.2497787806513));
#246588=CARTESIAN_POINT('Ctrl Pts',(6.68096865860481,2.21163644362759,92.4087331464764));
#246589=CARTESIAN_POINT('Ctrl Pts',(4.20242493593684,6.15359305132114,92.6206723009091));
#246590=CARTESIAN_POINT('Ctrl Pts',(-1.94549150901639,7.75610586077085,
92.8855962439505));
#246591=CARTESIAN_POINT('Ctrl Pts',(-7.58821172844422,2.54099194245058,
93.2035049756));
#246592=CARTESIAN_POINT('Ctrl Pts',(-6.45351601683708,-3.72520932719855,
93.4684289186413));
#246593=CARTESIAN_POINT('Ctrl Pts',(-2.72331761807264,-6.48154427981681,
93.6803680730743));
#246594=CARTESIAN_POINT('Ctrl Pts',(1.87923500742207,-7.21694337476191,
93.8923072275072));
#246595=CARTESIAN_POINT('Ctrl Pts',(6.05572534184949,-4.34928866009077,
94.1042463819404));
#246596=CARTESIAN_POINT('Ctrl Pts',(7.03420294428734,0.216123739231432,
94.3161855363733));
#246597=CARTESIAN_POINT('Ctrl Pts',(6.08974171663501,3.557297188467,94.4751399021981));
#246598=CARTESIAN_POINT('Ctrl Pts',(3.63707266225326,6.02481372538034,94.6340942680227));
#246599=CARTESIAN_POINT('Ctrl Pts',(-0.809294392038973,7.4075721643778,
94.8460334224561));
#246600=CARTESIAN_POINT('Ctrl Pts',(-6.52180455974154,4.62689751557925,
95.110957365497));
#246601=CARTESIAN_POINT('Ctrl Pts',(-7.41696003839753,-3.00438031482576,
95.4288660971467));
#246602=CARTESIAN_POINT('Ctrl Pts',(-2.47999196559578,-7.02671284183443,
95.693790040188));
#246603=CARTESIAN_POINT('Ctrl Pts',(2.14619595981811,-6.69482770519087,
95.905729194621));
#246604=CARTESIAN_POINT('Ctrl Pts',(6.12084864813841,-4.26039994768352,
96.117668349054));
#246605=CARTESIAN_POINT('Ctrl Pts',(7.42873212447804,0.634082240296726,
96.329607503487));
#246606=CARTESIAN_POINT('Ctrl Pts',(5.20311616774883,4.73859712119429,96.54154665792));
#246607=CARTESIAN_POINT('Ctrl Pts',(2.3128390179733,6.66258907177538,96.7005010237446));
#246608=CARTESIAN_POINT('Ctrl Pts',(-1.15502828417975,6.94208813245597,
96.8594553895697));
#246609=CARTESIAN_POINT('Ctrl Pts',(-5.43201614047265,5.10100808008528,
97.0713945440023));
#246610=CARTESIAN_POINT('Ctrl Pts',(-7.96332980896591,-0.726287607476431,
97.336318487044));
#246611=CARTESIAN_POINT('Ctrl Pts',(-3.68065275068506,-7.10565919645552,
97.6542272186931));
#246612=CARTESIAN_POINT('Ctrl Pts',(2.68557157262411,-6.95073800681144,
97.9191511617346));
#246613=CARTESIAN_POINT('Ctrl Pts',(5.98411332030606,-3.69015756707848,
98.1310903161675));
#246614=CARTESIAN_POINT('Ctrl Pts',(7.42039901460989,0.743958568481396,
98.3430294706007));
#246615=CARTESIAN_POINT('Ctrl Pts',(5.23102490745951,5.31267349667283,98.5549686250335));
#246616=CARTESIAN_POINT('Ctrl Pts',(0.871085834401703,6.98340389789852,
98.7669077794666));
#246617=CARTESIAN_POINT('Ctrl Pts',(-2.57575899047016,6.56542329826589,
98.9258621452915));
#246618=CARTESIAN_POINT('Ctrl Pts',(-5.39195028551125,4.52256012614725,
99.0848165111161));
#246619=CARTESIAN_POINT('Ctrl Pts',(-7.44377066676299,0.342579982032306,
99.2967556655493));
#246620=CARTESIAN_POINT('Ctrl Pts',(-5.57717992383078,-5.73037341124973,
99.5616796085902));
#246621=CARTESIAN_POINT('Ctrl Pts',(1.82480680749437,-7.79151316514454,
99.8795883402401));
#246622=CARTESIAN_POINT('Ctrl Pts',(6.56028118708693,-3.53380308695505,
100.144512283282));
#246623=CARTESIAN_POINT('Ctrl Pts',(6.94569097029563,1.08823345164734,100.356451437714));
#246624=CARTESIAN_POINT('Ctrl Pts',(5.15324079602841,5.39072399458448,100.568390592148));
#246625=CARTESIAN_POINT('Ctrl Pts',(0.518959445105794,7.43766108121687,
100.780329746581));
#246626=CARTESIAN_POINT('Ctrl Pts',(-3.87964291634347,5.87154931630021,
100.992268901014));
#246627=CARTESIAN_POINT('Ctrl Pts',(-6.22628588087141,3.31250382521457,
101.151223266838));
#246628=CARTESIAN_POINT('Ctrl Pts',(-7.03716322434527,-0.0707935729022975,
101.310177632663));
#246629=CARTESIAN_POINT('Ctrl Pts',(-5.87758272796004,-4.58051351481871,
101.522116787096));
#246630=CARTESIAN_POINT('Ctrl Pts',(-0.510288009116391,-7.98008279925033,
101.787040730138));
#246631=CARTESIAN_POINT('Ctrl Pts',(6.45314990690399,-4.73227784120117,
102.104949461787));
#246632=CARTESIAN_POINT('Ctrl Pts',(7.28170872274559,1.58169895622098,102.369873404829));
#246633=CARTESIAN_POINT('Ctrl Pts',(4.56873445735095,5.34355130585872,102.58181255926));
#246634=CARTESIAN_POINT('Ctrl Pts',(0.409112248512814,7.44636979042522,
102.793751713695));
#246635=CARTESIAN_POINT('Ctrl Pts',(-4.44255043452387,5.98764285018941,
103.005690868127));
#246636=CARTESIAN_POINT('Ctrl Pts',(-6.76557225813255,1.93746033561121,
103.21763002256));
#246637=CARTESIAN_POINT('Ctrl Pts',(-6.88406975831953,-1.53261248363403,
103.376584388385));
#246638=CARTESIAN_POINT('Ctrl Pts',(-5.29987470506708,-4.63011944625967,
103.535538754209));
#246639=CARTESIAN_POINT('Ctrl Pts',(-1.48626035448566,-7.30192529009538,
103.747477908643));
#246640=CARTESIAN_POINT('Ctrl Pts',(4.80188028755272,-6.39406451634251,
104.012401851684));
#246641=CARTESIAN_POINT('Ctrl Pts',(7.97970493153861,0.60158664619224,104.330310583333));
#246642=CARTESIAN_POINT('Ctrl Pts',(4.50309091527155,5.93693740238345,104.595234526375));
#246643=CARTESIAN_POINT('Ctrl Pts',(-0.00424202430133235,7.03042367893717,
104.807173680808));
#246644=CARTESIAN_POINT('Ctrl Pts',(-4.53166127269599,5.92282381952964,
105.019112835241));
#246645=CARTESIAN_POINT('Ctrl Pts',(-7.26869229106604,1.65958839550948,
105.231051989674));
#246646=CARTESIAN_POINT('Ctrl Pts',(-6.39954377280644,-2.927893446151,105.442991144107));
#246647=CARTESIAN_POINT('Ctrl Pts',(-4.23293848730191,-5.64105922900283,
105.601945509932));
#246648=CARTESIAN_POINT('Ctrl Pts',(-1.0151344149273,-6.96391988004401,
105.760899875757));
#246649=CARTESIAN_POINT('Ctrl Pts',(3.61945184567181,-6.51357437359197,
105.97283903019));
#246650=CARTESIAN_POINT('Ctrl Pts',(7.80596412511259,-1.73465829851099,
106.237762973231));
#246651=CARTESIAN_POINT('Ctrl Pts',(5.67071391215704,5.64629090764611,106.555671704879));
#246652=CARTESIAN_POINT('Ctrl Pts',(-0.43999446263257,7.43851183933139,
106.820595647922));
#246653=CARTESIAN_POINT('Ctrl Pts',(-4.57517952335123,5.33803404159604,
107.032534802355));
#246654=CARTESIAN_POINT('Ctrl Pts',(-7.2942345200308,1.55239771142301,107.244473956788));
#246655=CARTESIAN_POINT('Ctrl Pts',(-6.60104531689834,-3.46616819975131,
107.456413111221));
#246656=CARTESIAN_POINT('Ctrl Pts',(-2.95749367867577,-6.38591823253887,
107.668352265654));
#246657=CARTESIAN_POINT('Ctrl Pts',(0.45280817473929,-7.03805954928553,
107.827306631479));
#246658=CARTESIAN_POINT('Ctrl Pts',(3.75754306370802,-5.9504241949983,107.986260997303));
#246659=CARTESIAN_POINT('Ctrl Pts',(6.98542876397639,-2.59439159859546,
108.198200151736));
#246660=CARTESIAN_POINT('Ctrl Pts',(7.05801263346198,3.75853335771147,108.463124094776));
#246661=CARTESIAN_POINT('Ctrl Pts',(0.636022569376616,7.977034071542,108.781032826427));
#246662=CARTESIAN_POINT('Ctrl Pts',(-5.17159094025551,5.36467153306593,
109.045956769468));
#246663=CARTESIAN_POINT('Ctrl Pts',(-6.94699915125064,1.07985086593164,
109.257895923901));
#246664=CARTESIAN_POINT('Ctrl Pts',(-6.5507417414334,-3.56420797999802,
109.469835078334));
#246665=CARTESIAN_POINT('Ctrl Pts',(-2.76052246964758,-6.92586723517592,
109.681774232767));
#246666=CARTESIAN_POINT('Ctrl Pts',(1.90611313675836,-6.77447069828759,
109.8937133872));
#246667=CARTESIAN_POINT('Ctrl Pts',(4.92090686380152,-5.05212758154333,
110.052667753025));
#246668=CARTESIAN_POINT('Ctrl Pts',(6.72410997097836,-2.07678190338583,
110.21162211885));
#246669=CARTESIAN_POINT('Ctrl Pts',(6.99377104650249,2.57181829306715,110.423561273283));
#246670=CARTESIAN_POINT('Ctrl Pts',(2.91753815165707,7.44513844523824,110.688485216324));
#246671=CARTESIAN_POINT('Ctrl Pts',(-4.70438106111458,6.47351497404037,
111.006393947974));
#246672=CARTESIAN_POINT('Ctrl Pts',(-7.41739686016381,0.712234041486918,
111.271317891015));
#246673=CARTESIAN_POINT('Ctrl Pts',(-5.97965582250344,-3.69737627846169,
111.483257045448));
#246674=CARTESIAN_POINT('Ctrl Pts',(-2.6585521391701,-6.96763205192077,
111.695196199881));
#246675=CARTESIAN_POINT('Ctrl Pts',(2.40688039744279,-7.05656063653657,
111.907135354314));
#246676=CARTESIAN_POINT('Ctrl Pts',(5.85352257849701,-3.90678818917865,
112.119074508747));
#246677=CARTESIAN_POINT('Ctrl Pts',(7.0237094653069,-0.637826629546366,
112.278028874572));
#246678=CARTESIAN_POINT('Ctrl Pts',(6.45864842356448,2.79509186196614,112.436983240397));
#246679=CARTESIAN_POINT('Ctrl Pts',(3.64046886970194,6.50185121270724,112.648922394829));
#246680=CARTESIAN_POINT('Ctrl Pts',(-2.62528792232601,7.55314362765783,
112.913846337871));
#246681=CARTESIAN_POINT('Ctrl Pts',(-7.78356446813755,1.85841907481702,
113.23175506952));
#246682=CARTESIAN_POINT('Ctrl Pts',(-6.09793721850281,-4.28254774523508,
113.496679012562));
#246683=CARTESIAN_POINT('Ctrl Pts',(-2.13811533592251,-6.6974127773659,
113.708618166994));
#246684=CARTESIAN_POINT('Ctrl Pts',(2.51150415461734,-7.02197570267657,
113.920557321428));
#246685=CARTESIAN_POINT('Ctrl Pts',(6.41738577696525,-3.79542896841933,
114.132496475861));
#246686=CARTESIAN_POINT('Ctrl Pts',(6.9873624005399,0.83874144740873,114.344435630294));
#246687=CARTESIAN_POINT('Ctrl Pts',(5.75047732804611,4.08305375448665,114.503389996118));
#246688=CARTESIAN_POINT('Ctrl Pts',(3.0887558698379,6.32346939208084,114.662344361943));
#246689=CARTESIAN_POINT('Ctrl Pts',(-1.46267068722058,7.30668715932174,
114.874283516376));
#246690=CARTESIAN_POINT('Ctrl Pts',(-6.90623617109233,4.03063484878436,
115.139207459416));
#246691=CARTESIAN_POINT('Ctrl Pts',(-7.12147922422141,-3.64994944434576,
115.457116191067));
#246692=CARTESIAN_POINT('Ctrl Pts',(-1.84742697086673,-7.21886882401493,
115.722040134108));
#246693=CARTESIAN_POINT('Ctrl Pts',(2.73113731404155,-6.47825316516581,
115.933979288542));
#246694=CARTESIAN_POINT('Ctrl Pts',(6.47437422943836,-3.70111796959026,
116.145918442974));
#246695=CARTESIAN_POINT('Ctrl Pts',(7.3432935628495,1.29002361006491,116.357857597407));
#246696=CARTESIAN_POINT('Ctrl Pts',(4.76263815994754,5.18111940506021,116.56979675184));
#246697=CARTESIAN_POINT('Ctrl Pts',(1.71320557327797,6.84136273896434,116.728751117665));
#246698=CARTESIAN_POINT('Ctrl Pts',(-1.76578623661401,6.81239142611651,
116.88770548349));
#246699=CARTESIAN_POINT('Ctrl Pts',(-5.86275908921941,4.59947156151941,
117.099644637923));
#246700=CARTESIAN_POINT('Ctrl Pts',(-7.86761470489579,-1.42924952000916,
117.364568580964));
#246701=CARTESIAN_POINT('Ctrl Pts',(-3.03636497104356,-7.4039236253434,
117.682477312614));
#246702=CARTESIAN_POINT('Ctrl Pts',(3.2910724029975,-6.68534935132399,117.947401255655));
#246703=CARTESIAN_POINT('Ctrl Pts',(6.28763429065526,-3.14523927978571,
118.159340410088));
#246704=CARTESIAN_POINT('Ctrl Pts',(7.32525449056893,1.39872890012328,118.371279564521));
#246705=CARTESIAN_POINT('Ctrl Pts',(4.73955447373246,5.75541003363227,118.583218718954));
#246706=CARTESIAN_POINT('Ctrl Pts',(0.248691684925148,7.03312682794283,
118.795157873387));
#246707=CARTESIAN_POINT('Ctrl Pts',(-3.14754009632173,6.31128424367394,
118.954112239212));
#246708=CARTESIAN_POINT('Ctrl Pts',(-5.77158086774825,4.02685140812069,
119.113066605036));
#246709=CARTESIAN_POINT('Ctrl Pts',(-7.44483822588827,-0.318538182646105,
119.32500575947));
#246710=CARTESIAN_POINT('Ctrl Pts',(-5.04732477901245,-6.2021470403648,
119.589929702511));
#246711=CARTESIAN_POINT('Ctrl Pts',(2.50821648709916,-7.5991083253986,119.90783843416));
#246712=CARTESIAN_POINT('Ctrl Pts',(6.84767622506058,-2.93843220574519,
120.172762377201));
#246713=CARTESIAN_POINT('Ctrl Pts',(6.82190036566931,1.69957362329846,120.384701531635));
#246714=CARTESIAN_POINT('Ctrl Pts',(4.65515858481535,5.82625904314762,120.596640686067));
#246715=CARTESIAN_POINT('Ctrl Pts',(-0.142311384242204,7.45438587239934,
120.8085798405));
#246716=CARTESIAN_POINT('Ctrl Pts',(-4.3847915920812,5.50457293766677,121.020518994933));
#246717=CARTESIAN_POINT('Ctrl Pts',(-6.4953808316654,2.74760719791489,121.179473360757));
#246718=CARTESIAN_POINT('Ctrl Pts',(-7.00319219825473,-0.694245641214978,
121.338427726583));
#246719=CARTESIAN_POINT('Ctrl Pts',(-5.44846176167561,-5.08343852279241,
121.550366881016));
#246720=CARTESIAN_POINT('Ctrl Pts',(0.199025603378755,-7.99390418658736,
121.815290824057));
#246721=CARTESIAN_POINT('Ctrl Pts',(6.84719198522617,-4.1416855511679,122.133199555707));
#246722=CARTESIAN_POINT('Ctrl Pts',(7.11285791045668,2.22087952322351,122.398123498748));
#246723=CARTESIAN_POINT('Ctrl Pts',(4.07713379665675,5.72746498062536,122.610062653181));
#246724=CARTESIAN_POINT('Ctrl Pts',(-0.252498138968556,7.45332412937059,
122.822001807614));
#246725=CARTESIAN_POINT('Ctrl Pts',(-4.9557734764722,5.570316913301,123.033940962047));
#246726=CARTESIAN_POINT('Ctrl Pts',(-6.91066936372984,1.3301764835109,123.245880116479));
#246727=CARTESIAN_POINT('Ctrl Pts',(-6.72113466442141,-2.13674197906841,
123.404834482305));
#246728=CARTESIAN_POINT('Ctrl Pts',(-4.86863067375534,-5.08164474738352,
123.56378884813));
#246729=CARTESIAN_POINT('Ctrl Pts',(-0.833213279604876,-7.40491987898185,
123.775728002563));
#246730=CARTESIAN_POINT('Ctrl Pts',(5.3497118136926,-5.94329023736657,124.040651945604));
#246731=CARTESIAN_POINT('Ctrl Pts',(7.89497810268386,1.30649073683698,124.358560677254));
#246732=CARTESIAN_POINT('Ctrl Pts',(3.95915453003105,6.31269743598997,124.623484620295));
#246733=CARTESIAN_POINT('Ctrl Pts',(-0.627358669347987,7.00237789612389,
124.835423774728));
#246734=CARTESIAN_POINT('Ctrl Pts',(-5.0387884405164,5.49785475793592,125.04736292916));
#246735=CARTESIAN_POINT('Ctrl Pts',(-7.38718040302859,1.00880471738742,
125.259302083594));
#246736=CARTESIAN_POINT('Ctrl Pts',(-6.11484655033592,-3.48358611174239,
125.471241238027));
#246737=CARTESIAN_POINT('Ctrl Pts',(-3.71629016119966,-5.9940391140007,
125.630195603852));
#246738=CARTESIAN_POINT('Ctrl Pts',(-0.393900273250039,-7.02648707041972,
125.789149969676));
#246739=CARTESIAN_POINT('Ctrl Pts',(4.18252969766674,-6.16713289232418,
126.001089124109));
#246740=CARTESIAN_POINT('Ctrl Pts',(7.92899141691023,-1.03595870849268,
126.266013067151));
#246741=CARTESIAN_POINT('Ctrl Pts',(5.14794319741676,6.12668573728643,126.5839217988));
#246742=CARTESIAN_POINT('Ctrl Pts',(-1.09756652154811,7.37023752953711,
126.848845741841));
#246743=CARTESIAN_POINT('Ctrl Pts',(-5.03030326070806,4.91150936122904,
127.060784896274));
#246744=CARTESIAN_POINT('Ctrl Pts',(-7.40312138455938,0.899772000631177,
127.272724050707));
#246745=CARTESIAN_POINT('Ctrl Pts',(-6.2678456900933,-4.03760221788769,
127.484663205141));
#246746=CARTESIAN_POINT('Ctrl Pts',(-2.3798454468764,-6.62291900758731,
127.696602359573));
#246747=CARTESIAN_POINT('Ctrl Pts',(1.07483618433314,-6.97022558022683,
127.855556725398));
#246748=CARTESIAN_POINT('Ctrl Pts',(4.27016327274933,-5.59395956368158,
128.014511091223));
#246749=CARTESIAN_POINT('Ctrl Pts',(7.18788690585305,-1.96503552439061,
128.226450245656));
#246750=CARTESIAN_POINT('Ctrl Pts',(6.69710106796964,4.36931946881163,128.491374188697));
#246751=CARTESIAN_POINT('Ctrl Pts',(-0.0735156790465368,8.00201179280775,
128.809282920347));
#246752=CARTESIAN_POINT('Ctrl Pts',(-5.6267283505892,4.88517978990507,129.074206863388));
#246753=CARTESIAN_POINT('Ctrl Pts',(-7.01536900349605,0.459861767179577,
129.28614601782));
#246754=CARTESIAN_POINT('Ctrl Pts',(-6.20905045483426,-4.13079754248224,
129.498085172254));
#246755=CARTESIAN_POINT('Ctrl Pts',(-2.13579171655767,-7.14328460920958,
129.710024326687));
#246756=CARTESIAN_POINT('Ctrl Pts',(2.49905845342029,-6.57886216442336,
129.92196348112));
#246757=CARTESIAN_POINT('Ctrl Pts',(5.34932893123977,-4.59608501311821,
130.080917846945));
#246758=CARTESIAN_POINT('Ctrl Pts',(6.88171886404708,-1.47262468137094,
130.23987221277));
#246759=CARTESIAN_POINT('Ctrl Pts',(6.73829541317992,3.18158100768473,130.451811367203));
#246760=CARTESIAN_POINT('Ctrl Pts',(2.24616443495528,7.67442901235677,130.716735310244));
#246761=CARTESIAN_POINT('Ctrl Pts',(-5.25963831503589,6.03106972952018,
131.034644041893));
#246762=CARTESIAN_POINT('Ctrl Pts',(-7.45133207249597,0.0519986323146828,
131.299567984935));
#246763=CARTESIAN_POINT('Ctrl Pts',(-5.62840895579532,-4.21282419810638,
131.511507139368));
#246764=CARTESIAN_POINT('Ctrl Pts',(-2.03052093785896,-7.17584703111325,
131.723446293801));
#246765=CARTESIAN_POINT('Ctrl Pts',(3.02285754397351,-6.81545695676022,
131.935385448233));
#246766=CARTESIAN_POINT('Ctrl Pts',(6.17675831757049,-3.37259206154052,
132.147324602667));
#246767=CARTESIAN_POINT('Ctrl Pts',(7.0525991099684,-0.0127780854508224,
132.306278968491));
#246768=CARTESIAN_POINT('Ctrl Pts',(6.18548929096036,3.35654586625373,132.465233334316));
#246769=CARTESIAN_POINT('Ctrl Pts',(3.04985706012767,6.79893041704212,132.677172488749));
#246770=CARTESIAN_POINT('Ctrl Pts',(-3.28441953996838,7.29072722915634,
132.942096431791));
#246771=CARTESIAN_POINT('Ctrl Pts',(-7.91764928647446,1.16121778534561,
133.26000516344));
#246772=CARTESIAN_POINT('Ctrl Pts',(-5.69435888292606,-4.80617636085127,
133.524929106481));
#246773=CARTESIAN_POINT('Ctrl Pts',(-1.53608294498999,-6.86056291225426,
133.736868260914));
#246774=CARTESIAN_POINT('Ctrl Pts',(3.12400400176437,-6.77173505910424,
133.948807415348));
#246775=CARTESIAN_POINT('Ctrl Pts',(6.7285323860292,-3.21169351765348,134.16074656978));
#246776=CARTESIAN_POINT('Ctrl Pts',(6.88552088334561,1.45475674032299,134.372685724214));
#246777=CARTESIAN_POINT('Ctrl Pts',(5.36594907368235,4.57667142967609,134.531640090038));
#246778=CARTESIAN_POINT('Ctrl Pts',(2.51612483089831,6.57234904851573,134.690594455863));
#246779=CARTESIAN_POINT('Ctrl Pts',(-2.10453089563916,7.14829049743629,
134.902533610296));
#246780=CARTESIAN_POINT('Ctrl Pts',(-7.23631142511329,3.4026400329894,135.167457553337));
#246781=CARTESIAN_POINT('Ctrl Pts',(-6.76993212346154,-4.26677906377091,
135.485366284987));
#246782=CARTESIAN_POINT('Ctrl Pts',(-1.20033675469971,-7.35421719897996,
135.750290228028));
#246783=CARTESIAN_POINT('Ctrl Pts',(3.29460290356249,-6.21066501528404,
135.962229382461));
#246784=CARTESIAN_POINT('Ctrl Pts',(6.77687988267027,-3.11275537092704,
136.174168536894));
#246785=CARTESIAN_POINT('Ctrl Pts',(7.20016907646936,1.93591743114999,136.386107691327));
#246786=CARTESIAN_POINT('Ctrl Pts',(4.28452746621314,5.58272681899942,136.59804684576));
#246787=CARTESIAN_POINT('Ctrl Pts',(1.10038604404414,6.96655961965286,136.757001211585));
#246788=CARTESIAN_POINT('Ctrl Pts',(-2.36319085294511,6.62857044855553,
136.91595557741));
#246789=CARTESIAN_POINT('Ctrl Pts',(-6.24617402102025,4.06281286418076,
137.127894731842));
#246790=CARTESIAN_POINT('Ctrl Pts',(-7.71241073412867,-2.12320047247547,
137.392818674884));
#246791=CARTESIAN_POINT('Ctrl Pts',(-2.36391126028145,-7.63999480400491,
137.710727406533));
#246792=CARTESIAN_POINT('Ctrl Pts',(3.86350032495916,-6.37391496262723,
137.975651349575));
#246793=CARTESIAN_POINT('Ctrl Pts',(6.55130607618235,-2.56670467838789,
138.187590504008));
#246794=CARTESIAN_POINT('Ctrl Pts',(6.99717060324046,0.871685760892387,
138.346544869832));
#246795=CARTESIAN_POINT('Ctrl Pts',(5.71527044315637,4.1246109195803,138.505564005226));
#246796=CARTESIAN_POINT('Ctrl Pts',(3.93551302891977,5.61075906984116,138.611598352013));
#246797=CARTESIAN_POINT('Ctrl Pts',(2.91932841735868,6.09728744058681,138.66464791019));
#246798=CARTESIAN_POINT('Ctrl Pts',(3.93307528793212,-5.51266228421277,
138.));
#246799=CARTESIAN_POINT('Ctrl Pts',(4.08486176364148,-5.42349325184365,
138.));
#246800=CARTESIAN_POINT('Ctrl Pts',(4.2326846053822,-5.3283456569208,138.));
#246801=CARTESIAN_POINT('Ctrl Pts',(4.37614884579843,-5.22732383700901,
138.));
#246802=CARTESIAN_POINT('Ctrl Pts',(4.52391818469271,-5.12327053774114,
138.));
#246803=CARTESIAN_POINT('Ctrl Pts',(4.66706455466681,-5.01298603196517,
138.));
#246804=CARTESIAN_POINT('Ctrl Pts',(4.80542684321419,-4.89696515575036,
138.));
#246805=CARTESIAN_POINT('Ctrl Pts',(4.94590248835348,-4.77917216745124,
138.));
#246806=CARTESIAN_POINT('Ctrl Pts',(5.08144724969525,-4.6554658264225,138.));
#246807=CARTESIAN_POINT('Ctrl Pts',(5.21187009830291,-4.52631398537958,
138.));
#246808=CARTESIAN_POINT('Ctrl Pts',(5.34430862911351,-4.39516610552716,
138.));
#246809=CARTESIAN_POINT('Ctrl Pts',(5.47146622839557,-4.25840263867453,
138.));
#246810=CARTESIAN_POINT('Ctrl Pts',(5.59311244077779,-4.11646896172721,
138.));
#246811=CARTESIAN_POINT('Ctrl Pts',(5.69160061880562,-4.0015554846071,138.));
#246812=CARTESIAN_POINT('Ctrl Pts',(5.78647562580018,-3.8832519703199,138.));
#246813=CARTESIAN_POINT('Ctrl Pts',(5.87759730129057,-3.76177727698624,
138.));
#246814=CARTESIAN_POINT('Ctrl Pts',(5.89385220890071,-3.74010779048387,
138.));
#246815=CARTESIAN_POINT('Ctrl Pts',(5.90998883697244,-3.71833560735108,
138.));
#246816=CARTESIAN_POINT('Ctrl Pts',(5.92599314981512,-3.69648023992614,
138.));
#246817=CARTESIAN_POINT('Ctrl Pts',(6.03816674779205,-3.54329683097485,
138.));
#246818=CARTESIAN_POINT('Ctrl Pts',(6.14398755043199,-3.38583986628415,
138.));
#246819=CARTESIAN_POINT('Ctrl Pts',(6.24327612830652,-3.22462877876666,
138.));
#246820=CARTESIAN_POINT('Ctrl Pts',(6.34256470618104,-3.06341769124917,
138.));
#246821=CARTESIAN_POINT('Ctrl Pts',(6.43532148595384,-2.89845187871061,
138.));
#246822=CARTESIAN_POINT('Ctrl Pts',(6.52133729465314,-2.73020783048089,
138.));
#246823=CARTESIAN_POINT('Ctrl Pts',(6.54540235632602,-2.68313737380591,
138.));
#246824=CARTESIAN_POINT('Ctrl Pts',(6.56893957507926,-2.63581008860474,
138.));
#246825=CARTESIAN_POINT('Ctrl Pts',(6.59194388268069,-2.58823590697392,
138.));
#246826=CARTESIAN_POINT('Ctrl Pts',(6.67513605841707,-2.4161898820591,138.));
#246827=CARTESIAN_POINT('Ctrl Pts',(6.75136213437869,-2.24091709476537,
138.));
#246828=CARTESIAN_POINT('Ctrl Pts',(6.82055045941942,-2.06283511800934,
138.));
#246829=CARTESIAN_POINT('Ctrl Pts',(6.88991117243377,-1.88430943646505,
138.));
#246830=CARTESIAN_POINT('Ctrl Pts',(6.95219929984553,-1.7029599431334,138.));
#246831=CARTESIAN_POINT('Ctrl Pts',(7.00729619903557,-1.51918376131994,
138.));
#246832=CARTESIAN_POINT('Ctrl Pts',(7.02222200681774,-1.46939860090232,
138.));
#246833=CARTESIAN_POINT('Ctrl Pts',(7.03661979311897,-1.41943524787105,
138.));
#246834=CARTESIAN_POINT('Ctrl Pts',(7.05048657229512,-1.36930139115022,
138.));
#246835=CARTESIAN_POINT('Ctrl Pts',(7.05874094265755,-1.33945859811108,
138.));
#246836=CARTESIAN_POINT('Ctrl Pts',(7.06680715224607,-1.30955538787954,
138.));
#246837=CARTESIAN_POINT('Ctrl Pts',(7.07468452464019,-1.27959337136282,
138.));
#246838=CARTESIAN_POINT('Ctrl Pts',(7.08043946017635,-1.25770415945831,
138.));
#246839=CARTESIAN_POINT('Ctrl Pts',(7.08609267172794,-1.23578700025731,
138.));
#246840=CARTESIAN_POINT('Ctrl Pts',(7.09164164408561,-1.21385215425006,
138.));
#246841=CARTESIAN_POINT('Ctrl Pts',(7.13960279074919,-1.02426383075656,
138.));
#246842=CARTESIAN_POINT('Ctrl Pts',(7.17983529772245,-0.833148244170129,
138.));
#246843=CARTESIAN_POINT('Ctrl Pts',(7.21231481660431,-0.640965875669055,
138.));
#246844=CARTESIAN_POINT('Ctrl Pts',(7.2449502246749,-0.447861105773331,
138.));
#246845=CARTESIAN_POINT('Ctrl Pts',(7.26975831462569,-0.253678666482718,
138.));
#246846=CARTESIAN_POINT('Ctrl Pts',(7.28666906892299,-0.0588585281659345,
138.));
#246847=CARTESIAN_POINT('Ctrl Pts',(7.30350913847585,0.135147287415994,
138.));
#246848=CARTESIAN_POINT('Ctrl Pts',(7.31251796317501,0.329786136287213,
138.));
#246849=CARTESIAN_POINT('Ctrl Pts',(7.31357807545766,0.524640804216316,
138.));
#246850=CARTESIAN_POINT('Ctrl Pts',(7.31428603059942,0.654766986429571,
138.));
#246851=CARTESIAN_POINT('Ctrl Pts',(7.31144808502855,0.784989760971824,
138.));
#246852=CARTESIAN_POINT('Ctrl Pts',(7.30501644905709,0.915186995230226,
138.));
#246853=CARTESIAN_POINT('Ctrl Pts',(7.29541239991929,1.10960419187653,138.));
#246854=CARTESIAN_POINT('Ctrl Pts',(7.27779751519746,1.30396484924485,138.));
#246855=CARTESIAN_POINT('Ctrl Pts',(7.25233008411155,1.49781397277794,138.));
#246856=CARTESIAN_POINT('Ctrl Pts',(7.25064901849204,1.51060965271297,138.));
#246857=CARTESIAN_POINT('Ctrl Pts',(7.24893371970543,1.52340310188329,138.));
#246858=CARTESIAN_POINT('Ctrl Pts',(7.24718422537979,1.53619418840126,138.));
#246859=CARTESIAN_POINT('Ctrl Pts',(7.24401930498186,1.55933388656357,138.));
#246860=CARTESIAN_POINT('Ctrl Pts',(7.24074365388209,1.58245715953455,138.));
#246861=CARTESIAN_POINT('Ctrl Pts',(7.23735822289073,1.60556014491937,138.));
#246862=CARTESIAN_POINT('Ctrl Pts',(7.20913527842305,1.79816022308357,138.));
#246863=CARTESIAN_POINT('Ctrl Pts',(7.17327751050791,1.9894185177033,138.));
#246864=CARTESIAN_POINT('Ctrl Pts',(7.13006388188138,2.17888639203352,138.));
#246865=CARTESIAN_POINT('Ctrl Pts',(7.08581849473728,2.37287795713814,138.));
#246866=CARTESIAN_POINT('Ctrl Pts',(7.03386183221965,2.56499323052619,138.));
#246867=CARTESIAN_POINT('Ctrl Pts',(6.97443939096877,2.75475966696422,138.));
#246868=CARTESIAN_POINT('Ctrl Pts',(6.91464739397427,2.94570628508201,138.));
#246869=CARTESIAN_POINT('Ctrl Pts',(6.84729634168636,3.13427548648786,138.));
#246870=CARTESIAN_POINT('Ctrl Pts',(6.77258332983085,3.31998438996726,138.));
#246871=CARTESIAN_POINT('Ctrl Pts',(6.6981710488299,3.50494578781337,138.));
#246872=CARTESIAN_POINT('Ctrl Pts',(6.61645574690026,3.68707059386329,138.));
#246873=CARTESIAN_POINT('Ctrl Pts',(6.52758237206456,3.86586940628296,138.));
#246874=CARTESIAN_POINT('Ctrl Pts',(6.47276241379817,3.97615826898282,138.));
#246875=CARTESIAN_POINT('Ctrl Pts',(6.41521797292606,4.0851813670272,138.));
#246876=CARTESIAN_POINT('Ctrl Pts',(6.35497407499007,4.19281964495557,138.));
#246877=CARTESIAN_POINT('Ctrl Pts',(6.33797951959163,4.22318395968162,138.));
#246878=CARTESIAN_POINT('Ctrl Pts',(6.32077010570966,4.25343804897414,138.));
#246879=CARTESIAN_POINT('Ctrl Pts',(6.30334629954177,4.28357918000919,138.));
#246880=CARTESIAN_POINT('Ctrl Pts',(6.29076653244945,4.30534069438027,138.));
#246881=CARTESIAN_POINT('Ctrl Pts',(6.27807965496324,4.32703527814749,138.));
#246882=CARTESIAN_POINT('Ctrl Pts',(6.26528698879689,4.34866051885305,138.));
#246883=CARTESIAN_POINT('Ctrl Pts',(6.24226933205953,4.3875704975042,138.));
#246884=CARTESIAN_POINT('Ctrl Pts',(6.21890827852989,4.42625757737068,138.));
#246885=CARTESIAN_POINT('Ctrl Pts',(6.19520638596214,4.46471642251,138.));
#246886=CARTESIAN_POINT('Ctrl Pts',(6.08983107847159,4.63569908225763,138.));
#246887=CARTESIAN_POINT('Ctrl Pts',(5.97772289519015,4.80217182705261,138.));
#246888=CARTESIAN_POINT('Ctrl Pts',(5.85928943886702,4.96389424887306,138.));
#246889=CARTESIAN_POINT('Ctrl Pts',(5.73914075688195,5.12795883359771,138.));
#246890=CARTESIAN_POINT('Ctrl Pts',(5.61248195284315,5.28713503441401,138.));
#246891=CARTESIAN_POINT('Ctrl Pts',(5.47968893077447,5.44115076767619,138.));
#246892=CARTESIAN_POINT('Ctrl Pts',(5.35498558079184,5.58578395388301,138.));
#246893=CARTESIAN_POINT('Ctrl Pts',(5.22487190446606,5.7258664220397,138.));
#246894=CARTESIAN_POINT('Ctrl Pts',(5.08962417547183,5.86114996981617,138.));
#246895=CARTESIAN_POINT('Ctrl Pts',(5.06750037681787,5.88327962769994,138.));
#246896=CARTESIAN_POINT('Ctrl Pts',(5.04523816074071,5.90528168859171,138.));
#246897=CARTESIAN_POINT('Ctrl Pts',(5.02285166040568,5.9271425397572,138.));
#246898=CARTESIAN_POINT('Ctrl Pts',(4.87519656581737,6.07133059944996,138.));
#246899=CARTESIAN_POINT('Ctrl Pts',(4.72201394798034,6.20950353456649,138.));
#246900=CARTESIAN_POINT('Ctrl Pts',(4.56370622067795,6.34139593385774,138.));
#246901=CARTESIAN_POINT('Ctrl Pts',(4.40476463903515,6.47381642215128,138.));
#246902=CARTESIAN_POINT('Ctrl Pts',(4.24065639042664,6.59990650300305,138.));
#246903=CARTESIAN_POINT('Ctrl Pts',(4.0717452682137,6.71936805595367,138.));
#246904=CARTESIAN_POINT('Ctrl Pts',(3.90357067072022,6.8383087054515,138.));
#246905=CARTESIAN_POINT('Ctrl Pts',(3.73063450900765,6.95067899177625,138.));
#246906=CARTESIAN_POINT('Ctrl Pts',(3.55325979428486,7.05614801072615,138.));
#246907=CARTESIAN_POINT('Ctrl Pts',(3.50933718657416,7.08226489188482,138.));
#246908=CARTESIAN_POINT('Ctrl Pts',(3.46514225877028,7.10795840003617,138.));
#246909=CARTESIAN_POINT('Ctrl Pts',(3.42067962509738,7.13322310757512,138.));
#246910=CARTESIAN_POINT('Ctrl Pts',(3.42490370648426,7.13754033682968,8.));
#246911=CARTESIAN_POINT('Ctrl Pts',(3.60303338065709,7.03788846583432,7.99999999999999));
#246912=CARTESIAN_POINT('Ctrl Pts',(3.77686286893927,6.93118228361841,7.99999999999999));
#246913=CARTESIAN_POINT('Ctrl Pts',(3.94592285660953,6.8174072015925,7.99999999999999));
#246914=CARTESIAN_POINT('Ctrl Pts',(4.11679905550406,6.70240983401064,7.99999999999999));
#246915=CARTESIAN_POINT('Ctrl Pts',(4.28280321834002,6.5801903541098,8.));
#246916=CARTESIAN_POINT('Ctrl Pts',(4.44364270499849,6.45121617950757,8.));
#246917=CARTESIAN_POINT('Ctrl Pts',(4.60504482065505,6.32179084324012,8.));
#246918=CARTESIAN_POINT('Ctrl Pts',(4.76124648814143,6.18556280407072,8.));
#246919=CARTESIAN_POINT('Ctrl Pts',(4.9119102565287,6.04297273661884,8.));
#246920=CARTESIAN_POINT('Ctrl Pts',(4.94377744841198,6.01281322920191,8.));
#246921=CARTESIAN_POINT('Ctrl Pts',(4.97539672828523,5.9823690099197,8.));
#246922=CARTESIAN_POINT('Ctrl Pts',(5.00676463700424,5.95164411183574,8.));
#246923=CARTESIAN_POINT('Ctrl Pts',(5.02880360356028,5.93005692196675,8.));
#246924=CARTESIAN_POINT('Ctrl Pts',(5.05071989143719,5.90832975933061,8.));
#246925=CARTESIAN_POINT('Ctrl Pts',(5.07250778250975,5.88646852196407,8.));
#246926=CARTESIAN_POINT('Ctrl Pts',(5.158239465655,5.80044823350066,8.));
#246927=CARTESIAN_POINT('Ctrl Pts',(5.24189935706624,5.71243742897355,8.));
#246928=CARTESIAN_POINT('Ctrl Pts',(5.32342886913692,5.62253662790359,8.));
#246929=CARTESIAN_POINT('Ctrl Pts',(5.46097401376483,5.47086861994824,8.));
#246930=CARTESIAN_POINT('Ctrl Pts',(5.59246025169705,5.3138206439058,8.));
#246931=CARTESIAN_POINT('Ctrl Pts',(5.71758256421037,5.15184052730674,8.));
#246932=CARTESIAN_POINT('Ctrl Pts',(5.84206463687843,4.99068924868794,8.));
#246933=CARTESIAN_POINT('Ctrl Pts',(5.96024808036236,4.82465548939151,8.));
#246934=CARTESIAN_POINT('Ctrl Pts',(6.07178603797319,4.65415854388629,8.));
#246935=CARTESIAN_POINT('Ctrl Pts',(6.11249389133456,4.59193251066087,8.));
#246936=CARTESIAN_POINT('Ctrl Pts',(6.15231607804158,4.5291118128463,8.));
#246937=CARTESIAN_POINT('Ctrl Pts',(6.19123404625067,4.46571638178551,8.));
#246938=CARTESIAN_POINT('Ctrl Pts',(6.22207638996413,4.41547574064682,8.));
#246939=CARTESIAN_POINT('Ctrl Pts',(6.25235065951106,4.36487441132344,8.));
#246940=CARTESIAN_POINT('Ctrl Pts',(6.28204768525483,4.31392140458892,8.));
#246941=CARTESIAN_POINT('Ctrl Pts',(6.30046683332831,4.28231854361794,8.));
#246942=CARTESIAN_POINT('Ctrl Pts',(6.31866374179757,4.25058040510658,8.));
#246943=CARTESIAN_POINT('Ctrl Pts',(6.33662197851953,4.21873508832127,8.));
#246944=CARTESIAN_POINT('Ctrl Pts',(6.3877624699296,4.12804772437101,8.));
#246945=CARTESIAN_POINT('Ctrl Pts',(6.43699714916998,4.03644132373437,8.));
#246946=CARTESIAN_POINT('Ctrl Pts',(6.48428962272374,3.94397632605379,8.));
#246947=CARTESIAN_POINT('Ctrl Pts',(6.57567872566177,3.76529476097158,8.));
#246948=CARTESIAN_POINT('Ctrl Pts',(6.65981818510592,3.58340802051667,8.));
#246949=CARTESIAN_POINT('Ctrl Pts',(6.73660877174782,3.39873683092503,8.));
#246950=CARTESIAN_POINT('Ctrl Pts',(6.81347023922936,3.21389518230254,8.));
#246951=CARTESIAN_POINT('Ctrl Pts',(6.88296940124662,3.02626327931723,8.));
#246952=CARTESIAN_POINT('Ctrl Pts',(6.94495644380309,2.83624949096006,8.));
#246953=CARTESIAN_POINT('Ctrl Pts',(7.0065419660172,2.64746651469209,8.));
#246954=CARTESIAN_POINT('Ctrl Pts',(7.06071245336442,2.45633176848018,8.));
#246955=CARTESIAN_POINT('Ctrl Pts',(7.10726979491501,2.26324214781201,8.));
#246956=CARTESIAN_POINT('Ctrl Pts',(7.14496638496124,2.10690117064093,8.));
#246957=CARTESIAN_POINT('Ctrl Pts',(7.17767099659649,1.94927840699215,8.));
#246958=CARTESIAN_POINT('Ctrl Pts',(7.20525302507637,1.79058709511881,8.));
#246959=CARTESIAN_POINT('Ctrl Pts',(7.21612231004232,1.72805140846221,8.));
#246960=CARTESIAN_POINT('Ctrl Pts',(7.22619584448681,1.66534982996421,8.));
#246961=CARTESIAN_POINT('Ctrl Pts',(7.23546463629665,1.60249563050015,8.));
#246962=CARTESIAN_POINT('Ctrl Pts',(7.2414327693778,1.56202409604274,8.));
#246963=CARTESIAN_POINT('Ctrl Pts',(7.24706820793831,1.52148084492807,8.));
#246964=CARTESIAN_POINT('Ctrl Pts',(7.25236235321427,1.48091914014147,8.));
#246965=CARTESIAN_POINT('Ctrl Pts',(7.27761224616607,1.28746417235747,8.));
#246966=CARTESIAN_POINT('Ctrl Pts',(7.29513326182066,1.09340516848697,8.00000000000001));
#246967=CARTESIAN_POINT('Ctrl Pts',(7.30480364597534,0.899123198458447,
8.));
#246968=CARTESIAN_POINT('Ctrl Pts',(7.31392911010541,0.715788894437285,
8.));
#246969=CARTESIAN_POINT('Ctrl Pts',(7.31606343307754,0.532255537961043,
8.));
#246970=CARTESIAN_POINT('Ctrl Pts',(7.31106172364628,0.348843391340116,
8.));
#246971=CARTESIAN_POINT('Ctrl Pts',(7.30573789570327,0.153619193556052,
8.));
#246972=CARTESIAN_POINT('Ctrl Pts',(7.29232950872236,-0.0414684692841456,
8.00000000000001));
#246973=CARTESIAN_POINT('Ctrl Pts',(7.27096643466698,-0.235911858864235,
8.00000000000001));
#246974=CARTESIAN_POINT('Ctrl Pts',(7.24977413424447,-0.428800893301357,
8.00000000000001));
#246975=CARTESIAN_POINT('Ctrl Pts',(7.22075348912854,-0.62105660412465,
8.00000000000001));
#246976=CARTESIAN_POINT('Ctrl Pts',(7.18398479930742,-0.81216290480137,
8.00000000000001));
#246977=CARTESIAN_POINT('Ctrl Pts',(7.15738132160842,-0.950435229241711,
8.00000000000001));
#246978=CARTESIAN_POINT('Ctrl Pts',(7.12672073322938,-1.08810544329263,
8.));
#246979=CARTESIAN_POINT('Ctrl Pts',(7.0920194960254,-1.22496823775203,8.));
#246980=CARTESIAN_POINT('Ctrl Pts',(7.08350694221174,-1.25854202349559,
8.));
#246981=CARTESIAN_POINT('Ctrl Pts',(7.07475002512292,-1.29207103794083,
8.));
#246982=CARTESIAN_POINT('Ctrl Pts',(7.06575857857453,-1.32551742518055,
8.));
#246983=CARTESIAN_POINT('Ctrl Pts',(7.01585043134197,-1.51116577550707,
8.));
#246984=CARTESIAN_POINT('Ctrl Pts',(6.95866555411597,-1.69449496168078,
8.));
#246985=CARTESIAN_POINT('Ctrl Pts',(6.89436543997893,-1.87503604479795,
8.));
#246986=CARTESIAN_POINT('Ctrl Pts',(6.83023212431252,-2.0551087931858,8.));
#246987=CARTESIAN_POINT('Ctrl Pts',(6.75902012696239,-2.23240857725891,
8.));
#246988=CARTESIAN_POINT('Ctrl Pts',(6.68084233139359,-2.40644947611183,
8.));
#246989=CARTESIAN_POINT('Ctrl Pts',(6.6038005184819,-2.57796142871745,8.));
#246990=CARTESIAN_POINT('Ctrl Pts',(6.51999351024779,-2.7463090970057,8.00000000000001));
#246991=CARTESIAN_POINT('Ctrl Pts',(6.42948842321972,-2.91099803412343,
8.00000000000001));
#246992=CARTESIAN_POINT('Ctrl Pts',(6.39882586075824,-2.96679362514386,
8.));
#246993=CARTESIAN_POINT('Ctrl Pts',(6.36739415792422,-3.02216897199648,
8.));
#246994=CARTESIAN_POINT('Ctrl Pts',(6.33519494702265,-3.07710388684608,
8.));
#246995=CARTESIAN_POINT('Ctrl Pts',(6.26232290414108,-3.20143051965874,
8.00000000000001));
#246996=CARTESIAN_POINT('Ctrl Pts',(6.18552036272165,-3.32350222199875,
8.));
#246997=CARTESIAN_POINT('Ctrl Pts',(6.10490764005655,-3.44316034524444,
8.));
#246998=CARTESIAN_POINT('Ctrl Pts',(6.06827231631093,-3.49754027361023,
8.));
#246999=CARTESIAN_POINT('Ctrl Pts',(6.03084992728334,-3.5514215248963,8.00000000000001));
#247000=CARTESIAN_POINT('Ctrl Pts',(5.99265116460685,-3.6047882158074,8.));
#247001=CARTESIAN_POINT('Ctrl Pts',(5.96951316952572,-3.63711382389726,
8.));
#247002=CARTESIAN_POINT('Ctrl Pts',(5.9460907821855,-3.66924999344316,8.00000000000001));
#247003=CARTESIAN_POINT('Ctrl Pts',(5.92238485722257,-3.70119504522787,
8.));
#247004=CARTESIAN_POINT('Ctrl Pts',(5.90199196396135,-3.72867560261125,
8.));
#247005=CARTESIAN_POINT('Ctrl Pts',(5.88138869951439,-3.75601516977367,
8.));
#247006=CARTESIAN_POINT('Ctrl Pts',(5.86059722504908,-3.78318498211917,
8.));
#247007=CARTESIAN_POINT('Ctrl Pts',(5.74709140037064,-3.93151173796224,
8.));
#247008=CARTESIAN_POINT('Ctrl Pts',(5.62785777030339,-4.07494918288655,
8.00000000000001));
#247009=CARTESIAN_POINT('Ctrl Pts',(5.503232290236,-4.21322289775717,8.));
#247010=CARTESIAN_POINT('Ctrl Pts',(5.37820579271597,-4.35194154710566,
8.));
#247011=CARTESIAN_POINT('Ctrl Pts',(5.24775214698824,-4.48546363618437,
8.));
#247012=CARTESIAN_POINT('Ctrl Pts',(5.1121747072249,-4.61347432725512,8.));
#247013=CARTESIAN_POINT('Ctrl Pts',(4.97745627898038,-4.74067394932832,
8.));
#247014=CARTESIAN_POINT('Ctrl Pts',(4.83767821573056,-4.86243216978443,
8.));
#247015=CARTESIAN_POINT('Ctrl Pts',(4.69311114269838,-4.97839674800658,
8.));
#247016=CARTESIAN_POINT('Ctrl Pts',(4.55125768635081,-5.09218459671703,
8.));
#247017=CARTESIAN_POINT('Ctrl Pts',(4.40479277614842,-5.2003945083745,8.));
#247018=CARTESIAN_POINT('Ctrl Pts',(4.25395421979913,-5.30264739511277,
8.));
#247019=CARTESIAN_POINT('Ctrl Pts',(4.14773939891244,-5.37465002038917,
8.));
#247020=CARTESIAN_POINT('Ctrl Pts',(4.03935555221588,-5.443697940156,8.));
#247021=CARTESIAN_POINT('Ctrl Pts',(3.92888236737293,-5.50964357679762,
8.));
#247022=CARTESIAN_POINT('Origin',(0.,0.,138.));
#247023=CARTESIAN_POINT('Origin',(0.,0.,4.));
#247024=CARTESIAN_POINT('',(-10.,-1.22464679914735E-15,4.));
#247025=CARTESIAN_POINT('Origin',(0.,0.,4.));
#247026=CARTESIAN_POINT('',(-6.,7.34788079488412E-16,4.));
#247027=CARTESIAN_POINT('Origin',(0.,0.,4.));
#247028=CARTESIAN_POINT('Origin',(0.,0.,4.));
#247029=CARTESIAN_POINT('',(-10.,-1.22464679914735E-15,8.));
#247030=CARTESIAN_POINT('Origin',(0.,0.,8.));
#247031=CARTESIAN_POINT('',(-10.,-1.22464679914735E-15,4.));
#247032=CARTESIAN_POINT('Origin',(0.,0.,-36.));
#247033=CARTESIAN_POINT('',(-6.,-7.34788079488412E-16,-36.));
#247034=CARTESIAN_POINT('',(-6.,-7.34788079488412E-16,-36.));
#247035=CARTESIAN_POINT('',(-6.,-7.34788079488412E-16,-36.));
#247036=CARTESIAN_POINT('Origin',(0.,0.,-36.));
#247037=CARTESIAN_POINT('Origin',(0.,0.,8.));
#247038=CARTESIAN_POINT('Origin',(0.,0.,-36.));
#289359=UNCERTAINTY_MEASURE_WITH_UNIT(LENGTH_MEASURE(0.01),#289388,
'DISTANCE_ACCURACY_VALUE',
'Maximum model space distance between geometric entities at asserted c
onnectivities');
#289368=UNCERTAINTY_MEASURE_WITH_UNIT(LENGTH_MEASURE(0.01),#289388,
'DISTANCE_ACCURACY_VALUE',
'Maximum model space distance between geometric entities at asserted c
onnectivities');
#289378=(
GEOMETRIC_REPRESENTATION_CONTEXT(3)
GLOBAL_UNCERTAINTY_ASSIGNED_CONTEXT((#289359))
GLOBAL_UNIT_ASSIGNED_CONTEXT((#289388,#289390,#289391))
REPRESENTATION_CONTEXT('','3D')
);
#289387=(
GEOMETRIC_REPRESENTATION_CONTEXT(3)
GLOBAL_UNCERTAINTY_ASSIGNED_CONTEXT((#289368))
GLOBAL_UNIT_ASSIGNED_CONTEXT((#289388,#289390,#289391))
REPRESENTATION_CONTEXT('','3D')
);
#289388=(
LENGTH_UNIT()
NAMED_UNIT(*)
SI_UNIT(.MILLI.,.METRE.)
);
#289390=(
NAMED_UNIT(*)
PLANE_ANGLE_UNIT()
SI_UNIT($,.RADIAN.)
);
#289391=(
NAMED_UNIT(*)
SI_UNIT($,.STERADIAN.)
SOLID_ANGLE_UNIT()
);
#289401=SHAPE_DEFINITION_REPRESENTATION(#289419,#289462);
#289419=PRODUCT_DEFINITION_SHAPE('',$,#289481);
#289462=SHAPE_REPRESENTATION('',(#17584),#289378);
#289471=PRODUCT_DEFINITION_CONTEXT('part definition',#289527,'design');
#289481=PRODUCT_DEFINITION('Feed spindle','Feed spindle',#289499,#289471);
#289499=PRODUCT_DEFINITION_FORMATION('',$,#289538);
#289527=APPLICATION_CONTEXT(
'Core Data for Automotive Mechanical Design Process');
#289528=PRODUCT_CONTEXT('part definition',#289527,'mechanical');
#289538=PRODUCT('Feed spindle','Feed spindle',$,(#289528));
#289548=PRESENTATION_STYLE_ASSIGNMENT((#289555));
#289555=SURFACE_STYLE_USAGE(.BOTH.,#289562);
#289562=SURFACE_SIDE_STYLE('',(#289569));
#289569=SURFACE_STYLE_FILL_AREA(#289576);
#289576=FILL_AREA_STYLE('Opaque(104,114,127)',(#289583));
#289583=FILL_AREA_STYLE_COLOUR('Opaque(104,114,127)',#289590);
#289590=COLOUR_RGB('Opaque(104,114,127)',0.407843137254902,0.447058823529412,
0.498039215686275);
ENDSEC;
END-ISO-10303-21;
